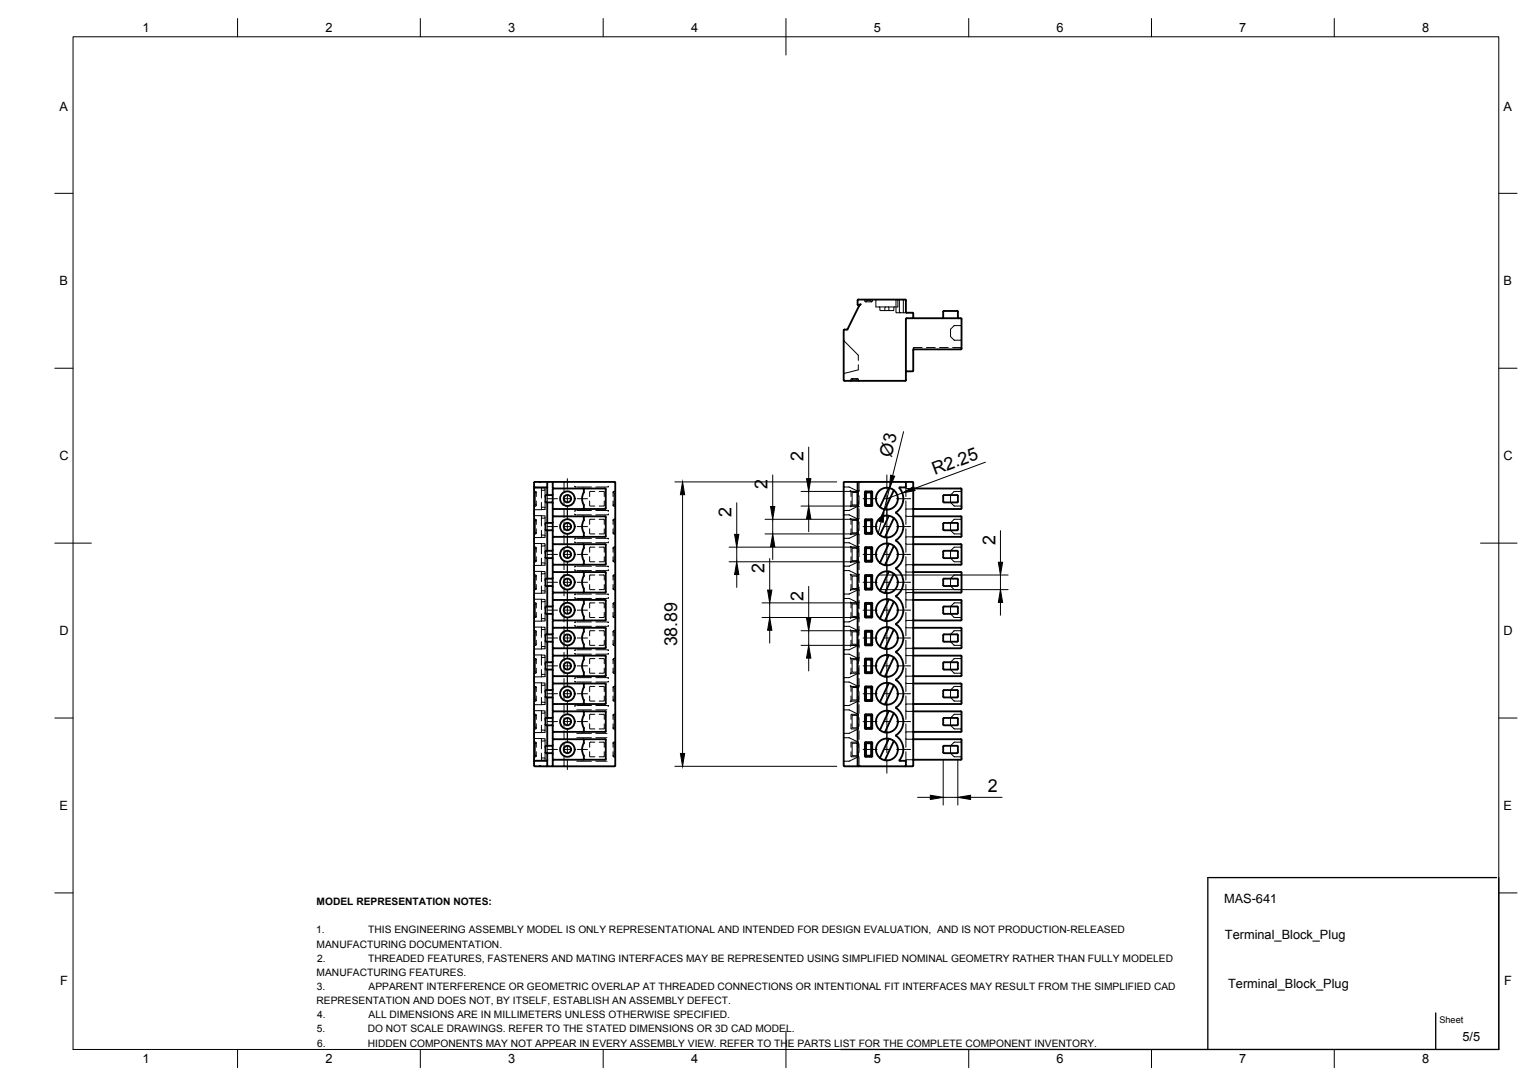
ISO-10303-21;
HEADER;
FILE_DESCRIPTION((''),'2;1');
FILE_NAME('Terminal_Block_Plug.step','2026-10-09T09:55:32-07:00',(''),(''),'','','');
FILE_SCHEMA (('AUTOMOTIVE_DESIGN { 1 0 10303 214 3 1 1 }'));
ENDSEC;
DATA;
#10=MECHANICAL_DESIGN_GEOMETRIC_PRESENTATION_REPRESENTATION('',(#83011,#83012,#83013,#83014,#83015,#83016,#83017,#83018,#83019,#83020,#83021,#83022,#83023,#83024,#83025,#83026,#83027,#83028,#83029,#83030,#83031,#83032,#83033,#83034,#83035,#83036,#83037,#83038,#83039,#83040,#83041,#83042,#83043,#83044,#83045,#83046,#83047,#83048,#83049,#83050,#83051,#83052,#83053,#83054,#83055,#83056,#83057,#83058,#83059,#83060,#83061,#83062,#83063,#83064,#83065,#83066,#83067,#83068,#83069,#83070,#83071,#83072,#83073,#83074,#83075,#83076,#83077,#83078,#83079,#83080,#83081,#83082,#83083,#83084,#83085,#83086,#83087,#83088,#83089,#83090,#83091,#83092,#83093,#83094,#83095,#83096,#83097,#83098,#83099,#83100,#83101,#83102,#83103,#83104,#83105,#83106,#83107,#83108,#83109,#83110,#83111,#83112,#83113,#83114,#83115,#83116,#83117,#83118,#83119,#83120,#83121,#83122,#83123,#83124,#83125,#83126,#83127,#83128,#83129,#83130,#83131,#83132,#83133,#83134,#83135,#83136,#83137,#83138,#83139,#83140,#83141,#83142,#83143,#83144,#83145,#83146,#83147,#83148,#83149,#83150,#83151,#83152,#83153,#83154,#83155,#83156,#83157,#83158,#83159,#83160,#83161,#83162,#83163,#83164,#83165,#83166,#83167,#83168,#83169,#83170,#83171,#83172,#83173,#83174,#83175,#83176,#83177,#83178,#83179,#83180,#83181,#83182,#83183,#83184,#83185,#83186,#83187,#83188,#83189,#83190,#83191,#83192,#83193,#83194,#83195,#83196,#83197,#83198,#83199,#83200,#83201,#83202,#83203,#83204,#83205,#83206,#83207,#83208,#83209,#83210,#83211,#83212,#83213,#83214,#83215,#83216,#83217,#83218,#83219,#83220,#83221,#83222,#83223,#83224,#83225,#83226,#83227,#83228,#83229,#83230,#83231,#83232,#83233,#83234,#83235,#83236,#83237,#83238,#83239,#83240,#83241,#83242,#83243,#83244,#83245,#83246,#83247,#83248,#83249,#83250,#83251,#83252,#83253,#83254,#83255,#83256,#83257,#83258,#83259,#83260,#83261,#83262,#83263,#83264,#83265,#83266,#83267,#83268,#83269,#83270,#83271,#83272,#83273,#83274,#83275,#83276,#83277,#83278,#83279,#83280,#83281,#83282,#83283,#83284,#83285,#83286,#83287,#83288,#83289,#83290,#83291,#83292,#83293,#83294,#83295,#83296,#83297,#83298,#83299,#83300,#83301,#83302,#83303,#83304,#83305,#83306,#83307,#83308,#83309,#83310,#83311,#83312,#83313,#83314,#83315,#83316,#83317,#83318,#83319,#83320,#83321,#83322,#83323,#83324,#83325,#83326,#83327,#83328,#83329,#83330,#83331,#83332,#83333,#83334,#83335,#83336,#83337,#83338,#83339,#83340,#83341,#83342,#83343,#83344,#83345,#83346,#83347,#83348,#83349,#83350,#83351,#83352,#83353,#83354,#83355,#83356,#83357,#83358,#83359,#83360,#83361,#83362,#83363,#83364,#83365,#83366,#83367,#83368,#83369,#83370,#83371,#83372,#83373,#83374,#83375,#83376,#83377,#83378,#83379,#83380,#83381,#83382,#83383,#83384,#83385,#83386,#83387,#83388,#83389,#83390,#83391,#83392,#83393,#83394,#83395,#83396,#83397,#83398,#83399,#83400,#83401,#83402,#83403,#83404,#83405,#83406,#83407,#83408,#83409,#83410,#83411,#83412,#83413,#83414,#83415,#83416,#83417,#83418,#83419,#83420,#83421,#83422,#83423,#83424,#83425,#83426,#83427,#83428,#83429,#83430,#83431,#83432,#83433,#83434,#83435,#83436,#83437,#83438,#83439,#83440,#83441,#83442,#83443,#83444,#83445,#83446,#83447,#83448,#83449,#83450,#83451,#83452,#83453,#83454,#83455,#83456,#83457,#83458,#83459,#83460,#83461,#83462,#83463,#83464,#83465,#83466,#83467,#83468,#83469,#83470,#83471,#83472,#83473,#83474,#83475,#83476,#83477,#83478,#83479,#83480,#83481,#83482,#83483,#83484,#83485,#83486,#83487,#83488,#83489,#83490,#83491,#83492,#83493,#83494,#83495,#83496,#83497,#83498,#83499,#83500,#83501,#83502,#83503,#83504,#83505,#83506,#83507,#83508,#83509,#83510,#83511,#83512,#83513,#83514,#83515,#83516,#83517,#83518,#83519,#83520,#83521,#83522,#83523,#83524,#83525,#83526,#83527,#83528,#83529,#83530,#83531,#83532,#83533,#83534,#83535,#83536,#83537,#83538,#83539,#83540,#83541,#83542,#83543,#83544,#83545,#83546,#83547,#83548,#83549,#83550,#83551,#83552,#83553,#83554,#83555,#83556,#83557,#83558,#83559,#83560,#83561,#83562,#83563,#83564,#83565,#83566,#83567,#83568,#83569,#83570,#83571,#83572,#83573,#83574,#83575,#83576,#83577,#83578,#83579,#83580,#83581,#83582,#83583,#83584,#83585,#83586,#83587,#83588,#83589,#83590,#83591,#83592,#83593,#83594,#83595,#83596,#83597,#83598,#83599,#83600,#83601,#83602,#83603,#83604,#83605,#83606,#83607,#83608,#83609,#83610,#83611,#83612,#83613,#83614,#83615,#83616,#83617,#83618,#83619,#83620,#83621,#83622,#83623,#83624,#83625,#83626,#83627,#83628,#83629,#83630,#83631,#83632,#83633,#83634,#83635,#83636,#83637,#83638,#83639,#83640,#83641,#83642,#83643,#83644,#83645,#83646,#83647,#83648,#83649,#83650,#83651,#83652,#83653,#83654,#83655,#83656,#83657,#83658,#83659,#83660,#83661,#83662,#83663,#83664,#83665,#83666,#83667,#83668,#83669,#83670,#83671,#83672,#83673,#83674,#83675,#83676,#83677,#83678,#83679,#83680,#83681,#83682,#83683,#83684,#83685,#83686,#83687,#83688,#83689,#83690,#83691,#83692,#83693,#83694,#83695,#83696,#83697,#83698,#83699,#83700,#83701,#83702,#83703,#83704,#83705,#83706,#83707,#83708,#83709,#83710,#83711,#83712,#83713,#83714,#83715,#83716,#83717,#83718,#83719,#83720,#83721,#83722,#83723,#83724,#83725,#83726,#83727,#83728,#83729,#83730,#83731,#83732,#83733,#83734,#83735,#83736,#83737,#83738,#83739,#83740,#83741,#83742,#83743,#83744,#83745,#83746,#83747,#83748,#83749,#83750,#83751,#83752,#83753,#83754,#83755,#83756,#83757,#83758,#83759,#83760,#83761,#83762,#83763,#83764,#83765,#83766,#83767,#83768,#83769,#83770,#83771,#83772,#83773,#83774,#83775,#83776,#83777,#83778,#83779,#83780,#83781,#83782,#83783,#83784,#83785,#83786,#83787,#83788,#83789,#83790,#83791,#83792,#83793,#83794,#83795,#83796,#83797,#83798,#83799,#83800,#83801,#83802,#83803,#83804,#83805,#83806,#83807,#83808,#83809,#83810,#83811,#83812,#83813,#83814,#83815,#83816,#83817,#83818,#83819,#83820,#83821,#83822,#83823,#83824,#83825,#83826,#83827,#83828,#83829,#83830,#83831,#83832,#83833,#83834,#83835,#83836,#83837,#83838,#83839,#83840,#83841,#83842,#83843,#83844,#83845,#83846,#83847,#83848,#83849,#83850,#83851,#83852,#83853,#83854,#83855,#83856,#83857,#83858,#83859,#83860,#83861,#83862,#83863,#83864,#83865,#83866,#83867,#83868,#83869,#83870,#83871,#83872,#83873,#83874,#83875,#83876,#83877,#83878,#83879,#83880,#83881,#83882,#83883,#83884,#83885,#83886,#83887,#83888,#83889,#83890,#83891,#83892,#83893,#83894,#83895,#83896,#83897,#83898,#83899,#83900,#83901,#83902,#83903,#83904,#83905,#83906,#83907,#83908,#83909,#83910,#83911,#83912,#83913,#83914,#83915,#83916,#83917,#83918,#83919,#83920,#83921,#83922,#83923,#83924,#83925,#83926,#83927,#83928,#83929,#83930,#83931,#83932,#83933,#83934,#83935,#83936,#83937,#83938,#83939,#83940,#83941,#83942,#83943,#83944,#83945,#83946,#83947,#83948,#83949,#83950,#83951,#83952,#83953,#83954,#83955,#83956,#83957,#83958,#83959,#83960,#83961,#83962,#83963,#83964,#83965,#83966,#83967,#83968,#83969,#83970,#83971,#83972,#83973,#83974,#83975,#83976,#83977,#83978,#83979,#83980,#83981,#83982,#83983,#83984,#83985,#83986,#83987,#83988,#83989,#83990,#83991,#83992,#83993,#83994,#83995,#83996,#83997,#83998,#83999,#84000,#84001,#84002,#84003,#84004,#84005,#84006,#84007,#84008,#84009,#84010,#84011,#84012,#84013,#84014,#84015,#84016,#84017,#84018,#84019,#84020,#84021,#84022,#84023,#84024,#84025,#84026,#84027,#84028,#84029,#84030,#84031,#84032,#84033,#84034,#84035,#84036,#84037,#84038,#84039,#84040,#84041,#84042,#84043,#84044,#84045,#84046,#84047,#84048,#84049,#84050,#84051,#84052,#84053,#84054,#84055,#84056,#84057,#84058,#84059,#84060,#84061,#84062,#84063,#84064,#84065,#84066,#84067,#84068,#84069,#84070,#84071,#84072,#84073,#84074,#84075,#84076,#84077,#84078,#84079,#84080,#84081,#84082,#84083,#84084,#84085,#84086,#84087,#84088,#84089,#84090,#84091,#84092,#84093,#84094,#84095,#84096,#84097,#84098,#84099,#84100,#84101,#84102,#84103,#84104,#84105,#84106,#84107,#84108,#84109,#84110,#84111,#84112,#84113,#84114,#84115,#84116,#84117,#84118,#84119,#84120,#84121,#84122,#84123,#84124,#84125,#84126,#84127,#84128,#84129,#84130,#84131,#84132,#84133,#84134,#84135,#84136,#84137,#84138,#84139,#84140,#84141,#84142,#84143,#84144,#84145,#84146,#84147,#84148,#84149,#84150,#84151,#84152,#84153,#84154,#84155,#84156,#84157,#84158,#84159,#84160,#84161,#84162,#84163,#84164,#84165,#84166,#84167,#84168,#84169,#84170,#84171,#84172,#84173,#84174,#84175,#84176,#84177,#84178,#84179,#84180,#84181,#84182,#84183,#84184,#84185,#84186,#84187,#84188,#84189,#84190,#84191,#84192,#84193,#84194,#84195,#84196,#84197,#84198,#84199,#84200,#84201,#84202,#84203,#84204,#84205,#84206,#84207,#84208,#84209,#84210,#84211,#84212,#84213,#84214,#84215,#84216,#84217,#84218,#84219,#84220,#84221,#84222,#84223,#84224,#84225,#84226,#84227,#84228,#84229,#84230,#84231,#84232,#84233,#84234,#84235,#84236,#84237,#84238,#84239,#84240,#84241,#84242,#84243,#84244,#84245,#84246,#84247,#84248,#84249,#84250,#84251,#84252,#84253,#84254,#84255,#84256,#84257,#84258,#84259,#84260,#84261,#84262,#84263,#84264,#84265,#84266,#84267,#84268,#84269,#84270,#84271,#84272,#84273,#84274,#84275,#84276,#84277,#84278,#84279,#84280,#84281,#84282,#84283,#84284,#84285,#84286,#84287,#84288,#84289,#84290,#84291,#84292,#84293,#84294,#84295,#84296,#84297,#84298,#84299,#84300,#84301,#84302,#84303,#84304,#84305,#84306,#84307,#84308,#84309,#84310,#84311,#84312,#84313,#84314,#84315,#84316,#84317,#84318,#84319,#84320,#84321,#84322,#84323,#84324,#84325,#84326,#84327,#84328,#84329,#84330,#84331,#84332,#84333,#84334,#84335,#84336,#84337,#84338,#84339,#84340,#84341,#84342,#84343,#84344,#84345,#84346,#84347,#84348,#84349,#84350,#84351,#84352,#84353,#84354,#84355,#84356,#84357,#84358,#84359,#84360,#84361,#84362,#84363,#84364,#84365,#84366,#84367,#84368,#84369,#84370,#84371,#84372,#84373,#84374,#84375,#84376,#84377,#84378,#84379,#84380,#84381,#84382,#84383,#84384,#84385,#84386,#84387,#84388,#84389,#84390,#84391,#84392,#84393,#84394,#84395,#84396,#84397,#84398,#84399,#84400,#84401,#84402,#84403,#84404,#84405,#84406,#84407,#84408,#84409,#84410,#84411,#84412,#84413,#84414,#84415,#84416,#84417,#84418,#84419,#84420,#84421,#84422,#84423,#84424,#84425,#84426,#84427,#84428,#84429,#84430,#84431,#84432,#84433,#84434,#84435,#84436,#84437,#84438,#84439,#84440,#84441,#84442,#84443,#84444,#84445,#84446,#84447,#84448,#84449,#84450,#84451,#84452,#84453,#84454,#84455,#84456,#84457,#84458,#84459,#84460,#84461,#84462,#84463,#84464,#84465,#84466,#84467,#84468,#84469,#84470,#84471,#84472,#84473,#84474,#84475,#84476,#84477,#84478,#84479,#84480,#84481,#84482,#84483,#84484,#84485,#84486,#84487,#84488,#84489,#84490,#84491,#84492,#84493,#84494,#84495,#84496,#84497,#84498,#84499,#84500,#84501,#84502,#84503,#84504,#84505,#84506,#84507,#84508,#84509,#84510,#84511,#84512,#84513,#84514,#84515,#84516,#84517,#84518,#84519,#84520,#84521,#84522,#84523,#84524,#84525,#84526,#84527,#84528,#84529,#84530,#84531,#84532,#84533,#84534,#84535,#84536,#84537,#84538,#84539,#84540,#84541,#84542,#84543,#84544,#84545,#84546,#84547,#84548,#84549,#84550,#84551,#84552,#84553,#84554,#84555,#84556,#84557,#84558,#84559,#84560,#84561,#84562,#84563,#84564,#84565,#84566,#84567,#84568,#84569,#84570,#84571,#84572,#84573,#84574,#84575,#84576,#84577,#84578,#84579,#84580,#84581,#84582,#84583,#84584,#84585,#84586,#84587,#84588,#84589,#84590,#84591,#84592,#84593,#84594,#84595,#84596,#84597,#84598,#84599,#84600,#84601,#84602,#84603,#84604,#84605,#84606,#84607,#84608,#84609,#84610,#84611,#84612,#84613,#84614,#84615,#84616,#84617,#84618,#84619,#84620,#84621,#84622,#84623,#84624,#84625,#84626,#84627,#84628,#84629,#84630,#84631,#84632,#84633,#84634,#84635,#84636,#84637,#84638,#84639,#84640,#84641,#84642,#84643,#84644,#84645,#84646,#84647,#84648,#84649,#84650,#84651,#84652,#84653,#84654,#84655,#84656,#84657,#84658,#84659,#84660,#84661,#84662,#84663,#84664,#84665,#84666,#84667,#84668,#84669,#84670,#84671,#84672,#84673,#84674,#84675,#84676,#84677,#84678,#84679,#84680,#84681,#84682,#84683,#84684,#84685,#84686,#84687,#84688,#84689,#84690,#84691,#84692,#84693,#84694,#84695,#84696,#84697,#84698,#84699,#84700,#84701,#84702,#84703,#84704,#84705,#84706,#84707,#84708,#84709,#84710,#84711,#84712,#84713,#84714,#84715,#84716,#84717,#84718,#84719,#84720,#84721,#84722,#84723,#84724,#84725,#84726,#84727,#84728,#84729,#84730,#84731,#84732,#84733,#84734,#84735,#84736,#84737,#84738,#84739,#84740,#84741,#84742,#84743,#84744,#84745,#84746,#84747,#84748,#84749,#84750,#84751,#84752,#84753,#84754,#84755,#84756,#84757,#84758,#84759,#84760,#84761,#84762,#84763,#84764,#84765,#84766,#84767,#84768,#84769,#84770,#84771,#84772,#84773,#84774,#84775,#84776,#84777,#84778,#84779,#84780,#84781,#84782,#84783,#84784,#84785,#84786,#84787,#84788,#84789,#84790,#84791,#84792,#84793,#84794,#84795,#84796,#84797,#84798,#84799,#84800,#84801,#84802,#84803,#84804,#84805,#84806,#84807,#84808,#84809,#84810,#84811,#84812,#84813,#84814,#84815,#84816,#84817,#84818,#84819,#84820,#84821,#84822,#84823,#84824,#84825,#84826,#84827,#84828,#84829,#84830,#84831,#84832,#84833,#84834,#84835,#84836,#84837,#84838,#84839,#84840,#84841,#84842,#84843,#84844,#84845,#84846,#84847,#84848,#84849,#84850,#84851,#84852,#84853,#84854,#84855,#84856,#84857,#84858,#84859,#84860,#84861,#84862,#84863,#84864,#84865,#84866,#84867,#84868,#84869,#84870,#84871,#84872,#84873,#84874,#84875,#84876,#84877,#84878,#84879,#84880,#84881,#84882,#84883,#84884,#84885,#84886,#84887,#84888,#84889,#84890,#84891,#84892,#84893,#84894,#84895,#84896,#84897,#84898,#84899,#84900,#84901,#84902,#84903,#84904,#84905,#84906,#84907,#84908,#84909,#84910,#84911,#84912,#84913,#84914,#84915,#84916,#84917,#84918,#84919,#84920,#84921,#84922,#84923,#84924,#84925,#84926,#84927,#84928,#84929,#84930,#84931,#84932,#84933,#84934,#84935,#84936,#84937,#84938,#84939,#84940,#84941,#84942,#84943,#84944,#84945,#84946,#84947,#84948,#84949,#84950,#84951,#84952,#84953,#84954,#84955,#84956,#84957,#84958,#84959,#84960,#84961,#84962,#84963,#84964,#84965,#84966,#84967,#84968,#84969,#84970,#84971,#84972,#84973,#84974,#84975,#84976,#84977,#84978,#84979,#84980,#84981,#84982,#84983,#84984,#84985,#84986,#84987,#84988,#84989,#84990,#84991,#84992,#84993,#84994,#84995,#84996,#84997,#84998,#84999,#85000,#85001,#85002,#85003,#85004,#85005,#85006,#85007,#85008,#85009,#85010,#85011,#85012,#85013,#85014,#85015,#85016,#85017,#85018,#85019,#85020,#85021,#85022,#85023,#85024,#85025,#85026,#85027,#85028,#85029,#85030,#85031,#85032,#85033,#85034,#85035,#85036,#85037,#85038,#85039,#85040,#85041,#85042,#85043,#85044,#85045,#85046,#85047,#85048,#85049,#85050,#85051,#85052,#85053,#85054,#85055,#85056,#85057,#85058,#85059,#85060,#85061,#85062,#85063,#85064,#85065,#85066,#85067,#85068,#85069,#85070,#85071,#85072,#85073,#85074,#85075,#85076,#85077,#85078,#85079,#85080,#85081,#85082,#85083,#85084,#85085,#85086,#85087,#85088,#85089,#85090,#85091,#85092,#85093,#85094,#85095,#85096,#85097,#85098,#85099,#85100,#85101,#85102,#85103,#85104,#85105,#85106,#85107,#85108,#85109,#85110,#85111,#85112,#85113,#85114,#85115,#85116,#85117,#85118,#85119,#85120,#85121,#85122,#85123,#85124,#85125,#85126,#85127,#85128,#85129,#85130,#85131,#85132,#85133,#85134,#85135,#85136,#85137,#85138,#85139,#85140,#85141,#85142,#85143,#85144,#85145,#85146,#85147,#85148,#85149,#85150,#85151,#85152,#85153,#85154,#85155,#85156,#85157,#85158,#85159,#85160,#85161,#85162,#85163,#85164,#85165,#85166,#85167,#85168,#85169,#85170,#85171,#85172,#85173,#85174,#85175,#85176,#85177,#85178,#85179,#85180,#85181,#85182,#85183,#85184,#85185,#85186,#85187,#85188,#85189,#85190,#85191,#85192,#85193,#85194,#85195,#85196,#85197,#85198,#85199,#85200,#85201,#85202,#85203,#85204,#85205,#85206,#85207,#85208,#85209,#85210,#85211,#85212,#85213,#85214,#85215,#85216,#85217,#85218,#85219,#85220,#85221,#85222,#85223,#85224,#85225,#85226,#85227,#85228,#85229,#85230,#85231,#85232,#85233,#85234,#85235,#85236,#85237,#85238,#85239,#85240,#85241,#85242,#85243,#85244,#85245,#85246,#85247,#85248,#85249,#85250,#85251,#85252,#85253,#85254,#85255,#85256,#85257,#85258,#85259,#85260,#85261,#85262,#85263,#85264,#85265,#85266,#85267,#85268,#85269,#85270,#85271,#85272,#85273,#85274,#85275,#85276,#85277,#85278,#85279,#85280,#85281,#85282,#85283,#85284,#85285,#85286,#85287,#85288,#85289,#85290,#85291,#85292,#85293,#85294,#85295,#85296,#85297,#85298,#85299,#85300,#85301,#85302,#85303,#85304,#85305,#85306,#85307,#85308,#85309,#85310,#85311,#85312,#85313,#85314,#85315,#85316,#85317,#85318,#85319,#85320,#85321,#85322,#85323,#85324,#85325,#85326,#85327,#85328,#85329,#85330,#85331,#85332,#85333,#85334,#85335,#85336,#85337,#85338,#85339,#85340,#85341,#85342,#85343,#85344,#85345,#85346,#85347,#85348,#85349,#85350,#85351,#85352,#85353,#85354,#85355,#85356,#85357,#85358,#85359,#85360,#85361,#85362,#85363,#85364,#85365,#85366),#170127);
#25=SHAPE_REPRESENTATION_RELATIONSHIP('SRR','None',#170146,#28) ;
#28=ADVANCED_BREP_SHAPE_REPRESENTATION('',(#33),#170126) ;
#33=MANIFOLD_SOLID_BREP('Body1',#91087) ;
#128=(
BOUNDED_SURFACE()
B_SPLINE_SURFACE(3,2,((#157489,#157490,#157491),(#157492,#157493,#157494),
(#157495,#157496,#157497),(#157498,#157499,#157500),(#157501,#157502,#157503),
(#157504,#157505,#157506)),.UNSPECIFIED.,.F.,.F.,.F.)
B_SPLINE_SURFACE_WITH_KNOTS((4,2,4),(3,3),(0.,0.785398163397448,1.5707963267949),
(0.,1.),.UNSPECIFIED.)
GEOMETRIC_REPRESENTATION_ITEM()
RATIONAL_B_SPLINE_SURFACE(((1.,0.923879532511288,1.),(1.,0.924029717224457,
1.),(1.,0.903812846803813,1.),(1.,0.828237960765067,1.),(1.,0.772793297349054,
1.),(1.,0.707106781186551,1.)))
REPRESENTATION_ITEM('')
SURFACE()
) ;
#129=(
BOUNDED_SURFACE()
B_SPLINE_SURFACE(3,2,((#157529,#157530,#157531),(#157532,#157533,#157534),
(#157535,#157536,#157537),(#157538,#157539,#157540),(#157541,#157542,#157543),
(#157544,#157545,#157546)),.UNSPECIFIED.,.F.,.F.,.F.)
B_SPLINE_SURFACE_WITH_KNOTS((4,2,4),(3,3),(1.5707963267949,2.35619449019234,
3.14159265358979),(0.,1.),.UNSPECIFIED.)
GEOMETRIC_REPRESENTATION_ITEM()
RATIONAL_B_SPLINE_SURFACE(((1.,0.707106781186551,1.),(1.,0.772793297349013,
1.),(1.,0.828237960765125,1.),(1.,0.903812846803755,1.),(1.,0.924029717224501,
1.),(1.,0.923879532511288,1.)))
REPRESENTATION_ITEM('')
SURFACE()
) ;
#130=(
BOUNDED_SURFACE()
B_SPLINE_SURFACE(3,2,((#157548,#157549,#157550),(#157551,#157552,#157553),
(#157554,#157555,#157556),(#157557,#157558,#157559),(#157560,#157561,#157562),
(#157563,#157564,#157565)),.UNSPECIFIED.,.F.,.F.,.F.)
B_SPLINE_SURFACE_WITH_KNOTS((4,2,4),(3,3),(4.71185725581867,5.49778714378214,
6.2837170317456),(0.,1.00053172456602),.UNSPECIFIED.)
GEOMETRIC_REPRESENTATION_ITEM()
RATIONAL_B_SPLINE_SURFACE(((1.,0.70690521752879,1.00031169139202),(1.,0.729483947708843,
1.00028768006101),(1.,0.750534083362416,1.00026529431252),(1.,0.779901566764209,
1.00023406348779),(1.,0.788212408697306,1.00022522533015),(1.,0.788092590029068,
1.00022535275121)))
REPRESENTATION_ITEM('')
SURFACE()
) ;
#131=(
BOUNDED_SURFACE()
B_SPLINE_SURFACE(3,2,((#157577,#157578,#157579),(#157580,#157581,#157582),
(#157583,#157584,#157585),(#157586,#157587,#157588),(#157589,#157590,#157591),
(#157592,#157593,#157594)),.UNSPECIFIED.,.F.,.F.,.F.)
B_SPLINE_SURFACE_WITH_KNOTS((4,2,4),(3,3),(3.14106092902388,3.92699081698724,
4.71292070495061),(0.,1.00053172456592),.UNSPECIFIED.)
GEOMETRIC_REPRESENTATION_ITEM()
RATIONAL_B_SPLINE_SURFACE(((1.,0.788092590029089,1.00022535275116),(1.,
0.788212408697304,1.0002252253301),(1.,0.77990156676426,1.00023406348774),
(1.,0.750534083362408,1.00026529431247),(1.,0.729483947708901,1.00028768006096),
(1.,0.706905217528829,1.00031169139196)))
REPRESENTATION_ITEM('')
SURFACE()
) ;
#132=(
BOUNDED_SURFACE()
B_SPLINE_SURFACE(3,2,((#157852,#157853,#157854),(#157855,#157856,#157857),
(#157858,#157859,#157860),(#157861,#157862,#157863),(#157864,#157865,#157866),
(#157867,#157868,#157869),(#157870,#157871,#157872),(#157873,#157874,#157875),
(#157876,#157877,#157878),(#157879,#157880,#157881)),.UNSPECIFIED.,.F.,
 .F.,.F.)
B_SPLINE_SURFACE_WITH_KNOTS((4,2,2,2,4),(3,3),(-3.3881317890172E-21,5.50005871024832E-5,
0.000110001174204966,0.000165001761307449,0.000220002348409933),(-9.32574651155486E-5,
1.),.UNSPECIFIED.)
GEOMETRIC_REPRESENTATION_ITEM()
RATIONAL_B_SPLINE_SURFACE(((1.00005463405283,0.707079466707411,1.),(1.00005694771662,
0.694674755787634,1.),(1.00005645688428,0.697306353922579,1.),(1.00005591567353,
0.70020805593976,1.),(1.0000556235962,0.701774028840071,1.),(1.00005562454822,
0.701768924610627,1.),(1.00005591789343,0.700196153956614,1.),(1.00005645795057,
0.697300636998118,1.),(1.00005694973354,0.694663942070733,1.),(1.00005463405283,
0.707079466707407,1.)))
REPRESENTATION_ITEM('')
SURFACE()
) ;
#133=(
BOUNDED_SURFACE()
B_SPLINE_SURFACE(3,2,((#157886,#157887,#157888),(#157889,#157890,#157891),
(#157892,#157893,#157894),(#157895,#157896,#157897),(#157898,#157899,#157900),
(#157901,#157902,#157903),(#157904,#157905,#157906),(#157907,#157908,#157909),
(#157910,#157911,#157912),(#157913,#157914,#157915)),.UNSPECIFIED.,.F.,
 .F.,.F.)
B_SPLINE_SURFACE_WITH_KNOTS((4,2,2,2,4),(3,3),(-1.89735380184963E-19,5.50005871024829E-5,
0.000110001174204966,0.000165001761307449,0.000220002348409932),(0.,1.00009325746512),
 .UNSPECIFIED.)
GEOMETRIC_REPRESENTATION_ITEM()
RATIONAL_B_SPLINE_SURFACE(((1.,0.707079466707407,1.00005463405283),(1.,
0.69467475578763,1.00005694771662),(1.,0.697306353922582,1.00005645688428),
(1.,0.700208055939751,1.00005591567353),(1.,0.701774028840056,1.0000556235962),
(1.,0.701768924610644,1.00005562454822),(1.,0.700196153956613,1.00005591789343),
(1.,0.697300636998124,1.00005645795057),(1.,0.694663942070735,1.00005694973354),
(1.,0.70707946670741,1.00005463405283)))
REPRESENTATION_ITEM('')
SURFACE()
) ;
#134=(
BOUNDED_SURFACE()
B_SPLINE_SURFACE(3,2,((#163040,#163041,#163042),(#163043,#163044,#163045),
(#163046,#163047,#163048),(#163049,#163050,#163051),(#163052,#163053,#163054),
(#163055,#163056,#163057)),.UNSPECIFIED.,.F.,.F.,.F.)
B_SPLINE_SURFACE_WITH_KNOTS((4,2,4),(3,3),(0.,0.785398163397448,1.5707963267949),
(0.,1.),.UNSPECIFIED.)
GEOMETRIC_REPRESENTATION_ITEM()
RATIONAL_B_SPLINE_SURFACE(((1.,0.923879532511288,1.),(1.,0.924029717224521,
1.),(1.,0.903812846803727,1.),(1.,0.828237960765152,1.),(1.,0.772793297348994,
1.),(1.,0.707106781186548,1.)))
REPRESENTATION_ITEM('')
SURFACE()
) ;
#135=(
BOUNDED_SURFACE()
B_SPLINE_SURFACE(3,2,((#163080,#163081,#163082),(#163083,#163084,#163085),
(#163086,#163087,#163088),(#163089,#163090,#163091),(#163092,#163093,#163094),
(#163095,#163096,#163097)),.UNSPECIFIED.,.F.,.F.,.F.)
B_SPLINE_SURFACE_WITH_KNOTS((4,2,4),(3,3),(1.5707963267949,2.35619449019234,
3.14159265358979),(0.,1.),.UNSPECIFIED.)
GEOMETRIC_REPRESENTATION_ITEM()
RATIONAL_B_SPLINE_SURFACE(((1.,0.707106781186551,1.),(1.,0.772793297348998,
1.),(1.,0.828237960765139,1.),(1.,0.90381284680374,1.),(1.,0.924029717224511,
1.),(1.,0.923879532511288,1.)))
REPRESENTATION_ITEM('')
SURFACE()
) ;
#136=(
BOUNDED_SURFACE()
B_SPLINE_SURFACE(3,2,((#163099,#163100,#163101),(#163102,#163103,#163104),
(#163105,#163106,#163107),(#163108,#163109,#163110),(#163111,#163112,#163113),
(#163114,#163115,#163116)),.UNSPECIFIED.,.F.,.F.,.F.)
B_SPLINE_SURFACE_WITH_KNOTS((4,2,4),(3,3),(4.71185725581866,5.49778714378214,
6.28371703174562),(0.,1.00053172456603),.UNSPECIFIED.)
GEOMETRIC_REPRESENTATION_ITEM()
RATIONAL_B_SPLINE_SURFACE(((1.,0.706905217528784,1.00031169139203),(1.,
0.729483947708883,1.00028768006102),(1.,0.750534083362363,1.00026529431253),
(1.,0.779901566764257,1.00023406348779),(1.,0.788212408697267,1.00022522533015),
(1.,0.788092590029066,1.00022535275121)))
REPRESENTATION_ITEM('')
SURFACE()
) ;
#137=(
BOUNDED_SURFACE()
B_SPLINE_SURFACE(3,2,((#163128,#163129,#163130),(#163131,#163132,#163133),
(#163134,#163135,#163136),(#163137,#163138,#163139),(#163140,#163141,#163142),
(#163143,#163144,#163145)),.UNSPECIFIED.,.F.,.F.,.F.)
B_SPLINE_SURFACE_WITH_KNOTS((4,2,4),(3,3),(3.14106092902389,3.92699081698724,
4.71292070495059),(0.,1.0005317245659),.UNSPECIFIED.)
GEOMETRIC_REPRESENTATION_ITEM()
RATIONAL_B_SPLINE_SURFACE(((1.,0.788092590029092,1.00022535275116),(1.,
0.788212408697299,1.0002252253301),(1.,0.779901566764274,1.00023406348774),
(1.,0.7505340833624,1.00026529431246),(1.,0.729483947708915,1.00028768006095),
(1.,0.706905217528834,1.00031169139195)))
REPRESENTATION_ITEM('')
SURFACE()
) ;
#138=(
BOUNDED_SURFACE()
B_SPLINE_SURFACE(3,2,((#163546,#163547,#163548),(#163549,#163550,#163551),
(#163552,#163553,#163554),(#163555,#163556,#163557),(#163558,#163559,#163560),
(#163561,#163562,#163563),(#163564,#163565,#163566),(#163567,#163568,#163569)),
 .UNSPECIFIED.,.F.,.F.,.F.)
B_SPLINE_SURFACE_WITH_KNOTS((4,2,2,4),(3,3),(1.5707963267949,2.35619449019234,
2.74889357189107,3.14159265358979),(0.,1.),.UNSPECIFIED.)
GEOMETRIC_REPRESENTATION_ITEM()
RATIONAL_B_SPLINE_SURFACE(((1.,1.,1.),(1.,1.00267605951749,1.),(1.,0.941599607549753,
1.),(1.,0.828238301901781,1.),(1.,0.787677905717216,1.),(1.,0.726552333979994,
1.),(1.,0.706675310150435,1.),(1.,0.707106781186544,1.)))
REPRESENTATION_ITEM('')
SURFACE()
) ;
#139=(
BOUNDED_SURFACE()
B_SPLINE_SURFACE(3,2,((#163573,#163574,#163575),(#163576,#163577,#163578),
(#163579,#163580,#163581),(#163582,#163583,#163584),(#163585,#163586,#163587),
(#163588,#163589,#163590),(#163591,#163592,#163593),(#163594,#163595,#163596)),
 .UNSPECIFIED.,.F.,.F.,.F.)
B_SPLINE_SURFACE_WITH_KNOTS((4,2,2,4),(3,3),(4.71238898038469,5.49778714378214,
5.89048622548086,6.28318530717959),(0.,1.),.UNSPECIFIED.)
GEOMETRIC_REPRESENTATION_ITEM()
RATIONAL_B_SPLINE_SURFACE(((1.,1.,1.),(1.,1.00267605951751,1.),(1.,0.941599607549725,
1.),(1.,0.828238301901795,1.),(1.,0.787677905717217,1.),(1.,0.726552333979995,
1.),(1.,0.706675310150434,1.),(1.,0.707106781186544,1.)))
REPRESENTATION_ITEM('')
SURFACE()
) ;
#140=(
BOUNDED_SURFACE()
B_SPLINE_SURFACE(3,2,((#163601,#163602,#163603),(#163604,#163605,#163606),
(#163607,#163608,#163609),(#163610,#163611,#163612),(#163613,#163614,#163615),
(#163616,#163617,#163618),(#163619,#163620,#163621),(#163622,#163623,#163624)),
 .UNSPECIFIED.,.F.,.F.,.F.)
B_SPLINE_SURFACE_WITH_KNOTS((4,2,2,4),(3,3),(1.5707963267949,2.35619449019234,
2.74889357189107,3.14159265358979),(0.,1.),.UNSPECIFIED.)
GEOMETRIC_REPRESENTATION_ITEM()
RATIONAL_B_SPLINE_SURFACE(((1.,1.,1.),(1.,1.00267605951744,1.),(1.,0.941599607549824,
1.),(1.,0.828238301901746,1.),(1.,0.787677905717207,1.),(1.,0.726552333980003,
1.),(1.,0.706675310150422,1.),(1.,0.707106781186548,1.)))
REPRESENTATION_ITEM('')
SURFACE()
) ;
#141=(
BOUNDED_SURFACE()
B_SPLINE_SURFACE(3,2,((#163646,#163647,#163648),(#163649,#163650,#163651),
(#163652,#163653,#163654),(#163655,#163656,#163657),(#163658,#163659,#163660),
(#163661,#163662,#163663),(#163664,#163665,#163666),(#163667,#163668,#163669)),
 .UNSPECIFIED.,.F.,.F.,.F.)
B_SPLINE_SURFACE_WITH_KNOTS((4,2,2,4),(3,3),(4.71238898038469,5.49778714378214,
5.89048622548086,6.28318530717959),(0.,1.),.UNSPECIFIED.)
GEOMETRIC_REPRESENTATION_ITEM()
RATIONAL_B_SPLINE_SURFACE(((1.,1.,1.),(1.,1.00267605951747,1.),(1.,0.941599607549785,
1.),(1.,0.828238301901765,1.),(1.,0.787677905717207,1.),(1.,0.726552333980003,
1.),(1.,0.706675310150422,1.),(1.,0.707106781186548,1.)))
REPRESENTATION_ITEM('')
SURFACE()
) ;
#142=(
BOUNDED_SURFACE()
B_SPLINE_SURFACE(3,2,((#163670,#163671,#163672),(#163673,#163674,#163675),
(#163676,#163677,#163678),(#163679,#163680,#163681),(#163682,#163683,#163684),
(#163685,#163686,#163687),(#163688,#163689,#163690),(#163691,#163692,#163693)),
 .UNSPECIFIED.,.F.,.F.,.F.)
B_SPLINE_SURFACE_WITH_KNOTS((4,2,2,4),(3,3),(3.38657131671666,3.71802573263366,
4.04948014855067,4.71238898038469),(-0.000420825309489484,1.00042070189283),
 .UNSPECIFIED.)
GEOMETRIC_REPRESENTATION_ITEM()
RATIONAL_B_SPLINE_SURFACE(((1.00022935632051,0.727377552434629,1.00022928902823),
(1.00021435583198,0.74520775606903,1.00021429294078),(1.00019031910525,
0.773778807684193,1.00019026326634),(1.00013753195033,0.836523812238417,
1.00013749159897),(1.00010896375305,0.870481157936262,1.0001089317835),
(1.00003378452308,0.959842312830291,1.00003377461082),(0.999998875499962,
1.00133662744396,0.999998875829887),(1.,1.,1.)))
REPRESENTATION_ITEM('')
SURFACE()
) ;
#143=(
BOUNDED_SURFACE()
B_SPLINE_SURFACE(3,2,((#163695,#163696,#163697),(#163698,#163699,#163700),
(#163701,#163702,#163703),(#163704,#163705,#163706)),.UNSPECIFIED.,.F.,
 .F.,.F.)
B_SPLINE_SURFACE_WITH_KNOTS((4,4),(3,3),(1.32581766366803,1.5707963267949),
(0.,1.),.UNSPECIFIED.)
GEOMETRIC_REPRESENTATION_ITEM()
RATIONAL_B_SPLINE_SURFACE(((1.,0.727606875108995,1.),(1.,0.721005575721677,
1.),(1.,0.714109499479742,1.),(1.,0.707106781186548,1.)))
REPRESENTATION_ITEM('')
SURFACE()
) ;
#144=(
BOUNDED_SURFACE()
B_SPLINE_SURFACE(3,2,((#163722,#163723,#163724),(#163725,#163726,#163727),
(#163728,#163729,#163730),(#163731,#163732,#163733)),.UNSPECIFIED.,.F.,
 .F.,.F.)
B_SPLINE_SURFACE_WITH_KNOTS((4,4),(3,3),(3.92699081698724,4.71238898038469),
(0.,1.),.UNSPECIFIED.)
GEOMETRIC_REPRESENTATION_ITEM()
RATIONAL_B_SPLINE_SURFACE(((1.,0.866025403784441,1.),(1.,0.82836361504933,
1.),(1.,0.772698924407957,1.),(1.,0.707106781186548,1.)))
REPRESENTATION_ITEM('')
SURFACE()
) ;
#145=(
BOUNDED_SURFACE()
B_SPLINE_SURFACE(3,2,((#163735,#163736,#163737),(#163738,#163739,#163740),
(#163741,#163742,#163743),(#163744,#163745,#163746)),.UNSPECIFIED.,.F.,
 .F.,.F.)
B_SPLINE_SURFACE_WITH_KNOTS((4,4),(3,3),(1.5707963267949,2.35619449019234),
(0.,1.),.UNSPECIFIED.)
GEOMETRIC_REPRESENTATION_ITEM()
RATIONAL_B_SPLINE_SURFACE(((1.,1.,1.),(1.,1.00150544078213,1.),(1.,0.943158245625731,
1.),(1.,0.866025403784441,1.)))
REPRESENTATION_ITEM('')
SURFACE()
) ;
#146=(
BOUNDED_SURFACE()
B_SPLINE_SURFACE(3,2,((#163747,#163748,#163749),(#163750,#163751,#163752),
(#163753,#163754,#163755),(#163756,#163757,#163758)),.UNSPECIFIED.,.F.,
 .F.,.F.)
B_SPLINE_SURFACE_WITH_KNOTS((4,4),(3,3),(7.06858347057708,7.85398163397448),
(0.,1.),.UNSPECIFIED.)
GEOMETRIC_REPRESENTATION_ITEM()
RATIONAL_B_SPLINE_SURFACE(((1.,0.866025403784455,1.),(1.,0.943158245625741,
1.),(1.,1.00150544078213,1.),(1.,1.,1.)))
REPRESENTATION_ITEM('')
SURFACE()
) ;
#147=(
BOUNDED_SURFACE()
B_SPLINE_SURFACE(3,2,((#163760,#163761,#163762),(#163763,#163764,#163765),
(#163766,#163767,#163768),(#163769,#163770,#163771)),.UNSPECIFIED.,.F.,
 .F.,.F.)
B_SPLINE_SURFACE_WITH_KNOTS((4,4),(3,3),(1.5707963267949,2.35619449019239),
(0.,1.),.UNSPECIFIED.)
GEOMETRIC_REPRESENTATION_ITEM()
RATIONAL_B_SPLINE_SURFACE(((1.,0.707106781186545,1.),(1.,0.77269892440796,
1.),(1.,0.82836361504934,1.),(1.,0.866025403784447,1.)))
REPRESENTATION_ITEM('')
SURFACE()
) ;
#148=(
BOUNDED_SURFACE()
B_SPLINE_SURFACE(3,2,((#163787,#163788,#163789),(#163790,#163791,#163792),
(#163793,#163794,#163795),(#163796,#163797,#163798)),.UNSPECIFIED.,.F.,
 .F.,.F.)
B_SPLINE_SURFACE_WITH_KNOTS((4,4),(3,3),(4.71238898038469,4.95736764351155),
(0.,1.),.UNSPECIFIED.)
GEOMETRIC_REPRESENTATION_ITEM()
RATIONAL_B_SPLINE_SURFACE(((1.,0.707106781186548,1.),(1.,0.714109499479746,
1.),(1.,0.721005575721676,1.),(1.,0.727606875108995,1.)))
REPRESENTATION_ITEM('')
SURFACE()
) ;
#149=(
BOUNDED_SURFACE()
B_SPLINE_SURFACE(3,2,((#163800,#163801,#163802),(#163803,#163804,#163805),
(#163806,#163807,#163808),(#163809,#163810,#163811),(#163812,#163813,#163814),
(#163815,#163816,#163817),(#163818,#163819,#163820),(#163821,#163822,#163823)),
 .UNSPECIFIED.,.F.,.F.,.F.)
B_SPLINE_SURFACE_WITH_KNOTS((4,2,2,4),(3,3),(3.38657131671666,3.71802573263366,
4.04948014855067,4.71238898038469),(-0.000420825307952133,1.00042070189548),
 .UNSPECIFIED.)
GEOMETRIC_REPRESENTATION_ITEM()
RATIONAL_B_SPLINE_SURFACE(((1.00022935631968,0.727377552434324,1.00022928902968),
(1.0002143558312,0.745207756068745,1.00021429294214),(1.00019031910455,
0.77377880768394,1.00019026326754),(1.00013753194982,0.836523812238234,
1.00013749159984),(1.00010896375265,0.87048115793612,1.00010893178419),
(1.00003378452295,0.959842312830239,1.00003377461103),(0.999998875499966,
1.00133662744397,0.99999887582988),(1.,1.,1.)))
REPRESENTATION_ITEM('')
SURFACE()
) ;
#150=(
BOUNDED_SURFACE()
B_SPLINE_SURFACE(3,2,((#164038,#164039,#164040),(#164041,#164042,#164043),
(#164044,#164045,#164046),(#164047,#164048,#164049),(#164050,#164051,#164052),
(#164053,#164054,#164055),(#164056,#164057,#164058),(#164059,#164060,#164061)),
 .UNSPECIFIED.,.F.,.F.,.F.)
B_SPLINE_SURFACE_WITH_KNOTS((4,2,2,4),(3,3),(1.5707963267949,2.35619449019234,
2.74889357189107,3.14159265358979),(0.,1.),.UNSPECIFIED.)
GEOMETRIC_REPRESENTATION_ITEM()
RATIONAL_B_SPLINE_SURFACE(((1.,1.,1.),(1.,1.00267605951747,1.),(1.,0.941599607549782,
1.),(1.,0.828238301901767,1.),(1.,0.787677905717159,1.),(1.,0.726552333980051,
1.),(1.,0.706675310150383,1.),(1.,0.707106781186548,1.)))
REPRESENTATION_ITEM('')
SURFACE()
) ;
#151=(
BOUNDED_SURFACE()
B_SPLINE_SURFACE(3,2,((#164065,#164066,#164067),(#164068,#164069,#164070),
(#164071,#164072,#164073),(#164074,#164075,#164076),(#164077,#164078,#164079),
(#164080,#164081,#164082),(#164083,#164084,#164085),(#164086,#164087,#164088)),
 .UNSPECIFIED.,.F.,.F.,.F.)
B_SPLINE_SURFACE_WITH_KNOTS((4,2,2,4),(3,3),(4.71238898038469,5.49778714378214,
5.89048622548086,6.28318530717959),(0.,1.),.UNSPECIFIED.)
GEOMETRIC_REPRESENTATION_ITEM()
RATIONAL_B_SPLINE_SURFACE(((1.,1.,1.),(1.,1.00267605951742,1.),(1.,0.941599607549842,
1.),(1.,0.828238301901737,1.),(1.,0.787677905717144,1.),(1.,0.726552333980065,
1.),(1.,0.706675310150372,1.),(1.,0.707106781186548,1.)))
REPRESENTATION_ITEM('')
SURFACE()
) ;
#152=(
BOUNDED_SURFACE()
B_SPLINE_SURFACE(3,2,((#164093,#164094,#164095),(#164096,#164097,#164098),
(#164099,#164100,#164101),(#164102,#164103,#164104),(#164105,#164106,#164107),
(#164108,#164109,#164110),(#164111,#164112,#164113),(#164114,#164115,#164116)),
 .UNSPECIFIED.,.F.,.F.,.F.)
B_SPLINE_SURFACE_WITH_KNOTS((4,2,2,4),(3,3),(1.5707963267949,2.35619449019234,
2.74889357189107,3.14159265358979),(0.,1.),.UNSPECIFIED.)
GEOMETRIC_REPRESENTATION_ITEM()
RATIONAL_B_SPLINE_SURFACE(((1.,1.,1.),(1.,1.0026760595174,1.),(1.,0.941599607549881,
1.),(1.,0.828238301901717,1.),(1.,0.787677905717207,1.),(1.,0.726552333980003,
1.),(1.,0.706675310150419,1.),(1.,0.707106781186548,1.)))
REPRESENTATION_ITEM('')
SURFACE()
) ;
#153=(
BOUNDED_SURFACE()
B_SPLINE_SURFACE(3,2,((#164138,#164139,#164140),(#164141,#164142,#164143),
(#164144,#164145,#164146),(#164147,#164148,#164149),(#164150,#164151,#164152),
(#164153,#164154,#164155),(#164156,#164157,#164158),(#164159,#164160,#164161)),
 .UNSPECIFIED.,.F.,.F.,.F.)
B_SPLINE_SURFACE_WITH_KNOTS((4,2,2,4),(3,3),(4.71238898038469,5.49778714378214,
5.89048622548086,6.28318530717959),(0.,1.),.UNSPECIFIED.)
GEOMETRIC_REPRESENTATION_ITEM()
RATIONAL_B_SPLINE_SURFACE(((1.,1.,1.),(1.,1.00267605951742,1.),(1.,0.941599607549842,
1.),(1.,0.828238301901737,1.),(1.,0.787677905717207,1.),(1.,0.726552333980003,
1.),(1.,0.706675310150423,1.),(1.,0.707106781186548,1.)))
REPRESENTATION_ITEM('')
SURFACE()
) ;
#154=(
BOUNDED_SURFACE()
B_SPLINE_SURFACE(3,2,((#164162,#164163,#164164),(#164165,#164166,#164167),
(#164168,#164169,#164170),(#164171,#164172,#164173),(#164174,#164175,#164176),
(#164177,#164178,#164179),(#164180,#164181,#164182),(#164183,#164184,#164185)),
 .UNSPECIFIED.,.F.,.F.,.F.)
B_SPLINE_SURFACE_WITH_KNOTS((4,2,2,4),(3,3),(3.38657131671666,3.71802573263366,
4.04948014855067,4.71238898038469),(-0.000420825308263448,1.00042070189224),
 .UNSPECIFIED.)
GEOMETRIC_REPRESENTATION_ITEM()
RATIONAL_B_SPLINE_SURFACE(((1.00022935631984,0.727377552435123,1.00022928902791),
(1.00021435583136,0.745207756069495,1.00021429294048),(1.0001903191047,
0.773778807684603,1.00019026326607),(1.00013753194992,0.836523812238713,
1.00013749159878),(1.00010896375274,0.8704811579365,1.00010893178334),(1.00003378452297,
0.959842312830357,1.00003377461078),(0.999998875499966,1.00133662744397,
0.999998875829888),(1.,1.,1.)))
REPRESENTATION_ITEM('')
SURFACE()
) ;
#155=(
BOUNDED_SURFACE()
B_SPLINE_SURFACE(3,2,((#164187,#164188,#164189),(#164190,#164191,#164192),
(#164193,#164194,#164195),(#164196,#164197,#164198)),.UNSPECIFIED.,.F.,
 .F.,.F.)
B_SPLINE_SURFACE_WITH_KNOTS((4,4),(3,3),(1.32581766366803,1.5707963267949),
(0.,1.),.UNSPECIFIED.)
GEOMETRIC_REPRESENTATION_ITEM()
RATIONAL_B_SPLINE_SURFACE(((1.,0.727606875108995,1.),(1.,0.721005575721675,
1.),(1.,0.71410949947975,1.),(1.,0.707106781186548,1.)))
REPRESENTATION_ITEM('')
SURFACE()
) ;
#156=(
BOUNDED_SURFACE()
B_SPLINE_SURFACE(3,2,((#164214,#164215,#164216),(#164217,#164218,#164219),
(#164220,#164221,#164222),(#164223,#164224,#164225)),.UNSPECIFIED.,.F.,
 .F.,.F.)
B_SPLINE_SURFACE_WITH_KNOTS((4,4),(3,3),(3.92699081698723,4.71238898038469),
(0.,1.),.UNSPECIFIED.)
GEOMETRIC_REPRESENTATION_ITEM()
RATIONAL_B_SPLINE_SURFACE(((1.,0.866025403784441,1.),(1.,0.828363615049339,
1.),(1.,0.772698924407948,1.),(1.,0.707106781186548,1.)))
REPRESENTATION_ITEM('')
SURFACE()
) ;
#157=(
BOUNDED_SURFACE()
B_SPLINE_SURFACE(3,2,((#164227,#164228,#164229),(#164230,#164231,#164232),
(#164233,#164234,#164235),(#164236,#164237,#164238)),.UNSPECIFIED.,.F.,
 .F.,.F.)
B_SPLINE_SURFACE_WITH_KNOTS((4,4),(3,3),(1.5707963267949,2.35619449019234),
(0.,1.),.UNSPECIFIED.)
GEOMETRIC_REPRESENTATION_ITEM()
RATIONAL_B_SPLINE_SURFACE(((1.,1.,1.),(1.,1.00150544078213,1.),(1.,0.943158245625731,
1.),(1.,0.866025403784441,1.)))
REPRESENTATION_ITEM('')
SURFACE()
) ;
#158=(
BOUNDED_SURFACE()
B_SPLINE_SURFACE(3,2,((#164239,#164240,#164241),(#164242,#164243,#164244),
(#164245,#164246,#164247),(#164248,#164249,#164250)),.UNSPECIFIED.,.F.,
 .F.,.F.)
B_SPLINE_SURFACE_WITH_KNOTS((4,4),(3,3),(7.06858347057708,7.85398163397448),
(0.,1.),.UNSPECIFIED.)
GEOMETRIC_REPRESENTATION_ITEM()
RATIONAL_B_SPLINE_SURFACE(((1.,0.866025403784455,1.),(1.,0.943158245625741,
1.),(1.,1.00150544078213,1.),(1.,1.,1.)))
REPRESENTATION_ITEM('')
SURFACE()
) ;
#159=(
BOUNDED_SURFACE()
B_SPLINE_SURFACE(3,2,((#164252,#164253,#164254),(#164255,#164256,#164257),
(#164258,#164259,#164260),(#164261,#164262,#164263)),.UNSPECIFIED.,.F.,
 .F.,.F.)
B_SPLINE_SURFACE_WITH_KNOTS((4,4),(3,3),(1.5707963267949,2.35619449019239),
(0.,1.),.UNSPECIFIED.)
GEOMETRIC_REPRESENTATION_ITEM()
RATIONAL_B_SPLINE_SURFACE(((1.,0.707106781186545,1.),(1.,0.772698924407959,
1.),(1.,0.828363615049342,1.),(1.,0.866025403784447,1.)))
REPRESENTATION_ITEM('')
SURFACE()
) ;
#160=(
BOUNDED_SURFACE()
B_SPLINE_SURFACE(3,2,((#164279,#164280,#164281),(#164282,#164283,#164284),
(#164285,#164286,#164287),(#164288,#164289,#164290)),.UNSPECIFIED.,.F.,
 .F.,.F.)
B_SPLINE_SURFACE_WITH_KNOTS((4,4),(3,3),(4.71238898038469,4.95736764351155),
(0.,1.),.UNSPECIFIED.)
GEOMETRIC_REPRESENTATION_ITEM()
RATIONAL_B_SPLINE_SURFACE(((1.,0.707106781186548,1.),(1.,0.714109499479743,
1.),(1.,0.721005575721684,1.),(1.,0.727606875108989,1.)))
REPRESENTATION_ITEM('')
SURFACE()
) ;
#161=(
BOUNDED_SURFACE()
B_SPLINE_SURFACE(3,2,((#164292,#164293,#164294),(#164295,#164296,#164297),
(#164298,#164299,#164300),(#164301,#164302,#164303),(#164304,#164305,#164306),
(#164307,#164308,#164309),(#164310,#164311,#164312),(#164313,#164314,#164315)),
 .UNSPECIFIED.,.F.,.F.,.F.)
B_SPLINE_SURFACE_WITH_KNOTS((4,2,2,4),(3,3),(3.38657131671666,3.71802573263366,
4.04948014855067,4.71238898038469),(-0.000420825308919027,1.00042070189557),
 .UNSPECIFIED.)
GEOMETRIC_REPRESENTATION_ITEM()
RATIONAL_B_SPLINE_SURFACE(((1.00022935632021,0.727377552434032,1.00022928902973),
(1.00021435583169,0.745207756068483,1.00021429294218),(1.00019031910499,
0.773778807683706,1.00019026326758),(1.00013753195014,0.836523812238065,
1.00013749159987),(1.0001089637529,0.870481157935983,1.0001089317842),(1.00003378452302,
0.959842312830197,1.00003377461104),(0.999998875499964,1.00133662744398,
0.999998875829879),(1.,1.,1.)))
REPRESENTATION_ITEM('')
SURFACE()
) ;
#162=(
BOUNDED_SURFACE()
B_SPLINE_SURFACE(3,2,((#164530,#164531,#164532),(#164533,#164534,#164535),
(#164536,#164537,#164538),(#164539,#164540,#164541),(#164542,#164543,#164544),
(#164545,#164546,#164547),(#164548,#164549,#164550),(#164551,#164552,#164553)),
 .UNSPECIFIED.,.F.,.F.,.F.)
B_SPLINE_SURFACE_WITH_KNOTS((4,2,2,4),(3,3),(1.5707963267949,2.35619449019234,
2.74889357189107,3.14159265358979),(0.,1.),.UNSPECIFIED.)
GEOMETRIC_REPRESENTATION_ITEM()
RATIONAL_B_SPLINE_SURFACE(((1.,1.,1.),(1.,1.00267605951747,1.),(1.,0.941599607549782,
1.),(1.,0.828238301901767,1.),(1.,0.787677905717283,1.),(1.,0.726552333979927,
1.),(1.,0.706675310150483,1.),(1.,0.707106781186548,1.)))
REPRESENTATION_ITEM('')
SURFACE()
) ;
#163=(
BOUNDED_SURFACE()
B_SPLINE_SURFACE(3,2,((#164557,#164558,#164559),(#164560,#164561,#164562),
(#164563,#164564,#164565),(#164566,#164567,#164568),(#164569,#164570,#164571),
(#164572,#164573,#164574),(#164575,#164576,#164577),(#164578,#164579,#164580)),
 .UNSPECIFIED.,.F.,.F.,.F.)
B_SPLINE_SURFACE_WITH_KNOTS((4,2,2,4),(3,3),(4.71238898038469,5.49778714378214,
5.89048622548086,6.28318530717959),(0.,1.),.UNSPECIFIED.)
GEOMETRIC_REPRESENTATION_ITEM()
RATIONAL_B_SPLINE_SURFACE(((1.,1.,1.),(1.,1.00267605951751,1.),(1.,0.941599607549728,
1.),(1.,0.828238301901794,1.),(1.,0.787677905717269,1.),(1.,0.726552333979941,
1.),(1.,0.706675310150473,1.),(1.,0.707106781186548,1.)))
REPRESENTATION_ITEM('')
SURFACE()
) ;
#164=(
BOUNDED_SURFACE()
B_SPLINE_SURFACE(3,2,((#164585,#164586,#164587),(#164588,#164589,#164590),
(#164591,#164592,#164593),(#164594,#164595,#164596),(#164597,#164598,#164599),
(#164600,#164601,#164602),(#164603,#164604,#164605),(#164606,#164607,#164608)),
 .UNSPECIFIED.,.F.,.F.,.F.)
B_SPLINE_SURFACE_WITH_KNOTS((4,2,2,4),(3,3),(1.5707963267949,2.35619449019234,
2.74889357189107,3.14159265358979),(0.,1.),.UNSPECIFIED.)
GEOMETRIC_REPRESENTATION_ITEM()
RATIONAL_B_SPLINE_SURFACE(((1.,1.,1.),(1.,1.00267605951739,1.),(1.,0.941599607549883,
1.),(1.,0.828238301901719,1.),(1.,0.787677905717209,1.),(1.,0.726552333979999,
1.),(1.,0.706675310150425,1.),(1.,0.707106781186548,1.)))
REPRESENTATION_ITEM('')
SURFACE()
) ;
#165=(
BOUNDED_SURFACE()
B_SPLINE_SURFACE(3,2,((#164630,#164631,#164632),(#164633,#164634,#164635),
(#164636,#164637,#164638),(#164639,#164640,#164641),(#164642,#164643,#164644),
(#164645,#164646,#164647),(#164648,#164649,#164650),(#164651,#164652,#164653)),
 .UNSPECIFIED.,.F.,.F.,.F.)
B_SPLINE_SURFACE_WITH_KNOTS((4,2,2,4),(3,3),(4.71238898038469,5.49778714378214,
5.89048622548086,6.28318530717959),(0.,1.),.UNSPECIFIED.)
GEOMETRIC_REPRESENTATION_ITEM()
RATIONAL_B_SPLINE_SURFACE(((1.,1.,1.),(1.,1.00267605951742,1.),(1.,0.941599607549841,
1.),(1.,0.82823830190174,1.),(1.,0.787677905717209,1.),(1.,0.726552333979999,
1.),(1.,0.706675310150426,1.),(1.,0.707106781186548,1.)))
REPRESENTATION_ITEM('')
SURFACE()
) ;
#166=(
BOUNDED_SURFACE()
B_SPLINE_SURFACE(3,2,((#164654,#164655,#164656),(#164657,#164658,#164659),
(#164660,#164661,#164662),(#164663,#164664,#164665),(#164666,#164667,#164668),
(#164669,#164670,#164671),(#164672,#164673,#164674),(#164675,#164676,#164677)),
 .UNSPECIFIED.,.F.,.F.,.F.)
B_SPLINE_SURFACE_WITH_KNOTS((4,2,2,4),(3,3),(3.38657131671666,3.71802573263366,
4.04948014855067,4.71238898038469),(-0.000420825307961358,1.00042070189188),
 .UNSPECIFIED.)
GEOMETRIC_REPRESENTATION_ITEM()
RATIONAL_B_SPLINE_SURFACE(((1.00022935631968,0.727377552435299,1.00022928902772),
(1.00021435583119,0.74520775606967,1.0002142929403),(1.00019031910456,0.773778807684758,
1.00019026326591),(1.00013753194983,0.836523812238825,1.00013749159866),
(1.00010896375265,0.870481157936586,1.00010893178325),(1.00003378452295,
0.959842312830383,1.00003377461075),(0.999998875499967,1.00133662744397,
0.999998875829889),(1.,1.,1.)))
REPRESENTATION_ITEM('')
SURFACE()
) ;
#167=(
BOUNDED_SURFACE()
B_SPLINE_SURFACE(3,2,((#164679,#164680,#164681),(#164682,#164683,#164684),
(#164685,#164686,#164687),(#164688,#164689,#164690)),.UNSPECIFIED.,.F.,
 .F.,.F.)
B_SPLINE_SURFACE_WITH_KNOTS((4,4),(3,3),(1.32581766366803,1.5707963267949),
(0.,1.),.UNSPECIFIED.)
GEOMETRIC_REPRESENTATION_ITEM()
RATIONAL_B_SPLINE_SURFACE(((1.,0.727606875108989,1.),(1.,0.721005575721685,
1.),(1.,0.714109499479745,1.),(1.,0.707106781186548,1.)))
REPRESENTATION_ITEM('')
SURFACE()
) ;
#168=(
BOUNDED_SURFACE()
B_SPLINE_SURFACE(3,2,((#164706,#164707,#164708),(#164709,#164710,#164711),
(#164712,#164713,#164714),(#164715,#164716,#164717)),.UNSPECIFIED.,.F.,
 .F.,.F.)
B_SPLINE_SURFACE_WITH_KNOTS((4,4),(3,3),(3.92699081698723,4.71238898038469),
(0.,1.),.UNSPECIFIED.)
GEOMETRIC_REPRESENTATION_ITEM()
RATIONAL_B_SPLINE_SURFACE(((1.,0.866025403784441,1.),(1.,0.828363615049344,
1.),(1.,0.772698924407949,1.),(1.,0.707106781186548,1.)))
REPRESENTATION_ITEM('')
SURFACE()
) ;
#169=(
BOUNDED_SURFACE()
B_SPLINE_SURFACE(3,2,((#164719,#164720,#164721),(#164722,#164723,#164724),
(#164725,#164726,#164727),(#164728,#164729,#164730)),.UNSPECIFIED.,.F.,
 .F.,.F.)
B_SPLINE_SURFACE_WITH_KNOTS((4,4),(3,3),(1.5707963267949,2.35619449019234),
(0.,1.),.UNSPECIFIED.)
GEOMETRIC_REPRESENTATION_ITEM()
RATIONAL_B_SPLINE_SURFACE(((1.,1.,1.),(1.,1.00150544078213,1.),(1.,0.943158245625731,
1.),(1.,0.866025403784441,1.)))
REPRESENTATION_ITEM('')
SURFACE()
) ;
#170=(
BOUNDED_SURFACE()
B_SPLINE_SURFACE(3,2,((#164731,#164732,#164733),(#164734,#164735,#164736),
(#164737,#164738,#164739),(#164740,#164741,#164742)),.UNSPECIFIED.,.F.,
 .F.,.F.)
B_SPLINE_SURFACE_WITH_KNOTS((4,4),(3,3),(7.06858347057709,7.85398163397448),
(0.,1.),.UNSPECIFIED.)
GEOMETRIC_REPRESENTATION_ITEM()
RATIONAL_B_SPLINE_SURFACE(((1.,0.866025403784455,1.),(1.,0.943158245625743,
1.),(1.,1.00150544078213,1.),(1.,1.,1.)))
REPRESENTATION_ITEM('')
SURFACE()
) ;
#171=(
BOUNDED_SURFACE()
B_SPLINE_SURFACE(3,2,((#164744,#164745,#164746),(#164747,#164748,#164749),
(#164750,#164751,#164752),(#164753,#164754,#164755)),.UNSPECIFIED.,.F.,
 .F.,.F.)
B_SPLINE_SURFACE_WITH_KNOTS((4,4),(3,3),(1.5707963267949,2.35619449019239),
(0.,1.),.UNSPECIFIED.)
GEOMETRIC_REPRESENTATION_ITEM()
RATIONAL_B_SPLINE_SURFACE(((1.,0.707106781186545,1.),(1.,0.772698924407961,
1.),(1.,0.828363615049341,1.),(1.,0.866025403784449,1.)))
REPRESENTATION_ITEM('')
SURFACE()
) ;
#172=(
BOUNDED_SURFACE()
B_SPLINE_SURFACE(3,2,((#164771,#164772,#164773),(#164774,#164775,#164776),
(#164777,#164778,#164779),(#164780,#164781,#164782)),.UNSPECIFIED.,.F.,
 .F.,.F.)
B_SPLINE_SURFACE_WITH_KNOTS((4,4),(3,3),(4.71238898038469,4.95736764351155),
(0.,1.),.UNSPECIFIED.)
GEOMETRIC_REPRESENTATION_ITEM()
RATIONAL_B_SPLINE_SURFACE(((1.,0.707106781186548,1.),(1.,0.714109499479746,
1.),(1.,0.721005575721676,1.),(1.,0.727606875108995,1.)))
REPRESENTATION_ITEM('')
SURFACE()
) ;
#173=(
BOUNDED_SURFACE()
B_SPLINE_SURFACE(3,2,((#164784,#164785,#164786),(#164787,#164788,#164789),
(#164790,#164791,#164792),(#164793,#164794,#164795),(#164796,#164797,#164798),
(#164799,#164800,#164801),(#164802,#164803,#164804),(#164805,#164806,#164807)),
 .UNSPECIFIED.,.F.,.F.,.F.)
B_SPLINE_SURFACE_WITH_KNOTS((4,2,2,4),(3,3),(3.38657131671666,3.71802573263366,
4.04948014855067,4.71238898038469),(-0.00042082530997056,1.00042070189335),
 .UNSPECIFIED.)
GEOMETRIC_REPRESENTATION_ITEM()
RATIONAL_B_SPLINE_SURFACE(((1.00022935632077,0.727377552434356,1.00022928902852),
(1.00021435583222,0.745207756068763,1.00021429294105),(1.00019031910547,
0.773778807683983,1.00019026326658),(1.00013753195048,0.836523812238235,
1.00013749159914),(1.00010896375318,0.870481157936081,1.00010893178364),
(1.00003378452311,0.95984231283035,1.00003377461086),(0.999998875499962,
1.00133662744389,0.999998875829885),(1.,1.,1.)))
REPRESENTATION_ITEM('')
SURFACE()
) ;
#174=(
BOUNDED_SURFACE()
B_SPLINE_SURFACE(3,2,((#165022,#165023,#165024),(#165025,#165026,#165027),
(#165028,#165029,#165030),(#165031,#165032,#165033),(#165034,#165035,#165036),
(#165037,#165038,#165039),(#165040,#165041,#165042),(#165043,#165044,#165045)),
 .UNSPECIFIED.,.F.,.F.,.F.)
B_SPLINE_SURFACE_WITH_KNOTS((4,2,2,4),(3,3),(1.5707963267949,2.35619449019234,
2.74889357189107,3.14159265358979),(0.,1.),.UNSPECIFIED.)
GEOMETRIC_REPRESENTATION_ITEM()
RATIONAL_B_SPLINE_SURFACE(((1.,1.,1.),(1.,1.00267605951743,1.),(1.,0.941599607549841,
1.),(1.,0.82823830190174,1.),(1.,0.787677905717223,1.),(1.,0.726552333979985,
1.),(1.,0.706675310150436,1.),(1.,0.707106781186548,1.)))
REPRESENTATION_ITEM('')
SURFACE()
) ;
#175=(
BOUNDED_SURFACE()
B_SPLINE_SURFACE(3,2,((#165049,#165050,#165051),(#165052,#165053,#165054),
(#165055,#165056,#165057),(#165058,#165059,#165060),(#165061,#165062,#165063),
(#165064,#165065,#165066),(#165067,#165068,#165069),(#165070,#165071,#165072)),
 .UNSPECIFIED.,.F.,.F.,.F.)
B_SPLINE_SURFACE_WITH_KNOTS((4,2,2,4),(3,3),(4.71238898038469,5.49778714378214,
5.89048622548086,6.28318530717959),(0.,1.),.UNSPECIFIED.)
GEOMETRIC_REPRESENTATION_ITEM()
RATIONAL_B_SPLINE_SURFACE(((1.,1.,1.),(1.,1.00267605951742,1.),(1.,0.941599607549841,
1.),(1.,0.82823830190174,1.),(1.,0.787677905717209,1.),(1.,0.726552333979999,
1.),(1.,0.706675310150426,1.),(1.,0.707106781186548,1.)))
REPRESENTATION_ITEM('')
SURFACE()
) ;
#176=(
BOUNDED_SURFACE()
B_SPLINE_SURFACE(3,2,((#165077,#165078,#165079),(#165080,#165081,#165082),
(#165083,#165084,#165085),(#165086,#165087,#165088),(#165089,#165090,#165091),
(#165092,#165093,#165094),(#165095,#165096,#165097),(#165098,#165099,#165100)),
 .UNSPECIFIED.,.F.,.F.,.F.)
B_SPLINE_SURFACE_WITH_KNOTS((4,2,2,4),(3,3),(1.5707963267949,2.35619449019234,
2.74889357189107,3.14159265358979),(0.,1.),.UNSPECIFIED.)
GEOMETRIC_REPRESENTATION_ITEM()
RATIONAL_B_SPLINE_SURFACE(((1.,1.,1.),(1.,1.00267605951739,1.),(1.,0.941599607549883,
1.),(1.,0.828238301901719,1.),(1.,0.787677905717209,1.),(1.,0.726552333979999,
1.),(1.,0.706675310150425,1.),(1.,0.707106781186548,1.)))
REPRESENTATION_ITEM('')
SURFACE()
) ;
#177=(
BOUNDED_SURFACE()
B_SPLINE_SURFACE(3,2,((#165122,#165123,#165124),(#165125,#165126,#165127),
(#165128,#165129,#165130),(#165131,#165132,#165133),(#165134,#165135,#165136),
(#165137,#165138,#165139),(#165140,#165141,#165142),(#165143,#165144,#165145)),
 .UNSPECIFIED.,.F.,.F.,.F.)
B_SPLINE_SURFACE_WITH_KNOTS((4,2,2,4),(3,3),(4.71238898038469,5.49778714378214,
5.89048622548086,6.28318530717959),(0.,1.),.UNSPECIFIED.)
GEOMETRIC_REPRESENTATION_ITEM()
RATIONAL_B_SPLINE_SURFACE(((1.,1.,1.),(1.,1.00267605951742,1.),(1.,0.941599607549841,
1.),(1.,0.82823830190174,1.),(1.,0.787677905717209,1.),(1.,0.726552333979999,
1.),(1.,0.706675310150426,1.),(1.,0.707106781186548,1.)))
REPRESENTATION_ITEM('')
SURFACE()
) ;
#178=(
BOUNDED_SURFACE()
B_SPLINE_SURFACE(3,2,((#165146,#165147,#165148),(#165149,#165150,#165151),
(#165152,#165153,#165154),(#165155,#165156,#165157),(#165158,#165159,#165160),
(#165161,#165162,#165163),(#165164,#165165,#165166),(#165167,#165168,#165169)),
 .UNSPECIFIED.,.F.,.F.,.F.)
B_SPLINE_SURFACE_WITH_KNOTS((4,2,2,4),(3,3),(3.38657131671666,3.71802573263366,
4.04948014855067,4.71238898038469),(-0.000420825307131761,1.00042070189354),
 .UNSPECIFIED.)
GEOMETRIC_REPRESENTATION_ITEM()
RATIONAL_B_SPLINE_SURFACE(((1.00022935631923,0.727377552435078,1.00022928902862),
(1.00021435583078,0.745207756069438,1.00021429294114),(1.00019031910419,
0.773778807684582,1.00019026326667),(1.00013753194956,0.836523812238669,
1.0001374915992),(1.00010896375244,0.870481157936476,1.00010893178368),
(1.00003378452288,0.959842312830354,1.00003377461088),(0.999998875499969,
1.00133662744396,0.999998875829884),(1.,1.,1.)))
REPRESENTATION_ITEM('')
SURFACE()
) ;
#179=(
BOUNDED_SURFACE()
B_SPLINE_SURFACE(3,2,((#165171,#165172,#165173),(#165174,#165175,#165176),
(#165177,#165178,#165179),(#165180,#165181,#165182)),.UNSPECIFIED.,.F.,
 .F.,.F.)
B_SPLINE_SURFACE_WITH_KNOTS((4,4),(3,3),(1.32581766366803,1.5707963267949),
(0.,1.),.UNSPECIFIED.)
GEOMETRIC_REPRESENTATION_ITEM()
RATIONAL_B_SPLINE_SURFACE(((1.,0.727606875108995,1.),(1.,0.721005575721675,
1.),(1.,0.71410949947975,1.),(1.,0.707106781186548,1.)))
REPRESENTATION_ITEM('')
SURFACE()
) ;
#180=(
BOUNDED_SURFACE()
B_SPLINE_SURFACE(3,2,((#165198,#165199,#165200),(#165201,#165202,#165203),
(#165204,#165205,#165206),(#165207,#165208,#165209)),.UNSPECIFIED.,.F.,
 .F.,.F.)
B_SPLINE_SURFACE_WITH_KNOTS((4,4),(3,3),(3.92699081698722,4.71238898038469),
(0.,1.),.UNSPECIFIED.)
GEOMETRIC_REPRESENTATION_ITEM()
RATIONAL_B_SPLINE_SURFACE(((1.,0.866025403784442,1.),(1.,0.828363615049333,
1.),(1.,0.772698924407957,1.),(1.,0.707106781186545,1.)))
REPRESENTATION_ITEM('')
SURFACE()
) ;
#181=(
BOUNDED_SURFACE()
B_SPLINE_SURFACE(3,2,((#165211,#165212,#165213),(#165214,#165215,#165216),
(#165217,#165218,#165219),(#165220,#165221,#165222)),.UNSPECIFIED.,.F.,
 .F.,.F.)
B_SPLINE_SURFACE_WITH_KNOTS((4,4),(3,3),(1.5707963267949,2.35619449019234),
(0.,1.),.UNSPECIFIED.)
GEOMETRIC_REPRESENTATION_ITEM()
RATIONAL_B_SPLINE_SURFACE(((1.,1.,1.),(1.,1.00150544078214,1.),(1.,0.943158245625729,
1.),(1.,0.866025403784442,1.)))
REPRESENTATION_ITEM('')
SURFACE()
) ;
#182=(
BOUNDED_SURFACE()
B_SPLINE_SURFACE(3,2,((#165223,#165224,#165225),(#165226,#165227,#165228),
(#165229,#165230,#165231),(#165232,#165233,#165234)),.UNSPECIFIED.,.F.,
 .F.,.F.)
B_SPLINE_SURFACE_WITH_KNOTS((4,4),(3,3),(7.06858347057709,7.85398163397448),
(0.,1.),.UNSPECIFIED.)
GEOMETRIC_REPRESENTATION_ITEM()
RATIONAL_B_SPLINE_SURFACE(((1.,0.866025403784455,1.),(1.,0.943158245625743,
1.),(1.,1.00150544078213,1.),(1.,1.,1.)))
REPRESENTATION_ITEM('')
SURFACE()
) ;
#183=(
BOUNDED_SURFACE()
B_SPLINE_SURFACE(3,2,((#165236,#165237,#165238),(#165239,#165240,#165241),
(#165242,#165243,#165244),(#165245,#165246,#165247)),.UNSPECIFIED.,.F.,
 .F.,.F.)
B_SPLINE_SURFACE_WITH_KNOTS((4,4),(3,3),(1.5707963267949,2.35619449019239),
(0.,1.),.UNSPECIFIED.)
GEOMETRIC_REPRESENTATION_ITEM()
RATIONAL_B_SPLINE_SURFACE(((1.,0.707106781186545,1.),(1.,0.772698924407961,
1.),(1.,0.828363615049341,1.),(1.,0.866025403784449,1.)))
REPRESENTATION_ITEM('')
SURFACE()
) ;
#184=(
BOUNDED_SURFACE()
B_SPLINE_SURFACE(3,2,((#165263,#165264,#165265),(#165266,#165267,#165268),
(#165269,#165270,#165271),(#165272,#165273,#165274)),.UNSPECIFIED.,.F.,
 .F.,.F.)
B_SPLINE_SURFACE_WITH_KNOTS((4,4),(3,3),(4.71238898038469,4.95736764351155),
(0.,1.),.UNSPECIFIED.)
GEOMETRIC_REPRESENTATION_ITEM()
RATIONAL_B_SPLINE_SURFACE(((1.,0.707106781186548,1.),(1.,0.714109499479746,
1.),(1.,0.721005575721676,1.),(1.,0.727606875108995,1.)))
REPRESENTATION_ITEM('')
SURFACE()
) ;
#185=(
BOUNDED_SURFACE()
B_SPLINE_SURFACE(3,2,((#165276,#165277,#165278),(#165279,#165280,#165281),
(#165282,#165283,#165284),(#165285,#165286,#165287),(#165288,#165289,#165290),
(#165291,#165292,#165293),(#165294,#165295,#165296),(#165297,#165298,#165299)),
 .UNSPECIFIED.,.F.,.F.,.F.)
B_SPLINE_SURFACE_WITH_KNOTS((4,2,2,4),(3,3),(3.38657131671666,3.71802573263366,
4.04948014855067,4.71238898038469),(-0.000420825309824966,1.00042070189421),
 .UNSPECIFIED.)
GEOMETRIC_REPRESENTATION_ITEM()
RATIONAL_B_SPLINE_SURFACE(((1.0002293563207,0.72737755243416,1.00022928902899),
(1.00021435583215,0.74520775606858,1.00021429294149),(1.0001903191054,0.77377880768382,
1.00019026326696),(1.00013753195043,0.836523812238119,1.00013749159943),
(1.00010896375314,0.870481157935989,1.00010893178386),(1.0000337845231,
0.959842312830321,1.00003377461093),(0.999998875499962,1.0013366274439,
0.999998875829883),(1.,1.,1.)))
REPRESENTATION_ITEM('')
SURFACE()
) ;
#186=(
BOUNDED_SURFACE()
B_SPLINE_SURFACE(3,2,((#165514,#165515,#165516),(#165517,#165518,#165519),
(#165520,#165521,#165522),(#165523,#165524,#165525),(#165526,#165527,#165528),
(#165529,#165530,#165531),(#165532,#165533,#165534),(#165535,#165536,#165537)),
 .UNSPECIFIED.,.F.,.F.,.F.)
B_SPLINE_SURFACE_WITH_KNOTS((4,2,2,4),(3,3),(1.5707963267949,2.35619449019234,
2.74889357189107,3.14159265358979),(0.,1.),.UNSPECIFIED.)
GEOMETRIC_REPRESENTATION_ITEM()
RATIONAL_B_SPLINE_SURFACE(((1.,1.,1.),(1.,1.00267605951751,1.),(1.,0.94159960754973,
1.),(1.,0.828238301901795,1.),(1.,0.787677905717223,1.),(1.,0.726552333979985,
1.),(1.,0.706675310150446,1.),(1.,0.707106781186535,1.)))
REPRESENTATION_ITEM('')
SURFACE()
) ;
#187=(
BOUNDED_SURFACE()
B_SPLINE_SURFACE(3,2,((#165541,#165542,#165543),(#165544,#165545,#165546),
(#165547,#165548,#165549),(#165550,#165551,#165552),(#165553,#165554,#165555),
(#165556,#165557,#165558),(#165559,#165560,#165561),(#165562,#165563,#165564)),
 .UNSPECIFIED.,.F.,.F.,.F.)
B_SPLINE_SURFACE_WITH_KNOTS((4,2,2,4),(3,3),(4.71238898038469,5.49778714378214,
5.89048622548086,6.28318530717959),(0.,1.),.UNSPECIFIED.)
GEOMETRIC_REPRESENTATION_ITEM()
RATIONAL_B_SPLINE_SURFACE(((1.,1.,1.),(1.,1.00267605951751,1.),(1.,0.94159960754973,
1.),(1.,0.828238301901796,1.),(1.,0.787677905717209,1.),(1.,0.726552333979999,
1.),(1.,0.706675310150435,1.),(1.,0.707106781186535,1.)))
REPRESENTATION_ITEM('')
SURFACE()
) ;
#188=(
BOUNDED_SURFACE()
B_SPLINE_SURFACE(3,2,((#165569,#165570,#165571),(#165572,#165573,#165574),
(#165575,#165576,#165577),(#165578,#165579,#165580),(#165581,#165582,#165583),
(#165584,#165585,#165586),(#165587,#165588,#165589),(#165590,#165591,#165592)),
 .UNSPECIFIED.,.F.,.F.,.F.)
B_SPLINE_SURFACE_WITH_KNOTS((4,2,2,4),(3,3),(1.5707963267949,2.35619449019234,
2.74889357189107,3.14159265358979),(0.,1.),.UNSPECIFIED.)
GEOMETRIC_REPRESENTATION_ITEM()
RATIONAL_B_SPLINE_SURFACE(((1.,1.,1.),(1.,1.00267605951731,1.),(1.,0.941599607549997,
1.),(1.,0.828238301901662,1.),(1.,0.787677905717218,1.),(1.,0.726552333980008,
1.),(1.,0.706675310150421,1.),(1.,0.707106781186548,1.)))
REPRESENTATION_ITEM('')
SURFACE()
) ;
#189=(
BOUNDED_SURFACE()
B_SPLINE_SURFACE(3,2,((#165614,#165615,#165616),(#165617,#165618,#165619),
(#165620,#165621,#165622),(#165623,#165624,#165625),(#165626,#165627,#165628),
(#165629,#165630,#165631),(#165632,#165633,#165634),(#165635,#165636,#165637)),
 .UNSPECIFIED.,.F.,.F.,.F.)
B_SPLINE_SURFACE_WITH_KNOTS((4,2,2,4),(3,3),(4.71238898038469,5.49778714378214,
5.89048622548086,6.28318530717959),(0.,1.),.UNSPECIFIED.)
GEOMETRIC_REPRESENTATION_ITEM()
RATIONAL_B_SPLINE_SURFACE(((1.,1.,1.),(1.,1.00267605951734,1.),(1.,0.941599607549954,
1.),(1.,0.828238301901683,1.),(1.,0.787677905717218,1.),(1.,0.726552333980008,
1.),(1.,0.706675310150422,1.),(1.,0.707106781186548,1.)))
REPRESENTATION_ITEM('')
SURFACE()
) ;
#190=(
BOUNDED_SURFACE()
B_SPLINE_SURFACE(3,2,((#165638,#165639,#165640),(#165641,#165642,#165643),
(#165644,#165645,#165646),(#165647,#165648,#165649),(#165650,#165651,#165652),
(#165653,#165654,#165655),(#165656,#165657,#165658),(#165659,#165660,#165661)),
 .UNSPECIFIED.,.F.,.F.,.F.)
B_SPLINE_SURFACE_WITH_KNOTS((4,2,2,4),(3,3),(3.38657131671666,3.71802573263366,
4.04948014855067,4.71238898038469),(-0.000420825307381943,1.00042070189293),
 .UNSPECIFIED.)
GEOMETRIC_REPRESENTATION_ITEM()
RATIONAL_B_SPLINE_SURFACE(((1.00022935631936,0.727377552435165,1.00022928902829),
(1.00021435583091,0.745207756069537,1.00021429294084),(1.0001903191043,
0.773778807684663,1.00019026326638),(1.00013753194964,0.836523812238728,
1.000137491599),(1.00010896375251,0.870481157936522,1.00010893178353),(1.0000337845229,
0.959842312830368,1.00003377461083),(0.999998875499968,1.00133662744396,
0.999998875829886),(1.,1.,1.)))
REPRESENTATION_ITEM('')
SURFACE()
) ;
#191=(
BOUNDED_SURFACE()
B_SPLINE_SURFACE(3,2,((#165663,#165664,#165665),(#165666,#165667,#165668),
(#165669,#165670,#165671),(#165672,#165673,#165674)),.UNSPECIFIED.,.F.,
 .F.,.F.)
B_SPLINE_SURFACE_WITH_KNOTS((4,4),(3,3),(1.32581766366803,1.5707963267949),
(0.,1.),.UNSPECIFIED.)
GEOMETRIC_REPRESENTATION_ITEM()
RATIONAL_B_SPLINE_SURFACE(((1.,0.727606875108984,1.),(1.,0.7210055757217,
1.),(1.,0.714109499479712,1.),(1.,0.70710678118656,1.)))
REPRESENTATION_ITEM('')
SURFACE()
) ;
#192=(
BOUNDED_SURFACE()
B_SPLINE_SURFACE(3,2,((#165690,#165691,#165692),(#165693,#165694,#165695),
(#165696,#165697,#165698),(#165699,#165700,#165701)),.UNSPECIFIED.,.F.,
 .F.,.F.)
B_SPLINE_SURFACE_WITH_KNOTS((4,4),(3,3),(3.92699081698722,4.71238898038469),
(0.,1.),.UNSPECIFIED.)
GEOMETRIC_REPRESENTATION_ITEM()
RATIONAL_B_SPLINE_SURFACE(((1.,0.866025403784442,1.),(1.,0.82836361504934,
1.),(1.,0.772698924407942,1.),(1.,0.707106781186558,1.)))
REPRESENTATION_ITEM('')
SURFACE()
) ;
#193=(
BOUNDED_SURFACE()
B_SPLINE_SURFACE(3,2,((#165703,#165704,#165705),(#165706,#165707,#165708),
(#165709,#165710,#165711),(#165712,#165713,#165714)),.UNSPECIFIED.,.F.,
 .F.,.F.)
B_SPLINE_SURFACE_WITH_KNOTS((4,4),(3,3),(1.5707963267949,2.35619449019234),
(0.,1.),.UNSPECIFIED.)
GEOMETRIC_REPRESENTATION_ITEM()
RATIONAL_B_SPLINE_SURFACE(((1.,1.,1.),(1.,1.00150544078214,1.),(1.,0.943158245625727,
1.),(1.,0.866025403784442,1.)))
REPRESENTATION_ITEM('')
SURFACE()
) ;
#194=(
BOUNDED_SURFACE()
B_SPLINE_SURFACE(3,2,((#165715,#165716,#165717),(#165718,#165719,#165720),
(#165721,#165722,#165723),(#165724,#165725,#165726)),.UNSPECIFIED.,.F.,
 .F.,.F.)
B_SPLINE_SURFACE_WITH_KNOTS((4,4),(3,3),(7.06858347057709,7.85398163397448),
(0.,1.),.UNSPECIFIED.)
GEOMETRIC_REPRESENTATION_ITEM()
RATIONAL_B_SPLINE_SURFACE(((1.,0.866025403784455,1.),(1.,0.943158245625744,
1.),(1.,1.00150544078213,1.),(1.,1.,1.)))
REPRESENTATION_ITEM('')
SURFACE()
) ;
#195=(
BOUNDED_SURFACE()
B_SPLINE_SURFACE(3,2,((#165728,#165729,#165730),(#165731,#165732,#165733),
(#165734,#165735,#165736),(#165737,#165738,#165739)),.UNSPECIFIED.,.F.,
 .F.,.F.)
B_SPLINE_SURFACE_WITH_KNOTS((4,4),(3,3),(1.5707963267949,2.35619449019239),
(0.,1.),.UNSPECIFIED.)
GEOMETRIC_REPRESENTATION_ITEM()
RATIONAL_B_SPLINE_SURFACE(((1.,0.707106781186533,1.),(1.,0.772698924407975,
1.),(1.,0.828363615049334,1.),(1.,0.866025403784449,1.)))
REPRESENTATION_ITEM('')
SURFACE()
) ;
#196=(
BOUNDED_SURFACE()
B_SPLINE_SURFACE(3,2,((#165755,#165756,#165757),(#165758,#165759,#165760),
(#165761,#165762,#165763),(#165764,#165765,#165766)),.UNSPECIFIED.,.F.,
 .F.,.F.)
B_SPLINE_SURFACE_WITH_KNOTS((4,4),(3,3),(4.71238898038469,4.95736764351155),
(0.,1.),.UNSPECIFIED.)
GEOMETRIC_REPRESENTATION_ITEM()
RATIONAL_B_SPLINE_SURFACE(((1.,0.707106781186535,1.),(1.,0.714109499479782,
1.),(1.,0.721005575721652,1.),(1.,0.727606875109006,1.)))
REPRESENTATION_ITEM('')
SURFACE()
) ;
#197=(
BOUNDED_SURFACE()
B_SPLINE_SURFACE(3,2,((#165768,#165769,#165770),(#165771,#165772,#165773),
(#165774,#165775,#165776),(#165777,#165778,#165779),(#165780,#165781,#165782),
(#165783,#165784,#165785),(#165786,#165787,#165788),(#165789,#165790,#165791)),
 .UNSPECIFIED.,.F.,.F.,.F.)
B_SPLINE_SURFACE_WITH_KNOTS((4,2,2,4),(3,3),(3.38657131671666,3.71802573263366,
4.04948014855067,4.71238898038469),(-0.00042082530954674,1.00042070189244),
 .UNSPECIFIED.)
GEOMETRIC_REPRESENTATION_ITEM()
RATIONAL_B_SPLINE_SURFACE(((1.00022935632055,0.727377552434729,1.00022928902802),
(1.000214355832,0.745207756069095,1.00021429294059),(1.00019031910528,0.773778807684285,
1.00019026326617),(1.00013753195035,0.836523812238453,1.00013749159884),
(1.00010896375307,0.870481157936255,1.0001089317834),(1.00003378452308,
0.959842312830403,1.00003377461079),(0.999998875499963,1.00133662744389,
0.999998875829888),(1.,1.,1.)))
REPRESENTATION_ITEM('')
SURFACE()
) ;
#198=(
BOUNDED_SURFACE()
B_SPLINE_SURFACE(3,2,((#166006,#166007,#166008),(#166009,#166010,#166011),
(#166012,#166013,#166014),(#166015,#166016,#166017),(#166018,#166019,#166020),
(#166021,#166022,#166023),(#166024,#166025,#166026),(#166027,#166028,#166029)),
 .UNSPECIFIED.,.F.,.F.,.F.)
B_SPLINE_SURFACE_WITH_KNOTS((4,2,2,4),(3,3),(1.5707963267949,2.35619449019234,
2.74889357189107,3.14159265358979),(0.,1.),.UNSPECIFIED.)
GEOMETRIC_REPRESENTATION_ITEM()
RATIONAL_B_SPLINE_SURFACE(((1.,1.,1.),(1.,1.00267605951743,1.),(1.,0.941599607549841,
1.),(1.,0.82823830190174,1.),(1.,0.787677905717349,1.),(1.,0.726552333979859,
1.),(1.,0.706675310150533,1.),(1.,0.707106781186548,1.)))
REPRESENTATION_ITEM('')
SURFACE()
) ;
#199=(
BOUNDED_SURFACE()
B_SPLINE_SURFACE(3,2,((#166033,#166034,#166035),(#166036,#166037,#166038),
(#166039,#166040,#166041),(#166042,#166043,#166044),(#166045,#166046,#166047),
(#166048,#166049,#166050),(#166051,#166052,#166053),(#166054,#166055,#166056)),
 .UNSPECIFIED.,.F.,.F.,.F.)
B_SPLINE_SURFACE_WITH_KNOTS((4,2,2,4),(3,3),(4.71238898038469,5.49778714378214,
5.89048622548086,6.28318530717959),(0.,1.),.UNSPECIFIED.)
GEOMETRIC_REPRESENTATION_ITEM()
RATIONAL_B_SPLINE_SURFACE(((1.,1.,1.),(1.,1.00267605951742,1.),(1.,0.941599607549841,
1.),(1.,0.82823830190174,1.),(1.,0.787677905717335,1.),(1.,0.726552333979873,
1.),(1.,0.706675310150523,1.),(1.,0.707106781186548,1.)))
REPRESENTATION_ITEM('')
SURFACE()
) ;
#200=(
BOUNDED_SURFACE()
B_SPLINE_SURFACE(3,2,((#166061,#166062,#166063),(#166064,#166065,#166066),
(#166067,#166068,#166069),(#166070,#166071,#166072),(#166073,#166074,#166075),
(#166076,#166077,#166078),(#166079,#166080,#166081),(#166082,#166083,#166084)),
 .UNSPECIFIED.,.F.,.F.,.F.)
B_SPLINE_SURFACE_WITH_KNOTS((4,2,2,4),(3,3),(1.5707963267949,2.35619449019234,
2.74889357189107,3.14159265358979),(0.,1.),.UNSPECIFIED.)
GEOMETRIC_REPRESENTATION_ITEM()
RATIONAL_B_SPLINE_SURFACE(((1.,1.,1.),(1.,1.00267605951739,1.),(1.,0.941599607549887,
1.),(1.,0.828238301901723,1.),(1.,0.787677905717337,1.),(1.,0.726552333979871,
1.),(1.,0.706675310150514,1.),(1.,0.707106781186548,1.)))
REPRESENTATION_ITEM('')
SURFACE()
) ;
#201=(
BOUNDED_SURFACE()
B_SPLINE_SURFACE(3,2,((#166106,#166107,#166108),(#166109,#166110,#166111),
(#166112,#166113,#166114),(#166115,#166116,#166117),(#166118,#166119,#166120),
(#166121,#166122,#166123),(#166124,#166125,#166126),(#166127,#166128,#166129)),
 .UNSPECIFIED.,.F.,.F.,.F.)
B_SPLINE_SURFACE_WITH_KNOTS((4,2,2,4),(3,3),(4.71238898038469,5.49778714378214,
5.89048622548086,6.28318530717959),(0.,1.),.UNSPECIFIED.)
GEOMETRIC_REPRESENTATION_ITEM()
RATIONAL_B_SPLINE_SURFACE(((1.,1.,1.),(1.,1.00267605951742,1.),(1.,0.941599607549844,
1.),(1.,0.828238301901744,1.),(1.,0.787677905717337,1.),(1.,0.726552333979871,
1.),(1.,0.706675310150515,1.),(1.,0.707106781186548,1.)))
REPRESENTATION_ITEM('')
SURFACE()
) ;
#202=(
BOUNDED_SURFACE()
B_SPLINE_SURFACE(3,2,((#166130,#166131,#166132),(#166133,#166134,#166135),
(#166136,#166137,#166138),(#166139,#166140,#166141),(#166142,#166143,#166144),
(#166145,#166146,#166147),(#166148,#166149,#166150),(#166151,#166152,#166153)),
 .UNSPECIFIED.,.F.,.F.,.F.)
B_SPLINE_SURFACE_WITH_KNOTS((4,2,2,4),(3,3),(3.38657131671666,3.71802573263366,
4.04948014855067,4.71238898038469),(-0.000420825307658434,1.00042070189319),
 .UNSPECIFIED.)
GEOMETRIC_REPRESENTATION_ITEM()
RATIONAL_B_SPLINE_SURFACE(((1.00022935631952,0.727377552435029,1.00022928902843),
(1.00021435583105,0.745207756069326,1.00021429294096),(1.00019031910442,
0.773778807684626,1.00019026326651),(1.00013753194973,0.836523812238567,
1.00013749159909),(1.00010896375258,0.870481157936425,1.00010893178359),
(1.00003378452293,0.959842312830407,1.00003377461085),(0.999998875499967,
1.00133662744392,0.999998875829886),(1.,1.,1.)))
REPRESENTATION_ITEM('')
SURFACE()
) ;
#203=(
BOUNDED_SURFACE()
B_SPLINE_SURFACE(3,2,((#166155,#166156,#166157),(#166158,#166159,#166160),
(#166161,#166162,#166163),(#166164,#166165,#166166)),.UNSPECIFIED.,.F.,
 .F.,.F.)
B_SPLINE_SURFACE_WITH_KNOTS((4,4),(3,3),(1.32581766366803,1.5707963267949),
(0.,1.),.UNSPECIFIED.)
GEOMETRIC_REPRESENTATION_ITEM()
RATIONAL_B_SPLINE_SURFACE(((1.,0.727606875108995,1.),(1.,0.72100557572167,
1.),(1.,0.714109499479753,1.),(1.,0.707106781186548,1.)))
REPRESENTATION_ITEM('')
SURFACE()
) ;
#204=(
BOUNDED_SURFACE()
B_SPLINE_SURFACE(3,2,((#166182,#166183,#166184),(#166185,#166186,#166187),
(#166188,#166189,#166190),(#166191,#166192,#166193)),.UNSPECIFIED.,.F.,
 .F.,.F.)
B_SPLINE_SURFACE_WITH_KNOTS((4,4),(3,3),(3.92699081698722,4.71238898038469),
(0.,1.),.UNSPECIFIED.)
GEOMETRIC_REPRESENTATION_ITEM()
RATIONAL_B_SPLINE_SURFACE(((1.,0.866025403784439,1.),(1.,0.828363615049346,
1.),(1.,0.772698924407957,1.),(1.,0.707106781186545,1.)))
REPRESENTATION_ITEM('')
SURFACE()
) ;
#205=(
BOUNDED_SURFACE()
B_SPLINE_SURFACE(3,2,((#166195,#166196,#166197),(#166198,#166199,#166200),
(#166201,#166202,#166203),(#166204,#166205,#166206)),.UNSPECIFIED.,.F.,
 .F.,.F.)
B_SPLINE_SURFACE_WITH_KNOTS((4,4),(3,3),(1.5707963267949,2.35619449019234),
(0.,1.),.UNSPECIFIED.)
GEOMETRIC_REPRESENTATION_ITEM()
RATIONAL_B_SPLINE_SURFACE(((1.,1.,1.),(1.,1.00150544078214,1.),(1.,0.943158245625728,
1.),(1.,0.866025403784442,1.)))
REPRESENTATION_ITEM('')
SURFACE()
) ;
#206=(
BOUNDED_SURFACE()
B_SPLINE_SURFACE(3,2,((#166207,#166208,#166209),(#166210,#166211,#166212),
(#166213,#166214,#166215),(#166216,#166217,#166218)),.UNSPECIFIED.,.F.,
 .F.,.F.)
B_SPLINE_SURFACE_WITH_KNOTS((4,4),(3,3),(7.06858347057709,7.85398163397448),
(0.,1.),.UNSPECIFIED.)
GEOMETRIC_REPRESENTATION_ITEM()
RATIONAL_B_SPLINE_SURFACE(((1.,0.866025403784455,1.),(1.,0.943158245625744,
1.),(1.,1.00150544078213,1.),(1.,1.,1.)))
REPRESENTATION_ITEM('')
SURFACE()
) ;
#207=(
BOUNDED_SURFACE()
B_SPLINE_SURFACE(3,2,((#166220,#166221,#166222),(#166223,#166224,#166225),
(#166226,#166227,#166228),(#166229,#166230,#166231)),.UNSPECIFIED.,.F.,
 .F.,.F.)
B_SPLINE_SURFACE_WITH_KNOTS((4,4),(3,3),(1.5707963267949,2.35619449019239),
(0.,1.),.UNSPECIFIED.)
GEOMETRIC_REPRESENTATION_ITEM()
RATIONAL_B_SPLINE_SURFACE(((1.,0.707106781186545,1.),(1.,0.772698924407971,
1.),(1.,0.828363615049334,1.),(1.,0.866025403784449,1.)))
REPRESENTATION_ITEM('')
SURFACE()
) ;
#208=(
BOUNDED_SURFACE()
B_SPLINE_SURFACE(3,2,((#166247,#166248,#166249),(#166250,#166251,#166252),
(#166253,#166254,#166255),(#166256,#166257,#166258)),.UNSPECIFIED.,.F.,
 .F.,.F.)
B_SPLINE_SURFACE_WITH_KNOTS((4,4),(3,3),(4.71238898038469,4.95736764351155),
(0.,1.),.UNSPECIFIED.)
GEOMETRIC_REPRESENTATION_ITEM()
RATIONAL_B_SPLINE_SURFACE(((1.,0.707106781186548,1.),(1.,0.714109499479749,
1.),(1.,0.721005575721671,1.),(1.,0.727606875108995,1.)))
REPRESENTATION_ITEM('')
SURFACE()
) ;
#209=(
BOUNDED_SURFACE()
B_SPLINE_SURFACE(3,2,((#166260,#166261,#166262),(#166263,#166264,#166265),
(#166266,#166267,#166268),(#166269,#166270,#166271),(#166272,#166273,#166274),
(#166275,#166276,#166277),(#166278,#166279,#166280),(#166281,#166282,#166283)),
 .UNSPECIFIED.,.F.,.F.,.F.)
B_SPLINE_SURFACE_WITH_KNOTS((4,2,2,4),(3,3),(3.38657131671666,3.71802573263366,
4.04948014855067,4.71238898038469),(-0.00042082530851535,1.00042070189436),
 .UNSPECIFIED.)
GEOMETRIC_REPRESENTATION_ITEM()
RATIONAL_B_SPLINE_SURFACE(((1.00022935631998,0.727377552434477,1.00022928902906),
(1.00021435583148,0.745207756068811,1.00021429294157),(1.00019031910481,
0.773778807684169,1.00019026326703),(1.00013753195001,0.836523812238236,
1.00013749159947),(1.0001089637528,0.870481157936111,1.0001089317839),(1.00003378452299,
0.95984231283043,1.00003377461095),(0.999998875499966,1.00133662744384,
0.999998875829883),(1.,1.,1.)))
REPRESENTATION_ITEM('')
SURFACE()
) ;
#210=(
BOUNDED_SURFACE()
B_SPLINE_SURFACE(3,2,((#166498,#166499,#166500),(#166501,#166502,#166503),
(#166504,#166505,#166506),(#166507,#166508,#166509),(#166510,#166511,#166512),
(#166513,#166514,#166515),(#166516,#166517,#166518),(#166519,#166520,#166521)),
 .UNSPECIFIED.,.F.,.F.,.F.)
B_SPLINE_SURFACE_WITH_KNOTS((4,2,2,4),(3,3),(1.5707963267949,2.35619449019234,
2.74889357189107,3.14159265358979),(0.,1.),.UNSPECIFIED.)
GEOMETRIC_REPRESENTATION_ITEM()
RATIONAL_B_SPLINE_SURFACE(((1.,1.,1.),(1.,1.00267605951734,1.),(1.,0.941599607549954,
1.),(1.,0.828238301901683,1.),(1.,0.787677905717223,1.),(1.,0.726552333979985,
1.),(1.,0.706675310150426,1.),(1.,0.70710678118656,1.)))
REPRESENTATION_ITEM('')
SURFACE()
) ;
#211=(
BOUNDED_SURFACE()
B_SPLINE_SURFACE(3,2,((#166525,#166526,#166527),(#166528,#166529,#166530),
(#166531,#166532,#166533),(#166534,#166535,#166536),(#166537,#166538,#166539),
(#166540,#166541,#166542),(#166543,#166544,#166545),(#166546,#166547,#166548)),
 .UNSPECIFIED.,.F.,.F.,.F.)
B_SPLINE_SURFACE_WITH_KNOTS((4,2,2,4),(3,3),(4.71238898038469,5.49778714378214,
5.89048622548086,6.28318530717959),(0.,1.),.UNSPECIFIED.)
GEOMETRIC_REPRESENTATION_ITEM()
RATIONAL_B_SPLINE_SURFACE(((1.,1.,1.),(1.,1.00267605951734,1.),(1.,0.941599607549954,
1.),(1.,0.828238301901683,1.),(1.,0.787677905717209,1.),(1.,0.726552333979999,
1.),(1.,0.706675310150416,1.),(1.,0.70710678118656,1.)))
REPRESENTATION_ITEM('')
SURFACE()
) ;
#212=(
BOUNDED_SURFACE()
B_SPLINE_SURFACE(3,2,((#166553,#166554,#166555),(#166556,#166557,#166558),
(#166559,#166560,#166561),(#166562,#166563,#166564),(#166565,#166566,#166567),
(#166568,#166569,#166570),(#166571,#166572,#166573),(#166574,#166575,#166576)),
 .UNSPECIFIED.,.F.,.F.,.F.)
B_SPLINE_SURFACE_WITH_KNOTS((4,2,2,4),(3,3),(1.5707963267949,2.35619449019234,
2.74889357189107,3.14159265358979),(0.,1.),.UNSPECIFIED.)
GEOMETRIC_REPRESENTATION_ITEM()
RATIONAL_B_SPLINE_SURFACE(((1.,1.,1.),(1.,1.00267605951746,1.),(1.,0.941599607549799,
1.),(1.,0.828238301901763,1.),(1.,0.787677905717196,1.),(1.,0.72655233398001,
1.),(1.,0.706675310150416,1.),(1.,0.707106781186548,1.)))
REPRESENTATION_ITEM('')
SURFACE()
) ;
#213=(
BOUNDED_SURFACE()
B_SPLINE_SURFACE(3,2,((#166598,#166599,#166600),(#166601,#166602,#166603),
(#166604,#166605,#166606),(#166607,#166608,#166609),(#166610,#166611,#166612),
(#166613,#166614,#166615),(#166616,#166617,#166618),(#166619,#166620,#166621)),
 .UNSPECIFIED.,.F.,.F.,.F.)
B_SPLINE_SURFACE_WITH_KNOTS((4,2,2,4),(3,3),(4.71238898038469,5.49778714378214,
5.89048622548086,6.28318530717959),(0.,1.),.UNSPECIFIED.)
GEOMETRIC_REPRESENTATION_ITEM()
RATIONAL_B_SPLINE_SURFACE(((1.,1.,1.),(1.,1.00267605951749,1.),(1.,0.941599607549756,
1.),(1.,0.828238301901784,1.),(1.,0.787677905717196,1.),(1.,0.72655233398001,
1.),(1.,0.706675310150417,1.),(1.,0.707106781186548,1.)))
REPRESENTATION_ITEM('')
SURFACE()
) ;
#214=(
BOUNDED_SURFACE()
B_SPLINE_SURFACE(3,2,((#166622,#166623,#166624),(#166625,#166626,#166627),
(#166628,#166629,#166630),(#166631,#166632,#166633),(#166634,#166635,#166636),
(#166637,#166638,#166639),(#166640,#166641,#166642),(#166643,#166644,#166645)),
 .UNSPECIFIED.,.F.,.F.,.F.)
B_SPLINE_SURFACE_WITH_KNOTS((4,2,2,4),(3,3),(3.38657131671666,3.71802573263366,
4.04948014855067,4.71238898038469),(-0.000420825308972864,1.00042070189455),
 .UNSPECIFIED.)
GEOMETRIC_REPRESENTATION_ITEM()
RATIONAL_B_SPLINE_SURFACE(((1.00022935632023,0.727377552434312,1.00022928902917),
(1.00021435583172,0.745207756068707,1.00021429294166),(1.00019031910501,
0.773778807683938,1.00019026326711),(1.00013753195016,0.836523812238204,
1.00013749159953),(1.00010896375292,0.870481157936108,1.00010893178394),
(1.00003378452303,0.959842312830239,1.00003377461096),(0.999998875499964,
1.00133662744397,0.999998875829882),(1.,1.,1.)))
REPRESENTATION_ITEM('')
SURFACE()
) ;
#215=(
BOUNDED_SURFACE()
B_SPLINE_SURFACE(3,2,((#166647,#166648,#166649),(#166650,#166651,#166652),
(#166653,#166654,#166655),(#166656,#166657,#166658)),.UNSPECIFIED.,.F.,
 .F.,.F.)
B_SPLINE_SURFACE_WITH_KNOTS((4,4),(3,3),(1.32581766366803,1.5707963267949),
(0.,1.),.UNSPECIFIED.)
GEOMETRIC_REPRESENTATION_ITEM()
RATIONAL_B_SPLINE_SURFACE(((1.,0.727606875109006,1.),(1.,0.72100557572165,
1.),(1.,0.714109499479786,1.),(1.,0.707106781186535,1.)))
REPRESENTATION_ITEM('')
SURFACE()
) ;
#216=(
BOUNDED_SURFACE()
B_SPLINE_SURFACE(3,2,((#166674,#166675,#166676),(#166677,#166678,#166679),
(#166680,#166681,#166682),(#166683,#166684,#166685)),.UNSPECIFIED.,.F.,
 .F.,.F.)
B_SPLINE_SURFACE_WITH_KNOTS((4,4),(3,3),(3.92699081698722,4.71238898038469),
(0.,1.),.UNSPECIFIED.)
GEOMETRIC_REPRESENTATION_ITEM()
RATIONAL_B_SPLINE_SURFACE(((1.,0.866025403784442,1.),(1.,0.828363615049326,
1.),(1.,0.772698924407971,1.),(1.,0.707106781186533,1.)))
REPRESENTATION_ITEM('')
SURFACE()
) ;
#217=(
BOUNDED_SURFACE()
B_SPLINE_SURFACE(3,2,((#166687,#166688,#166689),(#166690,#166691,#166692),
(#166693,#166694,#166695),(#166696,#166697,#166698)),.UNSPECIFIED.,.F.,
 .F.,.F.)
B_SPLINE_SURFACE_WITH_KNOTS((4,4),(3,3),(1.5707963267949,2.35619449019234),
(0.,1.),.UNSPECIFIED.)
GEOMETRIC_REPRESENTATION_ITEM()
RATIONAL_B_SPLINE_SURFACE(((1.,1.,1.),(1.,1.00150544078214,1.),(1.,0.943158245625729,
1.),(1.,0.866025403784442,1.)))
REPRESENTATION_ITEM('')
SURFACE()
) ;
#218=(
BOUNDED_SURFACE()
B_SPLINE_SURFACE(3,2,((#166699,#166700,#166701),(#166702,#166703,#166704),
(#166705,#166706,#166707),(#166708,#166709,#166710)),.UNSPECIFIED.,.F.,
 .F.,.F.)
B_SPLINE_SURFACE_WITH_KNOTS((4,4),(3,3),(7.06858347057706,7.85398163397448),
(0.,1.),.UNSPECIFIED.)
GEOMETRIC_REPRESENTATION_ITEM()
RATIONAL_B_SPLINE_SURFACE(((1.,0.866025403784446,1.),(1.,0.943158245625744,
1.),(1.,1.00150544078213,1.),(1.,1.,1.)))
REPRESENTATION_ITEM('')
SURFACE()
) ;
#219=(
BOUNDED_SURFACE()
B_SPLINE_SURFACE(3,2,((#166712,#166713,#166714),(#166715,#166716,#166717),
(#166718,#166719,#166720),(#166721,#166722,#166723)),.UNSPECIFIED.,.F.,
 .F.,.F.)
B_SPLINE_SURFACE_WITH_KNOTS((4,4),(3,3),(1.5707963267949,2.35619449019237),
(0.,1.),.UNSPECIFIED.)
GEOMETRIC_REPRESENTATION_ITEM()
RATIONAL_B_SPLINE_SURFACE(((1.,0.707106781186545,1.),(1.,0.772698924407959,
1.),(1.,0.828363615049336,1.),(1.,0.86602540378444,1.)))
REPRESENTATION_ITEM('')
SURFACE()
) ;
#220=(
BOUNDED_SURFACE()
B_SPLINE_SURFACE(3,2,((#166739,#166740,#166741),(#166742,#166743,#166744),
(#166745,#166746,#166747),(#166748,#166749,#166750)),.UNSPECIFIED.,.F.,
 .F.,.F.)
B_SPLINE_SURFACE_WITH_KNOTS((4,4),(3,3),(4.71238898038469,4.95736764351155),
(0.,1.),.UNSPECIFIED.)
GEOMETRIC_REPRESENTATION_ITEM()
RATIONAL_B_SPLINE_SURFACE(((1.,0.707106781186548,1.),(1.,0.714109499479746,
1.),(1.,0.721005575721677,1.),(1.,0.727606875108994,1.)))
REPRESENTATION_ITEM('')
SURFACE()
) ;
#221=(
BOUNDED_SURFACE()
B_SPLINE_SURFACE(3,2,((#166752,#166753,#166754),(#166755,#166756,#166757),
(#166758,#166759,#166760),(#166761,#166762,#166763),(#166764,#166765,#166766),
(#166767,#166768,#166769),(#166770,#166771,#166772),(#166773,#166774,#166775)),
 .UNSPECIFIED.,.F.,.F.,.F.)
B_SPLINE_SURFACE_WITH_KNOTS((4,2,2,4),(3,3),(3.38657131671663,3.71802573263365,
4.04948014855066,4.71238898038469),(-0.000420825310317862,1.0004207018963),
 .UNSPECIFIED.)
GEOMETRIC_REPRESENTATION_ITEM()
RATIONAL_B_SPLINE_SURFACE(((1.00022935632096,0.72737755243345,1.00022928903013),
(1.0002143558324,0.745207756067913,1.00021429294255),(1.00019031910563,
0.773778807683235,1.00019026326791),(1.0001375319506,0.83652381223769,1.00013749160011),
(1.00010896375327,0.870481157935671,1.0001089317844),(1.00003378452314,
0.959842312830171,1.0000337746111),(0.99999887549996,1.00133662744394,0.999998875829878),
(1.,1.,1.)))
REPRESENTATION_ITEM('')
SURFACE()
) ;
#222=(
BOUNDED_SURFACE()
B_SPLINE_SURFACE(3,2,((#166990,#166991,#166992),(#166993,#166994,#166995),
(#166996,#166997,#166998),(#166999,#167000,#167001),(#167002,#167003,#167004),
(#167005,#167006,#167007),(#167008,#167009,#167010),(#167011,#167012,#167013)),
 .UNSPECIFIED.,.F.,.F.,.F.)
B_SPLINE_SURFACE_WITH_KNOTS((4,2,2,4),(3,3),(1.5707963267949,2.35619449019234,
2.74889357189107,3.14159265358979),(0.,1.),.UNSPECIFIED.)
GEOMETRIC_REPRESENTATION_ITEM()
RATIONAL_B_SPLINE_SURFACE(((1.,1.,1.),(1.,1.00267605951749,1.),(1.,0.94159960754976,
1.),(1.,0.828238301901782,1.),(1.,0.787677905717208,1.),(1.,0.726552333979998,
1.),(1.,0.706675310150427,1.),(1.,0.707106781186548,1.)))
REPRESENTATION_ITEM('')
SURFACE()
) ;
#223=(
BOUNDED_SURFACE()
B_SPLINE_SURFACE(3,2,((#167017,#167018,#167019),(#167020,#167021,#167022),
(#167023,#167024,#167025),(#167026,#167027,#167028),(#167029,#167030,#167031),
(#167032,#167033,#167034),(#167035,#167036,#167037),(#167038,#167039,#167040)),
 .UNSPECIFIED.,.F.,.F.,.F.)
B_SPLINE_SURFACE_WITH_KNOTS((4,2,2,4),(3,3),(4.71238898038469,5.49778714378214,
5.89048622548086,6.28318530717959),(0.,1.),.UNSPECIFIED.)
GEOMETRIC_REPRESENTATION_ITEM()
RATIONAL_B_SPLINE_SURFACE(((1.,1.,1.),(1.,1.00267605951749,1.),(1.,0.941599607549756,
1.),(1.,0.828238301901784,1.),(1.,0.787677905717196,1.),(1.,0.72655233398001,
1.),(1.,0.706675310150417,1.),(1.,0.707106781186548,1.)))
REPRESENTATION_ITEM('')
SURFACE()
) ;
#224=(
BOUNDED_SURFACE()
B_SPLINE_SURFACE(3,2,((#167045,#167046,#167047),(#167048,#167049,#167050),
(#167051,#167052,#167053),(#167054,#167055,#167056),(#167057,#167058,#167059),
(#167060,#167061,#167062),(#167063,#167064,#167065),(#167066,#167067,#167068)),
 .UNSPECIFIED.,.F.,.F.,.F.)
B_SPLINE_SURFACE_WITH_KNOTS((4,2,2,4),(3,3),(1.5707963267949,2.35619449019234,
2.74889357189107,3.14159265358979),(0.,1.),.UNSPECIFIED.)
GEOMETRIC_REPRESENTATION_ITEM()
RATIONAL_B_SPLINE_SURFACE(((1.,1.,1.),(1.,1.00267605951746,1.),(1.,0.941599607549799,
1.),(1.,0.828238301901763,1.),(1.,0.787677905717196,1.),(1.,0.72655233398001,
1.),(1.,0.706675310150416,1.),(1.,0.707106781186548,1.)))
REPRESENTATION_ITEM('')
SURFACE()
) ;
#225=(
BOUNDED_SURFACE()
B_SPLINE_SURFACE(3,2,((#167090,#167091,#167092),(#167093,#167094,#167095),
(#167096,#167097,#167098),(#167099,#167100,#167101),(#167102,#167103,#167104),
(#167105,#167106,#167107),(#167108,#167109,#167110),(#167111,#167112,#167113)),
 .UNSPECIFIED.,.F.,.F.,.F.)
B_SPLINE_SURFACE_WITH_KNOTS((4,2,2,4),(3,3),(4.71238898038469,5.49778714378214,
5.89048622548086,6.28318530717959),(0.,1.),.UNSPECIFIED.)
GEOMETRIC_REPRESENTATION_ITEM()
RATIONAL_B_SPLINE_SURFACE(((1.,1.,1.),(1.,1.00267605951749,1.),(1.,0.941599607549756,
1.),(1.,0.828238301901784,1.),(1.,0.787677905717196,1.),(1.,0.72655233398001,
1.),(1.,0.706675310150417,1.),(1.,0.707106781186548,1.)))
REPRESENTATION_ITEM('')
SURFACE()
) ;
#226=(
BOUNDED_SURFACE()
B_SPLINE_SURFACE(3,2,((#167114,#167115,#167116),(#167117,#167118,#167119),
(#167120,#167121,#167122),(#167123,#167124,#167125),(#167126,#167127,#167128),
(#167129,#167130,#167131),(#167132,#167133,#167134),(#167135,#167136,#167137)),
 .UNSPECIFIED.,.F.,.F.,.F.)
B_SPLINE_SURFACE_WITH_KNOTS((4,2,2,4),(3,3),(3.38657131671664,3.71802573263365,
4.04948014855067,4.71238898038469),(-0.000420825293764194,1.00042070189636),
 .UNSPECIFIED.)
GEOMETRIC_REPRESENTATION_ITEM()
RATIONAL_B_SPLINE_SURFACE(((1.00022935631194,0.727377552437947,1.00022928903016),
(1.00021435582396,0.745207756072161,1.00021429294259),(1.00019031909813,
0.773778807686912,1.00019026326795),(1.00013753194518,0.836523812240446,
1.00013749160012),(1.00010896374898,0.870481157937832,1.00010893178441),
(1.00003378452181,0.959842312830787,1.0000337746111),(0.999998875500004,
1.00133662744395,0.999998875829878),(1.,1.,1.)))
REPRESENTATION_ITEM('')
SURFACE()
) ;
#227=(
BOUNDED_SURFACE()
B_SPLINE_SURFACE(3,2,((#167139,#167140,#167141),(#167142,#167143,#167144),
(#167145,#167146,#167147),(#167148,#167149,#167150)),.UNSPECIFIED.,.F.,
 .F.,.F.)
B_SPLINE_SURFACE_WITH_KNOTS((4,4),(3,3),(1.32581766366803,1.5707963267949),
(0.,1.),.UNSPECIFIED.)
GEOMETRIC_REPRESENTATION_ITEM()
RATIONAL_B_SPLINE_SURFACE(((1.,0.727606875108994,1.),(1.,0.721005575721676,
1.),(1.,0.714109499479749,1.),(1.,0.707106781186548,1.)))
REPRESENTATION_ITEM('')
SURFACE()
) ;
#228=(
BOUNDED_SURFACE()
B_SPLINE_SURFACE(3,2,((#167166,#167167,#167168),(#167169,#167170,#167171),
(#167172,#167173,#167174),(#167175,#167176,#167177)),.UNSPECIFIED.,.F.,
 .F.,.F.)
B_SPLINE_SURFACE_WITH_KNOTS((4,4),(3,3),(3.92699081698722,4.71238898038469),
(0.,1.),.UNSPECIFIED.)
GEOMETRIC_REPRESENTATION_ITEM()
RATIONAL_B_SPLINE_SURFACE(((1.,0.866025403784442,1.),(1.,0.828363615049332,
1.),(1.,0.772698924407958,1.),(1.,0.707106781186545,1.)))
REPRESENTATION_ITEM('')
SURFACE()
) ;
#229=(
BOUNDED_SURFACE()
B_SPLINE_SURFACE(3,2,((#167179,#167180,#167181),(#167182,#167183,#167184),
(#167185,#167186,#167187),(#167188,#167189,#167190)),.UNSPECIFIED.,.F.,
 .F.,.F.)
B_SPLINE_SURFACE_WITH_KNOTS((4,4),(3,3),(1.5707963267949,2.35619449019233),
(0.,1.),.UNSPECIFIED.)
GEOMETRIC_REPRESENTATION_ITEM()
RATIONAL_B_SPLINE_SURFACE(((1.,1.,1.),(1.,1.00150544078213,1.),(1.,0.943158245625741,
1.),(1.,0.866025403784444,1.)))
REPRESENTATION_ITEM('')
SURFACE()
) ;
#230=(
BOUNDED_SURFACE()
B_SPLINE_SURFACE(3,2,((#167191,#167192,#167193),(#167194,#167195,#167196),
(#167197,#167198,#167199),(#167200,#167201,#167202)),.UNSPECIFIED.,.F.,
 .F.,.F.)
B_SPLINE_SURFACE_WITH_KNOTS((4,4),(3,3),(7.06858347057706,7.85398163397448),
(0.,1.),.UNSPECIFIED.)
GEOMETRIC_REPRESENTATION_ITEM()
RATIONAL_B_SPLINE_SURFACE(((1.,0.866025403784446,1.),(1.,0.943158245625744,
1.),(1.,1.00150544078213,1.),(1.,1.,1.)))
REPRESENTATION_ITEM('')
SURFACE()
) ;
#231=(
BOUNDED_SURFACE()
B_SPLINE_SURFACE(3,2,((#167204,#167205,#167206),(#167207,#167208,#167209),
(#167210,#167211,#167212),(#167213,#167214,#167215)),.UNSPECIFIED.,.F.,
 .F.,.F.)
B_SPLINE_SURFACE_WITH_KNOTS((4,4),(3,3),(1.5707963267949,2.35619449019237),
(0.,1.),.UNSPECIFIED.)
GEOMETRIC_REPRESENTATION_ITEM()
RATIONAL_B_SPLINE_SURFACE(((1.,0.707106781186545,1.),(1.,0.772698924407959,
1.),(1.,0.828363615049336,1.),(1.,0.86602540378444,1.)))
REPRESENTATION_ITEM('')
SURFACE()
) ;
#232=(
BOUNDED_SURFACE()
B_SPLINE_SURFACE(3,2,((#167231,#167232,#167233),(#167234,#167235,#167236),
(#167237,#167238,#167239),(#167240,#167241,#167242)),.UNSPECIFIED.,.F.,
 .F.,.F.)
B_SPLINE_SURFACE_WITH_KNOTS((4,4),(3,3),(4.71238898038469,4.95736764351155),
(0.,1.),.UNSPECIFIED.)
GEOMETRIC_REPRESENTATION_ITEM()
RATIONAL_B_SPLINE_SURFACE(((1.,0.707106781186548,1.),(1.,0.714109499479746,
1.),(1.,0.721005575721677,1.),(1.,0.727606875108994,1.)))
REPRESENTATION_ITEM('')
SURFACE()
) ;
#233=(
BOUNDED_SURFACE()
B_SPLINE_SURFACE(3,2,((#167244,#167245,#167246),(#167247,#167248,#167249),
(#167250,#167251,#167252),(#167253,#167254,#167255),(#167256,#167257,#167258),
(#167259,#167260,#167261),(#167262,#167263,#167264),(#167265,#167266,#167267)),
 .UNSPECIFIED.,.F.,.F.,.F.)
B_SPLINE_SURFACE_WITH_KNOTS((4,2,2,4),(3,3),(3.38657131671663,3.71802573263365,
4.04948014855066,4.71238898038469),(-0.00042082531042703,1.00042070189448),
 .UNSPECIFIED.)
GEOMETRIC_REPRESENTATION_ITEM()
RATIONAL_B_SPLINE_SURFACE(((1.00022935632103,0.727377552433915,1.00022928902914),
(1.00021435583246,0.745207756068348,1.00021429294162),(1.00019031910567,
0.773778807683621,1.00019026326709),(1.00013753195063,0.836523812237968,
1.00013749159951),(1.00010896375329,0.870481157935892,1.00010893178393),
(1.00003378452315,0.959842312830238,1.00003377461096),(0.99999887549996,
1.00133662744394,0.999998875829883),(1.,1.,1.)))
REPRESENTATION_ITEM('')
SURFACE()
) ;
#234=(
BOUNDED_SURFACE()
B_SPLINE_SURFACE(3,2,((#168899,#168900,#168901),(#168902,#168903,#168904),
(#168905,#168906,#168907),(#168908,#168909,#168910),(#168911,#168912,#168913),
(#168914,#168915,#168916),(#168917,#168918,#168919),(#168920,#168921,#168922),
(#168923,#168924,#168925),(#168926,#168927,#168928)),.UNSPECIFIED.,.F.,
 .F.,.F.)
B_SPLINE_SURFACE_WITH_KNOTS((4,2,2,2,4),(3,3),(-3.3881317890172E-21,5.50005871024831E-5,
0.000110001174204966,0.000165001761307449,0.000220002348409932),(-9.32574651119021E-5,
1.),.UNSPECIFIED.)
GEOMETRIC_REPRESENTATION_ITEM()
RATIONAL_B_SPLINE_SURFACE(((1.00005463405283,0.707079466707422,1.),(1.00005694771662,
0.694674755787659,1.),(1.00005645688428,0.697306353922547,1.),(1.00005591567353,
0.700208055939803,1.),(1.0000556235962,0.701774028840045,1.),(1.00005562454822,
0.70176892461066,1.),(1.00005591789343,0.70019615395662,1.),(1.00005645795057,
0.697300636998116,1.),(1.00005694973354,0.694663942070735,1.),(1.00005463405283,
0.707079466707408,1.)))
REPRESENTATION_ITEM('')
SURFACE()
) ;
#235=(
BOUNDED_SURFACE()
B_SPLINE_SURFACE(3,2,((#168933,#168934,#168935),(#168936,#168937,#168938),
(#168939,#168940,#168941),(#168942,#168943,#168944),(#168945,#168946,#168947),
(#168948,#168949,#168950),(#168951,#168952,#168953),(#168954,#168955,#168956),
(#168957,#168958,#168959),(#168960,#168961,#168962)),.UNSPECIFIED.,.F.,
 .F.,.F.)
B_SPLINE_SURFACE_WITH_KNOTS((4,2,2,2,4),(3,3),(-3.3881317890172E-21,5.50005871024829E-5,
0.000110001174204966,0.000165001761307449,0.000220002348409932),(0.,1.00009325746509),
 .UNSPECIFIED.)
GEOMETRIC_REPRESENTATION_ITEM()
RATIONAL_B_SPLINE_SURFACE(((1.,0.707079466707414,1.00005463405282),(1.,
0.694674755787651,1.00005694771661),(1.,0.697306353922573,1.00005645688426),
(1.,0.700208055939776,1.00005591567352),(1.,0.701774028840086,1.00005562359619),
(1.,0.701768924610626,1.0000556245482),(1.,0.700196153956618,1.00005591789341),
(1.,0.697300636998131,1.00005645795056),(1.,0.694663942070735,1.00005694973353),
(1.,0.707079466707415,1.00005463405282)))
REPRESENTATION_ITEM('')
SURFACE()
) ;
#236=(
BOUNDED_SURFACE()
B_SPLINE_SURFACE(3,2,((#168967,#168968,#168969),(#168970,#168971,#168972),
(#168973,#168974,#168975),(#168976,#168977,#168978),(#168979,#168980,#168981),
(#168982,#168983,#168984),(#168985,#168986,#168987),(#168988,#168989,#168990),
(#168991,#168992,#168993),(#168994,#168995,#168996)),.UNSPECIFIED.,.F.,
 .F.,.F.)
B_SPLINE_SURFACE_WITH_KNOTS((4,2,2,2,4),(3,3),(0.,5.5000587102484E-5,0.000110001174204968,
0.000165001761307452,0.000220002348409936),(-9.32574651108896E-5,1.),
 .UNSPECIFIED.)
GEOMETRIC_REPRESENTATION_ITEM()
RATIONAL_B_SPLINE_SURFACE(((1.00005463405283,0.707079466707377,1.),(1.00005694771662,
0.694674755787608,1.),(1.00005645688428,0.697306353922581,1.),(1.00005591567353,
0.700208055939738,1.),(1.0000556235962,0.7017740288401,1.),(1.00005562454822,
0.701768924610595,1.),(1.00005591789342,0.700196153956602,1.),(1.00005645795057,
0.697300636998131,1.),(1.00005694973354,0.694663942070724,1.),(1.00005463405283,
0.70707946670741,1.)))
REPRESENTATION_ITEM('')
SURFACE()
) ;
#237=(
BOUNDED_SURFACE()
B_SPLINE_SURFACE(3,2,((#169001,#169002,#169003),(#169004,#169005,#169006),
(#169007,#169008,#169009),(#169010,#169011,#169012),(#169013,#169014,#169015),
(#169016,#169017,#169018),(#169019,#169020,#169021),(#169022,#169023,#169024),
(#169025,#169026,#169027),(#169028,#169029,#169030)),.UNSPECIFIED.,.F.,
 .F.,.F.)
B_SPLINE_SURFACE_WITH_KNOTS((4,2,2,2,4),(3,3),(0.,5.5000587102483E-5,0.000110001174204966,
0.000165001761307449,0.000220002348409932),(0.,1.00009325746509),
 .UNSPECIFIED.)
GEOMETRIC_REPRESENTATION_ITEM()
RATIONAL_B_SPLINE_SURFACE(((1.,0.707079466707415,1.00005463405282),(1.,
0.694674755787641,1.00005694771661),(1.,0.697306353922585,1.00005645688426),
(1.,0.700208055939766,1.00005591567351),(1.,0.701774028840102,1.00005562359619),
(1.,0.701768924610621,1.0000556245482),(1.,0.700196153956564,1.00005591789341),
(1.,0.697300636998199,1.00005645795056),(1.,0.694663942070693,1.00005694973353),
(1.,0.707079466707429,1.00005463405282)))
REPRESENTATION_ITEM('')
SURFACE()
) ;
#238=(
BOUNDED_SURFACE()
B_SPLINE_SURFACE(3,2,((#169035,#169036,#169037),(#169038,#169039,#169040),
(#169041,#169042,#169043),(#169044,#169045,#169046),(#169047,#169048,#169049),
(#169050,#169051,#169052),(#169053,#169054,#169055),(#169056,#169057,#169058),
(#169059,#169060,#169061),(#169062,#169063,#169064)),.UNSPECIFIED.,.F.,
 .F.,.F.)
B_SPLINE_SURFACE_WITH_KNOTS((4,2,2,2,4),(3,3),(6.7762635780344E-21,5.50005871024835E-5,
0.000110001174204967,0.00016500176130745,0.000220002348409934),(-9.32574651090946E-5,
1.),.UNSPECIFIED.)
GEOMETRIC_REPRESENTATION_ITEM()
RATIONAL_B_SPLINE_SURFACE(((1.00005463405283,0.707079466707396,1.),(1.00005694771662,
0.694674755787625,1.),(1.00005645688428,0.697306353922589,1.),(1.00005591567353,
0.700208055939743,1.),(1.0000556235962,0.701774028840088,1.),(1.00005562454822,
0.701768924610605,1.),(1.00005591789342,0.700196153956601,1.),(1.00005645795057,
0.697300636998125,1.),(1.00005694973354,0.694663942070733,1.),(1.00005463405283,
0.707079466707409,1.)))
REPRESENTATION_ITEM('')
SURFACE()
) ;
#239=(
BOUNDED_SURFACE()
B_SPLINE_SURFACE(3,2,((#169069,#169070,#169071),(#169072,#169073,#169074),
(#169075,#169076,#169077),(#169078,#169079,#169080),(#169081,#169082,#169083),
(#169084,#169085,#169086),(#169087,#169088,#169089),(#169090,#169091,#169092),
(#169093,#169094,#169095),(#169096,#169097,#169098)),.UNSPECIFIED.,.F.,
 .F.,.F.)
B_SPLINE_SURFACE_WITH_KNOTS((4,2,2,2,4),(3,3),(3.3881317890172E-21,5.50005871024834E-5,
0.000110001174204967,0.00016500176130745,0.000220002348409934),(0.,1.00009325746519),
 .UNSPECIFIED.)
GEOMETRIC_REPRESENTATION_ITEM()
RATIONAL_B_SPLINE_SURFACE(((1.,0.707079466707384,1.00005463405288),(1.,
0.694674755787592,1.00005694771667),(1.,0.697306353922578,1.00005645688433),
(1.,0.700208055939709,1.00005591567358),(1.,0.701774028840076,1.00005562359625),
(1.,0.701768924610577,1.00005562454827),(1.,0.700196153956582,1.00005591789348),
(1.,0.697300636998093,1.00005645795062),(1.,0.694663942070696,1.00005694973359),
(1.,0.70707946670737,1.00005463405288)))
REPRESENTATION_ITEM('')
SURFACE()
) ;
#240=(
BOUNDED_SURFACE()
B_SPLINE_SURFACE(3,2,((#169103,#169104,#169105),(#169106,#169107,#169108),
(#169109,#169110,#169111),(#169112,#169113,#169114),(#169115,#169116,#169117),
(#169118,#169119,#169120),(#169121,#169122,#169123),(#169124,#169125,#169126),
(#169127,#169128,#169129),(#169130,#169131,#169132)),.UNSPECIFIED.,.F.,
 .F.,.F.)
B_SPLINE_SURFACE_WITH_KNOTS((4,2,2,2,4),(3,3),(-3.3881317890172E-21,5.50005871024834E-5,
0.000110001174204967,0.00016500176130745,0.000220002348409933),(-9.32574651049742E-5,
1.),.UNSPECIFIED.)
GEOMETRIC_REPRESENTATION_ITEM()
RATIONAL_B_SPLINE_SURFACE(((1.00005463405282,0.707079466707415,1.),(1.00005694771662,
0.694674755787666,1.),(1.00005645688427,0.697306353922507,1.),(1.00005591567352,
0.700208055939813,1.),(1.0000556235962,0.701774028840077,1.),(1.00005562454821,
0.701768924610621,1.),(1.00005591789342,0.700196153956683,1.),(1.00005645795056,
0.697300636998053,1.),(1.00005694973354,0.694663942070781,1.),(1.00005463405282,
0.707079466707411,1.)))
REPRESENTATION_ITEM('')
SURFACE()
) ;
#241=(
BOUNDED_SURFACE()
B_SPLINE_SURFACE(3,2,((#169137,#169138,#169139),(#169140,#169141,#169142),
(#169143,#169144,#169145),(#169146,#169147,#169148),(#169149,#169150,#169151),
(#169152,#169153,#169154),(#169155,#169156,#169157),(#169158,#169159,#169160),
(#169161,#169162,#169163),(#169164,#169165,#169166)),.UNSPECIFIED.,.F.,
 .F.,.F.)
B_SPLINE_SURFACE_WITH_KNOTS((4,2,2,2,4),(3,3),(3.3881317890172E-21,5.50005871024834E-5,
0.000110001174204967,0.00016500176130745,0.000220002348409934),(0.,1.00009325746519),
 .UNSPECIFIED.)
GEOMETRIC_REPRESENTATION_ITEM()
RATIONAL_B_SPLINE_SURFACE(((1.,0.707079466707385,1.00005463405287),(1.,
0.694674755787593,1.00005694771667),(1.,0.69730635392258,1.00005645688432),
(1.,0.70020805593971,1.00005591567357),(1.,0.701774028840128,1.00005562359625),
(1.,0.701768924610516,1.00005562454826),(1.,0.700196153956523,1.00005591789347),
(1.,0.697300636998155,1.00005645795062),(1.,0.694663942070652,1.00005694973359),
(1.,0.707079466707371,1.00005463405287)))
REPRESENTATION_ITEM('')
SURFACE()
) ;
#242=(
BOUNDED_SURFACE()
B_SPLINE_SURFACE(3,2,((#169171,#169172,#169173),(#169174,#169175,#169176),
(#169177,#169178,#169179),(#169180,#169181,#169182),(#169183,#169184,#169185),
(#169186,#169187,#169188),(#169189,#169190,#169191),(#169192,#169193,#169194),
(#169195,#169196,#169197),(#169198,#169199,#169200)),.UNSPECIFIED.,.F.,
 .F.,.F.)
B_SPLINE_SURFACE_WITH_KNOTS((4,2,2,2,4),(3,3),(-3.3881317890172E-21,5.50005871024834E-5,
0.000110001174204967,0.00016500176130745,0.000220002348409933),(-9.3257465103702E-5,
1.),.UNSPECIFIED.)
GEOMETRIC_REPRESENTATION_ITEM()
RATIONAL_B_SPLINE_SURFACE(((1.00005463405282,0.707079466707416,1.),(1.00005694771662,
0.694674755787666,1.),(1.00005645688427,0.697306353922507,1.),(1.00005591567352,
0.700208055939814,1.),(1.0000556235962,0.701774028840078,1.),(1.00005562454821,
0.701768924610622,1.),(1.00005591789342,0.700196153956684,1.),(1.00005645795056,
0.697300636998054,1.),(1.00005694973353,0.694663942070781,1.),(1.00005463405282,
0.707079466707412,1.)))
REPRESENTATION_ITEM('')
SURFACE()
) ;
#243=(
BOUNDED_SURFACE()
B_SPLINE_SURFACE(3,2,((#169205,#169206,#169207),(#169208,#169209,#169210),
(#169211,#169212,#169213),(#169214,#169215,#169216),(#169217,#169218,#169219),
(#169220,#169221,#169222),(#169223,#169224,#169225),(#169226,#169227,#169228),
(#169229,#169230,#169231),(#169232,#169233,#169234)),.UNSPECIFIED.,.F.,
 .F.,.F.)
B_SPLINE_SURFACE_WITH_KNOTS((4,2,2,2,4),(3,3),(3.3881317890172E-21,5.50005871024832E-5,
0.000110001174204966,0.00016500176130745,0.000220002348409933),(0.,1.00009325746505),
 .UNSPECIFIED.)
GEOMETRIC_REPRESENTATION_ITEM()
RATIONAL_B_SPLINE_SURFACE(((1.,0.707079466707425,1.00005463405279),(1.,
0.694674755787719,1.00005694771658),(1.,0.697306353922511,1.00005645688424),
(1.,0.700208055939858,1.00005591567349),(1.,0.701774028840035,1.00005562359617),
(1.,0.701768924610702,1.00005562454818),(1.,0.700196153956624,1.00005591789339),
(1.,0.697300636998136,1.00005645795053),(1.,0.694663942070728,1.0000569497335),
(1.,0.707079466707431,1.00005463405279)))
REPRESENTATION_ITEM('')
SURFACE()
) ;
#244=(
BOUNDED_SURFACE()
B_SPLINE_SURFACE(3,2,((#169239,#169240,#169241),(#169242,#169243,#169244),
(#169245,#169246,#169247),(#169248,#169249,#169250),(#169251,#169252,#169253),
(#169254,#169255,#169256),(#169257,#169258,#169259),(#169260,#169261,#169262),
(#169263,#169264,#169265),(#169266,#169267,#169268)),.UNSPECIFIED.,.F.,
 .F.,.F.)
B_SPLINE_SURFACE_WITH_KNOTS((4,2,2,2,4),(3,3),(-3.3881317890172E-21,5.50005871024834E-5,
0.000110001174204967,0.00016500176130745,0.000220002348409933),(-9.32574651063451E-5,
1.),.UNSPECIFIED.)
GEOMETRIC_REPRESENTATION_ITEM()
RATIONAL_B_SPLINE_SURFACE(((1.00005463405282,0.707079466707415,1.),(1.00005694771662,
0.694674755787663,1.),(1.00005645688427,0.697306353922506,1.),(1.00005591567352,
0.700208055939813,1.),(1.0000556235962,0.701774028840077,1.),(1.00005562454821,
0.701768924610621,1.),(1.00005591789342,0.700196153956578,1.),(1.00005645795057,
0.697300636998158,1.),(1.00005694973354,0.6946639420707,1.),(1.00005463405282,
0.707079466707411,1.)))
REPRESENTATION_ITEM('')
SURFACE()
) ;
#245=(
BOUNDED_SURFACE()
B_SPLINE_SURFACE(3,2,((#169273,#169274,#169275),(#169276,#169277,#169278),
(#169279,#169280,#169281),(#169282,#169283,#169284),(#169285,#169286,#169287),
(#169288,#169289,#169290),(#169291,#169292,#169293),(#169294,#169295,#169296),
(#169297,#169298,#169299),(#169300,#169301,#169302)),.UNSPECIFIED.,.F.,
 .F.,.F.)
B_SPLINE_SURFACE_WITH_KNOTS((4,2,2,2,4),(3,3),(3.3881317890172E-21,5.50005871024832E-5,
0.000110001174204966,0.00016500176130745,0.000220002348409933),(0.,1.00009325746505),
 .UNSPECIFIED.)
GEOMETRIC_REPRESENTATION_ITEM()
RATIONAL_B_SPLINE_SURFACE(((1.,0.707079466707427,1.00005463405279),(1.,
0.694674755787585,1.00005694771658),(1.,0.6973063539227,1.00005645688424),
(1.,0.700208055939672,1.00005591567349),(1.,0.70177402884015,1.00005562359616),
(1.,0.701768924610591,1.00005562454818),(1.,0.700196153956506,1.00005591789339),
(1.,0.697300636998258,1.00005645795053),(1.,0.694663942070653,1.0000569497335),
(1.,0.707079466707433,1.00005463405279)))
REPRESENTATION_ITEM('')
SURFACE()
) ;
#246=(
BOUNDED_SURFACE()
B_SPLINE_SURFACE(3,2,((#169307,#169308,#169309),(#169310,#169311,#169312),
(#169313,#169314,#169315),(#169316,#169317,#169318),(#169319,#169320,#169321),
(#169322,#169323,#169324),(#169325,#169326,#169327),(#169328,#169329,#169330),
(#169331,#169332,#169333),(#169334,#169335,#169336)),.UNSPECIFIED.,.F.,
 .F.,.F.)
B_SPLINE_SURFACE_WITH_KNOTS((4,2,2,2,4),(3,3),(-3.3881317890172E-21,5.50005871024834E-5,
0.000110001174204967,0.00016500176130745,0.000220002348409933),(-9.32574651063668E-5,
1.),.UNSPECIFIED.)
GEOMETRIC_REPRESENTATION_ITEM()
RATIONAL_B_SPLINE_SURFACE(((1.00005463405283,0.707079466707403,1.),(1.00005694771662,
0.694674755787773,1.),(1.00005645688427,0.697306353922386,1.),(1.00005591567352,
0.700208055939933,1.),(1.0000556235962,0.701774028840204,1.),(1.00005562454821,
0.701768924610519,1.),(1.00005591789342,0.700196153956681,1.),(1.00005645795057,
0.697300636998076,1.),(1.00005694973354,0.694663942070754,1.),(1.00005463405283,
0.707079466707411,1.)))
REPRESENTATION_ITEM('')
SURFACE()
) ;
#247=(
BOUNDED_SURFACE()
B_SPLINE_SURFACE(3,2,((#169341,#169342,#169343),(#169344,#169345,#169346),
(#169347,#169348,#169349),(#169350,#169351,#169352),(#169353,#169354,#169355),
(#169356,#169357,#169358),(#169359,#169360,#169361),(#169362,#169363,#169364),
(#169365,#169366,#169367),(#169368,#169369,#169370)),.UNSPECIFIED.,.F.,
 .F.,.F.)
B_SPLINE_SURFACE_WITH_KNOTS((4,2,2,2,4),(3,3),(3.3881317890172E-21,5.50005871024832E-5,
0.000110001174204966,0.00016500176130745,0.000220002348409933),(0.,1.00009325746505),
 .UNSPECIFIED.)
GEOMETRIC_REPRESENTATION_ITEM()
RATIONAL_B_SPLINE_SURFACE(((1.,0.707079466707425,1.00005463405279),(1.,
0.694674755787727,1.00005694771658),(1.,0.69730635392251,1.00005645688424),
(1.,0.700208055939857,1.00005591567349),(1.,0.701774028839934,1.00005562359617),
(1.,0.701768924610827,1.00005562454818),(1.,0.700196153956623,1.00005591789339),
(1.,0.697300636998135,1.00005645795053),(1.,0.694663942070729,1.0000569497335),
(1.,0.707079466707418,1.00005463405279)))
REPRESENTATION_ITEM('')
SURFACE()
) ;
#248=(
BOUNDED_SURFACE()
B_SPLINE_SURFACE(3,2,((#169375,#169376,#169377),(#169378,#169379,#169380),
(#169381,#169382,#169383),(#169384,#169385,#169386),(#169387,#169388,#169389),
(#169390,#169391,#169392),(#169393,#169394,#169395),(#169396,#169397,#169398),
(#169399,#169400,#169401),(#169402,#169403,#169404)),.UNSPECIFIED.,.F.,
 .F.,.F.)
B_SPLINE_SURFACE_WITH_KNOTS((4,2,2,2,4),(3,3),(-3.3881317890172E-21,5.50005871024821E-5,
0.000110001174204964,0.000165001761307446,0.000220002348409928),(-9.325746516207E-5,
1.),.UNSPECIFIED.)
GEOMETRIC_REPRESENTATION_ITEM()
RATIONAL_B_SPLINE_SURFACE(((1.00005463405286,0.707079466707472,1.),(1.00005694771665,
0.6946747557876,1.),(1.00005645688431,0.697306353922669,1.),(1.00005591567356,
0.700208055939717,1.),(1.00005562359623,0.701774028840023,1.),(1.00005562454825,
0.701768924610666,1.),(1.00005591789346,0.700196153956725,1.),(1.0000564579506,
0.697300636997996,1.),(1.00005694973357,0.694663942070795,1.),(1.00005463405286,
0.707079466707395,1.)))
REPRESENTATION_ITEM('')
SURFACE()
) ;
#249=(
BOUNDED_SURFACE()
B_SPLINE_SURFACE(3,2,((#169409,#169410,#169411),(#169412,#169413,#169414),
(#169415,#169416,#169417),(#169418,#169419,#169420),(#169421,#169422,#169423),
(#169424,#169425,#169426),(#169427,#169428,#169429),(#169430,#169431,#169432),
(#169433,#169434,#169435),(#169436,#169437,#169438)),.UNSPECIFIED.,.F.,
 .F.,.F.)
B_SPLINE_SURFACE_WITH_KNOTS((4,2,2,2,4),(3,3),(3.3881317890172E-21,5.50005871024832E-5,
0.000110001174204966,0.00016500176130745,0.000220002348409933),(0.,1.00009325746505),
 .UNSPECIFIED.)
GEOMETRIC_REPRESENTATION_ITEM()
RATIONAL_B_SPLINE_SURFACE(((1.,0.707079466707427,1.00005463405279),(1.,
0.694674755787857,1.00005694771658),(1.,0.697306353922324,1.00005645688424),
(1.,0.700208055940047,1.00005591567349),(1.,0.701774028839924,1.00005562359616),
(1.,0.701768924610816,1.00005562454818),(1.,0.700196153956747,1.00005591789339),
(1.,0.697300636998016,1.00005645795053),(1.,0.694663942070808,1.0000569497335),
(1.,0.707079466707432,1.00005463405279)))
REPRESENTATION_ITEM('')
SURFACE()
) ;
#250=(
BOUNDED_SURFACE()
B_SPLINE_SURFACE(3,2,((#169443,#169444,#169445),(#169446,#169447,#169448),
(#169449,#169450,#169451),(#169452,#169453,#169454),(#169455,#169456,#169457),
(#169458,#169459,#169460),(#169461,#169462,#169463),(#169464,#169465,#169466),
(#169467,#169468,#169469),(#169470,#169471,#169472)),.UNSPECIFIED.,.F.,
 .F.,.F.)
B_SPLINE_SURFACE_WITH_KNOTS((4,2,2,2,4),(3,3),(-3.3881317890172E-21,5.50005871024821E-5,
0.000110001174204964,0.000165001761307446,0.000220002348409928),(-9.32574651622988E-5,
1.),.UNSPECIFIED.)
GEOMETRIC_REPRESENTATION_ITEM()
RATIONAL_B_SPLINE_SURFACE(((1.00005463405286,0.707079466707472,1.),(1.00005694771665,
0.6946747557876,1.),(1.00005645688431,0.697306353922669,1.),(1.00005591567356,
0.700208055939717,1.),(1.00005562359623,0.701774028840023,1.),(1.00005562454825,
0.701768924610666,1.),(1.00005591789346,0.700196153956725,1.),(1.0000564579506,
0.697300636997996,1.),(1.00005694973357,0.694663942070795,1.),(1.00005463405286,
0.707079466707394,1.)))
REPRESENTATION_ITEM('')
SURFACE()
) ;
#251=(
BOUNDED_SURFACE()
B_SPLINE_SURFACE(3,2,((#169477,#169478,#169479),(#169480,#169481,#169482),
(#169483,#169484,#169485),(#169486,#169487,#169488),(#169489,#169490,#169491),
(#169492,#169493,#169494),(#169495,#169496,#169497),(#169498,#169499,#169500),
(#169501,#169502,#169503),(#169504,#169505,#169506)),.UNSPECIFIED.,.F.,
 .F.,.F.)
B_SPLINE_SURFACE_WITH_KNOTS((4,2,2,2,4),(3,3),(0.,5.50005871024826E-5,0.000110001174204965,
0.000165001761307448,0.00022000234840993),(0.,1.00009325746516),
 .UNSPECIFIED.)
GEOMETRIC_REPRESENTATION_ITEM()
RATIONAL_B_SPLINE_SURFACE(((1.,0.707079466707393,1.00005463405286),(1.,
0.6946747557876,1.00005694771665),(1.,0.697306353922587,1.00005645688431),
(1.,0.700208055939715,1.00005591567356),(1.,0.701774028840065,1.00005562359623),
(1.,0.701768924610603,1.00005562454825),(1.,0.700196153956427,1.00005591789346),
(1.,0.697300636998359,1.0000564579506),(1.,0.694663942070582,1.00005694973357),
(1.,0.707079466707472,1.00005463405286)))
REPRESENTATION_ITEM('')
SURFACE()
) ;
#252=(
BOUNDED_SURFACE()
B_SPLINE_SURFACE(3,2,((#169610,#169611,#169612),(#169613,#169614,#169615),
(#169616,#169617,#169618),(#169619,#169620,#169621),(#169622,#169623,#169624),
(#169625,#169626,#169627),(#169628,#169629,#169630),(#169631,#169632,#169633),
(#169634,#169635,#169636),(#169637,#169638,#169639)),.UNSPECIFIED.,.F.,
 .F.,.F.)
B_SPLINE_SURFACE_WITH_KNOTS((4,2,2,2,4),(3,3),(-8.470329472543E-22,1.20923255006762E-5,
2.41846510013524E-5,4.83693020027048E-5,9.67386040054096E-5),(-0.000804444758851847,
1.00077659724948),.UNSPECIFIED.)
GEOMETRIC_REPRESENTATION_ITEM()
RATIONAL_B_SPLINE_SURFACE(((1.00092876437359,0.422280884438106,1.00089658833676),
(1.00092908313811,0.422082603407448,1.00089689605803),(1.00086201767711,
0.46379931855613,1.00083215400736),(1.00071445154572,0.555589849432173,
1.00068970014494),(1.00063665558035,0.603981258051229,1.00061459933661),
(1.00042751802664,0.734071048305621,1.00041270712717),(1.00031984666358,
0.801045844505129,1.00030876592199),(1.0000701654339,0.956355009333009,
1.00006773462836),(1.00000277537655,0.998273633088197,1.00000267922663),
(1.,1.,1.)))
REPRESENTATION_ITEM('')
SURFACE()
) ;
#253=(
BOUNDED_SURFACE()
B_SPLINE_SURFACE(3,2,((#169641,#169642,#169643),(#169644,#169645,#169646),
(#169647,#169648,#169649),(#169650,#169651,#169652),(#169653,#169654,#169655),
(#169656,#169657,#169658),(#169659,#169660,#169661),(#169662,#169663,#169664),
(#169665,#169666,#169667),(#169668,#169669,#169670)),.UNSPECIFIED.,.F.,
 .F.,.F.)
B_SPLINE_SURFACE_WITH_KNOTS((4,2,2,2,4),(3,3),(0.,9.64580201362678E-6,1.92916040272536E-5,
3.85832080545071E-5,7.71664161090142E-5),(-0.000370411631943625,1.00037041163331),
 .UNSPECIFIED.)
GEOMETRIC_REPRESENTATION_ITEM()
RATIONAL_B_SPLINE_SURFACE(((1.00032019601253,0.567623377417556,1.00032019601371),
(1.00032045653552,0.567271580252903,1.0003204565367),(1.00030818786187,
0.583838581291787,1.00030818786301),(1.00027173235979,0.63306626136058,
1.0002717323608),(1.00024819709674,0.664847099196012,1.00024819709766),
(1.00017892209811,0.758392579986913,1.00017892209877),(1.000134718753,0.818082558353675,
1.0001347187535),(1.00003314780627,0.955238866321452,1.00003314780639),
(0.999999834267815,1.00022379642419,0.999999834267814),(1.,1.,1.)))
REPRESENTATION_ITEM('')
SURFACE()
) ;
#254=(
BOUNDED_SURFACE()
B_SPLINE_SURFACE(3,2,((#169672,#169673,#169674),(#169675,#169676,#169677),
(#169678,#169679,#169680),(#169681,#169682,#169683),(#169684,#169685,#169686),
(#169687,#169688,#169689),(#169690,#169691,#169692),(#169693,#169694,#169695),
(#169696,#169697,#169698),(#169699,#169700,#169701)),.UNSPECIFIED.,.F.,
 .F.,.F.)
B_SPLINE_SURFACE_WITH_KNOTS((4,2,2,2,4),(3,3),(0.,9.64580201362836E-6,1.92916040272567E-5,
3.85832080545134E-5,7.71664161090269E-5),(-0.000370411633304617,1.00037041163335),
 .UNSPECIFIED.)
GEOMETRIC_REPRESENTATION_ITEM()
RATIONAL_B_SPLINE_SURFACE(((1.0003201960137,0.56762337741697,1.00032019601374),
(1.00032045653669,0.567271580252287,1.00032045653673),(1.00030818786301,
0.583838581291198,1.00030818786303),(1.00027173236079,0.633066261360079,
1.00027173236081),(1.00024819709765,0.664847099195498,1.00024819709767),
(1.00017892209876,0.758392579986697,1.00017892209878),(1.0001347187535,
0.818082558353415,1.00013471875351),(1.00003314780639,0.955238866321388,
1.00003314780639),(0.999999834267815,1.0002237964242,0.999999834267813),
(1.,1.,1.)))
REPRESENTATION_ITEM('')
SURFACE()
) ;
#255=(
BOUNDED_SURFACE()
B_SPLINE_SURFACE(3,2,((#169703,#169704,#169705),(#169706,#169707,#169708),
(#169709,#169710,#169711),(#169712,#169713,#169714),(#169715,#169716,#169717),
(#169718,#169719,#169720),(#169721,#169722,#169723),(#169724,#169725,#169726),
(#169727,#169728,#169729),(#169730,#169731,#169732)),.UNSPECIFIED.,.F.,
 .F.,.F.)
B_SPLINE_SURFACE_WITH_KNOTS((4,2,2,2,4),(3,3),(0.,9.64580201362833E-6,1.92916040272567E-5,
3.85832080545133E-5,7.71664161090267E-5),(-0.000370411633799105,1.00037041163132),
 .UNSPECIFIED.)
GEOMETRIC_REPRESENTATION_ITEM()
RATIONAL_B_SPLINE_SURFACE(((1.00032019601413,0.567623377417628,1.00032019601199),
(1.00032045653712,0.567271580252937,1.00032045653497),(1.00030818786341,
0.583838581291844,1.00030818786135),(1.00027173236115,0.63306626136063,
1.00027173235934),(1.00024819709798,0.66484709919601,1.00024819709632),
(1.000178922099,0.758392579987061,1.0001789220978),(1.00013471875369,0.818082558353688,
1.00013471875278),(1.00003314780643,0.955238866321459,1.00003314780621),
(0.999999834267814,1.00022379642419,0.999999834267815),(1.,1.,1.)))
REPRESENTATION_ITEM('')
SURFACE()
) ;
#256=(
BOUNDED_SURFACE()
B_SPLINE_SURFACE(3,2,((#169734,#169735,#169736),(#169737,#169738,#169739),
(#169740,#169741,#169742),(#169743,#169744,#169745),(#169746,#169747,#169748),
(#169749,#169750,#169751),(#169752,#169753,#169754),(#169755,#169756,#169757),
(#169758,#169759,#169760),(#169761,#169762,#169763)),.UNSPECIFIED.,.F.,
 .F.,.F.)
B_SPLINE_SURFACE_WITH_KNOTS((4,2,2,2,4),(3,3),(-4.25210539521659E-19,9.64580201362817E-6,
1.92916040272568E-5,3.8583208054514E-5,7.71664161090284E-5),(-0.00037041163343029,
1.00037041163324),.UNSPECIFIED.)
GEOMETRIC_REPRESENTATION_ITEM()
RATIONAL_B_SPLINE_SURFACE(((1.00032019601381,0.567623377416959,1.00032019601364),
(1.0003204565368,0.56727158025228,1.00032045653663),(1.00030818786311,0.583838581291188,
1.00030818786295),(1.00027173236089,0.633066261360063,1.00027173236074),
(1.00024819709774,0.664847099195502,1.00024819709761),(1.00017892209882,
0.758392579986709,1.00017892209873),(1.00013471875355,0.818082558353424,
1.00013471875348),(1.0000331478064,0.955238866321397,1.00003314780639),
(0.999999834267814,1.00022379642418,0.999999834267814),(1.,1.,1.)))
REPRESENTATION_ITEM('')
SURFACE()
) ;
#257=(
BOUNDED_SURFACE()
B_SPLINE_SURFACE(3,2,((#169765,#169766,#169767),(#169768,#169769,#169770),
(#169771,#169772,#169773),(#169774,#169775,#169776),(#169777,#169778,#169779),
(#169780,#169781,#169782),(#169783,#169784,#169785),(#169786,#169787,#169788),
(#169789,#169790,#169791),(#169792,#169793,#169794)),.UNSPECIFIED.,.F.,
 .F.,.F.)
B_SPLINE_SURFACE_WITH_KNOTS((4,2,2,2,4),(3,3),(-4.25210539521659E-19,9.64580201362817E-6,
1.92916040272568E-5,3.8583208054514E-5,7.71664161090284E-5),(-0.000370411633405951,
1.00037041163366),.UNSPECIFIED.)
GEOMETRIC_REPRESENTATION_ITEM()
RATIONAL_B_SPLINE_SURFACE(((1.00032019601379,0.567623377416788,1.00032019601401),
(1.00032045653678,0.567271580252109,1.00032045653699),(1.00030818786309,
0.583838581291024,1.0003081878633),(1.00027173236087,0.633066261359918,
1.00027173236105),(1.00024819709772,0.66484709919537,1.00024819709789),
(1.00017892209881,0.758392579986613,1.00017892209894),(1.00013471875354,
0.818082558353352,1.00013471875363),(1.0000331478064,0.955238866321379,
1.00003314780643),(0.999999834267814,1.00022379642418,0.999999834267814),
(1.,1.,1.)))
REPRESENTATION_ITEM('')
SURFACE()
) ;
#258=(
BOUNDED_SURFACE()
B_SPLINE_SURFACE(3,2,((#169796,#169797,#169798),(#169799,#169800,#169801),
(#169802,#169803,#169804),(#169805,#169806,#169807),(#169808,#169809,#169810),
(#169811,#169812,#169813),(#169814,#169815,#169816),(#169817,#169818,#169819),
(#169820,#169821,#169822),(#169823,#169824,#169825)),.UNSPECIFIED.,.F.,
 .F.,.F.)
B_SPLINE_SURFACE_WITH_KNOTS((4,2,2,2,4),(3,3),(-8.92772726406033E-19,9.64580201362776E-6,
1.92916040272564E-5,3.85832080545137E-5,7.71664161090283E-5),(-0.000370411626210755,
1.00037041164027),.UNSPECIFIED.)
GEOMETRIC_REPRESENTATION_ITEM()
RATIONAL_B_SPLINE_SURFACE(((1.00032019600757,0.567623377417044,1.00032019601972),
(1.00032045653055,0.567271580252367,1.00032045654271),(1.0003081878571,
0.583838581291261,1.0003081878688),(1.00027173235558,0.633066261360144,
1.0002717323659),(1.0002481970929,0.664847099195559,1.00024819710231),(1.00017892209533,
0.758392579986733,1.00017892210213),(1.00013471875092,0.818082558353452,
1.00013471875604),(1.00003314780575,0.955238866321398,1.00003314780701),
(0.999999834267817,1.00022379642419,0.99999983426781),(1.,1.,1.)))
REPRESENTATION_ITEM('')
SURFACE()
) ;
#259=(
BOUNDED_SURFACE()
B_SPLINE_SURFACE(3,2,((#169827,#169828,#169829),(#169830,#169831,#169832),
(#169833,#169834,#169835),(#169836,#169837,#169838),(#169839,#169840,#169841),
(#169842,#169843,#169844),(#169845,#169846,#169847),(#169848,#169849,#169850),
(#169851,#169852,#169853),(#169854,#169855,#169856)),.UNSPECIFIED.,.F.,
 .F.,.F.)
B_SPLINE_SURFACE_WITH_KNOTS((4,2,2,2,4),(3,3),(0.,9.64580201362838E-6,1.92916040272568E-5,
3.85832080545135E-5,7.71664161090271E-5),(-0.000370411640884523,1.00037041162619),
 .UNSPECIFIED.)
GEOMETRIC_REPRESENTATION_ITEM()
RATIONAL_B_SPLINE_SURFACE(((1.00032019602025,0.567623377416787,1.00032019600755),
(1.00032045654325,0.567271580252103,1.00032045653053),(1.00030818786931,
0.58383858129102,1.00030818785708),(1.00027173236636,0.633066261359912,
1.00027173235557),(1.00024819710274,0.66484709919538,1.00024819709289),
(1.00017892210243,0.758392579986544,1.00017892209533),(1.00013471875626,
0.81808255835334,1.00013471875092),(1.00003314780707,0.955238866321376,
1.00003314780575),(0.99999983426781,1.00022379642419,0.999999834267817),
(1.,1.,1.)))
REPRESENTATION_ITEM('')
SURFACE()
) ;
#260=(
BOUNDED_SURFACE()
B_SPLINE_SURFACE(3,2,((#169858,#169859,#169860),(#169861,#169862,#169863),
(#169864,#169865,#169866),(#169867,#169868,#169869),(#169870,#169871,#169872),
(#169873,#169874,#169875),(#169876,#169877,#169878),(#169879,#169880,#169881),
(#169882,#169883,#169884),(#169885,#169886,#169887)),.UNSPECIFIED.,.F.,
 .F.,.F.)
B_SPLINE_SURFACE_WITH_KNOTS((4,2,2,2,4),(3,3),(0.,9.64580201362832E-6,1.92916040272566E-5,
3.85832080545133E-5,7.71664161090265E-5),(-0.000370411633605454,1.00037041163324),
 .UNSPECIFIED.)
GEOMETRIC_REPRESENTATION_ITEM()
RATIONAL_B_SPLINE_SURFACE(((1.00032019601396,0.567623377416892,1.00032019601364),
(1.00032045653695,0.567271580252197,1.00032045653663),(1.00030818786325,
0.583838581291129,1.00030818786294),(1.00027173236101,0.633066261360012,
1.00027173236073),(1.00024819709786,0.664847099195459,1.00024819709761),
(1.00017892209891,0.758392579986615,1.00017892209872),(1.00013471875361,
0.8180825583534,1.00013471875347),(1.00003314780642,0.955238866321366,1.00003314780638),
(0.999999834267813,1.0002237964242,0.999999834267813),(1.,1.,1.)))
REPRESENTATION_ITEM('')
SURFACE()
) ;
#261=(
BOUNDED_SURFACE()
B_SPLINE_SURFACE(3,2,((#169893,#169894,#169895),(#169896,#169897,#169898),
(#169899,#169900,#169901),(#169902,#169903,#169904),(#169905,#169906,#169907),
(#169908,#169909,#169910),(#169911,#169912,#169913),(#169914,#169915,#169916),
(#169917,#169918,#169919),(#169920,#169921,#169922)),.UNSPECIFIED.,.F.,
 .F.,.F.)
B_SPLINE_SURFACE_WITH_KNOTS((4,2,2,2,4),(3,3),(0.,9.6458020136283E-6,1.92916040272566E-5,
3.85832080545132E-5,7.71664161090264E-5),(-0.000370411633385564,1.00037041163303),
 .UNSPECIFIED.)
GEOMETRIC_REPRESENTATION_ITEM()
RATIONAL_B_SPLINE_SURFACE(((1.00032019601377,0.567623377417072,1.00032019601346),
(1.00032045653676,0.567271580252374,1.00032045653645),(1.00030818786307,
0.58383858129131,1.00030818786277),(1.00027173236085,0.633066261360156,
1.00027173236059),(1.00024819709771,0.664847099195593,1.00024819709747),
(1.0001789220988,0.758392579986717,1.00017892209863),(1.00013471875353,
0.81808255835345,1.0001347187534),(1.0000331478064,0.955238866321428,1.00003314780636),
(0.999999834267813,1.00022379642417,0.999999834267814),(1.,1.,1.)))
REPRESENTATION_ITEM('')
SURFACE()
) ;
#262=(
BOUNDED_SURFACE()
B_SPLINE_SURFACE(3,2,((#169928,#169929,#169930),(#169931,#169932,#169933),
(#169934,#169935,#169936),(#169937,#169938,#169939),(#169940,#169941,#169942),
(#169943,#169944,#169945),(#169946,#169947,#169948),(#169949,#169950,#169951),
(#169952,#169953,#169954),(#169955,#169956,#169957)),.UNSPECIFIED.,.F.,
 .F.,.F.)
B_SPLINE_SURFACE_WITH_KNOTS((4,2,2,2,4),(3,3),(-4.26904605416167E-19,1.20923255006779E-5,
2.41846510013563E-5,4.8369302002713E-5,9.67386040054264E-5),(-0.000768510511548604,
1.00084741984056),.UNSPECIFIED.)
GEOMETRIC_REPRESENTATION_ITEM()
RATIONAL_B_SPLINE_SURFACE(((1.00088724495747,0.422260730021251,1.00097842287518),
(1.00088754947197,0.422062442073261,1.00097875868317),(1.00082348210054,
0.463780612559125,1.00090810741463),(1.00068251275493,0.555574345656711,
1.00075265132409),(1.00060819457483,0.603967442467466,1.00067069582031),
(1.00040840629136,0.734061771058594,1.0004503762512),(1.00030554826122,
0.801038903753378,1.00033694799359),(1.00006702876336,0.95635348672563,
1.00007391698856),(1.00000265130631,0.9982735728619,1.00000292376837),(1.,
1.,1.)))
REPRESENTATION_ITEM('')
SURFACE()
) ;
#263=(
BOUNDED_SURFACE()
B_SPLINE_SURFACE(3,2,((#170041,#170042,#170043),(#170044,#170045,#170046),
(#170047,#170048,#170049),(#170050,#170051,#170052),(#170053,#170054,#170055),
(#170056,#170057,#170058),(#170059,#170060,#170061),(#170062,#170063,#170064)),
 .UNSPECIFIED.,.F.,.F.,.F.)
B_SPLINE_SURFACE_WITH_KNOTS((4,2,2,4),(3,3),(3.40064005737571,3.72857728812795,
4.0565145188802,4.71238898038469),(0.,1.00035627873587),.UNSPECIFIED.)
GEOMETRIC_REPRESENTATION_ITEM()
RATIONAL_B_SPLINE_SURFACE(((1.,0.571144599242878,1.00030558412011),(1.,
0.605472570854249,1.00028112346745),(1.,0.655758245054346,1.00024529203457),
(1.,0.758559230914953,1.000172040424),(1.,0.810907017329345,1.00013473961766),
(1.,0.944519775683756,1.00003953284837),(1.,1.00147328708535,0.999998950198279),
(1.,1.,1.)))
REPRESENTATION_ITEM('')
SURFACE()
) ;
#264=(
BOUNDED_SURFACE()
B_SPLINE_SURFACE(3,2,((#170066,#170067,#170068),(#170069,#170070,#170071),
(#170072,#170073,#170074),(#170075,#170076,#170077)),.UNSPECIFIED.,.F.,
 .F.,.F.)
B_SPLINE_SURFACE_WITH_KNOTS((4,4),(3,3),(0.000567067675011747,0.00061979582196747),
(0.,1.),.UNSPECIFIED.)
GEOMETRIC_REPRESENTATION_ITEM()
RATIONAL_B_SPLINE_SURFACE(((1.,0.571297336894462,1.),(1.,0.558391514685631,
1.),(1.,0.550506809043631,1.),(1.,0.550571663591217,1.)))
REPRESENTATION_ITEM('')
SURFACE()
) ;
#265=(
BOUNDED_SURFACE()
B_SPLINE_SURFACE(3,2,((#170078,#170079,#170080),(#170081,#170082,#170083),
(#170084,#170085,#170086),(#170087,#170088,#170089),(#170090,#170091,#170092),
(#170093,#170094,#170095),(#170096,#170097,#170098),(#170099,#170100,#170101)),
 .UNSPECIFIED.,.F.,.F.,.F.)
B_SPLINE_SURFACE_WITH_KNOTS((4,2,2,4),(3,3),(6.54223271101527,6.87016994175507,
7.19810717249488,7.85398163397448),(-0.000356360340643563,1.00035627873694),
 .UNSPECIFIED.)
GEOMETRIC_REPRESENTATION_ITEM()
RATIONAL_B_SPLINE_SURFACE(((1.00030565413832,0.570991717771645,1.00030558412101),
(1.00028118788101,0.605331926871258,1.00028112346828),(1.00024534823811,
0.655635527273589,1.0002452920353),(1.00017207984346,0.758473160372548,
1.0001720404245),(1.00013477049042,0.810839608102769,1.00013473961805),
(1.00003954190649,0.944499997695579,1.00003953284848),(0.999998949957739,
1.00147381229284,0.999998950198277),(1.,1.,1.)))
REPRESENTATION_ITEM('')
SURFACE()
) ;
#266=(
BOUNDED_SURFACE()
B_SPLINE_SURFACE(3,2,((#170103,#170104,#170105),(#170106,#170107,#170108),
(#170109,#170110,#170111),(#170112,#170113,#170114)),.UNSPECIFIED.,.F.,
 .F.,.F.)
B_SPLINE_SURFACE_WITH_KNOTS((4,4),(3,3),(0.000567067675015788,0.000619795821981054),
(0.,1.00004537587559),.UNSPECIFIED.)
GEOMETRIC_REPRESENTATION_ITEM()
RATIONAL_B_SPLINE_SURFACE(((1.,0.571277884142694,1.00003890728278),(1.,
0.558371476316907,1.0000400785619),(1.,0.55048641289642,1.00004079414521),
(1.,0.550551270386939,1.00004078825928)))
REPRESENTATION_ITEM('')
SURFACE()
) ;
#367=ELLIPSE('',#98719,0.113705760628021,0.0999999999999901) ;
#368=ELLIPSE('',#98720,0.149345237620599,0.0999999999999305) ;
#369=ELLIPSE('',#98721,0.149345237620645,0.0999999999999468) ;
#370=ELLIPSE('',#98722,0.113705760627924,0.0999999999999499) ;
#371=ELLIPSE('',#98829,0.37480415029708,0.108393547954855) ;
#372=ELLIPSE('',#98830,0.293533022904216,0.0776808743108713) ;
#373=ELLIPSE('',#98841,0.0594417542785182,0.0546700434940687) ;
#374=ELLIPSE('',#98843,0.335126724531724,0.0994337530748851) ;
#375=ELLIPSE('',#98844,0.35994804660384,0.105243435885102) ;
#376=ELLIPSE('',#98845,0.108850968875591,0.0580464239932984) ;
#377=ELLIPSE('',#98864,0.0629103936951647,0.0573206382682852) ;
#378=ELLIPSE('',#98870,0.335126724504839,0.0994337530612308) ;
#379=ELLIPSE('',#98871,0.359948046537181,0.105243435873707) ;
#380=ELLIPSE('',#98875,0.0702807513773626,0.0453069706635111) ;
#381=ELLIPSE('',#98876,0.359930277252907,0.105237474483862) ;
#382=ELLIPSE('',#98877,0.335173749742838,0.0994597385892411) ;
#383=ELLIPSE('',#99074,0.111803398874898,0.0999999999999263) ;
#384=ELLIPSE('',#99089,0.111803398874933,0.0999999999999485) ;
#385=ELLIPSE('',#99211,0.113705760627989,0.0999999999999707) ;
#386=ELLIPSE('',#99212,0.149345237619608,0.0999999999995642) ;
#387=ELLIPSE('',#99213,0.149345237620654,0.0999999999999208) ;
#388=ELLIPSE('',#99214,0.113705760628105,0.100000000000041) ;
#389=ELLIPSE('',#99220,0.113705760628277,0.100000000000111) ;
#390=ELLIPSE('',#99221,0.149345237618997,0.0999999999993761) ;
#391=ELLIPSE('',#99222,0.149345237620065,0.0999999999997663) ;
#392=ELLIPSE('',#99223,0.113705760628311,0.100000000000123) ;
#393=ELLIPSE('',#99229,0.113705760628234,0.100000000000072) ;
#394=ELLIPSE('',#99230,0.149345237619401,0.0999999999995206) ;
#395=ELLIPSE('',#99231,0.149345237620857,0.100000000000031) ;
#396=ELLIPSE('',#99232,0.113705760627957,0.0999999999999554) ;
#397=ELLIPSE('',#99238,0.113705760628047,0.100000000000004) ;
#398=ELLIPSE('',#99239,0.149345237619215,0.0999999999994726) ;
#399=ELLIPSE('',#99240,0.14934523762126,0.10000000000015) ;
#400=ELLIPSE('',#99241,0.113705760628205,0.100000000000077) ;
#401=ELLIPSE('',#99247,0.113705760628038,0.0999999999999974) ;
#402=ELLIPSE('',#99248,0.149345237619726,0.0999999999996396) ;
#403=ELLIPSE('',#99249,0.149345237619801,0.0999999999996606) ;
#404=ELLIPSE('',#99250,0.11370576062794,0.0999999999999675) ;
#405=ELLIPSE('',#99256,0.113705760628114,0.100000000000042) ;
#406=ELLIPSE('',#99257,0.149345237621322,0.100000000000178) ;
#407=ELLIPSE('',#99258,0.14934523761991,0.0999999999997026) ;
#408=ELLIPSE('',#99259,0.113705760627855,0.0999999999999047) ;
#409=ELLIPSE('',#99265,0.113705760627948,0.099999999999958) ;
#410=ELLIPSE('',#99266,0.149345237620904,0.100000000000041) ;
#411=ELLIPSE('',#99267,0.149345237620801,0.100000000000004) ;
#412=ELLIPSE('',#99268,0.113705760627834,0.0999999999999106) ;
#413=ELLIPSE('',#99274,0.113705760628053,0.100000000000007) ;
#414=ELLIPSE('',#99275,0.149345237620591,0.0999999999999292) ;
#415=ELLIPSE('',#99276,0.149345237621263,0.100000000000161) ;
#416=ELLIPSE('',#99277,0.113705760627995,0.0999999999999786) ;
#417=ELLIPSE('',#99283,0.113705760627941,0.0999999999999602) ;
#418=ELLIPSE('',#99284,0.149345237620714,0.0999999999999713) ;
#419=ELLIPSE('',#99285,0.149345237620732,0.0999999999999782) ;
#420=ELLIPSE('',#99286,0.113705760627987,0.0999999999999783) ;
#421=ELLIPSE('',#99291,0.180453309435584,0.153056323384521) ;
#422=ELLIPSE('',#99292,0.180453309425237,0.153056323367989) ;
#423=ELLIPSE('',#99294,0.18045330947415,0.153056323451711) ;
#424=ELLIPSE('',#99295,0.180453309589905,0.153056323648943) ;
#425=ELLIPSE('',#99297,0.180453309654479,0.153056323758989) ;
#426=ELLIPSE('',#99298,0.180453309391707,0.15305632331313) ;
#427=ELLIPSE('',#99300,0.180453309365101,0.153056323267468) ;
#428=ELLIPSE('',#99301,0.180453309556384,0.153056323594097) ;
#429=ELLIPSE('',#99303,0.180453309198145,0.153056322983094) ;
#430=ELLIPSE('',#99304,0.180453309480796,0.153056323464846) ;
#431=ELLIPSE('',#99306,0.180453309173328,0.153056322941511) ;
#432=ELLIPSE('',#99307,0.180453309202449,0.153056322990444) ;
#433=ELLIPSE('',#99309,0.180453309242158,0.153056323057428) ;
#434=ELLIPSE('',#99310,0.180453309451238,0.153056323414422) ;
#435=ELLIPSE('',#99312,0.180453309481229,0.153056323465124) ;
#436=ELLIPSE('',#99313,0.180453309451544,0.153056323414031) ;
#437=ELLIPSE('',#99316,0.25539026404391,0.166311404124396) ;
#438=ELLIPSE('',#99317,0.255390264039982,0.166311404121025) ;
#439=ELLIPSE('',#99319,0.255390264047263,0.166311404128388) ;
#440=ELLIPSE('',#99320,0.255390264044952,0.166311404125431) ;
#441=ELLIPSE('',#99322,0.255390264049319,0.166311404131415) ;
#442=ELLIPSE('',#99323,0.255390264043609,0.166311404123759) ;
#443=ELLIPSE('',#99325,0.255390264047487,0.166311404129269) ;
#444=ELLIPSE('',#99326,0.255390264041227,0.166311404120253) ;
#445=ELLIPSE('',#99328,0.255390264048306,0.166311404130063) ;
#446=ELLIPSE('',#99329,0.255390264042795,0.166311404122152) ;
#447=ELLIPSE('',#99331,0.255390264044007,0.166311404124825) ;
#448=ELLIPSE('',#99332,0.255390264041525,0.166311404120579) ;
#449=ELLIPSE('',#99334,0.255390264028709,0.166311404112411) ;
#450=ELLIPSE('',#99335,0.255390264039117,0.166311404117828) ;
#451=ELLIPSE('',#99337,0.255390264033842,0.166311404118425) ;
#452=ELLIPSE('',#99338,0.255390264029649,0.166311404113467) ;
#453=ELLIPSE('',#100045,0.239471272541672,0.104190452490447) ;
#454=ELLIPSE('',#100046,0.239594752726074,0.104223676986789) ;
#455=ELLIPSE('',#100048,0.239594752697272,0.104223676980424) ;
#456=ELLIPSE('',#100049,0.239471272492843,0.104190452477864) ;
#457=ELLIPSE('',#100051,0.239594752684102,0.1042236769773) ;
#458=ELLIPSE('',#100052,0.239471272466969,0.10419045247166) ;
#459=ELLIPSE('',#100054,0.239594752734068,0.104223676990242) ;
#460=ELLIPSE('',#100055,0.239471272561877,0.104190452494461) ;
#461=ELLIPSE('',#100057,0.239471272527132,0.104190452486722) ;
#462=ELLIPSE('',#100058,0.239594752734183,0.104223676988681) ;
#463=ELLIPSE('',#100060,0.23959475268759,0.104223676978089) ;
#464=ELLIPSE('',#100061,0.239471272489249,0.104190452477087) ;
#465=ELLIPSE('',#100063,0.2395947526905,0.104223676978911) ;
#466=ELLIPSE('',#100064,0.239471272497335,0.104190452479123) ;
#467=ELLIPSE('',#100066,0.239594752708729,0.104223676983616) ;
#468=ELLIPSE('',#100067,0.239471272526268,0.104190452487083) ;
#469=ELLIPSE('',#100069,0.239471272514144,0.104190452483521) ;
#470=ELLIPSE('',#100070,0.239594752716605,0.104223676986095) ;
#471=ELLIPSE('',#100072,0.239594752699331,0.104223676981028) ;
#472=ELLIPSE('',#100073,0.239471272496544,0.10419045247883) ;
#473=ELLIPSE('',#100075,0.239594752723358,0.10422367698701) ;
#474=ELLIPSE('',#100076,0.239471272495837,0.104190452478645) ;
#475=ELLIPSE('',#100078,0.239594752698616,0.104223676981038) ;
#476=ELLIPSE('',#100079,0.239471272522506,0.104190452485985) ;
#477=ELLIPSE('',#100081,0.239471272517247,0.104190452484287) ;
#478=ELLIPSE('',#100082,0.239594752720674,0.104223676987029) ;
#479=ELLIPSE('',#100084,0.239594752709324,0.104223676983649) ;
#480=ELLIPSE('',#100085,0.239471272554278,0.104190452493733) ;
#481=ELLIPSE('',#100087,0.239594752719202,0.104223676985857) ;
#482=ELLIPSE('',#100088,0.239471272507799,0.104190452481569) ;
#483=ELLIPSE('',#100090,0.239594752706474,0.104223676983052) ;
#484=ELLIPSE('',#100091,0.239471272527043,0.104190452487123) ;
#485=ELLIPSE('',#100093,0.239471272527633,0.104190452486785) ;
#486=ELLIPSE('',#100094,0.239594752719546,0.104223676986731) ;
#487=ELLIPSE('',#100096,0.239594752703205,0.10422367698204) ;
#488=ELLIPSE('',#100097,0.239471272482974,0.10419045247551) ;
#489=ELLIPSE('',#100099,0.23959475271894,0.104223676985872) ;
#490=ELLIPSE('',#100100,0.239471272513673,0.104190452482924) ;
#491=ELLIPSE('',#100102,0.239594752701382,0.104223676981721) ;
#492=ELLIPSE('',#100103,0.239471272535599,0.104190452489416) ;
#493=ELLIPSE('',#100105,0.239471272525269,0.104190452486334) ;
#494=ELLIPSE('',#100106,0.239594752716578,0.104223676986044) ;
#495=ELLIPSE('',#100108,0.23959475276603,0.104223676998289) ;
#496=ELLIPSE('',#100109,0.239471272489896,0.104190452477545) ;
#497=ELLIPSE('',#100111,0.239594752717894,0.104223676985692) ;
#498=ELLIPSE('',#100112,0.239471272524125,0.10419045248605) ;
#499=ELLIPSE('',#100114,0.239594752691381,0.104223676979494) ;
#500=ELLIPSE('',#100115,0.239471272558152,0.10419045249462) ;
#501=ELLIPSE('',#100117,0.239471272517302,0.104190452484572) ;
#502=ELLIPSE('',#100118,0.239594752726099,0.104223676988114) ;
#503=ELLIPSE('',#100120,0.239594752760816,0.104223676997006) ;
#504=ELLIPSE('',#100121,0.239471272488601,0.104190452477342) ;
#505=ELLIPSE('',#100123,0.239594752734497,0.104223676990487) ;
#506=ELLIPSE('',#100124,0.239471272528897,0.104190452487192) ;
#507=ELLIPSE('',#100126,0.239594752719834,0.104223676986734) ;
#508=ELLIPSE('',#100127,0.239471272551583,0.104190452493005) ;
#509=ELLIPSE('',#100129,0.239471272526413,0.1041904524868) ;
#510=ELLIPSE('',#100130,0.239594752719693,0.104223676986493) ;
#511=ELLIPSE('',#100132,0.23959475272552,0.104223676988002) ;
#512=ELLIPSE('',#100133,0.23947127255968,0.104190452495628) ;
#513=ELLIPSE('',#100135,0.239594752745901,0.104223676993333) ;
#514=ELLIPSE('',#100136,0.239471272534012,0.104190452488509) ;
#515=ELLIPSE('',#100138,0.239594752723728,0.104223676987511) ;
#516=ELLIPSE('',#100139,0.239471272544375,0.10419045249119) ;
#517=ELLIPSE('',#100231,0.111803398874902,0.0999999999999214) ;
#518=ELLIPSE('',#100246,0.111803398875015,0.100000000000024) ;
#519=ELLIPSE('',#100249,0.19738899237826,0.0801201351308594) ;
#520=ELLIPSE('',#100250,0.197388988783904,0.0801201312644544) ;
#521=ELLIPSE('',#100251,0.111803398883664,0.100000000015977) ;
#522=ELLIPSE('',#100252,0.236436524449966,0.104276779744234) ;
#523=ELLIPSE('',#100253,0.222726289984573,0.0995178910570516) ;
#524=ELLIPSE('',#100255,0.222704123466412,0.099498796196121) ;
#525=ELLIPSE('',#100256,0.236408404049101,0.104269413800199) ;
#526=ELLIPSE('',#100257,0.236436524432732,0.104276779737213) ;
#527=ELLIPSE('',#100258,0.222726289984934,0.0995178910577687) ;
#528=ELLIPSE('',#100260,0.197388992378616,0.0801201351309043) ;
#529=ELLIPSE('',#100261,0.197388992379545,0.080120135131515) ;
#530=ELLIPSE('',#100263,0.222704123474636,0.0994987962024968) ;
#531=ELLIPSE('',#100264,0.236408404032557,0.104269413795424) ;
#532=ELLIPSE('',#100265,0.111803398978043,0.100000000180811) ;
#533=ELLIPSE('',#100266,0.197388988784215,0.080120131264687) ;
#534=ELLIPSE('',#100267,0.197388992379424,0.0801201351317529) ;
#535=ELLIPSE('',#100269,0.197388992379045,0.0801201351315553) ;
#536=ELLIPSE('',#100270,0.197388988782772,0.0801201312636463) ;
#537=ELLIPSE('',#100271,0.111803398854216,0.0999999999644239) ;
#538=ELLIPSE('',#100272,0.236436524483533,0.104276779754402) ;
#539=ELLIPSE('',#100273,0.222726289977912,0.0995178910519717) ;
#540=ELLIPSE('',#100275,0.2227041234645,0.0994987961949076) ;
#541=ELLIPSE('',#100276,0.236408403975384,0.104269413775528) ;
#542=ELLIPSE('',#100277,0.236436524415503,0.104276779732904) ;
#543=ELLIPSE('',#100278,0.222726289980937,0.0995178910544354) ;
#544=ELLIPSE('',#100280,0.197388992380326,0.0801201351322599) ;
#545=ELLIPSE('',#100281,0.197388992379516,0.0801201351314597) ;
#546=ELLIPSE('',#100283,0.222704123471206,0.0994987961995229) ;
#547=ELLIPSE('',#100284,0.236408404041556,0.104269413798962) ;
#548=ELLIPSE('',#100285,0.1118033989916,0.100000000205665) ;
#549=ELLIPSE('',#100286,0.197388988782326,0.0801201312633943) ;
#550=ELLIPSE('',#100287,0.197388992380803,0.0801201351327621) ;
#551=ELLIPSE('',#100289,0.197388992379311,0.0801201351317526) ;
#552=ELLIPSE('',#100290,0.197388988782863,0.0801201312636897) ;
#553=ELLIPSE('',#100291,0.111803398885653,0.100000000017746) ;
#554=ELLIPSE('',#100292,0.236436524510541,0.104276779762262) ;
#555=ELLIPSE('',#100293,0.222726289989238,0.0995178910616732) ;
#556=ELLIPSE('',#100295,0.222704123468478,0.099498796197896) ;
#557=ELLIPSE('',#100296,0.236408403942723,0.10426941376595) ;
#558=ELLIPSE('',#100297,0.236436524607894,0.10427677979644) ;
#559=ELLIPSE('',#100298,0.222726289996681,0.0995178910669966) ;
#560=ELLIPSE('',#100300,0.197388992379108,0.0801201351314067) ;
#561=ELLIPSE('',#100301,0.197388992378061,0.0801201351307853) ;
#562=ELLIPSE('',#100303,0.222704123464741,0.0994987961955434) ;
#563=ELLIPSE('',#100304,0.236408404096636,0.104269413815376) ;
#564=ELLIPSE('',#100305,0.111803399145635,0.100000000475424) ;
#565=ELLIPSE('',#100306,0.197388988779542,0.0801201312609667) ;
#566=ELLIPSE('',#100307,0.197388992378485,0.0801201351306929) ;
#567=ELLIPSE('',#100309,0.197388992378957,0.0801201351310294) ;
#568=ELLIPSE('',#100310,0.19738898878374,0.0801201312642938) ;
#569=ELLIPSE('',#100311,0.111803399036703,0.100000000285152) ;
#570=ELLIPSE('',#100312,0.236436524495273,0.104276779757397) ;
#571=ELLIPSE('',#100313,0.222726289990922,0.099517891062712) ;
#572=ELLIPSE('',#100315,0.222704123464531,0.0994987961947874) ;
#573=ELLIPSE('',#100316,0.236408404057535,0.10426941380379) ;
#574=ELLIPSE('',#100317,0.236436524486579,0.104276779756148) ;
#575=ELLIPSE('',#100318,0.222726289984491,0.0995178910572093) ;
#576=ELLIPSE('',#100320,0.197388992378839,0.0801201351314571) ;
#577=ELLIPSE('',#100321,0.197388992377843,0.0801201351307153) ;
#578=ELLIPSE('',#100323,0.222704123467226,0.0994987961965839) ;
#579=ELLIPSE('',#100324,0.236408404080475,0.104269413810236) ;
#580=ELLIPSE('',#100325,0.111803399487092,0.100000001075964) ;
#581=ELLIPSE('',#100326,0.197388988782072,0.080120131262859) ;
#582=ELLIPSE('',#100327,0.197388992379507,0.0801201351315046) ;
#583=ELLIPSE('',#100329,0.19738899237792,0.0801201351302709) ;
#584=ELLIPSE('',#100330,0.197388988782827,0.0801201312637812) ;
#585=ELLIPSE('',#100331,0.111803399293401,0.100000000733944) ;
#586=ELLIPSE('',#100332,0.236436524534394,0.104276779769979) ;
#587=ELLIPSE('',#100333,0.22272629000147,0.0995178910705121) ;
#588=ELLIPSE('',#100335,0.222704123464496,0.0994987961947227) ;
#589=ELLIPSE('',#100336,0.236408403913088,0.104269413756808) ;
#590=ELLIPSE('',#100337,0.236436524427347,0.104276779737167) ;
#591=ELLIPSE('',#100338,0.222726289994107,0.0995178910649231) ;
#592=ELLIPSE('',#100340,0.197388992379256,0.0801201351317907) ;
#593=ELLIPSE('',#100341,0.19738899237989,0.0801201351321866) ;
#594=ELLIPSE('',#100343,0.222704123455483,0.0994987961875182) ;
#595=ELLIPSE('',#100344,0.236408404037391,0.104269413796386) ;
#596=ELLIPSE('',#100345,0.111803399309713,0.100000000765477) ;
#597=ELLIPSE('',#100346,0.197388988785316,0.0801201312652288) ;
#598=ELLIPSE('',#100347,0.197388992379548,0.0801201351314808) ;
#599=ELLIPSE('',#100349,0.19738899237924,0.0801201351312266) ;
#600=ELLIPSE('',#100350,0.197388988776506,0.0801201312591199) ;
#601=ELLIPSE('',#100351,0.111803398888132,0.100000000025592) ;
#602=ELLIPSE('',#100352,0.236436524490662,0.104276779756003) ;
#603=ELLIPSE('',#100353,0.222726290011381,0.0995178910787348) ;
#604=ELLIPSE('',#100355,0.222704123464471,0.0994987961944618) ;
#605=ELLIPSE('',#100356,0.236408403978192,0.104269413778509) ;
#606=ELLIPSE('',#100357,0.236436524480116,0.104276779754641) ;
#607=ELLIPSE('',#100358,0.222726289983351,0.0995178910561129) ;
#608=ELLIPSE('',#100360,0.197388992377652,0.080120135130641) ;
#609=ELLIPSE('',#100361,0.197388992377957,0.0801201351307889) ;
#610=ELLIPSE('',#100363,0.222704123465533,0.0994987961961162) ;
#611=ELLIPSE('',#100364,0.236408404086778,0.104269413812232) ;
#612=ELLIPSE('',#100365,0.111803400137024,0.100000002213876) ;
#613=ELLIPSE('',#100366,0.1973889887795,0.0801201312608118) ;
#614=ELLIPSE('',#100367,0.197388992378253,0.0801201351305352) ;
#615=ELLIPSE('',#100369,0.197388992377339,0.080120135129837) ;
#616=ELLIPSE('',#100370,0.197388988783307,0.0801201312640243) ;
#617=ELLIPSE('',#100371,0.11180339860087,0.0999999995158049) ;
#618=ELLIPSE('',#100372,0.236436524487559,0.104276779755015) ;
#619=ELLIPSE('',#100373,0.222726290004162,0.0995178910729244) ;
#620=ELLIPSE('',#100375,0.222704123462615,0.0994987961928787) ;
#621=ELLIPSE('',#100376,0.236408404066321,0.104269413806983) ;
#622=ELLIPSE('',#100377,0.236436524282318,0.104276779688654) ;
#623=ELLIPSE('',#100378,0.222726289995458,0.0995178910658395) ;
#624=ELLIPSE('',#100380,0.197388992379746,0.0801201351321519) ;
#625=ELLIPSE('',#100381,0.197388992378042,0.0801201351301879) ;
#626=ELLIPSE('',#100383,0.222704123484497,0.099498796209647) ;
#627=ELLIPSE('',#100384,0.236408404052811,0.104269413801709) ;
#628=ELLIPSE('',#100385,0.111803399379941,0.100000000890385) ;
#629=ELLIPSE('',#100386,0.197388988782014,0.0801201312627937) ;
#630=ELLIPSE('',#100387,0.197388992380941,0.0801201351337526) ;
#631=ELLIPSE('',#100389,0.19738899238036,0.0801201351332252) ;
#632=ELLIPSE('',#100390,0.197388988775444,0.0801201312580623) ;
#633=ELLIPSE('',#100391,0.111803398688121,0.0999999996752641) ;
#634=ELLIPSE('',#100392,0.236436524475147,0.104276779747239) ;
#635=ELLIPSE('',#100393,0.222726289922601,0.0995178910101093) ;
#636=ELLIPSE('',#100395,0.222704123486384,0.0994987962122068) ;
#637=ELLIPSE('',#100396,0.236408404061106,0.104269413803139) ;
#638=ELLIPSE('',#100397,0.236436524346302,0.104276779709588) ;
#639=ELLIPSE('',#100398,0.22272628996843,0.0995178910441956) ;
#640=ELLIPSE('',#100400,0.197388992380072,0.0801201351314788) ;
#641=ELLIPSE('',#100401,0.197388992377762,0.0801201351300403) ;
#642=ELLIPSE('',#100403,0.22270412347746,0.0994987962033312) ;
#643=ELLIPSE('',#100404,0.236408404072224,0.104269413808533) ;
#644=ELLIPSE('',#100405,0.11180339854823,0.0999999994295695) ;
#645=ELLIPSE('',#100406,0.197388988782537,0.0801201312629481) ;
#646=ELLIPSE('',#100407,0.197388992380398,0.0801201351334049) ;
#714=FACE_BOUND('',#26275,.T.) ;
#715=FACE_BOUND('',#26276,.T.) ;
#716=FACE_BOUND('',#26277,.T.) ;
#717=FACE_BOUND('',#26278,.T.) ;
#718=FACE_BOUND('',#26279,.T.) ;
#719=FACE_BOUND('',#26280,.T.) ;
#720=FACE_BOUND('',#26281,.T.) ;
#721=FACE_BOUND('',#26282,.T.) ;
#722=FACE_BOUND('',#26283,.T.) ;
#723=FACE_BOUND('',#26284,.T.) ;
#724=FACE_BOUND('',#26285,.T.) ;
#725=FACE_BOUND('',#26286,.T.) ;
#726=FACE_BOUND('',#26287,.T.) ;
#727=FACE_BOUND('',#26288,.T.) ;
#728=FACE_BOUND('',#26289,.T.) ;
#729=FACE_BOUND('',#26290,.T.) ;
#730=FACE_BOUND('',#26291,.T.) ;
#731=FACE_BOUND('',#26292,.T.) ;
#732=FACE_BOUND('',#26293,.T.) ;
#733=FACE_BOUND('',#26294,.T.) ;
#734=FACE_BOUND('',#26296,.T.) ;
#735=FACE_BOUND('',#26298,.T.) ;
#736=FACE_BOUND('',#26300,.T.) ;
#737=FACE_BOUND('',#26302,.T.) ;
#738=FACE_BOUND('',#26304,.T.) ;
#739=FACE_BOUND('',#26306,.T.) ;
#740=FACE_BOUND('',#26308,.T.) ;
#741=FACE_BOUND('',#26310,.T.) ;
#742=FACE_BOUND('',#26312,.T.) ;
#743=FACE_BOUND('',#26337,.T.) ;
#744=FACE_BOUND('',#26338,.T.) ;
#745=FACE_BOUND('',#26339,.T.) ;
#746=FACE_BOUND('',#26340,.T.) ;
#747=FACE_BOUND('',#26341,.T.) ;
#748=FACE_BOUND('',#26342,.T.) ;
#749=FACE_BOUND('',#26343,.T.) ;
#750=FACE_BOUND('',#26344,.T.) ;
#751=FACE_BOUND('',#26345,.T.) ;
#752=FACE_BOUND('',#26346,.T.) ;
#753=FACE_BOUND('',#26348,.T.) ;
#754=FACE_BOUND('',#26356,.T.) ;
#755=FACE_BOUND('',#26357,.T.) ;
#756=FACE_BOUND('',#26358,.T.) ;
#757=FACE_BOUND('',#26359,.T.) ;
#758=FACE_BOUND('',#26360,.T.) ;
#759=FACE_BOUND('',#26361,.T.) ;
#760=FACE_BOUND('',#26362,.T.) ;
#761=FACE_BOUND('',#26363,.T.) ;
#762=FACE_BOUND('',#26364,.T.) ;
#763=FACE_BOUND('',#26365,.T.) ;
#764=FACE_BOUND('',#26380,.T.) ;
#765=FACE_BOUND('',#26396,.T.) ;
#766=FACE_BOUND('',#26403,.T.) ;
#767=FACE_BOUND('',#26715,.T.) ;
#768=FACE_BOUND('',#26721,.T.) ;
#769=FACE_BOUND('',#26727,.T.) ;
#770=FACE_BOUND('',#26733,.T.) ;
#771=FACE_BOUND('',#26739,.T.) ;
#772=FACE_BOUND('',#26745,.T.) ;
#773=FACE_BOUND('',#26751,.T.) ;
#774=FACE_BOUND('',#26757,.T.) ;
#775=FACE_BOUND('',#26763,.T.) ;
#776=FACE_BOUND('',#26817,.T.) ;
#777=FACE_BOUND('',#26822,.T.) ;
#778=FACE_BOUND('',#26827,.T.) ;
#779=FACE_BOUND('',#26832,.T.) ;
#780=FACE_BOUND('',#26837,.T.) ;
#781=FACE_BOUND('',#26842,.T.) ;
#782=FACE_BOUND('',#26847,.T.) ;
#783=FACE_BOUND('',#26852,.T.) ;
#784=FACE_BOUND('',#26857,.T.) ;
#785=FACE_BOUND('',#26904,.T.) ;
#786=FACE_BOUND('',#26910,.T.) ;
#787=FACE_BOUND('',#26916,.T.) ;
#788=FACE_BOUND('',#26922,.T.) ;
#789=FACE_BOUND('',#26928,.T.) ;
#790=FACE_BOUND('',#26934,.T.) ;
#791=FACE_BOUND('',#26940,.T.) ;
#792=FACE_BOUND('',#26946,.T.) ;
#793=FACE_BOUND('',#26952,.T.) ;
#1513=PLANE('',#98472) ;
#1514=PLANE('',#98523) ;
#1515=PLANE('',#98528) ;
#1516=PLANE('',#98533) ;
#1517=PLANE('',#98538) ;
#1518=PLANE('',#98543) ;
#1519=PLANE('',#98548) ;
#1520=PLANE('',#98553) ;
#1521=PLANE('',#98558) ;
#1522=PLANE('',#98563) ;
#1523=PLANE('',#98568) ;
#1524=PLANE('',#98569) ;
#1525=PLANE('',#98570) ;
#1526=PLANE('',#98571) ;
#1527=PLANE('',#98572) ;
#1528=PLANE('',#98573) ;
#1529=PLANE('',#98574) ;
#1530=PLANE('',#98575) ;
#1531=PLANE('',#98576) ;
#1532=PLANE('',#98577) ;
#1533=PLANE('',#98618) ;
#1534=PLANE('',#98622) ;
#1535=PLANE('',#98626) ;
#1536=PLANE('',#98630) ;
#1537=PLANE('',#98634) ;
#1538=PLANE('',#98638) ;
#1539=PLANE('',#98642) ;
#1540=PLANE('',#98646) ;
#1541=PLANE('',#98650) ;
#1542=PLANE('',#98654) ;
#1543=PLANE('',#98655) ;
#1544=PLANE('',#98684) ;
#1545=PLANE('',#98685) ;
#1546=PLANE('',#98690) ;
#1547=PLANE('',#98691) ;
#1548=PLANE('',#98692) ;
#1549=PLANE('',#98696) ;
#1550=PLANE('',#98697) ;
#1551=PLANE('',#98698) ;
#1552=PLANE('',#98699) ;
#1553=PLANE('',#98708) ;
#1554=PLANE('',#98712) ;
#1555=PLANE('',#98716) ;
#1556=PLANE('',#98717) ;
#1557=PLANE('',#98718) ;
#1558=PLANE('',#98723) ;
#1559=PLANE('',#98724) ;
#1560=PLANE('',#98725) ;
#1561=PLANE('',#98726) ;
#1562=PLANE('',#98727) ;
#1563=PLANE('',#98728) ;
#1564=PLANE('',#98729) ;
#1565=PLANE('',#98730) ;
#1566=PLANE('',#98731) ;
#1567=PLANE('',#98736) ;
#1568=PLANE('',#98737) ;
#1569=PLANE('',#98738) ;
#1570=PLANE('',#98739) ;
#1571=PLANE('',#98740) ;
#1572=PLANE('',#98741) ;
#1573=PLANE('',#98744) ;
#1574=PLANE('',#98745) ;
#1575=PLANE('',#98749) ;
#1576=PLANE('',#98750) ;
#1577=PLANE('',#98754) ;
#1578=PLANE('',#98755) ;
#1579=PLANE('',#98756) ;
#1580=PLANE('',#98760) ;
#1581=PLANE('',#98762) ;
#1582=PLANE('',#98763) ;
#1583=PLANE('',#98764) ;
#1584=PLANE('',#98765) ;
#1585=PLANE('',#98766) ;
#1586=PLANE('',#98767) ;
#1587=PLANE('',#98772) ;
#1588=PLANE('',#98773) ;
#1589=PLANE('',#98774) ;
#1590=PLANE('',#98775) ;
#1591=PLANE('',#98776) ;
#1592=PLANE('',#98777) ;
#1593=PLANE('',#98778) ;
#1594=PLANE('',#98779) ;
#1595=PLANE('',#98780) ;
#1596=PLANE('',#98785) ;
#1597=PLANE('',#98786) ;
#1598=PLANE('',#98794) ;
#1599=PLANE('',#98798) ;
#1600=PLANE('',#98802) ;
#1601=PLANE('',#98806) ;
#1602=PLANE('',#98807) ;
#1603=PLANE('',#99208) ;
#1604=PLANE('',#99209) ;
#1605=PLANE('',#99210) ;
#1606=PLANE('',#99215) ;
#1607=PLANE('',#99216) ;
#1608=PLANE('',#99217) ;
#1609=PLANE('',#99218) ;
#1610=PLANE('',#99219) ;
#1611=PLANE('',#99224) ;
#1612=PLANE('',#99225) ;
#1613=PLANE('',#99226) ;
#1614=PLANE('',#99227) ;
#1615=PLANE('',#99228) ;
#1616=PLANE('',#99233) ;
#1617=PLANE('',#99234) ;
#1618=PLANE('',#99235) ;
#1619=PLANE('',#99236) ;
#1620=PLANE('',#99237) ;
#1621=PLANE('',#99242) ;
#1622=PLANE('',#99243) ;
#1623=PLANE('',#99244) ;
#1624=PLANE('',#99245) ;
#1625=PLANE('',#99246) ;
#1626=PLANE('',#99251) ;
#1627=PLANE('',#99252) ;
#1628=PLANE('',#99253) ;
#1629=PLANE('',#99254) ;
#1630=PLANE('',#99255) ;
#1631=PLANE('',#99260) ;
#1632=PLANE('',#99261) ;
#1633=PLANE('',#99262) ;
#1634=PLANE('',#99263) ;
#1635=PLANE('',#99264) ;
#1636=PLANE('',#99269) ;
#1637=PLANE('',#99270) ;
#1638=PLANE('',#99271) ;
#1639=PLANE('',#99272) ;
#1640=PLANE('',#99273) ;
#1641=PLANE('',#99278) ;
#1642=PLANE('',#99279) ;
#1643=PLANE('',#99280) ;
#1644=PLANE('',#99281) ;
#1645=PLANE('',#99282) ;
#1646=PLANE('',#99287) ;
#1647=PLANE('',#99288) ;
#1648=PLANE('',#99289) ;
#1649=PLANE('',#99290) ;
#1650=PLANE('',#99293) ;
#1651=PLANE('',#99296) ;
#1652=PLANE('',#99299) ;
#1653=PLANE('',#99302) ;
#1654=PLANE('',#99305) ;
#1655=PLANE('',#99308) ;
#1656=PLANE('',#99311) ;
#1657=PLANE('',#99314) ;
#1658=PLANE('',#99315) ;
#1659=PLANE('',#99318) ;
#1660=PLANE('',#99321) ;
#1661=PLANE('',#99324) ;
#1662=PLANE('',#99327) ;
#1663=PLANE('',#99330) ;
#1664=PLANE('',#99333) ;
#1665=PLANE('',#99336) ;
#1666=PLANE('',#99339) ;
#1667=PLANE('',#99340) ;
#1668=PLANE('',#99341) ;
#1669=PLANE('',#99342) ;
#1670=PLANE('',#99343) ;
#1671=PLANE('',#99344) ;
#1672=PLANE('',#99345) ;
#1673=PLANE('',#99346) ;
#1674=PLANE('',#99347) ;
#1675=PLANE('',#99348) ;
#1676=PLANE('',#99349) ;
#1677=PLANE('',#99350) ;
#1678=PLANE('',#99351) ;
#1679=PLANE('',#99352) ;
#1680=PLANE('',#99353) ;
#1681=PLANE('',#99354) ;
#1682=PLANE('',#99355) ;
#1683=PLANE('',#99356) ;
#1684=PLANE('',#99357) ;
#1685=PLANE('',#99358) ;
#1686=PLANE('',#99359) ;
#1687=PLANE('',#99360) ;
#1688=PLANE('',#99361) ;
#1689=PLANE('',#99362) ;
#1690=PLANE('',#99363) ;
#1691=PLANE('',#99364) ;
#1692=PLANE('',#99365) ;
#1693=PLANE('',#99366) ;
#1694=PLANE('',#99367) ;
#1695=PLANE('',#99368) ;
#1696=PLANE('',#99369) ;
#1697=PLANE('',#99370) ;
#1698=PLANE('',#99371) ;
#1699=PLANE('',#99372) ;
#1700=PLANE('',#99373) ;
#1701=PLANE('',#99374) ;
#1702=PLANE('',#99375) ;
#1703=PLANE('',#99380) ;
#1704=PLANE('',#99381) ;
#1705=PLANE('',#99382) ;
#1706=PLANE('',#99383) ;
#1707=PLANE('',#99384) ;
#1708=PLANE('',#99389) ;
#1709=PLANE('',#99390) ;
#1710=PLANE('',#99391) ;
#1711=PLANE('',#99392) ;
#1712=PLANE('',#99393) ;
#1713=PLANE('',#99398) ;
#1714=PLANE('',#99399) ;
#1715=PLANE('',#99400) ;
#1716=PLANE('',#99401) ;
#1717=PLANE('',#99402) ;
#1718=PLANE('',#99407) ;
#1719=PLANE('',#99408) ;
#1720=PLANE('',#99409) ;
#1721=PLANE('',#99410) ;
#1722=PLANE('',#99411) ;
#1723=PLANE('',#99416) ;
#1724=PLANE('',#99417) ;
#1725=PLANE('',#99418) ;
#1726=PLANE('',#99419) ;
#1727=PLANE('',#99420) ;
#1728=PLANE('',#99425) ;
#1729=PLANE('',#99426) ;
#1730=PLANE('',#99427) ;
#1731=PLANE('',#99428) ;
#1732=PLANE('',#99429) ;
#1733=PLANE('',#99434) ;
#1734=PLANE('',#99435) ;
#1735=PLANE('',#99436) ;
#1736=PLANE('',#99437) ;
#1737=PLANE('',#99438) ;
#1738=PLANE('',#99443) ;
#1739=PLANE('',#99444) ;
#1740=PLANE('',#99445) ;
#1741=PLANE('',#99446) ;
#1742=PLANE('',#99447) ;
#1743=PLANE('',#99452) ;
#1744=PLANE('',#99453) ;
#1745=PLANE('',#99454) ;
#1746=PLANE('',#99455) ;
#1747=PLANE('',#99456) ;
#1748=PLANE('',#99457) ;
#1749=PLANE('',#99458) ;
#1750=PLANE('',#99459) ;
#1751=PLANE('',#99460) ;
#1752=PLANE('',#99461) ;
#1753=PLANE('',#99462) ;
#1754=PLANE('',#99463) ;
#1755=PLANE('',#99464) ;
#1756=PLANE('',#99465) ;
#1757=PLANE('',#99469) ;
#1758=PLANE('',#99470) ;
#1759=PLANE('',#99474) ;
#1760=PLANE('',#99475) ;
#1761=PLANE('',#99479) ;
#1762=PLANE('',#99480) ;
#1763=PLANE('',#99484) ;
#1764=PLANE('',#99485) ;
#1765=PLANE('',#99489) ;
#1766=PLANE('',#99490) ;
#1767=PLANE('',#99494) ;
#1768=PLANE('',#99495) ;
#1769=PLANE('',#99499) ;
#1770=PLANE('',#99500) ;
#1771=PLANE('',#99504) ;
#1772=PLANE('',#99505) ;
#1773=PLANE('',#99509) ;
#1774=PLANE('',#99510) ;
#1775=PLANE('',#99514) ;
#1776=PLANE('',#99515) ;
#1777=PLANE('',#99519) ;
#1778=PLANE('',#99520) ;
#1779=PLANE('',#99524) ;
#1780=PLANE('',#99525) ;
#1781=PLANE('',#99529) ;
#1782=PLANE('',#99530) ;
#1783=PLANE('',#99534) ;
#1784=PLANE('',#99535) ;
#1785=PLANE('',#99539) ;
#1786=PLANE('',#99540) ;
#1787=PLANE('',#99544) ;
#1788=PLANE('',#99545) ;
#1789=PLANE('',#99549) ;
#1790=PLANE('',#99550) ;
#1791=PLANE('',#99554) ;
#1792=PLANE('',#99555) ;
#1793=PLANE('',#99556) ;
#1794=PLANE('',#99560) ;
#1795=PLANE('',#99562) ;
#1796=PLANE('',#99563) ;
#1797=PLANE('',#99567) ;
#1798=PLANE('',#99569) ;
#1799=PLANE('',#99570) ;
#1800=PLANE('',#99574) ;
#1801=PLANE('',#99576) ;
#1802=PLANE('',#99577) ;
#1803=PLANE('',#99581) ;
#1804=PLANE('',#99583) ;
#1805=PLANE('',#99584) ;
#1806=PLANE('',#99588) ;
#1807=PLANE('',#99590) ;
#1808=PLANE('',#99591) ;
#1809=PLANE('',#99595) ;
#1810=PLANE('',#99597) ;
#1811=PLANE('',#99598) ;
#1812=PLANE('',#99602) ;
#1813=PLANE('',#99604) ;
#1814=PLANE('',#99605) ;
#1815=PLANE('',#99609) ;
#1816=PLANE('',#99611) ;
#1817=PLANE('',#99612) ;
#1818=PLANE('',#99616) ;
#1819=PLANE('',#99618) ;
#1820=PLANE('',#99619) ;
#1821=PLANE('',#99620) ;
#1822=PLANE('',#99621) ;
#1823=PLANE('',#99622) ;
#1824=PLANE('',#99623) ;
#1825=PLANE('',#99624) ;
#1826=PLANE('',#99625) ;
#1827=PLANE('',#99626) ;
#1828=PLANE('',#99627) ;
#1829=PLANE('',#99628) ;
#1830=PLANE('',#99629) ;
#1831=PLANE('',#99630) ;
#1832=PLANE('',#99631) ;
#1833=PLANE('',#99632) ;
#1834=PLANE('',#99633) ;
#1835=PLANE('',#99634) ;
#1836=PLANE('',#99635) ;
#1837=PLANE('',#99636) ;
#1838=PLANE('',#99637) ;
#1839=PLANE('',#99638) ;
#1840=PLANE('',#99639) ;
#1841=PLANE('',#99640) ;
#1842=PLANE('',#99641) ;
#1843=PLANE('',#99642) ;
#1844=PLANE('',#99643) ;
#1845=PLANE('',#99644) ;
#1846=PLANE('',#99645) ;
#1847=PLANE('',#99646) ;
#1848=PLANE('',#99647) ;
#1849=PLANE('',#99648) ;
#1850=PLANE('',#99649) ;
#1851=PLANE('',#99650) ;
#1852=PLANE('',#99651) ;
#1853=PLANE('',#99652) ;
#1854=PLANE('',#99653) ;
#1855=PLANE('',#99654) ;
#1856=PLANE('',#99655) ;
#1857=PLANE('',#99656) ;
#1858=PLANE('',#99657) ;
#1859=PLANE('',#99658) ;
#1860=PLANE('',#99659) ;
#1861=PLANE('',#99660) ;
#1862=PLANE('',#99661) ;
#1863=PLANE('',#99662) ;
#1864=PLANE('',#99663) ;
#1865=PLANE('',#99668) ;
#1866=PLANE('',#99669) ;
#1867=PLANE('',#99670) ;
#1868=PLANE('',#99671) ;
#1869=PLANE('',#99672) ;
#1870=PLANE('',#99677) ;
#1871=PLANE('',#99678) ;
#1872=PLANE('',#99679) ;
#1873=PLANE('',#99680) ;
#1874=PLANE('',#99681) ;
#1875=PLANE('',#99686) ;
#1876=PLANE('',#99687) ;
#1877=PLANE('',#99688) ;
#1878=PLANE('',#99689) ;
#1879=PLANE('',#99690) ;
#1880=PLANE('',#99695) ;
#1881=PLANE('',#99696) ;
#1882=PLANE('',#99697) ;
#1883=PLANE('',#99698) ;
#1884=PLANE('',#99699) ;
#1885=PLANE('',#99704) ;
#1886=PLANE('',#99705) ;
#1887=PLANE('',#99706) ;
#1888=PLANE('',#99707) ;
#1889=PLANE('',#99708) ;
#1890=PLANE('',#99713) ;
#1891=PLANE('',#99714) ;
#1892=PLANE('',#99715) ;
#1893=PLANE('',#99716) ;
#1894=PLANE('',#99717) ;
#1895=PLANE('',#99722) ;
#1896=PLANE('',#99723) ;
#1897=PLANE('',#99724) ;
#1898=PLANE('',#99725) ;
#1899=PLANE('',#99726) ;
#1900=PLANE('',#99731) ;
#1901=PLANE('',#99732) ;
#1902=PLANE('',#99733) ;
#1903=PLANE('',#99734) ;
#1904=PLANE('',#99735) ;
#1905=PLANE('',#99740) ;
#1906=PLANE('',#99741) ;
#1907=PLANE('',#99742) ;
#1908=PLANE('',#99743) ;
#1909=PLANE('',#99744) ;
#1910=PLANE('',#99745) ;
#1911=PLANE('',#99746) ;
#1912=PLANE('',#99747) ;
#1913=PLANE('',#99748) ;
#1914=PLANE('',#99749) ;
#1915=PLANE('',#99750) ;
#1916=PLANE('',#99751) ;
#1917=PLANE('',#99752) ;
#1918=PLANE('',#99753) ;
#1919=PLANE('',#99754) ;
#1920=PLANE('',#99755) ;
#1921=PLANE('',#99756) ;
#1922=PLANE('',#99757) ;
#1923=PLANE('',#99758) ;
#1924=PLANE('',#99759) ;
#1925=PLANE('',#99760) ;
#1926=PLANE('',#99761) ;
#1927=PLANE('',#99762) ;
#1928=PLANE('',#99763) ;
#1929=PLANE('',#99764) ;
#1930=PLANE('',#99765) ;
#1931=PLANE('',#99766) ;
#1932=PLANE('',#99767) ;
#1933=PLANE('',#99768) ;
#1934=PLANE('',#99769) ;
#1935=PLANE('',#99770) ;
#1936=PLANE('',#99771) ;
#1937=PLANE('',#99772) ;
#1938=PLANE('',#99773) ;
#1939=PLANE('',#99774) ;
#1940=PLANE('',#99775) ;
#1941=PLANE('',#99776) ;
#1942=PLANE('',#99777) ;
#1943=PLANE('',#99778) ;
#1944=PLANE('',#99779) ;
#1945=PLANE('',#99780) ;
#1946=PLANE('',#99781) ;
#1947=PLANE('',#99782) ;
#1948=PLANE('',#99783) ;
#1949=PLANE('',#99784) ;
#1950=PLANE('',#99785) ;
#1951=PLANE('',#99786) ;
#1952=PLANE('',#99787) ;
#1953=PLANE('',#99788) ;
#1954=PLANE('',#99792) ;
#1955=PLANE('',#99796) ;
#1956=PLANE('',#99800) ;
#1957=PLANE('',#99804) ;
#1958=PLANE('',#99805) ;
#1959=PLANE('',#99809) ;
#1960=PLANE('',#99813) ;
#1961=PLANE('',#99817) ;
#1962=PLANE('',#99821) ;
#1963=PLANE('',#99822) ;
#1964=PLANE('',#99826) ;
#1965=PLANE('',#99830) ;
#1966=PLANE('',#99834) ;
#1967=PLANE('',#99838) ;
#1968=PLANE('',#99839) ;
#1969=PLANE('',#99843) ;
#1970=PLANE('',#99847) ;
#1971=PLANE('',#99851) ;
#1972=PLANE('',#99855) ;
#1973=PLANE('',#99856) ;
#1974=PLANE('',#99860) ;
#1975=PLANE('',#99864) ;
#1976=PLANE('',#99868) ;
#1977=PLANE('',#99872) ;
#1978=PLANE('',#99873) ;
#1979=PLANE('',#99877) ;
#1980=PLANE('',#99881) ;
#1981=PLANE('',#99885) ;
#1982=PLANE('',#99889) ;
#1983=PLANE('',#99890) ;
#1984=PLANE('',#99894) ;
#1985=PLANE('',#99898) ;
#1986=PLANE('',#99902) ;
#1987=PLANE('',#99906) ;
#1988=PLANE('',#99907) ;
#1989=PLANE('',#99911) ;
#1990=PLANE('',#99915) ;
#1991=PLANE('',#99919) ;
#1992=PLANE('',#99923) ;
#1993=PLANE('',#99924) ;
#1994=PLANE('',#99928) ;
#1995=PLANE('',#99932) ;
#1996=PLANE('',#99936) ;
#1997=PLANE('',#99940) ;
#1998=PLANE('',#99941) ;
#2197=B_SPLINE_CURVE_WITH_KNOTS('',3,(#152042,#152043,#152044,#152045,#152046,
#152047,#152048,#152049,#152050,#152051,#152052,#152053,#152054,#152055,
#152056,#152057,#152058,#152059,#152060,#152061,#152062,#152063,#152064,
#152065,#152066,#152067,#152068,#152069,#152070,#152071,#152072,#152073,
#152074,#152075,#152076,#152077,#152078,#152079,#152080,#152081,#152082,
#152083,#152084,#152085,#152086,#152087,#152088,#152089,#152090,#152091,
#152092,#152093,#152094,#152095,#152096,#152097,#152098,#152099,#152100,
#152101,#152102,#152103,#152104,#152105,#152106,#152107,#152108,#152109,
#152110,#152111,#152112,#152113,#152114,#152115,#152116,#152117,#152118,
#152119,#152120),.UNSPECIFIED.,.F.,.F.,(4,2,2,2,2,2,2,2,2,1,2,2,2,2,2,2,
2,2,1,2,2,2,2,2,2,2,2,2,2,1,2,2,2,2,2,2,2,2,2,2,4),(-2.04439259789017E-6,
0.,1.16813469870535E-6,2.3362693974107E-6,4.67253879482139E-6,9.34507758964279E-6,
1.56893443514872E-5,2.5897054707271E-5,3.53798289796446E-5,3.67345110185551E-5,
3.74570081059741E-5,3.91084300200745E-5,4.3512221791009E-5,4.45654530819768E-5,
6.26353541277857E-5,6.56193588433549E-5,7.12078702674521E-5,7.16407948146347E-5,
7.25009999533889E-5,7.34840915405366E-5,7.61056691062638E-5,8.65919793691728E-5,
8.89786567925481E-5,9.40446697643188E-5,9.57333407549091E-5,9.79849020756961E-5,
0.000106991147358844,0.000113571562047159,0.000119834164740902,0.000121170237394284,
0.000122506310047666,0.00012517845535443,0.000130522745967958,0.000132049686143252,
0.000136121526610702,0.000138121518246153,0.000141418986123913,0.000147599170335016,
0.000149659231738717,0.000157899477353521,0.000165007876130274),
 .UNSPECIFIED.) ;
#2198=B_SPLINE_CURVE_WITH_KNOTS('',3,(#152123,#152124,#152125,#152126,#152127,
#152128,#152129,#152130,#152131,#152132,#152133,#152134,#152135,#152136,
#152137,#152138,#152139,#152140,#152141,#152142,#152143,#152144,#152145,
#152146,#152147,#152148,#152149,#152150,#152151,#152152,#152153,#152154,
#152155,#152156,#152157,#152158,#152159,#152160,#152161,#152162,#152163,
#152164,#152165,#152166,#152167,#152168,#152169,#152170,#152171,#152172),
 .UNSPECIFIED.,.F.,.F.,(4,2,2,2,2,2,2,2,2,2,2,2,2,2,2,2,2,2,2,2,2,2,2,2,
4),(-2.08053324537705E-6,4.2351647362715E-22,1.73126834661496E-6,3.96468142042611E-6,
7.52178969731147E-6,1.32303807352218E-5,2.25750184175543E-5,3.87948997653528E-5,
5.72367363101908E-5,6.41156850334219E-5,7.29633420205792E-5,7.57300836966956E-5,
9.46996266571652E-5,9.75514675378546E-5,0.000111620796538317,0.000116439892133749,
0.000117409636556728,0.000134179897042086,0.000142027094744281,0.000142768074549618,
0.000154973322944091,0.000157365523939564,0.000159579629273015,0.000173553148900826,
0.000174961243144783),.UNSPECIFIED.) ;
#2199=B_SPLINE_CURVE_WITH_KNOTS('',3,(#152186,#152187,#152188,#152189,#152190,
#152191,#152192,#152193,#152194,#152195,#152196,#152197,#152198,#152199,
#152200,#152201,#152202,#152203,#152204,#152205,#152206,#152207,#152208,
#152209,#152210,#152211,#152212,#152213,#152214,#152215,#152216,#152217,
#152218,#152219,#152220,#152221,#152222,#152223,#152224,#152225,#152226,
#152227,#152228,#152229,#152230,#152231,#152232,#152233,#152234,#152235,
#152236,#152237,#152238,#152239,#152240,#152241,#152242,#152243,#152244,
#152245,#152246,#152247,#152248,#152249,#152250,#152251,#152252,#152253,
#152254,#152255,#152256,#152257,#152258,#152259,#152260,#152261,#152262,
#152263,#152264),.UNSPECIFIED.,.F.,.F.,(4,2,2,2,2,2,2,2,2,1,2,2,2,2,2,2,
2,2,1,2,2,2,2,2,2,2,2,2,2,1,2,2,2,2,2,2,2,2,2,2,4),(-2.0443925978901E-6,
-4.2351647362715E-22,1.16813469870574E-6,2.33626939741147E-6,4.67253879482294E-6,
9.34507758964589E-6,1.56893443514892E-5,2.5897054707273E-5,3.53798289796464E-5,
3.67345110185569E-5,3.74570081059758E-5,3.91084300200762E-5,4.35122217910106E-5,
4.45654530819776E-5,6.26353541267333E-5,6.56193588433769E-5,7.12078702674526E-5,
7.16407948146629E-5,7.2500999953418E-5,7.34840915405668E-5,7.61056691062967E-5,
8.65919793692166E-5,8.89786567925514E-5,9.40446697643274E-5,9.57333407549194E-5,
9.79849020757087E-5,0.000106991147358866,0.000113571562047158,0.000119834164740905,
0.000121170237394289,0.000122506310047672,0.000125178455354439,0.000130522745967973,
0.000132049686143269,0.000136121526610723,0.000138121518246146,0.000141418986123914,
0.000147599170335021,0.000149659231738723,0.000157899477353533,0.000165007876130275),
 .UNSPECIFIED.) ;
#2200=B_SPLINE_CURVE_WITH_KNOTS('',3,(#152267,#152268,#152269,#152270,#152271,
#152272,#152273,#152274,#152275,#152276,#152277,#152278,#152279,#152280,
#152281,#152282,#152283,#152284,#152285,#152286,#152287,#152288,#152289,
#152290,#152291,#152292,#152293,#152294,#152295,#152296,#152297,#152298,
#152299,#152300,#152301,#152302,#152303,#152304,#152305,#152306,#152307,
#152308,#152309,#152310,#152311,#152312,#152313,#152314,#152315,#152316,
#152317,#152318,#152319,#152320,#152321,#152322,#152323,#152324,#152325,
#152326,#152327,#152328,#152329,#152330,#152331,#152332,#152333,#152334,
#152335,#152336,#152337,#152338,#152339,#152340,#152341,#152342,#152343,
#152344,#152345,#152346,#152347),.UNSPECIFIED.,.F.,.F.,(4,2,2,2,2,2,2,2,
2,2,1,2,2,2,2,2,2,2,2,1,2,2,2,2,2,2,2,2,2,2,1,2,2,2,2,2,2,2,2,2,2,4),(-2.04439259788975E-6,
-1.02219629894488E-6,0.,1.16813469870559E-6,2.33626939741118E-6,4.67253879482236E-6,
9.34507758964471E-6,1.56893443514874E-5,2.58970547072708E-5,3.53798289796441E-5,
3.67345110185546E-5,3.74570081059735E-5,3.91084300200739E-5,4.35122217910083E-5,
4.45654530819754E-5,6.26353541276203E-5,6.56193588433579E-5,7.12078702674436E-5,
7.1640794814638E-5,7.25009999533923E-5,7.348409154054E-5,7.61056691062674E-5,
8.65919793691769E-5,8.89786567925471E-5,9.40446697643204E-5,9.57333407549114E-5,
9.79849020756996E-5,0.000106991147358852,0.000113571562047158,0.000119834164740902,
0.000121170237394284,0.000122506310047666,0.00012517845535443,0.000130522745967958,
0.000132049686143252,0.000136121526610702,0.000138121518246153,0.000141418986123913,
0.000147599170335002,0.000149659231738699,0.000157899477353485,0.000165007876130273),
 .UNSPECIFIED.) ;
#2201=B_SPLINE_CURVE_WITH_KNOTS('',3,(#152361,#152362,#152363,#152364,#152365,
#152366,#152367,#152368,#152369,#152370,#152371,#152372,#152373,#152374,
#152375,#152376,#152377,#152378,#152379,#152380,#152381,#152382,#152383,
#152384,#152385,#152386,#152387,#152388,#152389,#152390,#152391,#152392,
#152393,#152394,#152395,#152396,#152397,#152398,#152399,#152400,#152401,
#152402,#152403,#152404,#152405,#152406,#152407,#152408,#152409,#152410,
#152411,#152412,#152413,#152414,#152415,#152416,#152417,#152418,#152419,
#152420,#152421,#152422,#152423,#152424,#152425,#152426,#152427,#152428,
#152429,#152430,#152431,#152432,#152433,#152434,#152435,#152436,#152437,
#152438,#152439,#152440,#152441,#152442),.UNSPECIFIED.,.F.,.F.,(4,2,1,2,
2,2,2,2,2,2,2,1,2,2,2,2,2,2,2,2,1,2,2,2,2,2,2,2,2,2,2,1,2,2,2,2,2,2,2,2,
2,2,4),(-2.04439246668907E-6,-1.98050532921559E-6,-1.02219629894998E-6,
0.,1.16813469870384E-6,2.33626939740767E-6,4.67253879481535E-6,9.34507758963069E-6,
1.56893443514762E-5,2.58970547072613E-5,3.53798289796358E-5,3.67345110185464E-5,
3.74570081059654E-5,3.9108430020066E-5,4.35122217910009E-5,4.45654530819649E-5,
6.26353541268739E-5,6.56193588433615E-5,7.12078702674378E-5,7.16407948146413E-5,
7.25009999533956E-5,7.34840915405433E-5,7.61056691062706E-5,8.65919793691797E-5,
8.89786567925395E-5,9.40446697643135E-5,9.57333407549048E-5,9.79849020756933E-5,
0.000106991147358847,0.000113571562047149,0.000119834164740893,0.000121170237394276,
0.00012250631004766,0.000125178455354427,0.000130522745967961,0.000132049686143256,
0.000136121526610711,0.00013812151824614,0.000141418986123901,0.000147599170334991,
0.000149659231738688,0.000157899477353475,0.000165007876130261),
 .UNSPECIFIED.) ;
#2202=B_SPLINE_CURVE_WITH_KNOTS('',3,(#152445,#152446,#152447,#152448,#152449,
#152450,#152451,#152452,#152453,#152454,#152455,#152456,#152457,#152458,
#152459,#152460,#152461,#152462,#152463,#152464,#152465,#152466,#152467,
#152468,#152469,#152470,#152471,#152472,#152473,#152474,#152475,#152476,
#152477,#152478,#152479,#152480,#152481,#152482,#152483,#152484,#152485,
#152486,#152487,#152488,#152489,#152490,#152491,#152492,#152493,#152494,
#152495,#152496,#152497,#152498,#152499,#152500,#152501,#152502,#152503,
#152504,#152505,#152506,#152507,#152508,#152509,#152510,#152511,#152512,
#152513,#152514,#152515,#152516,#152517,#152518,#152519,#152520,#152521,
#152522,#152523),.UNSPECIFIED.,.F.,.F.,(4,2,2,2,2,2,2,2,2,1,2,2,2,2,2,2,
2,2,1,2,2,2,2,2,2,2,2,2,2,1,2,2,2,2,2,2,2,2,2,2,4),(-2.04439259788986E-6,
0.,1.16813469870571E-6,2.33626939741142E-6,4.67253879482284E-6,9.34507758964569E-6,
1.56893443514882E-5,2.58970547072723E-5,3.53798289796464E-5,3.6734511018557E-5,
3.7457008105976E-5,3.91084300200765E-5,4.35122217910112E-5,4.45654530819765E-5,
6.26353541265572E-5,6.56193588433932E-5,7.12078702674494E-5,7.16407948146812E-5,
7.25009999534366E-5,7.34840915405856E-5,7.61056691063164E-5,8.65919793692397E-5,
8.89786567925485E-5,9.40446697643211E-5,9.57333407549119E-5,9.79849020756997E-5,
0.000106991147358851,0.000113571562047157,0.000119834164740902,0.000121170237394286,
0.000122506310047671,0.000125178455354439,0.000130522745967977,0.000132049686143273,
0.00013612152661073,0.00013812151824615,0.000141418986123912,0.000147599170335004,
0.000149659231738701,0.000157899477353491,0.000165007876130273),
 .UNSPECIFIED.) ;
#2203=B_SPLINE_CURVE_WITH_KNOTS('',3,(#152537,#152538,#152539,#152540,#152541,
#152542,#152543,#152544,#152545,#152546,#152547,#152548,#152549,#152550,
#152551,#152552,#152553,#152554,#152555,#152556,#152557,#152558,#152559,
#152560,#152561,#152562,#152563,#152564,#152565,#152566,#152567,#152568,
#152569,#152570,#152571,#152572,#152573,#152574,#152575,#152576,#152577,
#152578,#152579,#152580,#152581,#152582,#152583,#152584,#152585,#152586,
#152587,#152588,#152589,#152590,#152591,#152592,#152593,#152594,#152595,
#152596,#152597,#152598,#152599,#152600,#152601,#152602,#152603,#152604,
#152605,#152606,#152607,#152608,#152609,#152610,#152611,#152612,#152613,
#152614,#152615,#152616),.UNSPECIFIED.,.F.,.F.,(4,1,2,2,2,2,2,2,2,2,1,2,
2,2,2,2,2,2,2,1,2,2,2,2,2,2,2,2,2,2,1,2,2,2,2,2,2,2,2,2,2,4),(-2.04439259788173E-6,
-1.02219629894086E-6,0.,1.16813469870681E-6,2.33626939741361E-6,4.67253879482722E-6,
9.34507758965445E-6,1.56893443514986E-5,2.58970547072802E-5,3.53798289796539E-5,
3.67345110185645E-5,3.74570081059834E-5,3.91084300200839E-5,4.35122217910184E-5,
4.45654530819858E-5,6.26353541299918E-5,6.56193588433716E-5,7.1207870267458E-5,
7.16407948146529E-5,7.25009999534074E-5,7.34840915405553E-5,7.61056691062832E-5,
8.65919793691949E-5,8.89786567925583E-5,9.40446697643248E-5,9.57333407549136E-5,
9.79849020756987E-5,0.000106991147358839,0.000113571562047167,0.000119834164740911,
0.000121170237394293,0.000122506310047674,0.000125178455354437,0.000130522745967964,
0.000132049686143257,0.000136121526610706,0.000138121518246156,0.00014141898612392,
0.000147599170335024,0.000149659231738725,0.00015789947735353,0.000165007876130282),
 .UNSPECIFIED.) ;
#2204=B_SPLINE_CURVE_WITH_KNOTS('',3,(#152619,#152620,#152621,#152622,#152623,
#152624,#152625,#152626,#152627,#152628,#152629,#152630,#152631,#152632,
#152633,#152634,#152635,#152636,#152637,#152638,#152639,#152640,#152641,
#152642,#152643,#152644,#152645,#152646,#152647,#152648,#152649,#152650,
#152651,#152652,#152653,#152654,#152655,#152656,#152657,#152658,#152659,
#152660,#152661,#152662,#152663,#152664,#152665,#152666,#152667,#152668,
#152669,#152670,#152671,#152672,#152673,#152674,#152675,#152676,#152677,
#152678,#152679,#152680,#152681,#152682,#152683,#152684,#152685,#152686,
#152687,#152688,#152689,#152690,#152691,#152692,#152693,#152694,#152695,
#152696,#152697,#152698,#152699),.UNSPECIFIED.,.F.,.F.,(4,2,2,2,2,2,2,2,
2,2,1,2,2,2,2,2,2,2,2,1,2,2,2,2,2,2,2,2,2,2,1,2,2,2,2,2,2,2,2,2,2,4),(-2.0443925978812E-6,
-1.0221962989406E-6,4.2351647362715E-22,1.1681346987067E-6,2.33626939741339E-6,
4.67253879482678E-6,9.34507758965356E-6,1.56893443514987E-5,2.58970547072825E-5,
3.53798289796548E-5,3.67345110185651E-5,3.7457008105984E-5,3.91084300200842E-5,
4.35122217910181E-5,4.45654530819845E-5,6.2635354127915E-5,6.56193588433688E-5,
7.12078702674513E-5,7.16407948146474E-5,7.25009999534015E-5,7.3484091540549E-5,
7.61056691062757E-5,8.65919793691826E-5,8.89786567925572E-5,9.40446697643321E-5,
9.57333407549237E-5,9.79849020757126E-5,0.000106991147358868,0.000113571562047162,
0.000119834164740911,0.000121170237394293,0.000122506310047674,0.000125178455354437,
0.000130522745967964,0.000132049686143257,0.000136121526610706,0.000138121518246158,
0.000141418986123922,0.00014759917033502,0.00014965923173872,0.000157899477353517,
0.000165007876130284),.UNSPECIFIED.) ;
#2205=B_SPLINE_CURVE_WITH_KNOTS('',3,(#152713,#152714,#152715,#152716,#152717,
#152718,#152719,#152720,#152721,#152722,#152723,#152724,#152725,#152726,
#152727,#152728,#152729,#152730,#152731,#152732,#152733,#152734,#152735,
#152736,#152737,#152738,#152739,#152740,#152741,#152742,#152743,#152744,
#152745,#152746,#152747,#152748,#152749,#152750,#152751,#152752,#152753,
#152754,#152755,#152756,#152757,#152758,#152759,#152760,#152761,#152762,
#152763,#152764,#152765,#152766,#152767,#152768,#152769,#152770,#152771,
#152772,#152773,#152774,#152775,#152776,#152777,#152778,#152779,#152780,
#152781,#152782,#152783,#152784,#152785,#152786,#152787,#152788,#152789,
#152790,#152791),.UNSPECIFIED.,.F.,.F.,(4,2,2,2,2,2,2,2,2,1,2,2,2,2,2,2,
2,2,1,2,2,2,2,2,2,2,2,2,2,1,2,2,2,2,2,2,2,2,2,2,4),(-2.04439259789012E-6,
-4.2351647362715E-22,1.16813469870576E-6,2.33626939741152E-6,4.67253879482304E-6,
9.34507758964607E-6,1.56893443514891E-5,2.5897054707274E-5,3.53798289796481E-5,
3.67345110185587E-5,3.74570081059777E-5,3.91084300200782E-5,4.35122217910129E-5,
4.45654530819766E-5,6.26353541292069E-5,6.56193588434199E-5,7.12078702674474E-5,
7.16407948147103E-5,7.25009999534661E-5,7.34840915406156E-5,7.61056691063475E-5,
8.6591979369275E-5,8.89786567925508E-5,9.40446697643281E-5,9.57333407549205E-5,
9.79849020757104E-5,0.00010699114735887,0.000113571562047157,0.000119834164740904,
0.00012117023739429,0.000122506310047677,0.00012517845535445,0.000130522745967996,
0.000132049686143294,0.000136121526610758,0.000138121518246149,0.000141418986123913,
0.000147599170334991,0.000149659231738683,0.000157899477353454,0.000165007876130274),
 .UNSPECIFIED.) ;
#2206=B_SPLINE_CURVE_WITH_KNOTS('',3,(#152794,#152795,#152796,#152797,#152798,
#152799,#152800,#152801,#152802,#152803,#152804,#152805,#152806,#152807,
#152808,#152809,#152810,#152811,#152812,#152813,#152814,#152815,#152816,
#152817,#152818,#152819,#152820,#152821,#152822,#152823,#152824,#152825,
#152826,#152827,#152828,#152829,#152830,#152831,#152832,#152833,#152834,
#152835,#152836,#152837,#152838,#152839,#152840,#152841,#152842,#152843,
#152844,#152845,#152846,#152847,#152848,#152849,#152850,#152851,#152852,
#152853,#152854,#152855,#152856,#152857,#152858,#152859,#152860,#152861,
#152862,#152863,#152864,#152865,#152866,#152867,#152868,#152869,#152870,
#152871,#152872,#152873,#152874),.UNSPECIFIED.,.F.,.F.,(4,2,2,2,2,2,2,2,
2,2,1,2,2,2,2,2,2,2,2,1,2,2,2,2,2,2,2,2,2,2,1,2,2,2,2,2,2,2,2,2,2,4),(-2.04439259790034E-6,
-1.02219629895017E-6,0.,1.16813469870406E-6,2.33626939740812E-6,4.67253879481623E-6,
9.34507758963246E-6,1.56893443514797E-5,2.58970547072656E-5,3.53798289796408E-5,
3.67345110185516E-5,3.74570081059706E-5,3.91084300200713E-5,4.35122217910066E-5,
4.45654530819667E-5,6.26353541284101E-5,6.5619358843395E-5,7.12078702674452E-5,
7.1640794814688E-5,7.25009999534442E-5,7.34840915405941E-5,7.61056691063271E-5,
8.65919793692592E-5,8.89786567925412E-5,9.40446697643201E-5,9.5733340754913E-5,
9.79849020757036E-5,0.000106991147358866,0.000113571562047154,0.000119834164740894,
0.000121170237394276,0.000122506310047659,0.000125178455354423,0.000130522745967953,
0.000132049686143247,0.000136121526610698,0.000138121518246142,0.000141418986123903,
0.000147599170334999,0.000149659231738698,0.000157899477353493,0.000165007876130263),
 .UNSPECIFIED.) ;
#2207=B_SPLINE_CURVE_WITH_KNOTS('',3,(#152888,#152889,#152890,#152891,#152892,
#152893,#152894,#152895,#152896,#152897,#152898,#152899,#152900,#152901,
#152902,#152903,#152904,#152905,#152906,#152907,#152908,#152909,#152910,
#152911,#152912,#152913,#152914,#152915,#152916,#152917,#152918,#152919,
#152920,#152921,#152922,#152923,#152924,#152925,#152926,#152927,#152928,
#152929,#152930,#152931,#152932,#152933,#152934,#152935,#152936,#152937,
#152938,#152939,#152940,#152941,#152942,#152943,#152944,#152945,#152946,
#152947,#152948,#152949,#152950,#152951,#152952,#152953,#152954,#152955,
#152956,#152957,#152958,#152959,#152960,#152961,#152962,#152963,#152964,
#152965,#152966),.UNSPECIFIED.,.F.,.F.,(4,2,2,2,2,2,2,2,2,1,2,2,2,2,2,2,
2,2,1,2,2,2,2,2,2,2,2,2,2,1,2,2,2,2,2,2,2,2,2,2,4),(-2.04439259789012E-6,
-4.2351647362715E-22,1.16813469870576E-6,2.33626939741152E-6,4.67253879482304E-6,
9.34507758964607E-6,1.56893443514891E-5,2.5897054707274E-5,3.53798289796481E-5,
3.67345110185587E-5,3.74570081059777E-5,3.91084300200782E-5,4.35122217910129E-5,
4.45654530819766E-5,6.26353541312969E-5,6.56193588434229E-5,7.12078702674478E-5,
7.16407948147216E-5,7.25009999534786E-5,7.34840915406294E-5,7.61056691063649E-5,
8.65919793693069E-5,8.89786567925508E-5,9.4044669764314E-5,9.57333407549018E-5,
9.79849020756854E-5,0.00010699114735882,0.00011357156204716,0.000119834164740904,
0.000121170237394285,0.000122506310047666,0.000125178455354429,0.000130522745967953,
0.000132049686143246,0.000136121526610693,0.000138121518246146,0.000141418986123913,
0.00014759917033499,0.000149659231738683,0.000157899477353452,0.000165007876130274),
 .UNSPECIFIED.) ;
#2208=B_SPLINE_CURVE_WITH_KNOTS('',3,(#152969,#152970,#152971,#152972,#152973,
#152974,#152975,#152976,#152977,#152978,#152979,#152980,#152981,#152982,
#152983,#152984,#152985,#152986,#152987,#152988,#152989,#152990,#152991,
#152992,#152993,#152994,#152995,#152996,#152997,#152998,#152999,#153000,
#153001,#153002,#153003,#153004,#153005,#153006,#153007,#153008,#153009,
#153010,#153011,#153012,#153013,#153014,#153015,#153016,#153017,#153018,
#153019,#153020,#153021,#153022,#153023,#153024,#153025,#153026,#153027,
#153028,#153029,#153030,#153031,#153032,#153033,#153034,#153035,#153036,
#153037,#153038,#153039,#153040,#153041,#153042,#153043,#153044,#153045,
#153046,#153047,#153048,#153049),.UNSPECIFIED.,.F.,.F.,(4,2,2,2,2,2,2,2,
2,2,1,2,2,2,2,2,2,2,2,1,2,2,2,2,2,2,2,2,2,2,1,2,2,2,2,2,2,2,2,2,2,4),(-2.04439259789012E-6,
-1.02219629894506E-6,-4.2351647362715E-22,1.16813469870576E-6,2.33626939741152E-6,
4.67253879482304E-6,9.34507758964607E-6,1.56893443514891E-5,2.5897054707274E-5,
3.53798289796481E-5,3.67345110185587E-5,3.74570081059777E-5,3.91084300200782E-5,
4.35122217910129E-5,4.45654530819766E-5,6.26353541222793E-5,6.56193588434281E-5,
7.12078702674497E-5,7.16407948147244E-5,7.2500999953481E-5,7.34840915406315E-5,
7.61056691063659E-5,8.65919793693037E-5,8.89786567925508E-5,9.40446697643295E-5,
9.57333407549224E-5,9.79849020757129E-5,0.000106991147358875,0.000113571562047159,
0.000119834164740904,0.000121170237394286,0.000122506310047668,0.000125178455354432,
0.00013052274596796,0.000132049686143254,0.000136121526610704,0.000138121518246146,
0.000141418986123913,0.000147599170335,0.000149659231738696,0.000157899477353478,
0.000165007876130274),.UNSPECIFIED.) ;
#2209=B_SPLINE_CURVE_WITH_KNOTS('',3,(#153063,#153064,#153065,#153066,#153067,
#153068,#153069,#153070,#153071,#153072,#153073,#153074,#153075,#153076,
#153077,#153078,#153079,#153080,#153081,#153082,#153083,#153084,#153085,
#153086,#153087,#153088,#153089,#153090,#153091,#153092,#153093,#153094,
#153095,#153096,#153097,#153098,#153099,#153100,#153101,#153102,#153103,
#153104,#153105,#153106,#153107,#153108,#153109,#153110,#153111,#153112,
#153113,#153114,#153115,#153116,#153117,#153118,#153119,#153120,#153121,
#153122,#153123,#153124,#153125,#153126,#153127,#153128,#153129,#153130,
#153131,#153132,#153133,#153134,#153135,#153136,#153137,#153138,#153139,
#153140,#153141),.UNSPECIFIED.,.F.,.F.,(4,2,2,2,2,2,2,2,2,1,2,2,2,2,2,2,
2,2,1,2,2,2,2,2,2,2,2,2,2,1,2,2,2,2,2,2,2,2,2,2,4),(-2.04439259789117E-6,
4.2351647362715E-22,1.16813469870585E-6,2.3362693974117E-6,4.67253879482341E-6,
9.34507758964682E-6,1.56893443514892E-5,2.58970547072705E-5,3.53798289796436E-5,
3.67345110185541E-5,3.7457008105973E-5,3.91084300200733E-5,4.35122217910076E-5,
4.45654530819785E-5,6.26353541292637E-5,6.56193588433652E-5,7.12078702674523E-5,
7.16407948146479E-5,7.25009999534026E-5,7.34840915405508E-5,7.61056691062794E-5,
8.65919793691936E-5,8.89786567925488E-5,9.40446697643019E-5,9.57333407548862E-5,
9.79849020756654E-5,0.000106991147358782,0.000113571562047156,0.000119834164740906,
0.000121170237394291,0.000122506310047676,0.000125178455354446,0.000130522745967985,
0.000132049686143282,0.000136121526610741,0.000138121518246147,0.000141418986123914,
0.000147599170334984,0.000149659231738674,0.000157899477353434,0.000165007876130277),
 .UNSPECIFIED.) ;
#2210=B_SPLINE_CURVE_WITH_KNOTS('',3,(#153144,#153145,#153146,#153147,#153148,
#153149,#153150,#153151,#153152,#153153,#153154,#153155,#153156,#153157,
#153158,#153159,#153160,#153161,#153162,#153163,#153164,#153165,#153166,
#153167,#153168,#153169,#153170,#153171,#153172,#153173,#153174,#153175,
#153176,#153177,#153178,#153179,#153180,#153181,#153182,#153183,#153184,
#153185,#153186,#153187,#153188,#153189,#153190,#153191,#153192,#153193,
#153194,#153195,#153196,#153197,#153198,#153199,#153200,#153201,#153202,
#153203,#153204,#153205,#153206,#153207,#153208,#153209,#153210,#153211,
#153212,#153213,#153214,#153215,#153216,#153217,#153218,#153219,#153220,
#153221,#153222,#153223,#153224),.UNSPECIFIED.,.F.,.F.,(4,2,2,2,2,2,2,2,
2,2,1,2,2,2,2,2,2,2,2,1,2,2,2,2,2,2,2,2,2,2,1,2,2,2,2,2,2,2,2,2,2,4),(-2.04439259789012E-6,
-1.02219629894506E-6,-4.2351647362715E-22,1.16813469870576E-6,2.33626939741152E-6,
4.67253879482304E-6,9.34507758964607E-6,1.56893443514891E-5,2.5897054707274E-5,
3.53798289796481E-5,3.67345110185587E-5,3.74570081059777E-5,3.91084300200782E-5,
4.35122217910129E-5,4.45654530819766E-5,6.26353541228085E-5,6.56193588434328E-5,
7.12078702674523E-5,7.16407948147346E-5,7.2500999953492E-5,7.34840915406433E-5,
7.61056691063801E-5,8.65919793693274E-5,8.89786567925508E-5,9.40446697643413E-5,
9.57333407549381E-5,9.79849020757339E-5,0.000106991147358917,0.000113571562047154,
0.000119834164740904,0.000121170237394293,0.000122506310047682,0.000125178455354461,
0.000130522745968017,0.000132049686143319,0.000136121526610791,0.000138121518246147,
0.000141418986123913,0.000147599170334984,0.000149659231738674,0.000157899477353436,
0.000165007876130274),.UNSPECIFIED.) ;
#2211=B_SPLINE_CURVE_WITH_KNOTS('',3,(#153238,#153239,#153240,#153241,#153242,
#153243,#153244,#153245,#153246,#153247,#153248,#153249,#153250,#153251,
#153252,#153253,#153254,#153255,#153256,#153257,#153258,#153259,#153260,
#153261,#153262,#153263,#153264,#153265,#153266,#153267,#153268,#153269,
#153270,#153271,#153272,#153273,#153274,#153275,#153276,#153277,#153278,
#153279,#153280,#153281,#153282,#153283,#153284,#153285,#153286,#153287,
#153288,#153289,#153290,#153291,#153292,#153293,#153294,#153295,#153296,
#153297,#153298,#153299,#153300,#153301,#153302,#153303,#153304,#153305,
#153306,#153307,#153308,#153309,#153310,#153311,#153312,#153313,#153314,
#153315,#153316,#153317,#153318),.UNSPECIFIED.,.F.,.F.,(4,2,2,2,2,2,2,2,
2,2,1,2,2,2,2,2,2,2,2,1,2,2,2,2,2,2,2,2,2,2,1,2,2,2,2,2,2,2,2,2,2,4),(-2.04439259788935E-6,
-1.02219629894467E-6,0.,1.16813469870576E-6,2.33626939741152E-6,4.67253879482303E-6,
9.34507758964606E-6,1.56893443514906E-5,2.5897054707276E-5,3.53798289796491E-5,
3.67345110185596E-5,3.74570081059785E-5,3.91084300200788E-5,4.35122217910131E-5,
4.45654530819802E-5,6.26353541287885E-5,6.56193588433466E-5,7.12078702674531E-5,
7.16407948146223E-5,7.25009999533759E-5,7.3484091540523E-5,7.61056691062484E-5,
8.65919793691503E-5,8.89786567925503E-5,9.40446697643058E-5,9.57333407548909E-5,
9.79849020756711E-5,0.000106991147358792,0.000113571562047162,0.000119834164740905,
0.000121170237394295,0.000122506310047685,0.000125178455354465,0.000130522745968025,
0.000132049686143328,0.000136121526610802,0.000138121518246146,0.000141418986123915,
0.000147599170335001,0.000149659231738696,0.000157899477353478,0.000165007876130276),
 .UNSPECIFIED.) ;
#2212=B_SPLINE_CURVE_WITH_KNOTS('',3,(#153321,#153322,#153323,#153324,#153325,
#153326,#153327,#153328,#153329,#153330,#153331,#153332,#153333,#153334,
#153335,#153336,#153337,#153338,#153339,#153340,#153341,#153342,#153343,
#153344,#153345,#153346,#153347,#153348,#153349,#153350,#153351,#153352,
#153353,#153354,#153355,#153356,#153357,#153358,#153359,#153360,#153361,
#153362,#153363,#153364,#153365,#153366,#153367,#153368,#153369,#153370,
#153371,#153372,#153373,#153374,#153375,#153376,#153377,#153378,#153379,
#153380,#153381,#153382,#153383,#153384,#153385,#153386,#153387,#153388,
#153389,#153390,#153391,#153392,#153393,#153394,#153395,#153396,#153397,
#153398,#153399,#153400),.UNSPECIFIED.,.F.,.F.,(4,1,2,2,2,2,2,2,2,2,1,2,
2,2,2,2,2,2,2,1,2,2,2,2,2,2,2,2,2,2,1,2,2,2,2,2,2,2,2,2,2,4),(-2.04439259788868E-6,
-1.02219629894434E-6,0.,1.16813469870521E-6,2.33626939741041E-6,4.67253879482083E-6,
9.34507758964166E-6,1.56893443514874E-5,2.58970547072727E-5,3.53798289796463E-5,
3.67345110185568E-5,3.74570081059758E-5,3.91084300200762E-5,4.35122217910107E-5,
4.45654530819764E-5,6.26353541299785E-5,6.56193588432828E-5,7.1207870267458E-5,
7.16407948145442E-5,7.25009999532958E-5,7.34840915404405E-5,7.61056691061598E-5,
8.65919793690367E-5,8.89786567925501E-5,9.40446697643433E-5,9.57333407549411E-5,
9.7984902075738E-5,0.000106991147358926,0.000113571562047156,0.0001198341647409,
0.000121170237394275,0.00012250631004765,0.000125178455354399,0.000130522745967899,
0.000132049686143184,0.000136121526610612,0.000138121518246142,0.000141418986123913,
0.000147599170335002,0.000149659231738699,0.000157899477353484,0.000165007876130273),
 .UNSPECIFIED.) ;
#2213=B_SPLINE_CURVE_WITH_KNOTS('',3,(#153414,#153415,#153416,#153417,#153418,
#153419,#153420,#153421,#153422,#153423,#153424,#153425,#153426,#153427,
#153428,#153429,#153430,#153431,#153432,#153433,#153434,#153435,#153436,
#153437,#153438,#153439,#153440,#153441,#153442,#153443,#153444,#153445,
#153446,#153447,#153448,#153449,#153450,#153451,#153452,#153453,#153454,
#153455,#153456,#153457,#153458,#153459,#153460,#153461,#153462,#153463,
#153464,#153465,#153466,#153467,#153468,#153469,#153470,#153471,#153472,
#153473,#153474,#153475,#153476,#153477,#153478,#153479,#153480,#153481,
#153482,#153483,#153484,#153485,#153486,#153487,#153488,#153489,#153490,
#153491,#153492,#153493),.UNSPECIFIED.,.F.,.F.,(4,1,2,2,2,2,2,2,2,2,1,2,
2,2,2,2,2,2,2,1,2,2,2,2,2,2,2,2,2,2,1,2,2,2,2,2,2,2,2,2,2,4),(-2.04439259788983E-6,
-1.02219629894492E-6,0.,1.16813469870562E-6,2.33626939741123E-6,4.67253879482247E-6,
9.34507758964493E-6,1.56893443514854E-5,2.58970547072686E-5,3.537982897964E-5,
3.67345110185502E-5,3.7457008105969E-5,3.9108430020069E-5,4.35122217910025E-5,
4.45654530819757E-5,6.26353541202787E-5,6.56193588433876E-5,7.12078702674454E-5,
7.16407948146769E-5,7.25009999534325E-5,7.34840915405817E-5,7.61056691063131E-5,
8.65919793692386E-5,8.89786567925425E-5,9.40446697643215E-5,9.57333407549146E-5,
9.79849020757052E-5,0.000106991147358868,0.000113571562047158,0.000119834164740895,
0.000121170237394282,0.000122506310047669,0.000125178455354443,0.000130522745967992,
0.000132049686143291,0.000136121526610757,0.000138121518246138,0.000141418986123904,
0.000147599170334986,0.000149659231738681,0.000157899477353457,0.000165007876130264),
 .UNSPECIFIED.) ;
#2214=B_SPLINE_CURVE_WITH_KNOTS('',3,(#153496,#153497,#153498,#153499,#153500,
#153501,#153502,#153503,#153504,#153505,#153506,#153507,#153508,#153509,
#153510,#153511,#153512,#153513,#153514,#153515,#153516,#153517,#153518,
#153519,#153520,#153521,#153522,#153523,#153524,#153525,#153526,#153527,
#153528,#153529,#153530,#153531,#153532,#153533,#153534,#153535,#153536,
#153537,#153538,#153539,#153540,#153541,#153542,#153543,#153544,#153545,
#153546,#153547,#153548,#153549,#153550,#153551,#153552,#153553,#153554,
#153555,#153556,#153557,#153558,#153559,#153560,#153561,#153562,#153563,
#153564,#153565,#153566,#153567,#153568,#153569,#153570,#153571,#153572,
#153573,#153574),.UNSPECIFIED.,.F.,.F.,(4,2,2,2,2,2,2,2,2,1,2,2,2,2,2,2,
2,2,1,2,2,2,2,2,2,2,2,2,2,1,2,2,2,2,2,2,2,2,2,2,4),(-2.04439259789041E-6,
0.,1.16813469870559E-6,2.33626939741119E-6,4.67253879482237E-6,9.34507758964474E-6,
1.56893443514909E-5,2.5897054707274E-5,3.53798289796484E-5,3.6734511018559E-5,
3.74570081059781E-5,3.91084300200786E-5,4.35122217910135E-5,4.4565453081976E-5,
6.26353541290543E-5,6.56193588433348E-5,7.12078702674495E-5,7.16407948146086E-5,
7.2500999953362E-5,7.34840915405088E-5,7.61056691062334E-5,8.6591979369132E-5,
8.89786567925493E-5,9.4044669764311E-5,9.57333407548982E-5,9.79849020756812E-5,
0.000106991147358813,0.00011357156204716,0.000119834164740903,0.000121170237394283,
0.000122506310047663,0.000125178455354423,0.000130522745967942,0.000132049686143234,
0.000136121526610677,0.000138121518246148,0.000141418986123912,0.000147599170335,
0.000149659231738696,0.000157899477353481,0.000165007876130272),
 .UNSPECIFIED.) ;
#2215=B_SPLINE_CURVE_WITH_KNOTS('',3,(#153588,#153589,#153590,#153591,#153592,
#153593,#153594,#153595,#153596,#153597,#153598,#153599,#153600,#153601,
#153602,#153603,#153604,#153605,#153606,#153607,#153608,#153609,#153610,
#153611,#153612,#153613,#153614,#153615,#153616,#153617,#153618,#153619,
#153620,#153621,#153622,#153623,#153624,#153625,#153626,#153627,#153628,
#153629,#153630,#153631,#153632,#153633,#153634,#153635,#153636,#153637),
 .UNSPECIFIED.,.F.,.F.,(4,2,2,2,2,2,2,2,2,2,2,2,2,2,2,2,2,2,2,2,2,2,2,2,
4),(-2.0805332453777E-6,-4.2351647362715E-22,1.73126834661512E-6,3.9646814204225E-6,
7.52178969731448E-6,1.32303807352205E-5,2.25750184175528E-5,3.87948997653525E-5,
5.72571304993316E-5,6.41156850332471E-5,7.29633420187519E-5,7.57300836966873E-5,
9.46996265562493E-5,9.75514675378132E-5,0.000111620796538463,0.000116439892133737,
0.00011740963655672,0.000134179897041995,0.000142027094744273,0.000142768074549612,
0.000154973322948364,0.000157365523939684,0.000159579629273007,0.000173553148905421,
0.000174961243144775),.UNSPECIFIED.) ;
#2216=B_SPLINE_CURVE_WITH_KNOTS('',3,(#153640,#153641,#153642,#153643,#153644,
#153645,#153646,#153647,#153648,#153649,#153650,#153651,#153652,#153653,
#153654,#153655,#153656,#153657,#153658,#153659,#153660,#153661,#153662,
#153663,#153664,#153665,#153666,#153667,#153668,#153669,#153670,#153671,
#153672,#153673,#153674,#153675,#153676,#153677,#153678,#153679,#153680,
#153681,#153682,#153683,#153684,#153685,#153686,#153687,#153688,#153689,
#153690,#153691,#153692,#153693,#153694,#153695,#153696,#153697,#153698,
#153699,#153700,#153701,#153702,#153703,#153704,#153705,#153706,#153707,
#153708,#153709,#153710,#153711,#153712,#153713,#153714,#153715,#153716,
#153717,#153718),.UNSPECIFIED.,.F.,.F.,(4,2,2,2,2,2,2,2,2,1,2,2,2,2,2,2,
2,2,1,2,2,2,2,2,2,2,2,2,2,1,2,2,2,2,2,2,2,2,2,2,4),(-2.04439259789194E-6,
0.,1.16813469870674E-6,2.33626939741348E-6,4.67253879482696E-6,9.34507758965391E-6,
1.5689344351494E-5,2.58970547072731E-5,3.5379828979644E-5,3.67345110185541E-5,
3.74570081059728E-5,3.91084300200728E-5,4.3512221791006E-5,4.45654530819813E-5,
6.26353541219344E-5,6.56193588435038E-5,7.12078702674442E-5,7.16407948148223E-5,
7.25009999535821E-5,7.34840915407362E-5,7.61056691064803E-5,8.65919793694568E-5,
8.8978656792545E-5,9.4044669764307E-5,9.57333407548944E-5,9.79849020756775E-5,
0.00010699114735881,0.000113571562047152,0.000119834164740901,0.000121170237394268,
0.000122506310047635,0.000125178455354369,0.000130522745967838,0.000132049686143115,
0.000136121526610519,0.000138121518246145,0.000141418986123913,0.000147599170334989,
0.000149659231738682,0.00015789947735345,0.000165007876130276),
 .UNSPECIFIED.) ;
#2217=B_SPLINE_CURVE_WITH_KNOTS('',3,(#153914,#153915,#153916,#153917,#153918,
#153919,#153920,#153921,#153922,#153923),.UNSPECIFIED.,.F.,.F.,(4,2,2,2,
4),(0.015568479421891,0.0195166960586068,0.0234649126953226,0.0272193439053862,
0.0309737751154498),.UNSPECIFIED.) ;
#2218=B_SPLINE_CURVE_WITH_KNOTS('',3,(#153927,#153928,#153929,#153930,#153931,
#153932,#153933,#153934,#153935,#153936),.UNSPECIFIED.,.F.,.F.,(4,2,2,2,
4),(-0.0304066187772768,-0.0266397364244227,-0.0228728540715686,-0.0190171760180443,
-0.0151614979645201),.UNSPECIFIED.) ;
#2219=B_SPLINE_CURVE_WITH_KNOTS('',3,(#153940,#153941,#153942,#153943,#153944,
#153945,#153946,#153947,#153948,#153949),.UNSPECIFIED.,.F.,.F.,(4,2,2,2,
4),(-0.045651798047763,-0.0418195667444863,-0.0379873354412096,-0.0341969771092432,
-0.0304066187772768),.UNSPECIFIED.) ;
#2220=B_SPLINE_CURVE_WITH_KNOTS('',3,(#153953,#153954,#153955,#153956,#153957,
#153958,#153959,#153960,#153961,#153962,#153963,#153964,#153965,#153966,
#153967,#153968,#153969,#153970,#153971,#153972,#153973,#153974,#153975,
#153976,#153977,#153978,#153979,#153980,#153981,#153982,#153983),
 .UNSPECIFIED.,.F.,.F.,(4,3,3,3,3,3,3,3,3,3,4),(0.,1.7421454496146E-5,3.27267941377286E-5,
5.03532648038955E-5,6.54304063451112E-5,8.35242149508461E-5,9.84987277349577E-5,
0.000117634019508126,0.000132578862231984,0.000151533502617316,0.000159722162354116),
 .UNSPECIFIED.) ;
#2221=B_SPLINE_CURVE_WITH_KNOTS('',3,(#153987,#153988,#153989,#153990,#153991,
#153992,#153993,#153994,#153995,#153996),.UNSPECIFIED.,.F.,.F.,(4,2,2,2,
4),(0.015568479421891,0.0195166960586069,0.0234649126953227,0.0272193439053863,
0.0309737751154499),.UNSPECIFIED.) ;
#2222=B_SPLINE_CURVE_WITH_KNOTS('',3,(#154000,#154001,#154002,#154003,#154004,
#154005,#154006,#154007,#154008,#154009),.UNSPECIFIED.,.F.,.F.,(4,2,2,2,
4),(-0.0304066810505573,-0.0266163227185909,-0.0228259643866245,-0.0189937330833478,
-0.0151615017800711),.UNSPECIFIED.) ;
#2223=B_SPLINE_CURVE_WITH_KNOTS('',3,(#154013,#154014,#154015,#154016,#154017,
#154018,#154019,#154020,#154021,#154022),.UNSPECIFIED.,.F.,.F.,(4,2,2,2,
4),(-0.045651801863314,-0.0417961238097898,-0.0379404457562656,-0.0341735634034114,
-0.0304066810505573),.UNSPECIFIED.) ;
#2224=B_SPLINE_CURVE_WITH_KNOTS('',3,(#154026,#154027,#154028,#154029,#154030,
#154031,#154032,#154033,#154034,#154035,#154036,#154037,#154038,#154039,
#154040,#154041,#154042,#154043,#154044,#154045,#154046,#154047,#154048,
#154049,#154050,#154051,#154052,#154053,#154054,#154055,#154056),
 .UNSPECIFIED.,.F.,.F.,(4,3,3,3,3,3,3,3,3,3,4),(0.,1.74214544961505E-5,
3.27267941377285E-5,5.03532648039079E-5,6.54304063451121E-5,8.35242149508558E-5,
9.84987277349571E-5,0.000117634019508131,0.000132578862231983,0.0001515335026173,
0.000159722162354115),.UNSPECIFIED.) ;
#2225=B_SPLINE_CURVE_WITH_KNOTS('',3,(#154064,#154065,#154066,#154067,#154068,
#154069,#154070,#154071,#154072,#154073),.UNSPECIFIED.,.F.,.F.,(4,2,2,2,
4),(0.0155684794218909,0.0195166960586067,0.0234649126953226,0.0272193439053862,
0.0309737751154498),.UNSPECIFIED.) ;
#2226=B_SPLINE_CURVE_WITH_KNOTS('',3,(#154077,#154078,#154079,#154080,#154081,
#154082,#154083,#154084,#154085,#154086),.UNSPECIFIED.,.F.,.F.,(4,2,2,2,
4),(-0.0304066187772767,-0.0266397364244226,-0.0228728540715685,-0.0190171760180443,
-0.0151614979645201),.UNSPECIFIED.) ;
#2227=B_SPLINE_CURVE_WITH_KNOTS('',3,(#154090,#154091,#154092,#154093,#154094,
#154095,#154096,#154097,#154098,#154099),.UNSPECIFIED.,.F.,.F.,(4,2,2,2,
4),(-0.0456517980477629,-0.0418195667444862,-0.0379873354412095,-0.0341969771092431,
-0.0304066187772767),.UNSPECIFIED.) ;
#2228=B_SPLINE_CURVE_WITH_KNOTS('',3,(#154103,#154104,#154105,#154106,#154107,
#154108,#154109,#154110,#154111,#154112,#154113,#154114,#154115,#154116,
#154117,#154118,#154119,#154120,#154121,#154122,#154123,#154124,#154125,
#154126,#154127,#154128,#154129,#154130,#154131,#154132,#154133),
 .UNSPECIFIED.,.F.,.F.,(4,3,3,3,3,3,3,3,3,3,4),(0.,1.74214544961512E-5,
3.27267941377284E-5,5.0353264803915E-5,6.54304063451114E-5,8.35242149508516E-5,
9.84987277349568E-5,0.000117634019508137,0.000132578862231983,0.0001515335026173,
0.000159722162354115),.UNSPECIFIED.) ;
#2229=B_SPLINE_CURVE_WITH_KNOTS('',3,(#154137,#154138,#154139,#154140,#154141,
#154142,#154143,#154144,#154145,#154146),.UNSPECIFIED.,.F.,.F.,(4,2,2,2,
4),(0.0155684794218909,0.0195166960586068,0.0234649126953226,0.0272193439053862,
0.0309737751154498),.UNSPECIFIED.) ;
#2230=B_SPLINE_CURVE_WITH_KNOTS('',3,(#154150,#154151,#154152,#154153,#154154,
#154155,#154156,#154157,#154158,#154159),.UNSPECIFIED.,.F.,.F.,(4,2,2,2,
4),(-0.0304066810505572,-0.0266163227185908,-0.0228259643866244,-0.0189937330833477,
-0.015161501780071),.UNSPECIFIED.) ;
#2231=B_SPLINE_CURVE_WITH_KNOTS('',3,(#154163,#154164,#154165,#154166,#154167,
#154168,#154169,#154170,#154171,#154172),.UNSPECIFIED.,.F.,.F.,(4,2,2,2,
4),(-0.0456518018633139,-0.0417961238097897,-0.0379404457562655,-0.0341735634034114,
-0.0304066810505572),.UNSPECIFIED.) ;
#2232=B_SPLINE_CURVE_WITH_KNOTS('',3,(#154176,#154177,#154178,#154179,#154180,
#154181,#154182,#154183,#154184,#154185,#154186,#154187,#154188,#154189,
#154190,#154191,#154192,#154193,#154194,#154195,#154196,#154197,#154198,
#154199,#154200,#154201,#154202,#154203,#154204,#154205,#154206),
 .UNSPECIFIED.,.F.,.F.,(4,3,3,3,3,3,3,3,3,3,4),(0.,1.74214544961498E-5,
3.27267941377288E-5,5.03532648039088E-5,6.54304063451117E-5,8.35242149508504E-5,
9.84987277349565E-5,0.000117634019508152,0.000132578862231984,0.000151533502617308,
0.000159722162354116),.UNSPECIFIED.) ;
#2233=B_SPLINE_CURVE_WITH_KNOTS('',3,(#154214,#154215,#154216,#154217,#154218,
#154219,#154220,#154221,#154222,#154223),.UNSPECIFIED.,.F.,.F.,(4,2,2,2,
4),(0.015568479421891,0.0195166960586068,0.0234649126953226,0.0272193439053862,
0.0309737751154498),.UNSPECIFIED.) ;
#2234=B_SPLINE_CURVE_WITH_KNOTS('',3,(#154227,#154228,#154229,#154230,#154231,
#154232,#154233,#154234,#154235,#154236),.UNSPECIFIED.,.F.,.F.,(4,2,2,2,
4),(-0.0304066187772769,-0.0266397364244227,-0.0228728540715686,-0.0190171760180443,
-0.0151614979645201),.UNSPECIFIED.) ;
#2235=B_SPLINE_CURVE_WITH_KNOTS('',3,(#154240,#154241,#154242,#154243,#154244,
#154245,#154246,#154247,#154248,#154249),.UNSPECIFIED.,.F.,.F.,(4,2,2,2,
4),(-0.0456517980477632,-0.0418195667444864,-0.0379873354412097,-0.0341969771092433,
-0.0304066187772769),.UNSPECIFIED.) ;
#2236=B_SPLINE_CURVE_WITH_KNOTS('',3,(#154253,#154254,#154255,#154256,#154257,
#154258,#154259,#154260,#154261,#154262,#154263,#154264,#154265,#154266,
#154267,#154268,#154269,#154270,#154271,#154272,#154273,#154274,#154275,
#154276,#154277,#154278,#154279,#154280,#154281,#154282,#154283),
 .UNSPECIFIED.,.F.,.F.,(4,3,3,3,3,3,3,3,3,3,4),(0.,1.74214544961577E-5,
3.27267941377284E-5,5.0353264803909E-5,6.54304063451126E-5,8.35242149508578E-5,
9.84987277349568E-5,0.000117634019508136,0.000132578862231983,0.000151533502617318,
0.000159722162354101),.UNSPECIFIED.) ;
#2237=B_SPLINE_CURVE_WITH_KNOTS('',3,(#154287,#154288,#154289,#154290,#154291,
#154292,#154293,#154294,#154295,#154296),.UNSPECIFIED.,.F.,.F.,(4,2,2,2,
4),(0.015568479421891,0.0195166960586068,0.0234649126953226,0.0272193439053862,
0.0309737751154499),.UNSPECIFIED.) ;
#2238=B_SPLINE_CURVE_WITH_KNOTS('',3,(#154300,#154301,#154302,#154303,#154304,
#154305,#154306,#154307,#154308,#154309),.UNSPECIFIED.,.F.,.F.,(4,2,2,2,
4),(-0.0304066810505573,-0.0266163227185909,-0.0228259643866245,-0.0189937330833478,
-0.0151615017800711),.UNSPECIFIED.) ;
#2239=B_SPLINE_CURVE_WITH_KNOTS('',3,(#154313,#154314,#154315,#154316,#154317,
#154318,#154319,#154320,#154321,#154322),.UNSPECIFIED.,.F.,.F.,(4,2,2,2,
4),(-0.045651801863314,-0.0417961238097898,-0.0379404457562655,-0.0341735634034114,
-0.0304066810505573),.UNSPECIFIED.) ;
#2240=B_SPLINE_CURVE_WITH_KNOTS('',3,(#154326,#154327,#154328,#154329,#154330,
#154331,#154332,#154333,#154334,#154335,#154336,#154337,#154338,#154339,
#154340,#154341,#154342,#154343,#154344,#154345,#154346,#154347,#154348,
#154349,#154350,#154351,#154352,#154353,#154354,#154355,#154356),
 .UNSPECIFIED.,.F.,.F.,(4,3,3,3,3,3,3,3,3,3,4),(0.,1.74214544961458E-5,
3.27267941377285E-5,5.03532648039101E-5,6.54304063451128E-5,8.35242149508591E-5,
9.84987277349573E-5,0.000117634019508134,0.000132578862231983,0.000151533502617299,
0.000159722162354101),.UNSPECIFIED.) ;
#2241=B_SPLINE_CURVE_WITH_KNOTS('',3,(#154364,#154365,#154366,#154367,#154368,
#154369,#154370,#154371,#154372,#154373),.UNSPECIFIED.,.F.,.F.,(4,2,2,2,
4),(0.015568479421891,0.0195166960586068,0.0234649126953226,0.0272193439053863,
0.0309737751154499),.UNSPECIFIED.) ;
#2242=B_SPLINE_CURVE_WITH_KNOTS('',3,(#154377,#154378,#154379,#154380,#154381,
#154382,#154383,#154384,#154385,#154386),.UNSPECIFIED.,.F.,.F.,(4,2,2,2,
4),(-0.0304066187772769,-0.0266397364244227,-0.0228728540715686,-0.0190171760180443,
-0.0151614979645201),.UNSPECIFIED.) ;
#2243=B_SPLINE_CURVE_WITH_KNOTS('',3,(#154390,#154391,#154392,#154393,#154394,
#154395,#154396,#154397,#154398,#154399),.UNSPECIFIED.,.F.,.F.,(4,2,2,2,
4),(-0.0456517980477631,-0.0418195667444864,-0.0379873354412096,-0.0341969771092433,
-0.0304066187772769),.UNSPECIFIED.) ;
#2244=B_SPLINE_CURVE_WITH_KNOTS('',3,(#154403,#154404,#154405,#154406,#154407,
#154408,#154409,#154410,#154411,#154412,#154413,#154414,#154415,#154416,
#154417,#154418,#154419,#154420,#154421,#154422,#154423,#154424,#154425,
#154426,#154427,#154428,#154429,#154430,#154431,#154432,#154433),
 .UNSPECIFIED.,.F.,.F.,(4,3,3,3,3,3,3,3,3,3,4),(0.,1.74214544961475E-5,
3.27267941377288E-5,5.03532648039243E-5,6.54304063451135E-5,8.35242149508581E-5,
9.84987277349581E-5,0.000117634019508135,0.000132578862231985,0.000151533502617287,
0.000159722162354101),.UNSPECIFIED.) ;
#2245=B_SPLINE_CURVE_WITH_KNOTS('',3,(#154437,#154438,#154439,#154440,#154441,
#154442,#154443,#154444,#154445,#154446),.UNSPECIFIED.,.F.,.F.,(4,2,2,2,
4),(0.015568479421891,0.0195166960586068,0.0234649126953226,0.0272193439053862,
0.0309737751154498),.UNSPECIFIED.) ;
#2246=B_SPLINE_CURVE_WITH_KNOTS('',3,(#154450,#154451,#154452,#154453,#154454,
#154455,#154456,#154457,#154458,#154459),.UNSPECIFIED.,.F.,.F.,(4,2,2,2,
4),(-0.0304066810505574,-0.026616322718591,-0.0228259643866246,-0.0189937330833478,
-0.0151615017800711),.UNSPECIFIED.) ;
#2247=B_SPLINE_CURVE_WITH_KNOTS('',3,(#154463,#154464,#154465,#154466,#154467,
#154468,#154469,#154470,#154471,#154472),.UNSPECIFIED.,.F.,.F.,(4,2,2,2,
4),(-0.0456518018633141,-0.0417961238097898,-0.0379404457562656,-0.0341735634034115,
-0.0304066810505573),.UNSPECIFIED.) ;
#2248=B_SPLINE_CURVE_WITH_KNOTS('',3,(#154476,#154477,#154478,#154479,#154480,
#154481,#154482,#154483,#154484,#154485,#154486,#154487,#154488,#154489,
#154490,#154491,#154492,#154493,#154494,#154495,#154496,#154497,#154498,
#154499,#154500,#154501,#154502,#154503,#154504,#154505,#154506),
 .UNSPECIFIED.,.F.,.F.,(4,3,3,3,3,3,3,3,3,3,4),(0.,1.74214544961482E-5,
3.27267941377286E-5,5.03532648038853E-5,6.54304063451119E-5,8.3524214950871E-5,
9.84987277349562E-5,0.000117634019508187,0.000132578862231985,0.000151533502617321,
0.000159722162354102),.UNSPECIFIED.) ;
#2249=B_SPLINE_CURVE_WITH_KNOTS('',3,(#154514,#154515,#154516,#154517,#154518,
#154519,#154520,#154521,#154522,#154523),.UNSPECIFIED.,.F.,.F.,(4,2,2,2,
4),(0.0155684794218922,0.0195166960586076,0.023464912695323,0.0272193439053864,
0.0309737751154497),.UNSPECIFIED.) ;
#2250=B_SPLINE_CURVE_WITH_KNOTS('',3,(#154527,#154528,#154529,#154530,#154531,
#154532,#154533,#154534,#154535,#154536),.UNSPECIFIED.,.F.,.F.,(4,2,2,2,
4),(-0.0304066187772768,-0.0266397364244227,-0.0228728540715685,-0.0190171760180443,
-0.0151614979645201),.UNSPECIFIED.) ;
#2251=B_SPLINE_CURVE_WITH_KNOTS('',3,(#154540,#154541,#154542,#154543,#154544,
#154545,#154546,#154547,#154548,#154549),.UNSPECIFIED.,.F.,.F.,(4,2,2,2,
4),(-0.0456517980477629,-0.0418195667444862,-0.0379873354412095,-0.0341969771092431,
-0.0304066187772767),.UNSPECIFIED.) ;
#2252=B_SPLINE_CURVE_WITH_KNOTS('',3,(#154553,#154554,#154555,#154556,#154557,
#154558,#154559,#154560,#154561,#154562,#154563,#154564,#154565,#154566,
#154567,#154568,#154569,#154570,#154571,#154572,#154573,#154574,#154575,
#154576,#154577,#154578,#154579,#154580,#154581,#154582,#154583),
 .UNSPECIFIED.,.F.,.F.,(4,3,3,3,3,3,3,3,3,3,4),(0.,1.74214544961346E-5,
3.27267941377278E-5,5.03532648038744E-5,6.54304063451099E-5,8.35242149508715E-5,
9.84987277349543E-5,0.000117634019508116,0.000132578862231983,0.000151533502617351,
0.000159722162354115),.UNSPECIFIED.) ;
#2253=B_SPLINE_CURVE_WITH_KNOTS('',3,(#154587,#154588,#154589,#154590,#154591,
#154592,#154593,#154594,#154595,#154596),.UNSPECIFIED.,.F.,.F.,(4,2,2,2,
4),(0.0155684794218919,0.0195166960586074,0.0234649126953229,0.0272193439053863,
0.0309737751154497),.UNSPECIFIED.) ;
#2254=B_SPLINE_CURVE_WITH_KNOTS('',3,(#154600,#154601,#154602,#154603,#154604,
#154605,#154606,#154607,#154608,#154609),.UNSPECIFIED.,.F.,.F.,(4,2,2,2,
4),(-0.0304066810505573,-0.0266163227185909,-0.0228259643866245,-0.0189937330833478,
-0.0151615017800711),.UNSPECIFIED.) ;
#2255=B_SPLINE_CURVE_WITH_KNOTS('',3,(#154613,#154614,#154615,#154616,#154617,
#154618,#154619,#154620,#154621,#154622),.UNSPECIFIED.,.F.,.F.,(4,2,2,2,
4),(-0.0456518018633141,-0.0417961238097899,-0.0379404457562657,-0.0341735634034116,
-0.0304066810505575),.UNSPECIFIED.) ;
#2256=B_SPLINE_CURVE_WITH_KNOTS('',3,(#154626,#154627,#154628,#154629,#154630,
#154631,#154632,#154633,#154634,#154635,#154636,#154637,#154638,#154639,
#154640,#154641,#154642,#154643,#154644,#154645,#154646,#154647,#154648,
#154649,#154650,#154651,#154652,#154653,#154654,#154655,#154656),
 .UNSPECIFIED.,.F.,.F.,(4,3,3,3,3,3,3,3,3,3,4),(0.,1.74214544961505E-5,
3.27267941377287E-5,5.03532648039035E-5,6.54304063451121E-5,8.35242149508726E-5,
9.84987277349566E-5,0.000117634019508169,0.000132578862231986,0.000151533502617341,
0.000159722162354098),.UNSPECIFIED.) ;
#2257=B_SPLINE_CURVE_WITH_KNOTS('',3,(#154664,#154665,#154666,#154667,#154668,
#154669,#154670,#154671,#154672,#154673),.UNSPECIFIED.,.F.,.F.,(4,2,2,2,
4),(0.0155684794218919,0.0195166960586075,0.023464912695323,0.0272193439053864,
0.0309737751154497),.UNSPECIFIED.) ;
#2258=B_SPLINE_CURVE_WITH_KNOTS('',3,(#154677,#154678,#154679,#154680,#154681,
#154682,#154683,#154684,#154685,#154686),.UNSPECIFIED.,.F.,.F.,(4,2,2,2,
4),(-0.0304066187772767,-0.0266397364244226,-0.0228728540715685,-0.0190171760180443,
-0.0151614979645201),.UNSPECIFIED.) ;
#2259=B_SPLINE_CURVE_WITH_KNOTS('',3,(#154690,#154691,#154692,#154693,#154694,
#154695,#154696,#154697,#154698,#154699),.UNSPECIFIED.,.F.,.F.,(4,2,2,2,
4),(-0.0456517980477628,-0.0418195667444863,-0.0379873354412098,-0.0341969771092433,
-0.0304066187772768),.UNSPECIFIED.) ;
#2260=B_SPLINE_CURVE_WITH_KNOTS('',3,(#154703,#154704,#154705,#154706,#154707,
#154708,#154709,#154710,#154711,#154712,#154713,#154714,#154715,#154716,
#154717,#154718,#154719,#154720,#154721,#154722,#154723,#154724,#154725,
#154726,#154727,#154728,#154729,#154730,#154731,#154732,#154733),
 .UNSPECIFIED.,.F.,.F.,(4,3,3,3,3,3,3,3,3,3,4),(0.,1.74214544961313E-5,
3.27267941377278E-5,5.03532648038729E-5,6.54304063451099E-5,8.35242149508288E-5,
9.84987277349543E-5,0.000117634019508168,0.000132578862231983,0.000151533502617396,
0.000159722162354101),.UNSPECIFIED.) ;
#2261=B_SPLINE_CURVE_WITH_KNOTS('',3,(#154737,#154738,#154739,#154740,#154741,
#154742,#154743,#154744,#154745,#154746),.UNSPECIFIED.,.F.,.F.,(4,2,2,2,
4),(0.0155684794218909,0.0195166960586067,0.0234649126953226,0.0272193439053862,
0.0309737751154498),.UNSPECIFIED.) ;
#2262=B_SPLINE_CURVE_WITH_KNOTS('',3,(#154750,#154751,#154752,#154753,#154754,
#154755,#154756,#154757,#154758,#154759),.UNSPECIFIED.,.F.,.F.,(4,2,2,2,
4),(-0.0304066810505572,-0.0266163227185908,-0.0228259643866244,-0.0189937330833477,
-0.0151615017800711),.UNSPECIFIED.) ;
#2263=B_SPLINE_CURVE_WITH_KNOTS('',3,(#154763,#154764,#154765,#154766,#154767,
#154768,#154769,#154770,#154771,#154772),.UNSPECIFIED.,.F.,.F.,(4,2,2,2,
4),(-0.0456518018633141,-0.0417961238097899,-0.0379404457562657,-0.0341735634034116,
-0.0304066810505575),.UNSPECIFIED.) ;
#2264=B_SPLINE_CURVE_WITH_KNOTS('',3,(#154776,#154777,#154778,#154779,#154780,
#154781,#154782,#154783,#154784,#154785,#154786,#154787,#154788,#154789,
#154790,#154791,#154792,#154793,#154794,#154795,#154796,#154797,#154798,
#154799,#154800,#154801,#154802,#154803,#154804,#154805,#154806),
 .UNSPECIFIED.,.F.,.F.,(4,3,3,3,3,3,3,3,3,3,4),(0.,1.74214544961324E-5,
3.27267941377287E-5,5.03532648039218E-5,6.54304063451121E-5,8.35242149508849E-5,
9.84987277349566E-5,0.000117634019508209,0.000132578862231986,0.000151533502617305,
0.000159722162354113),.UNSPECIFIED.) ;
#2265=B_SPLINE_CURVE_WITH_KNOTS('',3,(#154814,#154815,#154816,#154817,#154818,
#154819,#154820,#154821,#154822,#154823),.UNSPECIFIED.,.F.,.F.,(4,2,2,2,
4),(0.0155684794218922,0.0195166960586077,0.0234649126953232,0.0272193439053865,
0.0309737751154498),.UNSPECIFIED.) ;
#2266=B_SPLINE_CURVE_WITH_KNOTS('',3,(#154827,#154828,#154829,#154830,#154831,
#154832,#154833,#154834,#154835,#154836),.UNSPECIFIED.,.F.,.F.,(4,2,2,2,
4),(-0.0304066187772767,-0.0266397364244226,-0.0228728540715685,-0.0190171760180443,
-0.0151614979645201),.UNSPECIFIED.) ;
#2267=B_SPLINE_CURVE_WITH_KNOTS('',3,(#154840,#154841,#154842,#154843,#154844,
#154845,#154846,#154847,#154848,#154849),.UNSPECIFIED.,.F.,.F.,(4,2,2,2,
4),(-0.0456517980477626,-0.0418195667444861,-0.0379873354412096,-0.0341969771092432,
-0.0304066187772767),.UNSPECIFIED.) ;
#2268=B_SPLINE_CURVE_WITH_KNOTS('',3,(#154853,#154854,#154855,#154856,#154857,
#154858,#154859,#154860,#154861,#154862,#154863,#154864,#154865,#154866,
#154867,#154868,#154869,#154870,#154871,#154872,#154873,#154874,#154875,
#154876,#154877,#154878,#154879,#154880,#154881,#154882,#154883),
 .UNSPECIFIED.,.F.,.F.,(4,3,3,3,3,3,3,3,3,3,4),(0.,1.74214544961345E-5,
3.27267941377278E-5,5.03532648038844E-5,6.54304063451099E-5,8.3524214950855E-5,
9.84987277349543E-5,0.000117634019508163,0.000132578862231983,0.00015153350261733,
0.000159722162354115),.UNSPECIFIED.) ;
#2269=B_SPLINE_CURVE_WITH_KNOTS('',3,(#154887,#154888,#154889,#154890,#154891,
#154892,#154893,#154894,#154895,#154896),.UNSPECIFIED.,.F.,.F.,(4,2,2,2,
4),(0.0155684794218909,0.0195166960586067,0.0234649126953226,0.0272193439053862,
0.0309737751154498),.UNSPECIFIED.) ;
#2270=B_SPLINE_CURVE_WITH_KNOTS('',3,(#154900,#154901,#154902,#154903,#154904,
#154905,#154906,#154907,#154908,#154909),.UNSPECIFIED.,.F.,.F.,(4,2,2,2,
4),(-0.0304066810505572,-0.0266163227185908,-0.0228259643866244,-0.0189937330833477,
-0.0151615017800711),.UNSPECIFIED.) ;
#2271=B_SPLINE_CURVE_WITH_KNOTS('',3,(#154913,#154914,#154915,#154916,#154917,
#154918,#154919,#154920,#154921,#154922),.UNSPECIFIED.,.F.,.F.,(4,2,2,2,
4),(-0.0456518018633141,-0.0417961238097899,-0.0379404457562657,-0.0341735634034116,
-0.0304066810505575),.UNSPECIFIED.) ;
#2272=B_SPLINE_CURVE_WITH_KNOTS('',3,(#154926,#154927,#154928,#154929,#154930,
#154931,#154932,#154933,#154934,#154935,#154936,#154937,#154938,#154939,
#154940,#154941,#154942,#154943,#154944,#154945,#154946,#154947,#154948,
#154949,#154950,#154951,#154952,#154953,#154954,#154955,#154956),
 .UNSPECIFIED.,.F.,.F.,(4,3,3,3,3,3,3,3,3,3,4),(0.,1.74214544961354E-5,
3.27267941377287E-5,5.03532648039094E-5,6.54304063451121E-5,8.35242149508793E-5,
9.84987277349566E-5,0.000117634019508197,0.000132578862231986,0.000151533502617206,
0.000159722162354098),.UNSPECIFIED.) ;
#2273=B_SPLINE_CURVE_WITH_KNOTS('',3,(#154964,#154965,#154966,#154967,#154968,
#154969,#154970,#154971,#154972,#154973),.UNSPECIFIED.,.F.,.F.,(4,2,2,2,
4),(0.0155684794218921,0.0195166960586076,0.0234649126953232,0.0272193439053865,
0.0309737751154498),.UNSPECIFIED.) ;
#2274=B_SPLINE_CURVE_WITH_KNOTS('',3,(#154977,#154978,#154979,#154980,#154981,
#154982,#154983,#154984,#154985,#154986),.UNSPECIFIED.,.F.,.F.,(4,2,2,2,
4),(-0.0304066187772767,-0.0266397364244226,-0.0228728540715685,-0.0190171760180442,
-0.01516149796452),.UNSPECIFIED.) ;
#2275=B_SPLINE_CURVE_WITH_KNOTS('',3,(#154990,#154991,#154992,#154993,#154994,
#154995,#154996,#154997,#154998,#154999),.UNSPECIFIED.,.F.,.F.,(4,2,2,2,
4),(-0.0456517980477622,-0.0418195667444857,-0.0379873354412092,-0.0341969771092428,
-0.0304066187772765),.UNSPECIFIED.) ;
#2276=B_SPLINE_CURVE_WITH_KNOTS('',3,(#155003,#155004,#155005,#155006,#155007,
#155008,#155009,#155010,#155011,#155012,#155013,#155014,#155015,#155016,
#155017,#155018,#155019,#155020,#155021,#155022,#155023,#155024,#155025,
#155026,#155027,#155028,#155029,#155030,#155031,#155032,#155033),
 .UNSPECIFIED.,.F.,.F.,(4,3,3,3,3,3,3,3,3,3,4),(0.,1.74214544961244E-5,
3.27267941377278E-5,5.03532648038767E-5,6.54304063451099E-5,8.3524214950855E-5,
9.84987277349543E-5,0.000117634019508207,0.000132578862231983,0.000151533502617196,
0.000159722162354101),.UNSPECIFIED.) ;
#2277=B_SPLINE_CURVE_WITH_KNOTS('',3,(#155037,#155038,#155039,#155040,#155041,
#155042,#155043,#155044,#155045,#155046),.UNSPECIFIED.,.F.,.F.,(4,2,2,2,
4),(0.015568479421892,0.0195166960586076,0.0234649126953231,0.0272193439053864,
0.0309737751154497),.UNSPECIFIED.) ;
#2278=B_SPLINE_CURVE_WITH_KNOTS('',3,(#155050,#155051,#155052,#155053,#155054,
#155055,#155056,#155057,#155058,#155059),.UNSPECIFIED.,.F.,.F.,(4,2,2,2,
4),(-0.0304066810505572,-0.0266163227185908,-0.0228259643866244,-0.0189937330833477,
-0.0151615017800711),.UNSPECIFIED.) ;
#2279=B_SPLINE_CURVE_WITH_KNOTS('',3,(#155063,#155064,#155065,#155066,#155067,
#155068,#155069,#155070,#155071,#155072),.UNSPECIFIED.,.F.,.F.,(4,2,2,2,
4),(-0.0456518018633141,-0.0417961238097899,-0.0379404457562657,-0.0341735634034116,
-0.0304066810505575),.UNSPECIFIED.) ;
#2280=B_SPLINE_CURVE_WITH_KNOTS('',3,(#155076,#155077,#155078,#155079,#155080,
#155081,#155082,#155083,#155084,#155085,#155086,#155087,#155088,#155089,
#155090,#155091,#155092,#155093,#155094,#155095,#155096,#155097,#155098,
#155099,#155100,#155101,#155102,#155103,#155104,#155105,#155106),
 .UNSPECIFIED.,.F.,.F.,(4,3,3,3,3,3,3,3,3,3,4),(0.,1.74214544961202E-5,
3.27267941377275E-5,5.03532648039345E-5,6.54304063451101E-5,8.35242149508574E-5,
9.84987277349543E-5,0.000117634019508031,0.000132578862231981,0.000151533502617366,
0.000159722162354098),.UNSPECIFIED.) ;
#2281=B_SPLINE_CURVE_WITH_KNOTS('',3,(#155114,#155115,#155116,#155117,#155118,
#155119,#155120,#155121,#155122,#155123),.UNSPECIFIED.,.F.,.F.,(4,2,2,2,
4),(0.0155684794218921,0.0195166960586076,0.0234649126953232,0.0272193439053865,
0.0309737751154498),.UNSPECIFIED.) ;
#2282=B_SPLINE_CURVE_WITH_KNOTS('',3,(#155127,#155128,#155129,#155130,#155131,
#155132,#155133,#155134,#155135,#155136),.UNSPECIFIED.,.F.,.F.,(4,2,2,2,
4),(-0.0304066187772767,-0.0266397364244226,-0.0228728540715685,-0.0190171760180442,
-0.01516149796452),.UNSPECIFIED.) ;
#2283=B_SPLINE_CURVE_WITH_KNOTS('',3,(#155140,#155141,#155142,#155143,#155144,
#155145,#155146,#155147,#155148,#155149),.UNSPECIFIED.,.F.,.F.,(4,2,2,2,
4),(-0.0456517980477626,-0.041819566744486,-0.0379873354412094,-0.034196977109243,
-0.0304066187772766),.UNSPECIFIED.) ;
#2284=B_SPLINE_CURVE_WITH_KNOTS('',3,(#155153,#155154,#155155,#155156,#155157,
#155158,#155159,#155160,#155161,#155162,#155163,#155164,#155165,#155166,
#155167,#155168,#155169,#155170,#155171,#155172,#155173,#155174,#155175,
#155176,#155177,#155178,#155179,#155180,#155181,#155182,#155183),
 .UNSPECIFIED.,.F.,.F.,(4,3,3,3,3,3,3,3,3,3,4),(0.,1.74214544961506E-5,
3.27267941377281E-5,5.03532648039511E-5,6.54304063451099E-5,8.35242149508654E-5,
9.84987277349558E-5,0.000117634019508106,0.000132578862231983,0.000151533502617118,
0.000159722162354107),.UNSPECIFIED.) ;
#2285=B_SPLINE_CURVE_WITH_KNOTS('',3,(#155187,#155188,#155189,#155190,#155191,
#155192,#155193,#155194,#155195,#155196),.UNSPECIFIED.,.F.,.F.,(4,2,2,2,
4),(0.0155684794218909,0.0195166960586068,0.0234649126953227,0.0272193439053862,
0.0309737751154498),.UNSPECIFIED.) ;
#2286=B_SPLINE_CURVE_WITH_KNOTS('',3,(#155200,#155201,#155202,#155203,#155204,
#155205,#155206,#155207,#155208,#155209),.UNSPECIFIED.,.F.,.F.,(4,2,2,2,
4),(-0.0304066810505572,-0.0266163227185907,-0.0228259643866243,-0.0189937330833476,
-0.0151615017800709),.UNSPECIFIED.) ;
#2287=B_SPLINE_CURVE_WITH_KNOTS('',3,(#155213,#155214,#155215,#155216,#155217,
#155218,#155219,#155220,#155221,#155222),.UNSPECIFIED.,.F.,.F.,(4,2,2,2,
4),(-0.0456518018633141,-0.0417961238097899,-0.0379404457562657,-0.0341735634034116,
-0.0304066810505575),.UNSPECIFIED.) ;
#2288=B_SPLINE_CURVE_WITH_KNOTS('',3,(#155226,#155227,#155228,#155229,#155230,
#155231,#155232,#155233,#155234,#155235,#155236,#155237,#155238,#155239,
#155240,#155241,#155242,#155243,#155244,#155245,#155246,#155247,#155248,
#155249,#155250,#155251,#155252,#155253,#155254,#155255,#155256),
 .UNSPECIFIED.,.F.,.F.,(4,3,3,3,3,3,3,3,3,3,4),(0.,1.74214544961235E-5,
3.27267941377286E-5,5.03532648039153E-5,6.54304063451125E-5,8.35242149508653E-5,
9.84987277349577E-5,0.000117634019508158,0.000132578862231986,0.000151533502617377,
0.000159722162354107),.UNSPECIFIED.) ;
#2289=B_SPLINE_CURVE_WITH_KNOTS('',3,(#155354,#155355,#155356,#155357,#155358,
#155359,#155360,#155361,#155362,#155363),.UNSPECIFIED.,.F.,.F.,(4,2,2,2,
4),(0.015568479421891,0.0195166960586068,0.0234649126953226,0.0272193439053862,
0.0309737751154498),.UNSPECIFIED.) ;
#2290=B_SPLINE_CURVE_WITH_KNOTS('',3,(#155367,#155368,#155369,#155370,#155371,
#155372,#155373,#155374,#155375,#155376),.UNSPECIFIED.,.F.,.F.,(4,2,2,2,
4),(-0.0304066187772769,-0.0266397364244227,-0.0228728540715685,-0.0190171760180443,
-0.0151614979645201),.UNSPECIFIED.) ;
#2291=B_SPLINE_CURVE_WITH_KNOTS('',3,(#155380,#155381,#155382,#155383,#155384,
#155385,#155386,#155387,#155388,#155389),.UNSPECIFIED.,.F.,.F.,(4,2,2,2,
4),(-0.0456517980477631,-0.0418195667444864,-0.0379873354412096,-0.0341969771092432,
-0.0304066187772769),.UNSPECIFIED.) ;
#2292=B_SPLINE_CURVE_WITH_KNOTS('',3,(#155393,#155394,#155395,#155396,#155397,
#155398,#155399,#155400,#155401,#155402,#155403,#155404,#155405,#155406,
#155407,#155408,#155409,#155410,#155411,#155412,#155413,#155414,#155415,
#155416,#155417,#155418,#155419,#155420,#155421,#155422,#155423),
 .UNSPECIFIED.,.F.,.F.,(4,3,3,3,3,3,3,3,3,3,4),(0.,1.74214544961506E-5,
3.27267941377286E-5,5.03532648039032E-5,6.54304063451112E-5,8.35242149508585E-5,
9.8498727734957E-5,0.000117634019508128,0.000132578862231984,0.000151533502617294,
0.000159722162354116),.UNSPECIFIED.) ;
#2293=B_SPLINE_CURVE_WITH_KNOTS('',3,(#155427,#155428,#155429,#155430,#155431,
#155432,#155433,#155434,#155435,#155436),.UNSPECIFIED.,.F.,.F.,(4,2,2,2,
4),(0.015568479421891,0.0195166960586068,0.0234649126953226,0.0272193439053862,
0.0309737751154498),.UNSPECIFIED.) ;
#2294=B_SPLINE_CURVE_WITH_KNOTS('',3,(#155440,#155441,#155442,#155443,#155444,
#155445,#155446,#155447,#155448,#155449),.UNSPECIFIED.,.F.,.F.,(4,2,2,2,
4),(-0.0304066810505573,-0.0266163227185909,-0.0228259643866245,-0.0189937330833478,
-0.0151615017800711),.UNSPECIFIED.) ;
#2295=B_SPLINE_CURVE_WITH_KNOTS('',3,(#155453,#155454,#155455,#155456,#155457,
#155458,#155459,#155460,#155461,#155462),.UNSPECIFIED.,.F.,.F.,(4,2,2,2,
4),(-0.045651801863314,-0.0417961238097898,-0.0379404457562656,-0.0341735634034115,
-0.0304066810505573),.UNSPECIFIED.) ;
#2296=B_SPLINE_CURVE_WITH_KNOTS('',3,(#155466,#155467,#155468,#155469,#155470,
#155471,#155472,#155473,#155474,#155475,#155476,#155477,#155478,#155479,
#155480,#155481,#155482,#155483,#155484,#155485,#155486,#155487,#155488,
#155489,#155490,#155491,#155492,#155493,#155494,#155495,#155496),
 .UNSPECIFIED.,.F.,.F.,(4,3,3,3,3,3,3,3,3,3,4),(0.,1.74214544961524E-5,
3.27267941377286E-5,5.03532648039125E-5,6.54304063451117E-5,8.35242149508611E-5,
9.84987277349575E-5,0.000117634019508132,0.000132578862231984,0.000151533502617307,
0.000159722162354116),.UNSPECIFIED.) ;
#2297=B_SPLINE_CURVE_WITH_KNOTS('',3,(#156379,#156380,#156381,#156382,#156383,
#156384),.UNSPECIFIED.,.F.,.F.,(4,2,4),(3.14159265358979,3.92699081698724,
4.71238898038469),.UNSPECIFIED.) ;
#2298=B_SPLINE_CURVE_WITH_KNOTS('',3,(#156388,#156389,#156390,#156391,#156392,
#156393),.UNSPECIFIED.,.F.,.F.,(4,2,4),(4.71238898038469,5.49778714378214,
6.28318530717959),.UNSPECIFIED.) ;
#2299=B_SPLINE_CURVE_WITH_KNOTS('',3,(#156397,#156398,#156399,#156400,#156401,
#156402),.UNSPECIFIED.,.F.,.F.,(4,2,4),(0.,0.785398163397448,1.5707963267949),
 .UNSPECIFIED.) ;
#2300=B_SPLINE_CURVE_WITH_KNOTS('',3,(#156406,#156407,#156408,#156409,#156410,
#156411),.UNSPECIFIED.,.F.,.F.,(4,2,4),(1.5707963267949,2.35619449019234,
3.14159265358979),.UNSPECIFIED.) ;
#2301=B_SPLINE_CURVE_WITH_KNOTS('',3,(#156479,#156480,#156481,#156482,#156483,
#156484),.UNSPECIFIED.,.F.,.F.,(4,2,4),(3.14159265358979,3.92699081698724,
4.71238898038469),.UNSPECIFIED.) ;
#2302=B_SPLINE_CURVE_WITH_KNOTS('',3,(#156488,#156489,#156490,#156491,#156492,
#156493),.UNSPECIFIED.,.F.,.F.,(4,2,4),(4.71238898038469,5.49778714378214,
6.28318530717959),.UNSPECIFIED.) ;
#2303=B_SPLINE_CURVE_WITH_KNOTS('',3,(#156497,#156498,#156499,#156500,#156501,
#156502),.UNSPECIFIED.,.F.,.F.,(4,2,4),(0.,0.785398163397448,1.5707963267949),
 .UNSPECIFIED.) ;
#2304=B_SPLINE_CURVE_WITH_KNOTS('',3,(#156506,#156507,#156508,#156509,#156510,
#156511),.UNSPECIFIED.,.F.,.F.,(4,2,4),(1.5707963267949,2.35619449019234,
3.14159265358979),.UNSPECIFIED.) ;
#2305=B_SPLINE_CURVE_WITH_KNOTS('',3,(#157479,#157480,#157481,#157482,#157483,
#157484),.UNSPECIFIED.,.F.,.F.,(4,2,4),(4.71238898038469,5.49778714378214,
6.28318530717959),.UNSPECIFIED.) ;
#2306=B_SPLINE_CURVE_WITH_KNOTS('',3,(#157514,#157515,#157516,#157517,#157518,
#157519),.UNSPECIFIED.,.F.,.F.,(4,2,4),(3.14159265358979,3.92699081698724,
4.71238898038469),.UNSPECIFIED.) ;
#2307=B_SPLINE_CURVE_WITH_KNOTS('',3,(#157689,#157690,#157691,#157692,#157693,
#157694,#157695,#157696,#157697,#157698,#157699,#157700,#157701,#157702,
#157703,#157704,#157705,#157706,#157707,#157708,#157709,#157710,#157711,
#157712,#157713,#157714,#157715,#157716,#157717,#157718,#157719,#157720,
#157721,#157722),.UNSPECIFIED.,.F.,.F.,(4,2,2,2,2,2,2,2,2,2,2,2,2,2,2,2,
4),(0.,8.71783727051651E-6,1.76441105356865E-5,3.58270994901032E-5,4.83658434534696E-5,
6.68919645678521E-5,7.05613987999434E-5,8.27232142756399E-5,9.8736263280299E-5,
0.000104111574538336,0.000114567411933631,0.000115616565506963,0.000123791392829713,
0.00012426720927833,0.000126967031952651,0.00013254691974501,0.000134871234237328),
 .UNSPECIFIED.) ;
#2308=B_SPLINE_CURVE_WITH_KNOTS('',3,(#157729,#157730,#157731,#157732,#157733,
#157734,#157735,#157736,#157737,#157738,#157739,#157740,#157741,#157742,
#157743,#157744,#157745,#157746,#157747,#157748,#157749,#157750,#157751,
#157752,#157753,#157754),.UNSPECIFIED.,.F.,.F.,(4,2,2,2,2,2,2,2,2,2,2,2,
4),(0.,5.70004774914365E-6,8.25511347640861E-6,9.93040049428829E-6,2.64556965229606E-5,
3.0587336112473E-5,4.24593515817714E-5,6.43784914888441E-5,7.66562101644909E-5,
9.74321373320278E-5,9.92796257088233E-5,0.000111632960404945,0.000135309975333051),
 .UNSPECIFIED.) ;
#2309=B_SPLINE_CURVE_WITH_KNOTS('',3,(#157757,#157758,#157759,#157760,#157761,
#157762,#157763,#157764,#157765,#157766,#157767,#157768,#157769,#157770,
#157771,#157772,#157773,#157774,#157775,#157776,#157777,#157778,#157779,
#157780,#157781,#157782,#157783,#157784,#157785,#157786,#157787,#157788,
#157789,#157790,#157791,#157792,#157793,#157794,#157795,#157796,#157797,
#157798,#157799,#157800,#157801,#157802,#157803,#157804,#157805,#157806,
#157807,#157808,#157809,#157810,#157811),.UNSPECIFIED.,.F.,.F.,(4,3,3,3,
3,3,3,3,3,3,3,3,3,3,3,3,3,3,4),(0.,1.96170179200463E-5,2.35258500143173E-5,
3.58003153605657E-5,5.29187212185648E-5,5.64435994881288E-5,5.82792926524093E-5,
7.046492538053E-5,8.72923312905478E-5,9.05038369578109E-5,9.22578228185112E-5,
0.000103663146463144,0.000113866005521512,0.000117768598772948,0.000124579094175181,
0.000129312863866852,0.000130178750830806,0.000132692979584748,0.000134419842078312),
 .UNSPECIFIED.) ;
#2310=B_SPLINE_CURVE_WITH_KNOTS('',3,(#157820,#157821,#157822,#157823,#157824,
#157825,#157826,#157827,#157828,#157829,#157830,#157831,#157832,#157833,
#157834,#157835,#157836,#157837,#157838,#157839,#157840,#157841,#157842,
#157843,#157844,#157845),.UNSPECIFIED.,.F.,.F.,(4,2,2,2,2,2,2,2,2,2,2,2,
4),(2.16840434497101E-19,5.55321021973507E-6,8.2551134764302E-6,1.91711188535186E-5,
3.04852632940551E-5,5.08165579103458E-5,5.19149958125389E-5,6.39742577536716E-5,
8.61162395509796E-5,9.85980048375157E-5,0.000117622240611177,0.000125683481931498,
0.000134262298488522),.UNSPECIFIED.) ;
#2311=B_SPLINE_CURVE_WITH_KNOTS('',3,(#161903,#161904,#161905,#161906,#161907,
#161908,#161909,#161910,#161911,#161912,#161913,#161914,#161915,#161916),
 .UNSPECIFIED.,.F.,.F.,(4,2,2,2,2,2,4),(0.784956998631289,0.966941694311738,
1.14311721215536,1.16348181627601,1.34745079132926,1.51752882030803,1.5707963267949),
 .UNSPECIFIED.) ;
#2312=B_SPLINE_CURVE_WITH_KNOTS('',3,(#161918,#161919,#161920,#161921,#161922,
#161923,#161924,#161925,#161926,#161927,#161928,#161929,#161930,#161931),
 .UNSPECIFIED.,.F.,.F.,(4,2,2,2,2,2,4),(1.5707963267949,1.74016540886056,
1.92604436639238,2.10178657601615,2.12292067848492,2.30714825223632,2.35663565495862),
 .UNSPECIFIED.) ;
#2313=B_SPLINE_CURVE_WITH_KNOTS('',3,(#161935,#161936,#161937,#161938,#161939,
#161940,#161941,#161942,#161943,#161944,#161945,#161946,#161947,#161948),
 .UNSPECIFIED.,.F.,.F.,(4,2,2,2,2,2,4),(1.5707963267949,1.74016540886327,
1.92604436640156,2.10178657606191,2.12292067849459,2.30714825224118,2.35663565495873),
 .UNSPECIFIED.) ;
#2314=B_SPLINE_CURVE_WITH_KNOTS('',3,(#161952,#161953,#161954,#161955,#161956,
#161957,#161958,#161959,#161960,#161961,#161962,#161963,#161964,#161965),
 .UNSPECIFIED.,.F.,.F.,(4,2,2,2,2,2,4),(3.92654965222093,4.10853434790149,
4.28470986572121,4.30507446986523,4.48904344491852,4.65912147389766,4.71238898038469),
 .UNSPECIFIED.) ;
#2315=B_SPLINE_CURVE_WITH_KNOTS('',3,(#161968,#161969,#161970,#161971,#161972,
#161973,#161974,#161975,#161976,#161977,#161978,#161979,#161980,#161981),
 .UNSPECIFIED.,.F.,.F.,(4,2,2,2,2,2,4),(4.71238898038469,4.88175806245295,
5.06763701999115,5.24337922965399,5.26451333208407,5.44874090583052,5.49822830854846),
 .UNSPECIFIED.) ;
#2316=B_SPLINE_CURVE_WITH_KNOTS('',3,(#161985,#161986,#161987,#161988,#161989,
#161990,#161991,#161992,#161993,#161994,#161995,#161996,#161997,#161998),
 .UNSPECIFIED.,.F.,.F.,(4,2,2,2,2,2,4),(0.784956998631145,0.96694169431173,
1.14311721212928,1.16348181627549,1.34745079132874,1.51752882030789,1.5707963267949),
 .UNSPECIFIED.) ;
#2317=B_SPLINE_CURVE_WITH_KNOTS('',3,(#162001,#162002,#162003,#162004,#162005,
#162006,#162007,#162008,#162009,#162010,#162011,#162012,#162013,#162014),
 .UNSPECIFIED.,.F.,.F.,(4,2,2,2,2,2,4),(4.71238898038469,4.88175806245252,
5.06763701999072,5.24337922963828,5.26451333208419,5.44874090583056,5.49822830854825),
 .UNSPECIFIED.) ;
#2318=B_SPLINE_CURVE_WITH_KNOTS('',3,(#162018,#162019,#162020,#162021,#162022,
#162023,#162024,#162025,#162026,#162027,#162028,#162029,#162030,#162031),
 .UNSPECIFIED.,.F.,.F.,(4,2,2,2,2,2,4),(3.92654965222105,4.1085343479052,
4.28470986576985,4.30507446986799,4.48904344491476,4.65912147389089,4.71238898038469),
 .UNSPECIFIED.) ;
#2319=B_SPLINE_CURVE_WITH_KNOTS('',3,(#162035,#162036,#162037,#162038,#162039,
#162040,#162041,#162042,#162043,#162044,#162045,#162046,#162047,#162048),
 .UNSPECIFIED.,.F.,.F.,(4,2,2,2,2,2,4),(0.784956998631336,0.966941694311724,
1.14311721213576,1.16348181627607,1.34745079132915,1.51752882030789,1.5707963267949),
 .UNSPECIFIED.) ;
#2320=B_SPLINE_CURVE_WITH_KNOTS('',3,(#162050,#162051,#162052,#162053,#162054,
#162055,#162056,#162057,#162058,#162059,#162060,#162061,#162062,#162063),
 .UNSPECIFIED.,.F.,.F.,(4,2,2,2,2,2,4),(1.5707963267949,1.74016540886059,
1.92604436639241,2.10178657602066,2.122920678485,2.30714825223642,2.35663565495861),
 .UNSPECIFIED.) ;
#2321=B_SPLINE_CURVE_WITH_KNOTS('',3,(#162067,#162068,#162069,#162070,#162071,
#162072,#162073,#162074,#162075,#162076,#162077,#162078,#162079,#162080),
 .UNSPECIFIED.,.F.,.F.,(4,2,2,2,2,2,4),(1.5707963267949,1.74016540886221,
1.92604436639984,2.10178657605964,2.12292067849308,2.30714825223984,2.3566356549586),
 .UNSPECIFIED.) ;
#2322=B_SPLINE_CURVE_WITH_KNOTS('',3,(#162084,#162085,#162086,#162087,#162088,
#162089,#162090,#162091,#162092,#162093,#162094,#162095,#162096,#162097),
 .UNSPECIFIED.,.F.,.F.,(4,2,2,2,2,2,4),(3.92654965222098,4.10853434790153,
4.28470986572269,4.30507446986533,4.48904344491862,4.6591214738977,4.71238898038469),
 .UNSPECIFIED.) ;
#2323=B_SPLINE_CURVE_WITH_KNOTS('',3,(#162100,#162101,#162102,#162103,#162104,
#162105,#162106,#162107,#162108,#162109,#162110,#162111,#162112,#162113),
 .UNSPECIFIED.,.F.,.F.,(4,2,2,2,2,2,4),(4.71238898038469,4.88175806245294,
5.06763701999115,5.24337922965432,5.26451333208408,5.44874090583055,5.49822830854844),
 .UNSPECIFIED.) ;
#2324=B_SPLINE_CURVE_WITH_KNOTS('',3,(#162117,#162118,#162119,#162120,#162121,
#162122,#162123,#162124,#162125,#162126,#162127,#162128,#162129,#162130),
 .UNSPECIFIED.,.F.,.F.,(4,2,2,2,2,2,4),(0.784956998631396,0.96694169431207,
1.14311721213661,1.16348181627586,1.34745079132829,1.51752882030632,1.5707963267949),
 .UNSPECIFIED.) ;
#2325=B_SPLINE_CURVE_WITH_KNOTS('',3,(#162133,#162134,#162135,#162136,#162137,
#162138,#162139,#162140,#162141,#162142,#162143,#162144,#162145,#162146),
 .UNSPECIFIED.,.F.,.F.,(4,2,2,2,2,2,4),(4.71238898038469,4.88175806245104,
5.06763701998726,5.243379229698,5.26451333208011,5.44874090582758,5.49822830854818),
 .UNSPECIFIED.) ;
#2326=B_SPLINE_CURVE_WITH_KNOTS('',3,(#162150,#162151,#162152,#162153,#162154,
#162155,#162156,#162157,#162158,#162159,#162160,#162161,#162162,#162163),
 .UNSPECIFIED.,.F.,.F.,(4,2,2,2,2,2,4),(3.92654965222123,4.1085343479017,
4.28470986568251,4.30507446986548,4.48904344491786,4.65912147389568,4.71238898038469),
 .UNSPECIFIED.) ;
#2327=B_SPLINE_CURVE_WITH_KNOTS('',3,(#162167,#162168,#162169,#162170,#162171,
#162172,#162173,#162174,#162175,#162176,#162177,#162178,#162179,#162180),
 .UNSPECIFIED.,.F.,.F.,(4,2,2,2,2,2,4),(0.784956998631411,0.966941694312594,
1.14311721209517,1.16348181627623,1.3474507913276,1.51752882030504,1.5707963267949),
 .UNSPECIFIED.) ;
#2328=B_SPLINE_CURVE_WITH_KNOTS('',3,(#162182,#162183,#162184,#162185,#162186,
#162187,#162188,#162189,#162190,#162191,#162192,#162193,#162194,#162195),
 .UNSPECIFIED.,.F.,.F.,(4,2,2,2,2,2,4),(1.5707963267949,1.74016540886207,
1.92604436639947,2.10178657612721,2.12292067849245,2.30714825223912,2.35663565495845),
 .UNSPECIFIED.) ;
#2329=B_SPLINE_CURVE_WITH_KNOTS('',3,(#162199,#162200,#162201,#162202,#162203,
#162204,#162205,#162206,#162207,#162208,#162209,#162210,#162211,#162212),
 .UNSPECIFIED.,.F.,.F.,(4,2,2,2,2,2,4),(1.5707963267949,1.74016540886209,
1.92604436639968,2.10178657607307,2.12292067849299,2.30714825223981,2.35663565495851),
 .UNSPECIFIED.) ;
#2330=B_SPLINE_CURVE_WITH_KNOTS('',3,(#162216,#162217,#162218,#162219,#162220,
#162221,#162222,#162223,#162224,#162225,#162226,#162227,#162228,#162229),
 .UNSPECIFIED.,.F.,.F.,(4,2,2,2,2,2,4),(3.92654965222121,4.10853434790169,
4.28470986572592,4.30507446986558,4.48904344491809,4.65912147389607,4.71238898038469),
 .UNSPECIFIED.) ;
#2331=B_SPLINE_CURVE_WITH_KNOTS('',3,(#162232,#162233,#162234,#162235,#162236,
#162237,#162238,#162239,#162240,#162241,#162242,#162243,#162244,#162245),
 .UNSPECIFIED.,.F.,.F.,(4,2,2,2,2,2,4),(4.71238898038469,4.88175806245171,
5.06763701998878,5.24337922965182,5.26451333208185,5.44874090582863,5.49822830854819),
 .UNSPECIFIED.) ;
#2332=B_SPLINE_CURVE_WITH_KNOTS('',3,(#162249,#162250,#162251,#162252,#162253,
#162254,#162255,#162256,#162257,#162258,#162259,#162260,#162261,#162262),
 .UNSPECIFIED.,.F.,.F.,(4,2,2,2,2,2,4),(0.784956998631413,0.966941694312171,
1.14311721212413,1.163481816276,1.34745079132843,1.51752882030641,1.5707963267949),
 .UNSPECIFIED.) ;
#2333=B_SPLINE_CURVE_WITH_KNOTS('',3,(#162265,#162266,#162267,#162268,#162269,
#162270,#162271,#162272,#162273,#162274,#162275,#162276,#162277,#162278),
 .UNSPECIFIED.,.F.,.F.,(4,2,2,2,2,2,4),(4.71238898038469,4.88175806245124,
5.06763701998751,5.24337922969634,5.2645133320804,5.44874090582779,5.49822830854818),
 .UNSPECIFIED.) ;
#2334=B_SPLINE_CURVE_WITH_KNOTS('',3,(#162282,#162283,#162284,#162285,#162286,
#162287,#162288,#162289,#162290,#162291,#162292,#162293,#162294,#162295),
 .UNSPECIFIED.,.F.,.F.,(4,2,2,2,2,2,4),(3.92654965222121,4.10853434790165,
4.28470986568095,4.30507446986543,4.48904344491779,4.65912147389564,4.71238898038469),
 .UNSPECIFIED.) ;
#2335=B_SPLINE_CURVE_WITH_KNOTS('',3,(#162299,#162300,#162301,#162302,#162303,
#162304,#162305,#162306,#162307,#162308,#162309,#162310,#162311,#162312),
 .UNSPECIFIED.,.F.,.F.,(4,2,2,2,2,2,4),(0.784956998631375,0.966941694312727,
1.14311721209632,1.16348181627625,1.34745079132752,1.51752882030494,1.5707963267949),
 .UNSPECIFIED.) ;
#2336=B_SPLINE_CURVE_WITH_KNOTS('',3,(#162314,#162315,#162316,#162317,#162318,
#162319,#162320,#162321,#162322,#162323,#162324,#162325,#162326,#162327),
 .UNSPECIFIED.,.F.,.F.,(4,2,2,2,2,2,4),(1.5707963267949,1.74016540886203,
1.9260443663994,2.10178657612866,2.1229206784924,2.30714825223906,2.35663565495846),
 .UNSPECIFIED.) ;
#2337=B_SPLINE_CURVE_WITH_KNOTS('',3,(#162331,#162332,#162333,#162334,#162335,
#162336,#162337,#162338,#162339,#162340,#162341,#162342,#162343,#162344),
 .UNSPECIFIED.,.F.,.F.,(4,2,2,2,2,2,4),(1.5707963267949,1.74016540886207,
1.92604436639964,2.10178657606564,2.122920678493,2.30714825223986,2.35663565495852),
 .UNSPECIFIED.) ;
#2338=B_SPLINE_CURVE_WITH_KNOTS('',3,(#162348,#162349,#162350,#162351,#162352,
#162353,#162354,#162355,#162356,#162357,#162358,#162359,#162360,#162361),
 .UNSPECIFIED.,.F.,.F.,(4,2,2,2,2,2,4),(3.92654965222121,4.10853434790162,
4.28470986571305,4.30507446986553,4.48904344491808,4.65912147389608,4.71238898038469),
 .UNSPECIFIED.) ;
#2339=B_SPLINE_CURVE_WITH_KNOTS('',3,(#162364,#162365,#162366,#162367,#162368,
#162369,#162370,#162371,#162372,#162373,#162374,#162375,#162376,#162377),
 .UNSPECIFIED.,.F.,.F.,(4,2,2,2,2,2,4),(4.71238898038469,4.88175806245168,
5.06763701998876,5.24337922964848,5.26451333208179,5.44874090582859,5.49822830854817),
 .UNSPECIFIED.) ;
#2340=B_SPLINE_CURVE_WITH_KNOTS('',3,(#162381,#162382,#162383,#162384,#162385,
#162386,#162387,#162388,#162389,#162390,#162391,#162392,#162393,#162394),
 .UNSPECIFIED.,.F.,.F.,(4,2,2,2,2,2,4),(0.784956998631362,0.966941694311931,
1.14311721213235,1.16348181627574,1.34745079132811,1.51752882030616,1.5707963267949),
 .UNSPECIFIED.) ;
#2341=B_SPLINE_CURVE_WITH_KNOTS('',3,(#162397,#162398,#162399,#162400,#162401,
#162402,#162403,#162404,#162405,#162406,#162407,#162408,#162409,#162410),
 .UNSPECIFIED.,.F.,.F.,(4,2,2,2,2,2,4),(4.71238898038469,4.88175806245117,
5.06763701998738,5.24337922970193,5.26451333208026,5.44874090582769,5.49822830854819),
 .UNSPECIFIED.) ;
#2342=B_SPLINE_CURVE_WITH_KNOTS('',3,(#162414,#162415,#162416,#162417,#162418,
#162419,#162420,#162421,#162422,#162423,#162424,#162425,#162426,#162427),
 .UNSPECIFIED.,.F.,.F.,(4,2,2,2,2,2,4),(3.92654965222123,4.1085343479017,
4.28470986570811,4.30507446986548,4.48904344491786,4.65912147389568,4.71238898038469),
 .UNSPECIFIED.) ;
#2343=B_SPLINE_CURVE_WITH_KNOTS('',3,(#162431,#162432,#162433,#162434,#162435,
#162436,#162437,#162438,#162439,#162440,#162441,#162442,#162443,#162444),
 .UNSPECIFIED.,.F.,.F.,(4,2,2,2,2,2,4),(0.784956998631398,0.966941694312289,
1.14311721210181,1.16348181627595,1.34745079132735,1.51752882030477,1.5707963267949),
 .UNSPECIFIED.) ;
#2344=B_SPLINE_CURVE_WITH_KNOTS('',3,(#162446,#162447,#162448,#162449,#162450,
#162451,#162452,#162453,#162454,#162455,#162456,#162457,#162458,#162459),
 .UNSPECIFIED.,.F.,.F.,(4,2,2,2,2,2,4),(1.5707963267949,1.74016540886207,
1.92604436639947,2.10178657613724,2.12292067849245,2.3071482522391,2.35663565495846),
 .UNSPECIFIED.) ;
#2345=B_SPLINE_CURVE_WITH_KNOTS('',3,(#162463,#162464,#162465,#162466,#162467,
#162468,#162469,#162470,#162471,#162472,#162473,#162474,#162475,#162476),
 .UNSPECIFIED.,.F.,.F.,(4,2,2,2,2,2,4),(1.5707963267949,1.74016540886204,
1.9260443663996,2.10178657605896,2.12292067849293,2.30714825223977,2.35663565495851),
 .UNSPECIFIED.) ;
#2346=B_SPLINE_CURVE_WITH_KNOTS('',3,(#162480,#162481,#162482,#162483,#162484,
#162485,#162486,#162487,#162488,#162489,#162490,#162491,#162492,#162493),
 .UNSPECIFIED.,.F.,.F.,(4,2,2,2,2,2,4),(3.92654965222119,4.10853434790172,
4.28470986572196,4.3050744698657,4.48904344491821,4.6591214738962,4.71238898038469),
 .UNSPECIFIED.) ;
#2347=B_SPLINE_CURVE_WITH_KNOTS('',3,(#162496,#162497,#162498,#162499,#162500,
#162501,#162502,#162503,#162504,#162505,#162506,#162507,#162508,#162509),
 .UNSPECIFIED.,.F.,.F.,(4,2,2,2,2,2,4),(4.71238898038469,4.88175806245162,
5.06763701998873,5.2433792296528,5.26451333208183,5.44874090582879,5.49822830854821),
 .UNSPECIFIED.) ;
#2348=B_SPLINE_CURVE_WITH_KNOTS('',3,(#162513,#162514,#162515,#162516,#162517,
#162518,#162519,#162520,#162521,#162522,#162523,#162524,#162525,#162526),
 .UNSPECIFIED.,.F.,.F.,(4,2,2,2,2,2,4),(0.784956998631419,0.966941694312359,
1.14311721212337,1.16348181627619,1.34745079132836,1.51752882030628,1.5707963267949),
 .UNSPECIFIED.) ;
#2349=B_SPLINE_CURVE_WITH_KNOTS('',3,(#162529,#162530,#162531,#162532,#162533,
#162534,#162535,#162536,#162537,#162538,#162539,#162540,#162541,#162542),
 .UNSPECIFIED.,.F.,.F.,(4,2,2,2,2,2,4),(4.71238898038469,4.88175806245117,
5.06763701998736,5.24337922970041,5.26451333208017,5.44874090582767,5.49822830854818),
 .UNSPECIFIED.) ;
#2350=B_SPLINE_CURVE_WITH_KNOTS('',3,(#162546,#162547,#162548,#162549,#162550,
#162551,#162552,#162553,#162554,#162555,#162556,#162557,#162558,#162559),
 .UNSPECIFIED.,.F.,.F.,(4,2,2,2,2,2,4),(3.92654965222123,4.10853434790176,
4.28470986571068,4.30507446986555,4.48904344491787,4.65912147389569,4.71238898038469),
 .UNSPECIFIED.) ;
#2351=B_SPLINE_CURVE_WITH_KNOTS('',3,(#162563,#162564,#162565,#162566,#162567,
#162568,#162569,#162570,#162571,#162572,#162573,#162574,#162575,#162576),
 .UNSPECIFIED.,.F.,.F.,(4,2,2,2,2,2,4),(0.784956998631419,0.966941694312394,
1.14311721209636,1.16348181627596,1.34745079132737,1.51752882030475,1.5707963267949),
 .UNSPECIFIED.) ;
#2352=B_SPLINE_CURVE_WITH_KNOTS('',3,(#162578,#162579,#162580,#162581,#162582,
#162583,#162584,#162585,#162586,#162587,#162588,#162589,#162590,#162591),
 .UNSPECIFIED.,.F.,.F.,(4,2,2,2,2,2,4),(1.5707963267949,1.74016540886206,
1.92604436639944,2.1017865761314,2.1229206784924,2.30714825223909,2.35663565495846),
 .UNSPECIFIED.) ;
#2353=B_SPLINE_CURVE_WITH_KNOTS('',3,(#162595,#162596,#162597,#162598,#162599,
#162600,#162601,#162602,#162603,#162604,#162605,#162606,#162607,#162608),
 .UNSPECIFIED.,.F.,.F.,(4,2,2,2,2,2,4),(1.5707963267949,1.74016540886189,
1.92604436639889,2.10178657606285,2.12292067849207,2.30714825223932,2.35663565495855),
 .UNSPECIFIED.) ;
#2354=B_SPLINE_CURVE_WITH_KNOTS('',3,(#162612,#162613,#162614,#162615,#162616,
#162617,#162618,#162619,#162620,#162621,#162622,#162623,#162624,#162625),
 .UNSPECIFIED.,.F.,.F.,(4,2,2,2,2,2,4),(3.92654965222116,4.10853434790171,
4.28470986572152,4.30507446986565,4.48904344491819,4.65912147389622,4.71238898038469),
 .UNSPECIFIED.) ;
#2355=B_SPLINE_CURVE_WITH_KNOTS('',3,(#162628,#162629,#162630,#162631,#162632,
#162633,#162634,#162635,#162636,#162637,#162638,#162639,#162640,#162641),
 .UNSPECIFIED.,.F.,.F.,(4,2,2,2,2,2,4),(4.71238898038469,4.88175806245176,
5.06763701998884,5.24337922965909,5.26451333208186,5.44874090582875,5.49822830854823),
 .UNSPECIFIED.) ;
#2356=B_SPLINE_CURVE_WITH_KNOTS('',3,(#162645,#162646,#162647,#162648,#162649,
#162650,#162651,#162652,#162653,#162654,#162655,#162656,#162657,#162658),
 .UNSPECIFIED.,.F.,.F.,(4,2,2,2,2,2,4),(0.784956998631252,0.966941694313067,
1.14311721213665,1.16348181627663,1.34745079132838,1.51752882030642,1.5707963267949),
 .UNSPECIFIED.) ;
#2357=B_SPLINE_CURVE_WITH_KNOTS('',3,(#162661,#162662,#162663,#162664,#162665,
#162666,#162667,#162668,#162669,#162670,#162671,#162672,#162673,#162674),
 .UNSPECIFIED.,.F.,.F.,(4,2,2,2,2,2,4),(4.71238898038469,4.88175806245219,
5.06763701999001,5.24337922963567,5.26451333208336,5.44874090582993,5.4982283085483),
 .UNSPECIFIED.) ;
#2358=B_SPLINE_CURVE_WITH_KNOTS('',3,(#162678,#162679,#162680,#162681,#162682,
#162683,#162684,#162685,#162686,#162687,#162688,#162689,#162690,#162691),
 .UNSPECIFIED.,.F.,.F.,(4,2,2,2,2,2,4),(3.92654965222115,4.10853434790203,
4.28470986568823,4.3050744698658,4.48904344491754,4.65912147389529,4.71238898038469),
 .UNSPECIFIED.) ;
#2359=B_SPLINE_CURVE_WITH_KNOTS('',3,(#162695,#162696,#162697,#162698,#162699,
#162700,#162701,#162702,#162703,#162704,#162705,#162706,#162707,#162708),
 .UNSPECIFIED.,.F.,.F.,(4,2,2,2,2,2,4),(0.784956998631286,0.966941694311768,
1.14311721213309,1.16348181627596,1.34745079132886,1.5175288203073,1.5707963267949),
 .UNSPECIFIED.) ;
#2360=B_SPLINE_CURVE_WITH_KNOTS('',3,(#162710,#162711,#162712,#162713,#162714,
#162715,#162716,#162717,#162718,#162719,#162720,#162721,#162722,#162723),
 .UNSPECIFIED.,.F.,.F.,(4,2,2,2,2,2,4),(1.5707963267949,1.74016540886205,
1.926044366399,2.10178657613527,2.12292067849206,2.30714825223934,2.35663565495854),
 .UNSPECIFIED.) ;
#2361=B_SPLINE_CURVE_WITH_KNOTS('',3,(#162727,#162728,#162729,#162730,#162731,
#162732,#162733,#162734,#162735,#162736,#162737,#162738,#162739,#162740),
 .UNSPECIFIED.,.F.,.F.,(4,2,2,2,2,2,4),(1.5707963267949,1.74016540886187,
1.9260443663989,2.10178657606494,2.1229206784921,2.30714825223936,2.35663565495855),
 .UNSPECIFIED.) ;
#2362=B_SPLINE_CURVE_WITH_KNOTS('',3,(#162744,#162745,#162746,#162747,#162748,
#162749,#162750,#162751,#162752,#162753,#162754,#162755,#162756,#162757),
 .UNSPECIFIED.,.F.,.F.,(4,2,2,2,2,2,4),(3.92654965222115,4.10853434790176,
4.28470986571692,4.3050744698657,4.48904344491822,4.65912147389629,4.71238898038469),
 .UNSPECIFIED.) ;
#2363=B_SPLINE_CURVE_WITH_KNOTS('',3,(#162760,#162761,#162762,#162763,#162764,
#162765,#162766,#162767,#162768,#162769,#162770,#162771,#162772,#162773),
 .UNSPECIFIED.,.F.,.F.,(4,2,2,2,2,2,4),(4.71238898038469,4.88175806245178,
5.06763701998822,5.24337922965634,5.26451333208117,5.44874090582883,5.4982283085483),
 .UNSPECIFIED.) ;
#2364=B_SPLINE_CURVE_WITH_KNOTS('',3,(#162777,#162778,#162779,#162780,#162781,
#162782,#162783,#162784,#162785,#162786,#162787,#162788,#162789,#162790),
 .UNSPECIFIED.,.F.,.F.,(4,2,2,2,2,2,4),(0.784956998631253,0.966941694312816,
1.1431172121299,1.16348181627639,1.34745079132795,1.51752882030599,1.5707963267949),
 .UNSPECIFIED.) ;
#2365=B_SPLINE_CURVE_WITH_KNOTS('',3,(#162793,#162794,#162795,#162796,#162797,
#162798,#162799,#162800,#162801,#162802,#162803,#162804,#162805,#162806),
 .UNSPECIFIED.,.F.,.F.,(4,2,2,2,2,2,4),(4.71238898038469,4.88175806245208,
5.06763701998989,5.24337922963223,5.26451333208325,5.4487409058299,5.49822830854831),
 .UNSPECIFIED.) ;
#2366=B_SPLINE_CURVE_WITH_KNOTS('',3,(#162810,#162811,#162812,#162813,#162814,
#162815,#162816,#162817,#162818,#162819,#162820,#162821,#162822,#162823),
 .UNSPECIFIED.,.F.,.F.,(4,2,2,2,2,2,4),(3.92654965222114,4.10853434790186,
4.2847098656881,4.30507446986561,4.48904344491734,4.65912147389511,4.71238898038469),
 .UNSPECIFIED.) ;
#2367=B_SPLINE_CURVE_WITH_KNOTS('',3,(#162827,#162828,#162829,#162830,#162831,
#162832,#162833,#162834,#162835,#162836,#162837,#162838,#162839,#162840),
 .UNSPECIFIED.,.F.,.F.,(4,2,2,2,2,2,4),(0.784956998631275,0.966941694311846,
1.14311721212765,1.16348181627603,1.34745079132913,1.51752882030757,1.5707963267949),
 .UNSPECIFIED.) ;
#2368=B_SPLINE_CURVE_WITH_KNOTS('',3,(#162842,#162843,#162844,#162845,#162846,
#162847,#162848,#162849,#162850,#162851,#162852,#162853,#162854,#162855),
 .UNSPECIFIED.,.F.,.F.,(4,2,2,2,2,2,4),(1.5707963267949,1.74016540886206,
1.92604436639903,2.10178657606026,2.12292067849211,2.30714825223937,2.35663565495855),
 .UNSPECIFIED.) ;
#2369=B_SPLINE_CURVE_WITH_KNOTS('',3,(#162859,#162860,#162861,#162862,#162863,
#162864,#162865,#162866,#162867,#162868,#162869,#162870,#162871,#162872),
 .UNSPECIFIED.,.F.,.F.,(4,2,2,2,2,2,4),(1.5707963267949,1.74016540886233,
1.92604436640004,2.10178657606526,2.12292067849322,2.30714825223986,2.35663565495855),
 .UNSPECIFIED.) ;
#2370=B_SPLINE_CURVE_WITH_KNOTS('',3,(#162876,#162877,#162878,#162879,#162880,
#162881,#162882,#162883,#162884,#162885,#162886,#162887,#162888,#162889),
 .UNSPECIFIED.,.F.,.F.,(4,2,2,2,2,2,4),(3.92654965222116,4.10853434790169,
4.28470986572823,4.30507446986562,4.48904344491821,4.65912147389623,4.71238898038469),
 .UNSPECIFIED.) ;
#2371=B_SPLINE_CURVE_WITH_KNOTS('',3,(#162892,#162893,#162894,#162895,#162896,
#162897,#162898,#162899,#162900,#162901,#162902,#162903,#162904,#162905),
 .UNSPECIFIED.,.F.,.F.,(4,2,2,2,2,2,4),(4.71238898038469,4.88175806245184,
5.06763701998833,5.24337922965272,5.26451333208122,5.44874090582878,5.49822830854832),
 .UNSPECIFIED.) ;
#2372=B_SPLINE_CURVE_WITH_KNOTS('',3,(#162909,#162910,#162911,#162912,#162913,
#162914,#162915,#162916,#162917,#162918,#162919,#162920,#162921,#162922),
 .UNSPECIFIED.,.F.,.F.,(4,2,2,2,2,2,4),(0.784956998631356,0.966941694311965,
1.14311721213089,1.16348181627574,1.34745079132755,1.51752882030535,1.5707963267949),
 .UNSPECIFIED.) ;
#2373=B_SPLINE_CURVE_WITH_KNOTS('',3,(#162925,#162926,#162927,#162928,#162929,
#162930,#162931,#162932,#162933,#162934,#162935,#162936,#162937,#162938),
 .UNSPECIFIED.,.F.,.F.,(4,2,2,2,2,2,4),(4.71238898038469,4.88175806245187,
5.06763701998943,5.24337922964722,5.26451333208265,5.44874090582937,5.49822830854828),
 .UNSPECIFIED.) ;
#2374=B_SPLINE_CURVE_WITH_KNOTS('',3,(#162942,#162943,#162944,#162945,#162946,
#162947,#162948,#162949,#162950,#162951,#162952,#162953,#162954,#162955),
 .UNSPECIFIED.,.F.,.F.,(4,2,2,2,2,2,4),(3.92654965222114,4.10853434790249,
4.28470986571866,4.30507446986622,4.48904344491771,4.65912147389542,4.71238898038469),
 .UNSPECIFIED.) ;
#2375=B_SPLINE_CURVE_WITH_KNOTS('',3,(#163030,#163031,#163032,#163033,#163034,
#163035),.UNSPECIFIED.,.F.,.F.,(4,2,4),(4.71238898038469,5.49778714378214,
6.28318530717959),.UNSPECIFIED.) ;
#2376=B_SPLINE_CURVE_WITH_KNOTS('',3,(#163065,#163066,#163067,#163068,#163069,
#163070),.UNSPECIFIED.,.F.,.F.,(4,2,4),(3.14159265358979,3.92699081698724,
4.71238898038469),.UNSPECIFIED.) ;
#2377=B_SPLINE_CURVE_WITH_KNOTS('',3,(#167426,#167427,#167428,#167429,#167430,
#167431,#167432,#167433,#167434,#167435,#167436,#167437,#167438,#167439,
#167440,#167441,#167442,#167443,#167444,#167445,#167446,#167447,#167448,
#167449,#167450,#167451),.UNSPECIFIED.,.F.,.F.,(4,2,2,2,2,2,2,2,2,2,2,2,
4),(6.1331736667335E-19,5.70004774914534E-6,8.25511347640713E-6,9.93040049428836E-6,
2.64556965228396E-5,3.0587336112471E-5,4.24593515817707E-5,6.43784914888407E-5,
7.6656210164489E-5,9.74321373319979E-5,9.92796257088188E-5,0.000111632960404942,
0.000135309975333047),.UNSPECIFIED.) ;
#2378=B_SPLINE_CURVE_WITH_KNOTS('',3,(#167458,#167459,#167460,#167461,#167462,
#167463,#167464,#167465,#167466,#167467,#167468,#167469,#167470,#167471,
#167472,#167473,#167474,#167475,#167476,#167477,#167478,#167479,#167480,
#167481,#167482,#167483,#167484,#167485,#167486,#167487,#167488,#167489,
#167490,#167491),.UNSPECIFIED.,.F.,.F.,(4,2,2,2,2,2,2,2,2,2,2,2,2,2,2,2,
4),(0.,8.71783727051893E-6,1.76441105360345E-5,3.58270994901034E-5,4.83658434534685E-5,
6.68919645679043E-5,7.05613987999435E-5,8.27232142756391E-5,9.87362632805838E-5,
0.000104111574538336,0.000114567411933464,0.000115616565506961,0.000123791392829615,
0.000124267209278334,0.000126967031952647,0.000132546919744955,0.000134871234237328),
 .UNSPECIFIED.) ;
#2379=B_SPLINE_CURVE_WITH_KNOTS('',3,(#167493,#167494,#167495,#167496,#167497,
#167498,#167499,#167500,#167501,#167502,#167503,#167504,#167505,#167506,
#167507,#167508,#167509,#167510,#167511,#167512,#167513,#167514,#167515,
#167516,#167517,#167518),.UNSPECIFIED.,.F.,.F.,(4,2,2,2,2,2,2,2,2,2,2,2,
4),(4.33680868994202E-19,5.700047749144E-6,8.25511347640865E-6,9.93040049428814E-6,
2.64556965230734E-5,3.05873361124735E-5,4.24593515817708E-5,6.43784914888414E-5,
7.66562101644896E-5,9.74321373319674E-5,9.92796257088195E-5,0.000111632960404942,
0.000135309975333047),.UNSPECIFIED.) ;
#2380=B_SPLINE_CURVE_WITH_KNOTS('',3,(#167522,#167523,#167524,#167525,#167526,
#167527,#167528,#167529,#167530,#167531,#167532,#167533,#167534,#167535,
#167536,#167537,#167538,#167539,#167540,#167541,#167542,#167543,#167544,
#167545,#167546,#167547),.UNSPECIFIED.,.F.,.F.,(4,2,2,2,2,2,2,2,2,2,2,2,
4),(9.69739903612216E-19,5.70004774917064E-6,8.25511347641042E-6,9.93040049429001E-6,
2.64556965230525E-5,3.05873361124729E-5,4.24593515817735E-5,6.43784914888468E-5,
7.6656210164492E-5,9.74321373319885E-5,9.92796257088266E-5,0.000111632960404945,
0.000135309975333051),.UNSPECIFIED.) ;
#2381=B_SPLINE_CURVE_WITH_KNOTS('',3,(#167554,#167555,#167556,#167557,#167558,
#167559,#167560,#167561,#167562,#167563,#167564,#167565,#167566,#167567,
#167568,#167569,#167570,#167571,#167572,#167573,#167574,#167575,#167576,
#167577,#167578,#167579,#167580,#167581,#167582,#167583,#167584,#167585,
#167586,#167587),.UNSPECIFIED.,.F.,.F.,(4,2,2,2,2,2,2,2,2,2,2,2,2,2,2,2,
4),(0.,8.71783727085515E-6,1.7644110536621E-5,3.58270994901043E-5,4.83658434534726E-5,
6.68919645677967E-5,7.05613987999456E-5,8.27232142756448E-5,9.87362632804046E-5,
0.000104111574538337,0.00011456741193359,0.000115616565506969,0.000123791392829788,
0.000124267209278257,0.00012696703195266,0.000132546919745185,0.000134871234237334),
 .UNSPECIFIED.) ;
#2382=B_SPLINE_CURVE_WITH_KNOTS('',3,(#167591,#167592,#167593,#167594,#167595,
#167596,#167597,#167598,#167599,#167600,#167601,#167602,#167603,#167604,
#167605,#167606,#167607,#167608,#167609,#167610,#167611,#167612,#167613,
#167614,#167615,#167616),.UNSPECIFIED.,.F.,.F.,(4,2,2,2,2,2,2,2,2,2,2,2,
4),(9.69739903612216E-19,5.70004774915885E-6,8.25511347641042E-6,9.93040049429001E-6,
2.64556965230698E-5,3.05873361124735E-5,4.24593515817735E-5,6.43784914888452E-5,
7.6656210164492E-5,9.74321373321103E-5,9.92796257088256E-5,0.000111632960404945,
0.000135309975333051),.UNSPECIFIED.) ;
#2383=B_SPLINE_CURVE_WITH_KNOTS('',3,(#167623,#167624,#167625,#167626,#167627,
#167628,#167629,#167630,#167631,#167632,#167633,#167634,#167635,#167636,
#167637,#167638,#167639,#167640,#167641,#167642,#167643,#167644,#167645,
#167646,#167647,#167648,#167649,#167650,#167651,#167652,#167653,#167654,
#167655,#167656),.UNSPECIFIED.,.F.,.F.,(4,2,2,2,2,2,2,2,2,2,2,2,2,2,2,2,
4),(0.,8.717837270643E-6,1.76441105351036E-5,3.58270994901016E-5,4.83658434534694E-5,
6.68919645660009E-5,7.05613987999433E-5,8.27232142756404E-5,9.8736263280134E-5,
0.000104111574538333,0.000114567411932816,0.000115616565506965,0.000123791392829682,
0.000124267209278245,0.000126967031952653,0.000132546919745188,0.00013487123423733),
 .UNSPECIFIED.) ;
#2384=B_SPLINE_CURVE_WITH_KNOTS('',3,(#167660,#167661,#167662,#167663,#167664,
#167665,#167666,#167667,#167668,#167669,#167670,#167671,#167672,#167673,
#167674,#167675,#167676,#167677,#167678,#167679,#167680,#167681,#167682,
#167683,#167684,#167685),.UNSPECIFIED.,.F.,.F.,(4,2,2,2,2,2,2,2,2,2,2,2,
4),(0.,5.70004774913574E-6,8.2551134764029E-6,9.93040049428637E-6,2.64556965229031E-5,
3.05873361124737E-5,4.24593515817696E-5,6.43784914888402E-5,7.66562101644865E-5,
9.74321373305911E-5,9.92796257088035E-5,0.000111632960404936,0.00013530997533304),
 .UNSPECIFIED.) ;
#2385=B_SPLINE_CURVE_WITH_KNOTS('',3,(#167692,#167693,#167694,#167695,#167696,
#167697,#167698,#167699,#167700,#167701,#167702,#167703,#167704,#167705,
#167706,#167707,#167708,#167709,#167710,#167711,#167712,#167713,#167714,
#167715,#167716,#167717,#167718,#167719,#167720,#167721,#167722,#167723,
#167724,#167725),.UNSPECIFIED.,.F.,.F.,(4,2,2,2,2,2,2,2,2,2,2,2,2,2,2,2,
4),(0.,1.27221745291788E-5,3.17734837391886E-5,3.5827099490101E-5,4.83658434534691E-5,
6.6891964566145E-5,7.0561398799944E-5,8.272321427564E-5,9.87362632794886E-5,
0.00010411157453835,0.000114567411933352,0.000115616565506964,0.000123791392830442,
0.00012426720927844,0.000126967031952657,0.000132546919744853,0.000134871234237328),
 .UNSPECIFIED.) ;
#2386=B_SPLINE_CURVE_WITH_KNOTS('',3,(#167729,#167730,#167731,#167732,#167733,
#167734,#167735,#167736,#167737,#167738,#167739,#167740,#167741,#167742,
#167743,#167744,#167745,#167746,#167747,#167748,#167749,#167750,#167751,
#167752,#167753,#167754),.UNSPECIFIED.,.F.,.F.,(4,2,2,2,2,2,2,2,2,2,2,2,
4),(0.,5.70004774912575E-6,8.2551134764029E-6,9.93040049428637E-6,2.64556965228879E-5,
3.05873361124728E-5,4.24593515817696E-5,6.43784914888337E-5,7.66562101644865E-5,
9.74321373308457E-5,9.92796257088009E-5,0.000111632960404936,0.00013530997533304),
 .UNSPECIFIED.) ;
#2387=B_SPLINE_CURVE_WITH_KNOTS('',3,(#167761,#167762,#167763,#167764,#167765,
#167766,#167767,#167768,#167769,#167770,#167771,#167772,#167773,#167774,
#167775,#167776,#167777,#167778,#167779,#167780,#167781,#167782,#167783,
#167784,#167785,#167786,#167787,#167788,#167789,#167790,#167791,#167792,
#167793,#167794),.UNSPECIFIED.,.F.,.F.,(4,2,2,2,2,2,2,2,2,2,2,2,2,2,2,2,
4),(0.,8.71783727022481E-6,1.7644110536595E-5,3.58270994901018E-5,4.83658434534691E-5,
6.68919645661972E-5,7.05613987999443E-5,8.272321427564E-5,9.87362632793253E-5,
0.00010411157453835,0.000114567411933539,0.000115616565506964,0.000123791392830457,
0.000124267209278436,0.000126967031952657,0.000132546919744863,0.000134871234237328),
 .UNSPECIFIED.) ;
#2388=B_SPLINE_CURVE_WITH_KNOTS('',3,(#167798,#167799,#167800,#167801,#167802,
#167803,#167804,#167805,#167806,#167807,#167808,#167809,#167810,#167811,
#167812,#167813,#167814,#167815,#167816,#167817,#167818,#167819,#167820,
#167821,#167822,#167823),.UNSPECIFIED.,.F.,.F.,(4,2,2,2,2,2,2,2,2,2,2,2,
4),(0.,5.70004774913546E-6,8.2551134764029E-6,9.93040049428637E-6,2.64556965229398E-5,
3.05873361124753E-5,4.24593515817696E-5,6.43784914888368E-5,7.66562101644865E-5,
9.74321373310438E-5,9.92796257088069E-5,0.000111632960404936,0.00013530997533304),
 .UNSPECIFIED.) ;
#2389=B_SPLINE_CURVE_WITH_KNOTS('',3,(#167830,#167831,#167832,#167833,#167834,
#167835,#167836,#167837,#167838,#167839,#167840,#167841,#167842,#167843,
#167844,#167845,#167846,#167847,#167848,#167849,#167850,#167851,#167852,
#167853,#167854,#167855,#167856,#167857,#167858,#167859,#167860,#167861,
#167862,#167863),.UNSPECIFIED.,.F.,.F.,(4,2,2,2,2,2,2,2,2,2,2,2,2,2,2,2,
4),(0.,8.7178372714199E-6,1.76441105365042E-5,3.58270994900995E-5,4.83658434534691E-5,
6.68919645658283E-5,7.0561398799945E-5,8.272321427564E-5,9.87362632792552E-5,
0.000104111574538349,0.000114567411933256,0.000115616565506964,0.000123791392830476,
0.000124267209278436,0.000126967031952657,0.000132546919744827,0.000134871234237328),
 .UNSPECIFIED.) ;
#2390=B_SPLINE_CURVE_WITH_KNOTS('',3,(#167867,#167868,#167869,#167870,#167871,
#167872,#167873,#167874,#167875,#167876,#167877,#167878,#167879,#167880,
#167881,#167882,#167883,#167884,#167885,#167886,#167887,#167888,#167889,
#167890,#167891,#167892),.UNSPECIFIED.,.F.,.F.,(4,2,2,2,2,2,2,2,2,2,2,2,
4),(0.,5.7000477491356E-6,8.2551134764029E-6,9.93040049428637E-6,2.64556965228419E-5,
3.05873361124732E-5,4.24593515817696E-5,6.43784914888367E-5,7.66562101644865E-5,
9.74321373305317E-5,9.92796257088022E-5,0.000111632960404936,0.00013530997533304),
 .UNSPECIFIED.) ;
#2391=B_SPLINE_CURVE_WITH_KNOTS('',3,(#167899,#167900,#167901,#167902,#167903,
#167904,#167905,#167906,#167907,#167908,#167909,#167910,#167911,#167912,
#167913,#167914,#167915,#167916,#167917,#167918,#167919,#167920,#167921,
#167922,#167923,#167924,#167925,#167926,#167927,#167928,#167929,#167930,
#167931,#167932),.UNSPECIFIED.,.F.,.F.,(4,2,2,2,2,2,2,2,2,2,2,2,2,2,2,2,
4),(0.,1.27221745291788E-5,3.17734837391183E-5,3.58270994901062E-5,4.83658434534691E-5,
6.68919645661017E-5,7.05613987999452E-5,8.272321427564E-5,9.87362632793197E-5,
0.000104111574538349,0.00011456741193351,0.000115616565506964,0.000123791392830282,
0.000124267209278427,0.000126967031952657,0.000132546919744846,0.000134871234237328),
 .UNSPECIFIED.) ;
#2392=B_SPLINE_CURVE_WITH_KNOTS('',3,(#167936,#167937,#167938,#167939,#167940,
#167941,#167942,#167943,#167944,#167945,#167946,#167947,#167948,#167949,
#167950,#167951,#167952,#167953,#167954,#167955,#167956,#167957,#167958,
#167959,#167960,#167961),.UNSPECIFIED.,.F.,.F.,(4,2,2,2,2,2,2,2,2,2,2,2,
4),(5.65450672847475E-18,5.70004774919696E-6,8.25511347639078E-6,9.93040049428371E-6,
2.64556965223417E-5,3.05873361124641E-5,4.24593515817652E-5,6.43784914888292E-5,
7.66562101644793E-5,9.74321373329595E-5,9.92796257088198E-5,0.000111632960404932,
0.000135309975333043),.UNSPECIFIED.) ;
#2393=B_SPLINE_CURVE_WITH_KNOTS('',3,(#167968,#167969,#167970,#167971,#167972,
#167973,#167974,#167975,#167976,#167977,#167978,#167979,#167980,#167981,
#167982,#167983,#167984,#167985,#167986,#167987,#167988,#167989,#167990,
#167991,#167992,#167993,#167994,#167995,#167996,#167997,#167998,#167999,
#168000,#168001),.UNSPECIFIED.,.F.,.F.,(4,2,2,2,2,2,2,2,2,2,2,2,2,2,2,2,
4),(0.,1.27221745291825E-5,3.17734837389246E-5,3.58270994900963E-5,4.8365843453465E-5,
6.68919645660607E-5,7.05613987999433E-5,8.27232142756395E-5,9.87362632792754E-5,
0.000104111574538343,0.000114567411932696,0.000115616565506954,0.000123791392829404,
0.000124267209278547,0.000126967031952634,0.000132546919744699,0.000134871234237319),
 .UNSPECIFIED.) ;
#2394=B_SPLINE_CURVE_WITH_KNOTS('',3,(#168008,#168009,#168010,#168011,#168012,
#168013,#168014,#168015,#168016,#168017,#168018,#168019,#168020,#168021,
#168022,#168023,#168024,#168025,#168026,#168027,#168028,#168029,#168030,
#168031,#168032,#168033,#168034,#168035,#168036,#168037,#168038,#168039,
#168040,#168041),.UNSPECIFIED.,.F.,.F.,(4,2,2,2,2,2,2,2,2,2,2,2,2,2,2,2,
4),(0.,1.27221745291825E-5,3.17734837389621E-5,3.58270994901002E-5,4.8365843453465E-5,
6.68919645658703E-5,7.05613987999433E-5,8.27232142756395E-5,9.87362632795784E-5,
0.000104111574538341,0.000114567411933155,0.000115616565506954,0.000123791392830688,
0.00012426720927855,0.000126967031952634,0.000132546919744675,0.000134871234237319),
 .UNSPECIFIED.) ;
#2395=B_SPLINE_CURVE_WITH_KNOTS('',3,(#168044,#168045,#168046,#168047,#168048,
#168049,#168050,#168051,#168052,#168053,#168054,#168055,#168056,#168057,
#168058,#168059,#168060,#168061,#168062,#168063,#168064,#168065,#168066,
#168067,#168068,#168069,#168070,#168071,#168072,#168073,#168074,#168075,
#168076,#168077,#168078,#168079,#168080,#168081,#168082,#168083,#168084,
#168085,#168086,#168087,#168088,#168089,#168090,#168091,#168092,#168093,
#168094,#168095,#168096,#168097,#168098),.UNSPECIFIED.,.F.,.F.,(4,3,3,3,
3,3,3,3,3,3,3,3,3,3,3,3,3,3,4),(0.,1.96170179200497E-5,2.35258500143173E-5,
3.58003153605656E-5,5.29187212186161E-5,5.64435994880342E-5,5.827929265241E-5,
7.04649253805291E-5,8.72923312913114E-5,9.05038369578067E-5,9.22578228185119E-5,
0.000103663146463146,0.00011386600552152,0.000117768598772948,0.000124579094175181,
0.000129312863866763,0.000130178750830829,0.000132692979584749,0.000134419842078313),
 .UNSPECIFIED.) ;
#2396=B_SPLINE_CURVE_WITH_KNOTS('',3,(#168107,#168108,#168109,#168110,#168111,
#168112,#168113,#168114,#168115,#168116,#168117,#168118,#168119,#168120,
#168121,#168122,#168123,#168124,#168125,#168126,#168127,#168128,#168129,
#168130,#168131,#168132),.UNSPECIFIED.,.F.,.F.,(4,2,2,2,2,2,2,2,2,2,2,2,
4),(0.,5.55321021973765E-6,8.25511347643081E-6,1.91711188535185E-5,3.04852632940538E-5,
5.08165579102967E-5,5.19149958125378E-5,6.39742577536705E-5,8.61162395509785E-5,
9.85980048375137E-5,0.000117622240611127,0.000125683481931241,0.00013426229848852),
 .UNSPECIFIED.) ;
#2397=B_SPLINE_CURVE_WITH_KNOTS('',3,(#168139,#168140,#168141,#168142,#168143,
#168144,#168145,#168146,#168147,#168148,#168149,#168150,#168151,#168152,
#168153,#168154,#168155,#168156,#168157,#168158,#168159,#168160,#168161,
#168162,#168163,#168164,#168165,#168166,#168167,#168168,#168169,#168170,
#168171,#168172,#168173,#168174,#168175,#168176,#168177,#168178,#168179,
#168180,#168181,#168182,#168183,#168184,#168185,#168186,#168187,#168188,
#168189,#168190,#168191,#168192,#168193),.UNSPECIFIED.,.F.,.F.,(4,3,3,3,
3,3,3,3,3,3,3,3,3,3,3,3,3,3,4),(0.,1.96170179200542E-5,2.35258500143173E-5,
3.58003153605654E-5,5.29187212186038E-5,5.64435994880909E-5,5.8279292652409E-5,
7.04649253805292E-5,8.72923312915481E-5,9.05038369577458E-5,9.22578228185104E-5,
0.000103663146463144,0.000113866005521528,0.000117768598772953,0.00012457909417518,
0.000129312863866768,0.00013017875083082,0.000132692979584748,0.000134419842078312),
 .UNSPECIFIED.) ;
#2398=B_SPLINE_CURVE_WITH_KNOTS('',3,(#168202,#168203,#168204,#168205,#168206,
#168207,#168208,#168209,#168210,#168211,#168212,#168213,#168214,#168215,
#168216,#168217,#168218,#168219,#168220,#168221,#168222,#168223,#168224,
#168225,#168226,#168227),.UNSPECIFIED.,.F.,.F.,(4,2,2,2,2,2,2,2,2,2,2,2,
4),(0.,5.55321021971803E-6,8.2551134764307E-6,1.91711188535182E-5,3.04852632940564E-5,
5.08165579104009E-5,5.1914995812538E-5,6.39742577536707E-5,8.61162395509773E-5,
9.85980048375135E-5,0.000117622240611135,0.000125683481931497,0.00013426229848852),
 .UNSPECIFIED.) ;
#2399=B_SPLINE_CURVE_WITH_KNOTS('',3,(#168234,#168235,#168236,#168237,#168238,
#168239,#168240,#168241,#168242,#168243,#168244,#168245,#168246,#168247,
#168248,#168249,#168250,#168251,#168252,#168253,#168254,#168255,#168256,
#168257,#168258,#168259,#168260,#168261,#168262,#168263,#168264,#168265,
#168266,#168267,#168268,#168269,#168270,#168271,#168272,#168273,#168274,
#168275,#168276,#168277,#168278,#168279,#168280,#168281,#168282,#168283,
#168284,#168285,#168286,#168287,#168288),.UNSPECIFIED.,.F.,.F.,(4,3,3,3,
3,3,3,3,3,3,3,3,3,3,3,3,3,3,4),(0.,1.96170179192311E-5,2.35258500143173E-5,
3.58003153605661E-5,5.29187212162782E-5,5.6443599488185E-5,5.82792926524099E-5,
7.046492538053E-5,8.72923312900606E-5,9.05038369578505E-5,9.22578228185119E-5,
0.000103663146463143,0.000113866005521194,0.000117768598772959,0.000124579094175181,
0.000129312863866605,0.000130178750830851,0.000132692979584745,0.000134419842078313),
 .UNSPECIFIED.) ;
#2400=B_SPLINE_CURVE_WITH_KNOTS('',3,(#168297,#168298,#168299,#168300,#168301,
#168302,#168303,#168304,#168305,#168306,#168307,#168308,#168309,#168310,
#168311,#168312,#168313,#168314,#168315,#168316,#168317,#168318,#168319,
#168320,#168321,#168322),.UNSPECIFIED.,.F.,.F.,(4,2,2,2,2,2,2,2,2,2,2,2,
4),(0.,5.55321021971055E-6,8.25511347643257E-6,1.91711188535176E-5,3.04852632940549E-5,
5.08165579107018E-5,5.19149958125369E-5,6.39742577536715E-5,8.61162395509772E-5,
9.85980048375149E-5,0.000117622240611143,0.00012568348193157,0.00013426229848852),
 .UNSPECIFIED.) ;
#2401=B_SPLINE_CURVE_WITH_KNOTS('',3,(#168329,#168330,#168331,#168332,#168333,
#168334,#168335,#168336,#168337,#168338,#168339,#168340,#168341,#168342,
#168343,#168344,#168345,#168346,#168347,#168348,#168349,#168350,#168351,
#168352,#168353,#168354,#168355,#168356,#168357,#168358,#168359,#168360,
#168361,#168362,#168363,#168364,#168365,#168366,#168367,#168368,#168369,
#168370,#168371,#168372,#168373,#168374,#168375,#168376,#168377,#168378,
#168379,#168380,#168381,#168382,#168383),.UNSPECIFIED.,.F.,.F.,(4,3,3,3,
3,3,3,3,3,3,3,3,3,3,3,3,3,3,4),(0.,1.96170179203663E-5,2.35258500143174E-5,
3.58003153605658E-5,5.2918721219628E-5,5.64435994880167E-5,5.82792926524091E-5,
7.04649253805322E-5,8.72923312915083E-5,9.05038369581538E-5,9.2257822818511E-5,
0.000103663146463142,0.00011386600552163,0.000117768598772992,0.000124579094175182,
0.000129312863867062,0.0001301787508309,0.000132692979584746,0.000134419842078314),
 .UNSPECIFIED.) ;
#2402=B_SPLINE_CURVE_WITH_KNOTS('',3,(#168392,#168393,#168394,#168395,#168396,
#168397,#168398,#168399,#168400,#168401,#168402,#168403,#168404,#168405,
#168406,#168407,#168408,#168409,#168410,#168411,#168412,#168413,#168414,
#168415,#168416,#168417),.UNSPECIFIED.,.F.,.F.,(4,2,2,2,2,2,2,2,2,2,2,2,
4),(0.,5.55321021972969E-6,8.25511347643257E-6,1.91711188535176E-5,3.04852632940556E-5,
5.08165579107454E-5,5.19149958125369E-5,6.39742577536697E-5,8.61162395509772E-5,
9.85980048375132E-5,0.000117622240611155,0.00012568348193195,0.00013426229848852),
 .UNSPECIFIED.) ;
#2403=B_SPLINE_CURVE_WITH_KNOTS('',3,(#168424,#168425,#168426,#168427,#168428,
#168429,#168430,#168431,#168432,#168433,#168434,#168435,#168436,#168437,
#168438,#168439,#168440,#168441,#168442,#168443,#168444,#168445,#168446,
#168447,#168448,#168449,#168450,#168451,#168452,#168453,#168454,#168455,
#168456,#168457,#168458,#168459,#168460,#168461,#168462,#168463,#168464,
#168465,#168466,#168467,#168468,#168469,#168470,#168471,#168472,#168473,
#168474,#168475,#168476,#168477,#168478),.UNSPECIFIED.,.F.,.F.,(4,3,3,3,
3,3,3,3,3,3,3,3,3,3,3,3,3,3,4),(0.,1.96170179208962E-5,2.35258500143174E-5,
3.58003153605662E-5,5.29187212198585E-5,5.64435994880185E-5,5.82792926524091E-5,
7.04649253805333E-5,8.72923312910633E-5,9.05038369581232E-5,9.2257822818511E-5,
0.000103663146463146,0.000113866005521589,0.000117768598772995,0.000124579094175182,
0.000129312863867127,0.000130178750830904,0.000132692979584746,0.000134419842078314),
 .UNSPECIFIED.) ;
#2404=B_SPLINE_CURVE_WITH_KNOTS('',3,(#168487,#168488,#168489,#168490,#168491,
#168492,#168493,#168494,#168495,#168496,#168497,#168498,#168499,#168500,
#168501,#168502,#168503,#168504,#168505,#168506,#168507,#168508,#168509,
#168510,#168511,#168512),.UNSPECIFIED.,.F.,.F.,(4,2,2,2,2,2,2,2,2,2,2,2,
4),(0.,5.55321021973998E-6,8.25511347643153E-6,1.91711188535163E-5,3.0485263294052E-5,
5.0816557910318E-5,5.19149958125372E-5,6.39742577536688E-5,8.61162395509784E-5,
9.85980048375113E-5,0.000117622240611307,0.000125683481932561,0.000134262298488521),
 .UNSPECIFIED.) ;
#2405=B_SPLINE_CURVE_WITH_KNOTS('',3,(#168519,#168520,#168521,#168522,#168523,
#168524,#168525,#168526,#168527,#168528,#168529,#168530,#168531,#168532,
#168533,#168534,#168535,#168536,#168537,#168538,#168539,#168540,#168541,
#168542,#168543,#168544,#168545,#168546,#168547,#168548,#168549,#168550,
#168551,#168552,#168553,#168554,#168555,#168556,#168557,#168558,#168559,
#168560,#168561,#168562,#168563,#168564,#168565,#168566,#168567,#168568,
#168569,#168570,#168571,#168572,#168573),.UNSPECIFIED.,.F.,.F.,(4,3,3,3,
3,3,3,3,3,3,3,3,3,3,3,3,3,3,4),(0.,1.96170179192042E-5,2.35258500143174E-5,
3.58003153605655E-5,5.2918721218618E-5,5.64435994880514E-5,5.82792926524091E-5,
7.04649253805306E-5,8.72923312917556E-5,9.05038369587251E-5,9.2257822818511E-5,
0.000103663146463134,0.000113866005521224,0.000117768598772955,0.000124579094175182,
0.0001293128638668,0.000130178750830747,0.000132692979584746,0.000134419842078314),
 .UNSPECIFIED.) ;
#2406=B_SPLINE_CURVE_WITH_KNOTS('',3,(#168582,#168583,#168584,#168585,#168586,
#168587,#168588,#168589,#168590,#168591,#168592,#168593,#168594,#168595,
#168596,#168597,#168598,#168599,#168600,#168601,#168602,#168603,#168604,
#168605,#168606,#168607),.UNSPECIFIED.,.F.,.F.,(4,2,2,2,2,2,2,2,2,2,2,2,
4),(0.,5.55321021976979E-6,8.25511347643153E-6,1.91711188535163E-5,3.0485263294054E-5,
5.08165579104287E-5,5.19149958125372E-5,6.39742577536726E-5,8.61162395509784E-5,
9.85980048375128E-5,0.000117622240611284,0.000125683481932007,0.000134262298488521),
 .UNSPECIFIED.) ;
#2407=B_SPLINE_CURVE_WITH_KNOTS('',3,(#168614,#168615,#168616,#168617,#168618,
#168619,#168620,#168621,#168622,#168623,#168624,#168625,#168626,#168627,
#168628,#168629,#168630,#168631,#168632,#168633,#168634,#168635,#168636,
#168637,#168638,#168639,#168640,#168641,#168642,#168643,#168644,#168645,
#168646,#168647,#168648,#168649,#168650,#168651,#168652,#168653,#168654,
#168655,#168656,#168657,#168658,#168659,#168660,#168661,#168662,#168663,
#168664,#168665,#168666,#168667,#168668),.UNSPECIFIED.,.F.,.F.,(4,3,3,3,
3,3,3,3,3,3,3,3,3,3,3,3,3,3,4),(0.,1.96170179208898E-5,2.35258500143174E-5,
3.58003153605655E-5,5.29187212199216E-5,5.64435994880236E-5,5.82792926524091E-5,
7.04649253805303E-5,8.7292331290714E-5,9.05038369585905E-5,9.2257822818511E-5,
0.000103663146463137,0.00011386600552116,0.000117768598772957,0.000124579094175182,
0.000129312863866651,0.000130178750830784,0.000132692979584746,0.000134419842078314),
 .UNSPECIFIED.) ;
#2408=B_SPLINE_CURVE_WITH_KNOTS('',3,(#168677,#168678,#168679,#168680,#168681,
#168682,#168683,#168684,#168685,#168686,#168687,#168688,#168689,#168690,
#168691,#168692,#168693,#168694,#168695,#168696,#168697,#168698,#168699,
#168700,#168701,#168702),.UNSPECIFIED.,.F.,.F.,(4,2,2,2,2,2,2,2,2,2,2,2,
4),(0.,5.55321021976964E-6,8.25511347643153E-6,1.91711188535163E-5,3.04852632940513E-5,
5.08165579102757E-5,5.19149958125372E-5,6.39742577536695E-5,8.61162395509784E-5,
9.85980048375118E-5,0.000117622240611266,0.000125683481932165,0.000134262298488521),
 .UNSPECIFIED.) ;
#2409=B_SPLINE_CURVE_WITH_KNOTS('',3,(#168709,#168710,#168711,#168712,#168713,
#168714,#168715,#168716,#168717,#168718,#168719,#168720,#168721,#168722,
#168723,#168724,#168725,#168726,#168727,#168728,#168729,#168730,#168731,
#168732,#168733,#168734,#168735,#168736,#168737,#168738,#168739,#168740,
#168741,#168742,#168743,#168744,#168745,#168746,#168747,#168748,#168749,
#168750,#168751,#168752,#168753,#168754,#168755,#168756,#168757,#168758,
#168759,#168760,#168761,#168762,#168763),.UNSPECIFIED.,.F.,.F.,(4,3,3,3,
3,3,3,3,3,3,3,3,3,3,3,3,3,3,4),(0.,1.96170179198987E-5,2.35258500143176E-5,
3.58003153605645E-5,5.29187212179511E-5,5.64435994874837E-5,5.82792926524096E-5,
7.04649253805232E-5,8.72923312922054E-5,9.05038369575662E-5,9.22578228185116E-5,
0.000103663146463143,0.000113866005521635,0.000117768598772949,0.000124579094175177,
0.000129312863866761,0.000130178750830864,0.000132692979584753,0.000134419842078312),
 .UNSPECIFIED.) ;
#2410=B_SPLINE_CURVE_WITH_KNOTS('',3,(#168772,#168773,#168774,#168775,#168776,
#168777,#168778,#168779,#168780,#168781,#168782,#168783,#168784,#168785,
#168786,#168787,#168788,#168789,#168790,#168791,#168792,#168793,#168794,
#168795,#168796,#168797),.UNSPECIFIED.,.F.,.F.,(4,2,2,2,2,2,2,2,2,2,2,2,
4),(0.,5.55321021972859E-6,8.25511347643153E-6,1.91711188535163E-5,3.0485263294052E-5,
5.08165579103031E-5,5.19149958125372E-5,6.39742577536713E-5,8.61162395509784E-5,
9.85980048375125E-5,0.000117622240611228,0.000125683481931749,0.000134262298488521),
 .UNSPECIFIED.) ;
#2411=B_SPLINE_CURVE_WITH_KNOTS('',3,(#168804,#168805,#168806,#168807,#168808,
#168809,#168810,#168811,#168812,#168813,#168814,#168815,#168816,#168817,
#168818,#168819,#168820,#168821,#168822,#168823,#168824,#168825,#168826,
#168827,#168828,#168829,#168830,#168831,#168832,#168833,#168834,#168835,
#168836,#168837,#168838,#168839,#168840,#168841,#168842,#168843,#168844,
#168845,#168846,#168847,#168848,#168849,#168850,#168851,#168852,#168853,
#168854,#168855,#168856,#168857,#168858),.UNSPECIFIED.,.F.,.F.,(4,3,3,3,
3,3,3,3,3,3,3,3,3,3,3,3,3,3,4),(0.,1.96170179200225E-5,2.35258500143176E-5,
3.58003153605643E-5,5.29187212193709E-5,5.64435994873347E-5,5.82792926524096E-5,
7.04649253805203E-5,8.72923312916406E-5,9.05038369574672E-5,9.22578228185116E-5,
0.000103663146463146,0.000113866005521278,0.000117768598772934,0.000124579094175177,
0.00012931286386678,0.00013017875083066,0.000132692979584753,0.000134419842078312),
 .UNSPECIFIED.) ;
#2412=B_SPLINE_CURVE_WITH_KNOTS('',3,(#168867,#168868,#168869,#168870,#168871,
#168872,#168873,#168874,#168875,#168876,#168877,#168878,#168879,#168880,
#168881,#168882,#168883,#168884,#168885,#168886,#168887,#168888,#168889,
#168890,#168891,#168892),.UNSPECIFIED.,.F.,.F.,(4,2,2,2,2,2,2,2,2,2,2,2,
4),(0.,5.55321021961745E-6,8.25511347643483E-6,1.91711188535197E-5,3.04852632940677E-5,
5.08165579107201E-5,5.19149958125403E-5,6.39742577536799E-5,8.61162395509805E-5,
9.85980048375172E-5,0.000117622240610844,0.000125683481932884,0.000134262298488518),
 .UNSPECIFIED.) ;
#2413=B_SPLINE_CURVE_WITH_KNOTS('',3,(#169558,#169559,#169560,#169561,#169562,
#169563,#169564,#169565,#169566,#169567,#169568,#169569,#169570,#169571,
#169572,#169573,#169574,#169575,#169576,#169577,#169578,#169579,#169580,
#169581,#169582,#169583,#169584,#169585,#169586,#169587,#169588,#169589,
#169590,#169591,#169592,#169593,#169594,#169595,#169596,#169597,#169598,
#169599,#169600,#169601,#169602,#169603,#169604,#169605,#169606,#169607),
 .UNSPECIFIED.,.F.,.F.,(4,2,2,2,2,2,2,2,2,2,2,2,2,2,2,2,2,2,2,2,2,2,2,2,
4),(-2.08039868634433E-6,0.,1.80285080514979E-6,4.0751335740202E-6,7.68982405736938E-6,
1.34802948057236E-5,2.29326054193163E-5,3.92630132602966E-5,5.80367880477344E-5,
6.50818237188975E-5,7.31401178077086E-5,7.59246603911382E-5,9.50727127604295E-5,
9.80359284023885E-5,0.000112225222383658,0.000116796661227539,0.000117770724301747,
0.000134602167593749,0.000142446541904567,0.000143188584796264,0.000155450849073387,
0.000157760323312202,0.000160014008022128,0.000173898693194695,0.000175397121695959),
 .UNSPECIFIED.) ;
#2414=B_SPLINE_CURVE_WITH_KNOTS('',3,(#169958,#169959,#169960,#169961,#169962,
#169963,#169964,#169965,#169966,#169967,#169968,#169969,#169970,#169971,
#169972,#169973,#169974,#169975,#169976,#169977,#169978,#169979,#169980,
#169981,#169982,#169983,#169984,#169985,#169986,#169987,#169988,#169989,
#169990,#169991,#169992,#169993,#169994,#169995,#169996,#169997,#169998,
#169999,#170000,#170001,#170002,#170003,#170004,#170005,#170006,#170007),
 .UNSPECIFIED.,.F.,.F.,(4,2,2,2,2,2,2,2,2,2,2,2,2,2,2,2,2,2,2,2,2,2,2,2,
4),(-2.08039868634673E-6,0.,1.80285080513718E-6,4.07513357401502E-6,7.68982405736462E-6,
1.34802948057175E-5,2.29326054193016E-5,3.92630132602916E-5,5.80367882596256E-5,
6.50818237191735E-5,7.31401178093195E-5,7.59246603911372E-5,9.50727128359684E-5,
9.80359284024087E-5,0.000112225222382539,0.000116796661227535,0.00011777072430175,
0.000134602167593809,0.000142446541904572,0.000143188584796265,0.000155450849073815,
0.000157760323312273,0.000160014008022131,0.000173898693194877,0.000175397121695963),
 .UNSPECIFIED.) ;
#2420=CONICAL_SURFACE('',#98416,1.,0.78539816339745) ;
#2421=CONICAL_SURFACE('',#98418,1.,0.78539816339745) ;
#2422=CONICAL_SURFACE('',#98420,1.,0.78539816339745) ;
#2423=CONICAL_SURFACE('',#98422,1.,0.78539816339745) ;
#2424=CONICAL_SURFACE('',#98424,1.,0.78539816339745) ;
#2425=CONICAL_SURFACE('',#98426,1.,0.78539816339745) ;
#2426=CONICAL_SURFACE('',#98428,1.,0.78539816339745) ;
#2427=CONICAL_SURFACE('',#98430,0.999999999999999,0.78539816339745) ;
#2428=CONICAL_SURFACE('',#98432,1.,0.78539816339745) ;
#2429=CONICAL_SURFACE('',#98469,1.,0.78539816339745) ;
#5767=LINE('',#152015,#11321) ;
#5768=LINE('',#152018,#11322) ;
#5769=LINE('',#153721,#11323) ;
#5770=LINE('',#153722,#11324) ;
#5771=LINE('',#153725,#11325) ;
#5772=LINE('',#153726,#11326) ;
#5773=LINE('',#153729,#11327) ;
#5774=LINE('',#153730,#11328) ;
#5775=LINE('',#153733,#11329) ;
#5776=LINE('',#153734,#11330) ;
#5777=LINE('',#153737,#11331) ;
#5778=LINE('',#153738,#11332) ;
#5779=LINE('',#153741,#11333) ;
#5780=LINE('',#153742,#11334) ;
#5781=LINE('',#153745,#11335) ;
#5782=LINE('',#153746,#11336) ;
#5783=LINE('',#153925,#11337) ;
#5784=LINE('',#153951,#11338) ;
#5785=LINE('',#153998,#11339) ;
#5786=LINE('',#154024,#11340) ;
#5787=LINE('',#154058,#11341) ;
#5788=LINE('',#154075,#11342) ;
#5789=LINE('',#154101,#11343) ;
#5790=LINE('',#154148,#11344) ;
#5791=LINE('',#154174,#11345) ;
#5792=LINE('',#154208,#11346) ;
#5793=LINE('',#154225,#11347) ;
#5794=LINE('',#154251,#11348) ;
#5795=LINE('',#154298,#11349) ;
#5796=LINE('',#154324,#11350) ;
#5797=LINE('',#154358,#11351) ;
#5798=LINE('',#154375,#11352) ;
#5799=LINE('',#154401,#11353) ;
#5800=LINE('',#154448,#11354) ;
#5801=LINE('',#154474,#11355) ;
#5802=LINE('',#154508,#11356) ;
#5803=LINE('',#154525,#11357) ;
#5804=LINE('',#154551,#11358) ;
#5805=LINE('',#154598,#11359) ;
#5806=LINE('',#154624,#11360) ;
#5807=LINE('',#154658,#11361) ;
#5808=LINE('',#154675,#11362) ;
#5809=LINE('',#154701,#11363) ;
#5810=LINE('',#154748,#11364) ;
#5811=LINE('',#154774,#11365) ;
#5812=LINE('',#154808,#11366) ;
#5813=LINE('',#154825,#11367) ;
#5814=LINE('',#154851,#11368) ;
#5815=LINE('',#154898,#11369) ;
#5816=LINE('',#154924,#11370) ;
#5817=LINE('',#154958,#11371) ;
#5818=LINE('',#154975,#11372) ;
#5819=LINE('',#155001,#11373) ;
#5820=LINE('',#155048,#11374) ;
#5821=LINE('',#155074,#11375) ;
#5822=LINE('',#155108,#11376) ;
#5823=LINE('',#155125,#11377) ;
#5824=LINE('',#155151,#11378) ;
#5825=LINE('',#155198,#11379) ;
#5826=LINE('',#155224,#11380) ;
#5827=LINE('',#155258,#11381) ;
#5828=LINE('',#155262,#11382) ;
#5829=LINE('',#155266,#11383) ;
#5830=LINE('',#155270,#11384) ;
#5831=LINE('',#155274,#11385) ;
#5832=LINE('',#155278,#11386) ;
#5833=LINE('',#155282,#11387) ;
#5834=LINE('',#155286,#11388) ;
#5835=LINE('',#155290,#11389) ;
#5836=LINE('',#155294,#11390) ;
#5837=LINE('',#155296,#11391) ;
#5838=LINE('',#155298,#11392) ;
#5839=LINE('',#155300,#11393) ;
#5840=LINE('',#155302,#11394) ;
#5841=LINE('',#155304,#11395) ;
#5842=LINE('',#155306,#11396) ;
#5843=LINE('',#155308,#11397) ;
#5844=LINE('',#155310,#11398) ;
#5845=LINE('',#155312,#11399) ;
#5846=LINE('',#155333,#11400) ;
#5847=LINE('',#155334,#11401) ;
#5848=LINE('',#155338,#11402) ;
#5849=LINE('',#155339,#11403) ;
#5850=LINE('',#155343,#11404) ;
#5851=LINE('',#155344,#11405) ;
#5852=LINE('',#155347,#11406) ;
#5853=LINE('',#155348,#11407) ;
#5854=LINE('',#155365,#11408) ;
#5855=LINE('',#155391,#11409) ;
#5856=LINE('',#155438,#11410) ;
#5857=LINE('',#155464,#11411) ;
#5858=LINE('',#155498,#11412) ;
#5859=LINE('',#155502,#11413) ;
#5860=LINE('',#155504,#11414) ;
#5861=LINE('',#155508,#11415) ;
#5862=LINE('',#155510,#11416) ;
#5863=LINE('',#155512,#11417) ;
#5864=LINE('',#155513,#11418) ;
#5865=LINE('',#155525,#11419) ;
#5866=LINE('',#155527,#11420) ;
#5867=LINE('',#155528,#11421) ;
#5868=LINE('',#155533,#11422) ;
#5869=LINE('',#155537,#11423) ;
#5870=LINE('',#155541,#11424) ;
#5871=LINE('',#155544,#11425) ;
#5872=LINE('',#155549,#11426) ;
#5873=LINE('',#155553,#11427) ;
#5874=LINE('',#155557,#11428) ;
#5875=LINE('',#155560,#11429) ;
#5876=LINE('',#155565,#11430) ;
#5877=LINE('',#155569,#11431) ;
#5878=LINE('',#155573,#11432) ;
#5879=LINE('',#155576,#11433) ;
#5880=LINE('',#155581,#11434) ;
#5881=LINE('',#155585,#11435) ;
#5882=LINE('',#155589,#11436) ;
#5883=LINE('',#155592,#11437) ;
#5884=LINE('',#155597,#11438) ;
#5885=LINE('',#155601,#11439) ;
#5886=LINE('',#155605,#11440) ;
#5887=LINE('',#155608,#11441) ;
#5888=LINE('',#155613,#11442) ;
#5889=LINE('',#155617,#11443) ;
#5890=LINE('',#155621,#11444) ;
#5891=LINE('',#155624,#11445) ;
#5892=LINE('',#155629,#11446) ;
#5893=LINE('',#155633,#11447) ;
#5894=LINE('',#155637,#11448) ;
#5895=LINE('',#155640,#11449) ;
#5896=LINE('',#155645,#11450) ;
#5897=LINE('',#155649,#11451) ;
#5898=LINE('',#155653,#11452) ;
#5899=LINE('',#155656,#11453) ;
#5900=LINE('',#155661,#11454) ;
#5901=LINE('',#155665,#11455) ;
#5902=LINE('',#155669,#11456) ;
#5903=LINE('',#155672,#11457) ;
#5904=LINE('',#155677,#11458) ;
#5905=LINE('',#155681,#11459) ;
#5906=LINE('',#155685,#11460) ;
#5907=LINE('',#155688,#11461) ;
#5908=LINE('',#155692,#11462) ;
#5909=LINE('',#155694,#11463) ;
#5910=LINE('',#155696,#11464) ;
#5911=LINE('',#155697,#11465) ;
#5912=LINE('',#155700,#11466) ;
#5913=LINE('',#155704,#11467) ;
#5914=LINE('',#155708,#11468) ;
#5915=LINE('',#155712,#11469) ;
#5916=LINE('',#155717,#11470) ;
#5917=LINE('',#155719,#11471) ;
#5918=LINE('',#155721,#11472) ;
#5919=LINE('',#155722,#11473) ;
#5920=LINE('',#155725,#11474) ;
#5921=LINE('',#155729,#11475) ;
#5922=LINE('',#155733,#11476) ;
#5923=LINE('',#155737,#11477) ;
#5924=LINE('',#155742,#11478) ;
#5925=LINE('',#155744,#11479) ;
#5926=LINE('',#155746,#11480) ;
#5927=LINE('',#155747,#11481) ;
#5928=LINE('',#155750,#11482) ;
#5929=LINE('',#155754,#11483) ;
#5930=LINE('',#155758,#11484) ;
#5931=LINE('',#155762,#11485) ;
#5932=LINE('',#155767,#11486) ;
#5933=LINE('',#155769,#11487) ;
#5934=LINE('',#155771,#11488) ;
#5935=LINE('',#155772,#11489) ;
#5936=LINE('',#155775,#11490) ;
#5937=LINE('',#155779,#11491) ;
#5938=LINE('',#155783,#11492) ;
#5939=LINE('',#155787,#11493) ;
#5940=LINE('',#155792,#11494) ;
#5941=LINE('',#155794,#11495) ;
#5942=LINE('',#155796,#11496) ;
#5943=LINE('',#155797,#11497) ;
#5944=LINE('',#155800,#11498) ;
#5945=LINE('',#155804,#11499) ;
#5946=LINE('',#155808,#11500) ;
#5947=LINE('',#155812,#11501) ;
#5948=LINE('',#155817,#11502) ;
#5949=LINE('',#155819,#11503) ;
#5950=LINE('',#155821,#11504) ;
#5951=LINE('',#155822,#11505) ;
#5952=LINE('',#155825,#11506) ;
#5953=LINE('',#155829,#11507) ;
#5954=LINE('',#155833,#11508) ;
#5955=LINE('',#155837,#11509) ;
#5956=LINE('',#155842,#11510) ;
#5957=LINE('',#155844,#11511) ;
#5958=LINE('',#155846,#11512) ;
#5959=LINE('',#155847,#11513) ;
#5960=LINE('',#155850,#11514) ;
#5961=LINE('',#155854,#11515) ;
#5962=LINE('',#155858,#11516) ;
#5963=LINE('',#155862,#11517) ;
#5964=LINE('',#155867,#11518) ;
#5965=LINE('',#155869,#11519) ;
#5966=LINE('',#155871,#11520) ;
#5967=LINE('',#155872,#11521) ;
#5968=LINE('',#155875,#11522) ;
#5969=LINE('',#155879,#11523) ;
#5970=LINE('',#155883,#11524) ;
#5971=LINE('',#155887,#11525) ;
#5972=LINE('',#155892,#11526) ;
#5973=LINE('',#155894,#11527) ;
#5974=LINE('',#155896,#11528) ;
#5975=LINE('',#155897,#11529) ;
#5976=LINE('',#155900,#11530) ;
#5977=LINE('',#155904,#11531) ;
#5978=LINE('',#155908,#11532) ;
#5979=LINE('',#155912,#11533) ;
#5980=LINE('',#155915,#11534) ;
#5981=LINE('',#155917,#11535) ;
#5982=LINE('',#155919,#11536) ;
#5983=LINE('',#155921,#11537) ;
#5984=LINE('',#155923,#11538) ;
#5985=LINE('',#155925,#11539) ;
#5986=LINE('',#155927,#11540) ;
#5987=LINE('',#155929,#11541) ;
#5988=LINE('',#155931,#11542) ;
#5989=LINE('',#155935,#11543) ;
#5990=LINE('',#155937,#11544) ;
#5991=LINE('',#155939,#11545) ;
#5992=LINE('',#155941,#11546) ;
#5993=LINE('',#155943,#11547) ;
#5994=LINE('',#155949,#11548) ;
#5995=LINE('',#155955,#11549) ;
#5996=LINE('',#155961,#11550) ;
#5997=LINE('',#155967,#11551) ;
#5998=LINE('',#155973,#11552) ;
#5999=LINE('',#155979,#11553) ;
#6000=LINE('',#155985,#11554) ;
#6001=LINE('',#155991,#11555) ;
#6002=LINE('',#155997,#11556) ;
#6003=LINE('',#156003,#11557) ;
#6004=LINE('',#156009,#11558) ;
#6005=LINE('',#156015,#11559) ;
#6006=LINE('',#156021,#11560) ;
#6007=LINE('',#156027,#11561) ;
#6008=LINE('',#156033,#11562) ;
#6009=LINE('',#156039,#11563) ;
#6010=LINE('',#156045,#11564) ;
#6011=LINE('',#156051,#11565) ;
#6012=LINE('',#156057,#11566) ;
#6013=LINE('',#156066,#11567) ;
#6014=LINE('',#156068,#11568) ;
#6015=LINE('',#156070,#11569) ;
#6016=LINE('',#156072,#11570) ;
#6017=LINE('',#156074,#11571) ;
#6018=LINE('',#156083,#11572) ;
#6019=LINE('',#156085,#11573) ;
#6020=LINE('',#156087,#11574) ;
#6021=LINE('',#156089,#11575) ;
#6022=LINE('',#156091,#11576) ;
#6023=LINE('',#156100,#11577) ;
#6024=LINE('',#156102,#11578) ;
#6025=LINE('',#156104,#11579) ;
#6026=LINE('',#156106,#11580) ;
#6027=LINE('',#156108,#11581) ;
#6028=LINE('',#156117,#11582) ;
#6029=LINE('',#156119,#11583) ;
#6030=LINE('',#156121,#11584) ;
#6031=LINE('',#156123,#11585) ;
#6032=LINE('',#156125,#11586) ;
#6033=LINE('',#156134,#11587) ;
#6034=LINE('',#156136,#11588) ;
#6035=LINE('',#156138,#11589) ;
#6036=LINE('',#156140,#11590) ;
#6037=LINE('',#156142,#11591) ;
#6038=LINE('',#156151,#11592) ;
#6039=LINE('',#156153,#11593) ;
#6040=LINE('',#156155,#11594) ;
#6041=LINE('',#156157,#11595) ;
#6042=LINE('',#156159,#11596) ;
#6043=LINE('',#156168,#11597) ;
#6044=LINE('',#156170,#11598) ;
#6045=LINE('',#156172,#11599) ;
#6046=LINE('',#156174,#11600) ;
#6047=LINE('',#156176,#11601) ;
#6048=LINE('',#156185,#11602) ;
#6049=LINE('',#156187,#11603) ;
#6050=LINE('',#156189,#11604) ;
#6051=LINE('',#156191,#11605) ;
#6052=LINE('',#156193,#11606) ;
#6053=LINE('',#156202,#11607) ;
#6054=LINE('',#156204,#11608) ;
#6055=LINE('',#156206,#11609) ;
#6056=LINE('',#156208,#11610) ;
#6057=LINE('',#156210,#11611) ;
#6058=LINE('',#156217,#11612) ;
#6059=LINE('',#156219,#11613) ;
#6060=LINE('',#156221,#11614) ;
#6061=LINE('',#156222,#11615) ;
#6062=LINE('',#156226,#11616) ;
#6063=LINE('',#156228,#11617) ;
#6064=LINE('',#156230,#11618) ;
#6065=LINE('',#156232,#11619) ;
#6066=LINE('',#156236,#11620) ;
#6067=LINE('',#156240,#11621) ;
#6068=LINE('',#156242,#11622) ;
#6069=LINE('',#156244,#11623) ;
#6070=LINE('',#156248,#11624) ;
#6071=LINE('',#156252,#11625) ;
#6072=LINE('',#156254,#11626) ;
#6073=LINE('',#156256,#11627) ;
#6074=LINE('',#156260,#11628) ;
#6075=LINE('',#156264,#11629) ;
#6076=LINE('',#156266,#11630) ;
#6077=LINE('',#156268,#11631) ;
#6078=LINE('',#156272,#11632) ;
#6079=LINE('',#156276,#11633) ;
#6080=LINE('',#156278,#11634) ;
#6081=LINE('',#156280,#11635) ;
#6082=LINE('',#156284,#11636) ;
#6083=LINE('',#156288,#11637) ;
#6084=LINE('',#156290,#11638) ;
#6085=LINE('',#156292,#11639) ;
#6086=LINE('',#156296,#11640) ;
#6087=LINE('',#156300,#11641) ;
#6088=LINE('',#156302,#11642) ;
#6089=LINE('',#156304,#11643) ;
#6090=LINE('',#156308,#11644) ;
#6091=LINE('',#156312,#11645) ;
#6092=LINE('',#156314,#11646) ;
#6093=LINE('',#156316,#11647) ;
#6094=LINE('',#156320,#11648) ;
#6095=LINE('',#156324,#11649) ;
#6096=LINE('',#156326,#11650) ;
#6097=LINE('',#156328,#11651) ;
#6098=LINE('',#156332,#11652) ;
#6099=LINE('',#156336,#11653) ;
#6100=LINE('',#156338,#11654) ;
#6101=LINE('',#156340,#11655) ;
#6102=LINE('',#156344,#11656) ;
#6103=LINE('',#156348,#11657) ;
#6104=LINE('',#156350,#11658) ;
#6105=LINE('',#156351,#11659) ;
#6106=LINE('',#156355,#11660) ;
#6107=LINE('',#156361,#11661) ;
#6108=LINE('',#156371,#11662) ;
#6109=LINE('',#156373,#11663) ;
#6110=LINE('',#156375,#11664) ;
#6111=LINE('',#156376,#11665) ;
#6112=LINE('',#156386,#11666) ;
#6113=LINE('',#156395,#11667) ;
#6114=LINE('',#156404,#11668) ;
#6115=LINE('',#156412,#11669) ;
#6116=LINE('',#156415,#11670) ;
#6117=LINE('',#156417,#11671) ;
#6118=LINE('',#156419,#11672) ;
#6119=LINE('',#156420,#11673) ;
#6120=LINE('',#156423,#11674) ;
#6121=LINE('',#156425,#11675) ;
#6122=LINE('',#156427,#11676) ;
#6123=LINE('',#156428,#11677) ;
#6124=LINE('',#156431,#11678) ;
#6125=LINE('',#156433,#11679) ;
#6126=LINE('',#156435,#11680) ;
#6127=LINE('',#156436,#11681) ;
#6128=LINE('',#156439,#11682) ;
#6129=LINE('',#156441,#11683) ;
#6130=LINE('',#156443,#11684) ;
#6131=LINE('',#156444,#11685) ;
#6132=LINE('',#156447,#11686) ;
#6133=LINE('',#156449,#11687) ;
#6134=LINE('',#156451,#11688) ;
#6135=LINE('',#156452,#11689) ;
#6136=LINE('',#156455,#11690) ;
#6137=LINE('',#156457,#11691) ;
#6138=LINE('',#156459,#11692) ;
#6139=LINE('',#156460,#11693) ;
#6140=LINE('',#156463,#11694) ;
#6141=LINE('',#156465,#11695) ;
#6142=LINE('',#156467,#11696) ;
#6143=LINE('',#156468,#11697) ;
#6144=LINE('',#156471,#11698) ;
#6145=LINE('',#156473,#11699) ;
#6146=LINE('',#156475,#11700) ;
#6147=LINE('',#156476,#11701) ;
#6148=LINE('',#156486,#11702) ;
#6149=LINE('',#156495,#11703) ;
#6150=LINE('',#156504,#11704) ;
#6151=LINE('',#156512,#11705) ;
#6152=LINE('',#156516,#11706) ;
#6153=LINE('',#156518,#11707) ;
#6154=LINE('',#156520,#11708) ;
#6155=LINE('',#156521,#11709) ;
#6156=LINE('',#156524,#11710) ;
#6157=LINE('',#156528,#11711) ;
#6158=LINE('',#156532,#11712) ;
#6159=LINE('',#156536,#11713) ;
#6160=LINE('',#156541,#11714) ;
#6161=LINE('',#156543,#11715) ;
#6162=LINE('',#156545,#11716) ;
#6163=LINE('',#156546,#11717) ;
#6164=LINE('',#156548,#11718) ;
#6165=LINE('',#156552,#11719) ;
#6166=LINE('',#156554,#11720) ;
#6167=LINE('',#156556,#11721) ;
#6168=LINE('',#156558,#11722) ;
#6169=LINE('',#156565,#11723) ;
#6170=LINE('',#156569,#11724) ;
#6171=LINE('',#156571,#11725) ;
#6172=LINE('',#156573,#11726) ;
#6173=LINE('',#156574,#11727) ;
#6174=LINE('',#156577,#11728) ;
#6175=LINE('',#156579,#11729) ;
#6176=LINE('',#156580,#11730) ;
#6177=LINE('',#156584,#11731) ;
#6178=LINE('',#156586,#11732) ;
#6179=LINE('',#156588,#11733) ;
#6180=LINE('',#156589,#11734) ;
#6181=LINE('',#156593,#11735) ;
#6182=LINE('',#156595,#11736) ;
#6183=LINE('',#156597,#11737) ;
#6184=LINE('',#156598,#11738) ;
#6185=LINE('',#156601,#11739) ;
#6186=LINE('',#156603,#11740) ;
#6187=LINE('',#156605,#11741) ;
#6188=LINE('',#156606,#11742) ;
#6189=LINE('',#156609,#11743) ;
#6190=LINE('',#156611,#11744) ;
#6191=LINE('',#156613,#11745) ;
#6192=LINE('',#156614,#11746) ;
#6193=LINE('',#156617,#11747) ;
#6194=LINE('',#156619,#11748) ;
#6195=LINE('',#156621,#11749) ;
#6196=LINE('',#156622,#11750) ;
#6197=LINE('',#156625,#11751) ;
#6198=LINE('',#156627,#11752) ;
#6199=LINE('',#156629,#11753) ;
#6200=LINE('',#156630,#11754) ;
#6201=LINE('',#156633,#11755) ;
#6202=LINE('',#156635,#11756) ;
#6203=LINE('',#156637,#11757) ;
#6204=LINE('',#156638,#11758) ;
#6205=LINE('',#156641,#11759) ;
#6206=LINE('',#156643,#11760) ;
#6207=LINE('',#156645,#11761) ;
#6208=LINE('',#156646,#11762) ;
#6209=LINE('',#156649,#11763) ;
#6210=LINE('',#156651,#11764) ;
#6211=LINE('',#156653,#11765) ;
#6212=LINE('',#156654,#11766) ;
#6213=LINE('',#156657,#11767) ;
#6214=LINE('',#156659,#11768) ;
#6215=LINE('',#156661,#11769) ;
#6216=LINE('',#156662,#11770) ;
#6217=LINE('',#156667,#11771) ;
#6218=LINE('',#156671,#11772) ;
#6219=LINE('',#156675,#11773) ;
#6220=LINE('',#156678,#11774) ;
#6221=LINE('',#156683,#11775) ;
#6222=LINE('',#156687,#11776) ;
#6223=LINE('',#156691,#11777) ;
#6224=LINE('',#156694,#11778) ;
#6225=LINE('',#156698,#11779) ;
#6226=LINE('',#156700,#11780) ;
#6227=LINE('',#156702,#11781) ;
#6228=LINE('',#156706,#11782) ;
#6229=LINE('',#156708,#11783) ;
#6230=LINE('',#156710,#11784) ;
#6231=LINE('',#156714,#11785) ;
#6232=LINE('',#156716,#11786) ;
#6233=LINE('',#156718,#11787) ;
#6234=LINE('',#156720,#11788) ;
#6235=LINE('',#156724,#11789) ;
#6236=LINE('',#156725,#11790) ;
#6237=LINE('',#156729,#11791) ;
#6238=LINE('',#156731,#11792) ;
#6239=LINE('',#156733,#11793) ;
#6240=LINE('',#156735,#11794) ;
#6241=LINE('',#156737,#11795) ;
#6242=LINE('',#156741,#11796) ;
#6243=LINE('',#156743,#11797) ;
#6244=LINE('',#156745,#11798) ;
#6245=LINE('',#156747,#11799) ;
#6246=LINE('',#156751,#11800) ;
#6247=LINE('',#156753,#11801) ;
#6248=LINE('',#156755,#11802) ;
#6249=LINE('',#156760,#11803) ;
#6250=LINE('',#156762,#11804) ;
#6251=LINE('',#156764,#11805) ;
#6252=LINE('',#156765,#11806) ;
#6253=LINE('',#156769,#11807) ;
#6254=LINE('',#156771,#11808) ;
#6255=LINE('',#156773,#11809) ;
#6256=LINE('',#156774,#11810) ;
#6257=LINE('',#156778,#11811) ;
#6258=LINE('',#156782,#11812) ;
#6259=LINE('',#156786,#11813) ;
#6260=LINE('',#156791,#11814) ;
#6261=LINE('',#156793,#11815) ;
#6262=LINE('',#156794,#11816) ;
#6263=LINE('',#156798,#11817) ;
#6264=LINE('',#156800,#11818) ;
#6265=LINE('',#156802,#11819) ;
#6266=LINE('',#156803,#11820) ;
#6267=LINE('',#156807,#11821) ;
#6268=LINE('',#156808,#11822) ;
#6269=LINE('',#156810,#11823) ;
#6270=LINE('',#156812,#11824) ;
#6271=LINE('',#156813,#11825) ;
#6272=LINE('',#156817,#11826) ;
#6273=LINE('',#156818,#11827) ;
#6274=LINE('',#156820,#11828) ;
#6275=LINE('',#156822,#11829) ;
#6276=LINE('',#156823,#11830) ;
#6277=LINE('',#156827,#11831) ;
#6278=LINE('',#156829,#11832) ;
#6279=LINE('',#156831,#11833) ;
#6280=LINE('',#156832,#11834) ;
#6281=LINE('',#156836,#11835) ;
#6282=LINE('',#156838,#11836) ;
#6283=LINE('',#156840,#11837) ;
#6284=LINE('',#156841,#11838) ;
#6285=LINE('',#156845,#11839) ;
#6286=LINE('',#156847,#11840) ;
#6287=LINE('',#156849,#11841) ;
#6288=LINE('',#156850,#11842) ;
#6289=LINE('',#156854,#11843) ;
#6290=LINE('',#156856,#11844) ;
#6291=LINE('',#156858,#11845) ;
#6292=LINE('',#156859,#11846) ;
#6293=LINE('',#156863,#11847) ;
#6294=LINE('',#156865,#11848) ;
#6295=LINE('',#156867,#11849) ;
#6296=LINE('',#156868,#11850) ;
#6297=LINE('',#156871,#11851) ;
#6298=LINE('',#156875,#11852) ;
#6299=LINE('',#156879,#11853) ;
#6300=LINE('',#156883,#11854) ;
#6301=LINE('',#156887,#11855) ;
#6302=LINE('',#156889,#11856) ;
#6303=LINE('',#156890,#11857) ;
#6304=LINE('',#156893,#11858) ;
#6305=LINE('',#156895,#11859) ;
#6306=LINE('',#156896,#11860) ;
#6307=LINE('',#156900,#11861) ;
#6308=LINE('',#156901,#11862) ;
#6309=LINE('',#156902,#11863) ;
#6310=LINE('',#156905,#11864) ;
#6311=LINE('',#156907,#11865) ;
#6312=LINE('',#156908,#11866) ;
#6313=LINE('',#156912,#11867) ;
#6314=LINE('',#156914,#11868) ;
#6315=LINE('',#156916,#11869) ;
#6316=LINE('',#156917,#11870) ;
#6317=LINE('',#156920,#11871) ;
#6318=LINE('',#156922,#11872) ;
#6319=LINE('',#156925,#11873) ;
#6320=LINE('',#156927,#11874) ;
#6321=LINE('',#156931,#11875) ;
#6322=LINE('',#156932,#11876) ;
#6323=LINE('',#156936,#11877) ;
#6324=LINE('',#156938,#11878) ;
#6325=LINE('',#156940,#11879) ;
#6326=LINE('',#156941,#11880) ;
#6327=LINE('',#156949,#11881) ;
#6328=LINE('',#156951,#11882) ;
#6329=LINE('',#156953,#11883) ;
#6330=LINE('',#156955,#11884) ;
#6331=LINE('',#156959,#11885) ;
#6332=LINE('',#156961,#11886) ;
#6333=LINE('',#156962,#11887) ;
#6334=LINE('',#156966,#11888) ;
#6335=LINE('',#156968,#11889) ;
#6336=LINE('',#156970,#11890) ;
#6337=LINE('',#156971,#11891) ;
#6338=LINE('',#156975,#11892) ;
#6339=LINE('',#156981,#11893) ;
#6340=LINE('',#156983,#11894) ;
#6341=LINE('',#156985,#11895) ;
#6342=LINE('',#156989,#11896) ;
#6343=LINE('',#156991,#11897) ;
#6344=LINE('',#156992,#11898) ;
#6345=LINE('',#156995,#11899) ;
#6346=LINE('',#156997,#11900) ;
#6347=LINE('',#156998,#11901) ;
#6348=LINE('',#157002,#11902) ;
#6349=LINE('',#157004,#11903) ;
#6350=LINE('',#157006,#11904) ;
#6351=LINE('',#157007,#11905) ;
#6352=LINE('',#157011,#11906) ;
#6353=LINE('',#157013,#11907) ;
#6354=LINE('',#157015,#11908) ;
#6355=LINE('',#157016,#11909) ;
#6356=LINE('',#157020,#11910) ;
#6357=LINE('',#157024,#11911) ;
#6358=LINE('',#157029,#11912) ;
#6359=LINE('',#157033,#11913) ;
#6360=LINE('',#157035,#11914) ;
#6361=LINE('',#157037,#11915) ;
#6362=LINE('',#157038,#11916) ;
#6363=LINE('',#157043,#11917) ;
#6364=LINE('',#157045,#11918) ;
#6365=LINE('',#157047,#11919) ;
#6366=LINE('',#157048,#11920) ;
#6367=LINE('',#157052,#11921) ;
#6368=LINE('',#157054,#11922) ;
#6369=LINE('',#157056,#11923) ;
#6370=LINE('',#157057,#11924) ;
#6371=LINE('',#157061,#11925) ;
#6372=LINE('',#157063,#11926) ;
#6373=LINE('',#157065,#11927) ;
#6374=LINE('',#157066,#11928) ;
#6375=LINE('',#157070,#11929) ;
#6376=LINE('',#157072,#11930) ;
#6377=LINE('',#157074,#11931) ;
#6378=LINE('',#157075,#11932) ;
#6379=LINE('',#157079,#11933) ;
#6380=LINE('',#157081,#11934) ;
#6381=LINE('',#157083,#11935) ;
#6382=LINE('',#157084,#11936) ;
#6383=LINE('',#157087,#11937) ;
#6384=LINE('',#157091,#11938) ;
#6385=LINE('',#157095,#11939) ;
#6386=LINE('',#157099,#11940) ;
#6387=LINE('',#157104,#11941) ;
#6388=LINE('',#157105,#11942) ;
#6389=LINE('',#157106,#11943) ;
#6390=LINE('',#157110,#11944) ;
#6391=LINE('',#157111,#11945) ;
#6392=LINE('',#157112,#11946) ;
#6393=LINE('',#157115,#11947) ;
#6394=LINE('',#157117,#11948) ;
#6395=LINE('',#157118,#11949) ;
#6396=LINE('',#157122,#11950) ;
#6397=LINE('',#157123,#11951) ;
#6398=LINE('',#157124,#11952) ;
#6399=LINE('',#157128,#11953) ;
#6400=LINE('',#157130,#11954) ;
#6401=LINE('',#157132,#11955) ;
#6402=LINE('',#157133,#11956) ;
#6403=LINE('',#157135,#11957) ;
#6404=LINE('',#157137,#11958) ;
#6405=LINE('',#157138,#11959) ;
#6406=LINE('',#157140,#11960) ;
#6407=LINE('',#157141,#11961) ;
#6408=LINE('',#157143,#11962) ;
#6409=LINE('',#157144,#11963) ;
#6410=LINE('',#157151,#11964) ;
#6411=LINE('',#157153,#11965) ;
#6412=LINE('',#157154,#11966) ;
#6413=LINE('',#157158,#11967) ;
#6414=LINE('',#157159,#11968) ;
#6415=LINE('',#157160,#11969) ;
#6416=LINE('',#157168,#11970) ;
#6417=LINE('',#157172,#11971) ;
#6418=LINE('',#157176,#11972) ;
#6419=LINE('',#157178,#11973) ;
#6420=LINE('',#157179,#11974) ;
#6421=LINE('',#157184,#11975) ;
#6422=LINE('',#157188,#11976) ;
#6423=LINE('',#157190,#11977) ;
#6424=LINE('',#157191,#11978) ;
#6425=LINE('',#157196,#11979) ;
#6426=LINE('',#157200,#11980) ;
#6427=LINE('',#157202,#11981) ;
#6428=LINE('',#157203,#11982) ;
#6429=LINE('',#157208,#11983) ;
#6430=LINE('',#157211,#11984) ;
#6431=LINE('',#157212,#11985) ;
#6432=LINE('',#157216,#11986) ;
#6433=LINE('',#157218,#11987) ;
#6434=LINE('',#157220,#11988) ;
#6435=LINE('',#157221,#11989) ;
#6436=LINE('',#157921,#11990) ;
#6437=LINE('',#157923,#11991) ;
#6438=LINE('',#157925,#11992) ;
#6439=LINE('',#157926,#11993) ;
#6440=LINE('',#157930,#11994) ;
#6441=LINE('',#157932,#11995) ;
#6442=LINE('',#157934,#11996) ;
#6443=LINE('',#157935,#11997) ;
#6444=LINE('',#157939,#11998) ;
#6445=LINE('',#157943,#11999) ;
#6446=LINE('',#157947,#12000) ;
#6447=LINE('',#157952,#12001) ;
#6448=LINE('',#157954,#12002) ;
#6449=LINE('',#157955,#12003) ;
#6450=LINE('',#157959,#12004) ;
#6451=LINE('',#157961,#12005) ;
#6452=LINE('',#157963,#12006) ;
#6453=LINE('',#157964,#12007) ;
#6454=LINE('',#157968,#12008) ;
#6455=LINE('',#157970,#12009) ;
#6456=LINE('',#157972,#12010) ;
#6457=LINE('',#157973,#12011) ;
#6458=LINE('',#157977,#12012) ;
#6459=LINE('',#157979,#12013) ;
#6460=LINE('',#157981,#12014) ;
#6461=LINE('',#157982,#12015) ;
#6462=LINE('',#157986,#12016) ;
#6463=LINE('',#157990,#12017) ;
#6464=LINE('',#157994,#12018) ;
#6465=LINE('',#157999,#12019) ;
#6466=LINE('',#158001,#12020) ;
#6467=LINE('',#158002,#12021) ;
#6468=LINE('',#158006,#12022) ;
#6469=LINE('',#158008,#12023) ;
#6470=LINE('',#158010,#12024) ;
#6471=LINE('',#158011,#12025) ;
#6472=LINE('',#158015,#12026) ;
#6473=LINE('',#158017,#12027) ;
#6474=LINE('',#158019,#12028) ;
#6475=LINE('',#158020,#12029) ;
#6476=LINE('',#158024,#12030) ;
#6477=LINE('',#158026,#12031) ;
#6478=LINE('',#158028,#12032) ;
#6479=LINE('',#158029,#12033) ;
#6480=LINE('',#158033,#12034) ;
#6481=LINE('',#158037,#12035) ;
#6482=LINE('',#158041,#12036) ;
#6483=LINE('',#158046,#12037) ;
#6484=LINE('',#158048,#12038) ;
#6485=LINE('',#158049,#12039) ;
#6486=LINE('',#158053,#12040) ;
#6487=LINE('',#158055,#12041) ;
#6488=LINE('',#158057,#12042) ;
#6489=LINE('',#158058,#12043) ;
#6490=LINE('',#158062,#12044) ;
#6491=LINE('',#158064,#12045) ;
#6492=LINE('',#158066,#12046) ;
#6493=LINE('',#158067,#12047) ;
#6494=LINE('',#158071,#12048) ;
#6495=LINE('',#158073,#12049) ;
#6496=LINE('',#158075,#12050) ;
#6497=LINE('',#158076,#12051) ;
#6498=LINE('',#158080,#12052) ;
#6499=LINE('',#158084,#12053) ;
#6500=LINE('',#158088,#12054) ;
#6501=LINE('',#158093,#12055) ;
#6502=LINE('',#158095,#12056) ;
#6503=LINE('',#158096,#12057) ;
#6504=LINE('',#158100,#12058) ;
#6505=LINE('',#158102,#12059) ;
#6506=LINE('',#158104,#12060) ;
#6507=LINE('',#158105,#12061) ;
#6508=LINE('',#158109,#12062) ;
#6509=LINE('',#158111,#12063) ;
#6510=LINE('',#158113,#12064) ;
#6511=LINE('',#158114,#12065) ;
#6512=LINE('',#158118,#12066) ;
#6513=LINE('',#158120,#12067) ;
#6514=LINE('',#158122,#12068) ;
#6515=LINE('',#158123,#12069) ;
#6516=LINE('',#158127,#12070) ;
#6517=LINE('',#158131,#12071) ;
#6518=LINE('',#158135,#12072) ;
#6519=LINE('',#158140,#12073) ;
#6520=LINE('',#158142,#12074) ;
#6521=LINE('',#158143,#12075) ;
#6522=LINE('',#158147,#12076) ;
#6523=LINE('',#158149,#12077) ;
#6524=LINE('',#158151,#12078) ;
#6525=LINE('',#158152,#12079) ;
#6526=LINE('',#158156,#12080) ;
#6527=LINE('',#158158,#12081) ;
#6528=LINE('',#158160,#12082) ;
#6529=LINE('',#158161,#12083) ;
#6530=LINE('',#158165,#12084) ;
#6531=LINE('',#158167,#12085) ;
#6532=LINE('',#158169,#12086) ;
#6533=LINE('',#158170,#12087) ;
#6534=LINE('',#158174,#12088) ;
#6535=LINE('',#158178,#12089) ;
#6536=LINE('',#158182,#12090) ;
#6537=LINE('',#158187,#12091) ;
#6538=LINE('',#158189,#12092) ;
#6539=LINE('',#158190,#12093) ;
#6540=LINE('',#158194,#12094) ;
#6541=LINE('',#158196,#12095) ;
#6542=LINE('',#158198,#12096) ;
#6543=LINE('',#158199,#12097) ;
#6544=LINE('',#158203,#12098) ;
#6545=LINE('',#158205,#12099) ;
#6546=LINE('',#158207,#12100) ;
#6547=LINE('',#158208,#12101) ;
#6548=LINE('',#158212,#12102) ;
#6549=LINE('',#158214,#12103) ;
#6550=LINE('',#158216,#12104) ;
#6551=LINE('',#158217,#12105) ;
#6552=LINE('',#158221,#12106) ;
#6553=LINE('',#158225,#12107) ;
#6554=LINE('',#158229,#12108) ;
#6555=LINE('',#158234,#12109) ;
#6556=LINE('',#158236,#12110) ;
#6557=LINE('',#158237,#12111) ;
#6558=LINE('',#158241,#12112) ;
#6559=LINE('',#158243,#12113) ;
#6560=LINE('',#158245,#12114) ;
#6561=LINE('',#158246,#12115) ;
#6562=LINE('',#158250,#12116) ;
#6563=LINE('',#158252,#12117) ;
#6564=LINE('',#158254,#12118) ;
#6565=LINE('',#158255,#12119) ;
#6566=LINE('',#158259,#12120) ;
#6567=LINE('',#158261,#12121) ;
#6568=LINE('',#158263,#12122) ;
#6569=LINE('',#158264,#12123) ;
#6570=LINE('',#158268,#12124) ;
#6571=LINE('',#158272,#12125) ;
#6572=LINE('',#158276,#12126) ;
#6573=LINE('',#158281,#12127) ;
#6574=LINE('',#158283,#12128) ;
#6575=LINE('',#158284,#12129) ;
#6576=LINE('',#158288,#12130) ;
#6577=LINE('',#158290,#12131) ;
#6578=LINE('',#158292,#12132) ;
#6579=LINE('',#158293,#12133) ;
#6580=LINE('',#158297,#12134) ;
#6581=LINE('',#158299,#12135) ;
#6582=LINE('',#158301,#12136) ;
#6583=LINE('',#158302,#12137) ;
#6584=LINE('',#158306,#12138) ;
#6585=LINE('',#158308,#12139) ;
#6586=LINE('',#158310,#12140) ;
#6587=LINE('',#158311,#12141) ;
#6588=LINE('',#158315,#12142) ;
#6589=LINE('',#158319,#12143) ;
#6590=LINE('',#158323,#12144) ;
#6591=LINE('',#158328,#12145) ;
#6592=LINE('',#158330,#12146) ;
#6593=LINE('',#158331,#12147) ;
#6594=LINE('',#158335,#12148) ;
#6595=LINE('',#158337,#12149) ;
#6596=LINE('',#158339,#12150) ;
#6597=LINE('',#158340,#12151) ;
#6598=LINE('',#158344,#12152) ;
#6599=LINE('',#158345,#12153) ;
#6600=LINE('',#158347,#12154) ;
#6601=LINE('',#158349,#12155) ;
#6602=LINE('',#158350,#12156) ;
#6603=LINE('',#158354,#12157) ;
#6604=LINE('',#158358,#12158) ;
#6605=LINE('',#158359,#12159) ;
#6606=LINE('',#158361,#12160) ;
#6607=LINE('',#158363,#12161) ;
#6608=LINE('',#158368,#12162) ;
#6609=LINE('',#158372,#12163) ;
#6610=LINE('',#158373,#12164) ;
#6611=LINE('',#158375,#12165) ;
#6612=LINE('',#158377,#12166) ;
#6613=LINE('',#158382,#12167) ;
#6614=LINE('',#158386,#12168) ;
#6615=LINE('',#158387,#12169) ;
#6616=LINE('',#158389,#12170) ;
#6617=LINE('',#158391,#12171) ;
#6618=LINE('',#158396,#12172) ;
#6619=LINE('',#158400,#12173) ;
#6620=LINE('',#158401,#12174) ;
#6621=LINE('',#158403,#12175) ;
#6622=LINE('',#158405,#12176) ;
#6623=LINE('',#158410,#12177) ;
#6624=LINE('',#158414,#12178) ;
#6625=LINE('',#158415,#12179) ;
#6626=LINE('',#158417,#12180) ;
#6627=LINE('',#158419,#12181) ;
#6628=LINE('',#158424,#12182) ;
#6629=LINE('',#158428,#12183) ;
#6630=LINE('',#158429,#12184) ;
#6631=LINE('',#158431,#12185) ;
#6632=LINE('',#158433,#12186) ;
#6633=LINE('',#158438,#12187) ;
#6634=LINE('',#158442,#12188) ;
#6635=LINE('',#158443,#12189) ;
#6636=LINE('',#158445,#12190) ;
#6637=LINE('',#158447,#12191) ;
#6638=LINE('',#158452,#12192) ;
#6639=LINE('',#158456,#12193) ;
#6640=LINE('',#158457,#12194) ;
#6641=LINE('',#158459,#12195) ;
#6642=LINE('',#158461,#12196) ;
#6643=LINE('',#158466,#12197) ;
#6644=LINE('',#158467,#12198) ;
#6645=LINE('',#158469,#12199) ;
#6646=LINE('',#158471,#12200) ;
#6647=LINE('',#158472,#12201) ;
#6648=LINE('',#158476,#12202) ;
#6649=LINE('',#158480,#12203) ;
#6650=LINE('',#158481,#12204) ;
#6651=LINE('',#158483,#12205) ;
#6652=LINE('',#158485,#12206) ;
#6653=LINE('',#158490,#12207) ;
#6654=LINE('',#158494,#12208) ;
#6655=LINE('',#158495,#12209) ;
#6656=LINE('',#158497,#12210) ;
#6657=LINE('',#158499,#12211) ;
#6658=LINE('',#158504,#12212) ;
#6659=LINE('',#158508,#12213) ;
#6660=LINE('',#158509,#12214) ;
#6661=LINE('',#158511,#12215) ;
#6662=LINE('',#158513,#12216) ;
#6663=LINE('',#158518,#12217) ;
#6664=LINE('',#158522,#12218) ;
#6665=LINE('',#158523,#12219) ;
#6666=LINE('',#158525,#12220) ;
#6667=LINE('',#158527,#12221) ;
#6668=LINE('',#158532,#12222) ;
#6669=LINE('',#158536,#12223) ;
#6670=LINE('',#158537,#12224) ;
#6671=LINE('',#158539,#12225) ;
#6672=LINE('',#158541,#12226) ;
#6673=LINE('',#158546,#12227) ;
#6674=LINE('',#158550,#12228) ;
#6675=LINE('',#158551,#12229) ;
#6676=LINE('',#158553,#12230) ;
#6677=LINE('',#158555,#12231) ;
#6678=LINE('',#158560,#12232) ;
#6679=LINE('',#158564,#12233) ;
#6680=LINE('',#158565,#12234) ;
#6681=LINE('',#158567,#12235) ;
#6682=LINE('',#158569,#12236) ;
#6683=LINE('',#158574,#12237) ;
#6684=LINE('',#158578,#12238) ;
#6685=LINE('',#158579,#12239) ;
#6686=LINE('',#158581,#12240) ;
#6687=LINE('',#158583,#12241) ;
#6688=LINE('',#158588,#12242) ;
#6689=LINE('',#158590,#12243) ;
#6690=LINE('',#158592,#12244) ;
#6691=LINE('',#158593,#12245) ;
#6692=LINE('',#158597,#12246) ;
#6693=LINE('',#158599,#12247) ;
#6694=LINE('',#158601,#12248) ;
#6695=LINE('',#158602,#12249) ;
#6696=LINE('',#158606,#12250) ;
#6697=LINE('',#158608,#12251) ;
#6698=LINE('',#158610,#12252) ;
#6699=LINE('',#158611,#12253) ;
#6700=LINE('',#158615,#12254) ;
#6701=LINE('',#158617,#12255) ;
#6702=LINE('',#158619,#12256) ;
#6703=LINE('',#158620,#12257) ;
#6704=LINE('',#158624,#12258) ;
#6705=LINE('',#158626,#12259) ;
#6706=LINE('',#158628,#12260) ;
#6707=LINE('',#158629,#12261) ;
#6708=LINE('',#158633,#12262) ;
#6709=LINE('',#158635,#12263) ;
#6710=LINE('',#158637,#12264) ;
#6711=LINE('',#158638,#12265) ;
#6712=LINE('',#158642,#12266) ;
#6713=LINE('',#158644,#12267) ;
#6714=LINE('',#158646,#12268) ;
#6715=LINE('',#158647,#12269) ;
#6716=LINE('',#158651,#12270) ;
#6717=LINE('',#158653,#12271) ;
#6718=LINE('',#158655,#12272) ;
#6719=LINE('',#158656,#12273) ;
#6720=LINE('',#158660,#12274) ;
#6721=LINE('',#158662,#12275) ;
#6722=LINE('',#158664,#12276) ;
#6723=LINE('',#158665,#12277) ;
#6724=LINE('',#158669,#12278) ;
#6725=LINE('',#158671,#12279) ;
#6726=LINE('',#158673,#12280) ;
#6727=LINE('',#158674,#12281) ;
#6728=LINE('',#158678,#12282) ;
#6729=LINE('',#158680,#12283) ;
#6730=LINE('',#158682,#12284) ;
#6731=LINE('',#158683,#12285) ;
#6732=LINE('',#158687,#12286) ;
#6733=LINE('',#158689,#12287) ;
#6734=LINE('',#158691,#12288) ;
#6735=LINE('',#158692,#12289) ;
#6736=LINE('',#158696,#12290) ;
#6737=LINE('',#158698,#12291) ;
#6738=LINE('',#158700,#12292) ;
#6739=LINE('',#158701,#12293) ;
#6740=LINE('',#158705,#12294) ;
#6741=LINE('',#158707,#12295) ;
#6742=LINE('',#158709,#12296) ;
#6743=LINE('',#158710,#12297) ;
#6744=LINE('',#158714,#12298) ;
#6745=LINE('',#158716,#12299) ;
#6746=LINE('',#158718,#12300) ;
#6747=LINE('',#158719,#12301) ;
#6748=LINE('',#158723,#12302) ;
#6749=LINE('',#158725,#12303) ;
#6750=LINE('',#158727,#12304) ;
#6751=LINE('',#158728,#12305) ;
#6752=LINE('',#158732,#12306) ;
#6753=LINE('',#158734,#12307) ;
#6754=LINE('',#158736,#12308) ;
#6755=LINE('',#158737,#12309) ;
#6756=LINE('',#158741,#12310) ;
#6757=LINE('',#158743,#12311) ;
#6758=LINE('',#158745,#12312) ;
#6759=LINE('',#158746,#12313) ;
#6760=LINE('',#158750,#12314) ;
#6761=LINE('',#158752,#12315) ;
#6762=LINE('',#158754,#12316) ;
#6763=LINE('',#158755,#12317) ;
#6764=LINE('',#158759,#12318) ;
#6765=LINE('',#158761,#12319) ;
#6766=LINE('',#158763,#12320) ;
#6767=LINE('',#158764,#12321) ;
#6768=LINE('',#158768,#12322) ;
#6769=LINE('',#158770,#12323) ;
#6770=LINE('',#158772,#12324) ;
#6771=LINE('',#158773,#12325) ;
#6772=LINE('',#158777,#12326) ;
#6773=LINE('',#158779,#12327) ;
#6774=LINE('',#158781,#12328) ;
#6775=LINE('',#158782,#12329) ;
#6776=LINE('',#158786,#12330) ;
#6777=LINE('',#158788,#12331) ;
#6778=LINE('',#158790,#12332) ;
#6779=LINE('',#158791,#12333) ;
#6780=LINE('',#158795,#12334) ;
#6781=LINE('',#158797,#12335) ;
#6782=LINE('',#158799,#12336) ;
#6783=LINE('',#158800,#12337) ;
#6784=LINE('',#158804,#12338) ;
#6785=LINE('',#158806,#12339) ;
#6786=LINE('',#158808,#12340) ;
#6787=LINE('',#158809,#12341) ;
#6788=LINE('',#158813,#12342) ;
#6789=LINE('',#158815,#12343) ;
#6790=LINE('',#158817,#12344) ;
#6791=LINE('',#158818,#12345) ;
#6792=LINE('',#158822,#12346) ;
#6793=LINE('',#158824,#12347) ;
#6794=LINE('',#158826,#12348) ;
#6795=LINE('',#158827,#12349) ;
#6796=LINE('',#158831,#12350) ;
#6797=LINE('',#158833,#12351) ;
#6798=LINE('',#158835,#12352) ;
#6799=LINE('',#158836,#12353) ;
#6800=LINE('',#158840,#12354) ;
#6801=LINE('',#158842,#12355) ;
#6802=LINE('',#158844,#12356) ;
#6803=LINE('',#158845,#12357) ;
#6804=LINE('',#158849,#12358) ;
#6805=LINE('',#158851,#12359) ;
#6806=LINE('',#158853,#12360) ;
#6807=LINE('',#158854,#12361) ;
#6808=LINE('',#158858,#12362) ;
#6809=LINE('',#158860,#12363) ;
#6810=LINE('',#158862,#12364) ;
#6811=LINE('',#158863,#12365) ;
#6812=LINE('',#158867,#12366) ;
#6813=LINE('',#158869,#12367) ;
#6814=LINE('',#158871,#12368) ;
#6815=LINE('',#158872,#12369) ;
#6816=LINE('',#158876,#12370) ;
#6817=LINE('',#158878,#12371) ;
#6818=LINE('',#158880,#12372) ;
#6819=LINE('',#158881,#12373) ;
#6820=LINE('',#158885,#12374) ;
#6821=LINE('',#158887,#12375) ;
#6822=LINE('',#158889,#12376) ;
#6823=LINE('',#158890,#12377) ;
#6824=LINE('',#158894,#12378) ;
#6825=LINE('',#158896,#12379) ;
#6826=LINE('',#158898,#12380) ;
#6827=LINE('',#158899,#12381) ;
#6828=LINE('',#158903,#12382) ;
#6829=LINE('',#158905,#12383) ;
#6830=LINE('',#158907,#12384) ;
#6831=LINE('',#158908,#12385) ;
#6832=LINE('',#158912,#12386) ;
#6833=LINE('',#158914,#12387) ;
#6834=LINE('',#158916,#12388) ;
#6835=LINE('',#158917,#12389) ;
#6836=LINE('',#158920,#12390) ;
#6837=LINE('',#158924,#12391) ;
#6838=LINE('',#158928,#12392) ;
#6839=LINE('',#158932,#12393) ;
#6840=LINE('',#158936,#12394) ;
#6841=LINE('',#158938,#12395) ;
#6842=LINE('',#158939,#12396) ;
#6843=LINE('',#158942,#12397) ;
#6844=LINE('',#158944,#12398) ;
#6845=LINE('',#158945,#12399) ;
#6846=LINE('',#158949,#12400) ;
#6847=LINE('',#158950,#12401) ;
#6848=LINE('',#158951,#12402) ;
#6849=LINE('',#158954,#12403) ;
#6850=LINE('',#158956,#12404) ;
#6851=LINE('',#158957,#12405) ;
#6852=LINE('',#158961,#12406) ;
#6853=LINE('',#158963,#12407) ;
#6854=LINE('',#158965,#12408) ;
#6855=LINE('',#158966,#12409) ;
#6856=LINE('',#158969,#12410) ;
#6857=LINE('',#158973,#12411) ;
#6858=LINE('',#158977,#12412) ;
#6859=LINE('',#158981,#12413) ;
#6860=LINE('',#158985,#12414) ;
#6861=LINE('',#158987,#12415) ;
#6862=LINE('',#158988,#12416) ;
#6863=LINE('',#158991,#12417) ;
#6864=LINE('',#158993,#12418) ;
#6865=LINE('',#158994,#12419) ;
#6866=LINE('',#158998,#12420) ;
#6867=LINE('',#158999,#12421) ;
#6868=LINE('',#159000,#12422) ;
#6869=LINE('',#159003,#12423) ;
#6870=LINE('',#159005,#12424) ;
#6871=LINE('',#159006,#12425) ;
#6872=LINE('',#159010,#12426) ;
#6873=LINE('',#159012,#12427) ;
#6874=LINE('',#159014,#12428) ;
#6875=LINE('',#159015,#12429) ;
#6876=LINE('',#159018,#12430) ;
#6877=LINE('',#159022,#12431) ;
#6878=LINE('',#159026,#12432) ;
#6879=LINE('',#159030,#12433) ;
#6880=LINE('',#159034,#12434) ;
#6881=LINE('',#159036,#12435) ;
#6882=LINE('',#159037,#12436) ;
#6883=LINE('',#159040,#12437) ;
#6884=LINE('',#159042,#12438) ;
#6885=LINE('',#159043,#12439) ;
#6886=LINE('',#159047,#12440) ;
#6887=LINE('',#159048,#12441) ;
#6888=LINE('',#159049,#12442) ;
#6889=LINE('',#159052,#12443) ;
#6890=LINE('',#159054,#12444) ;
#6891=LINE('',#159055,#12445) ;
#6892=LINE('',#159059,#12446) ;
#6893=LINE('',#159061,#12447) ;
#6894=LINE('',#159063,#12448) ;
#6895=LINE('',#159064,#12449) ;
#6896=LINE('',#159067,#12450) ;
#6897=LINE('',#159071,#12451) ;
#6898=LINE('',#159075,#12452) ;
#6899=LINE('',#159079,#12453) ;
#6900=LINE('',#159083,#12454) ;
#6901=LINE('',#159085,#12455) ;
#6902=LINE('',#159086,#12456) ;
#6903=LINE('',#159089,#12457) ;
#6904=LINE('',#159091,#12458) ;
#6905=LINE('',#159092,#12459) ;
#6906=LINE('',#159096,#12460) ;
#6907=LINE('',#159097,#12461) ;
#6908=LINE('',#159098,#12462) ;
#6909=LINE('',#159101,#12463) ;
#6910=LINE('',#159103,#12464) ;
#6911=LINE('',#159104,#12465) ;
#6912=LINE('',#159108,#12466) ;
#6913=LINE('',#159110,#12467) ;
#6914=LINE('',#159112,#12468) ;
#6915=LINE('',#159113,#12469) ;
#6916=LINE('',#159116,#12470) ;
#6917=LINE('',#159120,#12471) ;
#6918=LINE('',#159124,#12472) ;
#6919=LINE('',#159128,#12473) ;
#6920=LINE('',#159132,#12474) ;
#6921=LINE('',#159134,#12475) ;
#6922=LINE('',#159135,#12476) ;
#6923=LINE('',#159138,#12477) ;
#6924=LINE('',#159140,#12478) ;
#6925=LINE('',#159141,#12479) ;
#6926=LINE('',#159145,#12480) ;
#6927=LINE('',#159146,#12481) ;
#6928=LINE('',#159147,#12482) ;
#6929=LINE('',#159150,#12483) ;
#6930=LINE('',#159152,#12484) ;
#6931=LINE('',#159153,#12485) ;
#6932=LINE('',#159157,#12486) ;
#6933=LINE('',#159159,#12487) ;
#6934=LINE('',#159161,#12488) ;
#6935=LINE('',#159162,#12489) ;
#6936=LINE('',#159165,#12490) ;
#6937=LINE('',#159169,#12491) ;
#6938=LINE('',#159173,#12492) ;
#6939=LINE('',#159177,#12493) ;
#6940=LINE('',#159181,#12494) ;
#6941=LINE('',#159183,#12495) ;
#6942=LINE('',#159184,#12496) ;
#6943=LINE('',#159187,#12497) ;
#6944=LINE('',#159189,#12498) ;
#6945=LINE('',#159190,#12499) ;
#6946=LINE('',#159194,#12500) ;
#6947=LINE('',#159195,#12501) ;
#6948=LINE('',#159196,#12502) ;
#6949=LINE('',#159199,#12503) ;
#6950=LINE('',#159201,#12504) ;
#6951=LINE('',#159202,#12505) ;
#6952=LINE('',#159206,#12506) ;
#6953=LINE('',#159208,#12507) ;
#6954=LINE('',#159210,#12508) ;
#6955=LINE('',#159211,#12509) ;
#6956=LINE('',#159214,#12510) ;
#6957=LINE('',#159218,#12511) ;
#6958=LINE('',#159222,#12512) ;
#6959=LINE('',#159226,#12513) ;
#6960=LINE('',#159230,#12514) ;
#6961=LINE('',#159232,#12515) ;
#6962=LINE('',#159233,#12516) ;
#6963=LINE('',#159236,#12517) ;
#6964=LINE('',#159238,#12518) ;
#6965=LINE('',#159239,#12519) ;
#6966=LINE('',#159243,#12520) ;
#6967=LINE('',#159244,#12521) ;
#6968=LINE('',#159245,#12522) ;
#6969=LINE('',#159248,#12523) ;
#6970=LINE('',#159250,#12524) ;
#6971=LINE('',#159251,#12525) ;
#6972=LINE('',#159255,#12526) ;
#6973=LINE('',#159257,#12527) ;
#6974=LINE('',#159259,#12528) ;
#6975=LINE('',#159260,#12529) ;
#6976=LINE('',#159263,#12530) ;
#6977=LINE('',#159267,#12531) ;
#6978=LINE('',#159271,#12532) ;
#6979=LINE('',#159275,#12533) ;
#6980=LINE('',#159279,#12534) ;
#6981=LINE('',#159281,#12535) ;
#6982=LINE('',#159282,#12536) ;
#6983=LINE('',#159285,#12537) ;
#6984=LINE('',#159287,#12538) ;
#6985=LINE('',#159288,#12539) ;
#6986=LINE('',#159292,#12540) ;
#6987=LINE('',#159293,#12541) ;
#6988=LINE('',#159294,#12542) ;
#6989=LINE('',#159297,#12543) ;
#6990=LINE('',#159299,#12544) ;
#6991=LINE('',#159300,#12545) ;
#6992=LINE('',#159304,#12546) ;
#6993=LINE('',#159306,#12547) ;
#6994=LINE('',#159308,#12548) ;
#6995=LINE('',#159309,#12549) ;
#6996=LINE('',#159312,#12550) ;
#6997=LINE('',#159316,#12551) ;
#6998=LINE('',#159320,#12552) ;
#6999=LINE('',#159324,#12553) ;
#7000=LINE('',#159328,#12554) ;
#7001=LINE('',#159330,#12555) ;
#7002=LINE('',#159331,#12556) ;
#7003=LINE('',#159334,#12557) ;
#7004=LINE('',#159336,#12558) ;
#7005=LINE('',#159337,#12559) ;
#7006=LINE('',#159341,#12560) ;
#7007=LINE('',#159342,#12561) ;
#7008=LINE('',#159343,#12562) ;
#7009=LINE('',#159346,#12563) ;
#7010=LINE('',#159348,#12564) ;
#7011=LINE('',#159349,#12565) ;
#7012=LINE('',#159353,#12566) ;
#7013=LINE('',#159355,#12567) ;
#7014=LINE('',#159357,#12568) ;
#7015=LINE('',#159358,#12569) ;
#7016=LINE('',#159362,#12570) ;
#7017=LINE('',#159364,#12571) ;
#7018=LINE('',#159366,#12572) ;
#7019=LINE('',#159367,#12573) ;
#7020=LINE('',#159371,#12574) ;
#7021=LINE('',#159373,#12575) ;
#7022=LINE('',#159375,#12576) ;
#7023=LINE('',#159376,#12577) ;
#7024=LINE('',#159380,#12578) ;
#7025=LINE('',#159382,#12579) ;
#7026=LINE('',#159384,#12580) ;
#7027=LINE('',#159385,#12581) ;
#7028=LINE('',#159389,#12582) ;
#7029=LINE('',#159391,#12583) ;
#7030=LINE('',#159393,#12584) ;
#7031=LINE('',#159394,#12585) ;
#7032=LINE('',#159398,#12586) ;
#7033=LINE('',#159400,#12587) ;
#7034=LINE('',#159402,#12588) ;
#7035=LINE('',#159403,#12589) ;
#7036=LINE('',#159407,#12590) ;
#7037=LINE('',#159409,#12591) ;
#7038=LINE('',#159411,#12592) ;
#7039=LINE('',#159412,#12593) ;
#7040=LINE('',#159416,#12594) ;
#7041=LINE('',#159418,#12595) ;
#7042=LINE('',#159420,#12596) ;
#7043=LINE('',#159421,#12597) ;
#7044=LINE('',#159425,#12598) ;
#7045=LINE('',#159427,#12599) ;
#7046=LINE('',#159429,#12600) ;
#7047=LINE('',#159430,#12601) ;
#7048=LINE('',#159438,#12602) ;
#7049=LINE('',#159440,#12603) ;
#7050=LINE('',#159442,#12604) ;
#7051=LINE('',#159444,#12605) ;
#7052=LINE('',#159448,#12606) ;
#7053=LINE('',#159450,#12607) ;
#7054=LINE('',#159451,#12608) ;
#7055=LINE('',#159455,#12609) ;
#7056=LINE('',#159457,#12610) ;
#7057=LINE('',#159459,#12611) ;
#7058=LINE('',#159460,#12612) ;
#7059=LINE('',#159464,#12613) ;
#7060=LINE('',#159470,#12614) ;
#7061=LINE('',#159472,#12615) ;
#7062=LINE('',#159474,#12616) ;
#7063=LINE('',#159478,#12617) ;
#7064=LINE('',#159480,#12618) ;
#7065=LINE('',#159481,#12619) ;
#7066=LINE('',#159485,#12620) ;
#7067=LINE('',#159487,#12621) ;
#7068=LINE('',#159489,#12622) ;
#7069=LINE('',#159490,#12623) ;
#7070=LINE('',#159498,#12624) ;
#7071=LINE('',#159500,#12625) ;
#7072=LINE('',#159502,#12626) ;
#7073=LINE('',#159504,#12627) ;
#7074=LINE('',#159508,#12628) ;
#7075=LINE('',#159510,#12629) ;
#7076=LINE('',#159511,#12630) ;
#7077=LINE('',#159515,#12631) ;
#7078=LINE('',#159517,#12632) ;
#7079=LINE('',#159519,#12633) ;
#7080=LINE('',#159520,#12634) ;
#7081=LINE('',#159524,#12635) ;
#7082=LINE('',#159530,#12636) ;
#7083=LINE('',#159532,#12637) ;
#7084=LINE('',#159534,#12638) ;
#7085=LINE('',#159538,#12639) ;
#7086=LINE('',#159540,#12640) ;
#7087=LINE('',#159541,#12641) ;
#7088=LINE('',#159545,#12642) ;
#7089=LINE('',#159547,#12643) ;
#7090=LINE('',#159549,#12644) ;
#7091=LINE('',#159550,#12645) ;
#7092=LINE('',#159558,#12646) ;
#7093=LINE('',#159560,#12647) ;
#7094=LINE('',#159562,#12648) ;
#7095=LINE('',#159564,#12649) ;
#7096=LINE('',#159568,#12650) ;
#7097=LINE('',#159570,#12651) ;
#7098=LINE('',#159571,#12652) ;
#7099=LINE('',#159575,#12653) ;
#7100=LINE('',#159577,#12654) ;
#7101=LINE('',#159579,#12655) ;
#7102=LINE('',#159580,#12656) ;
#7103=LINE('',#159584,#12657) ;
#7104=LINE('',#159590,#12658) ;
#7105=LINE('',#159592,#12659) ;
#7106=LINE('',#159594,#12660) ;
#7107=LINE('',#159598,#12661) ;
#7108=LINE('',#159600,#12662) ;
#7109=LINE('',#159601,#12663) ;
#7110=LINE('',#159605,#12664) ;
#7111=LINE('',#159607,#12665) ;
#7112=LINE('',#159609,#12666) ;
#7113=LINE('',#159610,#12667) ;
#7114=LINE('',#159618,#12668) ;
#7115=LINE('',#159620,#12669) ;
#7116=LINE('',#159622,#12670) ;
#7117=LINE('',#159624,#12671) ;
#7118=LINE('',#159628,#12672) ;
#7119=LINE('',#159630,#12673) ;
#7120=LINE('',#159631,#12674) ;
#7121=LINE('',#159635,#12675) ;
#7122=LINE('',#159637,#12676) ;
#7123=LINE('',#159639,#12677) ;
#7124=LINE('',#159640,#12678) ;
#7125=LINE('',#159644,#12679) ;
#7126=LINE('',#159650,#12680) ;
#7127=LINE('',#159652,#12681) ;
#7128=LINE('',#159654,#12682) ;
#7129=LINE('',#159658,#12683) ;
#7130=LINE('',#159660,#12684) ;
#7131=LINE('',#159661,#12685) ;
#7132=LINE('',#159665,#12686) ;
#7133=LINE('',#159667,#12687) ;
#7134=LINE('',#159669,#12688) ;
#7135=LINE('',#159670,#12689) ;
#7136=LINE('',#159678,#12690) ;
#7137=LINE('',#159680,#12691) ;
#7138=LINE('',#159682,#12692) ;
#7139=LINE('',#159684,#12693) ;
#7140=LINE('',#159688,#12694) ;
#7141=LINE('',#159690,#12695) ;
#7142=LINE('',#159691,#12696) ;
#7143=LINE('',#159695,#12697) ;
#7144=LINE('',#159697,#12698) ;
#7145=LINE('',#159699,#12699) ;
#7146=LINE('',#159700,#12700) ;
#7147=LINE('',#159704,#12701) ;
#7148=LINE('',#159710,#12702) ;
#7149=LINE('',#159712,#12703) ;
#7150=LINE('',#159714,#12704) ;
#7151=LINE('',#159718,#12705) ;
#7152=LINE('',#159720,#12706) ;
#7153=LINE('',#159721,#12707) ;
#7154=LINE('',#159725,#12708) ;
#7155=LINE('',#159727,#12709) ;
#7156=LINE('',#159729,#12710) ;
#7157=LINE('',#159730,#12711) ;
#7158=LINE('',#159738,#12712) ;
#7159=LINE('',#159740,#12713) ;
#7160=LINE('',#159742,#12714) ;
#7161=LINE('',#159744,#12715) ;
#7162=LINE('',#159748,#12716) ;
#7163=LINE('',#159750,#12717) ;
#7164=LINE('',#159751,#12718) ;
#7165=LINE('',#159755,#12719) ;
#7166=LINE('',#159757,#12720) ;
#7167=LINE('',#159759,#12721) ;
#7168=LINE('',#159760,#12722) ;
#7169=LINE('',#159764,#12723) ;
#7170=LINE('',#159770,#12724) ;
#7171=LINE('',#159772,#12725) ;
#7172=LINE('',#159774,#12726) ;
#7173=LINE('',#159778,#12727) ;
#7174=LINE('',#159780,#12728) ;
#7175=LINE('',#159781,#12729) ;
#7176=LINE('',#159785,#12730) ;
#7177=LINE('',#159787,#12731) ;
#7178=LINE('',#159789,#12732) ;
#7179=LINE('',#159790,#12733) ;
#7180=LINE('',#159798,#12734) ;
#7181=LINE('',#159800,#12735) ;
#7182=LINE('',#159802,#12736) ;
#7183=LINE('',#159804,#12737) ;
#7184=LINE('',#159808,#12738) ;
#7185=LINE('',#159810,#12739) ;
#7186=LINE('',#159811,#12740) ;
#7187=LINE('',#159815,#12741) ;
#7188=LINE('',#159817,#12742) ;
#7189=LINE('',#159819,#12743) ;
#7190=LINE('',#159820,#12744) ;
#7191=LINE('',#159824,#12745) ;
#7192=LINE('',#159830,#12746) ;
#7193=LINE('',#159832,#12747) ;
#7194=LINE('',#159834,#12748) ;
#7195=LINE('',#159838,#12749) ;
#7196=LINE('',#159840,#12750) ;
#7197=LINE('',#159841,#12751) ;
#7198=LINE('',#159845,#12752) ;
#7199=LINE('',#159847,#12753) ;
#7200=LINE('',#159849,#12754) ;
#7201=LINE('',#159850,#12755) ;
#7202=LINE('',#159858,#12756) ;
#7203=LINE('',#159860,#12757) ;
#7204=LINE('',#159862,#12758) ;
#7205=LINE('',#159864,#12759) ;
#7206=LINE('',#159868,#12760) ;
#7207=LINE('',#159870,#12761) ;
#7208=LINE('',#159871,#12762) ;
#7209=LINE('',#159875,#12763) ;
#7210=LINE('',#159877,#12764) ;
#7211=LINE('',#159879,#12765) ;
#7212=LINE('',#159880,#12766) ;
#7213=LINE('',#159884,#12767) ;
#7214=LINE('',#159890,#12768) ;
#7215=LINE('',#159892,#12769) ;
#7216=LINE('',#159894,#12770) ;
#7217=LINE('',#159898,#12771) ;
#7218=LINE('',#159900,#12772) ;
#7219=LINE('',#159901,#12773) ;
#7220=LINE('',#159905,#12774) ;
#7221=LINE('',#159907,#12775) ;
#7222=LINE('',#159909,#12776) ;
#7223=LINE('',#159910,#12777) ;
#7224=LINE('',#159918,#12778) ;
#7225=LINE('',#159920,#12779) ;
#7226=LINE('',#159922,#12780) ;
#7227=LINE('',#159924,#12781) ;
#7228=LINE('',#159928,#12782) ;
#7229=LINE('',#159930,#12783) ;
#7230=LINE('',#159931,#12784) ;
#7231=LINE('',#159935,#12785) ;
#7232=LINE('',#159937,#12786) ;
#7233=LINE('',#159939,#12787) ;
#7234=LINE('',#159940,#12788) ;
#7235=LINE('',#159944,#12789) ;
#7236=LINE('',#159950,#12790) ;
#7237=LINE('',#159952,#12791) ;
#7238=LINE('',#159954,#12792) ;
#7239=LINE('',#159958,#12793) ;
#7240=LINE('',#159960,#12794) ;
#7241=LINE('',#159961,#12795) ;
#7242=LINE('',#159965,#12796) ;
#7243=LINE('',#159967,#12797) ;
#7244=LINE('',#159969,#12798) ;
#7245=LINE('',#159970,#12799) ;
#7246=LINE('',#159974,#12800) ;
#7247=LINE('',#159976,#12801) ;
#7248=LINE('',#159978,#12802) ;
#7249=LINE('',#159979,#12803) ;
#7250=LINE('',#159983,#12804) ;
#7251=LINE('',#159985,#12805) ;
#7252=LINE('',#159987,#12806) ;
#7253=LINE('',#159988,#12807) ;
#7254=LINE('',#159992,#12808) ;
#7255=LINE('',#159996,#12809) ;
#7256=LINE('',#160001,#12810) ;
#7257=LINE('',#160005,#12811) ;
#7258=LINE('',#160007,#12812) ;
#7259=LINE('',#160009,#12813) ;
#7260=LINE('',#160010,#12814) ;
#7261=LINE('',#160014,#12815) ;
#7262=LINE('',#160016,#12816) ;
#7263=LINE('',#160018,#12817) ;
#7264=LINE('',#160019,#12818) ;
#7265=LINE('',#160023,#12819) ;
#7266=LINE('',#160025,#12820) ;
#7267=LINE('',#160027,#12821) ;
#7268=LINE('',#160028,#12822) ;
#7269=LINE('',#160032,#12823) ;
#7270=LINE('',#160036,#12824) ;
#7271=LINE('',#160041,#12825) ;
#7272=LINE('',#160045,#12826) ;
#7273=LINE('',#160047,#12827) ;
#7274=LINE('',#160049,#12828) ;
#7275=LINE('',#160050,#12829) ;
#7276=LINE('',#160054,#12830) ;
#7277=LINE('',#160056,#12831) ;
#7278=LINE('',#160058,#12832) ;
#7279=LINE('',#160059,#12833) ;
#7280=LINE('',#160063,#12834) ;
#7281=LINE('',#160065,#12835) ;
#7282=LINE('',#160067,#12836) ;
#7283=LINE('',#160068,#12837) ;
#7284=LINE('',#160072,#12838) ;
#7285=LINE('',#160076,#12839) ;
#7286=LINE('',#160081,#12840) ;
#7287=LINE('',#160085,#12841) ;
#7288=LINE('',#160087,#12842) ;
#7289=LINE('',#160089,#12843) ;
#7290=LINE('',#160090,#12844) ;
#7291=LINE('',#160094,#12845) ;
#7292=LINE('',#160096,#12846) ;
#7293=LINE('',#160098,#12847) ;
#7294=LINE('',#160099,#12848) ;
#7295=LINE('',#160103,#12849) ;
#7296=LINE('',#160105,#12850) ;
#7297=LINE('',#160107,#12851) ;
#7298=LINE('',#160108,#12852) ;
#7299=LINE('',#160112,#12853) ;
#7300=LINE('',#160116,#12854) ;
#7301=LINE('',#160121,#12855) ;
#7302=LINE('',#160125,#12856) ;
#7303=LINE('',#160127,#12857) ;
#7304=LINE('',#160129,#12858) ;
#7305=LINE('',#160130,#12859) ;
#7306=LINE('',#160134,#12860) ;
#7307=LINE('',#160136,#12861) ;
#7308=LINE('',#160138,#12862) ;
#7309=LINE('',#160139,#12863) ;
#7310=LINE('',#160143,#12864) ;
#7311=LINE('',#160145,#12865) ;
#7312=LINE('',#160147,#12866) ;
#7313=LINE('',#160148,#12867) ;
#7314=LINE('',#160152,#12868) ;
#7315=LINE('',#160156,#12869) ;
#7316=LINE('',#160161,#12870) ;
#7317=LINE('',#160165,#12871) ;
#7318=LINE('',#160167,#12872) ;
#7319=LINE('',#160169,#12873) ;
#7320=LINE('',#160170,#12874) ;
#7321=LINE('',#160174,#12875) ;
#7322=LINE('',#160176,#12876) ;
#7323=LINE('',#160178,#12877) ;
#7324=LINE('',#160179,#12878) ;
#7325=LINE('',#160183,#12879) ;
#7326=LINE('',#160185,#12880) ;
#7327=LINE('',#160187,#12881) ;
#7328=LINE('',#160188,#12882) ;
#7329=LINE('',#160192,#12883) ;
#7330=LINE('',#160196,#12884) ;
#7331=LINE('',#160201,#12885) ;
#7332=LINE('',#160205,#12886) ;
#7333=LINE('',#160207,#12887) ;
#7334=LINE('',#160209,#12888) ;
#7335=LINE('',#160210,#12889) ;
#7336=LINE('',#160214,#12890) ;
#7337=LINE('',#160216,#12891) ;
#7338=LINE('',#160218,#12892) ;
#7339=LINE('',#160219,#12893) ;
#7340=LINE('',#160223,#12894) ;
#7341=LINE('',#160225,#12895) ;
#7342=LINE('',#160227,#12896) ;
#7343=LINE('',#160228,#12897) ;
#7344=LINE('',#160232,#12898) ;
#7345=LINE('',#160236,#12899) ;
#7346=LINE('',#160241,#12900) ;
#7347=LINE('',#160245,#12901) ;
#7348=LINE('',#160247,#12902) ;
#7349=LINE('',#160249,#12903) ;
#7350=LINE('',#160250,#12904) ;
#7351=LINE('',#160254,#12905) ;
#7352=LINE('',#160256,#12906) ;
#7353=LINE('',#160258,#12907) ;
#7354=LINE('',#160259,#12908) ;
#7355=LINE('',#160263,#12909) ;
#7356=LINE('',#160265,#12910) ;
#7357=LINE('',#160267,#12911) ;
#7358=LINE('',#160268,#12912) ;
#7359=LINE('',#160272,#12913) ;
#7360=LINE('',#160276,#12914) ;
#7361=LINE('',#160281,#12915) ;
#7362=LINE('',#160285,#12916) ;
#7363=LINE('',#160287,#12917) ;
#7364=LINE('',#160289,#12918) ;
#7365=LINE('',#160290,#12919) ;
#7366=LINE('',#160294,#12920) ;
#7367=LINE('',#160296,#12921) ;
#7368=LINE('',#160298,#12922) ;
#7369=LINE('',#160299,#12923) ;
#7370=LINE('',#160303,#12924) ;
#7371=LINE('',#160305,#12925) ;
#7372=LINE('',#160307,#12926) ;
#7373=LINE('',#160308,#12927) ;
#7374=LINE('',#160312,#12928) ;
#7375=LINE('',#160316,#12929) ;
#7376=LINE('',#160321,#12930) ;
#7377=LINE('',#160325,#12931) ;
#7378=LINE('',#160327,#12932) ;
#7379=LINE('',#160329,#12933) ;
#7380=LINE('',#160330,#12934) ;
#7381=LINE('',#160343,#12935) ;
#7382=LINE('',#160345,#12936) ;
#7383=LINE('',#160347,#12937) ;
#7384=LINE('',#160348,#12938) ;
#7385=LINE('',#160352,#12939) ;
#7386=LINE('',#160354,#12940) ;
#7387=LINE('',#160356,#12941) ;
#7388=LINE('',#160357,#12942) ;
#7389=LINE('',#160361,#12943) ;
#7390=LINE('',#160363,#12944) ;
#7391=LINE('',#160365,#12945) ;
#7392=LINE('',#160366,#12946) ;
#7393=LINE('',#160370,#12947) ;
#7394=LINE('',#160372,#12948) ;
#7395=LINE('',#160374,#12949) ;
#7396=LINE('',#160375,#12950) ;
#7397=LINE('',#160379,#12951) ;
#7398=LINE('',#160381,#12952) ;
#7399=LINE('',#160383,#12953) ;
#7400=LINE('',#160384,#12954) ;
#7401=LINE('',#160388,#12955) ;
#7402=LINE('',#160390,#12956) ;
#7403=LINE('',#160392,#12957) ;
#7404=LINE('',#160393,#12958) ;
#7405=LINE('',#160397,#12959) ;
#7406=LINE('',#160399,#12960) ;
#7407=LINE('',#160401,#12961) ;
#7408=LINE('',#160402,#12962) ;
#7409=LINE('',#160406,#12963) ;
#7410=LINE('',#160408,#12964) ;
#7411=LINE('',#160410,#12965) ;
#7412=LINE('',#160411,#12966) ;
#7413=LINE('',#160415,#12967) ;
#7414=LINE('',#160417,#12968) ;
#7415=LINE('',#160419,#12969) ;
#7416=LINE('',#160420,#12970) ;
#7417=LINE('',#160424,#12971) ;
#7418=LINE('',#160426,#12972) ;
#7419=LINE('',#160428,#12973) ;
#7420=LINE('',#160429,#12974) ;
#7421=LINE('',#160433,#12975) ;
#7422=LINE('',#160435,#12976) ;
#7423=LINE('',#160437,#12977) ;
#7424=LINE('',#160438,#12978) ;
#7425=LINE('',#160442,#12979) ;
#7426=LINE('',#160444,#12980) ;
#7427=LINE('',#160446,#12981) ;
#7428=LINE('',#160447,#12982) ;
#7429=LINE('',#160451,#12983) ;
#7430=LINE('',#160453,#12984) ;
#7431=LINE('',#160455,#12985) ;
#7432=LINE('',#160456,#12986) ;
#7433=LINE('',#160460,#12987) ;
#7434=LINE('',#160462,#12988) ;
#7435=LINE('',#160464,#12989) ;
#7436=LINE('',#160465,#12990) ;
#7437=LINE('',#160469,#12991) ;
#7438=LINE('',#160471,#12992) ;
#7439=LINE('',#160473,#12993) ;
#7440=LINE('',#160474,#12994) ;
#7441=LINE('',#160478,#12995) ;
#7442=LINE('',#160480,#12996) ;
#7443=LINE('',#160482,#12997) ;
#7444=LINE('',#160483,#12998) ;
#7445=LINE('',#160487,#12999) ;
#7446=LINE('',#160489,#13000) ;
#7447=LINE('',#160491,#13001) ;
#7448=LINE('',#160492,#13002) ;
#7449=LINE('',#160496,#13003) ;
#7450=LINE('',#160498,#13004) ;
#7451=LINE('',#160500,#13005) ;
#7452=LINE('',#160501,#13006) ;
#7453=LINE('',#160505,#13007) ;
#7454=LINE('',#160507,#13008) ;
#7455=LINE('',#160509,#13009) ;
#7456=LINE('',#160510,#13010) ;
#7457=LINE('',#160514,#13011) ;
#7458=LINE('',#160516,#13012) ;
#7459=LINE('',#160518,#13013) ;
#7460=LINE('',#160519,#13014) ;
#7461=LINE('',#160523,#13015) ;
#7462=LINE('',#160525,#13016) ;
#7463=LINE('',#160527,#13017) ;
#7464=LINE('',#160528,#13018) ;
#7465=LINE('',#160532,#13019) ;
#7466=LINE('',#160534,#13020) ;
#7467=LINE('',#160536,#13021) ;
#7468=LINE('',#160537,#13022) ;
#7469=LINE('',#160541,#13023) ;
#7470=LINE('',#160543,#13024) ;
#7471=LINE('',#160545,#13025) ;
#7472=LINE('',#160546,#13026) ;
#7473=LINE('',#160550,#13027) ;
#7474=LINE('',#160552,#13028) ;
#7475=LINE('',#160554,#13029) ;
#7476=LINE('',#160555,#13030) ;
#7477=LINE('',#160559,#13031) ;
#7478=LINE('',#160561,#13032) ;
#7479=LINE('',#160563,#13033) ;
#7480=LINE('',#160564,#13034) ;
#7481=LINE('',#160568,#13035) ;
#7482=LINE('',#160570,#13036) ;
#7483=LINE('',#160572,#13037) ;
#7484=LINE('',#160573,#13038) ;
#7485=LINE('',#160577,#13039) ;
#7486=LINE('',#160579,#13040) ;
#7487=LINE('',#160581,#13041) ;
#7488=LINE('',#160582,#13042) ;
#7489=LINE('',#160586,#13043) ;
#7490=LINE('',#160588,#13044) ;
#7491=LINE('',#160590,#13045) ;
#7492=LINE('',#160591,#13046) ;
#7493=LINE('',#160595,#13047) ;
#7494=LINE('',#160597,#13048) ;
#7495=LINE('',#160599,#13049) ;
#7496=LINE('',#160600,#13050) ;
#7497=LINE('',#160604,#13051) ;
#7498=LINE('',#160606,#13052) ;
#7499=LINE('',#160608,#13053) ;
#7500=LINE('',#160609,#13054) ;
#7501=LINE('',#160613,#13055) ;
#7502=LINE('',#160615,#13056) ;
#7503=LINE('',#160617,#13057) ;
#7504=LINE('',#160618,#13058) ;
#7505=LINE('',#160622,#13059) ;
#7506=LINE('',#160624,#13060) ;
#7507=LINE('',#160626,#13061) ;
#7508=LINE('',#160627,#13062) ;
#7509=LINE('',#160631,#13063) ;
#7510=LINE('',#160633,#13064) ;
#7511=LINE('',#160635,#13065) ;
#7512=LINE('',#160636,#13066) ;
#7513=LINE('',#160640,#13067) ;
#7514=LINE('',#160642,#13068) ;
#7515=LINE('',#160644,#13069) ;
#7516=LINE('',#160645,#13070) ;
#7517=LINE('',#160649,#13071) ;
#7518=LINE('',#160651,#13072) ;
#7519=LINE('',#160653,#13073) ;
#7520=LINE('',#160654,#13074) ;
#7521=LINE('',#160658,#13075) ;
#7522=LINE('',#160660,#13076) ;
#7523=LINE('',#160662,#13077) ;
#7524=LINE('',#160663,#13078) ;
#7525=LINE('',#160667,#13079) ;
#7526=LINE('',#160669,#13080) ;
#7527=LINE('',#160671,#13081) ;
#7528=LINE('',#160672,#13082) ;
#7529=LINE('',#160675,#13083) ;
#7530=LINE('',#160679,#13084) ;
#7531=LINE('',#160683,#13085) ;
#7532=LINE('',#160687,#13086) ;
#7533=LINE('',#160692,#13087) ;
#7534=LINE('',#160693,#13088) ;
#7535=LINE('',#160694,#13089) ;
#7536=LINE('',#160698,#13090) ;
#7537=LINE('',#160699,#13091) ;
#7538=LINE('',#160700,#13092) ;
#7539=LINE('',#160703,#13093) ;
#7540=LINE('',#160705,#13094) ;
#7541=LINE('',#160706,#13095) ;
#7542=LINE('',#160710,#13096) ;
#7543=LINE('',#160711,#13097) ;
#7544=LINE('',#160712,#13098) ;
#7545=LINE('',#160716,#13099) ;
#7546=LINE('',#160718,#13100) ;
#7547=LINE('',#160720,#13101) ;
#7548=LINE('',#160721,#13102) ;
#7549=LINE('',#160724,#13103) ;
#7550=LINE('',#160728,#13104) ;
#7551=LINE('',#160732,#13105) ;
#7552=LINE('',#160736,#13106) ;
#7553=LINE('',#160741,#13107) ;
#7554=LINE('',#160742,#13108) ;
#7555=LINE('',#160743,#13109) ;
#7556=LINE('',#160747,#13110) ;
#7557=LINE('',#160748,#13111) ;
#7558=LINE('',#160749,#13112) ;
#7559=LINE('',#160752,#13113) ;
#7560=LINE('',#160754,#13114) ;
#7561=LINE('',#160755,#13115) ;
#7562=LINE('',#160759,#13116) ;
#7563=LINE('',#160760,#13117) ;
#7564=LINE('',#160761,#13118) ;
#7565=LINE('',#160765,#13119) ;
#7566=LINE('',#160767,#13120) ;
#7567=LINE('',#160769,#13121) ;
#7568=LINE('',#160770,#13122) ;
#7569=LINE('',#160773,#13123) ;
#7570=LINE('',#160777,#13124) ;
#7571=LINE('',#160781,#13125) ;
#7572=LINE('',#160785,#13126) ;
#7573=LINE('',#160790,#13127) ;
#7574=LINE('',#160791,#13128) ;
#7575=LINE('',#160792,#13129) ;
#7576=LINE('',#160796,#13130) ;
#7577=LINE('',#160797,#13131) ;
#7578=LINE('',#160798,#13132) ;
#7579=LINE('',#160801,#13133) ;
#7580=LINE('',#160803,#13134) ;
#7581=LINE('',#160804,#13135) ;
#7582=LINE('',#160808,#13136) ;
#7583=LINE('',#160809,#13137) ;
#7584=LINE('',#160810,#13138) ;
#7585=LINE('',#160814,#13139) ;
#7586=LINE('',#160816,#13140) ;
#7587=LINE('',#160818,#13141) ;
#7588=LINE('',#160819,#13142) ;
#7589=LINE('',#160822,#13143) ;
#7590=LINE('',#160826,#13144) ;
#7591=LINE('',#160830,#13145) ;
#7592=LINE('',#160834,#13146) ;
#7593=LINE('',#160839,#13147) ;
#7594=LINE('',#160840,#13148) ;
#7595=LINE('',#160841,#13149) ;
#7596=LINE('',#160845,#13150) ;
#7597=LINE('',#160846,#13151) ;
#7598=LINE('',#160847,#13152) ;
#7599=LINE('',#160850,#13153) ;
#7600=LINE('',#160852,#13154) ;
#7601=LINE('',#160853,#13155) ;
#7602=LINE('',#160857,#13156) ;
#7603=LINE('',#160858,#13157) ;
#7604=LINE('',#160859,#13158) ;
#7605=LINE('',#160863,#13159) ;
#7606=LINE('',#160865,#13160) ;
#7607=LINE('',#160867,#13161) ;
#7608=LINE('',#160868,#13162) ;
#7609=LINE('',#160871,#13163) ;
#7610=LINE('',#160875,#13164) ;
#7611=LINE('',#160879,#13165) ;
#7612=LINE('',#160883,#13166) ;
#7613=LINE('',#160888,#13167) ;
#7614=LINE('',#160889,#13168) ;
#7615=LINE('',#160890,#13169) ;
#7616=LINE('',#160894,#13170) ;
#7617=LINE('',#160895,#13171) ;
#7618=LINE('',#160896,#13172) ;
#7619=LINE('',#160899,#13173) ;
#7620=LINE('',#160901,#13174) ;
#7621=LINE('',#160902,#13175) ;
#7622=LINE('',#160906,#13176) ;
#7623=LINE('',#160907,#13177) ;
#7624=LINE('',#160908,#13178) ;
#7625=LINE('',#160912,#13179) ;
#7626=LINE('',#160914,#13180) ;
#7627=LINE('',#160916,#13181) ;
#7628=LINE('',#160917,#13182) ;
#7629=LINE('',#160920,#13183) ;
#7630=LINE('',#160924,#13184) ;
#7631=LINE('',#160928,#13185) ;
#7632=LINE('',#160932,#13186) ;
#7633=LINE('',#160937,#13187) ;
#7634=LINE('',#160938,#13188) ;
#7635=LINE('',#160939,#13189) ;
#7636=LINE('',#160943,#13190) ;
#7637=LINE('',#160944,#13191) ;
#7638=LINE('',#160945,#13192) ;
#7639=LINE('',#160948,#13193) ;
#7640=LINE('',#160950,#13194) ;
#7641=LINE('',#160951,#13195) ;
#7642=LINE('',#160955,#13196) ;
#7643=LINE('',#160956,#13197) ;
#7644=LINE('',#160957,#13198) ;
#7645=LINE('',#160961,#13199) ;
#7646=LINE('',#160963,#13200) ;
#7647=LINE('',#160965,#13201) ;
#7648=LINE('',#160966,#13202) ;
#7649=LINE('',#160969,#13203) ;
#7650=LINE('',#160973,#13204) ;
#7651=LINE('',#160977,#13205) ;
#7652=LINE('',#160981,#13206) ;
#7653=LINE('',#160986,#13207) ;
#7654=LINE('',#160987,#13208) ;
#7655=LINE('',#160988,#13209) ;
#7656=LINE('',#160992,#13210) ;
#7657=LINE('',#160993,#13211) ;
#7658=LINE('',#160994,#13212) ;
#7659=LINE('',#160997,#13213) ;
#7660=LINE('',#160999,#13214) ;
#7661=LINE('',#161000,#13215) ;
#7662=LINE('',#161004,#13216) ;
#7663=LINE('',#161005,#13217) ;
#7664=LINE('',#161006,#13218) ;
#7665=LINE('',#161010,#13219) ;
#7666=LINE('',#161012,#13220) ;
#7667=LINE('',#161014,#13221) ;
#7668=LINE('',#161015,#13222) ;
#7669=LINE('',#161018,#13223) ;
#7670=LINE('',#161022,#13224) ;
#7671=LINE('',#161026,#13225) ;
#7672=LINE('',#161030,#13226) ;
#7673=LINE('',#161035,#13227) ;
#7674=LINE('',#161036,#13228) ;
#7675=LINE('',#161037,#13229) ;
#7676=LINE('',#161041,#13230) ;
#7677=LINE('',#161042,#13231) ;
#7678=LINE('',#161043,#13232) ;
#7679=LINE('',#161046,#13233) ;
#7680=LINE('',#161048,#13234) ;
#7681=LINE('',#161049,#13235) ;
#7682=LINE('',#161053,#13236) ;
#7683=LINE('',#161054,#13237) ;
#7684=LINE('',#161055,#13238) ;
#7685=LINE('',#161059,#13239) ;
#7686=LINE('',#161061,#13240) ;
#7687=LINE('',#161063,#13241) ;
#7688=LINE('',#161064,#13242) ;
#7689=LINE('',#161067,#13243) ;
#7690=LINE('',#161071,#13244) ;
#7691=LINE('',#161075,#13245) ;
#7692=LINE('',#161079,#13246) ;
#7693=LINE('',#161084,#13247) ;
#7694=LINE('',#161085,#13248) ;
#7695=LINE('',#161086,#13249) ;
#7696=LINE('',#161090,#13250) ;
#7697=LINE('',#161091,#13251) ;
#7698=LINE('',#161092,#13252) ;
#7699=LINE('',#161095,#13253) ;
#7700=LINE('',#161097,#13254) ;
#7701=LINE('',#161098,#13255) ;
#7702=LINE('',#161102,#13256) ;
#7703=LINE('',#161103,#13257) ;
#7704=LINE('',#161104,#13258) ;
#7705=LINE('',#161108,#13259) ;
#7706=LINE('',#161110,#13260) ;
#7707=LINE('',#161112,#13261) ;
#7708=LINE('',#161113,#13262) ;
#7709=LINE('',#161117,#13263) ;
#7710=LINE('',#161119,#13264) ;
#7711=LINE('',#161121,#13265) ;
#7712=LINE('',#161122,#13266) ;
#7713=LINE('',#161126,#13267) ;
#7714=LINE('',#161128,#13268) ;
#7715=LINE('',#161130,#13269) ;
#7716=LINE('',#161131,#13270) ;
#7717=LINE('',#161135,#13271) ;
#7718=LINE('',#161137,#13272) ;
#7719=LINE('',#161139,#13273) ;
#7720=LINE('',#161140,#13274) ;
#7721=LINE('',#161144,#13275) ;
#7722=LINE('',#161146,#13276) ;
#7723=LINE('',#161148,#13277) ;
#7724=LINE('',#161149,#13278) ;
#7725=LINE('',#161153,#13279) ;
#7726=LINE('',#161155,#13280) ;
#7727=LINE('',#161157,#13281) ;
#7728=LINE('',#161158,#13282) ;
#7729=LINE('',#161162,#13283) ;
#7730=LINE('',#161164,#13284) ;
#7731=LINE('',#161166,#13285) ;
#7732=LINE('',#161167,#13286) ;
#7733=LINE('',#161171,#13287) ;
#7734=LINE('',#161173,#13288) ;
#7735=LINE('',#161175,#13289) ;
#7736=LINE('',#161176,#13290) ;
#7737=LINE('',#161180,#13291) ;
#7738=LINE('',#161182,#13292) ;
#7739=LINE('',#161184,#13293) ;
#7740=LINE('',#161185,#13294) ;
#7741=LINE('',#161187,#13295) ;
#7742=LINE('',#161189,#13296) ;
#7743=LINE('',#161191,#13297) ;
#7744=LINE('',#161193,#13298) ;
#7745=LINE('',#161195,#13299) ;
#7746=LINE('',#161197,#13300) ;
#7747=LINE('',#161199,#13301) ;
#7748=LINE('',#161201,#13302) ;
#7749=LINE('',#161203,#13303) ;
#7750=LINE('',#161205,#13304) ;
#7751=LINE('',#161206,#13305) ;
#7752=LINE('',#161208,#13306) ;
#7753=LINE('',#161209,#13307) ;
#7754=LINE('',#161211,#13308) ;
#7755=LINE('',#161212,#13309) ;
#7756=LINE('',#161214,#13310) ;
#7757=LINE('',#161215,#13311) ;
#7758=LINE('',#161217,#13312) ;
#7759=LINE('',#161218,#13313) ;
#7760=LINE('',#161220,#13314) ;
#7761=LINE('',#161221,#13315) ;
#7762=LINE('',#161223,#13316) ;
#7763=LINE('',#161224,#13317) ;
#7764=LINE('',#161226,#13318) ;
#7765=LINE('',#161227,#13319) ;
#7766=LINE('',#161229,#13320) ;
#7767=LINE('',#161230,#13321) ;
#7768=LINE('',#161232,#13322) ;
#7769=LINE('',#161233,#13323) ;
#7770=LINE('',#161235,#13324) ;
#7771=LINE('',#161236,#13325) ;
#7772=LINE('',#161238,#13326) ;
#7773=LINE('',#161239,#13327) ;
#7774=LINE('',#161241,#13328) ;
#7775=LINE('',#161242,#13329) ;
#7776=LINE('',#161244,#13330) ;
#7777=LINE('',#161245,#13331) ;
#7778=LINE('',#161247,#13332) ;
#7779=LINE('',#161248,#13333) ;
#7780=LINE('',#161250,#13334) ;
#7781=LINE('',#161251,#13335) ;
#7782=LINE('',#161253,#13336) ;
#7783=LINE('',#161254,#13337) ;
#7784=LINE('',#161256,#13338) ;
#7785=LINE('',#161257,#13339) ;
#7786=LINE('',#161259,#13340) ;
#7787=LINE('',#161260,#13341) ;
#7788=LINE('',#161262,#13342) ;
#7789=LINE('',#161263,#13343) ;
#7790=LINE('',#161265,#13344) ;
#7791=LINE('',#161266,#13345) ;
#7792=LINE('',#161268,#13346) ;
#7793=LINE('',#161269,#13347) ;
#7794=LINE('',#161271,#13348) ;
#7795=LINE('',#161272,#13349) ;
#7796=LINE('',#161274,#13350) ;
#7797=LINE('',#161275,#13351) ;
#7798=LINE('',#161277,#13352) ;
#7799=LINE('',#161278,#13353) ;
#7800=LINE('',#161280,#13354) ;
#7801=LINE('',#161281,#13355) ;
#7802=LINE('',#161283,#13356) ;
#7803=LINE('',#161284,#13357) ;
#7804=LINE('',#161288,#13358) ;
#7805=LINE('',#161292,#13359) ;
#7806=LINE('',#161296,#13360) ;
#7807=LINE('',#161298,#13361) ;
#7808=LINE('',#161299,#13362) ;
#7809=LINE('',#161304,#13363) ;
#7810=LINE('',#161308,#13364) ;
#7811=LINE('',#161310,#13365) ;
#7812=LINE('',#161311,#13366) ;
#7813=LINE('',#161316,#13367) ;
#7814=LINE('',#161320,#13368) ;
#7815=LINE('',#161322,#13369) ;
#7816=LINE('',#161323,#13370) ;
#7817=LINE('',#161328,#13371) ;
#7818=LINE('',#161331,#13372) ;
#7819=LINE('',#161332,#13373) ;
#7820=LINE('',#161336,#13374) ;
#7821=LINE('',#161338,#13375) ;
#7822=LINE('',#161340,#13376) ;
#7823=LINE('',#161341,#13377) ;
#7824=LINE('',#161345,#13378) ;
#7825=LINE('',#161349,#13379) ;
#7826=LINE('',#161353,#13380) ;
#7827=LINE('',#161355,#13381) ;
#7828=LINE('',#161356,#13382) ;
#7829=LINE('',#161361,#13383) ;
#7830=LINE('',#161365,#13384) ;
#7831=LINE('',#161367,#13385) ;
#7832=LINE('',#161368,#13386) ;
#7833=LINE('',#161373,#13387) ;
#7834=LINE('',#161377,#13388) ;
#7835=LINE('',#161379,#13389) ;
#7836=LINE('',#161380,#13390) ;
#7837=LINE('',#161385,#13391) ;
#7838=LINE('',#161388,#13392) ;
#7839=LINE('',#161389,#13393) ;
#7840=LINE('',#161393,#13394) ;
#7841=LINE('',#161395,#13395) ;
#7842=LINE('',#161397,#13396) ;
#7843=LINE('',#161398,#13397) ;
#7844=LINE('',#161402,#13398) ;
#7845=LINE('',#161406,#13399) ;
#7846=LINE('',#161410,#13400) ;
#7847=LINE('',#161412,#13401) ;
#7848=LINE('',#161413,#13402) ;
#7849=LINE('',#161418,#13403) ;
#7850=LINE('',#161422,#13404) ;
#7851=LINE('',#161424,#13405) ;
#7852=LINE('',#161425,#13406) ;
#7853=LINE('',#161430,#13407) ;
#7854=LINE('',#161434,#13408) ;
#7855=LINE('',#161436,#13409) ;
#7856=LINE('',#161437,#13410) ;
#7857=LINE('',#161442,#13411) ;
#7858=LINE('',#161445,#13412) ;
#7859=LINE('',#161446,#13413) ;
#7860=LINE('',#161450,#13414) ;
#7861=LINE('',#161452,#13415) ;
#7862=LINE('',#161454,#13416) ;
#7863=LINE('',#161455,#13417) ;
#7864=LINE('',#161459,#13418) ;
#7865=LINE('',#161463,#13419) ;
#7866=LINE('',#161467,#13420) ;
#7867=LINE('',#161469,#13421) ;
#7868=LINE('',#161470,#13422) ;
#7869=LINE('',#161475,#13423) ;
#7870=LINE('',#161479,#13424) ;
#7871=LINE('',#161481,#13425) ;
#7872=LINE('',#161482,#13426) ;
#7873=LINE('',#161487,#13427) ;
#7874=LINE('',#161491,#13428) ;
#7875=LINE('',#161493,#13429) ;
#7876=LINE('',#161494,#13430) ;
#7877=LINE('',#161499,#13431) ;
#7878=LINE('',#161502,#13432) ;
#7879=LINE('',#161503,#13433) ;
#7880=LINE('',#161507,#13434) ;
#7881=LINE('',#161509,#13435) ;
#7882=LINE('',#161511,#13436) ;
#7883=LINE('',#161512,#13437) ;
#7884=LINE('',#161516,#13438) ;
#7885=LINE('',#161520,#13439) ;
#7886=LINE('',#161524,#13440) ;
#7887=LINE('',#161526,#13441) ;
#7888=LINE('',#161527,#13442) ;
#7889=LINE('',#161532,#13443) ;
#7890=LINE('',#161536,#13444) ;
#7891=LINE('',#161538,#13445) ;
#7892=LINE('',#161539,#13446) ;
#7893=LINE('',#161544,#13447) ;
#7894=LINE('',#161548,#13448) ;
#7895=LINE('',#161550,#13449) ;
#7896=LINE('',#161551,#13450) ;
#7897=LINE('',#161556,#13451) ;
#7898=LINE('',#161559,#13452) ;
#7899=LINE('',#161560,#13453) ;
#7900=LINE('',#161564,#13454) ;
#7901=LINE('',#161566,#13455) ;
#7902=LINE('',#161568,#13456) ;
#7903=LINE('',#161569,#13457) ;
#7904=LINE('',#161573,#13458) ;
#7905=LINE('',#161577,#13459) ;
#7906=LINE('',#161581,#13460) ;
#7907=LINE('',#161583,#13461) ;
#7908=LINE('',#161584,#13462) ;
#7909=LINE('',#161589,#13463) ;
#7910=LINE('',#161593,#13464) ;
#7911=LINE('',#161595,#13465) ;
#7912=LINE('',#161596,#13466) ;
#7913=LINE('',#161601,#13467) ;
#7914=LINE('',#161605,#13468) ;
#7915=LINE('',#161607,#13469) ;
#7916=LINE('',#161608,#13470) ;
#7917=LINE('',#161613,#13471) ;
#7918=LINE('',#161616,#13472) ;
#7919=LINE('',#161617,#13473) ;
#7920=LINE('',#161621,#13474) ;
#7921=LINE('',#161623,#13475) ;
#7922=LINE('',#161625,#13476) ;
#7923=LINE('',#161626,#13477) ;
#7924=LINE('',#161630,#13478) ;
#7925=LINE('',#161634,#13479) ;
#7926=LINE('',#161638,#13480) ;
#7927=LINE('',#161640,#13481) ;
#7928=LINE('',#161641,#13482) ;
#7929=LINE('',#161646,#13483) ;
#7930=LINE('',#161650,#13484) ;
#7931=LINE('',#161652,#13485) ;
#7932=LINE('',#161653,#13486) ;
#7933=LINE('',#161658,#13487) ;
#7934=LINE('',#161662,#13488) ;
#7935=LINE('',#161664,#13489) ;
#7936=LINE('',#161665,#13490) ;
#7937=LINE('',#161670,#13491) ;
#7938=LINE('',#161673,#13492) ;
#7939=LINE('',#161674,#13493) ;
#7940=LINE('',#161678,#13494) ;
#7941=LINE('',#161680,#13495) ;
#7942=LINE('',#161682,#13496) ;
#7943=LINE('',#161683,#13497) ;
#7944=LINE('',#161687,#13498) ;
#7945=LINE('',#161691,#13499) ;
#7946=LINE('',#161695,#13500) ;
#7947=LINE('',#161697,#13501) ;
#7948=LINE('',#161698,#13502) ;
#7949=LINE('',#161703,#13503) ;
#7950=LINE('',#161707,#13504) ;
#7951=LINE('',#161709,#13505) ;
#7952=LINE('',#161710,#13506) ;
#7953=LINE('',#161715,#13507) ;
#7954=LINE('',#161719,#13508) ;
#7955=LINE('',#161721,#13509) ;
#7956=LINE('',#161722,#13510) ;
#7957=LINE('',#161727,#13511) ;
#7958=LINE('',#161730,#13512) ;
#7959=LINE('',#161731,#13513) ;
#7960=LINE('',#161735,#13514) ;
#7961=LINE('',#161737,#13515) ;
#7962=LINE('',#161739,#13516) ;
#7963=LINE('',#161740,#13517) ;
#7964=LINE('',#161744,#13518) ;
#7965=LINE('',#161748,#13519) ;
#7966=LINE('',#161752,#13520) ;
#7967=LINE('',#161754,#13521) ;
#7968=LINE('',#161755,#13522) ;
#7969=LINE('',#161760,#13523) ;
#7970=LINE('',#161764,#13524) ;
#7971=LINE('',#161766,#13525) ;
#7972=LINE('',#161767,#13526) ;
#7973=LINE('',#161772,#13527) ;
#7974=LINE('',#161776,#13528) ;
#7975=LINE('',#161778,#13529) ;
#7976=LINE('',#161779,#13530) ;
#7977=LINE('',#161784,#13531) ;
#7978=LINE('',#161787,#13532) ;
#7979=LINE('',#161788,#13533) ;
#7980=LINE('',#161792,#13534) ;
#7981=LINE('',#161794,#13535) ;
#7982=LINE('',#161796,#13536) ;
#7983=LINE('',#161797,#13537) ;
#11321=VECTOR('',#120481,1000.) ;
#11322=VECTOR('',#120484,1000.) ;
#11323=VECTOR('',#120659,1000.) ;
#11324=VECTOR('',#120660,1000.) ;
#11325=VECTOR('',#120665,1000.) ;
#11326=VECTOR('',#120666,1000.) ;
#11327=VECTOR('',#120671,1000.) ;
#11328=VECTOR('',#120672,1000.) ;
#11329=VECTOR('',#120677,1000.) ;
#11330=VECTOR('',#120678,1000.) ;
#11331=VECTOR('',#120683,1000.) ;
#11332=VECTOR('',#120684,1000.) ;
#11333=VECTOR('',#120689,1000.) ;
#11334=VECTOR('',#120690,1000.) ;
#11335=VECTOR('',#120695,1000.) ;
#11336=VECTOR('',#120696,1000.) ;
#11337=VECTOR('',#120917,1000.) ;
#11338=VECTOR('',#120920,1000.) ;
#11339=VECTOR('',#120923,1000.) ;
#11340=VECTOR('',#120926,1000.) ;
#11341=VECTOR('',#120929,1.5) ;
#11342=VECTOR('',#120934,1000.) ;
#11343=VECTOR('',#120937,1000.) ;
#11344=VECTOR('',#120940,1000.) ;
#11345=VECTOR('',#120943,1000.) ;
#11346=VECTOR('',#120946,1.5) ;
#11347=VECTOR('',#120951,1000.) ;
#11348=VECTOR('',#120954,1000.) ;
#11349=VECTOR('',#120957,1000.) ;
#11350=VECTOR('',#120960,1000.) ;
#11351=VECTOR('',#120963,1.5) ;
#11352=VECTOR('',#120968,1000.) ;
#11353=VECTOR('',#120971,1000.) ;
#11354=VECTOR('',#120974,1000.) ;
#11355=VECTOR('',#120977,1000.) ;
#11356=VECTOR('',#120980,1.5) ;
#11357=VECTOR('',#120985,1000.) ;
#11358=VECTOR('',#120988,1000.) ;
#11359=VECTOR('',#120991,1000.) ;
#11360=VECTOR('',#120994,1000.) ;
#11361=VECTOR('',#120997,1.5) ;
#11362=VECTOR('',#121002,1000.) ;
#11363=VECTOR('',#121005,1000.) ;
#11364=VECTOR('',#121008,1000.) ;
#11365=VECTOR('',#121011,1000.) ;
#11366=VECTOR('',#121014,1.5) ;
#11367=VECTOR('',#121019,1000.) ;
#11368=VECTOR('',#121022,1000.) ;
#11369=VECTOR('',#121025,1000.) ;
#11370=VECTOR('',#121028,1000.) ;
#11371=VECTOR('',#121031,1.5) ;
#11372=VECTOR('',#121036,1000.) ;
#11373=VECTOR('',#121039,1000.) ;
#11374=VECTOR('',#121042,1000.) ;
#11375=VECTOR('',#121045,1000.) ;
#11376=VECTOR('',#121048,1.5) ;
#11377=VECTOR('',#121053,1000.) ;
#11378=VECTOR('',#121056,1000.) ;
#11379=VECTOR('',#121059,1000.) ;
#11380=VECTOR('',#121062,1000.) ;
#11381=VECTOR('',#121065,1.5) ;
#11382=VECTOR('',#121070,1.) ;
#11383=VECTOR('',#121075,1.) ;
#11384=VECTOR('',#121080,1.) ;
#11385=VECTOR('',#121085,1.) ;
#11386=VECTOR('',#121090,1.) ;
#11387=VECTOR('',#121095,1.) ;
#11388=VECTOR('',#121100,1.) ;
#11389=VECTOR('',#121105,0.999999999999999) ;
#11390=VECTOR('',#121110,1.) ;
#11391=VECTOR('',#121113,1.) ;
#11392=VECTOR('',#121116,0.999999999999999) ;
#11393=VECTOR('',#121119,1.) ;
#11394=VECTOR('',#121122,1.) ;
#11395=VECTOR('',#121125,1.) ;
#11396=VECTOR('',#121128,1.) ;
#11397=VECTOR('',#121131,1.) ;
#11398=VECTOR('',#121134,1.) ;
#11399=VECTOR('',#121137,1.) ;
#11400=VECTOR('',#121166,1000.) ;
#11401=VECTOR('',#121167,1000.) ;
#11402=VECTOR('',#121172,1000.) ;
#11403=VECTOR('',#121173,1000.) ;
#11404=VECTOR('',#121178,1000.) ;
#11405=VECTOR('',#121179,1000.) ;
#11406=VECTOR('',#121184,1000.) ;
#11407=VECTOR('',#121185,1000.) ;
#11408=VECTOR('',#121190,1000.) ;
#11409=VECTOR('',#121193,1000.) ;
#11410=VECTOR('',#121196,1000.) ;
#11411=VECTOR('',#121199,1000.) ;
#11412=VECTOR('',#121202,1.5) ;
#11413=VECTOR('',#121207,1.) ;
#11414=VECTOR('',#121210,1.) ;
#11415=VECTOR('',#121213,1000.) ;
#11416=VECTOR('',#121214,1000.) ;
#11417=VECTOR('',#121215,1000.) ;
#11418=VECTOR('',#121216,1000.) ;
#11419=VECTOR('',#121237,1000.) ;
#11420=VECTOR('',#121238,1000.) ;
#11421=VECTOR('',#121239,1000.) ;
#11422=VECTOR('',#121242,1000.) ;
#11423=VECTOR('',#121245,1000.) ;
#11424=VECTOR('',#121248,1000.) ;
#11425=VECTOR('',#121251,1000.) ;
#11426=VECTOR('',#121254,1000.) ;
#11427=VECTOR('',#121257,1000.) ;
#11428=VECTOR('',#121260,1000.) ;
#11429=VECTOR('',#121263,1000.) ;
#11430=VECTOR('',#121266,1000.) ;
#11431=VECTOR('',#121269,1000.) ;
#11432=VECTOR('',#121272,1000.) ;
#11433=VECTOR('',#121275,1000.) ;
#11434=VECTOR('',#121278,1000.) ;
#11435=VECTOR('',#121281,1000.) ;
#11436=VECTOR('',#121284,1000.) ;
#11437=VECTOR('',#121287,1000.) ;
#11438=VECTOR('',#121290,1000.) ;
#11439=VECTOR('',#121293,1000.) ;
#11440=VECTOR('',#121296,1000.) ;
#11441=VECTOR('',#121299,1000.) ;
#11442=VECTOR('',#121302,1000.) ;
#11443=VECTOR('',#121305,1000.) ;
#11444=VECTOR('',#121308,1000.) ;
#11445=VECTOR('',#121311,1000.) ;
#11446=VECTOR('',#121314,1000.) ;
#11447=VECTOR('',#121317,1000.) ;
#11448=VECTOR('',#121320,1000.) ;
#11449=VECTOR('',#121323,1000.) ;
#11450=VECTOR('',#121326,1000.) ;
#11451=VECTOR('',#121329,1000.) ;
#11452=VECTOR('',#121332,1000.) ;
#11453=VECTOR('',#121335,1000.) ;
#11454=VECTOR('',#121338,1000.) ;
#11455=VECTOR('',#121341,1000.) ;
#11456=VECTOR('',#121344,1000.) ;
#11457=VECTOR('',#121347,1000.) ;
#11458=VECTOR('',#121350,1000.) ;
#11459=VECTOR('',#121353,1000.) ;
#11460=VECTOR('',#121356,1000.) ;
#11461=VECTOR('',#121359,1000.) ;
#11462=VECTOR('',#121362,1000.) ;
#11463=VECTOR('',#121363,1000.) ;
#11464=VECTOR('',#121364,1000.) ;
#11465=VECTOR('',#121365,1000.) ;
#11466=VECTOR('',#121366,1000.) ;
#11467=VECTOR('',#121369,1000.) ;
#11468=VECTOR('',#121372,1000.) ;
#11469=VECTOR('',#121375,1000.) ;
#11470=VECTOR('',#121380,1000.) ;
#11471=VECTOR('',#121381,1000.) ;
#11472=VECTOR('',#121382,1000.) ;
#11473=VECTOR('',#121383,1000.) ;
#11474=VECTOR('',#121384,1000.) ;
#11475=VECTOR('',#121387,1000.) ;
#11476=VECTOR('',#121390,1000.) ;
#11477=VECTOR('',#121393,1000.) ;
#11478=VECTOR('',#121398,1000.) ;
#11479=VECTOR('',#121399,1000.) ;
#11480=VECTOR('',#121400,1000.) ;
#11481=VECTOR('',#121401,1000.) ;
#11482=VECTOR('',#121402,1000.) ;
#11483=VECTOR('',#121405,1000.) ;
#11484=VECTOR('',#121408,1000.) ;
#11485=VECTOR('',#121411,1000.) ;
#11486=VECTOR('',#121416,1000.) ;
#11487=VECTOR('',#121417,1000.) ;
#11488=VECTOR('',#121418,1000.) ;
#11489=VECTOR('',#121419,1000.) ;
#11490=VECTOR('',#121420,1000.) ;
#11491=VECTOR('',#121423,1000.) ;
#11492=VECTOR('',#121426,1000.) ;
#11493=VECTOR('',#121429,1000.) ;
#11494=VECTOR('',#121434,1000.) ;
#11495=VECTOR('',#121435,1000.) ;
#11496=VECTOR('',#121436,1000.) ;
#11497=VECTOR('',#121437,1000.) ;
#11498=VECTOR('',#121438,1000.) ;
#11499=VECTOR('',#121441,1000.) ;
#11500=VECTOR('',#121444,1000.) ;
#11501=VECTOR('',#121447,1000.) ;
#11502=VECTOR('',#121452,1000.) ;
#11503=VECTOR('',#121453,1000.) ;
#11504=VECTOR('',#121454,1000.) ;
#11505=VECTOR('',#121455,1000.) ;
#11506=VECTOR('',#121456,1000.) ;
#11507=VECTOR('',#121459,1000.) ;
#11508=VECTOR('',#121462,1000.) ;
#11509=VECTOR('',#121465,1000.) ;
#11510=VECTOR('',#121470,1000.) ;
#11511=VECTOR('',#121471,1000.) ;
#11512=VECTOR('',#121472,1000.) ;
#11513=VECTOR('',#121473,1000.) ;
#11514=VECTOR('',#121474,1000.) ;
#11515=VECTOR('',#121477,1000.) ;
#11516=VECTOR('',#121480,1000.) ;
#11517=VECTOR('',#121483,1000.) ;
#11518=VECTOR('',#121488,1000.) ;
#11519=VECTOR('',#121489,1000.) ;
#11520=VECTOR('',#121490,1000.) ;
#11521=VECTOR('',#121491,1000.) ;
#11522=VECTOR('',#121492,1000.) ;
#11523=VECTOR('',#121495,1000.) ;
#11524=VECTOR('',#121498,1000.) ;
#11525=VECTOR('',#121501,1000.) ;
#11526=VECTOR('',#121506,1000.) ;
#11527=VECTOR('',#121507,1000.) ;
#11528=VECTOR('',#121508,1000.) ;
#11529=VECTOR('',#121509,1000.) ;
#11530=VECTOR('',#121510,1000.) ;
#11531=VECTOR('',#121513,1000.) ;
#11532=VECTOR('',#121516,1000.) ;
#11533=VECTOR('',#121519,1000.) ;
#11534=VECTOR('',#121524,1000.) ;
#11535=VECTOR('',#121527,1000.) ;
#11536=VECTOR('',#121530,1000.) ;
#11537=VECTOR('',#121533,1000.) ;
#11538=VECTOR('',#121536,1000.) ;
#11539=VECTOR('',#121539,1000.) ;
#11540=VECTOR('',#121542,1000.) ;
#11541=VECTOR('',#121545,1000.) ;
#11542=VECTOR('',#121548,1000.) ;
#11543=VECTOR('',#121551,1000.) ;
#11544=VECTOR('',#121552,1000.) ;
#11545=VECTOR('',#121553,1000.) ;
#11546=VECTOR('',#121554,1000.) ;
#11547=VECTOR('',#121555,1000.) ;
#11548=VECTOR('',#121560,1000.) ;
#11549=VECTOR('',#121565,1000.) ;
#11550=VECTOR('',#121570,1000.) ;
#11551=VECTOR('',#121575,1000.) ;
#11552=VECTOR('',#121580,1000.) ;
#11553=VECTOR('',#121585,1000.) ;
#11554=VECTOR('',#121590,1000.) ;
#11555=VECTOR('',#121595,1000.) ;
#11556=VECTOR('',#121600,1000.) ;
#11557=VECTOR('',#121605,1000.) ;
#11558=VECTOR('',#121610,1000.) ;
#11559=VECTOR('',#121615,1000.) ;
#11560=VECTOR('',#121620,1000.) ;
#11561=VECTOR('',#121625,1000.) ;
#11562=VECTOR('',#121630,1000.) ;
#11563=VECTOR('',#121635,1000.) ;
#11564=VECTOR('',#121640,1000.) ;
#11565=VECTOR('',#121645,1000.) ;
#11566=VECTOR('',#121650,1000.) ;
#11567=VECTOR('',#121659,1000.) ;
#11568=VECTOR('',#121660,1000.) ;
#11569=VECTOR('',#121661,1000.) ;
#11570=VECTOR('',#121662,1000.) ;
#11571=VECTOR('',#121663,1000.) ;
#11572=VECTOR('',#121672,1000.) ;
#11573=VECTOR('',#121673,1000.) ;
#11574=VECTOR('',#121674,1000.) ;
#11575=VECTOR('',#121675,1000.) ;
#11576=VECTOR('',#121676,1000.) ;
#11577=VECTOR('',#121685,1000.) ;
#11578=VECTOR('',#121686,1000.) ;
#11579=VECTOR('',#121687,1000.) ;
#11580=VECTOR('',#121688,1000.) ;
#11581=VECTOR('',#121689,1000.) ;
#11582=VECTOR('',#121698,1000.) ;
#11583=VECTOR('',#121699,1000.) ;
#11584=VECTOR('',#121700,1000.) ;
#11585=VECTOR('',#121701,1000.) ;
#11586=VECTOR('',#121702,1000.) ;
#11587=VECTOR('',#121711,1000.) ;
#11588=VECTOR('',#121712,1000.) ;
#11589=VECTOR('',#121713,1000.) ;
#11590=VECTOR('',#121714,1000.) ;
#11591=VECTOR('',#121715,1000.) ;
#11592=VECTOR('',#121724,1000.) ;
#11593=VECTOR('',#121725,1000.) ;
#11594=VECTOR('',#121726,1000.) ;
#11595=VECTOR('',#121727,1000.) ;
#11596=VECTOR('',#121728,1000.) ;
#11597=VECTOR('',#121737,1000.) ;
#11598=VECTOR('',#121738,1000.) ;
#11599=VECTOR('',#121739,1000.) ;
#11600=VECTOR('',#121740,1000.) ;
#11601=VECTOR('',#121741,1000.) ;
#11602=VECTOR('',#121750,1000.) ;
#11603=VECTOR('',#121751,1000.) ;
#11604=VECTOR('',#121752,1000.) ;
#11605=VECTOR('',#121753,1000.) ;
#11606=VECTOR('',#121754,1000.) ;
#11607=VECTOR('',#121763,1000.) ;
#11608=VECTOR('',#121764,1000.) ;
#11609=VECTOR('',#121765,1000.) ;
#11610=VECTOR('',#121766,1000.) ;
#11611=VECTOR('',#121767,1000.) ;
#11612=VECTOR('',#121774,1000.) ;
#11613=VECTOR('',#121775,1000.) ;
#11614=VECTOR('',#121776,1000.) ;
#11615=VECTOR('',#121777,1000.) ;
#11616=VECTOR('',#121780,1000.) ;
#11617=VECTOR('',#121781,1000.) ;
#11618=VECTOR('',#121782,1000.) ;
#11619=VECTOR('',#121783,1000.) ;
#11620=VECTOR('',#121786,1000.) ;
#11621=VECTOR('',#121789,1000.) ;
#11622=VECTOR('',#121790,1000.) ;
#11623=VECTOR('',#121791,1000.) ;
#11624=VECTOR('',#121794,1000.) ;
#11625=VECTOR('',#121797,1000.) ;
#11626=VECTOR('',#121798,1000.) ;
#11627=VECTOR('',#121799,1000.) ;
#11628=VECTOR('',#121802,1000.) ;
#11629=VECTOR('',#121805,1000.) ;
#11630=VECTOR('',#121806,1000.) ;
#11631=VECTOR('',#121807,1000.) ;
#11632=VECTOR('',#121810,1000.) ;
#11633=VECTOR('',#121813,1000.) ;
#11634=VECTOR('',#121814,1000.) ;
#11635=VECTOR('',#121815,1000.) ;
#11636=VECTOR('',#121818,1000.) ;
#11637=VECTOR('',#121821,1000.) ;
#11638=VECTOR('',#121822,1000.) ;
#11639=VECTOR('',#121823,1000.) ;
#11640=VECTOR('',#121826,1000.) ;
#11641=VECTOR('',#121829,1000.) ;
#11642=VECTOR('',#121830,1000.) ;
#11643=VECTOR('',#121831,1000.) ;
#11644=VECTOR('',#121834,1000.) ;
#11645=VECTOR('',#121837,1000.) ;
#11646=VECTOR('',#121838,1000.) ;
#11647=VECTOR('',#121839,1000.) ;
#11648=VECTOR('',#121842,1000.) ;
#11649=VECTOR('',#121845,1000.) ;
#11650=VECTOR('',#121846,1000.) ;
#11651=VECTOR('',#121847,1000.) ;
#11652=VECTOR('',#121850,1000.) ;
#11653=VECTOR('',#121853,1000.) ;
#11654=VECTOR('',#121854,1000.) ;
#11655=VECTOR('',#121855,1000.) ;
#11656=VECTOR('',#121858,1000.) ;
#11657=VECTOR('',#121861,1000.) ;
#11658=VECTOR('',#121862,1000.) ;
#11659=VECTOR('',#121863,1000.) ;
#11660=VECTOR('',#121866,1000.) ;
#11661=VECTOR('',#121873,1000.) ;
#11662=VECTOR('',#121884,1000.) ;
#11663=VECTOR('',#121885,1000.) ;
#11664=VECTOR('',#121886,1000.) ;
#11665=VECTOR('',#121887,1000.) ;
#11666=VECTOR('',#121888,1000.) ;
#11667=VECTOR('',#121889,1000.) ;
#11668=VECTOR('',#121890,1000.) ;
#11669=VECTOR('',#121891,1000.) ;
#11670=VECTOR('',#121892,1000.) ;
#11671=VECTOR('',#121893,1000.) ;
#11672=VECTOR('',#121894,1000.) ;
#11673=VECTOR('',#121895,1000.) ;
#11674=VECTOR('',#121896,1000.) ;
#11675=VECTOR('',#121897,1000.) ;
#11676=VECTOR('',#121898,1000.) ;
#11677=VECTOR('',#121899,1000.) ;
#11678=VECTOR('',#121900,1000.) ;
#11679=VECTOR('',#121901,1000.) ;
#11680=VECTOR('',#121902,1000.) ;
#11681=VECTOR('',#121903,1000.) ;
#11682=VECTOR('',#121904,1000.) ;
#11683=VECTOR('',#121905,1000.) ;
#11684=VECTOR('',#121906,1000.) ;
#11685=VECTOR('',#121907,1000.) ;
#11686=VECTOR('',#121908,1000.) ;
#11687=VECTOR('',#121909,1000.) ;
#11688=VECTOR('',#121910,1000.) ;
#11689=VECTOR('',#121911,1000.) ;
#11690=VECTOR('',#121912,1000.) ;
#11691=VECTOR('',#121913,1000.) ;
#11692=VECTOR('',#121914,1000.) ;
#11693=VECTOR('',#121915,1000.) ;
#11694=VECTOR('',#121916,1000.) ;
#11695=VECTOR('',#121917,1000.) ;
#11696=VECTOR('',#121918,1000.) ;
#11697=VECTOR('',#121919,1000.) ;
#11698=VECTOR('',#121920,1000.) ;
#11699=VECTOR('',#121921,1000.) ;
#11700=VECTOR('',#121922,1000.) ;
#11701=VECTOR('',#121923,1000.) ;
#11702=VECTOR('',#121924,1000.) ;
#11703=VECTOR('',#121925,1000.) ;
#11704=VECTOR('',#121926,1000.) ;
#11705=VECTOR('',#121927,1000.) ;
#11706=VECTOR('',#121930,1000.) ;
#11707=VECTOR('',#121931,1000.) ;
#11708=VECTOR('',#121932,1000.) ;
#11709=VECTOR('',#121933,1000.) ;
#11710=VECTOR('',#121934,1000.) ;
#11711=VECTOR('',#121937,1000.) ;
#11712=VECTOR('',#121940,1000.) ;
#11713=VECTOR('',#121943,1000.) ;
#11714=VECTOR('',#121948,1000.) ;
#11715=VECTOR('',#121949,1000.) ;
#11716=VECTOR('',#121950,1000.) ;
#11717=VECTOR('',#121951,1000.) ;
#11718=VECTOR('',#121954,1000.) ;
#11719=VECTOR('',#121957,1000.) ;
#11720=VECTOR('',#121958,1000.) ;
#11721=VECTOR('',#121959,1000.) ;
#11722=VECTOR('',#121960,1000.) ;
#11723=VECTOR('',#121967,1000.) ;
#11724=VECTOR('',#121970,1000.) ;
#11725=VECTOR('',#121971,1000.) ;
#11726=VECTOR('',#121972,1000.) ;
#11727=VECTOR('',#121973,1000.) ;
#11728=VECTOR('',#121976,1000.) ;
#11729=VECTOR('',#121977,1000.) ;
#11730=VECTOR('',#121978,1000.) ;
#11731=VECTOR('',#121981,1000.) ;
#11732=VECTOR('',#121982,1000.) ;
#11733=VECTOR('',#121983,1000.) ;
#11734=VECTOR('',#121984,1000.) ;
#11735=VECTOR('',#121987,1000.) ;
#11736=VECTOR('',#121988,1000.) ;
#11737=VECTOR('',#121989,1000.) ;
#11738=VECTOR('',#121990,1000.) ;
#11739=VECTOR('',#121991,1000.) ;
#11740=VECTOR('',#121992,1000.) ;
#11741=VECTOR('',#121993,1000.) ;
#11742=VECTOR('',#121994,1000.) ;
#11743=VECTOR('',#121995,1000.) ;
#11744=VECTOR('',#121996,1000.) ;
#11745=VECTOR('',#121997,1000.) ;
#11746=VECTOR('',#121998,1000.) ;
#11747=VECTOR('',#121999,1000.) ;
#11748=VECTOR('',#122000,1000.) ;
#11749=VECTOR('',#122001,1000.) ;
#11750=VECTOR('',#122002,1000.) ;
#11751=VECTOR('',#122003,1000.) ;
#11752=VECTOR('',#122004,1000.) ;
#11753=VECTOR('',#122005,1000.) ;
#11754=VECTOR('',#122006,1000.) ;
#11755=VECTOR('',#122007,1000.) ;
#11756=VECTOR('',#122008,1000.) ;
#11757=VECTOR('',#122009,1000.) ;
#11758=VECTOR('',#122010,1000.) ;
#11759=VECTOR('',#122011,1000.) ;
#11760=VECTOR('',#122012,1000.) ;
#11761=VECTOR('',#122013,1000.) ;
#11762=VECTOR('',#122014,1000.) ;
#11763=VECTOR('',#122015,1000.) ;
#11764=VECTOR('',#122016,1000.) ;
#11765=VECTOR('',#122017,1000.) ;
#11766=VECTOR('',#122018,1000.) ;
#11767=VECTOR('',#122019,1000.) ;
#11768=VECTOR('',#122020,1000.) ;
#11769=VECTOR('',#122021,1000.) ;
#11770=VECTOR('',#122022,1000.) ;
#11771=VECTOR('',#122025,1000.) ;
#11772=VECTOR('',#122028,1000.) ;
#11773=VECTOR('',#122031,1000.) ;
#11774=VECTOR('',#122034,1000.) ;
#11775=VECTOR('',#122037,1000.) ;
#11776=VECTOR('',#122040,1000.) ;
#11777=VECTOR('',#122043,1000.) ;
#11778=VECTOR('',#122046,1000.) ;
#11779=VECTOR('',#122049,1000.) ;
#11780=VECTOR('',#122050,1000.) ;
#11781=VECTOR('',#122051,1000.) ;
#11782=VECTOR('',#122054,1000.) ;
#11783=VECTOR('',#122055,1000.) ;
#11784=VECTOR('',#122056,1000.) ;
#11785=VECTOR('',#122059,1000.) ;
#11786=VECTOR('',#122060,1000.) ;
#11787=VECTOR('',#122061,1000.) ;
#11788=VECTOR('',#122062,1000.) ;
#11789=VECTOR('',#122065,1000.) ;
#11790=VECTOR('',#122066,1000.) ;
#11791=VECTOR('',#122069,1000.) ;
#11792=VECTOR('',#122070,1000.) ;
#11793=VECTOR('',#122071,1000.) ;
#11794=VECTOR('',#122072,1000.) ;
#11795=VECTOR('',#122073,1000.) ;
#11796=VECTOR('',#122076,1000.) ;
#11797=VECTOR('',#122077,1000.) ;
#11798=VECTOR('',#122078,1000.) ;
#11799=VECTOR('',#122079,1000.) ;
#11800=VECTOR('',#122082,1000.) ;
#11801=VECTOR('',#122083,1000.) ;
#11802=VECTOR('',#122084,1000.) ;
#11803=VECTOR('',#122089,1000.) ;
#11804=VECTOR('',#122090,1000.) ;
#11805=VECTOR('',#122091,1000.) ;
#11806=VECTOR('',#122092,1000.) ;
#11807=VECTOR('',#122095,1000.) ;
#11808=VECTOR('',#122096,1000.) ;
#11809=VECTOR('',#122097,1000.) ;
#11810=VECTOR('',#122098,1000.) ;
#11811=VECTOR('',#122101,1000.) ;
#11812=VECTOR('',#122104,1000.) ;
#11813=VECTOR('',#122107,1000.) ;
#11814=VECTOR('',#122114,1000.) ;
#11815=VECTOR('',#122115,1000.) ;
#11816=VECTOR('',#122116,1000.) ;
#11817=VECTOR('',#122119,1000.) ;
#11818=VECTOR('',#122120,1000.) ;
#11819=VECTOR('',#122121,1000.) ;
#11820=VECTOR('',#122122,1000.) ;
#11821=VECTOR('',#122125,1000.) ;
#11822=VECTOR('',#122126,1000.) ;
#11823=VECTOR('',#122127,1000.) ;
#11824=VECTOR('',#122128,1000.) ;
#11825=VECTOR('',#122129,1000.) ;
#11826=VECTOR('',#122132,1000.) ;
#11827=VECTOR('',#122133,1000.) ;
#11828=VECTOR('',#122134,1000.) ;
#11829=VECTOR('',#122135,1000.) ;
#11830=VECTOR('',#122136,1000.) ;
#11831=VECTOR('',#122139,1000.) ;
#11832=VECTOR('',#122140,1000.) ;
#11833=VECTOR('',#122141,1000.) ;
#11834=VECTOR('',#122142,1000.) ;
#11835=VECTOR('',#122145,1000.) ;
#11836=VECTOR('',#122146,1000.) ;
#11837=VECTOR('',#122147,1000.) ;
#11838=VECTOR('',#122148,1000.) ;
#11839=VECTOR('',#122151,1000.) ;
#11840=VECTOR('',#122152,1000.) ;
#11841=VECTOR('',#122153,1000.) ;
#11842=VECTOR('',#122154,1000.) ;
#11843=VECTOR('',#122157,1000.) ;
#11844=VECTOR('',#122158,1000.) ;
#11845=VECTOR('',#122159,1000.) ;
#11846=VECTOR('',#122160,1000.) ;
#11847=VECTOR('',#122163,1000.) ;
#11848=VECTOR('',#122164,1000.) ;
#11849=VECTOR('',#122165,1000.) ;
#11850=VECTOR('',#122166,1000.) ;
#11851=VECTOR('',#122167,1000.) ;
#11852=VECTOR('',#122170,1000.) ;
#11853=VECTOR('',#122173,1000.) ;
#11854=VECTOR('',#122176,1000.) ;
#11855=VECTOR('',#122181,1000.) ;
#11856=VECTOR('',#122182,1000.) ;
#11857=VECTOR('',#122183,1000.) ;
#11858=VECTOR('',#122186,1000.) ;
#11859=VECTOR('',#122187,1000.) ;
#11860=VECTOR('',#122188,1000.) ;
#11861=VECTOR('',#122191,1000.) ;
#11862=VECTOR('',#122192,1000.) ;
#11863=VECTOR('',#122193,1000.) ;
#11864=VECTOR('',#122196,1000.) ;
#11865=VECTOR('',#122197,1000.) ;
#11866=VECTOR('',#122198,1000.) ;
#11867=VECTOR('',#122201,1000.) ;
#11868=VECTOR('',#122202,1000.) ;
#11869=VECTOR('',#122203,1000.) ;
#11870=VECTOR('',#122204,1000.) ;
#11871=VECTOR('',#122207,1000.) ;
#11872=VECTOR('',#122208,1000.) ;
#11873=VECTOR('',#122211,1000.) ;
#11874=VECTOR('',#122212,1000.) ;
#11875=VECTOR('',#122215,1000.) ;
#11876=VECTOR('',#122216,1000.) ;
#11877=VECTOR('',#122219,1000.) ;
#11878=VECTOR('',#122220,1000.) ;
#11879=VECTOR('',#122221,1000.) ;
#11880=VECTOR('',#122222,1000.) ;
#11881=VECTOR('',#122229,1000.) ;
#11882=VECTOR('',#122230,1000.) ;
#11883=VECTOR('',#122231,1000.) ;
#11884=VECTOR('',#122232,1000.) ;
#11885=VECTOR('',#122235,1000.) ;
#11886=VECTOR('',#122236,1000.) ;
#11887=VECTOR('',#122237,1000.) ;
#11888=VECTOR('',#122240,1000.) ;
#11889=VECTOR('',#122241,1000.) ;
#11890=VECTOR('',#122242,1000.) ;
#11891=VECTOR('',#122243,1000.) ;
#11892=VECTOR('',#122246,1000.) ;
#11893=VECTOR('',#122251,1000.) ;
#11894=VECTOR('',#122252,1000.) ;
#11895=VECTOR('',#122253,1000.) ;
#11896=VECTOR('',#122256,1000.) ;
#11897=VECTOR('',#122257,1000.) ;
#11898=VECTOR('',#122258,1000.) ;
#11899=VECTOR('',#122261,1000.) ;
#11900=VECTOR('',#122262,1000.) ;
#11901=VECTOR('',#122263,1000.) ;
#11902=VECTOR('',#122266,1000.) ;
#11903=VECTOR('',#122267,1000.) ;
#11904=VECTOR('',#122268,1000.) ;
#11905=VECTOR('',#122269,1000.) ;
#11906=VECTOR('',#122272,1000.) ;
#11907=VECTOR('',#122273,1000.) ;
#11908=VECTOR('',#122274,1000.) ;
#11909=VECTOR('',#122275,1000.) ;
#11910=VECTOR('',#122278,1000.) ;
#11911=VECTOR('',#122281,1000.) ;
#11912=VECTOR('',#122286,1000.) ;
#11913=VECTOR('',#122289,1000.) ;
#11914=VECTOR('',#122290,1000.) ;
#11915=VECTOR('',#122291,1000.) ;
#11916=VECTOR('',#122292,1000.) ;
#11917=VECTOR('',#122297,1000.) ;
#11918=VECTOR('',#122298,1000.) ;
#11919=VECTOR('',#122299,1000.) ;
#11920=VECTOR('',#122300,1000.) ;
#11921=VECTOR('',#122303,1000.) ;
#11922=VECTOR('',#122304,1000.) ;
#11923=VECTOR('',#122305,1000.) ;
#11924=VECTOR('',#122306,1000.) ;
#11925=VECTOR('',#122309,1000.) ;
#11926=VECTOR('',#122310,1000.) ;
#11927=VECTOR('',#122311,1000.) ;
#11928=VECTOR('',#122312,1000.) ;
#11929=VECTOR('',#122315,1000.) ;
#11930=VECTOR('',#122316,1000.) ;
#11931=VECTOR('',#122317,1000.) ;
#11932=VECTOR('',#122318,1000.) ;
#11933=VECTOR('',#122321,1000.) ;
#11934=VECTOR('',#122322,1000.) ;
#11935=VECTOR('',#122323,1000.) ;
#11936=VECTOR('',#122324,1000.) ;
#11937=VECTOR('',#122325,1000.) ;
#11938=VECTOR('',#122328,1000.) ;
#11939=VECTOR('',#122331,1000.) ;
#11940=VECTOR('',#122334,1000.) ;
#11941=VECTOR('',#122339,1000.) ;
#11942=VECTOR('',#122340,1000.) ;
#11943=VECTOR('',#122341,1000.) ;
#11944=VECTOR('',#122344,1000.) ;
#11945=VECTOR('',#122345,1000.) ;
#11946=VECTOR('',#122346,1000.) ;
#11947=VECTOR('',#122349,1000.) ;
#11948=VECTOR('',#122350,1000.) ;
#11949=VECTOR('',#122351,1000.) ;
#11950=VECTOR('',#122354,1000.) ;
#11951=VECTOR('',#122355,1000.) ;
#11952=VECTOR('',#122356,1000.) ;
#11953=VECTOR('',#122359,1000.) ;
#11954=VECTOR('',#122360,1000.) ;
#11955=VECTOR('',#122361,1000.) ;
#11956=VECTOR('',#122362,1000.) ;
#11957=VECTOR('',#122365,1000.) ;
#11958=VECTOR('',#122368,1000.) ;
#11959=VECTOR('',#122369,1000.) ;
#11960=VECTOR('',#122372,1000.) ;
#11961=VECTOR('',#122373,1000.) ;
#11962=VECTOR('',#122376,1000.) ;
#11963=VECTOR('',#122377,1000.) ;
#11964=VECTOR('',#122388,1000.) ;
#11965=VECTOR('',#122389,1000.) ;
#11966=VECTOR('',#122390,1000.) ;
#11967=VECTOR('',#122393,1000.) ;
#11968=VECTOR('',#122394,1000.) ;
#11969=VECTOR('',#122395,1000.) ;
#11970=VECTOR('',#122406,1000.) ;
#11971=VECTOR('',#122409,1000.) ;
#11972=VECTOR('',#122414,1000.) ;
#11973=VECTOR('',#122415,1000.) ;
#11974=VECTOR('',#122416,1000.) ;
#11975=VECTOR('',#122421,1000.) ;
#11976=VECTOR('',#122426,1000.) ;
#11977=VECTOR('',#122427,1000.) ;
#11978=VECTOR('',#122428,1000.) ;
#11979=VECTOR('',#122433,1000.) ;
#11980=VECTOR('',#122438,1000.) ;
#11981=VECTOR('',#122439,1000.) ;
#11982=VECTOR('',#122440,1000.) ;
#11983=VECTOR('',#122445,1000.) ;
#11984=VECTOR('',#122450,1000.) ;
#11985=VECTOR('',#122451,1000.) ;
#11986=VECTOR('',#122454,1000.) ;
#11987=VECTOR('',#122455,1000.) ;
#11988=VECTOR('',#122456,1000.) ;
#11989=VECTOR('',#122457,1000.) ;
#11990=VECTOR('',#123260,1000.) ;
#11991=VECTOR('',#123261,1000.) ;
#11992=VECTOR('',#123262,1000.) ;
#11993=VECTOR('',#123263,1000.) ;
#11994=VECTOR('',#123266,1000.) ;
#11995=VECTOR('',#123267,1000.) ;
#11996=VECTOR('',#123268,1000.) ;
#11997=VECTOR('',#123269,1000.) ;
#11998=VECTOR('',#123272,1000.) ;
#11999=VECTOR('',#123275,1000.) ;
#12000=VECTOR('',#123278,1000.) ;
#12001=VECTOR('',#123285,1000.) ;
#12002=VECTOR('',#123286,1000.) ;
#12003=VECTOR('',#123287,1000.) ;
#12004=VECTOR('',#123290,1000.) ;
#12005=VECTOR('',#123291,1000.) ;
#12006=VECTOR('',#123292,1000.) ;
#12007=VECTOR('',#123293,1000.) ;
#12008=VECTOR('',#123296,1000.) ;
#12009=VECTOR('',#123297,1000.) ;
#12010=VECTOR('',#123298,1000.) ;
#12011=VECTOR('',#123299,1000.) ;
#12012=VECTOR('',#123302,1000.) ;
#12013=VECTOR('',#123303,1000.) ;
#12014=VECTOR('',#123304,1000.) ;
#12015=VECTOR('',#123305,1000.) ;
#12016=VECTOR('',#123308,1000.) ;
#12017=VECTOR('',#123311,1000.) ;
#12018=VECTOR('',#123314,1000.) ;
#12019=VECTOR('',#123321,1000.) ;
#12020=VECTOR('',#123322,1000.) ;
#12021=VECTOR('',#123323,1000.) ;
#12022=VECTOR('',#123326,1000.) ;
#12023=VECTOR('',#123327,1000.) ;
#12024=VECTOR('',#123328,1000.) ;
#12025=VECTOR('',#123329,1000.) ;
#12026=VECTOR('',#123332,1000.) ;
#12027=VECTOR('',#123333,1000.) ;
#12028=VECTOR('',#123334,1000.) ;
#12029=VECTOR('',#123335,1000.) ;
#12030=VECTOR('',#123338,1000.) ;
#12031=VECTOR('',#123339,1000.) ;
#12032=VECTOR('',#123340,1000.) ;
#12033=VECTOR('',#123341,1000.) ;
#12034=VECTOR('',#123344,1000.) ;
#12035=VECTOR('',#123347,1000.) ;
#12036=VECTOR('',#123350,1000.) ;
#12037=VECTOR('',#123357,1000.) ;
#12038=VECTOR('',#123358,1000.) ;
#12039=VECTOR('',#123359,1000.) ;
#12040=VECTOR('',#123362,1000.) ;
#12041=VECTOR('',#123363,1000.) ;
#12042=VECTOR('',#123364,1000.) ;
#12043=VECTOR('',#123365,1000.) ;
#12044=VECTOR('',#123368,1000.) ;
#12045=VECTOR('',#123369,1000.) ;
#12046=VECTOR('',#123370,1000.) ;
#12047=VECTOR('',#123371,1000.) ;
#12048=VECTOR('',#123374,1000.) ;
#12049=VECTOR('',#123375,1000.) ;
#12050=VECTOR('',#123376,1000.) ;
#12051=VECTOR('',#123377,1000.) ;
#12052=VECTOR('',#123380,1000.) ;
#12053=VECTOR('',#123383,1000.) ;
#12054=VECTOR('',#123386,1000.) ;
#12055=VECTOR('',#123393,1000.) ;
#12056=VECTOR('',#123394,1000.) ;
#12057=VECTOR('',#123395,1000.) ;
#12058=VECTOR('',#123398,1000.) ;
#12059=VECTOR('',#123399,1000.) ;
#12060=VECTOR('',#123400,1000.) ;
#12061=VECTOR('',#123401,1000.) ;
#12062=VECTOR('',#123404,1000.) ;
#12063=VECTOR('',#123405,1000.) ;
#12064=VECTOR('',#123406,1000.) ;
#12065=VECTOR('',#123407,1000.) ;
#12066=VECTOR('',#123410,1000.) ;
#12067=VECTOR('',#123411,1000.) ;
#12068=VECTOR('',#123412,1000.) ;
#12069=VECTOR('',#123413,1000.) ;
#12070=VECTOR('',#123416,1000.) ;
#12071=VECTOR('',#123419,1000.) ;
#12072=VECTOR('',#123422,1000.) ;
#12073=VECTOR('',#123429,1000.) ;
#12074=VECTOR('',#123430,1000.) ;
#12075=VECTOR('',#123431,1000.) ;
#12076=VECTOR('',#123434,1000.) ;
#12077=VECTOR('',#123435,1000.) ;
#12078=VECTOR('',#123436,1000.) ;
#12079=VECTOR('',#123437,1000.) ;
#12080=VECTOR('',#123440,1000.) ;
#12081=VECTOR('',#123441,1000.) ;
#12082=VECTOR('',#123442,1000.) ;
#12083=VECTOR('',#123443,1000.) ;
#12084=VECTOR('',#123446,1000.) ;
#12085=VECTOR('',#123447,1000.) ;
#12086=VECTOR('',#123448,1000.) ;
#12087=VECTOR('',#123449,1000.) ;
#12088=VECTOR('',#123452,1000.) ;
#12089=VECTOR('',#123455,1000.) ;
#12090=VECTOR('',#123458,1000.) ;
#12091=VECTOR('',#123465,1000.) ;
#12092=VECTOR('',#123466,1000.) ;
#12093=VECTOR('',#123467,1000.) ;
#12094=VECTOR('',#123470,1000.) ;
#12095=VECTOR('',#123471,1000.) ;
#12096=VECTOR('',#123472,1000.) ;
#12097=VECTOR('',#123473,1000.) ;
#12098=VECTOR('',#123476,1000.) ;
#12099=VECTOR('',#123477,1000.) ;
#12100=VECTOR('',#123478,1000.) ;
#12101=VECTOR('',#123479,1000.) ;
#12102=VECTOR('',#123482,1000.) ;
#12103=VECTOR('',#123483,1000.) ;
#12104=VECTOR('',#123484,1000.) ;
#12105=VECTOR('',#123485,1000.) ;
#12106=VECTOR('',#123488,1000.) ;
#12107=VECTOR('',#123491,1000.) ;
#12108=VECTOR('',#123494,1000.) ;
#12109=VECTOR('',#123501,1000.) ;
#12110=VECTOR('',#123502,1000.) ;
#12111=VECTOR('',#123503,1000.) ;
#12112=VECTOR('',#123506,1000.) ;
#12113=VECTOR('',#123507,1000.) ;
#12114=VECTOR('',#123508,1000.) ;
#12115=VECTOR('',#123509,1000.) ;
#12116=VECTOR('',#123512,1000.) ;
#12117=VECTOR('',#123513,1000.) ;
#12118=VECTOR('',#123514,1000.) ;
#12119=VECTOR('',#123515,1000.) ;
#12120=VECTOR('',#123518,1000.) ;
#12121=VECTOR('',#123519,1000.) ;
#12122=VECTOR('',#123520,1000.) ;
#12123=VECTOR('',#123521,1000.) ;
#12124=VECTOR('',#123524,1000.) ;
#12125=VECTOR('',#123527,1000.) ;
#12126=VECTOR('',#123530,1000.) ;
#12127=VECTOR('',#123537,1000.) ;
#12128=VECTOR('',#123538,1000.) ;
#12129=VECTOR('',#123539,1000.) ;
#12130=VECTOR('',#123542,1000.) ;
#12131=VECTOR('',#123543,1000.) ;
#12132=VECTOR('',#123544,1000.) ;
#12133=VECTOR('',#123545,1000.) ;
#12134=VECTOR('',#123548,1000.) ;
#12135=VECTOR('',#123549,1000.) ;
#12136=VECTOR('',#123550,1000.) ;
#12137=VECTOR('',#123551,1000.) ;
#12138=VECTOR('',#123554,1000.) ;
#12139=VECTOR('',#123555,1000.) ;
#12140=VECTOR('',#123556,1000.) ;
#12141=VECTOR('',#123557,1000.) ;
#12142=VECTOR('',#123560,1000.) ;
#12143=VECTOR('',#123563,1000.) ;
#12144=VECTOR('',#123566,1000.) ;
#12145=VECTOR('',#123573,1000.) ;
#12146=VECTOR('',#123574,1000.) ;
#12147=VECTOR('',#123575,1000.) ;
#12148=VECTOR('',#123578,1000.) ;
#12149=VECTOR('',#123579,1000.) ;
#12150=VECTOR('',#123580,1000.) ;
#12151=VECTOR('',#123581,1000.) ;
#12152=VECTOR('',#123584,1000.) ;
#12153=VECTOR('',#123585,1000.) ;
#12154=VECTOR('',#123586,1000.) ;
#12155=VECTOR('',#123587,1000.) ;
#12156=VECTOR('',#123588,1000.) ;
#12157=VECTOR('',#123591,1000.) ;
#12158=VECTOR('',#123594,1000.) ;
#12159=VECTOR('',#123595,1000.) ;
#12160=VECTOR('',#123596,1000.) ;
#12161=VECTOR('',#123597,1000.) ;
#12162=VECTOR('',#123602,1000.) ;
#12163=VECTOR('',#123605,1000.) ;
#12164=VECTOR('',#123606,1000.) ;
#12165=VECTOR('',#123607,1000.) ;
#12166=VECTOR('',#123608,1000.) ;
#12167=VECTOR('',#123613,1000.) ;
#12168=VECTOR('',#123616,1000.) ;
#12169=VECTOR('',#123617,1000.) ;
#12170=VECTOR('',#123618,1000.) ;
#12171=VECTOR('',#123619,1000.) ;
#12172=VECTOR('',#123624,1000.) ;
#12173=VECTOR('',#123627,1000.) ;
#12174=VECTOR('',#123628,1000.) ;
#12175=VECTOR('',#123629,1000.) ;
#12176=VECTOR('',#123630,1000.) ;
#12177=VECTOR('',#123635,1000.) ;
#12178=VECTOR('',#123638,1000.) ;
#12179=VECTOR('',#123639,1000.) ;
#12180=VECTOR('',#123640,1000.) ;
#12181=VECTOR('',#123641,1000.) ;
#12182=VECTOR('',#123646,1000.) ;
#12183=VECTOR('',#123649,1000.) ;
#12184=VECTOR('',#123650,1000.) ;
#12185=VECTOR('',#123651,1000.) ;
#12186=VECTOR('',#123652,1000.) ;
#12187=VECTOR('',#123657,1000.) ;
#12188=VECTOR('',#123660,1000.) ;
#12189=VECTOR('',#123661,1000.) ;
#12190=VECTOR('',#123662,1000.) ;
#12191=VECTOR('',#123663,1000.) ;
#12192=VECTOR('',#123668,1000.) ;
#12193=VECTOR('',#123671,1000.) ;
#12194=VECTOR('',#123672,1000.) ;
#12195=VECTOR('',#123673,1000.) ;
#12196=VECTOR('',#123674,1000.) ;
#12197=VECTOR('',#123679,1000.) ;
#12198=VECTOR('',#123680,1000.) ;
#12199=VECTOR('',#123681,1000.) ;
#12200=VECTOR('',#123682,1000.) ;
#12201=VECTOR('',#123683,1000.) ;
#12202=VECTOR('',#123686,1000.) ;
#12203=VECTOR('',#123689,1000.) ;
#12204=VECTOR('',#123690,1000.) ;
#12205=VECTOR('',#123691,1000.) ;
#12206=VECTOR('',#123692,1000.) ;
#12207=VECTOR('',#123697,1000.) ;
#12208=VECTOR('',#123700,1000.) ;
#12209=VECTOR('',#123701,1000.) ;
#12210=VECTOR('',#123702,1000.) ;
#12211=VECTOR('',#123703,1000.) ;
#12212=VECTOR('',#123708,1000.) ;
#12213=VECTOR('',#123711,1000.) ;
#12214=VECTOR('',#123712,1000.) ;
#12215=VECTOR('',#123713,1000.) ;
#12216=VECTOR('',#123714,1000.) ;
#12217=VECTOR('',#123719,1000.) ;
#12218=VECTOR('',#123722,1000.) ;
#12219=VECTOR('',#123723,1000.) ;
#12220=VECTOR('',#123724,1000.) ;
#12221=VECTOR('',#123725,1000.) ;
#12222=VECTOR('',#123730,1000.) ;
#12223=VECTOR('',#123733,1000.) ;
#12224=VECTOR('',#123734,1000.) ;
#12225=VECTOR('',#123735,1000.) ;
#12226=VECTOR('',#123736,1000.) ;
#12227=VECTOR('',#123741,1000.) ;
#12228=VECTOR('',#123744,1000.) ;
#12229=VECTOR('',#123745,1000.) ;
#12230=VECTOR('',#123746,1000.) ;
#12231=VECTOR('',#123747,1000.) ;
#12232=VECTOR('',#123752,1000.) ;
#12233=VECTOR('',#123755,1000.) ;
#12234=VECTOR('',#123756,1000.) ;
#12235=VECTOR('',#123757,1000.) ;
#12236=VECTOR('',#123758,1000.) ;
#12237=VECTOR('',#123763,1000.) ;
#12238=VECTOR('',#123766,1000.) ;
#12239=VECTOR('',#123767,1000.) ;
#12240=VECTOR('',#123768,1000.) ;
#12241=VECTOR('',#123769,1000.) ;
#12242=VECTOR('',#123774,1000.) ;
#12243=VECTOR('',#123775,1000.) ;
#12244=VECTOR('',#123776,1000.) ;
#12245=VECTOR('',#123777,1000.) ;
#12246=VECTOR('',#123780,1000.) ;
#12247=VECTOR('',#123781,1000.) ;
#12248=VECTOR('',#123782,1000.) ;
#12249=VECTOR('',#123783,1000.) ;
#12250=VECTOR('',#123786,1000.) ;
#12251=VECTOR('',#123787,1000.) ;
#12252=VECTOR('',#123788,1000.) ;
#12253=VECTOR('',#123789,1000.) ;
#12254=VECTOR('',#123792,1000.) ;
#12255=VECTOR('',#123793,1000.) ;
#12256=VECTOR('',#123794,1000.) ;
#12257=VECTOR('',#123795,1000.) ;
#12258=VECTOR('',#123798,1000.) ;
#12259=VECTOR('',#123799,1000.) ;
#12260=VECTOR('',#123800,1000.) ;
#12261=VECTOR('',#123801,1000.) ;
#12262=VECTOR('',#123804,1000.) ;
#12263=VECTOR('',#123805,1000.) ;
#12264=VECTOR('',#123806,1000.) ;
#12265=VECTOR('',#123807,1000.) ;
#12266=VECTOR('',#123810,1000.) ;
#12267=VECTOR('',#123811,1000.) ;
#12268=VECTOR('',#123812,1000.) ;
#12269=VECTOR('',#123813,1000.) ;
#12270=VECTOR('',#123816,1000.) ;
#12271=VECTOR('',#123817,1000.) ;
#12272=VECTOR('',#123818,1000.) ;
#12273=VECTOR('',#123819,1000.) ;
#12274=VECTOR('',#123822,1000.) ;
#12275=VECTOR('',#123823,1000.) ;
#12276=VECTOR('',#123824,1000.) ;
#12277=VECTOR('',#123825,1000.) ;
#12278=VECTOR('',#123828,1000.) ;
#12279=VECTOR('',#123829,1000.) ;
#12280=VECTOR('',#123830,1000.) ;
#12281=VECTOR('',#123831,1000.) ;
#12282=VECTOR('',#123834,1000.) ;
#12283=VECTOR('',#123835,1000.) ;
#12284=VECTOR('',#123836,1000.) ;
#12285=VECTOR('',#123837,1000.) ;
#12286=VECTOR('',#123840,1000.) ;
#12287=VECTOR('',#123841,1000.) ;
#12288=VECTOR('',#123842,1000.) ;
#12289=VECTOR('',#123843,1000.) ;
#12290=VECTOR('',#123846,1000.) ;
#12291=VECTOR('',#123847,1000.) ;
#12292=VECTOR('',#123848,1000.) ;
#12293=VECTOR('',#123849,1000.) ;
#12294=VECTOR('',#123852,1000.) ;
#12295=VECTOR('',#123853,1000.) ;
#12296=VECTOR('',#123854,1000.) ;
#12297=VECTOR('',#123855,1000.) ;
#12298=VECTOR('',#123858,1000.) ;
#12299=VECTOR('',#123859,1000.) ;
#12300=VECTOR('',#123860,1000.) ;
#12301=VECTOR('',#123861,1000.) ;
#12302=VECTOR('',#123864,1000.) ;
#12303=VECTOR('',#123865,1000.) ;
#12304=VECTOR('',#123866,1000.) ;
#12305=VECTOR('',#123867,1000.) ;
#12306=VECTOR('',#123870,1000.) ;
#12307=VECTOR('',#123871,1000.) ;
#12308=VECTOR('',#123872,1000.) ;
#12309=VECTOR('',#123873,1000.) ;
#12310=VECTOR('',#123876,1000.) ;
#12311=VECTOR('',#123877,1000.) ;
#12312=VECTOR('',#123878,1000.) ;
#12313=VECTOR('',#123879,1000.) ;
#12314=VECTOR('',#123882,1000.) ;
#12315=VECTOR('',#123883,1000.) ;
#12316=VECTOR('',#123884,1000.) ;
#12317=VECTOR('',#123885,1000.) ;
#12318=VECTOR('',#123888,1000.) ;
#12319=VECTOR('',#123889,1000.) ;
#12320=VECTOR('',#123890,1000.) ;
#12321=VECTOR('',#123891,1000.) ;
#12322=VECTOR('',#123894,1000.) ;
#12323=VECTOR('',#123895,1000.) ;
#12324=VECTOR('',#123896,1000.) ;
#12325=VECTOR('',#123897,1000.) ;
#12326=VECTOR('',#123900,1000.) ;
#12327=VECTOR('',#123901,1000.) ;
#12328=VECTOR('',#123902,1000.) ;
#12329=VECTOR('',#123903,1000.) ;
#12330=VECTOR('',#123906,1000.) ;
#12331=VECTOR('',#123907,1000.) ;
#12332=VECTOR('',#123908,1000.) ;
#12333=VECTOR('',#123909,1000.) ;
#12334=VECTOR('',#123912,1000.) ;
#12335=VECTOR('',#123913,1000.) ;
#12336=VECTOR('',#123914,1000.) ;
#12337=VECTOR('',#123915,1000.) ;
#12338=VECTOR('',#123918,1000.) ;
#12339=VECTOR('',#123919,1000.) ;
#12340=VECTOR('',#123920,1000.) ;
#12341=VECTOR('',#123921,1000.) ;
#12342=VECTOR('',#123924,1000.) ;
#12343=VECTOR('',#123925,1000.) ;
#12344=VECTOR('',#123926,1000.) ;
#12345=VECTOR('',#123927,1000.) ;
#12346=VECTOR('',#123930,1000.) ;
#12347=VECTOR('',#123931,1000.) ;
#12348=VECTOR('',#123932,1000.) ;
#12349=VECTOR('',#123933,1000.) ;
#12350=VECTOR('',#123936,1000.) ;
#12351=VECTOR('',#123937,1000.) ;
#12352=VECTOR('',#123938,1000.) ;
#12353=VECTOR('',#123939,1000.) ;
#12354=VECTOR('',#123942,1000.) ;
#12355=VECTOR('',#123943,1000.) ;
#12356=VECTOR('',#123944,1000.) ;
#12357=VECTOR('',#123945,1000.) ;
#12358=VECTOR('',#123948,1000.) ;
#12359=VECTOR('',#123949,1000.) ;
#12360=VECTOR('',#123950,1000.) ;
#12361=VECTOR('',#123951,1000.) ;
#12362=VECTOR('',#123954,1000.) ;
#12363=VECTOR('',#123955,1000.) ;
#12364=VECTOR('',#123956,1000.) ;
#12365=VECTOR('',#123957,1000.) ;
#12366=VECTOR('',#123960,1000.) ;
#12367=VECTOR('',#123961,1000.) ;
#12368=VECTOR('',#123962,1000.) ;
#12369=VECTOR('',#123963,1000.) ;
#12370=VECTOR('',#123966,1000.) ;
#12371=VECTOR('',#123967,1000.) ;
#12372=VECTOR('',#123968,1000.) ;
#12373=VECTOR('',#123969,1000.) ;
#12374=VECTOR('',#123972,1000.) ;
#12375=VECTOR('',#123973,1000.) ;
#12376=VECTOR('',#123974,1000.) ;
#12377=VECTOR('',#123975,1000.) ;
#12378=VECTOR('',#123978,1000.) ;
#12379=VECTOR('',#123979,1000.) ;
#12380=VECTOR('',#123980,1000.) ;
#12381=VECTOR('',#123981,1000.) ;
#12382=VECTOR('',#123984,1000.) ;
#12383=VECTOR('',#123985,1000.) ;
#12384=VECTOR('',#123986,1000.) ;
#12385=VECTOR('',#123987,1000.) ;
#12386=VECTOR('',#123990,1000.) ;
#12387=VECTOR('',#123991,1000.) ;
#12388=VECTOR('',#123992,1000.) ;
#12389=VECTOR('',#123993,1000.) ;
#12390=VECTOR('',#123994,1000.) ;
#12391=VECTOR('',#123997,1000.) ;
#12392=VECTOR('',#124000,1000.) ;
#12393=VECTOR('',#124003,1000.) ;
#12394=VECTOR('',#124008,1000.) ;
#12395=VECTOR('',#124009,1000.) ;
#12396=VECTOR('',#124010,1000.) ;
#12397=VECTOR('',#124013,1000.) ;
#12398=VECTOR('',#124014,1000.) ;
#12399=VECTOR('',#124015,1000.) ;
#12400=VECTOR('',#124018,1000.) ;
#12401=VECTOR('',#124019,1000.) ;
#12402=VECTOR('',#124020,1000.) ;
#12403=VECTOR('',#124023,1000.) ;
#12404=VECTOR('',#124024,1000.) ;
#12405=VECTOR('',#124025,1000.) ;
#12406=VECTOR('',#124028,1000.) ;
#12407=VECTOR('',#124029,1000.) ;
#12408=VECTOR('',#124030,1000.) ;
#12409=VECTOR('',#124031,1000.) ;
#12410=VECTOR('',#124032,1000.) ;
#12411=VECTOR('',#124035,1000.) ;
#12412=VECTOR('',#124038,1000.) ;
#12413=VECTOR('',#124041,1000.) ;
#12414=VECTOR('',#124046,1000.) ;
#12415=VECTOR('',#124047,1000.) ;
#12416=VECTOR('',#124048,1000.) ;
#12417=VECTOR('',#124051,1000.) ;
#12418=VECTOR('',#124052,1000.) ;
#12419=VECTOR('',#124053,1000.) ;
#12420=VECTOR('',#124056,1000.) ;
#12421=VECTOR('',#124057,1000.) ;
#12422=VECTOR('',#124058,1000.) ;
#12423=VECTOR('',#124061,1000.) ;
#12424=VECTOR('',#124062,1000.) ;
#12425=VECTOR('',#124063,1000.) ;
#12426=VECTOR('',#124066,1000.) ;
#12427=VECTOR('',#124067,1000.) ;
#12428=VECTOR('',#124068,1000.) ;
#12429=VECTOR('',#124069,1000.) ;
#12430=VECTOR('',#124070,1000.) ;
#12431=VECTOR('',#124073,1000.) ;
#12432=VECTOR('',#124076,1000.) ;
#12433=VECTOR('',#124079,1000.) ;
#12434=VECTOR('',#124084,1000.) ;
#12435=VECTOR('',#124085,1000.) ;
#12436=VECTOR('',#124086,1000.) ;
#12437=VECTOR('',#124089,1000.) ;
#12438=VECTOR('',#124090,1000.) ;
#12439=VECTOR('',#124091,1000.) ;
#12440=VECTOR('',#124094,1000.) ;
#12441=VECTOR('',#124095,1000.) ;
#12442=VECTOR('',#124096,1000.) ;
#12443=VECTOR('',#124099,1000.) ;
#12444=VECTOR('',#124100,1000.) ;
#12445=VECTOR('',#124101,1000.) ;
#12446=VECTOR('',#124104,1000.) ;
#12447=VECTOR('',#124105,1000.) ;
#12448=VECTOR('',#124106,1000.) ;
#12449=VECTOR('',#124107,1000.) ;
#12450=VECTOR('',#124108,1000.) ;
#12451=VECTOR('',#124111,1000.) ;
#12452=VECTOR('',#124114,1000.) ;
#12453=VECTOR('',#124117,1000.) ;
#12454=VECTOR('',#124122,1000.) ;
#12455=VECTOR('',#124123,1000.) ;
#12456=VECTOR('',#124124,1000.) ;
#12457=VECTOR('',#124127,1000.) ;
#12458=VECTOR('',#124128,1000.) ;
#12459=VECTOR('',#124129,1000.) ;
#12460=VECTOR('',#124132,1000.) ;
#12461=VECTOR('',#124133,1000.) ;
#12462=VECTOR('',#124134,1000.) ;
#12463=VECTOR('',#124137,1000.) ;
#12464=VECTOR('',#124138,1000.) ;
#12465=VECTOR('',#124139,1000.) ;
#12466=VECTOR('',#124142,1000.) ;
#12467=VECTOR('',#124143,1000.) ;
#12468=VECTOR('',#124144,1000.) ;
#12469=VECTOR('',#124145,1000.) ;
#12470=VECTOR('',#124146,1000.) ;
#12471=VECTOR('',#124149,1000.) ;
#12472=VECTOR('',#124152,1000.) ;
#12473=VECTOR('',#124155,1000.) ;
#12474=VECTOR('',#124160,1000.) ;
#12475=VECTOR('',#124161,1000.) ;
#12476=VECTOR('',#124162,1000.) ;
#12477=VECTOR('',#124165,1000.) ;
#12478=VECTOR('',#124166,1000.) ;
#12479=VECTOR('',#124167,1000.) ;
#12480=VECTOR('',#124170,1000.) ;
#12481=VECTOR('',#124171,1000.) ;
#12482=VECTOR('',#124172,1000.) ;
#12483=VECTOR('',#124175,1000.) ;
#12484=VECTOR('',#124176,1000.) ;
#12485=VECTOR('',#124177,1000.) ;
#12486=VECTOR('',#124180,1000.) ;
#12487=VECTOR('',#124181,1000.) ;
#12488=VECTOR('',#124182,1000.) ;
#12489=VECTOR('',#124183,1000.) ;
#12490=VECTOR('',#124184,1000.) ;
#12491=VECTOR('',#124187,1000.) ;
#12492=VECTOR('',#124190,1000.) ;
#12493=VECTOR('',#124193,1000.) ;
#12494=VECTOR('',#124198,1000.) ;
#12495=VECTOR('',#124199,1000.) ;
#12496=VECTOR('',#124200,1000.) ;
#12497=VECTOR('',#124203,1000.) ;
#12498=VECTOR('',#124204,1000.) ;
#12499=VECTOR('',#124205,1000.) ;
#12500=VECTOR('',#124208,1000.) ;
#12501=VECTOR('',#124209,1000.) ;
#12502=VECTOR('',#124210,1000.) ;
#12503=VECTOR('',#124213,1000.) ;
#12504=VECTOR('',#124214,1000.) ;
#12505=VECTOR('',#124215,1000.) ;
#12506=VECTOR('',#124218,1000.) ;
#12507=VECTOR('',#124219,1000.) ;
#12508=VECTOR('',#124220,1000.) ;
#12509=VECTOR('',#124221,1000.) ;
#12510=VECTOR('',#124222,1000.) ;
#12511=VECTOR('',#124225,1000.) ;
#12512=VECTOR('',#124228,1000.) ;
#12513=VECTOR('',#124231,1000.) ;
#12514=VECTOR('',#124236,1000.) ;
#12515=VECTOR('',#124237,1000.) ;
#12516=VECTOR('',#124238,1000.) ;
#12517=VECTOR('',#124241,1000.) ;
#12518=VECTOR('',#124242,1000.) ;
#12519=VECTOR('',#124243,1000.) ;
#12520=VECTOR('',#124246,1000.) ;
#12521=VECTOR('',#124247,1000.) ;
#12522=VECTOR('',#124248,1000.) ;
#12523=VECTOR('',#124251,1000.) ;
#12524=VECTOR('',#124252,1000.) ;
#12525=VECTOR('',#124253,1000.) ;
#12526=VECTOR('',#124256,1000.) ;
#12527=VECTOR('',#124257,1000.) ;
#12528=VECTOR('',#124258,1000.) ;
#12529=VECTOR('',#124259,1000.) ;
#12530=VECTOR('',#124260,1000.) ;
#12531=VECTOR('',#124263,1000.) ;
#12532=VECTOR('',#124266,1000.) ;
#12533=VECTOR('',#124269,1000.) ;
#12534=VECTOR('',#124274,1000.) ;
#12535=VECTOR('',#124275,1000.) ;
#12536=VECTOR('',#124276,1000.) ;
#12537=VECTOR('',#124279,1000.) ;
#12538=VECTOR('',#124280,1000.) ;
#12539=VECTOR('',#124281,1000.) ;
#12540=VECTOR('',#124284,1000.) ;
#12541=VECTOR('',#124285,1000.) ;
#12542=VECTOR('',#124286,1000.) ;
#12543=VECTOR('',#124289,1000.) ;
#12544=VECTOR('',#124290,1000.) ;
#12545=VECTOR('',#124291,1000.) ;
#12546=VECTOR('',#124294,1000.) ;
#12547=VECTOR('',#124295,1000.) ;
#12548=VECTOR('',#124296,1000.) ;
#12549=VECTOR('',#124297,1000.) ;
#12550=VECTOR('',#124298,1000.) ;
#12551=VECTOR('',#124301,1000.) ;
#12552=VECTOR('',#124304,1000.) ;
#12553=VECTOR('',#124307,1000.) ;
#12554=VECTOR('',#124312,1000.) ;
#12555=VECTOR('',#124313,1000.) ;
#12556=VECTOR('',#124314,1000.) ;
#12557=VECTOR('',#124317,1000.) ;
#12558=VECTOR('',#124318,1000.) ;
#12559=VECTOR('',#124319,1000.) ;
#12560=VECTOR('',#124322,1000.) ;
#12561=VECTOR('',#124323,1000.) ;
#12562=VECTOR('',#124324,1000.) ;
#12563=VECTOR('',#124327,1000.) ;
#12564=VECTOR('',#124328,1000.) ;
#12565=VECTOR('',#124329,1000.) ;
#12566=VECTOR('',#124332,1000.) ;
#12567=VECTOR('',#124333,1000.) ;
#12568=VECTOR('',#124334,1000.) ;
#12569=VECTOR('',#124335,1000.) ;
#12570=VECTOR('',#124338,1000.) ;
#12571=VECTOR('',#124339,1000.) ;
#12572=VECTOR('',#124340,1000.) ;
#12573=VECTOR('',#124341,1000.) ;
#12574=VECTOR('',#124344,1000.) ;
#12575=VECTOR('',#124345,1000.) ;
#12576=VECTOR('',#124346,1000.) ;
#12577=VECTOR('',#124347,1000.) ;
#12578=VECTOR('',#124350,1000.) ;
#12579=VECTOR('',#124351,1000.) ;
#12580=VECTOR('',#124352,1000.) ;
#12581=VECTOR('',#124353,1000.) ;
#12582=VECTOR('',#124356,1000.) ;
#12583=VECTOR('',#124357,1000.) ;
#12584=VECTOR('',#124358,1000.) ;
#12585=VECTOR('',#124359,1000.) ;
#12586=VECTOR('',#124362,1000.) ;
#12587=VECTOR('',#124363,1000.) ;
#12588=VECTOR('',#124364,1000.) ;
#12589=VECTOR('',#124365,1000.) ;
#12590=VECTOR('',#124368,1000.) ;
#12591=VECTOR('',#124369,1000.) ;
#12592=VECTOR('',#124370,1000.) ;
#12593=VECTOR('',#124371,1000.) ;
#12594=VECTOR('',#124374,1000.) ;
#12595=VECTOR('',#124375,1000.) ;
#12596=VECTOR('',#124376,1000.) ;
#12597=VECTOR('',#124377,1000.) ;
#12598=VECTOR('',#124380,1000.) ;
#12599=VECTOR('',#124381,1000.) ;
#12600=VECTOR('',#124382,1000.) ;
#12601=VECTOR('',#124383,1000.) ;
#12602=VECTOR('',#124390,1000.) ;
#12603=VECTOR('',#124391,1000.) ;
#12604=VECTOR('',#124392,1000.) ;
#12605=VECTOR('',#124393,1000.) ;
#12606=VECTOR('',#124396,1000.) ;
#12607=VECTOR('',#124397,1000.) ;
#12608=VECTOR('',#124398,1000.) ;
#12609=VECTOR('',#124401,1000.) ;
#12610=VECTOR('',#124402,1000.) ;
#12611=VECTOR('',#124403,1000.) ;
#12612=VECTOR('',#124404,1000.) ;
#12613=VECTOR('',#124407,1000.) ;
#12614=VECTOR('',#124412,1000.) ;
#12615=VECTOR('',#124413,1000.) ;
#12616=VECTOR('',#124414,1000.) ;
#12617=VECTOR('',#124417,1000.) ;
#12618=VECTOR('',#124418,1000.) ;
#12619=VECTOR('',#124419,1000.) ;
#12620=VECTOR('',#124422,1000.) ;
#12621=VECTOR('',#124423,1000.) ;
#12622=VECTOR('',#124424,1000.) ;
#12623=VECTOR('',#124425,1000.) ;
#12624=VECTOR('',#124432,1000.) ;
#12625=VECTOR('',#124433,1000.) ;
#12626=VECTOR('',#124434,1000.) ;
#12627=VECTOR('',#124435,1000.) ;
#12628=VECTOR('',#124438,1000.) ;
#12629=VECTOR('',#124439,1000.) ;
#12630=VECTOR('',#124440,1000.) ;
#12631=VECTOR('',#124443,1000.) ;
#12632=VECTOR('',#124444,1000.) ;
#12633=VECTOR('',#124445,1000.) ;
#12634=VECTOR('',#124446,1000.) ;
#12635=VECTOR('',#124449,1000.) ;
#12636=VECTOR('',#124454,1000.) ;
#12637=VECTOR('',#124455,1000.) ;
#12638=VECTOR('',#124456,1000.) ;
#12639=VECTOR('',#124459,1000.) ;
#12640=VECTOR('',#124460,1000.) ;
#12641=VECTOR('',#124461,1000.) ;
#12642=VECTOR('',#124464,1000.) ;
#12643=VECTOR('',#124465,1000.) ;
#12644=VECTOR('',#124466,1000.) ;
#12645=VECTOR('',#124467,1000.) ;
#12646=VECTOR('',#124474,1000.) ;
#12647=VECTOR('',#124475,1000.) ;
#12648=VECTOR('',#124476,1000.) ;
#12649=VECTOR('',#124477,1000.) ;
#12650=VECTOR('',#124480,1000.) ;
#12651=VECTOR('',#124481,1000.) ;
#12652=VECTOR('',#124482,1000.) ;
#12653=VECTOR('',#124485,1000.) ;
#12654=VECTOR('',#124486,1000.) ;
#12655=VECTOR('',#124487,1000.) ;
#12656=VECTOR('',#124488,1000.) ;
#12657=VECTOR('',#124491,1000.) ;
#12658=VECTOR('',#124496,1000.) ;
#12659=VECTOR('',#124497,1000.) ;
#12660=VECTOR('',#124498,1000.) ;
#12661=VECTOR('',#124501,1000.) ;
#12662=VECTOR('',#124502,1000.) ;
#12663=VECTOR('',#124503,1000.) ;
#12664=VECTOR('',#124506,1000.) ;
#12665=VECTOR('',#124507,1000.) ;
#12666=VECTOR('',#124508,1000.) ;
#12667=VECTOR('',#124509,1000.) ;
#12668=VECTOR('',#124516,1000.) ;
#12669=VECTOR('',#124517,1000.) ;
#12670=VECTOR('',#124518,1000.) ;
#12671=VECTOR('',#124519,1000.) ;
#12672=VECTOR('',#124522,1000.) ;
#12673=VECTOR('',#124523,1000.) ;
#12674=VECTOR('',#124524,1000.) ;
#12675=VECTOR('',#124527,1000.) ;
#12676=VECTOR('',#124528,1000.) ;
#12677=VECTOR('',#124529,1000.) ;
#12678=VECTOR('',#124530,1000.) ;
#12679=VECTOR('',#124533,1000.) ;
#12680=VECTOR('',#124538,1000.) ;
#12681=VECTOR('',#124539,1000.) ;
#12682=VECTOR('',#124540,1000.) ;
#12683=VECTOR('',#124543,1000.) ;
#12684=VECTOR('',#124544,1000.) ;
#12685=VECTOR('',#124545,1000.) ;
#12686=VECTOR('',#124548,1000.) ;
#12687=VECTOR('',#124549,1000.) ;
#12688=VECTOR('',#124550,1000.) ;
#12689=VECTOR('',#124551,1000.) ;
#12690=VECTOR('',#124558,1000.) ;
#12691=VECTOR('',#124559,1000.) ;
#12692=VECTOR('',#124560,1000.) ;
#12693=VECTOR('',#124561,1000.) ;
#12694=VECTOR('',#124564,1000.) ;
#12695=VECTOR('',#124565,1000.) ;
#12696=VECTOR('',#124566,1000.) ;
#12697=VECTOR('',#124569,1000.) ;
#12698=VECTOR('',#124570,1000.) ;
#12699=VECTOR('',#124571,1000.) ;
#12700=VECTOR('',#124572,1000.) ;
#12701=VECTOR('',#124575,1000.) ;
#12702=VECTOR('',#124580,1000.) ;
#12703=VECTOR('',#124581,1000.) ;
#12704=VECTOR('',#124582,1000.) ;
#12705=VECTOR('',#124585,1000.) ;
#12706=VECTOR('',#124586,1000.) ;
#12707=VECTOR('',#124587,1000.) ;
#12708=VECTOR('',#124590,1000.) ;
#12709=VECTOR('',#124591,1000.) ;
#12710=VECTOR('',#124592,1000.) ;
#12711=VECTOR('',#124593,1000.) ;
#12712=VECTOR('',#124600,1000.) ;
#12713=VECTOR('',#124601,1000.) ;
#12714=VECTOR('',#124602,1000.) ;
#12715=VECTOR('',#124603,1000.) ;
#12716=VECTOR('',#124606,1000.) ;
#12717=VECTOR('',#124607,1000.) ;
#12718=VECTOR('',#124608,1000.) ;
#12719=VECTOR('',#124611,1000.) ;
#12720=VECTOR('',#124612,1000.) ;
#12721=VECTOR('',#124613,1000.) ;
#12722=VECTOR('',#124614,1000.) ;
#12723=VECTOR('',#124617,1000.) ;
#12724=VECTOR('',#124622,1000.) ;
#12725=VECTOR('',#124623,1000.) ;
#12726=VECTOR('',#124624,1000.) ;
#12727=VECTOR('',#124627,1000.) ;
#12728=VECTOR('',#124628,1000.) ;
#12729=VECTOR('',#124629,1000.) ;
#12730=VECTOR('',#124632,1000.) ;
#12731=VECTOR('',#124633,1000.) ;
#12732=VECTOR('',#124634,1000.) ;
#12733=VECTOR('',#124635,1000.) ;
#12734=VECTOR('',#124642,1000.) ;
#12735=VECTOR('',#124643,1000.) ;
#12736=VECTOR('',#124644,1000.) ;
#12737=VECTOR('',#124645,1000.) ;
#12738=VECTOR('',#124648,1000.) ;
#12739=VECTOR('',#124649,1000.) ;
#12740=VECTOR('',#124650,1000.) ;
#12741=VECTOR('',#124653,1000.) ;
#12742=VECTOR('',#124654,1000.) ;
#12743=VECTOR('',#124655,1000.) ;
#12744=VECTOR('',#124656,1000.) ;
#12745=VECTOR('',#124659,1000.) ;
#12746=VECTOR('',#124664,1000.) ;
#12747=VECTOR('',#124665,1000.) ;
#12748=VECTOR('',#124666,1000.) ;
#12749=VECTOR('',#124669,1000.) ;
#12750=VECTOR('',#124670,1000.) ;
#12751=VECTOR('',#124671,1000.) ;
#12752=VECTOR('',#124674,1000.) ;
#12753=VECTOR('',#124675,1000.) ;
#12754=VECTOR('',#124676,1000.) ;
#12755=VECTOR('',#124677,1000.) ;
#12756=VECTOR('',#124684,1000.) ;
#12757=VECTOR('',#124685,1000.) ;
#12758=VECTOR('',#124686,1000.) ;
#12759=VECTOR('',#124687,1000.) ;
#12760=VECTOR('',#124690,1000.) ;
#12761=VECTOR('',#124691,1000.) ;
#12762=VECTOR('',#124692,1000.) ;
#12763=VECTOR('',#124695,1000.) ;
#12764=VECTOR('',#124696,1000.) ;
#12765=VECTOR('',#124697,1000.) ;
#12766=VECTOR('',#124698,1000.) ;
#12767=VECTOR('',#124701,1000.) ;
#12768=VECTOR('',#124706,1000.) ;
#12769=VECTOR('',#124707,1000.) ;
#12770=VECTOR('',#124708,1000.) ;
#12771=VECTOR('',#124711,1000.) ;
#12772=VECTOR('',#124712,1000.) ;
#12773=VECTOR('',#124713,1000.) ;
#12774=VECTOR('',#124716,1000.) ;
#12775=VECTOR('',#124717,1000.) ;
#12776=VECTOR('',#124718,1000.) ;
#12777=VECTOR('',#124719,1000.) ;
#12778=VECTOR('',#124726,1000.) ;
#12779=VECTOR('',#124727,1000.) ;
#12780=VECTOR('',#124728,1000.) ;
#12781=VECTOR('',#124729,1000.) ;
#12782=VECTOR('',#124732,1000.) ;
#12783=VECTOR('',#124733,1000.) ;
#12784=VECTOR('',#124734,1000.) ;
#12785=VECTOR('',#124737,1000.) ;
#12786=VECTOR('',#124738,1000.) ;
#12787=VECTOR('',#124739,1000.) ;
#12788=VECTOR('',#124740,1000.) ;
#12789=VECTOR('',#124743,1000.) ;
#12790=VECTOR('',#124748,1000.) ;
#12791=VECTOR('',#124749,1000.) ;
#12792=VECTOR('',#124750,1000.) ;
#12793=VECTOR('',#124753,1000.) ;
#12794=VECTOR('',#124754,1000.) ;
#12795=VECTOR('',#124755,1000.) ;
#12796=VECTOR('',#124758,1000.) ;
#12797=VECTOR('',#124759,1000.) ;
#12798=VECTOR('',#124760,1000.) ;
#12799=VECTOR('',#124761,1000.) ;
#12800=VECTOR('',#124764,1000.) ;
#12801=VECTOR('',#124765,1000.) ;
#12802=VECTOR('',#124766,1000.) ;
#12803=VECTOR('',#124767,1000.) ;
#12804=VECTOR('',#124770,1000.) ;
#12805=VECTOR('',#124771,1000.) ;
#12806=VECTOR('',#124772,1000.) ;
#12807=VECTOR('',#124773,1000.) ;
#12808=VECTOR('',#124776,1000.) ;
#12809=VECTOR('',#124779,1000.) ;
#12810=VECTOR('',#124784,1000.) ;
#12811=VECTOR('',#124787,1000.) ;
#12812=VECTOR('',#124788,1000.) ;
#12813=VECTOR('',#124789,1000.) ;
#12814=VECTOR('',#124790,1000.) ;
#12815=VECTOR('',#124793,1000.) ;
#12816=VECTOR('',#124794,1000.) ;
#12817=VECTOR('',#124795,1000.) ;
#12818=VECTOR('',#124796,1000.) ;
#12819=VECTOR('',#124799,1000.) ;
#12820=VECTOR('',#124800,1000.) ;
#12821=VECTOR('',#124801,1000.) ;
#12822=VECTOR('',#124802,1000.) ;
#12823=VECTOR('',#124805,1000.) ;
#12824=VECTOR('',#124808,1000.) ;
#12825=VECTOR('',#124813,1000.) ;
#12826=VECTOR('',#124816,1000.) ;
#12827=VECTOR('',#124817,1000.) ;
#12828=VECTOR('',#124818,1000.) ;
#12829=VECTOR('',#124819,1000.) ;
#12830=VECTOR('',#124822,1000.) ;
#12831=VECTOR('',#124823,1000.) ;
#12832=VECTOR('',#124824,1000.) ;
#12833=VECTOR('',#124825,1000.) ;
#12834=VECTOR('',#124828,1000.) ;
#12835=VECTOR('',#124829,1000.) ;
#12836=VECTOR('',#124830,1000.) ;
#12837=VECTOR('',#124831,1000.) ;
#12838=VECTOR('',#124834,1000.) ;
#12839=VECTOR('',#124837,1000.) ;
#12840=VECTOR('',#124842,1000.) ;
#12841=VECTOR('',#124845,1000.) ;
#12842=VECTOR('',#124846,1000.) ;
#12843=VECTOR('',#124847,1000.) ;
#12844=VECTOR('',#124848,1000.) ;
#12845=VECTOR('',#124851,1000.) ;
#12846=VECTOR('',#124852,1000.) ;
#12847=VECTOR('',#124853,1000.) ;
#12848=VECTOR('',#124854,1000.) ;
#12849=VECTOR('',#124857,1000.) ;
#12850=VECTOR('',#124858,1000.) ;
#12851=VECTOR('',#124859,1000.) ;
#12852=VECTOR('',#124860,1000.) ;
#12853=VECTOR('',#124863,1000.) ;
#12854=VECTOR('',#124866,1000.) ;
#12855=VECTOR('',#124871,1000.) ;
#12856=VECTOR('',#124874,1000.) ;
#12857=VECTOR('',#124875,1000.) ;
#12858=VECTOR('',#124876,1000.) ;
#12859=VECTOR('',#124877,1000.) ;
#12860=VECTOR('',#124880,1000.) ;
#12861=VECTOR('',#124881,1000.) ;
#12862=VECTOR('',#124882,1000.) ;
#12863=VECTOR('',#124883,1000.) ;
#12864=VECTOR('',#124886,1000.) ;
#12865=VECTOR('',#124887,1000.) ;
#12866=VECTOR('',#124888,1000.) ;
#12867=VECTOR('',#124889,1000.) ;
#12868=VECTOR('',#124892,1000.) ;
#12869=VECTOR('',#124895,1000.) ;
#12870=VECTOR('',#124900,1000.) ;
#12871=VECTOR('',#124903,1000.) ;
#12872=VECTOR('',#124904,1000.) ;
#12873=VECTOR('',#124905,1000.) ;
#12874=VECTOR('',#124906,1000.) ;
#12875=VECTOR('',#124909,1000.) ;
#12876=VECTOR('',#124910,1000.) ;
#12877=VECTOR('',#124911,1000.) ;
#12878=VECTOR('',#124912,1000.) ;
#12879=VECTOR('',#124915,1000.) ;
#12880=VECTOR('',#124916,1000.) ;
#12881=VECTOR('',#124917,1000.) ;
#12882=VECTOR('',#124918,1000.) ;
#12883=VECTOR('',#124921,1000.) ;
#12884=VECTOR('',#124924,1000.) ;
#12885=VECTOR('',#124929,1000.) ;
#12886=VECTOR('',#124932,1000.) ;
#12887=VECTOR('',#124933,1000.) ;
#12888=VECTOR('',#124934,1000.) ;
#12889=VECTOR('',#124935,1000.) ;
#12890=VECTOR('',#124938,1000.) ;
#12891=VECTOR('',#124939,1000.) ;
#12892=VECTOR('',#124940,1000.) ;
#12893=VECTOR('',#124941,1000.) ;
#12894=VECTOR('',#124944,1000.) ;
#12895=VECTOR('',#124945,1000.) ;
#12896=VECTOR('',#124946,1000.) ;
#12897=VECTOR('',#124947,1000.) ;
#12898=VECTOR('',#124950,1000.) ;
#12899=VECTOR('',#124953,1000.) ;
#12900=VECTOR('',#124958,1000.) ;
#12901=VECTOR('',#124961,1000.) ;
#12902=VECTOR('',#124962,1000.) ;
#12903=VECTOR('',#124963,1000.) ;
#12904=VECTOR('',#124964,1000.) ;
#12905=VECTOR('',#124967,1000.) ;
#12906=VECTOR('',#124968,1000.) ;
#12907=VECTOR('',#124969,1000.) ;
#12908=VECTOR('',#124970,1000.) ;
#12909=VECTOR('',#124973,1000.) ;
#12910=VECTOR('',#124974,1000.) ;
#12911=VECTOR('',#124975,1000.) ;
#12912=VECTOR('',#124976,1000.) ;
#12913=VECTOR('',#124979,1000.) ;
#12914=VECTOR('',#124982,1000.) ;
#12915=VECTOR('',#124987,1000.) ;
#12916=VECTOR('',#124990,1000.) ;
#12917=VECTOR('',#124991,1000.) ;
#12918=VECTOR('',#124992,1000.) ;
#12919=VECTOR('',#124993,1000.) ;
#12920=VECTOR('',#124996,1000.) ;
#12921=VECTOR('',#124997,1000.) ;
#12922=VECTOR('',#124998,1000.) ;
#12923=VECTOR('',#124999,1000.) ;
#12924=VECTOR('',#125002,1000.) ;
#12925=VECTOR('',#125003,1000.) ;
#12926=VECTOR('',#125004,1000.) ;
#12927=VECTOR('',#125005,1000.) ;
#12928=VECTOR('',#125008,1000.) ;
#12929=VECTOR('',#125011,1000.) ;
#12930=VECTOR('',#125016,1000.) ;
#12931=VECTOR('',#125019,1000.) ;
#12932=VECTOR('',#125020,1000.) ;
#12933=VECTOR('',#125021,1000.) ;
#12934=VECTOR('',#125022,1000.) ;
#12935=VECTOR('',#125043,1000.) ;
#12936=VECTOR('',#125044,1000.) ;
#12937=VECTOR('',#125045,1000.) ;
#12938=VECTOR('',#125046,1000.) ;
#12939=VECTOR('',#125049,1000.) ;
#12940=VECTOR('',#125050,1000.) ;
#12941=VECTOR('',#125051,1000.) ;
#12942=VECTOR('',#125052,1000.) ;
#12943=VECTOR('',#125055,1000.) ;
#12944=VECTOR('',#125056,1000.) ;
#12945=VECTOR('',#125057,1000.) ;
#12946=VECTOR('',#125058,1000.) ;
#12947=VECTOR('',#125061,1000.) ;
#12948=VECTOR('',#125062,1000.) ;
#12949=VECTOR('',#125063,1000.) ;
#12950=VECTOR('',#125064,1000.) ;
#12951=VECTOR('',#125067,1000.) ;
#12952=VECTOR('',#125068,1000.) ;
#12953=VECTOR('',#125069,1000.) ;
#12954=VECTOR('',#125070,1000.) ;
#12955=VECTOR('',#125073,1000.) ;
#12956=VECTOR('',#125074,1000.) ;
#12957=VECTOR('',#125075,1000.) ;
#12958=VECTOR('',#125076,1000.) ;
#12959=VECTOR('',#125079,1000.) ;
#12960=VECTOR('',#125080,1000.) ;
#12961=VECTOR('',#125081,1000.) ;
#12962=VECTOR('',#125082,1000.) ;
#12963=VECTOR('',#125085,1000.) ;
#12964=VECTOR('',#125086,1000.) ;
#12965=VECTOR('',#125087,1000.) ;
#12966=VECTOR('',#125088,1000.) ;
#12967=VECTOR('',#125091,1000.) ;
#12968=VECTOR('',#125092,1000.) ;
#12969=VECTOR('',#125093,1000.) ;
#12970=VECTOR('',#125094,1000.) ;
#12971=VECTOR('',#125097,1000.) ;
#12972=VECTOR('',#125098,1000.) ;
#12973=VECTOR('',#125099,1000.) ;
#12974=VECTOR('',#125100,1000.) ;
#12975=VECTOR('',#125103,1000.) ;
#12976=VECTOR('',#125104,1000.) ;
#12977=VECTOR('',#125105,1000.) ;
#12978=VECTOR('',#125106,1000.) ;
#12979=VECTOR('',#125109,1000.) ;
#12980=VECTOR('',#125110,1000.) ;
#12981=VECTOR('',#125111,1000.) ;
#12982=VECTOR('',#125112,1000.) ;
#12983=VECTOR('',#125115,1000.) ;
#12984=VECTOR('',#125116,1000.) ;
#12985=VECTOR('',#125117,1000.) ;
#12986=VECTOR('',#125118,1000.) ;
#12987=VECTOR('',#125121,1000.) ;
#12988=VECTOR('',#125122,1000.) ;
#12989=VECTOR('',#125123,1000.) ;
#12990=VECTOR('',#125124,1000.) ;
#12991=VECTOR('',#125127,1000.) ;
#12992=VECTOR('',#125128,1000.) ;
#12993=VECTOR('',#125129,1000.) ;
#12994=VECTOR('',#125130,1000.) ;
#12995=VECTOR('',#125133,1000.) ;
#12996=VECTOR('',#125134,1000.) ;
#12997=VECTOR('',#125135,1000.) ;
#12998=VECTOR('',#125136,1000.) ;
#12999=VECTOR('',#125139,1000.) ;
#13000=VECTOR('',#125140,1000.) ;
#13001=VECTOR('',#125141,1000.) ;
#13002=VECTOR('',#125142,1000.) ;
#13003=VECTOR('',#125145,1000.) ;
#13004=VECTOR('',#125146,1000.) ;
#13005=VECTOR('',#125147,1000.) ;
#13006=VECTOR('',#125148,1000.) ;
#13007=VECTOR('',#125151,1000.) ;
#13008=VECTOR('',#125152,1000.) ;
#13009=VECTOR('',#125153,1000.) ;
#13010=VECTOR('',#125154,1000.) ;
#13011=VECTOR('',#125157,1000.) ;
#13012=VECTOR('',#125158,1000.) ;
#13013=VECTOR('',#125159,1000.) ;
#13014=VECTOR('',#125160,1000.) ;
#13015=VECTOR('',#125163,1000.) ;
#13016=VECTOR('',#125164,1000.) ;
#13017=VECTOR('',#125165,1000.) ;
#13018=VECTOR('',#125166,1000.) ;
#13019=VECTOR('',#125169,1000.) ;
#13020=VECTOR('',#125170,1000.) ;
#13021=VECTOR('',#125171,1000.) ;
#13022=VECTOR('',#125172,1000.) ;
#13023=VECTOR('',#125175,1000.) ;
#13024=VECTOR('',#125176,1000.) ;
#13025=VECTOR('',#125177,1000.) ;
#13026=VECTOR('',#125178,1000.) ;
#13027=VECTOR('',#125181,1000.) ;
#13028=VECTOR('',#125182,1000.) ;
#13029=VECTOR('',#125183,1000.) ;
#13030=VECTOR('',#125184,1000.) ;
#13031=VECTOR('',#125187,1000.) ;
#13032=VECTOR('',#125188,1000.) ;
#13033=VECTOR('',#125189,1000.) ;
#13034=VECTOR('',#125190,1000.) ;
#13035=VECTOR('',#125193,1000.) ;
#13036=VECTOR('',#125194,1000.) ;
#13037=VECTOR('',#125195,1000.) ;
#13038=VECTOR('',#125196,1000.) ;
#13039=VECTOR('',#125199,1000.) ;
#13040=VECTOR('',#125200,1000.) ;
#13041=VECTOR('',#125201,1000.) ;
#13042=VECTOR('',#125202,1000.) ;
#13043=VECTOR('',#125205,1000.) ;
#13044=VECTOR('',#125206,1000.) ;
#13045=VECTOR('',#125207,1000.) ;
#13046=VECTOR('',#125208,1000.) ;
#13047=VECTOR('',#125211,1000.) ;
#13048=VECTOR('',#125212,1000.) ;
#13049=VECTOR('',#125213,1000.) ;
#13050=VECTOR('',#125214,1000.) ;
#13051=VECTOR('',#125217,1000.) ;
#13052=VECTOR('',#125218,1000.) ;
#13053=VECTOR('',#125219,1000.) ;
#13054=VECTOR('',#125220,1000.) ;
#13055=VECTOR('',#125223,1000.) ;
#13056=VECTOR('',#125224,1000.) ;
#13057=VECTOR('',#125225,1000.) ;
#13058=VECTOR('',#125226,1000.) ;
#13059=VECTOR('',#125229,1000.) ;
#13060=VECTOR('',#125230,1000.) ;
#13061=VECTOR('',#125231,1000.) ;
#13062=VECTOR('',#125232,1000.) ;
#13063=VECTOR('',#125235,1000.) ;
#13064=VECTOR('',#125236,1000.) ;
#13065=VECTOR('',#125237,1000.) ;
#13066=VECTOR('',#125238,1000.) ;
#13067=VECTOR('',#125241,1000.) ;
#13068=VECTOR('',#125242,1000.) ;
#13069=VECTOR('',#125243,1000.) ;
#13070=VECTOR('',#125244,1000.) ;
#13071=VECTOR('',#125247,1000.) ;
#13072=VECTOR('',#125248,1000.) ;
#13073=VECTOR('',#125249,1000.) ;
#13074=VECTOR('',#125250,1000.) ;
#13075=VECTOR('',#125253,1000.) ;
#13076=VECTOR('',#125254,1000.) ;
#13077=VECTOR('',#125255,1000.) ;
#13078=VECTOR('',#125256,1000.) ;
#13079=VECTOR('',#125259,1000.) ;
#13080=VECTOR('',#125260,1000.) ;
#13081=VECTOR('',#125261,1000.) ;
#13082=VECTOR('',#125262,1000.) ;
#13083=VECTOR('',#125263,1000.) ;
#13084=VECTOR('',#125266,1000.) ;
#13085=VECTOR('',#125269,1000.) ;
#13086=VECTOR('',#125272,1000.) ;
#13087=VECTOR('',#125277,1000.) ;
#13088=VECTOR('',#125278,1000.) ;
#13089=VECTOR('',#125279,1000.) ;
#13090=VECTOR('',#125282,1000.) ;
#13091=VECTOR('',#125283,1000.) ;
#13092=VECTOR('',#125284,1000.) ;
#13093=VECTOR('',#125287,1000.) ;
#13094=VECTOR('',#125288,1000.) ;
#13095=VECTOR('',#125289,1000.) ;
#13096=VECTOR('',#125292,1000.) ;
#13097=VECTOR('',#125293,1000.) ;
#13098=VECTOR('',#125294,1000.) ;
#13099=VECTOR('',#125297,1000.) ;
#13100=VECTOR('',#125298,1000.) ;
#13101=VECTOR('',#125299,1000.) ;
#13102=VECTOR('',#125300,1000.) ;
#13103=VECTOR('',#125301,1000.) ;
#13104=VECTOR('',#125304,1000.) ;
#13105=VECTOR('',#125307,1000.) ;
#13106=VECTOR('',#125310,1000.) ;
#13107=VECTOR('',#125315,1000.) ;
#13108=VECTOR('',#125316,1000.) ;
#13109=VECTOR('',#125317,1000.) ;
#13110=VECTOR('',#125320,1000.) ;
#13111=VECTOR('',#125321,1000.) ;
#13112=VECTOR('',#125322,1000.) ;
#13113=VECTOR('',#125325,1000.) ;
#13114=VECTOR('',#125326,1000.) ;
#13115=VECTOR('',#125327,1000.) ;
#13116=VECTOR('',#125330,1000.) ;
#13117=VECTOR('',#125331,1000.) ;
#13118=VECTOR('',#125332,1000.) ;
#13119=VECTOR('',#125335,1000.) ;
#13120=VECTOR('',#125336,1000.) ;
#13121=VECTOR('',#125337,1000.) ;
#13122=VECTOR('',#125338,1000.) ;
#13123=VECTOR('',#125339,1000.) ;
#13124=VECTOR('',#125342,1000.) ;
#13125=VECTOR('',#125345,1000.) ;
#13126=VECTOR('',#125348,1000.) ;
#13127=VECTOR('',#125353,1000.) ;
#13128=VECTOR('',#125354,1000.) ;
#13129=VECTOR('',#125355,1000.) ;
#13130=VECTOR('',#125358,1000.) ;
#13131=VECTOR('',#125359,1000.) ;
#13132=VECTOR('',#125360,1000.) ;
#13133=VECTOR('',#125363,1000.) ;
#13134=VECTOR('',#125364,1000.) ;
#13135=VECTOR('',#125365,1000.) ;
#13136=VECTOR('',#125368,1000.) ;
#13137=VECTOR('',#125369,1000.) ;
#13138=VECTOR('',#125370,1000.) ;
#13139=VECTOR('',#125373,1000.) ;
#13140=VECTOR('',#125374,1000.) ;
#13141=VECTOR('',#125375,1000.) ;
#13142=VECTOR('',#125376,1000.) ;
#13143=VECTOR('',#125377,1000.) ;
#13144=VECTOR('',#125380,1000.) ;
#13145=VECTOR('',#125383,1000.) ;
#13146=VECTOR('',#125386,1000.) ;
#13147=VECTOR('',#125391,1000.) ;
#13148=VECTOR('',#125392,1000.) ;
#13149=VECTOR('',#125393,1000.) ;
#13150=VECTOR('',#125396,1000.) ;
#13151=VECTOR('',#125397,1000.) ;
#13152=VECTOR('',#125398,1000.) ;
#13153=VECTOR('',#125401,1000.) ;
#13154=VECTOR('',#125402,1000.) ;
#13155=VECTOR('',#125403,1000.) ;
#13156=VECTOR('',#125406,1000.) ;
#13157=VECTOR('',#125407,1000.) ;
#13158=VECTOR('',#125408,1000.) ;
#13159=VECTOR('',#125411,1000.) ;
#13160=VECTOR('',#125412,1000.) ;
#13161=VECTOR('',#125413,1000.) ;
#13162=VECTOR('',#125414,1000.) ;
#13163=VECTOR('',#125415,1000.) ;
#13164=VECTOR('',#125418,1000.) ;
#13165=VECTOR('',#125421,1000.) ;
#13166=VECTOR('',#125424,1000.) ;
#13167=VECTOR('',#125429,1000.) ;
#13168=VECTOR('',#125430,1000.) ;
#13169=VECTOR('',#125431,1000.) ;
#13170=VECTOR('',#125434,1000.) ;
#13171=VECTOR('',#125435,1000.) ;
#13172=VECTOR('',#125436,1000.) ;
#13173=VECTOR('',#125439,1000.) ;
#13174=VECTOR('',#125440,1000.) ;
#13175=VECTOR('',#125441,1000.) ;
#13176=VECTOR('',#125444,1000.) ;
#13177=VECTOR('',#125445,1000.) ;
#13178=VECTOR('',#125446,1000.) ;
#13179=VECTOR('',#125449,1000.) ;
#13180=VECTOR('',#125450,1000.) ;
#13181=VECTOR('',#125451,1000.) ;
#13182=VECTOR('',#125452,1000.) ;
#13183=VECTOR('',#125453,1000.) ;
#13184=VECTOR('',#125456,1000.) ;
#13185=VECTOR('',#125459,1000.) ;
#13186=VECTOR('',#125462,1000.) ;
#13187=VECTOR('',#125467,1000.) ;
#13188=VECTOR('',#125468,1000.) ;
#13189=VECTOR('',#125469,1000.) ;
#13190=VECTOR('',#125472,1000.) ;
#13191=VECTOR('',#125473,1000.) ;
#13192=VECTOR('',#125474,1000.) ;
#13193=VECTOR('',#125477,1000.) ;
#13194=VECTOR('',#125478,1000.) ;
#13195=VECTOR('',#125479,1000.) ;
#13196=VECTOR('',#125482,1000.) ;
#13197=VECTOR('',#125483,1000.) ;
#13198=VECTOR('',#125484,1000.) ;
#13199=VECTOR('',#125487,1000.) ;
#13200=VECTOR('',#125488,1000.) ;
#13201=VECTOR('',#125489,1000.) ;
#13202=VECTOR('',#125490,1000.) ;
#13203=VECTOR('',#125491,1000.) ;
#13204=VECTOR('',#125494,1000.) ;
#13205=VECTOR('',#125497,1000.) ;
#13206=VECTOR('',#125500,1000.) ;
#13207=VECTOR('',#125505,1000.) ;
#13208=VECTOR('',#125506,1000.) ;
#13209=VECTOR('',#125507,1000.) ;
#13210=VECTOR('',#125510,1000.) ;
#13211=VECTOR('',#125511,1000.) ;
#13212=VECTOR('',#125512,1000.) ;
#13213=VECTOR('',#125515,1000.) ;
#13214=VECTOR('',#125516,1000.) ;
#13215=VECTOR('',#125517,1000.) ;
#13216=VECTOR('',#125520,1000.) ;
#13217=VECTOR('',#125521,1000.) ;
#13218=VECTOR('',#125522,1000.) ;
#13219=VECTOR('',#125525,1000.) ;
#13220=VECTOR('',#125526,1000.) ;
#13221=VECTOR('',#125527,1000.) ;
#13222=VECTOR('',#125528,1000.) ;
#13223=VECTOR('',#125529,1000.) ;
#13224=VECTOR('',#125532,1000.) ;
#13225=VECTOR('',#125535,1000.) ;
#13226=VECTOR('',#125538,1000.) ;
#13227=VECTOR('',#125543,1000.) ;
#13228=VECTOR('',#125544,1000.) ;
#13229=VECTOR('',#125545,1000.) ;
#13230=VECTOR('',#125548,1000.) ;
#13231=VECTOR('',#125549,1000.) ;
#13232=VECTOR('',#125550,1000.) ;
#13233=VECTOR('',#125553,1000.) ;
#13234=VECTOR('',#125554,1000.) ;
#13235=VECTOR('',#125555,1000.) ;
#13236=VECTOR('',#125558,1000.) ;
#13237=VECTOR('',#125559,1000.) ;
#13238=VECTOR('',#125560,1000.) ;
#13239=VECTOR('',#125563,1000.) ;
#13240=VECTOR('',#125564,1000.) ;
#13241=VECTOR('',#125565,1000.) ;
#13242=VECTOR('',#125566,1000.) ;
#13243=VECTOR('',#125567,1000.) ;
#13244=VECTOR('',#125570,1000.) ;
#13245=VECTOR('',#125573,1000.) ;
#13246=VECTOR('',#125576,1000.) ;
#13247=VECTOR('',#125581,1000.) ;
#13248=VECTOR('',#125582,1000.) ;
#13249=VECTOR('',#125583,1000.) ;
#13250=VECTOR('',#125586,1000.) ;
#13251=VECTOR('',#125587,1000.) ;
#13252=VECTOR('',#125588,1000.) ;
#13253=VECTOR('',#125591,1000.) ;
#13254=VECTOR('',#125592,1000.) ;
#13255=VECTOR('',#125593,1000.) ;
#13256=VECTOR('',#125596,1000.) ;
#13257=VECTOR('',#125597,1000.) ;
#13258=VECTOR('',#125598,1000.) ;
#13259=VECTOR('',#125601,1000.) ;
#13260=VECTOR('',#125602,1000.) ;
#13261=VECTOR('',#125603,1000.) ;
#13262=VECTOR('',#125604,1000.) ;
#13263=VECTOR('',#125607,1000.) ;
#13264=VECTOR('',#125608,1000.) ;
#13265=VECTOR('',#125609,1000.) ;
#13266=VECTOR('',#125610,1000.) ;
#13267=VECTOR('',#125613,1000.) ;
#13268=VECTOR('',#125614,1000.) ;
#13269=VECTOR('',#125615,1000.) ;
#13270=VECTOR('',#125616,1000.) ;
#13271=VECTOR('',#125619,1000.) ;
#13272=VECTOR('',#125620,1000.) ;
#13273=VECTOR('',#125621,1000.) ;
#13274=VECTOR('',#125622,1000.) ;
#13275=VECTOR('',#125625,1000.) ;
#13276=VECTOR('',#125626,1000.) ;
#13277=VECTOR('',#125627,1000.) ;
#13278=VECTOR('',#125628,1000.) ;
#13279=VECTOR('',#125631,1000.) ;
#13280=VECTOR('',#125632,1000.) ;
#13281=VECTOR('',#125633,1000.) ;
#13282=VECTOR('',#125634,1000.) ;
#13283=VECTOR('',#125637,1000.) ;
#13284=VECTOR('',#125638,1000.) ;
#13285=VECTOR('',#125639,1000.) ;
#13286=VECTOR('',#125640,1000.) ;
#13287=VECTOR('',#125643,1000.) ;
#13288=VECTOR('',#125644,1000.) ;
#13289=VECTOR('',#125645,1000.) ;
#13290=VECTOR('',#125646,1000.) ;
#13291=VECTOR('',#125649,1000.) ;
#13292=VECTOR('',#125650,1000.) ;
#13293=VECTOR('',#125651,1000.) ;
#13294=VECTOR('',#125652,1000.) ;
#13295=VECTOR('',#125655,1000.) ;
#13296=VECTOR('',#125658,1000.) ;
#13297=VECTOR('',#125661,1000.) ;
#13298=VECTOR('',#125664,1000.) ;
#13299=VECTOR('',#125667,1000.) ;
#13300=VECTOR('',#125670,1000.) ;
#13301=VECTOR('',#125673,1000.) ;
#13302=VECTOR('',#125676,1000.) ;
#13303=VECTOR('',#125679,1000.) ;
#13304=VECTOR('',#125682,1000.) ;
#13305=VECTOR('',#125683,1000.) ;
#13306=VECTOR('',#125686,1000.) ;
#13307=VECTOR('',#125687,1000.) ;
#13308=VECTOR('',#125690,1000.) ;
#13309=VECTOR('',#125691,1000.) ;
#13310=VECTOR('',#125694,1000.) ;
#13311=VECTOR('',#125695,1000.) ;
#13312=VECTOR('',#125698,1000.) ;
#13313=VECTOR('',#125699,1000.) ;
#13314=VECTOR('',#125702,1000.) ;
#13315=VECTOR('',#125703,1000.) ;
#13316=VECTOR('',#125706,1000.) ;
#13317=VECTOR('',#125707,1000.) ;
#13318=VECTOR('',#125710,1000.) ;
#13319=VECTOR('',#125711,1000.) ;
#13320=VECTOR('',#125714,1000.) ;
#13321=VECTOR('',#125715,1000.) ;
#13322=VECTOR('',#125718,1000.) ;
#13323=VECTOR('',#125719,1000.) ;
#13324=VECTOR('',#125722,1000.) ;
#13325=VECTOR('',#125723,1000.) ;
#13326=VECTOR('',#125726,1000.) ;
#13327=VECTOR('',#125727,1000.) ;
#13328=VECTOR('',#125730,1000.) ;
#13329=VECTOR('',#125731,1000.) ;
#13330=VECTOR('',#125734,1000.) ;
#13331=VECTOR('',#125735,1000.) ;
#13332=VECTOR('',#125738,1000.) ;
#13333=VECTOR('',#125739,1000.) ;
#13334=VECTOR('',#125742,1000.) ;
#13335=VECTOR('',#125743,1000.) ;
#13336=VECTOR('',#125746,1000.) ;
#13337=VECTOR('',#125747,1000.) ;
#13338=VECTOR('',#125750,1000.) ;
#13339=VECTOR('',#125751,1000.) ;
#13340=VECTOR('',#125754,1000.) ;
#13341=VECTOR('',#125755,1000.) ;
#13342=VECTOR('',#125758,1000.) ;
#13343=VECTOR('',#125759,1000.) ;
#13344=VECTOR('',#125762,1000.) ;
#13345=VECTOR('',#125763,1000.) ;
#13346=VECTOR('',#125766,1000.) ;
#13347=VECTOR('',#125767,1000.) ;
#13348=VECTOR('',#125770,1000.) ;
#13349=VECTOR('',#125771,1000.) ;
#13350=VECTOR('',#125774,1000.) ;
#13351=VECTOR('',#125775,1000.) ;
#13352=VECTOR('',#125778,1000.) ;
#13353=VECTOR('',#125779,1000.) ;
#13354=VECTOR('',#125782,1000.) ;
#13355=VECTOR('',#125783,1000.) ;
#13356=VECTOR('',#125786,1000.) ;
#13357=VECTOR('',#125787,1000.) ;
#13358=VECTOR('',#125790,1000.) ;
#13359=VECTOR('',#125793,1000.) ;
#13360=VECTOR('',#125798,1000.) ;
#13361=VECTOR('',#125799,1000.) ;
#13362=VECTOR('',#125800,1000.) ;
#13363=VECTOR('',#125805,1000.) ;
#13364=VECTOR('',#125810,1000.) ;
#13365=VECTOR('',#125811,1000.) ;
#13366=VECTOR('',#125812,1000.) ;
#13367=VECTOR('',#125817,1000.) ;
#13368=VECTOR('',#125822,1000.) ;
#13369=VECTOR('',#125823,1000.) ;
#13370=VECTOR('',#125824,1000.) ;
#13371=VECTOR('',#125829,1000.) ;
#13372=VECTOR('',#125834,1000.) ;
#13373=VECTOR('',#125835,1000.) ;
#13374=VECTOR('',#125838,1000.) ;
#13375=VECTOR('',#125839,1000.) ;
#13376=VECTOR('',#125840,1000.) ;
#13377=VECTOR('',#125841,1000.) ;
#13378=VECTOR('',#125844,1000.) ;
#13379=VECTOR('',#125847,1000.) ;
#13380=VECTOR('',#125852,1000.) ;
#13381=VECTOR('',#125853,1000.) ;
#13382=VECTOR('',#125854,1000.) ;
#13383=VECTOR('',#125859,1000.) ;
#13384=VECTOR('',#125864,1000.) ;
#13385=VECTOR('',#125865,1000.) ;
#13386=VECTOR('',#125866,1000.) ;
#13387=VECTOR('',#125871,1000.) ;
#13388=VECTOR('',#125876,1000.) ;
#13389=VECTOR('',#125877,1000.) ;
#13390=VECTOR('',#125878,1000.) ;
#13391=VECTOR('',#125883,1000.) ;
#13392=VECTOR('',#125888,1000.) ;
#13393=VECTOR('',#125889,1000.) ;
#13394=VECTOR('',#125892,1000.) ;
#13395=VECTOR('',#125893,1000.) ;
#13396=VECTOR('',#125894,1000.) ;
#13397=VECTOR('',#125895,1000.) ;
#13398=VECTOR('',#125898,1000.) ;
#13399=VECTOR('',#125901,1000.) ;
#13400=VECTOR('',#125906,1000.) ;
#13401=VECTOR('',#125907,1000.) ;
#13402=VECTOR('',#125908,1000.) ;
#13403=VECTOR('',#125913,1000.) ;
#13404=VECTOR('',#125918,1000.) ;
#13405=VECTOR('',#125919,1000.) ;
#13406=VECTOR('',#125920,1000.) ;
#13407=VECTOR('',#125925,1000.) ;
#13408=VECTOR('',#125930,1000.) ;
#13409=VECTOR('',#125931,1000.) ;
#13410=VECTOR('',#125932,1000.) ;
#13411=VECTOR('',#125937,1000.) ;
#13412=VECTOR('',#125942,1000.) ;
#13413=VECTOR('',#125943,1000.) ;
#13414=VECTOR('',#125946,1000.) ;
#13415=VECTOR('',#125947,1000.) ;
#13416=VECTOR('',#125948,1000.) ;
#13417=VECTOR('',#125949,1000.) ;
#13418=VECTOR('',#125952,1000.) ;
#13419=VECTOR('',#125955,1000.) ;
#13420=VECTOR('',#125960,1000.) ;
#13421=VECTOR('',#125961,1000.) ;
#13422=VECTOR('',#125962,1000.) ;
#13423=VECTOR('',#125967,1000.) ;
#13424=VECTOR('',#125972,1000.) ;
#13425=VECTOR('',#125973,1000.) ;
#13426=VECTOR('',#125974,1000.) ;
#13427=VECTOR('',#125979,1000.) ;
#13428=VECTOR('',#125984,1000.) ;
#13429=VECTOR('',#125985,1000.) ;
#13430=VECTOR('',#125986,1000.) ;
#13431=VECTOR('',#125991,1000.) ;
#13432=VECTOR('',#125996,1000.) ;
#13433=VECTOR('',#125997,1000.) ;
#13434=VECTOR('',#126000,1000.) ;
#13435=VECTOR('',#126001,1000.) ;
#13436=VECTOR('',#126002,1000.) ;
#13437=VECTOR('',#126003,1000.) ;
#13438=VECTOR('',#126006,1000.) ;
#13439=VECTOR('',#126009,1000.) ;
#13440=VECTOR('',#126014,1000.) ;
#13441=VECTOR('',#126015,1000.) ;
#13442=VECTOR('',#126016,1000.) ;
#13443=VECTOR('',#126021,1000.) ;
#13444=VECTOR('',#126026,1000.) ;
#13445=VECTOR('',#126027,1000.) ;
#13446=VECTOR('',#126028,1000.) ;
#13447=VECTOR('',#126033,1000.) ;
#13448=VECTOR('',#126038,1000.) ;
#13449=VECTOR('',#126039,1000.) ;
#13450=VECTOR('',#126040,1000.) ;
#13451=VECTOR('',#126045,1000.) ;
#13452=VECTOR('',#126050,1000.) ;
#13453=VECTOR('',#126051,1000.) ;
#13454=VECTOR('',#126054,1000.) ;
#13455=VECTOR('',#126055,1000.) ;
#13456=VECTOR('',#126056,1000.) ;
#13457=VECTOR('',#126057,1000.) ;
#13458=VECTOR('',#126060,1000.) ;
#13459=VECTOR('',#126063,1000.) ;
#13460=VECTOR('',#126068,1000.) ;
#13461=VECTOR('',#126069,1000.) ;
#13462=VECTOR('',#126070,1000.) ;
#13463=VECTOR('',#126075,1000.) ;
#13464=VECTOR('',#126080,1000.) ;
#13465=VECTOR('',#126081,1000.) ;
#13466=VECTOR('',#126082,1000.) ;
#13467=VECTOR('',#126087,1000.) ;
#13468=VECTOR('',#126092,1000.) ;
#13469=VECTOR('',#126093,1000.) ;
#13470=VECTOR('',#126094,1000.) ;
#13471=VECTOR('',#126099,1000.) ;
#13472=VECTOR('',#126104,1000.) ;
#13473=VECTOR('',#126105,1000.) ;
#13474=VECTOR('',#126108,1000.) ;
#13475=VECTOR('',#126109,1000.) ;
#13476=VECTOR('',#126110,1000.) ;
#13477=VECTOR('',#126111,1000.) ;
#13478=VECTOR('',#126114,1000.) ;
#13479=VECTOR('',#126117,1000.) ;
#13480=VECTOR('',#126122,1000.) ;
#13481=VECTOR('',#126123,1000.) ;
#13482=VECTOR('',#126124,1000.) ;
#13483=VECTOR('',#126129,1000.) ;
#13484=VECTOR('',#126134,1000.) ;
#13485=VECTOR('',#126135,1000.) ;
#13486=VECTOR('',#126136,1000.) ;
#13487=VECTOR('',#126141,1000.) ;
#13488=VECTOR('',#126146,1000.) ;
#13489=VECTOR('',#126147,1000.) ;
#13490=VECTOR('',#126148,1000.) ;
#13491=VECTOR('',#126153,1000.) ;
#13492=VECTOR('',#126158,1000.) ;
#13493=VECTOR('',#126159,1000.) ;
#13494=VECTOR('',#126162,1000.) ;
#13495=VECTOR('',#126163,1000.) ;
#13496=VECTOR('',#126164,1000.) ;
#13497=VECTOR('',#126165,1000.) ;
#13498=VECTOR('',#126168,1000.) ;
#13499=VECTOR('',#126171,1000.) ;
#13500=VECTOR('',#126176,1000.) ;
#13501=VECTOR('',#126177,1000.) ;
#13502=VECTOR('',#126178,1000.) ;
#13503=VECTOR('',#126183,1000.) ;
#13504=VECTOR('',#126188,1000.) ;
#13505=VECTOR('',#126189,1000.) ;
#13506=VECTOR('',#126190,1000.) ;
#13507=VECTOR('',#126195,1000.) ;
#13508=VECTOR('',#126200,1000.) ;
#13509=VECTOR('',#126201,1000.) ;
#13510=VECTOR('',#126202,1000.) ;
#13511=VECTOR('',#126207,1000.) ;
#13512=VECTOR('',#126212,1000.) ;
#13513=VECTOR('',#126213,1000.) ;
#13514=VECTOR('',#126216,1000.) ;
#13515=VECTOR('',#126217,1000.) ;
#13516=VECTOR('',#126218,1000.) ;
#13517=VECTOR('',#126219,1000.) ;
#13518=VECTOR('',#126222,1000.) ;
#13519=VECTOR('',#126225,1000.) ;
#13520=VECTOR('',#126230,1000.) ;
#13521=VECTOR('',#126231,1000.) ;
#13522=VECTOR('',#126232,1000.) ;
#13523=VECTOR('',#126237,1000.) ;
#13524=VECTOR('',#126242,1000.) ;
#13525=VECTOR('',#126243,1000.) ;
#13526=VECTOR('',#126244,1000.) ;
#13527=VECTOR('',#126249,1000.) ;
#13528=VECTOR('',#126254,1000.) ;
#13529=VECTOR('',#126255,1000.) ;
#13530=VECTOR('',#126256,1000.) ;
#13531=VECTOR('',#126261,1000.) ;
#13532=VECTOR('',#126266,1000.) ;
#13533=VECTOR('',#126267,1000.) ;
#13534=VECTOR('',#126270,1000.) ;
#13535=VECTOR('',#126271,1000.) ;
#13536=VECTOR('',#126272,1000.) ;
#13537=VECTOR('',#126273,1000.) ;
#15100=CYLINDRICAL_SURFACE('',#98152,0.0999999999999998) ;
#15101=CYLINDRICAL_SURFACE('',#98240,0.0645125000000003) ;
#15102=CYLINDRICAL_SURFACE('',#98242,0.0645125000000003) ;
#15103=CYLINDRICAL_SURFACE('',#98244,0.0645125000000003) ;
#15104=CYLINDRICAL_SURFACE('',#98246,0.0645125000000003) ;
#15105=CYLINDRICAL_SURFACE('',#98248,0.0645125000000003) ;
#15106=CYLINDRICAL_SURFACE('',#98250,0.0645125000000003) ;
#15107=CYLINDRICAL_SURFACE('',#98252,0.0645125000000003) ;
#15108=CYLINDRICAL_SURFACE('',#98362,1.5) ;
#15109=CYLINDRICAL_SURFACE('',#98368,1.5) ;
#15110=CYLINDRICAL_SURFACE('',#98374,1.5) ;
#15111=CYLINDRICAL_SURFACE('',#98380,1.5) ;
#15112=CYLINDRICAL_SURFACE('',#98386,1.5) ;
#15113=CYLINDRICAL_SURFACE('',#98392,1.5) ;
#15114=CYLINDRICAL_SURFACE('',#98398,1.5) ;
#15115=CYLINDRICAL_SURFACE('',#98404,1.5) ;
#15116=CYLINDRICAL_SURFACE('',#98410,1.5) ;
#15117=CYLINDRICAL_SURFACE('',#98434,1.) ;
#15118=CYLINDRICAL_SURFACE('',#98435,0.999999999999999) ;
#15119=CYLINDRICAL_SURFACE('',#98436,1.) ;
#15120=CYLINDRICAL_SURFACE('',#98437,1.) ;
#15121=CYLINDRICAL_SURFACE('',#98438,1.) ;
#15122=CYLINDRICAL_SURFACE('',#98439,1.) ;
#15123=CYLINDRICAL_SURFACE('',#98440,1.) ;
#15124=CYLINDRICAL_SURFACE('',#98441,1.) ;
#15125=CYLINDRICAL_SURFACE('',#98442,1.) ;
#15126=CYLINDRICAL_SURFACE('',#98455,0.0645125000000055) ;
#15127=CYLINDRICAL_SURFACE('',#98457,0.0645125000000061) ;
#15128=CYLINDRICAL_SURFACE('',#98459,0.0645124999999998) ;
#15129=CYLINDRICAL_SURFACE('',#98461,0.0645125000000003) ;
#15130=CYLINDRICAL_SURFACE('',#98463,1.5) ;
#15131=CYLINDRICAL_SURFACE('',#98471,1.) ;
#15132=CYLINDRICAL_SURFACE('',#98676,0.0999999999999998) ;
#15133=CYLINDRICAL_SURFACE('',#98679,0.0999999999999998) ;
#15134=CYLINDRICAL_SURFACE('',#98757,1.65625) ;
#15135=CYLINDRICAL_SURFACE('',#98781,2.25) ;
#15136=CYLINDRICAL_SURFACE('',#98783,2.25) ;
#15137=CYLINDRICAL_SURFACE('',#98787,2.25) ;
#15138=CYLINDRICAL_SURFACE('',#98789,2.25) ;
#15139=CYLINDRICAL_SURFACE('',#98791,0.0999999999999997) ;
#15140=CYLINDRICAL_SURFACE('',#98795,0.1) ;
#15141=CYLINDRICAL_SURFACE('',#98799,0.1) ;
#15142=CYLINDRICAL_SURFACE('',#98803,0.0999999999999997) ;
#15143=CYLINDRICAL_SURFACE('',#98808,0.0999999999999998) ;
#15144=CYLINDRICAL_SURFACE('',#98814,0.0999999999999998) ;
#15145=CYLINDRICAL_SURFACE('',#98817,0.1) ;
#15146=CYLINDRICAL_SURFACE('',#98819,0.1) ;
#15147=CYLINDRICAL_SURFACE('',#98821,0.100000000000003) ;
#15148=CYLINDRICAL_SURFACE('',#98824,0.0999999999999998) ;
#15149=CYLINDRICAL_SURFACE('',#98827,0.0999999999999998) ;
#15150=CYLINDRICAL_SURFACE('',#98836,0.0999999999999998) ;
#15151=CYLINDRICAL_SURFACE('',#98842,0.1) ;
#15152=CYLINDRICAL_SURFACE('',#98847,0.0999999999999998) ;
#15153=CYLINDRICAL_SURFACE('',#98849,0.1) ;
#15154=CYLINDRICAL_SURFACE('',#98851,0.1) ;
#15155=CYLINDRICAL_SURFACE('',#98853,0.100000000000003) ;
#15156=CYLINDRICAL_SURFACE('',#98856,0.0999999999999998) ;
#15157=CYLINDRICAL_SURFACE('',#98865,0.1) ;
#15158=CYLINDRICAL_SURFACE('',#98867,0.100000000000003) ;
#15159=CYLINDRICAL_SURFACE('',#98869,0.100000000000003) ;
#15160=CYLINDRICAL_SURFACE('',#98874,0.1) ;
#15161=CYLINDRICAL_SURFACE('',#98884,0.1) ;
#15162=CYLINDRICAL_SURFACE('',#98886,0.0999999999999994) ;
#15163=CYLINDRICAL_SURFACE('',#98888,0.1) ;
#15164=CYLINDRICAL_SURFACE('',#98891,0.0999999999999994) ;
#15165=CYLINDRICAL_SURFACE('',#98902,0.1) ;
#15166=CYLINDRICAL_SURFACE('',#98905,0.0999999999999994) ;
#15167=CYLINDRICAL_SURFACE('',#98907,0.1) ;
#15168=CYLINDRICAL_SURFACE('',#98911,0.0999999999999998) ;
#15169=CYLINDRICAL_SURFACE('',#98913,0.1) ;
#15170=CYLINDRICAL_SURFACE('',#98921,0.1) ;
#15171=CYLINDRICAL_SURFACE('',#98923,0.0999999999999998) ;
#15172=CYLINDRICAL_SURFACE('',#98925,0.1) ;
#15173=CYLINDRICAL_SURFACE('',#98927,0.1) ;
#15174=CYLINDRICAL_SURFACE('',#98930,0.1) ;
#15175=CYLINDRICAL_SURFACE('',#98940,0.1) ;
#15176=CYLINDRICAL_SURFACE('',#98942,0.0999999999999998) ;
#15177=CYLINDRICAL_SURFACE('',#98944,0.1) ;
#15178=CYLINDRICAL_SURFACE('',#98946,0.1) ;
#15179=CYLINDRICAL_SURFACE('',#98952,0.1) ;
#15180=CYLINDRICAL_SURFACE('',#98955,0.1) ;
#15181=CYLINDRICAL_SURFACE('',#98958,0.1) ;
#15182=CYLINDRICAL_SURFACE('',#98960,0.0999999999999998) ;
#15183=CYLINDRICAL_SURFACE('',#98966,0.1) ;
#15184=CYLINDRICAL_SURFACE('',#98970,0.1) ;
#15185=CYLINDRICAL_SURFACE('',#98972,0.1) ;
#15186=CYLINDRICAL_SURFACE('',#98978,0.1) ;
#15187=CYLINDRICAL_SURFACE('',#98980,0.0999999999999994) ;
#15188=CYLINDRICAL_SURFACE('',#98983,0.1) ;
#15189=CYLINDRICAL_SURFACE('',#98992,0.1) ;
#15190=CYLINDRICAL_SURFACE('',#98994,0.1) ;
#15191=CYLINDRICAL_SURFACE('',#98996,0.1) ;
#15192=CYLINDRICAL_SURFACE('',#98999,0.1) ;
#15193=CYLINDRICAL_SURFACE('',#99001,0.0999999999999998) ;
#15194=CYLINDRICAL_SURFACE('',#99003,0.1) ;
#15195=CYLINDRICAL_SURFACE('',#99014,0.1) ;
#15196=CYLINDRICAL_SURFACE('',#99016,0.1) ;
#15197=CYLINDRICAL_SURFACE('',#99018,0.0999999999999998) ;
#15198=CYLINDRICAL_SURFACE('',#99020,0.1) ;
#15199=CYLINDRICAL_SURFACE('',#99026,0.1) ;
#15200=CYLINDRICAL_SURFACE('',#99027,0.1) ;
#15201=CYLINDRICAL_SURFACE('',#99029,0.1) ;
#15202=CYLINDRICAL_SURFACE('',#99032,0.1) ;
#15203=CYLINDRICAL_SURFACE('',#99038,0.1) ;
#15204=CYLINDRICAL_SURFACE('',#99040,0.1) ;
#15205=CYLINDRICAL_SURFACE('',#99042,0.1) ;
#15206=CYLINDRICAL_SURFACE('',#99044,0.1) ;
#15207=CYLINDRICAL_SURFACE('',#99050,0.1) ;
#15208=CYLINDRICAL_SURFACE('',#99051,0.1) ;
#15209=CYLINDRICAL_SURFACE('',#99056,0.1) ;
#15210=CYLINDRICAL_SURFACE('',#99057,0.1) ;
#15211=CYLINDRICAL_SURFACE('',#99059,0.1) ;
#15212=CYLINDRICAL_SURFACE('',#99065,0.1) ;
#15213=CYLINDRICAL_SURFACE('',#99067,0.1) ;
#15214=CYLINDRICAL_SURFACE('',#99069,0.1) ;
#15215=CYLINDRICAL_SURFACE('',#99071,0.1) ;
#15216=CYLINDRICAL_SURFACE('',#99073,0.1) ;
#15217=CYLINDRICAL_SURFACE('',#99079,0.1) ;
#15218=CYLINDRICAL_SURFACE('',#99081,0.1) ;
#15219=CYLINDRICAL_SURFACE('',#99083,0.1) ;
#15220=CYLINDRICAL_SURFACE('',#99085,0.1) ;
#15221=CYLINDRICAL_SURFACE('',#99090,0.1) ;
#15222=CYLINDRICAL_SURFACE('',#99091,0.1) ;
#15223=CYLINDRICAL_SURFACE('',#99100,0.0999999999999998) ;
#15224=CYLINDRICAL_SURFACE('',#99102,0.0999999999999998) ;
#15225=CYLINDRICAL_SURFACE('',#99104,0.1) ;
#15226=CYLINDRICAL_SURFACE('',#99107,0.0999999999999998) ;
#15227=CYLINDRICAL_SURFACE('',#99109,0.1) ;
#15228=CYLINDRICAL_SURFACE('',#99111,0.1) ;
#15229=CYLINDRICAL_SURFACE('',#99122,0.0999999999999998) ;
#15230=CYLINDRICAL_SURFACE('',#99124,0.0999999999999998) ;
#15231=CYLINDRICAL_SURFACE('',#99126,0.0999999999999998) ;
#15232=CYLINDRICAL_SURFACE('',#99128,0.0999999999999998) ;
#15233=CYLINDRICAL_SURFACE('',#99134,0.1) ;
#15234=CYLINDRICAL_SURFACE('',#99135,0.1) ;
#15235=CYLINDRICAL_SURFACE('',#99137,0.0999999999999998) ;
#15236=CYLINDRICAL_SURFACE('',#99140,0.1) ;
#15237=CYLINDRICAL_SURFACE('',#99146,0.1) ;
#15238=CYLINDRICAL_SURFACE('',#99148,0.1) ;
#15239=CYLINDRICAL_SURFACE('',#99150,0.1) ;
#15240=CYLINDRICAL_SURFACE('',#99152,0.1) ;
#15241=CYLINDRICAL_SURFACE('',#99158,0.0999999999999998) ;
#15242=CYLINDRICAL_SURFACE('',#99159,0.0999999999999994) ;
#15243=CYLINDRICAL_SURFACE('',#99166,0.1) ;
#15244=CYLINDRICAL_SURFACE('',#99168,0.1) ;
#15245=CYLINDRICAL_SURFACE('',#99174,0.0999999999999994) ;
#15246=CYLINDRICAL_SURFACE('',#99175,0.1) ;
#15247=CYLINDRICAL_SURFACE('',#99176,0.1) ;
#15248=CYLINDRICAL_SURFACE('',#99177,0.1) ;
#15249=CYLINDRICAL_SURFACE('',#99178,0.1) ;
#15250=CYLINDRICAL_SURFACE('',#99179,0.0999999999999998) ;
#15251=CYLINDRICAL_SURFACE('',#99183,0.0999999999999998) ;
#15252=CYLINDRICAL_SURFACE('',#99190,0.1) ;
#15253=CYLINDRICAL_SURFACE('',#99196,0.1) ;
#15254=CYLINDRICAL_SURFACE('',#99557,1.65625) ;
#15255=CYLINDRICAL_SURFACE('',#99564,1.65625) ;
#15256=CYLINDRICAL_SURFACE('',#99571,1.65625) ;
#15257=CYLINDRICAL_SURFACE('',#99578,1.65625) ;
#15258=CYLINDRICAL_SURFACE('',#99585,1.65625) ;
#15259=CYLINDRICAL_SURFACE('',#99592,1.65625) ;
#15260=CYLINDRICAL_SURFACE('',#99599,1.65625) ;
#15261=CYLINDRICAL_SURFACE('',#99606,1.65625) ;
#15262=CYLINDRICAL_SURFACE('',#99613,1.65625) ;
#15263=CYLINDRICAL_SURFACE('',#99789,0.0999999999999994) ;
#15264=CYLINDRICAL_SURFACE('',#99793,0.1) ;
#15265=CYLINDRICAL_SURFACE('',#99797,0.1) ;
#15266=CYLINDRICAL_SURFACE('',#99801,0.0999999999999998) ;
#15267=CYLINDRICAL_SURFACE('',#99806,0.0999999999999994) ;
#15268=CYLINDRICAL_SURFACE('',#99810,0.0999999999999994) ;
#15269=CYLINDRICAL_SURFACE('',#99814,0.1) ;
#15270=CYLINDRICAL_SURFACE('',#99818,0.0999999999999994) ;
#15271=CYLINDRICAL_SURFACE('',#99823,0.0999999999999994) ;
#15272=CYLINDRICAL_SURFACE('',#99827,0.0999999999999994) ;
#15273=CYLINDRICAL_SURFACE('',#99831,0.0999999999999994) ;
#15274=CYLINDRICAL_SURFACE('',#99835,0.0999999999999994) ;
#15275=CYLINDRICAL_SURFACE('',#99840,0.0999999999999994) ;
#15276=CYLINDRICAL_SURFACE('',#99844,0.0999999999999994) ;
#15277=CYLINDRICAL_SURFACE('',#99848,0.0999999999999994) ;
#15278=CYLINDRICAL_SURFACE('',#99852,0.0999999999999994) ;
#15279=CYLINDRICAL_SURFACE('',#99857,0.0999999999999994) ;
#15280=CYLINDRICAL_SURFACE('',#99861,0.0999999999999994) ;
#15281=CYLINDRICAL_SURFACE('',#99865,0.0999999999999994) ;
#15282=CYLINDRICAL_SURFACE('',#99869,0.0999999999999994) ;
#15283=CYLINDRICAL_SURFACE('',#99874,0.0999999999999994) ;
#15284=CYLINDRICAL_SURFACE('',#99878,0.0999999999999994) ;
#15285=CYLINDRICAL_SURFACE('',#99882,0.0999999999999994) ;
#15286=CYLINDRICAL_SURFACE('',#99886,0.0999999999999994) ;
#15287=CYLINDRICAL_SURFACE('',#99891,0.0999999999999994) ;
#15288=CYLINDRICAL_SURFACE('',#99895,0.0999999999999994) ;
#15289=CYLINDRICAL_SURFACE('',#99899,0.0999999999999994) ;
#15290=CYLINDRICAL_SURFACE('',#99903,0.0999999999999994) ;
#15291=CYLINDRICAL_SURFACE('',#99908,0.0999999999999994) ;
#15292=CYLINDRICAL_SURFACE('',#99912,0.0999999999999994) ;
#15293=CYLINDRICAL_SURFACE('',#99916,0.0999999999999994) ;
#15294=CYLINDRICAL_SURFACE('',#99920,0.0999999999999994) ;
#15295=CYLINDRICAL_SURFACE('',#99925,0.100000000000003) ;
#15296=CYLINDRICAL_SURFACE('',#99929,0.100000000000003) ;
#15297=CYLINDRICAL_SURFACE('',#99933,0.100000000000003) ;
#15298=CYLINDRICAL_SURFACE('',#99937,0.100000000000003) ;
#15299=CYLINDRICAL_SURFACE('',#99948,0.1) ;
#15300=CYLINDRICAL_SURFACE('',#99950,0.0999999999999994) ;
#15301=CYLINDRICAL_SURFACE('',#99952,0.1) ;
#15302=CYLINDRICAL_SURFACE('',#99955,0.0999999999999994) ;
#15303=CYLINDRICAL_SURFACE('',#99966,0.0999999999999998) ;
#15304=CYLINDRICAL_SURFACE('',#99969,0.0999999999999994) ;
#15305=CYLINDRICAL_SURFACE('',#99971,0.0999999999999998) ;
#15306=CYLINDRICAL_SURFACE('',#99975,0.0999999999999998) ;
#15307=CYLINDRICAL_SURFACE('',#99977,0.1) ;
#15308=CYLINDRICAL_SURFACE('',#99985,0.0999999999999998) ;
#15309=CYLINDRICAL_SURFACE('',#99987,0.0999999999999998) ;
#15310=CYLINDRICAL_SURFACE('',#99989,0.1) ;
#15311=CYLINDRICAL_SURFACE('',#99991,0.1) ;
#15312=CYLINDRICAL_SURFACE('',#99994,0.1) ;
#15313=CYLINDRICAL_SURFACE('',#100004,0.0999999999999998) ;
#15314=CYLINDRICAL_SURFACE('',#100006,0.0999999999999998) ;
#15315=CYLINDRICAL_SURFACE('',#100008,0.1) ;
#15316=CYLINDRICAL_SURFACE('',#100010,0.1) ;
#15317=CYLINDRICAL_SURFACE('',#100016,0.1) ;
#15318=CYLINDRICAL_SURFACE('',#100019,0.1) ;
#15319=CYLINDRICAL_SURFACE('',#100021,0.0999999999999998) ;
#15320=CYLINDRICAL_SURFACE('',#100027,0.0999999999999998) ;
#15321=CYLINDRICAL_SURFACE('',#100031,0.1) ;
#15322=CYLINDRICAL_SURFACE('',#100033,0.1) ;
#15323=CYLINDRICAL_SURFACE('',#100039,0.0999999999999998) ;
#15324=CYLINDRICAL_SURFACE('',#100041,0.0999999999999994) ;
#15325=CYLINDRICAL_SURFACE('',#100044,0.100000000000003) ;
#15326=CYLINDRICAL_SURFACE('',#100047,0.0999999999999998) ;
#15327=CYLINDRICAL_SURFACE('',#100050,0.1) ;
#15328=CYLINDRICAL_SURFACE('',#100053,0.100000000000003) ;
#15329=CYLINDRICAL_SURFACE('',#100056,0.100000000000003) ;
#15330=CYLINDRICAL_SURFACE('',#100059,0.0999999999999998) ;
#15331=CYLINDRICAL_SURFACE('',#100062,0.1) ;
#15332=CYLINDRICAL_SURFACE('',#100065,0.0999999999999994) ;
#15333=CYLINDRICAL_SURFACE('',#100068,0.0999999999999994) ;
#15334=CYLINDRICAL_SURFACE('',#100071,0.0999999999999998) ;
#15335=CYLINDRICAL_SURFACE('',#100074,0.1) ;
#15336=CYLINDRICAL_SURFACE('',#100077,0.0999999999999994) ;
#15337=CYLINDRICAL_SURFACE('',#100080,0.0999999999999994) ;
#15338=CYLINDRICAL_SURFACE('',#100083,0.0999999999999998) ;
#15339=CYLINDRICAL_SURFACE('',#100086,0.1) ;
#15340=CYLINDRICAL_SURFACE('',#100089,0.0999999999999994) ;
#15341=CYLINDRICAL_SURFACE('',#100092,0.0999999999999994) ;
#15342=CYLINDRICAL_SURFACE('',#100095,0.0999999999999998) ;
#15343=CYLINDRICAL_SURFACE('',#100098,0.1) ;
#15344=CYLINDRICAL_SURFACE('',#100101,0.0999999999999994) ;
#15345=CYLINDRICAL_SURFACE('',#100104,0.0999999999999994) ;
#15346=CYLINDRICAL_SURFACE('',#100107,0.0999999999999998) ;
#15347=CYLINDRICAL_SURFACE('',#100110,0.1) ;
#15348=CYLINDRICAL_SURFACE('',#100113,0.0999999999999994) ;
#15349=CYLINDRICAL_SURFACE('',#100116,0.0999999999999994) ;
#15350=CYLINDRICAL_SURFACE('',#100119,0.0999999999999998) ;
#15351=CYLINDRICAL_SURFACE('',#100122,0.1) ;
#15352=CYLINDRICAL_SURFACE('',#100125,0.0999999999999994) ;
#15353=CYLINDRICAL_SURFACE('',#100128,0.0999999999999994) ;
#15354=CYLINDRICAL_SURFACE('',#100131,0.0999999999999998) ;
#15355=CYLINDRICAL_SURFACE('',#100134,0.1) ;
#15356=CYLINDRICAL_SURFACE('',#100137,0.1) ;
#15357=CYLINDRICAL_SURFACE('',#100140,0.0999999999999998) ;
#15358=CYLINDRICAL_SURFACE('',#100149,0.1) ;
#15359=CYLINDRICAL_SURFACE('',#100151,0.0999999999999998) ;
#15360=CYLINDRICAL_SURFACE('',#100153,0.0999999999999998) ;
#15361=CYLINDRICAL_SURFACE('',#100156,0.0999999999999998) ;
#15362=CYLINDRICAL_SURFACE('',#100158,0.0999999999999998) ;
#15363=CYLINDRICAL_SURFACE('',#100160,0.1) ;
#15364=CYLINDRICAL_SURFACE('',#100171,0.1) ;
#15365=CYLINDRICAL_SURFACE('',#100173,0.1) ;
#15366=CYLINDRICAL_SURFACE('',#100175,0.0999999999999998) ;
#15367=CYLINDRICAL_SURFACE('',#100177,0.1) ;
#15368=CYLINDRICAL_SURFACE('',#100183,0.1) ;
#15369=CYLINDRICAL_SURFACE('',#100184,0.0999999999999998) ;
#15370=CYLINDRICAL_SURFACE('',#100186,0.1) ;
#15371=CYLINDRICAL_SURFACE('',#100189,0.1) ;
#15372=CYLINDRICAL_SURFACE('',#100195,0.0999999999999998) ;
#15373=CYLINDRICAL_SURFACE('',#100197,0.0999999999999998) ;
#15374=CYLINDRICAL_SURFACE('',#100199,0.1) ;
#15375=CYLINDRICAL_SURFACE('',#100201,0.1) ;
#15376=CYLINDRICAL_SURFACE('',#100207,0.1) ;
#15377=CYLINDRICAL_SURFACE('',#100208,0.1) ;
#15378=CYLINDRICAL_SURFACE('',#100213,0.0999999999999998) ;
#15379=CYLINDRICAL_SURFACE('',#100214,0.1) ;
#15380=CYLINDRICAL_SURFACE('',#100216,0.1) ;
#15381=CYLINDRICAL_SURFACE('',#100222,0.1) ;
#15382=CYLINDRICAL_SURFACE('',#100224,0.1) ;
#15383=CYLINDRICAL_SURFACE('',#100226,0.1) ;
#15384=CYLINDRICAL_SURFACE('',#100228,0.1) ;
#15385=CYLINDRICAL_SURFACE('',#100230,0.1) ;
#15386=CYLINDRICAL_SURFACE('',#100236,0.0999999999999998) ;
#15387=CYLINDRICAL_SURFACE('',#100238,0.0999999999999998) ;
#15388=CYLINDRICAL_SURFACE('',#100240,0.1) ;
#15389=CYLINDRICAL_SURFACE('',#100242,0.1) ;
#15390=CYLINDRICAL_SURFACE('',#100247,0.1) ;
#15391=CYLINDRICAL_SURFACE('',#100248,0.1) ;
#15392=CYLINDRICAL_SURFACE('',#100254,0.1) ;
#15393=CYLINDRICAL_SURFACE('',#100259,0.1) ;
#15394=CYLINDRICAL_SURFACE('',#100262,0.1) ;
#15395=CYLINDRICAL_SURFACE('',#100268,0.1) ;
#15396=CYLINDRICAL_SURFACE('',#100274,0.1) ;
#15397=CYLINDRICAL_SURFACE('',#100279,0.1) ;
#15398=CYLINDRICAL_SURFACE('',#100282,0.1) ;
#15399=CYLINDRICAL_SURFACE('',#100288,0.1) ;
#15400=CYLINDRICAL_SURFACE('',#100294,0.1) ;
#15401=CYLINDRICAL_SURFACE('',#100299,0.1) ;
#15402=CYLINDRICAL_SURFACE('',#100302,0.1) ;
#15403=CYLINDRICAL_SURFACE('',#100308,0.1) ;
#15404=CYLINDRICAL_SURFACE('',#100314,0.1) ;
#15405=CYLINDRICAL_SURFACE('',#100319,0.1) ;
#15406=CYLINDRICAL_SURFACE('',#100322,0.1) ;
#15407=CYLINDRICAL_SURFACE('',#100328,0.1) ;
#15408=CYLINDRICAL_SURFACE('',#100334,0.1) ;
#15409=CYLINDRICAL_SURFACE('',#100339,0.1) ;
#15410=CYLINDRICAL_SURFACE('',#100342,0.1) ;
#15411=CYLINDRICAL_SURFACE('',#100348,0.1) ;
#15412=CYLINDRICAL_SURFACE('',#100354,0.1) ;
#15413=CYLINDRICAL_SURFACE('',#100359,0.1) ;
#15414=CYLINDRICAL_SURFACE('',#100362,0.1) ;
#15415=CYLINDRICAL_SURFACE('',#100368,0.1) ;
#15416=CYLINDRICAL_SURFACE('',#100374,0.1) ;
#15417=CYLINDRICAL_SURFACE('',#100379,0.1) ;
#15418=CYLINDRICAL_SURFACE('',#100382,0.1) ;
#15419=CYLINDRICAL_SURFACE('',#100388,0.1) ;
#15420=CYLINDRICAL_SURFACE('',#100394,0.1) ;
#15421=CYLINDRICAL_SURFACE('',#100399,0.1) ;
#15422=CYLINDRICAL_SURFACE('',#100402,0.1) ;
#15423=CYLINDRICAL_SURFACE('',#100408,0.1) ;
#15424=CYLINDRICAL_SURFACE('',#100417,0.0999999999999998) ;
#15425=CYLINDRICAL_SURFACE('',#100419,0.0999999999999998) ;
#15426=CYLINDRICAL_SURFACE('',#100421,0.1) ;
#15427=CYLINDRICAL_SURFACE('',#100424,0.0999999999999998) ;
#15428=CYLINDRICAL_SURFACE('',#100426,0.1) ;
#15429=CYLINDRICAL_SURFACE('',#100428,0.0999999999999998) ;
#15430=CYLINDRICAL_SURFACE('',#100439,0.0999999999999998) ;
#15431=CYLINDRICAL_SURFACE('',#100441,0.0999999999999998) ;
#15432=CYLINDRICAL_SURFACE('',#100443,0.0999999999999998) ;
#15433=CYLINDRICAL_SURFACE('',#100445,0.0999999999999998) ;
#15434=CYLINDRICAL_SURFACE('',#100451,0.0999999999999998) ;
#15435=CYLINDRICAL_SURFACE('',#100452,0.1) ;
#15436=CYLINDRICAL_SURFACE('',#100454,0.0999999999999998) ;
#15437=CYLINDRICAL_SURFACE('',#100457,0.0999999999999998) ;
#15438=CYLINDRICAL_SURFACE('',#100463,0.1) ;
#15439=CYLINDRICAL_SURFACE('',#100465,0.1) ;
#15440=CYLINDRICAL_SURFACE('',#100467,0.0999999999999998) ;
#15441=CYLINDRICAL_SURFACE('',#100469,0.0999999999999998) ;
#15442=CYLINDRICAL_SURFACE('',#100475,0.0999999999999998) ;
#15443=CYLINDRICAL_SURFACE('',#100476,0.0999999999999994) ;
#15444=CYLINDRICAL_SURFACE('',#100483,0.0999999999999998) ;
#15445=CYLINDRICAL_SURFACE('',#100485,0.1) ;
#15446=CYLINDRICAL_SURFACE('',#100491,0.0999999999999994) ;
#15447=CYLINDRICAL_SURFACE('',#100492,0.1) ;
#15448=CYLINDRICAL_SURFACE('',#100493,0.1) ;
#15449=CYLINDRICAL_SURFACE('',#100494,0.1) ;
#15450=CYLINDRICAL_SURFACE('',#100495,0.1) ;
#15451=CYLINDRICAL_SURFACE('',#100500,0.0999999999999994) ;
#15452=CYLINDRICAL_SURFACE('',#100502,0.1) ;
#15453=CYLINDRICAL_SURFACE('',#100506,0.1) ;
#15454=CYLINDRICAL_SURFACE('',#100517,0.0999999999999994) ;
#15455=CYLINDRICAL_SURFACE('',#100520,0.1) ;
#15456=CYLINDRICAL_SURFACE('',#100522,0.0999999999999998) ;
#15457=CYLINDRICAL_SURFACE('',#100526,0.0999999999999994) ;
#15458=CYLINDRICAL_SURFACE('',#100528,0.0999999999999994) ;
#15459=CYLINDRICAL_SURFACE('',#100530,0.0999999999999994) ;
#15460=CYLINDRICAL_SURFACE('',#100539,0.1) ;
#15461=CYLINDRICAL_SURFACE('',#100542,0.1) ;
#15462=CYLINDRICAL_SURFACE('',#100544,0.0999999999999998) ;
#15463=CYLINDRICAL_SURFACE('',#100546,0.0999999999999994) ;
#15464=CYLINDRICAL_SURFACE('',#100555,0.1) ;
#15465=CYLINDRICAL_SURFACE('',#100557,0.1) ;
#15466=CYLINDRICAL_SURFACE('',#100559,0.0999999999999998) ;
#15467=CYLINDRICAL_SURFACE('',#100561,0.0999999999999994) ;
#15468=CYLINDRICAL_SURFACE('',#100567,0.0999999999999998) ;
#15469=CYLINDRICAL_SURFACE('',#100569,0.1) ;
#15470=CYLINDRICAL_SURFACE('',#100571,0.1) ;
#15471=CYLINDRICAL_SURFACE('',#100574,0.1) ;
#15472=CYLINDRICAL_SURFACE('',#100581,0.0999999999999994) ;
#15473=CYLINDRICAL_SURFACE('',#100583,0.1) ;
#15474=CYLINDRICAL_SURFACE('',#100590,0.1) ;
#15475=CYLINDRICAL_SURFACE('',#100592,0.1) ;
#15476=CYLINDRICAL_SURFACE('',#100594,0.0999999999999998) ;
#15477=CYLINDRICAL_SURFACE('',#100596,0.0999999999999994) ;
#15478=CYLINDRICAL_SURFACE('',#100602,0.1) ;
#15479=CYLINDRICAL_SURFACE('',#100604,0.0999999999999994) ;
#15480=CYLINDRICAL_SURFACE('',#100608,0.0999999999999994) ;
#15481=CYLINDRICAL_SURFACE('',#100612,0.1) ;
#15482=CYLINDRICAL_SURFACE('',#100614,0.1) ;
#15483=CYLINDRICAL_SURFACE('',#100618,0.1) ;
#15484=CYLINDRICAL_SURFACE('',#100620,0.1) ;
#15485=CYLINDRICAL_SURFACE('',#100624,0.1) ;
#15486=CYLINDRICAL_SURFACE('',#100629,0.0999999999999998) ;
#15487=CYLINDRICAL_SURFACE('',#100631,0.1) ;
#15488=CYLINDRICAL_SURFACE('',#100635,0.0999999999999994) ;
#15489=CYLINDRICAL_SURFACE('',#100637,0.0999999999999994) ;
#15490=CYLINDRICAL_SURFACE('',#100641,0.1) ;
#15491=CYLINDRICAL_SURFACE('',#100647,0.1) ;
#15492=CYLINDRICAL_SURFACE('',#100649,0.0999999999999994) ;
#15493=CYLINDRICAL_SURFACE('',#100655,0.1) ;
#15494=CYLINDRICAL_SURFACE('',#100657,0.0999999999999994) ;
#15495=CYLINDRICAL_SURFACE('',#100660,0.1) ;
#15496=CYLINDRICAL_SURFACE('',#100662,0.1) ;
#15497=CYLINDRICAL_SURFACE('',#100665,0.0999999999999994) ;
#15498=CYLINDRICAL_SURFACE('',#100671,0.1) ;
#15499=CYLINDRICAL_SURFACE('',#100673,0.1) ;
#15500=CYLINDRICAL_SURFACE('',#100675,0.0999999999999994) ;
#15501=CYLINDRICAL_SURFACE('',#100677,0.0999999999999994) ;
#15502=CYLINDRICAL_SURFACE('',#100683,0.1) ;
#15503=CYLINDRICAL_SURFACE('',#100684,0.0999999999999994) ;
#15504=CYLINDRICAL_SURFACE('',#100693,0.0999999999999998) ;
#15505=CYLINDRICAL_SURFACE('',#100695,0.0999999999999998) ;
#15506=CYLINDRICAL_SURFACE('',#100697,0.0999999999999994) ;
#15507=CYLINDRICAL_SURFACE('',#100700,0.0999999999999998) ;
#15508=CYLINDRICAL_SURFACE('',#100702,0.1) ;
#15509=CYLINDRICAL_SURFACE('',#100704,0.1) ;
#15510=CYLINDRICAL_SURFACE('',#100715,0.0999999999999998) ;
#15511=CYLINDRICAL_SURFACE('',#100717,0.0999999999999998) ;
#15512=CYLINDRICAL_SURFACE('',#100719,0.0999999999999998) ;
#15513=CYLINDRICAL_SURFACE('',#100721,0.0999999999999998) ;
#15514=CYLINDRICAL_SURFACE('',#100727,0.1) ;
#15515=CYLINDRICAL_SURFACE('',#100728,0.0999999999999994) ;
#15516=CYLINDRICAL_SURFACE('',#100730,0.0999999999999998) ;
#15517=CYLINDRICAL_SURFACE('',#100733,0.1) ;
#15518=CYLINDRICAL_SURFACE('',#100739,0.0999999999999994) ;
#15519=CYLINDRICAL_SURFACE('',#100741,0.0999999999999994) ;
#15520=CYLINDRICAL_SURFACE('',#100743,0.1) ;
#15521=CYLINDRICAL_SURFACE('',#100745,0.1) ;
#15522=CYLINDRICAL_SURFACE('',#100751,0.0999999999999998) ;
#15523=CYLINDRICAL_SURFACE('',#100752,0.0999999999999994) ;
#15524=CYLINDRICAL_SURFACE('',#100759,0.1) ;
#15525=CYLINDRICAL_SURFACE('',#100761,0.0999999999999994) ;
#15526=CYLINDRICAL_SURFACE('',#100767,0.0999999999999994) ;
#15527=CYLINDRICAL_SURFACE('',#100768,0.0999999999999998) ;
#15528=CYLINDRICAL_SURFACE('',#100769,0.0999999999999998) ;
#15529=CYLINDRICAL_SURFACE('',#100770,0.0999999999999998) ;
#15530=CYLINDRICAL_SURFACE('',#100771,0.0999999999999998) ;
#15531=CYLINDRICAL_SURFACE('',#100776,0.0999999999999994) ;
#15532=CYLINDRICAL_SURFACE('',#100778,0.0999999999999994) ;
#15533=CYLINDRICAL_SURFACE('',#100782,0.0999999999999994) ;
#15534=CYLINDRICAL_SURFACE('',#100793,0.0999999999999994) ;
#15535=CYLINDRICAL_SURFACE('',#100796,0.0999999999999994) ;
#15536=CYLINDRICAL_SURFACE('',#100798,0.0999999999999998) ;
#15537=CYLINDRICAL_SURFACE('',#100802,0.0999999999999994) ;
#15538=CYLINDRICAL_SURFACE('',#100804,0.0999999999999994) ;
#15539=CYLINDRICAL_SURFACE('',#100806,0.0999999999999994) ;
#15540=CYLINDRICAL_SURFACE('',#100815,0.1) ;
#15541=CYLINDRICAL_SURFACE('',#100818,0.0999999999999994) ;
#15542=CYLINDRICAL_SURFACE('',#100820,0.0999999999999998) ;
#15543=CYLINDRICAL_SURFACE('',#100822,0.0999999999999994) ;
#15544=CYLINDRICAL_SURFACE('',#100831,0.0999999999999994) ;
#15545=CYLINDRICAL_SURFACE('',#100833,0.1) ;
#15546=CYLINDRICAL_SURFACE('',#100835,0.0999999999999998) ;
#15547=CYLINDRICAL_SURFACE('',#100837,0.0999999999999994) ;
#15548=CYLINDRICAL_SURFACE('',#100843,0.0999999999999998) ;
#15549=CYLINDRICAL_SURFACE('',#100845,0.1) ;
#15550=CYLINDRICAL_SURFACE('',#100847,0.1) ;
#15551=CYLINDRICAL_SURFACE('',#100850,0.1) ;
#15552=CYLINDRICAL_SURFACE('',#100857,0.0999999999999994) ;
#15553=CYLINDRICAL_SURFACE('',#100859,0.0999999999999994) ;
#15554=CYLINDRICAL_SURFACE('',#100866,0.0999999999999994) ;
#15555=CYLINDRICAL_SURFACE('',#100868,0.0999999999999994) ;
#15556=CYLINDRICAL_SURFACE('',#100870,0.0999999999999998) ;
#15557=CYLINDRICAL_SURFACE('',#100872,0.0999999999999994) ;
#15558=CYLINDRICAL_SURFACE('',#100878,0.1) ;
#15559=CYLINDRICAL_SURFACE('',#100880,0.0999999999999994) ;
#15560=CYLINDRICAL_SURFACE('',#100884,0.0999999999999994) ;
#15561=CYLINDRICAL_SURFACE('',#100888,0.1) ;
#15562=CYLINDRICAL_SURFACE('',#100890,0.0999999999999994) ;
#15563=CYLINDRICAL_SURFACE('',#100894,0.0999999999999994) ;
#15564=CYLINDRICAL_SURFACE('',#100896,0.1) ;
#15565=CYLINDRICAL_SURFACE('',#100900,0.1) ;
#15566=CYLINDRICAL_SURFACE('',#100905,0.0999999999999998) ;
#15567=CYLINDRICAL_SURFACE('',#100907,0.1) ;
#15568=CYLINDRICAL_SURFACE('',#100911,0.0999999999999994) ;
#15569=CYLINDRICAL_SURFACE('',#100913,0.0999999999999994) ;
#15570=CYLINDRICAL_SURFACE('',#100917,0.1) ;
#15571=CYLINDRICAL_SURFACE('',#100923,0.1) ;
#15572=CYLINDRICAL_SURFACE('',#100925,0.0999999999999994) ;
#15573=CYLINDRICAL_SURFACE('',#100931,0.0999999999999994) ;
#15574=CYLINDRICAL_SURFACE('',#100933,0.0999999999999994) ;
#15575=CYLINDRICAL_SURFACE('',#100936,0.0999999999999994) ;
#15576=CYLINDRICAL_SURFACE('',#100938,0.1) ;
#15577=CYLINDRICAL_SURFACE('',#100941,0.0999999999999994) ;
#15578=CYLINDRICAL_SURFACE('',#100947,0.0999999999999994) ;
#15579=CYLINDRICAL_SURFACE('',#100949,0.0999999999999994) ;
#15580=CYLINDRICAL_SURFACE('',#100951,0.0999999999999994) ;
#15581=CYLINDRICAL_SURFACE('',#100953,0.0999999999999994) ;
#15582=CYLINDRICAL_SURFACE('',#100959,0.1) ;
#15583=CYLINDRICAL_SURFACE('',#100960,0.0999999999999994) ;
#15584=CYLINDRICAL_SURFACE('',#100969,0.0999999999999998) ;
#15585=CYLINDRICAL_SURFACE('',#100971,0.0999999999999998) ;
#15586=CYLINDRICAL_SURFACE('',#100973,0.0999999999999994) ;
#15587=CYLINDRICAL_SURFACE('',#100976,0.0999999999999998) ;
#15588=CYLINDRICAL_SURFACE('',#100978,0.1) ;
#15589=CYLINDRICAL_SURFACE('',#100980,0.0999999999999994) ;
#15590=CYLINDRICAL_SURFACE('',#100991,0.0999999999999998) ;
#15591=CYLINDRICAL_SURFACE('',#100993,0.0999999999999998) ;
#15592=CYLINDRICAL_SURFACE('',#100995,0.0999999999999998) ;
#15593=CYLINDRICAL_SURFACE('',#100997,0.0999999999999998) ;
#15594=CYLINDRICAL_SURFACE('',#101003,0.0999999999999994) ;
#15595=CYLINDRICAL_SURFACE('',#101004,0.0999999999999994) ;
#15596=CYLINDRICAL_SURFACE('',#101006,0.0999999999999998) ;
#15597=CYLINDRICAL_SURFACE('',#101009,0.0999999999999994) ;
#15598=CYLINDRICAL_SURFACE('',#101015,0.0999999999999994) ;
#15599=CYLINDRICAL_SURFACE('',#101017,0.0999999999999994) ;
#15600=CYLINDRICAL_SURFACE('',#101019,0.0999999999999994) ;
#15601=CYLINDRICAL_SURFACE('',#101021,0.0999999999999994) ;
#15602=CYLINDRICAL_SURFACE('',#101027,0.0999999999999998) ;
#15603=CYLINDRICAL_SURFACE('',#101028,0.0999999999999994) ;
#15604=CYLINDRICAL_SURFACE('',#101035,0.0999999999999994) ;
#15605=CYLINDRICAL_SURFACE('',#101037,0.0999999999999994) ;
#15606=CYLINDRICAL_SURFACE('',#101043,0.0999999999999994) ;
#15607=CYLINDRICAL_SURFACE('',#101044,0.1) ;
#15608=CYLINDRICAL_SURFACE('',#101045,0.1) ;
#15609=CYLINDRICAL_SURFACE('',#101046,0.1) ;
#15610=CYLINDRICAL_SURFACE('',#101047,0.1) ;
#15611=CYLINDRICAL_SURFACE('',#101052,0.0999999999999994) ;
#15612=CYLINDRICAL_SURFACE('',#101054,0.0999999999999994) ;
#15613=CYLINDRICAL_SURFACE('',#101058,0.0999999999999994) ;
#15614=CYLINDRICAL_SURFACE('',#101069,0.0999999999999994) ;
#15615=CYLINDRICAL_SURFACE('',#101072,0.0999999999999994) ;
#15616=CYLINDRICAL_SURFACE('',#101074,0.0999999999999998) ;
#15617=CYLINDRICAL_SURFACE('',#101078,0.0999999999999994) ;
#15618=CYLINDRICAL_SURFACE('',#101080,0.0999999999999994) ;
#15619=CYLINDRICAL_SURFACE('',#101082,0.0999999999999994) ;
#15620=CYLINDRICAL_SURFACE('',#101091,0.1) ;
#15621=CYLINDRICAL_SURFACE('',#101094,0.0999999999999994) ;
#15622=CYLINDRICAL_SURFACE('',#101096,0.0999999999999998) ;
#15623=CYLINDRICAL_SURFACE('',#101098,0.0999999999999994) ;
#15624=CYLINDRICAL_SURFACE('',#101107,0.0999999999999994) ;
#15625=CYLINDRICAL_SURFACE('',#101109,0.1) ;
#15626=CYLINDRICAL_SURFACE('',#101111,0.0999999999999998) ;
#15627=CYLINDRICAL_SURFACE('',#101113,0.0999999999999994) ;
#15628=CYLINDRICAL_SURFACE('',#101119,0.0999999999999998) ;
#15629=CYLINDRICAL_SURFACE('',#101121,0.1) ;
#15630=CYLINDRICAL_SURFACE('',#101123,0.1) ;
#15631=CYLINDRICAL_SURFACE('',#101126,0.1) ;
#15632=CYLINDRICAL_SURFACE('',#101133,0.0999999999999994) ;
#15633=CYLINDRICAL_SURFACE('',#101135,0.0999999999999994) ;
#15634=CYLINDRICAL_SURFACE('',#101142,0.0999999999999994) ;
#15635=CYLINDRICAL_SURFACE('',#101144,0.0999999999999994) ;
#15636=CYLINDRICAL_SURFACE('',#101146,0.0999999999999998) ;
#15637=CYLINDRICAL_SURFACE('',#101148,0.0999999999999994) ;
#15638=CYLINDRICAL_SURFACE('',#101154,0.1) ;
#15639=CYLINDRICAL_SURFACE('',#101156,0.0999999999999994) ;
#15640=CYLINDRICAL_SURFACE('',#101160,0.0999999999999994) ;
#15641=CYLINDRICAL_SURFACE('',#101164,0.1) ;
#15642=CYLINDRICAL_SURFACE('',#101166,0.0999999999999994) ;
#15643=CYLINDRICAL_SURFACE('',#101170,0.0999999999999994) ;
#15644=CYLINDRICAL_SURFACE('',#101172,0.1) ;
#15645=CYLINDRICAL_SURFACE('',#101176,0.1) ;
#15646=CYLINDRICAL_SURFACE('',#101181,0.0999999999999998) ;
#15647=CYLINDRICAL_SURFACE('',#101183,0.1) ;
#15648=CYLINDRICAL_SURFACE('',#101187,0.0999999999999994) ;
#15649=CYLINDRICAL_SURFACE('',#101189,0.0999999999999994) ;
#15650=CYLINDRICAL_SURFACE('',#101193,0.1) ;
#15651=CYLINDRICAL_SURFACE('',#101199,0.1) ;
#15652=CYLINDRICAL_SURFACE('',#101201,0.0999999999999994) ;
#15653=CYLINDRICAL_SURFACE('',#101207,0.0999999999999994) ;
#15654=CYLINDRICAL_SURFACE('',#101209,0.0999999999999994) ;
#15655=CYLINDRICAL_SURFACE('',#101212,0.0999999999999994) ;
#15656=CYLINDRICAL_SURFACE('',#101214,0.1) ;
#15657=CYLINDRICAL_SURFACE('',#101217,0.0999999999999994) ;
#15658=CYLINDRICAL_SURFACE('',#101223,0.0999999999999994) ;
#15659=CYLINDRICAL_SURFACE('',#101225,0.0999999999999994) ;
#15660=CYLINDRICAL_SURFACE('',#101227,0.0999999999999994) ;
#15661=CYLINDRICAL_SURFACE('',#101229,0.0999999999999994) ;
#15662=CYLINDRICAL_SURFACE('',#101235,0.1) ;
#15663=CYLINDRICAL_SURFACE('',#101236,0.0999999999999994) ;
#15664=CYLINDRICAL_SURFACE('',#101245,0.0999999999999998) ;
#15665=CYLINDRICAL_SURFACE('',#101247,0.0999999999999998) ;
#15666=CYLINDRICAL_SURFACE('',#101249,0.0999999999999994) ;
#15667=CYLINDRICAL_SURFACE('',#101252,0.0999999999999998) ;
#15668=CYLINDRICAL_SURFACE('',#101254,0.1) ;
#15669=CYLINDRICAL_SURFACE('',#101256,0.0999999999999994) ;
#15670=CYLINDRICAL_SURFACE('',#101267,0.0999999999999998) ;
#15671=CYLINDRICAL_SURFACE('',#101269,0.0999999999999998) ;
#15672=CYLINDRICAL_SURFACE('',#101271,0.0999999999999998) ;
#15673=CYLINDRICAL_SURFACE('',#101273,0.0999999999999998) ;
#15674=CYLINDRICAL_SURFACE('',#101279,0.0999999999999994) ;
#15675=CYLINDRICAL_SURFACE('',#101280,0.0999999999999994) ;
#15676=CYLINDRICAL_SURFACE('',#101282,0.0999999999999998) ;
#15677=CYLINDRICAL_SURFACE('',#101285,0.0999999999999994) ;
#15678=CYLINDRICAL_SURFACE('',#101291,0.0999999999999994) ;
#15679=CYLINDRICAL_SURFACE('',#101293,0.0999999999999994) ;
#15680=CYLINDRICAL_SURFACE('',#101295,0.0999999999999994) ;
#15681=CYLINDRICAL_SURFACE('',#101297,0.0999999999999994) ;
#15682=CYLINDRICAL_SURFACE('',#101303,0.0999999999999998) ;
#15683=CYLINDRICAL_SURFACE('',#101304,0.0999999999999994) ;
#15684=CYLINDRICAL_SURFACE('',#101311,0.0999999999999994) ;
#15685=CYLINDRICAL_SURFACE('',#101313,0.0999999999999994) ;
#15686=CYLINDRICAL_SURFACE('',#101319,0.0999999999999994) ;
#15687=CYLINDRICAL_SURFACE('',#101320,0.1) ;
#15688=CYLINDRICAL_SURFACE('',#101321,0.1) ;
#15689=CYLINDRICAL_SURFACE('',#101322,0.1) ;
#15690=CYLINDRICAL_SURFACE('',#101323,0.1) ;
#15691=CYLINDRICAL_SURFACE('',#101328,0.0999999999999994) ;
#15692=CYLINDRICAL_SURFACE('',#101330,0.0999999999999994) ;
#15693=CYLINDRICAL_SURFACE('',#101334,0.0999999999999994) ;
#15694=CYLINDRICAL_SURFACE('',#101345,0.0999999999999994) ;
#15695=CYLINDRICAL_SURFACE('',#101348,0.0999999999999994) ;
#15696=CYLINDRICAL_SURFACE('',#101350,0.0999999999999998) ;
#15697=CYLINDRICAL_SURFACE('',#101354,0.0999999999999994) ;
#15698=CYLINDRICAL_SURFACE('',#101356,0.0999999999999994) ;
#15699=CYLINDRICAL_SURFACE('',#101358,0.0999999999999994) ;
#15700=CYLINDRICAL_SURFACE('',#101367,0.1) ;
#15701=CYLINDRICAL_SURFACE('',#101370,0.0999999999999994) ;
#15702=CYLINDRICAL_SURFACE('',#101372,0.0999999999999998) ;
#15703=CYLINDRICAL_SURFACE('',#101374,0.0999999999999994) ;
#15704=CYLINDRICAL_SURFACE('',#101383,0.0999999999999994) ;
#15705=CYLINDRICAL_SURFACE('',#101385,0.1) ;
#15706=CYLINDRICAL_SURFACE('',#101387,0.0999999999999998) ;
#15707=CYLINDRICAL_SURFACE('',#101389,0.0999999999999994) ;
#15708=CYLINDRICAL_SURFACE('',#101395,0.0999999999999998) ;
#15709=CYLINDRICAL_SURFACE('',#101397,0.1) ;
#15710=CYLINDRICAL_SURFACE('',#101399,0.1) ;
#15711=CYLINDRICAL_SURFACE('',#101402,0.1) ;
#15712=CYLINDRICAL_SURFACE('',#101409,0.0999999999999994) ;
#15713=CYLINDRICAL_SURFACE('',#101411,0.0999999999999994) ;
#15714=CYLINDRICAL_SURFACE('',#101418,0.0999999999999994) ;
#15715=CYLINDRICAL_SURFACE('',#101420,0.0999999999999994) ;
#15716=CYLINDRICAL_SURFACE('',#101422,0.0999999999999998) ;
#15717=CYLINDRICAL_SURFACE('',#101424,0.0999999999999994) ;
#15718=CYLINDRICAL_SURFACE('',#101430,0.1) ;
#15719=CYLINDRICAL_SURFACE('',#101432,0.0999999999999994) ;
#15720=CYLINDRICAL_SURFACE('',#101436,0.0999999999999994) ;
#15721=CYLINDRICAL_SURFACE('',#101440,0.1) ;
#15722=CYLINDRICAL_SURFACE('',#101442,0.0999999999999994) ;
#15723=CYLINDRICAL_SURFACE('',#101446,0.0999999999999994) ;
#15724=CYLINDRICAL_SURFACE('',#101448,0.1) ;
#15725=CYLINDRICAL_SURFACE('',#101452,0.1) ;
#15726=CYLINDRICAL_SURFACE('',#101457,0.0999999999999998) ;
#15727=CYLINDRICAL_SURFACE('',#101459,0.1) ;
#15728=CYLINDRICAL_SURFACE('',#101463,0.0999999999999994) ;
#15729=CYLINDRICAL_SURFACE('',#101465,0.0999999999999994) ;
#15730=CYLINDRICAL_SURFACE('',#101469,0.1) ;
#15731=CYLINDRICAL_SURFACE('',#101475,0.1) ;
#15732=CYLINDRICAL_SURFACE('',#101477,0.0999999999999994) ;
#15733=CYLINDRICAL_SURFACE('',#101483,0.0999999999999994) ;
#15734=CYLINDRICAL_SURFACE('',#101485,0.0999999999999994) ;
#15735=CYLINDRICAL_SURFACE('',#101488,0.0999999999999994) ;
#15736=CYLINDRICAL_SURFACE('',#101490,0.1) ;
#15737=CYLINDRICAL_SURFACE('',#101493,0.0999999999999994) ;
#15738=CYLINDRICAL_SURFACE('',#101499,0.0999999999999994) ;
#15739=CYLINDRICAL_SURFACE('',#101501,0.0999999999999994) ;
#15740=CYLINDRICAL_SURFACE('',#101503,0.0999999999999994) ;
#15741=CYLINDRICAL_SURFACE('',#101505,0.0999999999999994) ;
#15742=CYLINDRICAL_SURFACE('',#101511,0.1) ;
#15743=CYLINDRICAL_SURFACE('',#101512,0.0999999999999994) ;
#15744=CYLINDRICAL_SURFACE('',#101521,0.0999999999999998) ;
#15745=CYLINDRICAL_SURFACE('',#101523,0.0999999999999998) ;
#15746=CYLINDRICAL_SURFACE('',#101525,0.0999999999999994) ;
#15747=CYLINDRICAL_SURFACE('',#101528,0.0999999999999998) ;
#15748=CYLINDRICAL_SURFACE('',#101530,0.1) ;
#15749=CYLINDRICAL_SURFACE('',#101532,0.0999999999999994) ;
#15750=CYLINDRICAL_SURFACE('',#101543,0.0999999999999998) ;
#15751=CYLINDRICAL_SURFACE('',#101545,0.0999999999999998) ;
#15752=CYLINDRICAL_SURFACE('',#101547,0.0999999999999998) ;
#15753=CYLINDRICAL_SURFACE('',#101549,0.0999999999999998) ;
#15754=CYLINDRICAL_SURFACE('',#101555,0.0999999999999994) ;
#15755=CYLINDRICAL_SURFACE('',#101556,0.0999999999999994) ;
#15756=CYLINDRICAL_SURFACE('',#101558,0.0999999999999998) ;
#15757=CYLINDRICAL_SURFACE('',#101561,0.0999999999999994) ;
#15758=CYLINDRICAL_SURFACE('',#101567,0.0999999999999994) ;
#15759=CYLINDRICAL_SURFACE('',#101569,0.0999999999999994) ;
#15760=CYLINDRICAL_SURFACE('',#101571,0.0999999999999994) ;
#15761=CYLINDRICAL_SURFACE('',#101573,0.0999999999999994) ;
#15762=CYLINDRICAL_SURFACE('',#101579,0.0999999999999998) ;
#15763=CYLINDRICAL_SURFACE('',#101580,0.0999999999999994) ;
#15764=CYLINDRICAL_SURFACE('',#101587,0.0999999999999994) ;
#15765=CYLINDRICAL_SURFACE('',#101589,0.0999999999999994) ;
#15766=CYLINDRICAL_SURFACE('',#101595,0.0999999999999994) ;
#15767=CYLINDRICAL_SURFACE('',#101596,0.0999999999999995) ;
#15768=CYLINDRICAL_SURFACE('',#101597,0.0999999999999995) ;
#15769=CYLINDRICAL_SURFACE('',#101598,0.0999999999999995) ;
#15770=CYLINDRICAL_SURFACE('',#101599,0.0999999999999995) ;
#15771=CYLINDRICAL_SURFACE('',#101604,0.0999999999999994) ;
#15772=CYLINDRICAL_SURFACE('',#101606,0.0999999999999994) ;
#15773=CYLINDRICAL_SURFACE('',#101610,0.0999999999999994) ;
#15774=CYLINDRICAL_SURFACE('',#101621,0.0999999999999994) ;
#15775=CYLINDRICAL_SURFACE('',#101624,0.0999999999999994) ;
#15776=CYLINDRICAL_SURFACE('',#101626,0.0999999999999998) ;
#15777=CYLINDRICAL_SURFACE('',#101630,0.0999999999999994) ;
#15778=CYLINDRICAL_SURFACE('',#101632,0.0999999999999994) ;
#15779=CYLINDRICAL_SURFACE('',#101634,0.0999999999999994) ;
#15780=CYLINDRICAL_SURFACE('',#101643,0.1) ;
#15781=CYLINDRICAL_SURFACE('',#101646,0.0999999999999994) ;
#15782=CYLINDRICAL_SURFACE('',#101648,0.0999999999999998) ;
#15783=CYLINDRICAL_SURFACE('',#101650,0.0999999999999994) ;
#15784=CYLINDRICAL_SURFACE('',#101659,0.0999999999999994) ;
#15785=CYLINDRICAL_SURFACE('',#101661,0.1) ;
#15786=CYLINDRICAL_SURFACE('',#101663,0.0999999999999998) ;
#15787=CYLINDRICAL_SURFACE('',#101665,0.0999999999999994) ;
#15788=CYLINDRICAL_SURFACE('',#101671,0.0999999999999998) ;
#15789=CYLINDRICAL_SURFACE('',#101673,0.1) ;
#15790=CYLINDRICAL_SURFACE('',#101675,0.1) ;
#15791=CYLINDRICAL_SURFACE('',#101678,0.1) ;
#15792=CYLINDRICAL_SURFACE('',#101685,0.0999999999999994) ;
#15793=CYLINDRICAL_SURFACE('',#101687,0.0999999999999994) ;
#15794=CYLINDRICAL_SURFACE('',#101694,0.0999999999999994) ;
#15795=CYLINDRICAL_SURFACE('',#101696,0.0999999999999994) ;
#15796=CYLINDRICAL_SURFACE('',#101698,0.0999999999999998) ;
#15797=CYLINDRICAL_SURFACE('',#101700,0.0999999999999994) ;
#15798=CYLINDRICAL_SURFACE('',#101706,0.1) ;
#15799=CYLINDRICAL_SURFACE('',#101708,0.0999999999999994) ;
#15800=CYLINDRICAL_SURFACE('',#101712,0.0999999999999994) ;
#15801=CYLINDRICAL_SURFACE('',#101716,0.1) ;
#15802=CYLINDRICAL_SURFACE('',#101718,0.0999999999999994) ;
#15803=CYLINDRICAL_SURFACE('',#101722,0.0999999999999994) ;
#15804=CYLINDRICAL_SURFACE('',#101724,0.1) ;
#15805=CYLINDRICAL_SURFACE('',#101728,0.1) ;
#15806=CYLINDRICAL_SURFACE('',#101733,0.0999999999999998) ;
#15807=CYLINDRICAL_SURFACE('',#101735,0.1) ;
#15808=CYLINDRICAL_SURFACE('',#101739,0.0999999999999994) ;
#15809=CYLINDRICAL_SURFACE('',#101741,0.0999999999999994) ;
#15810=CYLINDRICAL_SURFACE('',#101745,0.1) ;
#15811=CYLINDRICAL_SURFACE('',#101751,0.1) ;
#15812=CYLINDRICAL_SURFACE('',#101753,0.0999999999999994) ;
#15813=CYLINDRICAL_SURFACE('',#101759,0.0999999999999994) ;
#15814=CYLINDRICAL_SURFACE('',#101761,0.0999999999999994) ;
#15815=CYLINDRICAL_SURFACE('',#101764,0.0999999999999994) ;
#15816=CYLINDRICAL_SURFACE('',#101766,0.1) ;
#15817=CYLINDRICAL_SURFACE('',#101769,0.0999999999999994) ;
#15818=CYLINDRICAL_SURFACE('',#101775,0.0999999999999994) ;
#15819=CYLINDRICAL_SURFACE('',#101777,0.0999999999999994) ;
#15820=CYLINDRICAL_SURFACE('',#101779,0.0999999999999994) ;
#15821=CYLINDRICAL_SURFACE('',#101781,0.0999999999999994) ;
#15822=CYLINDRICAL_SURFACE('',#101787,0.1) ;
#15823=CYLINDRICAL_SURFACE('',#101788,0.0999999999999994) ;
#15824=CYLINDRICAL_SURFACE('',#101797,0.0999999999999998) ;
#15825=CYLINDRICAL_SURFACE('',#101799,0.0999999999999998) ;
#15826=CYLINDRICAL_SURFACE('',#101801,0.0999999999999994) ;
#15827=CYLINDRICAL_SURFACE('',#101804,0.0999999999999998) ;
#15828=CYLINDRICAL_SURFACE('',#101806,0.1) ;
#15829=CYLINDRICAL_SURFACE('',#101808,0.0999999999999994) ;
#15830=CYLINDRICAL_SURFACE('',#101819,0.0999999999999998) ;
#15831=CYLINDRICAL_SURFACE('',#101821,0.0999999999999998) ;
#15832=CYLINDRICAL_SURFACE('',#101823,0.0999999999999998) ;
#15833=CYLINDRICAL_SURFACE('',#101825,0.0999999999999998) ;
#15834=CYLINDRICAL_SURFACE('',#101831,0.0999999999999994) ;
#15835=CYLINDRICAL_SURFACE('',#101832,0.0999999999999994) ;
#15836=CYLINDRICAL_SURFACE('',#101834,0.0999999999999998) ;
#15837=CYLINDRICAL_SURFACE('',#101837,0.0999999999999994) ;
#15838=CYLINDRICAL_SURFACE('',#101843,0.0999999999999994) ;
#15839=CYLINDRICAL_SURFACE('',#101845,0.0999999999999994) ;
#15840=CYLINDRICAL_SURFACE('',#101847,0.0999999999999994) ;
#15841=CYLINDRICAL_SURFACE('',#101849,0.0999999999999994) ;
#15842=CYLINDRICAL_SURFACE('',#101855,0.0999999999999998) ;
#15843=CYLINDRICAL_SURFACE('',#101856,0.0999999999999994) ;
#15844=CYLINDRICAL_SURFACE('',#101863,0.0999999999999994) ;
#15845=CYLINDRICAL_SURFACE('',#101865,0.0999999999999994) ;
#15846=CYLINDRICAL_SURFACE('',#101871,0.0999999999999994) ;
#15847=CYLINDRICAL_SURFACE('',#101872,0.0999999999999995) ;
#15848=CYLINDRICAL_SURFACE('',#101873,0.0999999999999995) ;
#15849=CYLINDRICAL_SURFACE('',#101874,0.0999999999999995) ;
#15850=CYLINDRICAL_SURFACE('',#101875,0.0999999999999995) ;
#15851=CYLINDRICAL_SURFACE('',#101880,0.0999999999999994) ;
#15852=CYLINDRICAL_SURFACE('',#101882,0.0999999999999994) ;
#15853=CYLINDRICAL_SURFACE('',#101886,0.0999999999999994) ;
#15854=CYLINDRICAL_SURFACE('',#101897,0.0999999999999994) ;
#15855=CYLINDRICAL_SURFACE('',#101900,0.0999999999999994) ;
#15856=CYLINDRICAL_SURFACE('',#101902,0.0999999999999998) ;
#15857=CYLINDRICAL_SURFACE('',#101906,0.0999999999999994) ;
#15858=CYLINDRICAL_SURFACE('',#101908,0.0999999999999994) ;
#15859=CYLINDRICAL_SURFACE('',#101910,0.0999999999999994) ;
#15860=CYLINDRICAL_SURFACE('',#101919,0.1) ;
#15861=CYLINDRICAL_SURFACE('',#101922,0.0999999999999994) ;
#15862=CYLINDRICAL_SURFACE('',#101924,0.0999999999999998) ;
#15863=CYLINDRICAL_SURFACE('',#101926,0.0999999999999994) ;
#15864=CYLINDRICAL_SURFACE('',#101935,0.0999999999999994) ;
#15865=CYLINDRICAL_SURFACE('',#101937,0.1) ;
#15866=CYLINDRICAL_SURFACE('',#101939,0.0999999999999998) ;
#15867=CYLINDRICAL_SURFACE('',#101941,0.0999999999999994) ;
#15868=CYLINDRICAL_SURFACE('',#101947,0.0999999999999998) ;
#15869=CYLINDRICAL_SURFACE('',#101949,0.1) ;
#15870=CYLINDRICAL_SURFACE('',#101951,0.1) ;
#15871=CYLINDRICAL_SURFACE('',#101954,0.1) ;
#15872=CYLINDRICAL_SURFACE('',#101961,0.0999999999999994) ;
#15873=CYLINDRICAL_SURFACE('',#101963,0.0999999999999994) ;
#15874=CYLINDRICAL_SURFACE('',#101970,0.0999999999999994) ;
#15875=CYLINDRICAL_SURFACE('',#101972,0.0999999999999994) ;
#15876=CYLINDRICAL_SURFACE('',#101974,0.0999999999999998) ;
#15877=CYLINDRICAL_SURFACE('',#101976,0.0999999999999994) ;
#15878=CYLINDRICAL_SURFACE('',#101982,0.1) ;
#15879=CYLINDRICAL_SURFACE('',#101984,0.0999999999999994) ;
#15880=CYLINDRICAL_SURFACE('',#101988,0.0999999999999994) ;
#15881=CYLINDRICAL_SURFACE('',#101992,0.1) ;
#15882=CYLINDRICAL_SURFACE('',#101994,0.0999999999999994) ;
#15883=CYLINDRICAL_SURFACE('',#101998,0.0999999999999994) ;
#15884=CYLINDRICAL_SURFACE('',#102000,0.1) ;
#15885=CYLINDRICAL_SURFACE('',#102004,0.1) ;
#15886=CYLINDRICAL_SURFACE('',#102009,0.0999999999999998) ;
#15887=CYLINDRICAL_SURFACE('',#102011,0.1) ;
#15888=CYLINDRICAL_SURFACE('',#102015,0.0999999999999994) ;
#15889=CYLINDRICAL_SURFACE('',#102017,0.0999999999999994) ;
#15890=CYLINDRICAL_SURFACE('',#102021,0.1) ;
#15891=CYLINDRICAL_SURFACE('',#102027,0.1) ;
#15892=CYLINDRICAL_SURFACE('',#102029,0.0999999999999994) ;
#15893=CYLINDRICAL_SURFACE('',#102035,0.0999999999999994) ;
#15894=CYLINDRICAL_SURFACE('',#102037,0.0999999999999994) ;
#15895=CYLINDRICAL_SURFACE('',#102040,0.0999999999999994) ;
#15896=CYLINDRICAL_SURFACE('',#102042,0.1) ;
#15897=CYLINDRICAL_SURFACE('',#102045,0.0999999999999994) ;
#15898=CYLINDRICAL_SURFACE('',#102051,0.0999999999999994) ;
#15899=CYLINDRICAL_SURFACE('',#102053,0.0999999999999994) ;
#15900=CYLINDRICAL_SURFACE('',#102055,0.0999999999999994) ;
#15901=CYLINDRICAL_SURFACE('',#102057,0.0999999999999994) ;
#15902=CYLINDRICAL_SURFACE('',#102063,0.1) ;
#15903=CYLINDRICAL_SURFACE('',#102064,0.0999999999999994) ;
#15904=CYLINDRICAL_SURFACE('',#102073,0.0999999999999998) ;
#15905=CYLINDRICAL_SURFACE('',#102075,0.0999999999999998) ;
#15906=CYLINDRICAL_SURFACE('',#102077,0.0999999999999994) ;
#15907=CYLINDRICAL_SURFACE('',#102080,0.0999999999999998) ;
#15908=CYLINDRICAL_SURFACE('',#102082,0.1) ;
#15909=CYLINDRICAL_SURFACE('',#102084,0.0999999999999994) ;
#15910=CYLINDRICAL_SURFACE('',#102095,0.0999999999999998) ;
#15911=CYLINDRICAL_SURFACE('',#102097,0.0999999999999998) ;
#15912=CYLINDRICAL_SURFACE('',#102099,0.0999999999999998) ;
#15913=CYLINDRICAL_SURFACE('',#102101,0.0999999999999998) ;
#15914=CYLINDRICAL_SURFACE('',#102107,0.0999999999999994) ;
#15915=CYLINDRICAL_SURFACE('',#102108,0.0999999999999994) ;
#15916=CYLINDRICAL_SURFACE('',#102110,0.0999999999999998) ;
#15917=CYLINDRICAL_SURFACE('',#102113,0.0999999999999994) ;
#15918=CYLINDRICAL_SURFACE('',#102119,0.0999999999999994) ;
#15919=CYLINDRICAL_SURFACE('',#102121,0.0999999999999994) ;
#15920=CYLINDRICAL_SURFACE('',#102123,0.0999999999999994) ;
#15921=CYLINDRICAL_SURFACE('',#102125,0.0999999999999994) ;
#15922=CYLINDRICAL_SURFACE('',#102131,0.0999999999999998) ;
#15923=CYLINDRICAL_SURFACE('',#102132,0.0999999999999994) ;
#15924=CYLINDRICAL_SURFACE('',#102139,0.0999999999999994) ;
#15925=CYLINDRICAL_SURFACE('',#102141,0.0999999999999994) ;
#15926=CYLINDRICAL_SURFACE('',#102147,0.0999999999999994) ;
#15927=CYLINDRICAL_SURFACE('',#102148,0.0999999999999995) ;
#15928=CYLINDRICAL_SURFACE('',#102149,0.0999999999999995) ;
#15929=CYLINDRICAL_SURFACE('',#102150,0.0999999999999995) ;
#15930=CYLINDRICAL_SURFACE('',#102151,0.0999999999999995) ;
#15931=CYLINDRICAL_SURFACE('',#102156,0.0999999999999994) ;
#15932=CYLINDRICAL_SURFACE('',#102158,0.0999999999999994) ;
#15933=CYLINDRICAL_SURFACE('',#102162,0.0999999999999994) ;
#15934=CYLINDRICAL_SURFACE('',#102173,0.0999999999999994) ;
#15935=CYLINDRICAL_SURFACE('',#102176,0.0999999999999994) ;
#15936=CYLINDRICAL_SURFACE('',#102178,0.0999999999999998) ;
#15937=CYLINDRICAL_SURFACE('',#102182,0.100000000000003) ;
#15938=CYLINDRICAL_SURFACE('',#102184,0.0999999999999994) ;
#15939=CYLINDRICAL_SURFACE('',#102186,0.100000000000003) ;
#15940=CYLINDRICAL_SURFACE('',#102195,0.1) ;
#15941=CYLINDRICAL_SURFACE('',#102198,0.0999999999999994) ;
#15942=CYLINDRICAL_SURFACE('',#102200,0.0999999999999998) ;
#15943=CYLINDRICAL_SURFACE('',#102202,0.100000000000003) ;
#15944=CYLINDRICAL_SURFACE('',#102211,0.0999999999999994) ;
#15945=CYLINDRICAL_SURFACE('',#102213,0.1) ;
#15946=CYLINDRICAL_SURFACE('',#102215,0.0999999999999998) ;
#15947=CYLINDRICAL_SURFACE('',#102217,0.100000000000003) ;
#15948=CYLINDRICAL_SURFACE('',#102223,0.0999999999999998) ;
#15949=CYLINDRICAL_SURFACE('',#102225,0.1) ;
#15950=CYLINDRICAL_SURFACE('',#102227,0.1) ;
#15951=CYLINDRICAL_SURFACE('',#102230,0.1) ;
#15952=CYLINDRICAL_SURFACE('',#102237,0.100000000000003) ;
#15953=CYLINDRICAL_SURFACE('',#102239,0.0999999999999994) ;
#15954=CYLINDRICAL_SURFACE('',#102246,0.0999999999999994) ;
#15955=CYLINDRICAL_SURFACE('',#102248,0.0999999999999994) ;
#15956=CYLINDRICAL_SURFACE('',#102250,0.0999999999999998) ;
#15957=CYLINDRICAL_SURFACE('',#102252,0.100000000000003) ;
#15958=CYLINDRICAL_SURFACE('',#102258,0.1) ;
#15959=CYLINDRICAL_SURFACE('',#102260,0.100000000000003) ;
#15960=CYLINDRICAL_SURFACE('',#102264,0.100000000000003) ;
#15961=CYLINDRICAL_SURFACE('',#102268,0.1) ;
#15962=CYLINDRICAL_SURFACE('',#102270,0.0999999999999994) ;
#15963=CYLINDRICAL_SURFACE('',#102274,0.0999999999999994) ;
#15964=CYLINDRICAL_SURFACE('',#102276,0.1) ;
#15965=CYLINDRICAL_SURFACE('',#102280,0.1) ;
#15966=CYLINDRICAL_SURFACE('',#102285,0.0999999999999998) ;
#15967=CYLINDRICAL_SURFACE('',#102287,0.1) ;
#15968=CYLINDRICAL_SURFACE('',#102291,0.100000000000003) ;
#15969=CYLINDRICAL_SURFACE('',#102293,0.0999999999999994) ;
#15970=CYLINDRICAL_SURFACE('',#102297,0.1) ;
#15971=CYLINDRICAL_SURFACE('',#102303,0.1) ;
#15972=CYLINDRICAL_SURFACE('',#102305,0.0999999999999994) ;
#15973=CYLINDRICAL_SURFACE('',#102311,0.0999999999999994) ;
#15974=CYLINDRICAL_SURFACE('',#102313,0.0999999999999994) ;
#15975=CYLINDRICAL_SURFACE('',#102316,0.0999999999999994) ;
#15976=CYLINDRICAL_SURFACE('',#102318,0.1) ;
#15977=CYLINDRICAL_SURFACE('',#102321,0.0999999999999994) ;
#15978=CYLINDRICAL_SURFACE('',#102327,0.0999999999999994) ;
#15979=CYLINDRICAL_SURFACE('',#102329,0.0999999999999994) ;
#15980=CYLINDRICAL_SURFACE('',#102331,0.0999999999999994) ;
#15981=CYLINDRICAL_SURFACE('',#102333,0.0999999999999994) ;
#15982=CYLINDRICAL_SURFACE('',#102339,0.1) ;
#15983=CYLINDRICAL_SURFACE('',#102340,0.100000000000003) ;
#15984=CYLINDRICAL_SURFACE('',#102349,0.0999999999999998) ;
#15985=CYLINDRICAL_SURFACE('',#102351,0.0999999999999998) ;
#15986=CYLINDRICAL_SURFACE('',#102353,0.100000000000003) ;
#15987=CYLINDRICAL_SURFACE('',#102356,0.0999999999999998) ;
#15988=CYLINDRICAL_SURFACE('',#102358,0.1) ;
#15989=CYLINDRICAL_SURFACE('',#102360,0.0999999999999994) ;
#15990=CYLINDRICAL_SURFACE('',#102371,0.0999999999999998) ;
#15991=CYLINDRICAL_SURFACE('',#102373,0.0999999999999998) ;
#15992=CYLINDRICAL_SURFACE('',#102375,0.0999999999999998) ;
#15993=CYLINDRICAL_SURFACE('',#102377,0.0999999999999998) ;
#15994=CYLINDRICAL_SURFACE('',#102383,0.0999999999999994) ;
#15995=CYLINDRICAL_SURFACE('',#102384,0.0999999999999994) ;
#15996=CYLINDRICAL_SURFACE('',#102386,0.0999999999999998) ;
#15997=CYLINDRICAL_SURFACE('',#102389,0.0999999999999994) ;
#15998=CYLINDRICAL_SURFACE('',#102395,0.0999999999999994) ;
#15999=CYLINDRICAL_SURFACE('',#102397,0.0999999999999994) ;
#16000=CYLINDRICAL_SURFACE('',#102399,0.0999999999999994) ;
#16001=CYLINDRICAL_SURFACE('',#102401,0.0999999999999994) ;
#16002=CYLINDRICAL_SURFACE('',#102407,0.0999999999999998) ;
#16003=CYLINDRICAL_SURFACE('',#102408,0.0999999999999994) ;
#16004=CYLINDRICAL_SURFACE('',#102415,0.0999999999999994) ;
#16005=CYLINDRICAL_SURFACE('',#102417,0.0999999999999994) ;
#16006=CYLINDRICAL_SURFACE('',#102423,0.0999999999999994) ;
#16007=CYLINDRICAL_SURFACE('',#102424,0.0999999999999995) ;
#16008=CYLINDRICAL_SURFACE('',#102425,0.0999999999999995) ;
#16009=CYLINDRICAL_SURFACE('',#102426,0.0999999999999995) ;
#16010=CYLINDRICAL_SURFACE('',#102427,0.0999999999999995) ;
#16011=CYLINDRICAL_SURFACE('',#102432,0.0999999999999994) ;
#16012=CYLINDRICAL_SURFACE('',#102434,0.100000000000003) ;
#16013=CYLINDRICAL_SURFACE('',#102438,0.100000000000003) ;
#16014=CYLINDRICAL_SURFACE('',#102449,0.0999999999999994) ;
#16015=CYLINDRICAL_SURFACE('',#102452,0.100000000000003) ;
#16016=CYLINDRICAL_SURFACE('',#102454,0.0999999999999998) ;
#16017=CYLINDRICAL_SURFACE('',#102458,0.100000000000003) ;
#16018=CYLINDRICAL_SURFACE('',#102460,0.0999999999999994) ;
#16019=CYLINDRICAL_SURFACE('',#102462,0.100000000000003) ;
#16020=CYLINDRICAL_SURFACE('',#102471,0.1) ;
#16021=CYLINDRICAL_SURFACE('',#102474,0.100000000000003) ;
#16022=CYLINDRICAL_SURFACE('',#102476,0.0999999999999998) ;
#16023=CYLINDRICAL_SURFACE('',#102478,0.100000000000003) ;
#16024=CYLINDRICAL_SURFACE('',#102487,0.100000000000003) ;
#16025=CYLINDRICAL_SURFACE('',#102489,0.1) ;
#16026=CYLINDRICAL_SURFACE('',#102491,0.0999999999999998) ;
#16027=CYLINDRICAL_SURFACE('',#102493,0.100000000000003) ;
#16028=CYLINDRICAL_SURFACE('',#102499,0.0999999999999998) ;
#16029=CYLINDRICAL_SURFACE('',#102501,0.1) ;
#16030=CYLINDRICAL_SURFACE('',#102503,0.1) ;
#16031=CYLINDRICAL_SURFACE('',#102506,0.1) ;
#16032=CYLINDRICAL_SURFACE('',#102513,0.100000000000003) ;
#16033=CYLINDRICAL_SURFACE('',#102515,0.100000000000003) ;
#16034=CYLINDRICAL_SURFACE('',#102522,0.100000000000003) ;
#16035=CYLINDRICAL_SURFACE('',#102524,0.100000000000003) ;
#16036=CYLINDRICAL_SURFACE('',#102526,0.0999999999999998) ;
#16037=CYLINDRICAL_SURFACE('',#102528,0.100000000000003) ;
#16038=CYLINDRICAL_SURFACE('',#102534,0.1) ;
#16039=CYLINDRICAL_SURFACE('',#102536,0.100000000000003) ;
#16040=CYLINDRICAL_SURFACE('',#102540,0.100000000000003) ;
#16041=CYLINDRICAL_SURFACE('',#102544,0.1) ;
#16042=CYLINDRICAL_SURFACE('',#102546,0.0999999999999994) ;
#16043=CYLINDRICAL_SURFACE('',#102550,0.100000000000003) ;
#16044=CYLINDRICAL_SURFACE('',#102552,0.1) ;
#16045=CYLINDRICAL_SURFACE('',#102556,0.1) ;
#16046=CYLINDRICAL_SURFACE('',#102561,0.0999999999999998) ;
#16047=CYLINDRICAL_SURFACE('',#102563,0.1) ;
#16048=CYLINDRICAL_SURFACE('',#102567,0.100000000000003) ;
#16049=CYLINDRICAL_SURFACE('',#102569,0.0999999999999994) ;
#16050=CYLINDRICAL_SURFACE('',#102573,0.1) ;
#16051=CYLINDRICAL_SURFACE('',#102579,0.1) ;
#16052=CYLINDRICAL_SURFACE('',#102581,0.100000000000003) ;
#16053=CYLINDRICAL_SURFACE('',#102587,0.100000000000003) ;
#16054=CYLINDRICAL_SURFACE('',#102589,0.0999999999999994) ;
#16055=CYLINDRICAL_SURFACE('',#102592,0.100000000000003) ;
#16056=CYLINDRICAL_SURFACE('',#102594,0.1) ;
#16057=CYLINDRICAL_SURFACE('',#102597,0.100000000000003) ;
#16058=CYLINDRICAL_SURFACE('',#102603,0.100000000000003) ;
#16059=CYLINDRICAL_SURFACE('',#102605,0.100000000000003) ;
#16060=CYLINDRICAL_SURFACE('',#102607,0.100000000000003) ;
#16061=CYLINDRICAL_SURFACE('',#102609,0.100000000000003) ;
#16062=CYLINDRICAL_SURFACE('',#102615,0.1) ;
#16063=CYLINDRICAL_SURFACE('',#102616,0.100000000000003) ;
#16064=CYLINDRICAL_SURFACE('',#102625,0.0999999999999998) ;
#16065=CYLINDRICAL_SURFACE('',#102627,0.0999999999999998) ;
#16066=CYLINDRICAL_SURFACE('',#102629,0.100000000000003) ;
#16067=CYLINDRICAL_SURFACE('',#102632,0.0999999999999998) ;
#16068=CYLINDRICAL_SURFACE('',#102634,0.1) ;
#16069=CYLINDRICAL_SURFACE('',#102636,0.100000000000003) ;
#16070=CYLINDRICAL_SURFACE('',#102647,0.0999999999999998) ;
#16071=CYLINDRICAL_SURFACE('',#102649,0.0999999999999998) ;
#16072=CYLINDRICAL_SURFACE('',#102651,0.0999999999999998) ;
#16073=CYLINDRICAL_SURFACE('',#102653,0.0999999999999998) ;
#16074=CYLINDRICAL_SURFACE('',#102659,0.100000000000003) ;
#16075=CYLINDRICAL_SURFACE('',#102660,0.100000000000003) ;
#16076=CYLINDRICAL_SURFACE('',#102662,0.0999999999999998) ;
#16077=CYLINDRICAL_SURFACE('',#102665,0.100000000000003) ;
#16078=CYLINDRICAL_SURFACE('',#102671,0.100000000000003) ;
#16079=CYLINDRICAL_SURFACE('',#102673,0.100000000000003) ;
#16080=CYLINDRICAL_SURFACE('',#102675,0.100000000000003) ;
#16081=CYLINDRICAL_SURFACE('',#102677,0.100000000000003) ;
#16082=CYLINDRICAL_SURFACE('',#102683,0.0999999999999998) ;
#16083=CYLINDRICAL_SURFACE('',#102684,0.0999999999999994) ;
#16084=CYLINDRICAL_SURFACE('',#102691,0.100000000000003) ;
#16085=CYLINDRICAL_SURFACE('',#102693,0.100000000000003) ;
#16086=CYLINDRICAL_SURFACE('',#102699,0.0999999999999994) ;
#16087=CYLINDRICAL_SURFACE('',#102700,0.0999999999999995) ;
#16088=CYLINDRICAL_SURFACE('',#102701,0.0999999999999995) ;
#16089=CYLINDRICAL_SURFACE('',#102702,0.0999999999999995) ;
#16090=CYLINDRICAL_SURFACE('',#102703,0.0999999999999995) ;
#16091=CYLINDRICAL_SURFACE('',#102704,0.0999999999999998) ;
#16092=CYLINDRICAL_SURFACE('',#102707,0.0999999999999998) ;
#16093=CYLINDRICAL_SURFACE('',#102710,0.0999999999999998) ;
#16094=CYLINDRICAL_SURFACE('',#102713,0.0999999999999998) ;
#16095=CYLINDRICAL_SURFACE('',#102716,0.0999999999999998) ;
#16096=CYLINDRICAL_SURFACE('',#102719,0.0999999999999998) ;
#16097=CYLINDRICAL_SURFACE('',#102722,0.0999999999999998) ;
#16098=CYLINDRICAL_SURFACE('',#102725,0.0999999999999998) ;
#16099=CYLINDRICAL_SURFACE('',#102728,0.0999999999999998) ;
#16100=CYLINDRICAL_SURFACE('',#102733,0.0999999999999998) ;
#16101=CYLINDRICAL_SURFACE('',#102741,0.0999999999999998) ;
#16102=CYLINDRICAL_SURFACE('',#102748,0.0999999999999998) ;
#16103=CYLINDRICAL_SURFACE('',#102755,0.0999999999999998) ;
#16104=CYLINDRICAL_SURFACE('',#102762,0.0999999999999998) ;
#16105=CYLINDRICAL_SURFACE('',#102769,0.0999999999999998) ;
#16106=CYLINDRICAL_SURFACE('',#102776,0.0999999999999998) ;
#16107=CYLINDRICAL_SURFACE('',#102783,0.0999999999999998) ;
#16108=CYLINDRICAL_SURFACE('',#102788,0.0999999999999998) ;
#16109=CYLINDRICAL_SURFACE('',#102795,0.1) ;
#16110=CYLINDRICAL_SURFACE('',#102801,0.0999999999999998) ;
#16111=CYLINDRICAL_SURFACE('',#102807,0.0999999999999994) ;
#16112=CYLINDRICAL_SURFACE('',#102813,0.1) ;
#16113=CYLINDRICAL_SURFACE('',#102819,0.0999999999999994) ;
#16114=CYLINDRICAL_SURFACE('',#102825,0.0999999999999994) ;
#16115=CYLINDRICAL_SURFACE('',#102831,0.0999999999999994) ;
#16116=CYLINDRICAL_SURFACE('',#102837,0.0999999999999994) ;
#16117=CYLINDRICAL_SURFACE('',#102843,0.0999999999999994) ;
#16118=CYLINDRICAL_SURFACE('',#102849,0.0999999999999994) ;
#16119=CYLINDRICAL_SURFACE('',#102855,0.0999999999999994) ;
#16120=CYLINDRICAL_SURFACE('',#102861,0.0999999999999994) ;
#16121=CYLINDRICAL_SURFACE('',#102867,0.0999999999999994) ;
#16122=CYLINDRICAL_SURFACE('',#102873,0.0999999999999994) ;
#16123=CYLINDRICAL_SURFACE('',#102879,0.100000000000003) ;
#16124=CYLINDRICAL_SURFACE('',#102885,0.0999999999999994) ;
#16125=CYLINDRICAL_SURFACE('',#102891,0.100000000000003) ;
#16126=CYLINDRICAL_SURFACE('',#102897,0.100000000000003) ;
#16127=CYLINDRICAL_SURFACE('',#102973,2.25) ;
#16128=CYLINDRICAL_SURFACE('',#102975,2.25) ;
#16129=CYLINDRICAL_SURFACE('',#102977,2.25) ;
#16130=CYLINDRICAL_SURFACE('',#102979,2.25) ;
#16131=CYLINDRICAL_SURFACE('',#102981,2.25) ;
#16132=CYLINDRICAL_SURFACE('',#102983,2.25) ;
#16133=CYLINDRICAL_SURFACE('',#102987,0.0999999999999998) ;
#16134=CYLINDRICAL_SURFACE('',#102991,0.0999999999999998) ;
#16135=CYLINDRICAL_SURFACE('',#102995,0.100000000000003) ;
#16136=CYLINDRICAL_SURFACE('',#102999,0.0999999999999998) ;
#16137=CYLINDRICAL_SURFACE('',#103006,0.1) ;
#16138=CYLINDRICAL_SURFACE('',#103008,0.0999999999999998) ;
#16139=CYLINDRICAL_SURFACE('',#103010,0.0999999999999998) ;
#16140=CYLINDRICAL_SURFACE('',#103017,0.0999999999999998) ;
#16141=CYLINDRICAL_SURFACE('',#103019,0.0999999999999998) ;
#16142=CYLINDRICAL_SURFACE('',#103021,0.0999999999999998) ;
#16143=CYLINDRICAL_SURFACE('',#103024,0.1) ;
#16144=CYLINDRICAL_SURFACE('',#103035,0.0999999999999998) ;
#16145=CYLINDRICAL_SURFACE('',#103040,0.0999999999999998) ;
#16146=CYLINDRICAL_SURFACE('',#103045,0.1) ;
#16147=CYLINDRICAL_SURFACE('',#103047,0.0999999999999998) ;
#16148=CYLINDRICAL_SURFACE('',#103054,0.1) ;
#16149=CYLINDRICAL_SURFACE('',#103056,0.0999999999999998) ;
#16150=CYLINDRICAL_SURFACE('',#103058,0.0999999999999998) ;
#16151=CYLINDRICAL_SURFACE('',#103060,0.0999999999999998) ;
#16152=CYLINDRICAL_SURFACE('',#103066,0.0999999999999998) ;
#16153=CYLINDRICAL_SURFACE('',#103068,0.0999999999999998) ;
#16154=CYLINDRICAL_SURFACE('',#103072,0.1) ;
#16689=SPHERICAL_SURFACE('',#98811,0.1) ;
#16690=SPHERICAL_SURFACE('',#98831,0.1) ;
#16691=SPHERICAL_SURFACE('',#98834,0.1) ;
#16692=SPHERICAL_SURFACE('',#98839,0.1) ;
#16693=SPHERICAL_SURFACE('',#98860,0.1) ;
#16694=SPHERICAL_SURFACE('',#98862,0.1) ;
#16695=SPHERICAL_SURFACE('',#98878,0.1) ;
#16696=SPHERICAL_SURFACE('',#98894,0.1) ;
#16697=SPHERICAL_SURFACE('',#98900,0.1) ;
#16698=SPHERICAL_SURFACE('',#98915,0.1) ;
#16699=SPHERICAL_SURFACE('',#98935,0.1) ;
#16700=SPHERICAL_SURFACE('',#98938,0.1) ;
#16701=SPHERICAL_SURFACE('',#98948,0.1) ;
#16702=SPHERICAL_SURFACE('',#98962,0.1) ;
#16703=SPHERICAL_SURFACE('',#99008,0.1) ;
#16704=SPHERICAL_SURFACE('',#99010,0.1) ;
#16705=SPHERICAL_SURFACE('',#99022,0.1) ;
#16706=SPHERICAL_SURFACE('',#99024,0.1) ;
#16707=SPHERICAL_SURFACE('',#99034,0.1) ;
#16708=SPHERICAL_SURFACE('',#99036,0.1) ;
#16709=SPHERICAL_SURFACE('',#99046,0.1) ;
#16710=SPHERICAL_SURFACE('',#99048,0.1) ;
#16711=SPHERICAL_SURFACE('',#99053,0.1) ;
#16712=SPHERICAL_SURFACE('',#99063,0.1) ;
#16713=SPHERICAL_SURFACE('',#99075,0.1) ;
#16714=SPHERICAL_SURFACE('',#99087,0.1) ;
#16715=SPHERICAL_SURFACE('',#99116,0.1) ;
#16716=SPHERICAL_SURFACE('',#99118,0.1) ;
#16717=SPHERICAL_SURFACE('',#99130,0.1) ;
#16718=SPHERICAL_SURFACE('',#99132,0.1) ;
#16719=SPHERICAL_SURFACE('',#99142,0.1) ;
#16720=SPHERICAL_SURFACE('',#99144,0.1) ;
#16721=SPHERICAL_SURFACE('',#99154,0.1) ;
#16722=SPHERICAL_SURFACE('',#99156,0.1) ;
#16723=SPHERICAL_SURFACE('',#99162,0.1) ;
#16724=SPHERICAL_SURFACE('',#99164,0.1) ;
#16725=SPHERICAL_SURFACE('',#99170,0.1) ;
#16726=SPHERICAL_SURFACE('',#99172,0.1) ;
#16727=SPHERICAL_SURFACE('',#99193,0.1) ;
#16728=SPHERICAL_SURFACE('',#99199,0.1) ;
#16729=SPHERICAL_SURFACE('',#99942,0.1) ;
#16730=SPHERICAL_SURFACE('',#99958,0.1) ;
#16731=SPHERICAL_SURFACE('',#99964,0.1) ;
#16732=SPHERICAL_SURFACE('',#99979,0.1) ;
#16733=SPHERICAL_SURFACE('',#99999,0.1) ;
#16734=SPHERICAL_SURFACE('',#100002,0.1) ;
#16735=SPHERICAL_SURFACE('',#100012,0.1) ;
#16736=SPHERICAL_SURFACE('',#100023,0.1) ;
#16737=SPHERICAL_SURFACE('',#100165,0.1) ;
#16738=SPHERICAL_SURFACE('',#100167,0.1) ;
#16739=SPHERICAL_SURFACE('',#100179,0.1) ;
#16740=SPHERICAL_SURFACE('',#100181,0.1) ;
#16741=SPHERICAL_SURFACE('',#100191,0.1) ;
#16742=SPHERICAL_SURFACE('',#100193,0.1) ;
#16743=SPHERICAL_SURFACE('',#100203,0.1) ;
#16744=SPHERICAL_SURFACE('',#100205,0.1) ;
#16745=SPHERICAL_SURFACE('',#100210,0.1) ;
#16746=SPHERICAL_SURFACE('',#100220,0.1) ;
#16747=SPHERICAL_SURFACE('',#100232,0.1) ;
#16748=SPHERICAL_SURFACE('',#100244,0.1) ;
#16749=SPHERICAL_SURFACE('',#100433,0.1) ;
#16750=SPHERICAL_SURFACE('',#100435,0.1) ;
#16751=SPHERICAL_SURFACE('',#100447,0.1) ;
#16752=SPHERICAL_SURFACE('',#100449,0.1) ;
#16753=SPHERICAL_SURFACE('',#100459,0.1) ;
#16754=SPHERICAL_SURFACE('',#100461,0.1) ;
#16755=SPHERICAL_SURFACE('',#100471,0.1) ;
#16756=SPHERICAL_SURFACE('',#100473,0.1) ;
#16757=SPHERICAL_SURFACE('',#100479,0.1) ;
#16758=SPHERICAL_SURFACE('',#100481,0.1) ;
#16759=SPHERICAL_SURFACE('',#100487,0.1) ;
#16760=SPHERICAL_SURFACE('',#100489,0.1) ;
#16761=SPHERICAL_SURFACE('',#100496,0.1) ;
#16762=SPHERICAL_SURFACE('',#100509,0.1) ;
#16763=SPHERICAL_SURFACE('',#100514,0.1) ;
#16764=SPHERICAL_SURFACE('',#100537,0.1) ;
#16765=SPHERICAL_SURFACE('',#100548,0.1) ;
#16766=SPHERICAL_SURFACE('',#100550,0.1) ;
#16767=SPHERICAL_SURFACE('',#100565,0.1) ;
#16768=SPHERICAL_SURFACE('',#100579,0.1) ;
#16769=SPHERICAL_SURFACE('',#100586,0.1) ;
#16770=SPHERICAL_SURFACE('',#100598,0.1) ;
#16771=SPHERICAL_SURFACE('',#100600,0.1) ;
#16772=SPHERICAL_SURFACE('',#100606,0.1) ;
#16773=SPHERICAL_SURFACE('',#100616,0.1) ;
#16774=SPHERICAL_SURFACE('',#100622,0.1) ;
#16775=SPHERICAL_SURFACE('',#100633,0.1) ;
#16776=SPHERICAL_SURFACE('',#100639,0.1) ;
#16777=SPHERICAL_SURFACE('',#100667,0.1) ;
#16778=SPHERICAL_SURFACE('',#100669,0.1) ;
#16779=SPHERICAL_SURFACE('',#100679,0.1) ;
#16780=SPHERICAL_SURFACE('',#100681,0.1) ;
#16781=SPHERICAL_SURFACE('',#100709,0.1) ;
#16782=SPHERICAL_SURFACE('',#100711,0.1) ;
#16783=SPHERICAL_SURFACE('',#100723,0.1) ;
#16784=SPHERICAL_SURFACE('',#100725,0.1) ;
#16785=SPHERICAL_SURFACE('',#100735,0.1) ;
#16786=SPHERICAL_SURFACE('',#100737,0.1) ;
#16787=SPHERICAL_SURFACE('',#100747,0.1) ;
#16788=SPHERICAL_SURFACE('',#100749,0.1) ;
#16789=SPHERICAL_SURFACE('',#100755,0.1) ;
#16790=SPHERICAL_SURFACE('',#100757,0.1) ;
#16791=SPHERICAL_SURFACE('',#100763,0.1) ;
#16792=SPHERICAL_SURFACE('',#100765,0.1) ;
#16793=SPHERICAL_SURFACE('',#100772,0.1) ;
#16794=SPHERICAL_SURFACE('',#100785,0.1) ;
#16795=SPHERICAL_SURFACE('',#100790,0.1) ;
#16796=SPHERICAL_SURFACE('',#100813,0.1) ;
#16797=SPHERICAL_SURFACE('',#100824,0.1) ;
#16798=SPHERICAL_SURFACE('',#100826,0.1) ;
#16799=SPHERICAL_SURFACE('',#100841,0.1) ;
#16800=SPHERICAL_SURFACE('',#100855,0.1) ;
#16801=SPHERICAL_SURFACE('',#100862,0.1) ;
#16802=SPHERICAL_SURFACE('',#100874,0.1) ;
#16803=SPHERICAL_SURFACE('',#100876,0.1) ;
#16804=SPHERICAL_SURFACE('',#100882,0.1) ;
#16805=SPHERICAL_SURFACE('',#100892,0.1) ;
#16806=SPHERICAL_SURFACE('',#100898,0.1) ;
#16807=SPHERICAL_SURFACE('',#100909,0.1) ;
#16808=SPHERICAL_SURFACE('',#100915,0.1) ;
#16809=SPHERICAL_SURFACE('',#100943,0.1) ;
#16810=SPHERICAL_SURFACE('',#100945,0.1) ;
#16811=SPHERICAL_SURFACE('',#100955,0.1) ;
#16812=SPHERICAL_SURFACE('',#100957,0.1) ;
#16813=SPHERICAL_SURFACE('',#100985,0.1) ;
#16814=SPHERICAL_SURFACE('',#100987,0.1) ;
#16815=SPHERICAL_SURFACE('',#100999,0.1) ;
#16816=SPHERICAL_SURFACE('',#101001,0.1) ;
#16817=SPHERICAL_SURFACE('',#101011,0.1) ;
#16818=SPHERICAL_SURFACE('',#101013,0.1) ;
#16819=SPHERICAL_SURFACE('',#101023,0.1) ;
#16820=SPHERICAL_SURFACE('',#101025,0.1) ;
#16821=SPHERICAL_SURFACE('',#101031,0.1) ;
#16822=SPHERICAL_SURFACE('',#101033,0.1) ;
#16823=SPHERICAL_SURFACE('',#101039,0.1) ;
#16824=SPHERICAL_SURFACE('',#101041,0.1) ;
#16825=SPHERICAL_SURFACE('',#101048,0.1) ;
#16826=SPHERICAL_SURFACE('',#101061,0.1) ;
#16827=SPHERICAL_SURFACE('',#101066,0.1) ;
#16828=SPHERICAL_SURFACE('',#101089,0.1) ;
#16829=SPHERICAL_SURFACE('',#101100,0.1) ;
#16830=SPHERICAL_SURFACE('',#101102,0.1) ;
#16831=SPHERICAL_SURFACE('',#101117,0.1) ;
#16832=SPHERICAL_SURFACE('',#101131,0.1) ;
#16833=SPHERICAL_SURFACE('',#101138,0.1) ;
#16834=SPHERICAL_SURFACE('',#101150,0.1) ;
#16835=SPHERICAL_SURFACE('',#101152,0.1) ;
#16836=SPHERICAL_SURFACE('',#101158,0.1) ;
#16837=SPHERICAL_SURFACE('',#101168,0.1) ;
#16838=SPHERICAL_SURFACE('',#101174,0.1) ;
#16839=SPHERICAL_SURFACE('',#101185,0.1) ;
#16840=SPHERICAL_SURFACE('',#101191,0.1) ;
#16841=SPHERICAL_SURFACE('',#101219,0.1) ;
#16842=SPHERICAL_SURFACE('',#101221,0.1) ;
#16843=SPHERICAL_SURFACE('',#101231,0.1) ;
#16844=SPHERICAL_SURFACE('',#101233,0.1) ;
#16845=SPHERICAL_SURFACE('',#101261,0.1) ;
#16846=SPHERICAL_SURFACE('',#101263,0.1) ;
#16847=SPHERICAL_SURFACE('',#101275,0.1) ;
#16848=SPHERICAL_SURFACE('',#101277,0.1) ;
#16849=SPHERICAL_SURFACE('',#101287,0.1) ;
#16850=SPHERICAL_SURFACE('',#101289,0.1) ;
#16851=SPHERICAL_SURFACE('',#101299,0.1) ;
#16852=SPHERICAL_SURFACE('',#101301,0.1) ;
#16853=SPHERICAL_SURFACE('',#101307,0.1) ;
#16854=SPHERICAL_SURFACE('',#101309,0.1) ;
#16855=SPHERICAL_SURFACE('',#101315,0.1) ;
#16856=SPHERICAL_SURFACE('',#101317,0.1) ;
#16857=SPHERICAL_SURFACE('',#101324,0.1) ;
#16858=SPHERICAL_SURFACE('',#101337,0.1) ;
#16859=SPHERICAL_SURFACE('',#101342,0.1) ;
#16860=SPHERICAL_SURFACE('',#101365,0.1) ;
#16861=SPHERICAL_SURFACE('',#101376,0.1) ;
#16862=SPHERICAL_SURFACE('',#101378,0.1) ;
#16863=SPHERICAL_SURFACE('',#101393,0.1) ;
#16864=SPHERICAL_SURFACE('',#101407,0.1) ;
#16865=SPHERICAL_SURFACE('',#101414,0.1) ;
#16866=SPHERICAL_SURFACE('',#101426,0.1) ;
#16867=SPHERICAL_SURFACE('',#101428,0.1) ;
#16868=SPHERICAL_SURFACE('',#101434,0.1) ;
#16869=SPHERICAL_SURFACE('',#101444,0.1) ;
#16870=SPHERICAL_SURFACE('',#101450,0.1) ;
#16871=SPHERICAL_SURFACE('',#101461,0.1) ;
#16872=SPHERICAL_SURFACE('',#101467,0.1) ;
#16873=SPHERICAL_SURFACE('',#101495,0.1) ;
#16874=SPHERICAL_SURFACE('',#101497,0.1) ;
#16875=SPHERICAL_SURFACE('',#101507,0.1) ;
#16876=SPHERICAL_SURFACE('',#101509,0.1) ;
#16877=SPHERICAL_SURFACE('',#101537,0.1) ;
#16878=SPHERICAL_SURFACE('',#101539,0.1) ;
#16879=SPHERICAL_SURFACE('',#101551,0.1) ;
#16880=SPHERICAL_SURFACE('',#101553,0.1) ;
#16881=SPHERICAL_SURFACE('',#101563,0.1) ;
#16882=SPHERICAL_SURFACE('',#101565,0.1) ;
#16883=SPHERICAL_SURFACE('',#101575,0.1) ;
#16884=SPHERICAL_SURFACE('',#101577,0.1) ;
#16885=SPHERICAL_SURFACE('',#101583,0.1) ;
#16886=SPHERICAL_SURFACE('',#101585,0.1) ;
#16887=SPHERICAL_SURFACE('',#101591,0.1) ;
#16888=SPHERICAL_SURFACE('',#101593,0.1) ;
#16889=SPHERICAL_SURFACE('',#101600,0.1) ;
#16890=SPHERICAL_SURFACE('',#101613,0.1) ;
#16891=SPHERICAL_SURFACE('',#101618,0.1) ;
#16892=SPHERICAL_SURFACE('',#101641,0.1) ;
#16893=SPHERICAL_SURFACE('',#101652,0.1) ;
#16894=SPHERICAL_SURFACE('',#101654,0.1) ;
#16895=SPHERICAL_SURFACE('',#101669,0.1) ;
#16896=SPHERICAL_SURFACE('',#101683,0.1) ;
#16897=SPHERICAL_SURFACE('',#101690,0.1) ;
#16898=SPHERICAL_SURFACE('',#101702,0.1) ;
#16899=SPHERICAL_SURFACE('',#101704,0.1) ;
#16900=SPHERICAL_SURFACE('',#101710,0.1) ;
#16901=SPHERICAL_SURFACE('',#101720,0.1) ;
#16902=SPHERICAL_SURFACE('',#101726,0.1) ;
#16903=SPHERICAL_SURFACE('',#101737,0.1) ;
#16904=SPHERICAL_SURFACE('',#101743,0.1) ;
#16905=SPHERICAL_SURFACE('',#101771,0.1) ;
#16906=SPHERICAL_SURFACE('',#101773,0.1) ;
#16907=SPHERICAL_SURFACE('',#101783,0.1) ;
#16908=SPHERICAL_SURFACE('',#101785,0.1) ;
#16909=SPHERICAL_SURFACE('',#101813,0.1) ;
#16910=SPHERICAL_SURFACE('',#101815,0.1) ;
#16911=SPHERICAL_SURFACE('',#101827,0.1) ;
#16912=SPHERICAL_SURFACE('',#101829,0.1) ;
#16913=SPHERICAL_SURFACE('',#101839,0.1) ;
#16914=SPHERICAL_SURFACE('',#101841,0.1) ;
#16915=SPHERICAL_SURFACE('',#101851,0.1) ;
#16916=SPHERICAL_SURFACE('',#101853,0.1) ;
#16917=SPHERICAL_SURFACE('',#101859,0.1) ;
#16918=SPHERICAL_SURFACE('',#101861,0.1) ;
#16919=SPHERICAL_SURFACE('',#101867,0.1) ;
#16920=SPHERICAL_SURFACE('',#101869,0.1) ;
#16921=SPHERICAL_SURFACE('',#101876,0.1) ;
#16922=SPHERICAL_SURFACE('',#101889,0.1) ;
#16923=SPHERICAL_SURFACE('',#101894,0.1) ;
#16924=SPHERICAL_SURFACE('',#101917,0.1) ;
#16925=SPHERICAL_SURFACE('',#101928,0.1) ;
#16926=SPHERICAL_SURFACE('',#101930,0.1) ;
#16927=SPHERICAL_SURFACE('',#101945,0.1) ;
#16928=SPHERICAL_SURFACE('',#101959,0.1) ;
#16929=SPHERICAL_SURFACE('',#101966,0.1) ;
#16930=SPHERICAL_SURFACE('',#101978,0.1) ;
#16931=SPHERICAL_SURFACE('',#101980,0.1) ;
#16932=SPHERICAL_SURFACE('',#101986,0.1) ;
#16933=SPHERICAL_SURFACE('',#101996,0.1) ;
#16934=SPHERICAL_SURFACE('',#102002,0.1) ;
#16935=SPHERICAL_SURFACE('',#102013,0.1) ;
#16936=SPHERICAL_SURFACE('',#102019,0.1) ;
#16937=SPHERICAL_SURFACE('',#102047,0.1) ;
#16938=SPHERICAL_SURFACE('',#102049,0.1) ;
#16939=SPHERICAL_SURFACE('',#102059,0.1) ;
#16940=SPHERICAL_SURFACE('',#102061,0.1) ;
#16941=SPHERICAL_SURFACE('',#102089,0.1) ;
#16942=SPHERICAL_SURFACE('',#102091,0.1) ;
#16943=SPHERICAL_SURFACE('',#102103,0.1) ;
#16944=SPHERICAL_SURFACE('',#102105,0.1) ;
#16945=SPHERICAL_SURFACE('',#102115,0.1) ;
#16946=SPHERICAL_SURFACE('',#102117,0.1) ;
#16947=SPHERICAL_SURFACE('',#102127,0.1) ;
#16948=SPHERICAL_SURFACE('',#102129,0.1) ;
#16949=SPHERICAL_SURFACE('',#102135,0.1) ;
#16950=SPHERICAL_SURFACE('',#102137,0.1) ;
#16951=SPHERICAL_SURFACE('',#102143,0.1) ;
#16952=SPHERICAL_SURFACE('',#102145,0.1) ;
#16953=SPHERICAL_SURFACE('',#102152,0.1) ;
#16954=SPHERICAL_SURFACE('',#102165,0.1) ;
#16955=SPHERICAL_SURFACE('',#102170,0.1) ;
#16956=SPHERICAL_SURFACE('',#102193,0.1) ;
#16957=SPHERICAL_SURFACE('',#102204,0.1) ;
#16958=SPHERICAL_SURFACE('',#102206,0.1) ;
#16959=SPHERICAL_SURFACE('',#102221,0.1) ;
#16960=SPHERICAL_SURFACE('',#102235,0.1) ;
#16961=SPHERICAL_SURFACE('',#102242,0.1) ;
#16962=SPHERICAL_SURFACE('',#102254,0.1) ;
#16963=SPHERICAL_SURFACE('',#102256,0.1) ;
#16964=SPHERICAL_SURFACE('',#102262,0.1) ;
#16965=SPHERICAL_SURFACE('',#102272,0.1) ;
#16966=SPHERICAL_SURFACE('',#102278,0.1) ;
#16967=SPHERICAL_SURFACE('',#102289,0.1) ;
#16968=SPHERICAL_SURFACE('',#102295,0.1) ;
#16969=SPHERICAL_SURFACE('',#102323,0.1) ;
#16970=SPHERICAL_SURFACE('',#102325,0.1) ;
#16971=SPHERICAL_SURFACE('',#102335,0.1) ;
#16972=SPHERICAL_SURFACE('',#102337,0.1) ;
#16973=SPHERICAL_SURFACE('',#102365,0.1) ;
#16974=SPHERICAL_SURFACE('',#102367,0.1) ;
#16975=SPHERICAL_SURFACE('',#102379,0.1) ;
#16976=SPHERICAL_SURFACE('',#102381,0.1) ;
#16977=SPHERICAL_SURFACE('',#102391,0.1) ;
#16978=SPHERICAL_SURFACE('',#102393,0.1) ;
#16979=SPHERICAL_SURFACE('',#102403,0.1) ;
#16980=SPHERICAL_SURFACE('',#102405,0.1) ;
#16981=SPHERICAL_SURFACE('',#102411,0.1) ;
#16982=SPHERICAL_SURFACE('',#102413,0.1) ;
#16983=SPHERICAL_SURFACE('',#102419,0.1) ;
#16984=SPHERICAL_SURFACE('',#102421,0.1) ;
#16985=SPHERICAL_SURFACE('',#102428,0.1) ;
#16986=SPHERICAL_SURFACE('',#102441,0.1) ;
#16987=SPHERICAL_SURFACE('',#102446,0.1) ;
#16988=SPHERICAL_SURFACE('',#102469,0.1) ;
#16989=SPHERICAL_SURFACE('',#102480,0.1) ;
#16990=SPHERICAL_SURFACE('',#102482,0.1) ;
#16991=SPHERICAL_SURFACE('',#102497,0.1) ;
#16992=SPHERICAL_SURFACE('',#102511,0.1) ;
#16993=SPHERICAL_SURFACE('',#102518,0.1) ;
#16994=SPHERICAL_SURFACE('',#102530,0.1) ;
#16995=SPHERICAL_SURFACE('',#102532,0.1) ;
#16996=SPHERICAL_SURFACE('',#102538,0.1) ;
#16997=SPHERICAL_SURFACE('',#102548,0.1) ;
#16998=SPHERICAL_SURFACE('',#102554,0.1) ;
#16999=SPHERICAL_SURFACE('',#102565,0.1) ;
#17000=SPHERICAL_SURFACE('',#102571,0.1) ;
#17001=SPHERICAL_SURFACE('',#102599,0.1) ;
#17002=SPHERICAL_SURFACE('',#102601,0.1) ;
#17003=SPHERICAL_SURFACE('',#102611,0.1) ;
#17004=SPHERICAL_SURFACE('',#102613,0.1) ;
#17005=SPHERICAL_SURFACE('',#102641,0.1) ;
#17006=SPHERICAL_SURFACE('',#102643,0.1) ;
#17007=SPHERICAL_SURFACE('',#102655,0.1) ;
#17008=SPHERICAL_SURFACE('',#102657,0.1) ;
#17009=SPHERICAL_SURFACE('',#102667,0.1) ;
#17010=SPHERICAL_SURFACE('',#102669,0.1) ;
#17011=SPHERICAL_SURFACE('',#102679,0.1) ;
#17012=SPHERICAL_SURFACE('',#102681,0.1) ;
#17013=SPHERICAL_SURFACE('',#102687,0.1) ;
#17014=SPHERICAL_SURFACE('',#102689,0.1) ;
#17015=SPHERICAL_SURFACE('',#102695,0.1) ;
#17016=SPHERICAL_SURFACE('',#102697,0.1) ;
#17017=SPHERICAL_SURFACE('',#102798,0.1) ;
#17018=SPHERICAL_SURFACE('',#102804,0.1) ;
#17019=SPHERICAL_SURFACE('',#102810,0.1) ;
#17020=SPHERICAL_SURFACE('',#102816,0.1) ;
#17021=SPHERICAL_SURFACE('',#102822,0.1) ;
#17022=SPHERICAL_SURFACE('',#102828,0.1) ;
#17023=SPHERICAL_SURFACE('',#102834,0.1) ;
#17024=SPHERICAL_SURFACE('',#102840,0.1) ;
#17025=SPHERICAL_SURFACE('',#102846,0.1) ;
#17026=SPHERICAL_SURFACE('',#102852,0.1) ;
#17027=SPHERICAL_SURFACE('',#102858,0.1) ;
#17028=SPHERICAL_SURFACE('',#102864,0.1) ;
#17029=SPHERICAL_SURFACE('',#102870,0.1) ;
#17030=SPHERICAL_SURFACE('',#102876,0.1) ;
#17031=SPHERICAL_SURFACE('',#102882,0.1) ;
#17032=SPHERICAL_SURFACE('',#102888,0.1) ;
#17033=SPHERICAL_SURFACE('',#102894,0.1) ;
#17034=SPHERICAL_SURFACE('',#102900,0.1) ;
#17035=SPHERICAL_SURFACE('',#102985,0.1) ;
#17036=SPHERICAL_SURFACE('',#102993,0.1) ;
#17037=SPHERICAL_SURFACE('',#102997,0.1) ;
#17038=SPHERICAL_SURFACE('',#103001,0.1) ;
#17039=SPHERICAL_SURFACE('',#103012,0.1) ;
#17040=SPHERICAL_SURFACE('',#103022,0.1) ;
#17041=SPHERICAL_SURFACE('',#103032,0.1) ;
#17042=SPHERICAL_SURFACE('',#103042,0.1) ;
#17043=SPHERICAL_SURFACE('',#103052,0.1) ;
#17044=SPHERICAL_SURFACE('',#103062,0.1) ;
#17045=SPHERICAL_SURFACE('',#103070,0.1) ;
#17046=SPHERICAL_SURFACE('',#103074,0.1) ;
#20398=FACE_OUTER_BOUND('',#26181,.T.) ;
#20399=FACE_OUTER_BOUND('',#26182,.T.) ;
#20400=FACE_OUTER_BOUND('',#26183,.T.) ;
#20401=FACE_OUTER_BOUND('',#26184,.T.) ;
#20402=FACE_OUTER_BOUND('',#26185,.T.) ;
#20403=FACE_OUTER_BOUND('',#26186,.T.) ;
#20404=FACE_OUTER_BOUND('',#26187,.T.) ;
#20405=FACE_OUTER_BOUND('',#26188,.T.) ;
#20406=FACE_OUTER_BOUND('',#26189,.T.) ;
#20407=FACE_OUTER_BOUND('',#26190,.T.) ;
#20408=FACE_OUTER_BOUND('',#26191,.T.) ;
#20409=FACE_OUTER_BOUND('',#26192,.T.) ;
#20410=FACE_OUTER_BOUND('',#26193,.T.) ;
#20411=FACE_OUTER_BOUND('',#26194,.T.) ;
#20412=FACE_OUTER_BOUND('',#26195,.T.) ;
#20413=FACE_OUTER_BOUND('',#26196,.T.) ;
#20414=FACE_OUTER_BOUND('',#26197,.T.) ;
#20415=FACE_OUTER_BOUND('',#26198,.T.) ;
#20416=FACE_OUTER_BOUND('',#26199,.T.) ;
#20417=FACE_OUTER_BOUND('',#26200,.T.) ;
#20418=FACE_OUTER_BOUND('',#26201,.T.) ;
#20419=FACE_OUTER_BOUND('',#26202,.T.) ;
#20420=FACE_OUTER_BOUND('',#26203,.T.) ;
#20421=FACE_OUTER_BOUND('',#26204,.T.) ;
#20422=FACE_OUTER_BOUND('',#26205,.T.) ;
#20423=FACE_OUTER_BOUND('',#26206,.T.) ;
#20424=FACE_OUTER_BOUND('',#26207,.T.) ;
#20425=FACE_OUTER_BOUND('',#26208,.T.) ;
#20426=FACE_OUTER_BOUND('',#26209,.T.) ;
#20427=FACE_OUTER_BOUND('',#26210,.T.) ;
#20428=FACE_OUTER_BOUND('',#26211,.T.) ;
#20429=FACE_OUTER_BOUND('',#26212,.T.) ;
#20430=FACE_OUTER_BOUND('',#26213,.T.) ;
#20431=FACE_OUTER_BOUND('',#26214,.T.) ;
#20432=FACE_OUTER_BOUND('',#26215,.T.) ;
#20433=FACE_OUTER_BOUND('',#26216,.T.) ;
#20434=FACE_OUTER_BOUND('',#26217,.T.) ;
#20435=FACE_OUTER_BOUND('',#26218,.T.) ;
#20436=FACE_OUTER_BOUND('',#26219,.T.) ;
#20437=FACE_OUTER_BOUND('',#26220,.T.) ;
#20438=FACE_OUTER_BOUND('',#26221,.T.) ;
#20439=FACE_OUTER_BOUND('',#26222,.T.) ;
#20440=FACE_OUTER_BOUND('',#26223,.T.) ;
#20441=FACE_OUTER_BOUND('',#26224,.T.) ;
#20442=FACE_OUTER_BOUND('',#26225,.T.) ;
#20443=FACE_OUTER_BOUND('',#26226,.T.) ;
#20444=FACE_OUTER_BOUND('',#26227,.T.) ;
#20445=FACE_OUTER_BOUND('',#26228,.T.) ;
#20446=FACE_OUTER_BOUND('',#26229,.T.) ;
#20447=FACE_OUTER_BOUND('',#26230,.T.) ;
#20448=FACE_OUTER_BOUND('',#26231,.T.) ;
#20449=FACE_OUTER_BOUND('',#26232,.T.) ;
#20450=FACE_OUTER_BOUND('',#26233,.T.) ;
#20451=FACE_OUTER_BOUND('',#26234,.T.) ;
#20452=FACE_OUTER_BOUND('',#26235,.T.) ;
#20453=FACE_OUTER_BOUND('',#26236,.T.) ;
#20454=FACE_OUTER_BOUND('',#26237,.T.) ;
#20455=FACE_OUTER_BOUND('',#26238,.T.) ;
#20456=FACE_OUTER_BOUND('',#26239,.T.) ;
#20457=FACE_OUTER_BOUND('',#26240,.T.) ;
#20458=FACE_OUTER_BOUND('',#26241,.T.) ;
#20459=FACE_OUTER_BOUND('',#26242,.T.) ;
#20460=FACE_OUTER_BOUND('',#26243,.T.) ;
#20461=FACE_OUTER_BOUND('',#26244,.T.) ;
#20462=FACE_OUTER_BOUND('',#26245,.T.) ;
#20463=FACE_OUTER_BOUND('',#26246,.T.) ;
#20464=FACE_OUTER_BOUND('',#26247,.T.) ;
#20465=FACE_OUTER_BOUND('',#26248,.T.) ;
#20466=FACE_OUTER_BOUND('',#26249,.T.) ;
#20467=FACE_OUTER_BOUND('',#26250,.T.) ;
#20468=FACE_OUTER_BOUND('',#26251,.T.) ;
#20469=FACE_OUTER_BOUND('',#26252,.T.) ;
#20470=FACE_OUTER_BOUND('',#26253,.T.) ;
#20471=FACE_OUTER_BOUND('',#26254,.T.) ;
#20472=FACE_OUTER_BOUND('',#26255,.T.) ;
#20473=FACE_OUTER_BOUND('',#26256,.T.) ;
#20474=FACE_OUTER_BOUND('',#26257,.T.) ;
#20475=FACE_OUTER_BOUND('',#26258,.T.) ;
#20476=FACE_OUTER_BOUND('',#26259,.T.) ;
#20477=FACE_OUTER_BOUND('',#26260,.T.) ;
#20478=FACE_OUTER_BOUND('',#26261,.T.) ;
#20479=FACE_OUTER_BOUND('',#26262,.T.) ;
#20480=FACE_OUTER_BOUND('',#26263,.T.) ;
#20481=FACE_OUTER_BOUND('',#26264,.T.) ;
#20482=FACE_OUTER_BOUND('',#26265,.T.) ;
#20483=FACE_OUTER_BOUND('',#26266,.T.) ;
#20484=FACE_OUTER_BOUND('',#26267,.T.) ;
#20485=FACE_OUTER_BOUND('',#26268,.T.) ;
#20486=FACE_OUTER_BOUND('',#26269,.T.) ;
#20487=FACE_OUTER_BOUND('',#26270,.T.) ;
#20488=FACE_OUTER_BOUND('',#26271,.T.) ;
#20489=FACE_OUTER_BOUND('',#26272,.T.) ;
#20490=FACE_OUTER_BOUND('',#26273,.T.) ;
#20491=FACE_OUTER_BOUND('',#26274,.T.) ;
#20492=FACE_OUTER_BOUND('',#26295,.T.) ;
#20493=FACE_OUTER_BOUND('',#26297,.T.) ;
#20494=FACE_OUTER_BOUND('',#26299,.T.) ;
#20495=FACE_OUTER_BOUND('',#26301,.T.) ;
#20496=FACE_OUTER_BOUND('',#26303,.T.) ;
#20497=FACE_OUTER_BOUND('',#26305,.T.) ;
#20498=FACE_OUTER_BOUND('',#26307,.T.) ;
#20499=FACE_OUTER_BOUND('',#26309,.T.) ;
#20500=FACE_OUTER_BOUND('',#26311,.T.) ;
#20501=FACE_OUTER_BOUND('',#26313,.T.) ;
#20502=FACE_OUTER_BOUND('',#26314,.T.) ;
#20503=FACE_OUTER_BOUND('',#26315,.T.) ;
#20504=FACE_OUTER_BOUND('',#26316,.T.) ;
#20505=FACE_OUTER_BOUND('',#26317,.T.) ;
#20506=FACE_OUTER_BOUND('',#26318,.T.) ;
#20507=FACE_OUTER_BOUND('',#26319,.T.) ;
#20508=FACE_OUTER_BOUND('',#26320,.T.) ;
#20509=FACE_OUTER_BOUND('',#26321,.T.) ;
#20510=FACE_OUTER_BOUND('',#26322,.T.) ;
#20511=FACE_OUTER_BOUND('',#26323,.T.) ;
#20512=FACE_OUTER_BOUND('',#26324,.T.) ;
#20513=FACE_OUTER_BOUND('',#26325,.T.) ;
#20514=FACE_OUTER_BOUND('',#26326,.T.) ;
#20515=FACE_OUTER_BOUND('',#26327,.T.) ;
#20516=FACE_OUTER_BOUND('',#26328,.T.) ;
#20517=FACE_OUTER_BOUND('',#26329,.T.) ;
#20518=FACE_OUTER_BOUND('',#26330,.T.) ;
#20519=FACE_OUTER_BOUND('',#26331,.T.) ;
#20520=FACE_OUTER_BOUND('',#26332,.T.) ;
#20521=FACE_OUTER_BOUND('',#26333,.T.) ;
#20522=FACE_OUTER_BOUND('',#26334,.T.) ;
#20523=FACE_OUTER_BOUND('',#26335,.T.) ;
#20524=FACE_OUTER_BOUND('',#26336,.T.) ;
#20525=FACE_OUTER_BOUND('',#26347,.T.) ;
#20526=FACE_OUTER_BOUND('',#26349,.T.) ;
#20527=FACE_OUTER_BOUND('',#26350,.T.) ;
#20528=FACE_OUTER_BOUND('',#26351,.T.) ;
#20529=FACE_OUTER_BOUND('',#26352,.T.) ;
#20530=FACE_OUTER_BOUND('',#26353,.T.) ;
#20531=FACE_OUTER_BOUND('',#26354,.T.) ;
#20532=FACE_OUTER_BOUND('',#26355,.T.) ;
#20533=FACE_OUTER_BOUND('',#26366,.T.) ;
#20534=FACE_OUTER_BOUND('',#26367,.T.) ;
#20535=FACE_OUTER_BOUND('',#26368,.T.) ;
#20536=FACE_OUTER_BOUND('',#26369,.T.) ;
#20537=FACE_OUTER_BOUND('',#26370,.T.) ;
#20538=FACE_OUTER_BOUND('',#26371,.T.) ;
#20539=FACE_OUTER_BOUND('',#26372,.T.) ;
#20540=FACE_OUTER_BOUND('',#26373,.T.) ;
#20541=FACE_OUTER_BOUND('',#26374,.T.) ;
#20542=FACE_OUTER_BOUND('',#26375,.T.) ;
#20543=FACE_OUTER_BOUND('',#26376,.T.) ;
#20544=FACE_OUTER_BOUND('',#26377,.T.) ;
#20545=FACE_OUTER_BOUND('',#26378,.T.) ;
#20546=FACE_OUTER_BOUND('',#26379,.T.) ;
#20547=FACE_OUTER_BOUND('',#26381,.T.) ;
#20548=FACE_OUTER_BOUND('',#26382,.T.) ;
#20549=FACE_OUTER_BOUND('',#26383,.T.) ;
#20550=FACE_OUTER_BOUND('',#26384,.T.) ;
#20551=FACE_OUTER_BOUND('',#26385,.T.) ;
#20552=FACE_OUTER_BOUND('',#26386,.T.) ;
#20553=FACE_OUTER_BOUND('',#26387,.T.) ;
#20554=FACE_OUTER_BOUND('',#26388,.T.) ;
#20555=FACE_OUTER_BOUND('',#26389,.T.) ;
#20556=FACE_OUTER_BOUND('',#26390,.T.) ;
#20557=FACE_OUTER_BOUND('',#26391,.T.) ;
#20558=FACE_OUTER_BOUND('',#26392,.T.) ;
#20559=FACE_OUTER_BOUND('',#26393,.T.) ;
#20560=FACE_OUTER_BOUND('',#26394,.T.) ;
#20561=FACE_OUTER_BOUND('',#26395,.T.) ;
#20562=FACE_OUTER_BOUND('',#26397,.T.) ;
#20563=FACE_OUTER_BOUND('',#26398,.T.) ;
#20564=FACE_OUTER_BOUND('',#26399,.T.) ;
#20565=FACE_OUTER_BOUND('',#26400,.T.) ;
#20566=FACE_OUTER_BOUND('',#26401,.T.) ;
#20567=FACE_OUTER_BOUND('',#26402,.T.) ;
#20568=FACE_OUTER_BOUND('',#26404,.T.) ;
#20569=FACE_OUTER_BOUND('',#26405,.T.) ;
#20570=FACE_OUTER_BOUND('',#26406,.T.) ;
#20571=FACE_OUTER_BOUND('',#26407,.T.) ;
#20572=FACE_OUTER_BOUND('',#26408,.T.) ;
#20573=FACE_OUTER_BOUND('',#26409,.T.) ;
#20574=FACE_OUTER_BOUND('',#26410,.T.) ;
#20575=FACE_OUTER_BOUND('',#26411,.T.) ;
#20576=FACE_OUTER_BOUND('',#26412,.T.) ;
#20577=FACE_OUTER_BOUND('',#26413,.T.) ;
#20578=FACE_OUTER_BOUND('',#26414,.T.) ;
#20579=FACE_OUTER_BOUND('',#26415,.T.) ;
#20580=FACE_OUTER_BOUND('',#26416,.T.) ;
#20581=FACE_OUTER_BOUND('',#26417,.T.) ;
#20582=FACE_OUTER_BOUND('',#26418,.T.) ;
#20583=FACE_OUTER_BOUND('',#26419,.T.) ;
#20584=FACE_OUTER_BOUND('',#26420,.T.) ;
#20585=FACE_OUTER_BOUND('',#26421,.T.) ;
#20586=FACE_OUTER_BOUND('',#26422,.T.) ;
#20587=FACE_OUTER_BOUND('',#26423,.T.) ;
#20588=FACE_OUTER_BOUND('',#26424,.T.) ;
#20589=FACE_OUTER_BOUND('',#26425,.T.) ;
#20590=FACE_OUTER_BOUND('',#26426,.T.) ;
#20591=FACE_OUTER_BOUND('',#26427,.T.) ;
#20592=FACE_OUTER_BOUND('',#26428,.T.) ;
#20593=FACE_OUTER_BOUND('',#26429,.T.) ;
#20594=FACE_OUTER_BOUND('',#26430,.T.) ;
#20595=FACE_OUTER_BOUND('',#26431,.T.) ;
#20596=FACE_OUTER_BOUND('',#26432,.T.) ;
#20597=FACE_OUTER_BOUND('',#26433,.T.) ;
#20598=FACE_OUTER_BOUND('',#26434,.T.) ;
#20599=FACE_OUTER_BOUND('',#26435,.T.) ;
#20600=FACE_OUTER_BOUND('',#26436,.T.) ;
#20601=FACE_OUTER_BOUND('',#26437,.T.) ;
#20602=FACE_OUTER_BOUND('',#26438,.T.) ;
#20603=FACE_OUTER_BOUND('',#26439,.T.) ;
#20604=FACE_OUTER_BOUND('',#26440,.T.) ;
#20605=FACE_OUTER_BOUND('',#26441,.T.) ;
#20606=FACE_OUTER_BOUND('',#26442,.T.) ;
#20607=FACE_OUTER_BOUND('',#26443,.T.) ;
#20608=FACE_OUTER_BOUND('',#26444,.T.) ;
#20609=FACE_OUTER_BOUND('',#26445,.T.) ;
#20610=FACE_OUTER_BOUND('',#26446,.T.) ;
#20611=FACE_OUTER_BOUND('',#26447,.T.) ;
#20612=FACE_OUTER_BOUND('',#26448,.T.) ;
#20613=FACE_OUTER_BOUND('',#26449,.T.) ;
#20614=FACE_OUTER_BOUND('',#26450,.T.) ;
#20615=FACE_OUTER_BOUND('',#26451,.T.) ;
#20616=FACE_OUTER_BOUND('',#26452,.T.) ;
#20617=FACE_OUTER_BOUND('',#26453,.T.) ;
#20618=FACE_OUTER_BOUND('',#26454,.T.) ;
#20619=FACE_OUTER_BOUND('',#26455,.T.) ;
#20620=FACE_OUTER_BOUND('',#26456,.T.) ;
#20621=FACE_OUTER_BOUND('',#26457,.T.) ;
#20622=FACE_OUTER_BOUND('',#26458,.T.) ;
#20623=FACE_OUTER_BOUND('',#26459,.T.) ;
#20624=FACE_OUTER_BOUND('',#26460,.T.) ;
#20625=FACE_OUTER_BOUND('',#26461,.T.) ;
#20626=FACE_OUTER_BOUND('',#26462,.T.) ;
#20627=FACE_OUTER_BOUND('',#26463,.T.) ;
#20628=FACE_OUTER_BOUND('',#26464,.T.) ;
#20629=FACE_OUTER_BOUND('',#26465,.T.) ;
#20630=FACE_OUTER_BOUND('',#26466,.T.) ;
#20631=FACE_OUTER_BOUND('',#26467,.T.) ;
#20632=FACE_OUTER_BOUND('',#26468,.T.) ;
#20633=FACE_OUTER_BOUND('',#26469,.T.) ;
#20634=FACE_OUTER_BOUND('',#26470,.T.) ;
#20635=FACE_OUTER_BOUND('',#26471,.T.) ;
#20636=FACE_OUTER_BOUND('',#26472,.T.) ;
#20637=FACE_OUTER_BOUND('',#26473,.T.) ;
#20638=FACE_OUTER_BOUND('',#26474,.T.) ;
#20639=FACE_OUTER_BOUND('',#26475,.T.) ;
#20640=FACE_OUTER_BOUND('',#26476,.T.) ;
#20641=FACE_OUTER_BOUND('',#26477,.T.) ;
#20642=FACE_OUTER_BOUND('',#26478,.T.) ;
#20643=FACE_OUTER_BOUND('',#26479,.T.) ;
#20644=FACE_OUTER_BOUND('',#26480,.T.) ;
#20645=FACE_OUTER_BOUND('',#26481,.T.) ;
#20646=FACE_OUTER_BOUND('',#26482,.T.) ;
#20647=FACE_OUTER_BOUND('',#26483,.T.) ;
#20648=FACE_OUTER_BOUND('',#26484,.T.) ;
#20649=FACE_OUTER_BOUND('',#26485,.T.) ;
#20650=FACE_OUTER_BOUND('',#26486,.T.) ;
#20651=FACE_OUTER_BOUND('',#26487,.T.) ;
#20652=FACE_OUTER_BOUND('',#26488,.T.) ;
#20653=FACE_OUTER_BOUND('',#26489,.T.) ;
#20654=FACE_OUTER_BOUND('',#26490,.T.) ;
#20655=FACE_OUTER_BOUND('',#26491,.T.) ;
#20656=FACE_OUTER_BOUND('',#26492,.T.) ;
#20657=FACE_OUTER_BOUND('',#26493,.T.) ;
#20658=FACE_OUTER_BOUND('',#26494,.T.) ;
#20659=FACE_OUTER_BOUND('',#26495,.T.) ;
#20660=FACE_OUTER_BOUND('',#26496,.T.) ;
#20661=FACE_OUTER_BOUND('',#26497,.T.) ;
#20662=FACE_OUTER_BOUND('',#26498,.T.) ;
#20663=FACE_OUTER_BOUND('',#26499,.T.) ;
#20664=FACE_OUTER_BOUND('',#26500,.T.) ;
#20665=FACE_OUTER_BOUND('',#26501,.T.) ;
#20666=FACE_OUTER_BOUND('',#26502,.T.) ;
#20667=FACE_OUTER_BOUND('',#26503,.T.) ;
#20668=FACE_OUTER_BOUND('',#26504,.T.) ;
#20669=FACE_OUTER_BOUND('',#26505,.T.) ;
#20670=FACE_OUTER_BOUND('',#26506,.T.) ;
#20671=FACE_OUTER_BOUND('',#26507,.T.) ;
#20672=FACE_OUTER_BOUND('',#26508,.T.) ;
#20673=FACE_OUTER_BOUND('',#26509,.T.) ;
#20674=FACE_OUTER_BOUND('',#26510,.T.) ;
#20675=FACE_OUTER_BOUND('',#26511,.T.) ;
#20676=FACE_OUTER_BOUND('',#26512,.T.) ;
#20677=FACE_OUTER_BOUND('',#26513,.T.) ;
#20678=FACE_OUTER_BOUND('',#26514,.T.) ;
#20679=FACE_OUTER_BOUND('',#26515,.T.) ;
#20680=FACE_OUTER_BOUND('',#26516,.T.) ;
#20681=FACE_OUTER_BOUND('',#26517,.T.) ;
#20682=FACE_OUTER_BOUND('',#26518,.T.) ;
#20683=FACE_OUTER_BOUND('',#26519,.T.) ;
#20684=FACE_OUTER_BOUND('',#26520,.T.) ;
#20685=FACE_OUTER_BOUND('',#26521,.T.) ;
#20686=FACE_OUTER_BOUND('',#26522,.T.) ;
#20687=FACE_OUTER_BOUND('',#26523,.T.) ;
#20688=FACE_OUTER_BOUND('',#26524,.T.) ;
#20689=FACE_OUTER_BOUND('',#26525,.T.) ;
#20690=FACE_OUTER_BOUND('',#26526,.T.) ;
#20691=FACE_OUTER_BOUND('',#26527,.T.) ;
#20692=FACE_OUTER_BOUND('',#26528,.T.) ;
#20693=FACE_OUTER_BOUND('',#26529,.T.) ;
#20694=FACE_OUTER_BOUND('',#26530,.T.) ;
#20695=FACE_OUTER_BOUND('',#26531,.T.) ;
#20696=FACE_OUTER_BOUND('',#26532,.T.) ;
#20697=FACE_OUTER_BOUND('',#26533,.T.) ;
#20698=FACE_OUTER_BOUND('',#26534,.T.) ;
#20699=FACE_OUTER_BOUND('',#26535,.T.) ;
#20700=FACE_OUTER_BOUND('',#26536,.T.) ;
#20701=FACE_OUTER_BOUND('',#26537,.T.) ;
#20702=FACE_OUTER_BOUND('',#26538,.T.) ;
#20703=FACE_OUTER_BOUND('',#26539,.T.) ;
#20704=FACE_OUTER_BOUND('',#26540,.T.) ;
#20705=FACE_OUTER_BOUND('',#26541,.T.) ;
#20706=FACE_OUTER_BOUND('',#26542,.T.) ;
#20707=FACE_OUTER_BOUND('',#26543,.T.) ;
#20708=FACE_OUTER_BOUND('',#26544,.T.) ;
#20709=FACE_OUTER_BOUND('',#26545,.T.) ;
#20710=FACE_OUTER_BOUND('',#26546,.T.) ;
#20711=FACE_OUTER_BOUND('',#26547,.T.) ;
#20712=FACE_OUTER_BOUND('',#26548,.T.) ;
#20713=FACE_OUTER_BOUND('',#26549,.T.) ;
#20714=FACE_OUTER_BOUND('',#26550,.T.) ;
#20715=FACE_OUTER_BOUND('',#26551,.T.) ;
#20716=FACE_OUTER_BOUND('',#26552,.T.) ;
#20717=FACE_OUTER_BOUND('',#26553,.T.) ;
#20718=FACE_OUTER_BOUND('',#26554,.T.) ;
#20719=FACE_OUTER_BOUND('',#26555,.T.) ;
#20720=FACE_OUTER_BOUND('',#26556,.T.) ;
#20721=FACE_OUTER_BOUND('',#26557,.T.) ;
#20722=FACE_OUTER_BOUND('',#26558,.T.) ;
#20723=FACE_OUTER_BOUND('',#26559,.T.) ;
#20724=FACE_OUTER_BOUND('',#26560,.T.) ;
#20725=FACE_OUTER_BOUND('',#26561,.T.) ;
#20726=FACE_OUTER_BOUND('',#26562,.T.) ;
#20727=FACE_OUTER_BOUND('',#26563,.T.) ;
#20728=FACE_OUTER_BOUND('',#26564,.T.) ;
#20729=FACE_OUTER_BOUND('',#26565,.T.) ;
#20730=FACE_OUTER_BOUND('',#26566,.T.) ;
#20731=FACE_OUTER_BOUND('',#26567,.T.) ;
#20732=FACE_OUTER_BOUND('',#26568,.T.) ;
#20733=FACE_OUTER_BOUND('',#26569,.T.) ;
#20734=FACE_OUTER_BOUND('',#26570,.T.) ;
#20735=FACE_OUTER_BOUND('',#26571,.T.) ;
#20736=FACE_OUTER_BOUND('',#26572,.T.) ;
#20737=FACE_OUTER_BOUND('',#26573,.T.) ;
#20738=FACE_OUTER_BOUND('',#26574,.T.) ;
#20739=FACE_OUTER_BOUND('',#26575,.T.) ;
#20740=FACE_OUTER_BOUND('',#26576,.T.) ;
#20741=FACE_OUTER_BOUND('',#26577,.T.) ;
#20742=FACE_OUTER_BOUND('',#26578,.T.) ;
#20743=FACE_OUTER_BOUND('',#26579,.T.) ;
#20744=FACE_OUTER_BOUND('',#26580,.T.) ;
#20745=FACE_OUTER_BOUND('',#26581,.T.) ;
#20746=FACE_OUTER_BOUND('',#26582,.T.) ;
#20747=FACE_OUTER_BOUND('',#26583,.T.) ;
#20748=FACE_OUTER_BOUND('',#26584,.T.) ;
#20749=FACE_OUTER_BOUND('',#26585,.T.) ;
#20750=FACE_OUTER_BOUND('',#26586,.T.) ;
#20751=FACE_OUTER_BOUND('',#26587,.T.) ;
#20752=FACE_OUTER_BOUND('',#26588,.T.) ;
#20753=FACE_OUTER_BOUND('',#26589,.T.) ;
#20754=FACE_OUTER_BOUND('',#26590,.T.) ;
#20755=FACE_OUTER_BOUND('',#26591,.T.) ;
#20756=FACE_OUTER_BOUND('',#26592,.T.) ;
#20757=FACE_OUTER_BOUND('',#26593,.T.) ;
#20758=FACE_OUTER_BOUND('',#26594,.T.) ;
#20759=FACE_OUTER_BOUND('',#26595,.T.) ;
#20760=FACE_OUTER_BOUND('',#26596,.T.) ;
#20761=FACE_OUTER_BOUND('',#26597,.T.) ;
#20762=FACE_OUTER_BOUND('',#26598,.T.) ;
#20763=FACE_OUTER_BOUND('',#26599,.T.) ;
#20764=FACE_OUTER_BOUND('',#26600,.T.) ;
#20765=FACE_OUTER_BOUND('',#26601,.T.) ;
#20766=FACE_OUTER_BOUND('',#26602,.T.) ;
#20767=FACE_OUTER_BOUND('',#26603,.T.) ;
#20768=FACE_OUTER_BOUND('',#26604,.T.) ;
#20769=FACE_OUTER_BOUND('',#26605,.T.) ;
#20770=FACE_OUTER_BOUND('',#26606,.T.) ;
#20771=FACE_OUTER_BOUND('',#26607,.T.) ;
#20772=FACE_OUTER_BOUND('',#26608,.T.) ;
#20773=FACE_OUTER_BOUND('',#26609,.T.) ;
#20774=FACE_OUTER_BOUND('',#26610,.T.) ;
#20775=FACE_OUTER_BOUND('',#26611,.T.) ;
#20776=FACE_OUTER_BOUND('',#26612,.T.) ;
#20777=FACE_OUTER_BOUND('',#26613,.T.) ;
#20778=FACE_OUTER_BOUND('',#26614,.T.) ;
#20779=FACE_OUTER_BOUND('',#26615,.T.) ;
#20780=FACE_OUTER_BOUND('',#26616,.T.) ;
#20781=FACE_OUTER_BOUND('',#26617,.T.) ;
#20782=FACE_OUTER_BOUND('',#26618,.T.) ;
#20783=FACE_OUTER_BOUND('',#26619,.T.) ;
#20784=FACE_OUTER_BOUND('',#26620,.T.) ;
#20785=FACE_OUTER_BOUND('',#26621,.T.) ;
#20786=FACE_OUTER_BOUND('',#26622,.T.) ;
#20787=FACE_OUTER_BOUND('',#26623,.T.) ;
#20788=FACE_OUTER_BOUND('',#26624,.T.) ;
#20789=FACE_OUTER_BOUND('',#26625,.T.) ;
#20790=FACE_OUTER_BOUND('',#26626,.T.) ;
#20791=FACE_OUTER_BOUND('',#26627,.T.) ;
#20792=FACE_OUTER_BOUND('',#26628,.T.) ;
#20793=FACE_OUTER_BOUND('',#26629,.T.) ;
#20794=FACE_OUTER_BOUND('',#26630,.T.) ;
#20795=FACE_OUTER_BOUND('',#26631,.T.) ;
#20796=FACE_OUTER_BOUND('',#26632,.T.) ;
#20797=FACE_OUTER_BOUND('',#26633,.T.) ;
#20798=FACE_OUTER_BOUND('',#26634,.T.) ;
#20799=FACE_OUTER_BOUND('',#26635,.T.) ;
#20800=FACE_OUTER_BOUND('',#26636,.T.) ;
#20801=FACE_OUTER_BOUND('',#26637,.T.) ;
#20802=FACE_OUTER_BOUND('',#26638,.T.) ;
#20803=FACE_OUTER_BOUND('',#26639,.T.) ;
#20804=FACE_OUTER_BOUND('',#26640,.T.) ;
#20805=FACE_OUTER_BOUND('',#26641,.T.) ;
#20806=FACE_OUTER_BOUND('',#26642,.T.) ;
#20807=FACE_OUTER_BOUND('',#26643,.T.) ;
#20808=FACE_OUTER_BOUND('',#26644,.T.) ;
#20809=FACE_OUTER_BOUND('',#26645,.T.) ;
#20810=FACE_OUTER_BOUND('',#26646,.T.) ;
#20811=FACE_OUTER_BOUND('',#26647,.T.) ;
#20812=FACE_OUTER_BOUND('',#26648,.T.) ;
#20813=FACE_OUTER_BOUND('',#26649,.T.) ;
#20814=FACE_OUTER_BOUND('',#26650,.T.) ;
#20815=FACE_OUTER_BOUND('',#26651,.T.) ;
#20816=FACE_OUTER_BOUND('',#26652,.T.) ;
#20817=FACE_OUTER_BOUND('',#26653,.T.) ;
#20818=FACE_OUTER_BOUND('',#26654,.T.) ;
#20819=FACE_OUTER_BOUND('',#26655,.T.) ;
#20820=FACE_OUTER_BOUND('',#26656,.T.) ;
#20821=FACE_OUTER_BOUND('',#26657,.T.) ;
#20822=FACE_OUTER_BOUND('',#26658,.T.) ;
#20823=FACE_OUTER_BOUND('',#26659,.T.) ;
#20824=FACE_OUTER_BOUND('',#26660,.T.) ;
#20825=FACE_OUTER_BOUND('',#26661,.T.) ;
#20826=FACE_OUTER_BOUND('',#26662,.T.) ;
#20827=FACE_OUTER_BOUND('',#26663,.T.) ;
#20828=FACE_OUTER_BOUND('',#26664,.T.) ;
#20829=FACE_OUTER_BOUND('',#26665,.T.) ;
#20830=FACE_OUTER_BOUND('',#26666,.T.) ;
#20831=FACE_OUTER_BOUND('',#26667,.T.) ;
#20832=FACE_OUTER_BOUND('',#26668,.T.) ;
#20833=FACE_OUTER_BOUND('',#26669,.T.) ;
#20834=FACE_OUTER_BOUND('',#26670,.T.) ;
#20835=FACE_OUTER_BOUND('',#26671,.T.) ;
#20836=FACE_OUTER_BOUND('',#26672,.T.) ;
#20837=FACE_OUTER_BOUND('',#26673,.T.) ;
#20838=FACE_OUTER_BOUND('',#26674,.T.) ;
#20839=FACE_OUTER_BOUND('',#26675,.T.) ;
#20840=FACE_OUTER_BOUND('',#26676,.T.) ;
#20841=FACE_OUTER_BOUND('',#26677,.T.) ;
#20842=FACE_OUTER_BOUND('',#26678,.T.) ;
#20843=FACE_OUTER_BOUND('',#26679,.T.) ;
#20844=FACE_OUTER_BOUND('',#26680,.T.) ;
#20845=FACE_OUTER_BOUND('',#26681,.T.) ;
#20846=FACE_OUTER_BOUND('',#26682,.T.) ;
#20847=FACE_OUTER_BOUND('',#26683,.T.) ;
#20848=FACE_OUTER_BOUND('',#26684,.T.) ;
#20849=FACE_OUTER_BOUND('',#26685,.T.) ;
#20850=FACE_OUTER_BOUND('',#26686,.T.) ;
#20851=FACE_OUTER_BOUND('',#26687,.T.) ;
#20852=FACE_OUTER_BOUND('',#26688,.T.) ;
#20853=FACE_OUTER_BOUND('',#26689,.T.) ;
#20854=FACE_OUTER_BOUND('',#26690,.T.) ;
#20855=FACE_OUTER_BOUND('',#26691,.T.) ;
#20856=FACE_OUTER_BOUND('',#26692,.T.) ;
#20857=FACE_OUTER_BOUND('',#26693,.T.) ;
#20858=FACE_OUTER_BOUND('',#26694,.T.) ;
#20859=FACE_OUTER_BOUND('',#26695,.T.) ;
#20860=FACE_OUTER_BOUND('',#26696,.T.) ;
#20861=FACE_OUTER_BOUND('',#26697,.T.) ;
#20862=FACE_OUTER_BOUND('',#26698,.T.) ;
#20863=FACE_OUTER_BOUND('',#26699,.T.) ;
#20864=FACE_OUTER_BOUND('',#26700,.T.) ;
#20865=FACE_OUTER_BOUND('',#26701,.T.) ;
#20866=FACE_OUTER_BOUND('',#26702,.T.) ;
#20867=FACE_OUTER_BOUND('',#26703,.T.) ;
#20868=FACE_OUTER_BOUND('',#26704,.T.) ;
#20869=FACE_OUTER_BOUND('',#26705,.T.) ;
#20870=FACE_OUTER_BOUND('',#26706,.T.) ;
#20871=FACE_OUTER_BOUND('',#26707,.T.) ;
#20872=FACE_OUTER_BOUND('',#26708,.T.) ;
#20873=FACE_OUTER_BOUND('',#26709,.T.) ;
#20874=FACE_OUTER_BOUND('',#26710,.T.) ;
#20875=FACE_OUTER_BOUND('',#26711,.T.) ;
#20876=FACE_OUTER_BOUND('',#26712,.T.) ;
#20877=FACE_OUTER_BOUND('',#26713,.T.) ;
#20878=FACE_OUTER_BOUND('',#26714,.T.) ;
#20879=FACE_OUTER_BOUND('',#26716,.T.) ;
#20880=FACE_OUTER_BOUND('',#26717,.T.) ;
#20881=FACE_OUTER_BOUND('',#26718,.T.) ;
#20882=FACE_OUTER_BOUND('',#26719,.T.) ;
#20883=FACE_OUTER_BOUND('',#26720,.T.) ;
#20884=FACE_OUTER_BOUND('',#26722,.T.) ;
#20885=FACE_OUTER_BOUND('',#26723,.T.) ;
#20886=FACE_OUTER_BOUND('',#26724,.T.) ;
#20887=FACE_OUTER_BOUND('',#26725,.T.) ;
#20888=FACE_OUTER_BOUND('',#26726,.T.) ;
#20889=FACE_OUTER_BOUND('',#26728,.T.) ;
#20890=FACE_OUTER_BOUND('',#26729,.T.) ;
#20891=FACE_OUTER_BOUND('',#26730,.T.) ;
#20892=FACE_OUTER_BOUND('',#26731,.T.) ;
#20893=FACE_OUTER_BOUND('',#26732,.T.) ;
#20894=FACE_OUTER_BOUND('',#26734,.T.) ;
#20895=FACE_OUTER_BOUND('',#26735,.T.) ;
#20896=FACE_OUTER_BOUND('',#26736,.T.) ;
#20897=FACE_OUTER_BOUND('',#26737,.T.) ;
#20898=FACE_OUTER_BOUND('',#26738,.T.) ;
#20899=FACE_OUTER_BOUND('',#26740,.T.) ;
#20900=FACE_OUTER_BOUND('',#26741,.T.) ;
#20901=FACE_OUTER_BOUND('',#26742,.T.) ;
#20902=FACE_OUTER_BOUND('',#26743,.T.) ;
#20903=FACE_OUTER_BOUND('',#26744,.T.) ;
#20904=FACE_OUTER_BOUND('',#26746,.T.) ;
#20905=FACE_OUTER_BOUND('',#26747,.T.) ;
#20906=FACE_OUTER_BOUND('',#26748,.T.) ;
#20907=FACE_OUTER_BOUND('',#26749,.T.) ;
#20908=FACE_OUTER_BOUND('',#26750,.T.) ;
#20909=FACE_OUTER_BOUND('',#26752,.T.) ;
#20910=FACE_OUTER_BOUND('',#26753,.T.) ;
#20911=FACE_OUTER_BOUND('',#26754,.T.) ;
#20912=FACE_OUTER_BOUND('',#26755,.T.) ;
#20913=FACE_OUTER_BOUND('',#26756,.T.) ;
#20914=FACE_OUTER_BOUND('',#26758,.T.) ;
#20915=FACE_OUTER_BOUND('',#26759,.T.) ;
#20916=FACE_OUTER_BOUND('',#26760,.T.) ;
#20917=FACE_OUTER_BOUND('',#26761,.T.) ;
#20918=FACE_OUTER_BOUND('',#26762,.T.) ;
#20919=FACE_OUTER_BOUND('',#26764,.T.) ;
#20920=FACE_OUTER_BOUND('',#26765,.T.) ;
#20921=FACE_OUTER_BOUND('',#26766,.T.) ;
#20922=FACE_OUTER_BOUND('',#26767,.T.) ;
#20923=FACE_OUTER_BOUND('',#26768,.T.) ;
#20924=FACE_OUTER_BOUND('',#26769,.T.) ;
#20925=FACE_OUTER_BOUND('',#26770,.T.) ;
#20926=FACE_OUTER_BOUND('',#26771,.T.) ;
#20927=FACE_OUTER_BOUND('',#26772,.T.) ;
#20928=FACE_OUTER_BOUND('',#26773,.T.) ;
#20929=FACE_OUTER_BOUND('',#26774,.T.) ;
#20930=FACE_OUTER_BOUND('',#26775,.T.) ;
#20931=FACE_OUTER_BOUND('',#26776,.T.) ;
#20932=FACE_OUTER_BOUND('',#26777,.T.) ;
#20933=FACE_OUTER_BOUND('',#26778,.T.) ;
#20934=FACE_OUTER_BOUND('',#26779,.T.) ;
#20935=FACE_OUTER_BOUND('',#26780,.T.) ;
#20936=FACE_OUTER_BOUND('',#26781,.T.) ;
#20937=FACE_OUTER_BOUND('',#26782,.T.) ;
#20938=FACE_OUTER_BOUND('',#26783,.T.) ;
#20939=FACE_OUTER_BOUND('',#26784,.T.) ;
#20940=FACE_OUTER_BOUND('',#26785,.T.) ;
#20941=FACE_OUTER_BOUND('',#26786,.T.) ;
#20942=FACE_OUTER_BOUND('',#26787,.T.) ;
#20943=FACE_OUTER_BOUND('',#26788,.T.) ;
#20944=FACE_OUTER_BOUND('',#26789,.T.) ;
#20945=FACE_OUTER_BOUND('',#26790,.T.) ;
#20946=FACE_OUTER_BOUND('',#26791,.T.) ;
#20947=FACE_OUTER_BOUND('',#26792,.T.) ;
#20948=FACE_OUTER_BOUND('',#26793,.T.) ;
#20949=FACE_OUTER_BOUND('',#26794,.T.) ;
#20950=FACE_OUTER_BOUND('',#26795,.T.) ;
#20951=FACE_OUTER_BOUND('',#26796,.T.) ;
#20952=FACE_OUTER_BOUND('',#26797,.T.) ;
#20953=FACE_OUTER_BOUND('',#26798,.T.) ;
#20954=FACE_OUTER_BOUND('',#26799,.T.) ;
#20955=FACE_OUTER_BOUND('',#26800,.T.) ;
#20956=FACE_OUTER_BOUND('',#26801,.T.) ;
#20957=FACE_OUTER_BOUND('',#26802,.T.) ;
#20958=FACE_OUTER_BOUND('',#26803,.T.) ;
#20959=FACE_OUTER_BOUND('',#26804,.T.) ;
#20960=FACE_OUTER_BOUND('',#26805,.T.) ;
#20961=FACE_OUTER_BOUND('',#26806,.T.) ;
#20962=FACE_OUTER_BOUND('',#26807,.T.) ;
#20963=FACE_OUTER_BOUND('',#26808,.T.) ;
#20964=FACE_OUTER_BOUND('',#26809,.T.) ;
#20965=FACE_OUTER_BOUND('',#26810,.T.) ;
#20966=FACE_OUTER_BOUND('',#26811,.T.) ;
#20967=FACE_OUTER_BOUND('',#26812,.T.) ;
#20968=FACE_OUTER_BOUND('',#26813,.T.) ;
#20969=FACE_OUTER_BOUND('',#26814,.T.) ;
#20970=FACE_OUTER_BOUND('',#26815,.T.) ;
#20971=FACE_OUTER_BOUND('',#26816,.T.) ;
#20972=FACE_OUTER_BOUND('',#26818,.T.) ;
#20973=FACE_OUTER_BOUND('',#26819,.T.) ;
#20974=FACE_OUTER_BOUND('',#26820,.T.) ;
#20975=FACE_OUTER_BOUND('',#26821,.T.) ;
#20976=FACE_OUTER_BOUND('',#26823,.T.) ;
#20977=FACE_OUTER_BOUND('',#26824,.T.) ;
#20978=FACE_OUTER_BOUND('',#26825,.T.) ;
#20979=FACE_OUTER_BOUND('',#26826,.T.) ;
#20980=FACE_OUTER_BOUND('',#26828,.T.) ;
#20981=FACE_OUTER_BOUND('',#26829,.T.) ;
#20982=FACE_OUTER_BOUND('',#26830,.T.) ;
#20983=FACE_OUTER_BOUND('',#26831,.T.) ;
#20984=FACE_OUTER_BOUND('',#26833,.T.) ;
#20985=FACE_OUTER_BOUND('',#26834,.T.) ;
#20986=FACE_OUTER_BOUND('',#26835,.T.) ;
#20987=FACE_OUTER_BOUND('',#26836,.T.) ;
#20988=FACE_OUTER_BOUND('',#26838,.T.) ;
#20989=FACE_OUTER_BOUND('',#26839,.T.) ;
#20990=FACE_OUTER_BOUND('',#26840,.T.) ;
#20991=FACE_OUTER_BOUND('',#26841,.T.) ;
#20992=FACE_OUTER_BOUND('',#26843,.T.) ;
#20993=FACE_OUTER_BOUND('',#26844,.T.) ;
#20994=FACE_OUTER_BOUND('',#26845,.T.) ;
#20995=FACE_OUTER_BOUND('',#26846,.T.) ;
#20996=FACE_OUTER_BOUND('',#26848,.T.) ;
#20997=FACE_OUTER_BOUND('',#26849,.T.) ;
#20998=FACE_OUTER_BOUND('',#26850,.T.) ;
#20999=FACE_OUTER_BOUND('',#26851,.T.) ;
#21000=FACE_OUTER_BOUND('',#26853,.T.) ;
#21001=FACE_OUTER_BOUND('',#26854,.T.) ;
#21002=FACE_OUTER_BOUND('',#26855,.T.) ;
#21003=FACE_OUTER_BOUND('',#26856,.T.) ;
#21004=FACE_OUTER_BOUND('',#26858,.T.) ;
#21005=FACE_OUTER_BOUND('',#26859,.T.) ;
#21006=FACE_OUTER_BOUND('',#26860,.T.) ;
#21007=FACE_OUTER_BOUND('',#26861,.T.) ;
#21008=FACE_OUTER_BOUND('',#26862,.T.) ;
#21009=FACE_OUTER_BOUND('',#26863,.T.) ;
#21010=FACE_OUTER_BOUND('',#26864,.T.) ;
#21011=FACE_OUTER_BOUND('',#26865,.T.) ;
#21012=FACE_OUTER_BOUND('',#26866,.T.) ;
#21013=FACE_OUTER_BOUND('',#26867,.T.) ;
#21014=FACE_OUTER_BOUND('',#26868,.T.) ;
#21015=FACE_OUTER_BOUND('',#26869,.T.) ;
#21016=FACE_OUTER_BOUND('',#26870,.T.) ;
#21017=FACE_OUTER_BOUND('',#26871,.T.) ;
#21018=FACE_OUTER_BOUND('',#26872,.T.) ;
#21019=FACE_OUTER_BOUND('',#26873,.T.) ;
#21020=FACE_OUTER_BOUND('',#26874,.T.) ;
#21021=FACE_OUTER_BOUND('',#26875,.T.) ;
#21022=FACE_OUTER_BOUND('',#26876,.T.) ;
#21023=FACE_OUTER_BOUND('',#26877,.T.) ;
#21024=FACE_OUTER_BOUND('',#26878,.T.) ;
#21025=FACE_OUTER_BOUND('',#26879,.T.) ;
#21026=FACE_OUTER_BOUND('',#26880,.T.) ;
#21027=FACE_OUTER_BOUND('',#26881,.T.) ;
#21028=FACE_OUTER_BOUND('',#26882,.T.) ;
#21029=FACE_OUTER_BOUND('',#26883,.T.) ;
#21030=FACE_OUTER_BOUND('',#26884,.T.) ;
#21031=FACE_OUTER_BOUND('',#26885,.T.) ;
#21032=FACE_OUTER_BOUND('',#26886,.T.) ;
#21033=FACE_OUTER_BOUND('',#26887,.T.) ;
#21034=FACE_OUTER_BOUND('',#26888,.T.) ;
#21035=FACE_OUTER_BOUND('',#26889,.T.) ;
#21036=FACE_OUTER_BOUND('',#26890,.T.) ;
#21037=FACE_OUTER_BOUND('',#26891,.T.) ;
#21038=FACE_OUTER_BOUND('',#26892,.T.) ;
#21039=FACE_OUTER_BOUND('',#26893,.T.) ;
#21040=FACE_OUTER_BOUND('',#26894,.T.) ;
#21041=FACE_OUTER_BOUND('',#26895,.T.) ;
#21042=FACE_OUTER_BOUND('',#26896,.T.) ;
#21043=FACE_OUTER_BOUND('',#26897,.T.) ;
#21044=FACE_OUTER_BOUND('',#26898,.T.) ;
#21045=FACE_OUTER_BOUND('',#26899,.T.) ;
#21046=FACE_OUTER_BOUND('',#26900,.T.) ;
#21047=FACE_OUTER_BOUND('',#26901,.T.) ;
#21048=FACE_OUTER_BOUND('',#26902,.T.) ;
#21049=FACE_OUTER_BOUND('',#26903,.T.) ;
#21050=FACE_OUTER_BOUND('',#26905,.T.) ;
#21051=FACE_OUTER_BOUND('',#26906,.T.) ;
#21052=FACE_OUTER_BOUND('',#26907,.T.) ;
#21053=FACE_OUTER_BOUND('',#26908,.T.) ;
#21054=FACE_OUTER_BOUND('',#26909,.T.) ;
#21055=FACE_OUTER_BOUND('',#26911,.T.) ;
#21056=FACE_OUTER_BOUND('',#26912,.T.) ;
#21057=FACE_OUTER_BOUND('',#26913,.T.) ;
#21058=FACE_OUTER_BOUND('',#26914,.T.) ;
#21059=FACE_OUTER_BOUND('',#26915,.T.) ;
#21060=FACE_OUTER_BOUND('',#26917,.T.) ;
#21061=FACE_OUTER_BOUND('',#26918,.T.) ;
#21062=FACE_OUTER_BOUND('',#26919,.T.) ;
#21063=FACE_OUTER_BOUND('',#26920,.T.) ;
#21064=FACE_OUTER_BOUND('',#26921,.T.) ;
#21065=FACE_OUTER_BOUND('',#26923,.T.) ;
#21066=FACE_OUTER_BOUND('',#26924,.T.) ;
#21067=FACE_OUTER_BOUND('',#26925,.T.) ;
#21068=FACE_OUTER_BOUND('',#26926,.T.) ;
#21069=FACE_OUTER_BOUND('',#26927,.T.) ;
#21070=FACE_OUTER_BOUND('',#26929,.T.) ;
#21071=FACE_OUTER_BOUND('',#26930,.T.) ;
#21072=FACE_OUTER_BOUND('',#26931,.T.) ;
#21073=FACE_OUTER_BOUND('',#26932,.T.) ;
#21074=FACE_OUTER_BOUND('',#26933,.T.) ;
#21075=FACE_OUTER_BOUND('',#26935,.T.) ;
#21076=FACE_OUTER_BOUND('',#26936,.T.) ;
#21077=FACE_OUTER_BOUND('',#26937,.T.) ;
#21078=FACE_OUTER_BOUND('',#26938,.T.) ;
#21079=FACE_OUTER_BOUND('',#26939,.T.) ;
#21080=FACE_OUTER_BOUND('',#26941,.T.) ;
#21081=FACE_OUTER_BOUND('',#26942,.T.) ;
#21082=FACE_OUTER_BOUND('',#26943,.T.) ;
#21083=FACE_OUTER_BOUND('',#26944,.T.) ;
#21084=FACE_OUTER_BOUND('',#26945,.T.) ;
#21085=FACE_OUTER_BOUND('',#26947,.T.) ;
#21086=FACE_OUTER_BOUND('',#26948,.T.) ;
#21087=FACE_OUTER_BOUND('',#26949,.T.) ;
#21088=FACE_OUTER_BOUND('',#26950,.T.) ;
#21089=FACE_OUTER_BOUND('',#26951,.T.) ;
#21090=FACE_OUTER_BOUND('',#26953,.T.) ;
#21091=FACE_OUTER_BOUND('',#26954,.T.) ;
#21092=FACE_OUTER_BOUND('',#26955,.T.) ;
#21093=FACE_OUTER_BOUND('',#26956,.T.) ;
#21094=FACE_OUTER_BOUND('',#26957,.T.) ;
#21095=FACE_OUTER_BOUND('',#26958,.T.) ;
#21096=FACE_OUTER_BOUND('',#26959,.T.) ;
#21097=FACE_OUTER_BOUND('',#26960,.T.) ;
#21098=FACE_OUTER_BOUND('',#26961,.T.) ;
#21099=FACE_OUTER_BOUND('',#26962,.T.) ;
#21100=FACE_OUTER_BOUND('',#26963,.T.) ;
#21101=FACE_OUTER_BOUND('',#26964,.T.) ;
#21102=FACE_OUTER_BOUND('',#26965,.T.) ;
#21103=FACE_OUTER_BOUND('',#26966,.T.) ;
#21104=FACE_OUTER_BOUND('',#26967,.T.) ;
#21105=FACE_OUTER_BOUND('',#26968,.T.) ;
#21106=FACE_OUTER_BOUND('',#26969,.T.) ;
#21107=FACE_OUTER_BOUND('',#26970,.T.) ;
#21108=FACE_OUTER_BOUND('',#26971,.T.) ;
#21109=FACE_OUTER_BOUND('',#26972,.T.) ;
#21110=FACE_OUTER_BOUND('',#26973,.T.) ;
#21111=FACE_OUTER_BOUND('',#26974,.T.) ;
#21112=FACE_OUTER_BOUND('',#26975,.T.) ;
#21113=FACE_OUTER_BOUND('',#26976,.T.) ;
#21114=FACE_OUTER_BOUND('',#26977,.T.) ;
#21115=FACE_OUTER_BOUND('',#26978,.T.) ;
#21116=FACE_OUTER_BOUND('',#26979,.T.) ;
#21117=FACE_OUTER_BOUND('',#26980,.T.) ;
#21118=FACE_OUTER_BOUND('',#26981,.T.) ;
#21119=FACE_OUTER_BOUND('',#26982,.T.) ;
#21120=FACE_OUTER_BOUND('',#26983,.T.) ;
#21121=FACE_OUTER_BOUND('',#26984,.T.) ;
#21122=FACE_OUTER_BOUND('',#26985,.T.) ;
#21123=FACE_OUTER_BOUND('',#26986,.T.) ;
#21124=FACE_OUTER_BOUND('',#26987,.T.) ;
#21125=FACE_OUTER_BOUND('',#26988,.T.) ;
#21126=FACE_OUTER_BOUND('',#26989,.T.) ;
#21127=FACE_OUTER_BOUND('',#26990,.T.) ;
#21128=FACE_OUTER_BOUND('',#26991,.T.) ;
#21129=FACE_OUTER_BOUND('',#26992,.T.) ;
#21130=FACE_OUTER_BOUND('',#26993,.T.) ;
#21131=FACE_OUTER_BOUND('',#26994,.T.) ;
#21132=FACE_OUTER_BOUND('',#26995,.T.) ;
#21133=FACE_OUTER_BOUND('',#26996,.T.) ;
#21134=FACE_OUTER_BOUND('',#26997,.T.) ;
#21135=FACE_OUTER_BOUND('',#26998,.T.) ;
#21136=FACE_OUTER_BOUND('',#26999,.T.) ;
#21137=FACE_OUTER_BOUND('',#27000,.T.) ;
#21138=FACE_OUTER_BOUND('',#27001,.T.) ;
#21139=FACE_OUTER_BOUND('',#27002,.T.) ;
#21140=FACE_OUTER_BOUND('',#27003,.T.) ;
#21141=FACE_OUTER_BOUND('',#27004,.T.) ;
#21142=FACE_OUTER_BOUND('',#27005,.T.) ;
#21143=FACE_OUTER_BOUND('',#27006,.T.) ;
#21144=FACE_OUTER_BOUND('',#27007,.T.) ;
#21145=FACE_OUTER_BOUND('',#27008,.T.) ;
#21146=FACE_OUTER_BOUND('',#27009,.T.) ;
#21147=FACE_OUTER_BOUND('',#27010,.T.) ;
#21148=FACE_OUTER_BOUND('',#27011,.T.) ;
#21149=FACE_OUTER_BOUND('',#27012,.T.) ;
#21150=FACE_OUTER_BOUND('',#27013,.T.) ;
#21151=FACE_OUTER_BOUND('',#27014,.T.) ;
#21152=FACE_OUTER_BOUND('',#27015,.T.) ;
#21153=FACE_OUTER_BOUND('',#27016,.T.) ;
#21154=FACE_OUTER_BOUND('',#27017,.T.) ;
#21155=FACE_OUTER_BOUND('',#27018,.T.) ;
#21156=FACE_OUTER_BOUND('',#27019,.T.) ;
#21157=FACE_OUTER_BOUND('',#27020,.T.) ;
#21158=FACE_OUTER_BOUND('',#27021,.T.) ;
#21159=FACE_OUTER_BOUND('',#27022,.T.) ;
#21160=FACE_OUTER_BOUND('',#27023,.T.) ;
#21161=FACE_OUTER_BOUND('',#27024,.T.) ;
#21162=FACE_OUTER_BOUND('',#27025,.T.) ;
#21163=FACE_OUTER_BOUND('',#27026,.T.) ;
#21164=FACE_OUTER_BOUND('',#27027,.T.) ;
#21165=FACE_OUTER_BOUND('',#27028,.T.) ;
#21166=FACE_OUTER_BOUND('',#27029,.T.) ;
#21167=FACE_OUTER_BOUND('',#27030,.T.) ;
#21168=FACE_OUTER_BOUND('',#27031,.T.) ;
#21169=FACE_OUTER_BOUND('',#27032,.T.) ;
#21170=FACE_OUTER_BOUND('',#27033,.T.) ;
#21171=FACE_OUTER_BOUND('',#27034,.T.) ;
#21172=FACE_OUTER_BOUND('',#27035,.T.) ;
#21173=FACE_OUTER_BOUND('',#27036,.T.) ;
#21174=FACE_OUTER_BOUND('',#27037,.T.) ;
#21175=FACE_OUTER_BOUND('',#27038,.T.) ;
#21176=FACE_OUTER_BOUND('',#27039,.T.) ;
#21177=FACE_OUTER_BOUND('',#27040,.T.) ;
#21178=FACE_OUTER_BOUND('',#27041,.T.) ;
#21179=FACE_OUTER_BOUND('',#27042,.T.) ;
#21180=FACE_OUTER_BOUND('',#27043,.T.) ;
#21181=FACE_OUTER_BOUND('',#27044,.T.) ;
#21182=FACE_OUTER_BOUND('',#27045,.T.) ;
#21183=FACE_OUTER_BOUND('',#27046,.T.) ;
#21184=FACE_OUTER_BOUND('',#27047,.T.) ;
#21185=FACE_OUTER_BOUND('',#27048,.T.) ;
#21186=FACE_OUTER_BOUND('',#27049,.T.) ;
#21187=FACE_OUTER_BOUND('',#27050,.T.) ;
#21188=FACE_OUTER_BOUND('',#27051,.T.) ;
#21189=FACE_OUTER_BOUND('',#27052,.T.) ;
#21190=FACE_OUTER_BOUND('',#27053,.T.) ;
#21191=FACE_OUTER_BOUND('',#27054,.T.) ;
#21192=FACE_OUTER_BOUND('',#27055,.T.) ;
#21193=FACE_OUTER_BOUND('',#27056,.T.) ;
#21194=FACE_OUTER_BOUND('',#27057,.T.) ;
#21195=FACE_OUTER_BOUND('',#27058,.T.) ;
#21196=FACE_OUTER_BOUND('',#27059,.T.) ;
#21197=FACE_OUTER_BOUND('',#27060,.T.) ;
#21198=FACE_OUTER_BOUND('',#27061,.T.) ;
#21199=FACE_OUTER_BOUND('',#27062,.T.) ;
#21200=FACE_OUTER_BOUND('',#27063,.T.) ;
#21201=FACE_OUTER_BOUND('',#27064,.T.) ;
#21202=FACE_OUTER_BOUND('',#27065,.T.) ;
#21203=FACE_OUTER_BOUND('',#27066,.T.) ;
#21204=FACE_OUTER_BOUND('',#27067,.T.) ;
#21205=FACE_OUTER_BOUND('',#27068,.T.) ;
#21206=FACE_OUTER_BOUND('',#27069,.T.) ;
#21207=FACE_OUTER_BOUND('',#27070,.T.) ;
#21208=FACE_OUTER_BOUND('',#27071,.T.) ;
#21209=FACE_OUTER_BOUND('',#27072,.T.) ;
#21210=FACE_OUTER_BOUND('',#27073,.T.) ;
#21211=FACE_OUTER_BOUND('',#27074,.T.) ;
#21212=FACE_OUTER_BOUND('',#27075,.T.) ;
#21213=FACE_OUTER_BOUND('',#27076,.T.) ;
#21214=FACE_OUTER_BOUND('',#27077,.T.) ;
#21215=FACE_OUTER_BOUND('',#27078,.T.) ;
#21216=FACE_OUTER_BOUND('',#27079,.T.) ;
#21217=FACE_OUTER_BOUND('',#27080,.T.) ;
#21218=FACE_OUTER_BOUND('',#27081,.T.) ;
#21219=FACE_OUTER_BOUND('',#27082,.T.) ;
#21220=FACE_OUTER_BOUND('',#27083,.T.) ;
#21221=FACE_OUTER_BOUND('',#27084,.T.) ;
#21222=FACE_OUTER_BOUND('',#27085,.T.) ;
#21223=FACE_OUTER_BOUND('',#27086,.T.) ;
#21224=FACE_OUTER_BOUND('',#27087,.T.) ;
#21225=FACE_OUTER_BOUND('',#27088,.T.) ;
#21226=FACE_OUTER_BOUND('',#27089,.T.) ;
#21227=FACE_OUTER_BOUND('',#27090,.T.) ;
#21228=FACE_OUTER_BOUND('',#27091,.T.) ;
#21229=FACE_OUTER_BOUND('',#27092,.T.) ;
#21230=FACE_OUTER_BOUND('',#27093,.T.) ;
#21231=FACE_OUTER_BOUND('',#27094,.T.) ;
#21232=FACE_OUTER_BOUND('',#27095,.T.) ;
#21233=FACE_OUTER_BOUND('',#27096,.T.) ;
#21234=FACE_OUTER_BOUND('',#27097,.T.) ;
#21235=FACE_OUTER_BOUND('',#27098,.T.) ;
#21236=FACE_OUTER_BOUND('',#27099,.T.) ;
#21237=FACE_OUTER_BOUND('',#27100,.T.) ;
#21238=FACE_OUTER_BOUND('',#27101,.T.) ;
#21239=FACE_OUTER_BOUND('',#27102,.T.) ;
#21240=FACE_OUTER_BOUND('',#27103,.T.) ;
#21241=FACE_OUTER_BOUND('',#27104,.T.) ;
#21242=FACE_OUTER_BOUND('',#27105,.T.) ;
#21243=FACE_OUTER_BOUND('',#27106,.T.) ;
#21244=FACE_OUTER_BOUND('',#27107,.T.) ;
#21245=FACE_OUTER_BOUND('',#27108,.T.) ;
#21246=FACE_OUTER_BOUND('',#27109,.T.) ;
#21247=FACE_OUTER_BOUND('',#27110,.T.) ;
#21248=FACE_OUTER_BOUND('',#27111,.T.) ;
#21249=FACE_OUTER_BOUND('',#27112,.T.) ;
#21250=FACE_OUTER_BOUND('',#27113,.T.) ;
#21251=FACE_OUTER_BOUND('',#27114,.T.) ;
#21252=FACE_OUTER_BOUND('',#27115,.T.) ;
#21253=FACE_OUTER_BOUND('',#27116,.T.) ;
#21254=FACE_OUTER_BOUND('',#27117,.T.) ;
#21255=FACE_OUTER_BOUND('',#27118,.T.) ;
#21256=FACE_OUTER_BOUND('',#27119,.T.) ;
#21257=FACE_OUTER_BOUND('',#27120,.T.) ;
#21258=FACE_OUTER_BOUND('',#27121,.T.) ;
#21259=FACE_OUTER_BOUND('',#27122,.T.) ;
#21260=FACE_OUTER_BOUND('',#27123,.T.) ;
#21261=FACE_OUTER_BOUND('',#27124,.T.) ;
#21262=FACE_OUTER_BOUND('',#27125,.T.) ;
#21263=FACE_OUTER_BOUND('',#27126,.T.) ;
#21264=FACE_OUTER_BOUND('',#27127,.T.) ;
#21265=FACE_OUTER_BOUND('',#27128,.T.) ;
#21266=FACE_OUTER_BOUND('',#27129,.T.) ;
#21267=FACE_OUTER_BOUND('',#27130,.T.) ;
#21268=FACE_OUTER_BOUND('',#27131,.T.) ;
#21269=FACE_OUTER_BOUND('',#27132,.T.) ;
#21270=FACE_OUTER_BOUND('',#27133,.T.) ;
#21271=FACE_OUTER_BOUND('',#27134,.T.) ;
#21272=FACE_OUTER_BOUND('',#27135,.T.) ;
#21273=FACE_OUTER_BOUND('',#27136,.T.) ;
#21274=FACE_OUTER_BOUND('',#27137,.T.) ;
#21275=FACE_OUTER_BOUND('',#27138,.T.) ;
#21276=FACE_OUTER_BOUND('',#27139,.T.) ;
#21277=FACE_OUTER_BOUND('',#27140,.T.) ;
#21278=FACE_OUTER_BOUND('',#27141,.T.) ;
#21279=FACE_OUTER_BOUND('',#27142,.T.) ;
#21280=FACE_OUTER_BOUND('',#27143,.T.) ;
#21281=FACE_OUTER_BOUND('',#27144,.T.) ;
#21282=FACE_OUTER_BOUND('',#27145,.T.) ;
#21283=FACE_OUTER_BOUND('',#27146,.T.) ;
#21284=FACE_OUTER_BOUND('',#27147,.T.) ;
#21285=FACE_OUTER_BOUND('',#27148,.T.) ;
#21286=FACE_OUTER_BOUND('',#27149,.T.) ;
#21287=FACE_OUTER_BOUND('',#27150,.T.) ;
#21288=FACE_OUTER_BOUND('',#27151,.T.) ;
#21289=FACE_OUTER_BOUND('',#27152,.T.) ;
#21290=FACE_OUTER_BOUND('',#27153,.T.) ;
#21291=FACE_OUTER_BOUND('',#27154,.T.) ;
#21292=FACE_OUTER_BOUND('',#27155,.T.) ;
#21293=FACE_OUTER_BOUND('',#27156,.T.) ;
#21294=FACE_OUTER_BOUND('',#27157,.T.) ;
#21295=FACE_OUTER_BOUND('',#27158,.T.) ;
#21296=FACE_OUTER_BOUND('',#27159,.T.) ;
#21297=FACE_OUTER_BOUND('',#27160,.T.) ;
#21298=FACE_OUTER_BOUND('',#27161,.T.) ;
#21299=FACE_OUTER_BOUND('',#27162,.T.) ;
#21300=FACE_OUTER_BOUND('',#27163,.T.) ;
#21301=FACE_OUTER_BOUND('',#27164,.T.) ;
#21302=FACE_OUTER_BOUND('',#27165,.T.) ;
#21303=FACE_OUTER_BOUND('',#27166,.T.) ;
#21304=FACE_OUTER_BOUND('',#27167,.T.) ;
#21305=FACE_OUTER_BOUND('',#27168,.T.) ;
#21306=FACE_OUTER_BOUND('',#27169,.T.) ;
#21307=FACE_OUTER_BOUND('',#27170,.T.) ;
#21308=FACE_OUTER_BOUND('',#27171,.T.) ;
#21309=FACE_OUTER_BOUND('',#27172,.T.) ;
#21310=FACE_OUTER_BOUND('',#27173,.T.) ;
#21311=FACE_OUTER_BOUND('',#27174,.T.) ;
#21312=FACE_OUTER_BOUND('',#27175,.T.) ;
#21313=FACE_OUTER_BOUND('',#27176,.T.) ;
#21314=FACE_OUTER_BOUND('',#27177,.T.) ;
#21315=FACE_OUTER_BOUND('',#27178,.T.) ;
#21316=FACE_OUTER_BOUND('',#27179,.T.) ;
#21317=FACE_OUTER_BOUND('',#27180,.T.) ;
#21318=FACE_OUTER_BOUND('',#27181,.T.) ;
#21319=FACE_OUTER_BOUND('',#27182,.T.) ;
#21320=FACE_OUTER_BOUND('',#27183,.T.) ;
#21321=FACE_OUTER_BOUND('',#27184,.T.) ;
#21322=FACE_OUTER_BOUND('',#27185,.T.) ;
#21323=FACE_OUTER_BOUND('',#27186,.T.) ;
#21324=FACE_OUTER_BOUND('',#27187,.T.) ;
#21325=FACE_OUTER_BOUND('',#27188,.T.) ;
#21326=FACE_OUTER_BOUND('',#27189,.T.) ;
#21327=FACE_OUTER_BOUND('',#27190,.T.) ;
#21328=FACE_OUTER_BOUND('',#27191,.T.) ;
#21329=FACE_OUTER_BOUND('',#27192,.T.) ;
#21330=FACE_OUTER_BOUND('',#27193,.T.) ;
#21331=FACE_OUTER_BOUND('',#27194,.T.) ;
#21332=FACE_OUTER_BOUND('',#27195,.T.) ;
#21333=FACE_OUTER_BOUND('',#27196,.T.) ;
#21334=FACE_OUTER_BOUND('',#27197,.T.) ;
#21335=FACE_OUTER_BOUND('',#27198,.T.) ;
#21336=FACE_OUTER_BOUND('',#27199,.T.) ;
#21337=FACE_OUTER_BOUND('',#27200,.T.) ;
#21338=FACE_OUTER_BOUND('',#27201,.T.) ;
#21339=FACE_OUTER_BOUND('',#27202,.T.) ;
#21340=FACE_OUTER_BOUND('',#27203,.T.) ;
#21341=FACE_OUTER_BOUND('',#27204,.T.) ;
#21342=FACE_OUTER_BOUND('',#27205,.T.) ;
#21343=FACE_OUTER_BOUND('',#27206,.T.) ;
#21344=FACE_OUTER_BOUND('',#27207,.T.) ;
#21345=FACE_OUTER_BOUND('',#27208,.T.) ;
#21346=FACE_OUTER_BOUND('',#27209,.T.) ;
#21347=FACE_OUTER_BOUND('',#27210,.T.) ;
#21348=FACE_OUTER_BOUND('',#27211,.T.) ;
#21349=FACE_OUTER_BOUND('',#27212,.T.) ;
#21350=FACE_OUTER_BOUND('',#27213,.T.) ;
#21351=FACE_OUTER_BOUND('',#27214,.T.) ;
#21352=FACE_OUTER_BOUND('',#27215,.T.) ;
#21353=FACE_OUTER_BOUND('',#27216,.T.) ;
#21354=FACE_OUTER_BOUND('',#27217,.T.) ;
#21355=FACE_OUTER_BOUND('',#27218,.T.) ;
#21356=FACE_OUTER_BOUND('',#27219,.T.) ;
#21357=FACE_OUTER_BOUND('',#27220,.T.) ;
#21358=FACE_OUTER_BOUND('',#27221,.T.) ;
#21359=FACE_OUTER_BOUND('',#27222,.T.) ;
#21360=FACE_OUTER_BOUND('',#27223,.T.) ;
#21361=FACE_OUTER_BOUND('',#27224,.T.) ;
#21362=FACE_OUTER_BOUND('',#27225,.T.) ;
#21363=FACE_OUTER_BOUND('',#27226,.T.) ;
#21364=FACE_OUTER_BOUND('',#27227,.T.) ;
#21365=FACE_OUTER_BOUND('',#27228,.T.) ;
#21366=FACE_OUTER_BOUND('',#27229,.T.) ;
#21367=FACE_OUTER_BOUND('',#27230,.T.) ;
#21368=FACE_OUTER_BOUND('',#27231,.T.) ;
#21369=FACE_OUTER_BOUND('',#27232,.T.) ;
#21370=FACE_OUTER_BOUND('',#27233,.T.) ;
#21371=FACE_OUTER_BOUND('',#27234,.T.) ;
#21372=FACE_OUTER_BOUND('',#27235,.T.) ;
#21373=FACE_OUTER_BOUND('',#27236,.T.) ;
#21374=FACE_OUTER_BOUND('',#27237,.T.) ;
#21375=FACE_OUTER_BOUND('',#27238,.T.) ;
#21376=FACE_OUTER_BOUND('',#27239,.T.) ;
#21377=FACE_OUTER_BOUND('',#27240,.T.) ;
#21378=FACE_OUTER_BOUND('',#27241,.T.) ;
#21379=FACE_OUTER_BOUND('',#27242,.T.) ;
#21380=FACE_OUTER_BOUND('',#27243,.T.) ;
#21381=FACE_OUTER_BOUND('',#27244,.T.) ;
#21382=FACE_OUTER_BOUND('',#27245,.T.) ;
#21383=FACE_OUTER_BOUND('',#27246,.T.) ;
#21384=FACE_OUTER_BOUND('',#27247,.T.) ;
#21385=FACE_OUTER_BOUND('',#27248,.T.) ;
#21386=FACE_OUTER_BOUND('',#27249,.T.) ;
#21387=FACE_OUTER_BOUND('',#27250,.T.) ;
#21388=FACE_OUTER_BOUND('',#27251,.T.) ;
#21389=FACE_OUTER_BOUND('',#27252,.T.) ;
#21390=FACE_OUTER_BOUND('',#27253,.T.) ;
#21391=FACE_OUTER_BOUND('',#27254,.T.) ;
#21392=FACE_OUTER_BOUND('',#27255,.T.) ;
#21393=FACE_OUTER_BOUND('',#27256,.T.) ;
#21394=FACE_OUTER_BOUND('',#27257,.T.) ;
#21395=FACE_OUTER_BOUND('',#27258,.T.) ;
#21396=FACE_OUTER_BOUND('',#27259,.T.) ;
#21397=FACE_OUTER_BOUND('',#27260,.T.) ;
#21398=FACE_OUTER_BOUND('',#27261,.T.) ;
#21399=FACE_OUTER_BOUND('',#27262,.T.) ;
#21400=FACE_OUTER_BOUND('',#27263,.T.) ;
#21401=FACE_OUTER_BOUND('',#27264,.T.) ;
#21402=FACE_OUTER_BOUND('',#27265,.T.) ;
#21403=FACE_OUTER_BOUND('',#27266,.T.) ;
#21404=FACE_OUTER_BOUND('',#27267,.T.) ;
#21405=FACE_OUTER_BOUND('',#27268,.T.) ;
#21406=FACE_OUTER_BOUND('',#27269,.T.) ;
#21407=FACE_OUTER_BOUND('',#27270,.T.) ;
#21408=FACE_OUTER_BOUND('',#27271,.T.) ;
#21409=FACE_OUTER_BOUND('',#27272,.T.) ;
#21410=FACE_OUTER_BOUND('',#27273,.T.) ;
#21411=FACE_OUTER_BOUND('',#27274,.T.) ;
#21412=FACE_OUTER_BOUND('',#27275,.T.) ;
#21413=FACE_OUTER_BOUND('',#27276,.T.) ;
#21414=FACE_OUTER_BOUND('',#27277,.T.) ;
#21415=FACE_OUTER_BOUND('',#27278,.T.) ;
#21416=FACE_OUTER_BOUND('',#27279,.T.) ;
#21417=FACE_OUTER_BOUND('',#27280,.T.) ;
#21418=FACE_OUTER_BOUND('',#27281,.T.) ;
#21419=FACE_OUTER_BOUND('',#27282,.T.) ;
#21420=FACE_OUTER_BOUND('',#27283,.T.) ;
#21421=FACE_OUTER_BOUND('',#27284,.T.) ;
#21422=FACE_OUTER_BOUND('',#27285,.T.) ;
#21423=FACE_OUTER_BOUND('',#27286,.T.) ;
#21424=FACE_OUTER_BOUND('',#27287,.T.) ;
#21425=FACE_OUTER_BOUND('',#27288,.T.) ;
#21426=FACE_OUTER_BOUND('',#27289,.T.) ;
#21427=FACE_OUTER_BOUND('',#27290,.T.) ;
#21428=FACE_OUTER_BOUND('',#27291,.T.) ;
#21429=FACE_OUTER_BOUND('',#27292,.T.) ;
#21430=FACE_OUTER_BOUND('',#27293,.T.) ;
#21431=FACE_OUTER_BOUND('',#27294,.T.) ;
#21432=FACE_OUTER_BOUND('',#27295,.T.) ;
#21433=FACE_OUTER_BOUND('',#27296,.T.) ;
#21434=FACE_OUTER_BOUND('',#27297,.T.) ;
#21435=FACE_OUTER_BOUND('',#27298,.T.) ;
#21436=FACE_OUTER_BOUND('',#27299,.T.) ;
#21437=FACE_OUTER_BOUND('',#27300,.T.) ;
#21438=FACE_OUTER_BOUND('',#27301,.T.) ;
#21439=FACE_OUTER_BOUND('',#27302,.T.) ;
#21440=FACE_OUTER_BOUND('',#27303,.T.) ;
#21441=FACE_OUTER_BOUND('',#27304,.T.) ;
#21442=FACE_OUTER_BOUND('',#27305,.T.) ;
#21443=FACE_OUTER_BOUND('',#27306,.T.) ;
#21444=FACE_OUTER_BOUND('',#27307,.T.) ;
#21445=FACE_OUTER_BOUND('',#27308,.T.) ;
#21446=FACE_OUTER_BOUND('',#27309,.T.) ;
#21447=FACE_OUTER_BOUND('',#27310,.T.) ;
#21448=FACE_OUTER_BOUND('',#27311,.T.) ;
#21449=FACE_OUTER_BOUND('',#27312,.T.) ;
#21450=FACE_OUTER_BOUND('',#27313,.T.) ;
#21451=FACE_OUTER_BOUND('',#27314,.T.) ;
#21452=FACE_OUTER_BOUND('',#27315,.T.) ;
#21453=FACE_OUTER_BOUND('',#27316,.T.) ;
#21454=FACE_OUTER_BOUND('',#27317,.T.) ;
#21455=FACE_OUTER_BOUND('',#27318,.T.) ;
#21456=FACE_OUTER_BOUND('',#27319,.T.) ;
#21457=FACE_OUTER_BOUND('',#27320,.T.) ;
#21458=FACE_OUTER_BOUND('',#27321,.T.) ;
#21459=FACE_OUTER_BOUND('',#27322,.T.) ;
#21460=FACE_OUTER_BOUND('',#27323,.T.) ;
#21461=FACE_OUTER_BOUND('',#27324,.T.) ;
#21462=FACE_OUTER_BOUND('',#27325,.T.) ;
#21463=FACE_OUTER_BOUND('',#27326,.T.) ;
#21464=FACE_OUTER_BOUND('',#27327,.T.) ;
#21465=FACE_OUTER_BOUND('',#27328,.T.) ;
#21466=FACE_OUTER_BOUND('',#27329,.T.) ;
#21467=FACE_OUTER_BOUND('',#27330,.T.) ;
#21468=FACE_OUTER_BOUND('',#27331,.T.) ;
#21469=FACE_OUTER_BOUND('',#27332,.T.) ;
#21470=FACE_OUTER_BOUND('',#27333,.T.) ;
#21471=FACE_OUTER_BOUND('',#27334,.T.) ;
#21472=FACE_OUTER_BOUND('',#27335,.T.) ;
#21473=FACE_OUTER_BOUND('',#27336,.T.) ;
#21474=FACE_OUTER_BOUND('',#27337,.T.) ;
#21475=FACE_OUTER_BOUND('',#27338,.T.) ;
#21476=FACE_OUTER_BOUND('',#27339,.T.) ;
#21477=FACE_OUTER_BOUND('',#27340,.T.) ;
#21478=FACE_OUTER_BOUND('',#27341,.T.) ;
#21479=FACE_OUTER_BOUND('',#27342,.T.) ;
#21480=FACE_OUTER_BOUND('',#27343,.T.) ;
#21481=FACE_OUTER_BOUND('',#27344,.T.) ;
#21482=FACE_OUTER_BOUND('',#27345,.T.) ;
#21483=FACE_OUTER_BOUND('',#27346,.T.) ;
#21484=FACE_OUTER_BOUND('',#27347,.T.) ;
#21485=FACE_OUTER_BOUND('',#27348,.T.) ;
#21486=FACE_OUTER_BOUND('',#27349,.T.) ;
#21487=FACE_OUTER_BOUND('',#27350,.T.) ;
#21488=FACE_OUTER_BOUND('',#27351,.T.) ;
#21489=FACE_OUTER_BOUND('',#27352,.T.) ;
#21490=FACE_OUTER_BOUND('',#27353,.T.) ;
#21491=FACE_OUTER_BOUND('',#27354,.T.) ;
#21492=FACE_OUTER_BOUND('',#27355,.T.) ;
#21493=FACE_OUTER_BOUND('',#27356,.T.) ;
#21494=FACE_OUTER_BOUND('',#27357,.T.) ;
#21495=FACE_OUTER_BOUND('',#27358,.T.) ;
#21496=FACE_OUTER_BOUND('',#27359,.T.) ;
#21497=FACE_OUTER_BOUND('',#27360,.T.) ;
#21498=FACE_OUTER_BOUND('',#27361,.T.) ;
#21499=FACE_OUTER_BOUND('',#27362,.T.) ;
#21500=FACE_OUTER_BOUND('',#27363,.T.) ;
#21501=FACE_OUTER_BOUND('',#27364,.T.) ;
#21502=FACE_OUTER_BOUND('',#27365,.T.) ;
#21503=FACE_OUTER_BOUND('',#27366,.T.) ;
#21504=FACE_OUTER_BOUND('',#27367,.T.) ;
#21505=FACE_OUTER_BOUND('',#27368,.T.) ;
#21506=FACE_OUTER_BOUND('',#27369,.T.) ;
#21507=FACE_OUTER_BOUND('',#27370,.T.) ;
#21508=FACE_OUTER_BOUND('',#27371,.T.) ;
#21509=FACE_OUTER_BOUND('',#27372,.T.) ;
#21510=FACE_OUTER_BOUND('',#27373,.T.) ;
#21511=FACE_OUTER_BOUND('',#27374,.T.) ;
#21512=FACE_OUTER_BOUND('',#27375,.T.) ;
#21513=FACE_OUTER_BOUND('',#27376,.T.) ;
#21514=FACE_OUTER_BOUND('',#27377,.T.) ;
#21515=FACE_OUTER_BOUND('',#27378,.T.) ;
#21516=FACE_OUTER_BOUND('',#27379,.T.) ;
#21517=FACE_OUTER_BOUND('',#27380,.T.) ;
#21518=FACE_OUTER_BOUND('',#27381,.T.) ;
#21519=FACE_OUTER_BOUND('',#27382,.T.) ;
#21520=FACE_OUTER_BOUND('',#27383,.T.) ;
#21521=FACE_OUTER_BOUND('',#27384,.T.) ;
#21522=FACE_OUTER_BOUND('',#27385,.T.) ;
#21523=FACE_OUTER_BOUND('',#27386,.T.) ;
#21524=FACE_OUTER_BOUND('',#27387,.T.) ;
#21525=FACE_OUTER_BOUND('',#27388,.T.) ;
#21526=FACE_OUTER_BOUND('',#27389,.T.) ;
#21527=FACE_OUTER_BOUND('',#27390,.T.) ;
#21528=FACE_OUTER_BOUND('',#27391,.T.) ;
#21529=FACE_OUTER_BOUND('',#27392,.T.) ;
#21530=FACE_OUTER_BOUND('',#27393,.T.) ;
#21531=FACE_OUTER_BOUND('',#27394,.T.) ;
#21532=FACE_OUTER_BOUND('',#27395,.T.) ;
#21533=FACE_OUTER_BOUND('',#27396,.T.) ;
#21534=FACE_OUTER_BOUND('',#27397,.T.) ;
#21535=FACE_OUTER_BOUND('',#27398,.T.) ;
#21536=FACE_OUTER_BOUND('',#27399,.T.) ;
#21537=FACE_OUTER_BOUND('',#27400,.T.) ;
#21538=FACE_OUTER_BOUND('',#27401,.T.) ;
#21539=FACE_OUTER_BOUND('',#27402,.T.) ;
#21540=FACE_OUTER_BOUND('',#27403,.T.) ;
#21541=FACE_OUTER_BOUND('',#27404,.T.) ;
#21542=FACE_OUTER_BOUND('',#27405,.T.) ;
#21543=FACE_OUTER_BOUND('',#27406,.T.) ;
#21544=FACE_OUTER_BOUND('',#27407,.T.) ;
#21545=FACE_OUTER_BOUND('',#27408,.T.) ;
#21546=FACE_OUTER_BOUND('',#27409,.T.) ;
#21547=FACE_OUTER_BOUND('',#27410,.T.) ;
#21548=FACE_OUTER_BOUND('',#27411,.T.) ;
#21549=FACE_OUTER_BOUND('',#27412,.T.) ;
#21550=FACE_OUTER_BOUND('',#27413,.T.) ;
#21551=FACE_OUTER_BOUND('',#27414,.T.) ;
#21552=FACE_OUTER_BOUND('',#27415,.T.) ;
#21553=FACE_OUTER_BOUND('',#27416,.T.) ;
#21554=FACE_OUTER_BOUND('',#27417,.T.) ;
#21555=FACE_OUTER_BOUND('',#27418,.T.) ;
#21556=FACE_OUTER_BOUND('',#27419,.T.) ;
#21557=FACE_OUTER_BOUND('',#27420,.T.) ;
#21558=FACE_OUTER_BOUND('',#27421,.T.) ;
#21559=FACE_OUTER_BOUND('',#27422,.T.) ;
#21560=FACE_OUTER_BOUND('',#27423,.T.) ;
#21561=FACE_OUTER_BOUND('',#27424,.T.) ;
#21562=FACE_OUTER_BOUND('',#27425,.T.) ;
#21563=FACE_OUTER_BOUND('',#27426,.T.) ;
#21564=FACE_OUTER_BOUND('',#27427,.T.) ;
#21565=FACE_OUTER_BOUND('',#27428,.T.) ;
#21566=FACE_OUTER_BOUND('',#27429,.T.) ;
#21567=FACE_OUTER_BOUND('',#27430,.T.) ;
#21568=FACE_OUTER_BOUND('',#27431,.T.) ;
#21569=FACE_OUTER_BOUND('',#27432,.T.) ;
#21570=FACE_OUTER_BOUND('',#27433,.T.) ;
#21571=FACE_OUTER_BOUND('',#27434,.T.) ;
#21572=FACE_OUTER_BOUND('',#27435,.T.) ;
#21573=FACE_OUTER_BOUND('',#27436,.T.) ;
#21574=FACE_OUTER_BOUND('',#27437,.T.) ;
#21575=FACE_OUTER_BOUND('',#27438,.T.) ;
#21576=FACE_OUTER_BOUND('',#27439,.T.) ;
#21577=FACE_OUTER_BOUND('',#27440,.T.) ;
#21578=FACE_OUTER_BOUND('',#27441,.T.) ;
#21579=FACE_OUTER_BOUND('',#27442,.T.) ;
#21580=FACE_OUTER_BOUND('',#27443,.T.) ;
#21581=FACE_OUTER_BOUND('',#27444,.T.) ;
#21582=FACE_OUTER_BOUND('',#27445,.T.) ;
#21583=FACE_OUTER_BOUND('',#27446,.T.) ;
#21584=FACE_OUTER_BOUND('',#27447,.T.) ;
#21585=FACE_OUTER_BOUND('',#27448,.T.) ;
#21586=FACE_OUTER_BOUND('',#27449,.T.) ;
#21587=FACE_OUTER_BOUND('',#27450,.T.) ;
#21588=FACE_OUTER_BOUND('',#27451,.T.) ;
#21589=FACE_OUTER_BOUND('',#27452,.T.) ;
#21590=FACE_OUTER_BOUND('',#27453,.T.) ;
#21591=FACE_OUTER_BOUND('',#27454,.T.) ;
#21592=FACE_OUTER_BOUND('',#27455,.T.) ;
#21593=FACE_OUTER_BOUND('',#27456,.T.) ;
#21594=FACE_OUTER_BOUND('',#27457,.T.) ;
#21595=FACE_OUTER_BOUND('',#27458,.T.) ;
#21596=FACE_OUTER_BOUND('',#27459,.T.) ;
#21597=FACE_OUTER_BOUND('',#27460,.T.) ;
#21598=FACE_OUTER_BOUND('',#27461,.T.) ;
#21599=FACE_OUTER_BOUND('',#27462,.T.) ;
#21600=FACE_OUTER_BOUND('',#27463,.T.) ;
#21601=FACE_OUTER_BOUND('',#27464,.T.) ;
#21602=FACE_OUTER_BOUND('',#27465,.T.) ;
#21603=FACE_OUTER_BOUND('',#27466,.T.) ;
#21604=FACE_OUTER_BOUND('',#27467,.T.) ;
#21605=FACE_OUTER_BOUND('',#27468,.T.) ;
#21606=FACE_OUTER_BOUND('',#27469,.T.) ;
#21607=FACE_OUTER_BOUND('',#27470,.T.) ;
#21608=FACE_OUTER_BOUND('',#27471,.T.) ;
#21609=FACE_OUTER_BOUND('',#27472,.T.) ;
#21610=FACE_OUTER_BOUND('',#27473,.T.) ;
#21611=FACE_OUTER_BOUND('',#27474,.T.) ;
#21612=FACE_OUTER_BOUND('',#27475,.T.) ;
#21613=FACE_OUTER_BOUND('',#27476,.T.) ;
#21614=FACE_OUTER_BOUND('',#27477,.T.) ;
#21615=FACE_OUTER_BOUND('',#27478,.T.) ;
#21616=FACE_OUTER_BOUND('',#27479,.T.) ;
#21617=FACE_OUTER_BOUND('',#27480,.T.) ;
#21618=FACE_OUTER_BOUND('',#27481,.T.) ;
#21619=FACE_OUTER_BOUND('',#27482,.T.) ;
#21620=FACE_OUTER_BOUND('',#27483,.T.) ;
#21621=FACE_OUTER_BOUND('',#27484,.T.) ;
#21622=FACE_OUTER_BOUND('',#27485,.T.) ;
#21623=FACE_OUTER_BOUND('',#27486,.T.) ;
#21624=FACE_OUTER_BOUND('',#27487,.T.) ;
#21625=FACE_OUTER_BOUND('',#27488,.T.) ;
#21626=FACE_OUTER_BOUND('',#27489,.T.) ;
#21627=FACE_OUTER_BOUND('',#27490,.T.) ;
#21628=FACE_OUTER_BOUND('',#27491,.T.) ;
#21629=FACE_OUTER_BOUND('',#27492,.T.) ;
#21630=FACE_OUTER_BOUND('',#27493,.T.) ;
#21631=FACE_OUTER_BOUND('',#27494,.T.) ;
#21632=FACE_OUTER_BOUND('',#27495,.T.) ;
#21633=FACE_OUTER_BOUND('',#27496,.T.) ;
#21634=FACE_OUTER_BOUND('',#27497,.T.) ;
#21635=FACE_OUTER_BOUND('',#27498,.T.) ;
#21636=FACE_OUTER_BOUND('',#27499,.T.) ;
#21637=FACE_OUTER_BOUND('',#27500,.T.) ;
#21638=FACE_OUTER_BOUND('',#27501,.T.) ;
#21639=FACE_OUTER_BOUND('',#27502,.T.) ;
#21640=FACE_OUTER_BOUND('',#27503,.T.) ;
#21641=FACE_OUTER_BOUND('',#27504,.T.) ;
#21642=FACE_OUTER_BOUND('',#27505,.T.) ;
#21643=FACE_OUTER_BOUND('',#27506,.T.) ;
#21644=FACE_OUTER_BOUND('',#27507,.T.) ;
#21645=FACE_OUTER_BOUND('',#27508,.T.) ;
#21646=FACE_OUTER_BOUND('',#27509,.T.) ;
#21647=FACE_OUTER_BOUND('',#27510,.T.) ;
#21648=FACE_OUTER_BOUND('',#27511,.T.) ;
#21649=FACE_OUTER_BOUND('',#27512,.T.) ;
#21650=FACE_OUTER_BOUND('',#27513,.T.) ;
#21651=FACE_OUTER_BOUND('',#27514,.T.) ;
#21652=FACE_OUTER_BOUND('',#27515,.T.) ;
#21653=FACE_OUTER_BOUND('',#27516,.T.) ;
#21654=FACE_OUTER_BOUND('',#27517,.T.) ;
#21655=FACE_OUTER_BOUND('',#27518,.T.) ;
#21656=FACE_OUTER_BOUND('',#27519,.T.) ;
#21657=FACE_OUTER_BOUND('',#27520,.T.) ;
#21658=FACE_OUTER_BOUND('',#27521,.T.) ;
#21659=FACE_OUTER_BOUND('',#27522,.T.) ;
#21660=FACE_OUTER_BOUND('',#27523,.T.) ;
#21661=FACE_OUTER_BOUND('',#27524,.T.) ;
#21662=FACE_OUTER_BOUND('',#27525,.T.) ;
#21663=FACE_OUTER_BOUND('',#27526,.T.) ;
#21664=FACE_OUTER_BOUND('',#27527,.T.) ;
#21665=FACE_OUTER_BOUND('',#27528,.T.) ;
#21666=FACE_OUTER_BOUND('',#27529,.T.) ;
#21667=FACE_OUTER_BOUND('',#27530,.T.) ;
#21668=FACE_OUTER_BOUND('',#27531,.T.) ;
#21669=FACE_OUTER_BOUND('',#27532,.T.) ;
#21670=FACE_OUTER_BOUND('',#27533,.T.) ;
#21671=FACE_OUTER_BOUND('',#27534,.T.) ;
#21672=FACE_OUTER_BOUND('',#27535,.T.) ;
#21673=FACE_OUTER_BOUND('',#27536,.T.) ;
#21674=FACE_OUTER_BOUND('',#27537,.T.) ;
#21675=FACE_OUTER_BOUND('',#27538,.T.) ;
#21676=FACE_OUTER_BOUND('',#27539,.T.) ;
#21677=FACE_OUTER_BOUND('',#27540,.T.) ;
#21678=FACE_OUTER_BOUND('',#27541,.T.) ;
#21679=FACE_OUTER_BOUND('',#27542,.T.) ;
#21680=FACE_OUTER_BOUND('',#27543,.T.) ;
#21681=FACE_OUTER_BOUND('',#27544,.T.) ;
#21682=FACE_OUTER_BOUND('',#27545,.T.) ;
#21683=FACE_OUTER_BOUND('',#27546,.T.) ;
#21684=FACE_OUTER_BOUND('',#27547,.T.) ;
#21685=FACE_OUTER_BOUND('',#27548,.T.) ;
#21686=FACE_OUTER_BOUND('',#27549,.T.) ;
#21687=FACE_OUTER_BOUND('',#27550,.T.) ;
#21688=FACE_OUTER_BOUND('',#27551,.T.) ;
#21689=FACE_OUTER_BOUND('',#27552,.T.) ;
#21690=FACE_OUTER_BOUND('',#27553,.T.) ;
#21691=FACE_OUTER_BOUND('',#27554,.T.) ;
#21692=FACE_OUTER_BOUND('',#27555,.T.) ;
#21693=FACE_OUTER_BOUND('',#27556,.T.) ;
#21694=FACE_OUTER_BOUND('',#27557,.T.) ;
#21695=FACE_OUTER_BOUND('',#27558,.T.) ;
#21696=FACE_OUTER_BOUND('',#27559,.T.) ;
#21697=FACE_OUTER_BOUND('',#27560,.T.) ;
#21698=FACE_OUTER_BOUND('',#27561,.T.) ;
#21699=FACE_OUTER_BOUND('',#27562,.T.) ;
#21700=FACE_OUTER_BOUND('',#27563,.T.) ;
#21701=FACE_OUTER_BOUND('',#27564,.T.) ;
#21702=FACE_OUTER_BOUND('',#27565,.T.) ;
#21703=FACE_OUTER_BOUND('',#27566,.T.) ;
#21704=FACE_OUTER_BOUND('',#27567,.T.) ;
#21705=FACE_OUTER_BOUND('',#27568,.T.) ;
#21706=FACE_OUTER_BOUND('',#27569,.T.) ;
#21707=FACE_OUTER_BOUND('',#27570,.T.) ;
#21708=FACE_OUTER_BOUND('',#27571,.T.) ;
#21709=FACE_OUTER_BOUND('',#27572,.T.) ;
#21710=FACE_OUTER_BOUND('',#27573,.T.) ;
#21711=FACE_OUTER_BOUND('',#27574,.T.) ;
#21712=FACE_OUTER_BOUND('',#27575,.T.) ;
#21713=FACE_OUTER_BOUND('',#27576,.T.) ;
#21714=FACE_OUTER_BOUND('',#27577,.T.) ;
#21715=FACE_OUTER_BOUND('',#27578,.T.) ;
#21716=FACE_OUTER_BOUND('',#27579,.T.) ;
#21717=FACE_OUTER_BOUND('',#27580,.T.) ;
#21718=FACE_OUTER_BOUND('',#27581,.T.) ;
#21719=FACE_OUTER_BOUND('',#27582,.T.) ;
#21720=FACE_OUTER_BOUND('',#27583,.T.) ;
#21721=FACE_OUTER_BOUND('',#27584,.T.) ;
#21722=FACE_OUTER_BOUND('',#27585,.T.) ;
#21723=FACE_OUTER_BOUND('',#27586,.T.) ;
#21724=FACE_OUTER_BOUND('',#27587,.T.) ;
#21725=FACE_OUTER_BOUND('',#27588,.T.) ;
#21726=FACE_OUTER_BOUND('',#27589,.T.) ;
#21727=FACE_OUTER_BOUND('',#27590,.T.) ;
#21728=FACE_OUTER_BOUND('',#27591,.T.) ;
#21729=FACE_OUTER_BOUND('',#27592,.T.) ;
#21730=FACE_OUTER_BOUND('',#27593,.T.) ;
#21731=FACE_OUTER_BOUND('',#27594,.T.) ;
#21732=FACE_OUTER_BOUND('',#27595,.T.) ;
#21733=FACE_OUTER_BOUND('',#27596,.T.) ;
#21734=FACE_OUTER_BOUND('',#27597,.T.) ;
#21735=FACE_OUTER_BOUND('',#27598,.T.) ;
#21736=FACE_OUTER_BOUND('',#27599,.T.) ;
#21737=FACE_OUTER_BOUND('',#27600,.T.) ;
#21738=FACE_OUTER_BOUND('',#27601,.T.) ;
#21739=FACE_OUTER_BOUND('',#27602,.T.) ;
#21740=FACE_OUTER_BOUND('',#27603,.T.) ;
#21741=FACE_OUTER_BOUND('',#27604,.T.) ;
#21742=FACE_OUTER_BOUND('',#27605,.T.) ;
#21743=FACE_OUTER_BOUND('',#27606,.T.) ;
#21744=FACE_OUTER_BOUND('',#27607,.T.) ;
#21745=FACE_OUTER_BOUND('',#27608,.T.) ;
#21746=FACE_OUTER_BOUND('',#27609,.T.) ;
#21747=FACE_OUTER_BOUND('',#27610,.T.) ;
#21748=FACE_OUTER_BOUND('',#27611,.T.) ;
#21749=FACE_OUTER_BOUND('',#27612,.T.) ;
#21750=FACE_OUTER_BOUND('',#27613,.T.) ;
#21751=FACE_OUTER_BOUND('',#27614,.T.) ;
#21752=FACE_OUTER_BOUND('',#27615,.T.) ;
#21753=FACE_OUTER_BOUND('',#27616,.T.) ;
#21754=FACE_OUTER_BOUND('',#27617,.T.) ;
#21755=FACE_OUTER_BOUND('',#27618,.T.) ;
#21756=FACE_OUTER_BOUND('',#27619,.T.) ;
#21757=FACE_OUTER_BOUND('',#27620,.T.) ;
#21758=FACE_OUTER_BOUND('',#27621,.T.) ;
#21759=FACE_OUTER_BOUND('',#27622,.T.) ;
#21760=FACE_OUTER_BOUND('',#27623,.T.) ;
#21761=FACE_OUTER_BOUND('',#27624,.T.) ;
#21762=FACE_OUTER_BOUND('',#27625,.T.) ;
#21763=FACE_OUTER_BOUND('',#27626,.T.) ;
#21764=FACE_OUTER_BOUND('',#27627,.T.) ;
#21765=FACE_OUTER_BOUND('',#27628,.T.) ;
#21766=FACE_OUTER_BOUND('',#27629,.T.) ;
#21767=FACE_OUTER_BOUND('',#27630,.T.) ;
#21768=FACE_OUTER_BOUND('',#27631,.T.) ;
#21769=FACE_OUTER_BOUND('',#27632,.T.) ;
#21770=FACE_OUTER_BOUND('',#27633,.T.) ;
#21771=FACE_OUTER_BOUND('',#27634,.T.) ;
#21772=FACE_OUTER_BOUND('',#27635,.T.) ;
#21773=FACE_OUTER_BOUND('',#27636,.T.) ;
#21774=FACE_OUTER_BOUND('',#27637,.T.) ;
#21775=FACE_OUTER_BOUND('',#27638,.T.) ;
#21776=FACE_OUTER_BOUND('',#27639,.T.) ;
#21777=FACE_OUTER_BOUND('',#27640,.T.) ;
#21778=FACE_OUTER_BOUND('',#27641,.T.) ;
#21779=FACE_OUTER_BOUND('',#27642,.T.) ;
#21780=FACE_OUTER_BOUND('',#27643,.T.) ;
#21781=FACE_OUTER_BOUND('',#27644,.T.) ;
#21782=FACE_OUTER_BOUND('',#27645,.T.) ;
#21783=FACE_OUTER_BOUND('',#27646,.T.) ;
#21784=FACE_OUTER_BOUND('',#27647,.T.) ;
#21785=FACE_OUTER_BOUND('',#27648,.T.) ;
#21786=FACE_OUTER_BOUND('',#27649,.T.) ;
#21787=FACE_OUTER_BOUND('',#27650,.T.) ;
#21788=FACE_OUTER_BOUND('',#27651,.T.) ;
#21789=FACE_OUTER_BOUND('',#27652,.T.) ;
#21790=FACE_OUTER_BOUND('',#27653,.T.) ;
#21791=FACE_OUTER_BOUND('',#27654,.T.) ;
#21792=FACE_OUTER_BOUND('',#27655,.T.) ;
#21793=FACE_OUTER_BOUND('',#27656,.T.) ;
#21794=FACE_OUTER_BOUND('',#27657,.T.) ;
#21795=FACE_OUTER_BOUND('',#27658,.T.) ;
#21796=FACE_OUTER_BOUND('',#27659,.T.) ;
#21797=FACE_OUTER_BOUND('',#27660,.T.) ;
#21798=FACE_OUTER_BOUND('',#27661,.T.) ;
#21799=FACE_OUTER_BOUND('',#27662,.T.) ;
#21800=FACE_OUTER_BOUND('',#27663,.T.) ;
#21801=FACE_OUTER_BOUND('',#27664,.T.) ;
#21802=FACE_OUTER_BOUND('',#27665,.T.) ;
#21803=FACE_OUTER_BOUND('',#27666,.T.) ;
#21804=FACE_OUTER_BOUND('',#27667,.T.) ;
#21805=FACE_OUTER_BOUND('',#27668,.T.) ;
#21806=FACE_OUTER_BOUND('',#27669,.T.) ;
#21807=FACE_OUTER_BOUND('',#27670,.T.) ;
#21808=FACE_OUTER_BOUND('',#27671,.T.) ;
#21809=FACE_OUTER_BOUND('',#27672,.T.) ;
#21810=FACE_OUTER_BOUND('',#27673,.T.) ;
#21811=FACE_OUTER_BOUND('',#27674,.T.) ;
#21812=FACE_OUTER_BOUND('',#27675,.T.) ;
#21813=FACE_OUTER_BOUND('',#27676,.T.) ;
#21814=FACE_OUTER_BOUND('',#27677,.T.) ;
#21815=FACE_OUTER_BOUND('',#27678,.T.) ;
#21816=FACE_OUTER_BOUND('',#27679,.T.) ;
#21817=FACE_OUTER_BOUND('',#27680,.T.) ;
#21818=FACE_OUTER_BOUND('',#27681,.T.) ;
#21819=FACE_OUTER_BOUND('',#27682,.T.) ;
#21820=FACE_OUTER_BOUND('',#27683,.T.) ;
#21821=FACE_OUTER_BOUND('',#27684,.T.) ;
#21822=FACE_OUTER_BOUND('',#27685,.T.) ;
#21823=FACE_OUTER_BOUND('',#27686,.T.) ;
#21824=FACE_OUTER_BOUND('',#27687,.T.) ;
#21825=FACE_OUTER_BOUND('',#27688,.T.) ;
#21826=FACE_OUTER_BOUND('',#27689,.T.) ;
#21827=FACE_OUTER_BOUND('',#27690,.T.) ;
#21828=FACE_OUTER_BOUND('',#27691,.T.) ;
#21829=FACE_OUTER_BOUND('',#27692,.T.) ;
#21830=FACE_OUTER_BOUND('',#27693,.T.) ;
#21831=FACE_OUTER_BOUND('',#27694,.T.) ;
#21832=FACE_OUTER_BOUND('',#27695,.T.) ;
#21833=FACE_OUTER_BOUND('',#27696,.T.) ;
#21834=FACE_OUTER_BOUND('',#27697,.T.) ;
#21835=FACE_OUTER_BOUND('',#27698,.T.) ;
#21836=FACE_OUTER_BOUND('',#27699,.T.) ;
#21837=FACE_OUTER_BOUND('',#27700,.T.) ;
#21838=FACE_OUTER_BOUND('',#27701,.T.) ;
#21839=FACE_OUTER_BOUND('',#27702,.T.) ;
#21840=FACE_OUTER_BOUND('',#27703,.T.) ;
#21841=FACE_OUTER_BOUND('',#27704,.T.) ;
#21842=FACE_OUTER_BOUND('',#27705,.T.) ;
#21843=FACE_OUTER_BOUND('',#27706,.T.) ;
#21844=FACE_OUTER_BOUND('',#27707,.T.) ;
#21845=FACE_OUTER_BOUND('',#27708,.T.) ;
#21846=FACE_OUTER_BOUND('',#27709,.T.) ;
#21847=FACE_OUTER_BOUND('',#27710,.T.) ;
#21848=FACE_OUTER_BOUND('',#27711,.T.) ;
#21849=FACE_OUTER_BOUND('',#27712,.T.) ;
#21850=FACE_OUTER_BOUND('',#27713,.T.) ;
#21851=FACE_OUTER_BOUND('',#27714,.T.) ;
#21852=FACE_OUTER_BOUND('',#27715,.T.) ;
#21853=FACE_OUTER_BOUND('',#27716,.T.) ;
#21854=FACE_OUTER_BOUND('',#27717,.T.) ;
#21855=FACE_OUTER_BOUND('',#27718,.T.) ;
#21856=FACE_OUTER_BOUND('',#27719,.T.) ;
#21857=FACE_OUTER_BOUND('',#27720,.T.) ;
#21858=FACE_OUTER_BOUND('',#27721,.T.) ;
#21859=FACE_OUTER_BOUND('',#27722,.T.) ;
#21860=FACE_OUTER_BOUND('',#27723,.T.) ;
#21861=FACE_OUTER_BOUND('',#27724,.T.) ;
#21862=FACE_OUTER_BOUND('',#27725,.T.) ;
#21863=FACE_OUTER_BOUND('',#27726,.T.) ;
#21864=FACE_OUTER_BOUND('',#27727,.T.) ;
#21865=FACE_OUTER_BOUND('',#27728,.T.) ;
#21866=FACE_OUTER_BOUND('',#27729,.T.) ;
#21867=FACE_OUTER_BOUND('',#27730,.T.) ;
#21868=FACE_OUTER_BOUND('',#27731,.T.) ;
#21869=FACE_OUTER_BOUND('',#27732,.T.) ;
#21870=FACE_OUTER_BOUND('',#27733,.T.) ;
#21871=FACE_OUTER_BOUND('',#27734,.T.) ;
#21872=FACE_OUTER_BOUND('',#27735,.T.) ;
#21873=FACE_OUTER_BOUND('',#27736,.T.) ;
#21874=FACE_OUTER_BOUND('',#27737,.T.) ;
#21875=FACE_OUTER_BOUND('',#27738,.T.) ;
#21876=FACE_OUTER_BOUND('',#27739,.T.) ;
#21877=FACE_OUTER_BOUND('',#27740,.T.) ;
#21878=FACE_OUTER_BOUND('',#27741,.T.) ;
#21879=FACE_OUTER_BOUND('',#27742,.T.) ;
#21880=FACE_OUTER_BOUND('',#27743,.T.) ;
#21881=FACE_OUTER_BOUND('',#27744,.T.) ;
#21882=FACE_OUTER_BOUND('',#27745,.T.) ;
#21883=FACE_OUTER_BOUND('',#27746,.T.) ;
#21884=FACE_OUTER_BOUND('',#27747,.T.) ;
#21885=FACE_OUTER_BOUND('',#27748,.T.) ;
#21886=FACE_OUTER_BOUND('',#27749,.T.) ;
#21887=FACE_OUTER_BOUND('',#27750,.T.) ;
#21888=FACE_OUTER_BOUND('',#27751,.T.) ;
#21889=FACE_OUTER_BOUND('',#27752,.T.) ;
#21890=FACE_OUTER_BOUND('',#27753,.T.) ;
#21891=FACE_OUTER_BOUND('',#27754,.T.) ;
#21892=FACE_OUTER_BOUND('',#27755,.T.) ;
#21893=FACE_OUTER_BOUND('',#27756,.T.) ;
#21894=FACE_OUTER_BOUND('',#27757,.T.) ;
#21895=FACE_OUTER_BOUND('',#27758,.T.) ;
#21896=FACE_OUTER_BOUND('',#27759,.T.) ;
#21897=FACE_OUTER_BOUND('',#27760,.T.) ;
#21898=FACE_OUTER_BOUND('',#27761,.T.) ;
#21899=FACE_OUTER_BOUND('',#27762,.T.) ;
#21900=FACE_OUTER_BOUND('',#27763,.T.) ;
#21901=FACE_OUTER_BOUND('',#27764,.T.) ;
#21902=FACE_OUTER_BOUND('',#27765,.T.) ;
#21903=FACE_OUTER_BOUND('',#27766,.T.) ;
#21904=FACE_OUTER_BOUND('',#27767,.T.) ;
#21905=FACE_OUTER_BOUND('',#27768,.T.) ;
#21906=FACE_OUTER_BOUND('',#27769,.T.) ;
#21907=FACE_OUTER_BOUND('',#27770,.T.) ;
#21908=FACE_OUTER_BOUND('',#27771,.T.) ;
#21909=FACE_OUTER_BOUND('',#27772,.T.) ;
#21910=FACE_OUTER_BOUND('',#27773,.T.) ;
#21911=FACE_OUTER_BOUND('',#27774,.T.) ;
#21912=FACE_OUTER_BOUND('',#27775,.T.) ;
#21913=FACE_OUTER_BOUND('',#27776,.T.) ;
#21914=FACE_OUTER_BOUND('',#27777,.T.) ;
#21915=FACE_OUTER_BOUND('',#27778,.T.) ;
#21916=FACE_OUTER_BOUND('',#27779,.T.) ;
#21917=FACE_OUTER_BOUND('',#27780,.T.) ;
#21918=FACE_OUTER_BOUND('',#27781,.T.) ;
#21919=FACE_OUTER_BOUND('',#27782,.T.) ;
#21920=FACE_OUTER_BOUND('',#27783,.T.) ;
#21921=FACE_OUTER_BOUND('',#27784,.T.) ;
#21922=FACE_OUTER_BOUND('',#27785,.T.) ;
#21923=FACE_OUTER_BOUND('',#27786,.T.) ;
#21924=FACE_OUTER_BOUND('',#27787,.T.) ;
#21925=FACE_OUTER_BOUND('',#27788,.T.) ;
#21926=FACE_OUTER_BOUND('',#27789,.T.) ;
#21927=FACE_OUTER_BOUND('',#27790,.T.) ;
#21928=FACE_OUTER_BOUND('',#27791,.T.) ;
#21929=FACE_OUTER_BOUND('',#27792,.T.) ;
#21930=FACE_OUTER_BOUND('',#27793,.T.) ;
#21931=FACE_OUTER_BOUND('',#27794,.T.) ;
#21932=FACE_OUTER_BOUND('',#27795,.T.) ;
#21933=FACE_OUTER_BOUND('',#27796,.T.) ;
#21934=FACE_OUTER_BOUND('',#27797,.T.) ;
#21935=FACE_OUTER_BOUND('',#27798,.T.) ;
#21936=FACE_OUTER_BOUND('',#27799,.T.) ;
#21937=FACE_OUTER_BOUND('',#27800,.T.) ;
#21938=FACE_OUTER_BOUND('',#27801,.T.) ;
#21939=FACE_OUTER_BOUND('',#27802,.T.) ;
#21940=FACE_OUTER_BOUND('',#27803,.T.) ;
#21941=FACE_OUTER_BOUND('',#27804,.T.) ;
#21942=FACE_OUTER_BOUND('',#27805,.T.) ;
#21943=FACE_OUTER_BOUND('',#27806,.T.) ;
#21944=FACE_OUTER_BOUND('',#27807,.T.) ;
#21945=FACE_OUTER_BOUND('',#27808,.T.) ;
#21946=FACE_OUTER_BOUND('',#27809,.T.) ;
#21947=FACE_OUTER_BOUND('',#27810,.T.) ;
#21948=FACE_OUTER_BOUND('',#27811,.T.) ;
#21949=FACE_OUTER_BOUND('',#27812,.T.) ;
#21950=FACE_OUTER_BOUND('',#27813,.T.) ;
#21951=FACE_OUTER_BOUND('',#27814,.T.) ;
#21952=FACE_OUTER_BOUND('',#27815,.T.) ;
#21953=FACE_OUTER_BOUND('',#27816,.T.) ;
#21954=FACE_OUTER_BOUND('',#27817,.T.) ;
#21955=FACE_OUTER_BOUND('',#27818,.T.) ;
#21956=FACE_OUTER_BOUND('',#27819,.T.) ;
#21957=FACE_OUTER_BOUND('',#27820,.T.) ;
#21958=FACE_OUTER_BOUND('',#27821,.T.) ;
#21959=FACE_OUTER_BOUND('',#27822,.T.) ;
#21960=FACE_OUTER_BOUND('',#27823,.T.) ;
#21961=FACE_OUTER_BOUND('',#27824,.T.) ;
#21962=FACE_OUTER_BOUND('',#27825,.T.) ;
#21963=FACE_OUTER_BOUND('',#27826,.T.) ;
#21964=FACE_OUTER_BOUND('',#27827,.T.) ;
#21965=FACE_OUTER_BOUND('',#27828,.T.) ;
#21966=FACE_OUTER_BOUND('',#27829,.T.) ;
#21967=FACE_OUTER_BOUND('',#27830,.T.) ;
#21968=FACE_OUTER_BOUND('',#27831,.T.) ;
#21969=FACE_OUTER_BOUND('',#27832,.T.) ;
#21970=FACE_OUTER_BOUND('',#27833,.T.) ;
#21971=FACE_OUTER_BOUND('',#27834,.T.) ;
#21972=FACE_OUTER_BOUND('',#27835,.T.) ;
#21973=FACE_OUTER_BOUND('',#27836,.T.) ;
#21974=FACE_OUTER_BOUND('',#27837,.T.) ;
#21975=FACE_OUTER_BOUND('',#27838,.T.) ;
#21976=FACE_OUTER_BOUND('',#27839,.T.) ;
#21977=FACE_OUTER_BOUND('',#27840,.T.) ;
#21978=FACE_OUTER_BOUND('',#27841,.T.) ;
#21979=FACE_OUTER_BOUND('',#27842,.T.) ;
#21980=FACE_OUTER_BOUND('',#27843,.T.) ;
#21981=FACE_OUTER_BOUND('',#27844,.T.) ;
#21982=FACE_OUTER_BOUND('',#27845,.T.) ;
#21983=FACE_OUTER_BOUND('',#27846,.T.) ;
#21984=FACE_OUTER_BOUND('',#27847,.T.) ;
#21985=FACE_OUTER_BOUND('',#27848,.T.) ;
#21986=FACE_OUTER_BOUND('',#27849,.T.) ;
#21987=FACE_OUTER_BOUND('',#27850,.T.) ;
#21988=FACE_OUTER_BOUND('',#27851,.T.) ;
#21989=FACE_OUTER_BOUND('',#27852,.T.) ;
#21990=FACE_OUTER_BOUND('',#27853,.T.) ;
#21991=FACE_OUTER_BOUND('',#27854,.T.) ;
#21992=FACE_OUTER_BOUND('',#27855,.T.) ;
#21993=FACE_OUTER_BOUND('',#27856,.T.) ;
#21994=FACE_OUTER_BOUND('',#27857,.T.) ;
#21995=FACE_OUTER_BOUND('',#27858,.T.) ;
#21996=FACE_OUTER_BOUND('',#27859,.T.) ;
#21997=FACE_OUTER_BOUND('',#27860,.T.) ;
#21998=FACE_OUTER_BOUND('',#27861,.T.) ;
#21999=FACE_OUTER_BOUND('',#27862,.T.) ;
#22000=FACE_OUTER_BOUND('',#27863,.T.) ;
#22001=FACE_OUTER_BOUND('',#27864,.T.) ;
#22002=FACE_OUTER_BOUND('',#27865,.T.) ;
#22003=FACE_OUTER_BOUND('',#27866,.T.) ;
#22004=FACE_OUTER_BOUND('',#27867,.T.) ;
#22005=FACE_OUTER_BOUND('',#27868,.T.) ;
#22006=FACE_OUTER_BOUND('',#27869,.T.) ;
#22007=FACE_OUTER_BOUND('',#27870,.T.) ;
#22008=FACE_OUTER_BOUND('',#27871,.T.) ;
#22009=FACE_OUTER_BOUND('',#27872,.T.) ;
#22010=FACE_OUTER_BOUND('',#27873,.T.) ;
#22011=FACE_OUTER_BOUND('',#27874,.T.) ;
#22012=FACE_OUTER_BOUND('',#27875,.T.) ;
#22013=FACE_OUTER_BOUND('',#27876,.T.) ;
#22014=FACE_OUTER_BOUND('',#27877,.T.) ;
#22015=FACE_OUTER_BOUND('',#27878,.T.) ;
#22016=FACE_OUTER_BOUND('',#27879,.T.) ;
#22017=FACE_OUTER_BOUND('',#27880,.T.) ;
#22018=FACE_OUTER_BOUND('',#27881,.T.) ;
#22019=FACE_OUTER_BOUND('',#27882,.T.) ;
#22020=FACE_OUTER_BOUND('',#27883,.T.) ;
#22021=FACE_OUTER_BOUND('',#27884,.T.) ;
#22022=FACE_OUTER_BOUND('',#27885,.T.) ;
#22023=FACE_OUTER_BOUND('',#27886,.T.) ;
#22024=FACE_OUTER_BOUND('',#27887,.T.) ;
#22025=FACE_OUTER_BOUND('',#27888,.T.) ;
#22026=FACE_OUTER_BOUND('',#27889,.T.) ;
#22027=FACE_OUTER_BOUND('',#27890,.T.) ;
#22028=FACE_OUTER_BOUND('',#27891,.T.) ;
#22029=FACE_OUTER_BOUND('',#27892,.T.) ;
#22030=FACE_OUTER_BOUND('',#27893,.T.) ;
#22031=FACE_OUTER_BOUND('',#27894,.T.) ;
#22032=FACE_OUTER_BOUND('',#27895,.T.) ;
#22033=FACE_OUTER_BOUND('',#27896,.T.) ;
#22034=FACE_OUTER_BOUND('',#27897,.T.) ;
#22035=FACE_OUTER_BOUND('',#27898,.T.) ;
#22036=FACE_OUTER_BOUND('',#27899,.T.) ;
#22037=FACE_OUTER_BOUND('',#27900,.T.) ;
#22038=FACE_OUTER_BOUND('',#27901,.T.) ;
#22039=FACE_OUTER_BOUND('',#27902,.T.) ;
#22040=FACE_OUTER_BOUND('',#27903,.T.) ;
#22041=FACE_OUTER_BOUND('',#27904,.T.) ;
#22042=FACE_OUTER_BOUND('',#27905,.T.) ;
#22043=FACE_OUTER_BOUND('',#27906,.T.) ;
#22044=FACE_OUTER_BOUND('',#27907,.T.) ;
#22045=FACE_OUTER_BOUND('',#27908,.T.) ;
#22046=FACE_OUTER_BOUND('',#27909,.T.) ;
#22047=FACE_OUTER_BOUND('',#27910,.T.) ;
#22048=FACE_OUTER_BOUND('',#27911,.T.) ;
#22049=FACE_OUTER_BOUND('',#27912,.T.) ;
#22050=FACE_OUTER_BOUND('',#27913,.T.) ;
#22051=FACE_OUTER_BOUND('',#27914,.T.) ;
#22052=FACE_OUTER_BOUND('',#27915,.T.) ;
#22053=FACE_OUTER_BOUND('',#27916,.T.) ;
#22054=FACE_OUTER_BOUND('',#27917,.T.) ;
#22055=FACE_OUTER_BOUND('',#27918,.T.) ;
#22056=FACE_OUTER_BOUND('',#27919,.T.) ;
#22057=FACE_OUTER_BOUND('',#27920,.T.) ;
#22058=FACE_OUTER_BOUND('',#27921,.T.) ;
#22059=FACE_OUTER_BOUND('',#27922,.T.) ;
#22060=FACE_OUTER_BOUND('',#27923,.T.) ;
#22061=FACE_OUTER_BOUND('',#27924,.T.) ;
#22062=FACE_OUTER_BOUND('',#27925,.T.) ;
#22063=FACE_OUTER_BOUND('',#27926,.T.) ;
#22064=FACE_OUTER_BOUND('',#27927,.T.) ;
#22065=FACE_OUTER_BOUND('',#27928,.T.) ;
#22066=FACE_OUTER_BOUND('',#27929,.T.) ;
#22067=FACE_OUTER_BOUND('',#27930,.T.) ;
#22068=FACE_OUTER_BOUND('',#27931,.T.) ;
#22069=FACE_OUTER_BOUND('',#27932,.T.) ;
#22070=FACE_OUTER_BOUND('',#27933,.T.) ;
#22071=FACE_OUTER_BOUND('',#27934,.T.) ;
#22072=FACE_OUTER_BOUND('',#27935,.T.) ;
#22073=FACE_OUTER_BOUND('',#27936,.T.) ;
#22074=FACE_OUTER_BOUND('',#27937,.T.) ;
#22075=FACE_OUTER_BOUND('',#27938,.T.) ;
#22076=FACE_OUTER_BOUND('',#27939,.T.) ;
#22077=FACE_OUTER_BOUND('',#27940,.T.) ;
#22078=FACE_OUTER_BOUND('',#27941,.T.) ;
#22079=FACE_OUTER_BOUND('',#27942,.T.) ;
#22080=FACE_OUTER_BOUND('',#27943,.T.) ;
#22081=FACE_OUTER_BOUND('',#27944,.T.) ;
#22082=FACE_OUTER_BOUND('',#27945,.T.) ;
#22083=FACE_OUTER_BOUND('',#27946,.T.) ;
#22084=FACE_OUTER_BOUND('',#27947,.T.) ;
#22085=FACE_OUTER_BOUND('',#27948,.T.) ;
#22086=FACE_OUTER_BOUND('',#27949,.T.) ;
#22087=FACE_OUTER_BOUND('',#27950,.T.) ;
#22088=FACE_OUTER_BOUND('',#27951,.T.) ;
#22089=FACE_OUTER_BOUND('',#27952,.T.) ;
#22090=FACE_OUTER_BOUND('',#27953,.T.) ;
#22091=FACE_OUTER_BOUND('',#27954,.T.) ;
#22092=FACE_OUTER_BOUND('',#27955,.T.) ;
#22093=FACE_OUTER_BOUND('',#27956,.T.) ;
#22094=FACE_OUTER_BOUND('',#27957,.T.) ;
#22095=FACE_OUTER_BOUND('',#27958,.T.) ;
#22096=FACE_OUTER_BOUND('',#27959,.T.) ;
#22097=FACE_OUTER_BOUND('',#27960,.T.) ;
#22098=FACE_OUTER_BOUND('',#27961,.T.) ;
#22099=FACE_OUTER_BOUND('',#27962,.T.) ;
#22100=FACE_OUTER_BOUND('',#27963,.T.) ;
#22101=FACE_OUTER_BOUND('',#27964,.T.) ;
#22102=FACE_OUTER_BOUND('',#27965,.T.) ;
#22103=FACE_OUTER_BOUND('',#27966,.T.) ;
#22104=FACE_OUTER_BOUND('',#27967,.T.) ;
#22105=FACE_OUTER_BOUND('',#27968,.T.) ;
#22106=FACE_OUTER_BOUND('',#27969,.T.) ;
#22107=FACE_OUTER_BOUND('',#27970,.T.) ;
#22108=FACE_OUTER_BOUND('',#27971,.T.) ;
#22109=FACE_OUTER_BOUND('',#27972,.T.) ;
#22110=FACE_OUTER_BOUND('',#27973,.T.) ;
#22111=FACE_OUTER_BOUND('',#27974,.T.) ;
#22112=FACE_OUTER_BOUND('',#27975,.T.) ;
#22113=FACE_OUTER_BOUND('',#27976,.T.) ;
#22114=FACE_OUTER_BOUND('',#27977,.T.) ;
#22115=FACE_OUTER_BOUND('',#27978,.T.) ;
#22116=FACE_OUTER_BOUND('',#27979,.T.) ;
#22117=FACE_OUTER_BOUND('',#27980,.T.) ;
#22118=FACE_OUTER_BOUND('',#27981,.T.) ;
#22119=FACE_OUTER_BOUND('',#27982,.T.) ;
#22120=FACE_OUTER_BOUND('',#27983,.T.) ;
#22121=FACE_OUTER_BOUND('',#27984,.T.) ;
#22122=FACE_OUTER_BOUND('',#27985,.T.) ;
#22123=FACE_OUTER_BOUND('',#27986,.T.) ;
#22124=FACE_OUTER_BOUND('',#27987,.T.) ;
#22125=FACE_OUTER_BOUND('',#27988,.T.) ;
#22126=FACE_OUTER_BOUND('',#27989,.T.) ;
#22127=FACE_OUTER_BOUND('',#27990,.T.) ;
#22128=FACE_OUTER_BOUND('',#27991,.T.) ;
#22129=FACE_OUTER_BOUND('',#27992,.T.) ;
#22130=FACE_OUTER_BOUND('',#27993,.T.) ;
#22131=FACE_OUTER_BOUND('',#27994,.T.) ;
#22132=FACE_OUTER_BOUND('',#27995,.T.) ;
#22133=FACE_OUTER_BOUND('',#27996,.T.) ;
#22134=FACE_OUTER_BOUND('',#27997,.T.) ;
#22135=FACE_OUTER_BOUND('',#27998,.T.) ;
#22136=FACE_OUTER_BOUND('',#27999,.T.) ;
#22137=FACE_OUTER_BOUND('',#28000,.T.) ;
#22138=FACE_OUTER_BOUND('',#28001,.T.) ;
#22139=FACE_OUTER_BOUND('',#28002,.T.) ;
#22140=FACE_OUTER_BOUND('',#28003,.T.) ;
#22141=FACE_OUTER_BOUND('',#28004,.T.) ;
#22142=FACE_OUTER_BOUND('',#28005,.T.) ;
#22143=FACE_OUTER_BOUND('',#28006,.T.) ;
#22144=FACE_OUTER_BOUND('',#28007,.T.) ;
#22145=FACE_OUTER_BOUND('',#28008,.T.) ;
#22146=FACE_OUTER_BOUND('',#28009,.T.) ;
#22147=FACE_OUTER_BOUND('',#28010,.T.) ;
#22148=FACE_OUTER_BOUND('',#28011,.T.) ;
#22149=FACE_OUTER_BOUND('',#28012,.T.) ;
#22150=FACE_OUTER_BOUND('',#28013,.T.) ;
#22151=FACE_OUTER_BOUND('',#28014,.T.) ;
#22152=FACE_OUTER_BOUND('',#28015,.T.) ;
#22153=FACE_OUTER_BOUND('',#28016,.T.) ;
#22154=FACE_OUTER_BOUND('',#28017,.T.) ;
#22155=FACE_OUTER_BOUND('',#28018,.T.) ;
#22156=FACE_OUTER_BOUND('',#28019,.T.) ;
#22157=FACE_OUTER_BOUND('',#28020,.T.) ;
#22158=FACE_OUTER_BOUND('',#28021,.T.) ;
#22159=FACE_OUTER_BOUND('',#28022,.T.) ;
#22160=FACE_OUTER_BOUND('',#28023,.T.) ;
#22161=FACE_OUTER_BOUND('',#28024,.T.) ;
#22162=FACE_OUTER_BOUND('',#28025,.T.) ;
#22163=FACE_OUTER_BOUND('',#28026,.T.) ;
#22164=FACE_OUTER_BOUND('',#28027,.T.) ;
#22165=FACE_OUTER_BOUND('',#28028,.T.) ;
#22166=FACE_OUTER_BOUND('',#28029,.T.) ;
#22167=FACE_OUTER_BOUND('',#28030,.T.) ;
#22168=FACE_OUTER_BOUND('',#28031,.T.) ;
#22169=FACE_OUTER_BOUND('',#28032,.T.) ;
#22170=FACE_OUTER_BOUND('',#28033,.T.) ;
#22171=FACE_OUTER_BOUND('',#28034,.T.) ;
#22172=FACE_OUTER_BOUND('',#28035,.T.) ;
#22173=FACE_OUTER_BOUND('',#28036,.T.) ;
#22174=FACE_OUTER_BOUND('',#28037,.T.) ;
#22175=FACE_OUTER_BOUND('',#28038,.T.) ;
#22176=FACE_OUTER_BOUND('',#28039,.T.) ;
#22177=FACE_OUTER_BOUND('',#28040,.T.) ;
#22178=FACE_OUTER_BOUND('',#28041,.T.) ;
#22179=FACE_OUTER_BOUND('',#28042,.T.) ;
#22180=FACE_OUTER_BOUND('',#28043,.T.) ;
#22181=FACE_OUTER_BOUND('',#28044,.T.) ;
#22182=FACE_OUTER_BOUND('',#28045,.T.) ;
#22183=FACE_OUTER_BOUND('',#28046,.T.) ;
#22184=FACE_OUTER_BOUND('',#28047,.T.) ;
#22185=FACE_OUTER_BOUND('',#28048,.T.) ;
#22186=FACE_OUTER_BOUND('',#28049,.T.) ;
#22187=FACE_OUTER_BOUND('',#28050,.T.) ;
#22188=FACE_OUTER_BOUND('',#28051,.T.) ;
#22189=FACE_OUTER_BOUND('',#28052,.T.) ;
#22190=FACE_OUTER_BOUND('',#28053,.T.) ;
#22191=FACE_OUTER_BOUND('',#28054,.T.) ;
#22192=FACE_OUTER_BOUND('',#28055,.T.) ;
#22193=FACE_OUTER_BOUND('',#28056,.T.) ;
#22194=FACE_OUTER_BOUND('',#28057,.T.) ;
#22195=FACE_OUTER_BOUND('',#28058,.T.) ;
#22196=FACE_OUTER_BOUND('',#28059,.T.) ;
#22197=FACE_OUTER_BOUND('',#28060,.T.) ;
#22198=FACE_OUTER_BOUND('',#28061,.T.) ;
#22199=FACE_OUTER_BOUND('',#28062,.T.) ;
#22200=FACE_OUTER_BOUND('',#28063,.T.) ;
#22201=FACE_OUTER_BOUND('',#28064,.T.) ;
#22202=FACE_OUTER_BOUND('',#28065,.T.) ;
#22203=FACE_OUTER_BOUND('',#28066,.T.) ;
#22204=FACE_OUTER_BOUND('',#28067,.T.) ;
#22205=FACE_OUTER_BOUND('',#28068,.T.) ;
#22206=FACE_OUTER_BOUND('',#28069,.T.) ;
#22207=FACE_OUTER_BOUND('',#28070,.T.) ;
#22208=FACE_OUTER_BOUND('',#28071,.T.) ;
#22209=FACE_OUTER_BOUND('',#28072,.T.) ;
#22210=FACE_OUTER_BOUND('',#28073,.T.) ;
#22211=FACE_OUTER_BOUND('',#28074,.T.) ;
#22212=FACE_OUTER_BOUND('',#28075,.T.) ;
#22213=FACE_OUTER_BOUND('',#28076,.T.) ;
#22214=FACE_OUTER_BOUND('',#28077,.T.) ;
#22215=FACE_OUTER_BOUND('',#28078,.T.) ;
#22216=FACE_OUTER_BOUND('',#28079,.T.) ;
#22217=FACE_OUTER_BOUND('',#28080,.T.) ;
#22218=FACE_OUTER_BOUND('',#28081,.T.) ;
#22219=FACE_OUTER_BOUND('',#28082,.T.) ;
#22220=FACE_OUTER_BOUND('',#28083,.T.) ;
#22221=FACE_OUTER_BOUND('',#28084,.T.) ;
#22222=FACE_OUTER_BOUND('',#28085,.T.) ;
#22223=FACE_OUTER_BOUND('',#28086,.T.) ;
#22224=FACE_OUTER_BOUND('',#28087,.T.) ;
#22225=FACE_OUTER_BOUND('',#28088,.T.) ;
#22226=FACE_OUTER_BOUND('',#28089,.T.) ;
#22227=FACE_OUTER_BOUND('',#28090,.T.) ;
#22228=FACE_OUTER_BOUND('',#28091,.T.) ;
#22229=FACE_OUTER_BOUND('',#28092,.T.) ;
#22230=FACE_OUTER_BOUND('',#28093,.T.) ;
#22231=FACE_OUTER_BOUND('',#28094,.T.) ;
#22232=FACE_OUTER_BOUND('',#28095,.T.) ;
#22233=FACE_OUTER_BOUND('',#28096,.T.) ;
#22234=FACE_OUTER_BOUND('',#28097,.T.) ;
#22235=FACE_OUTER_BOUND('',#28098,.T.) ;
#22236=FACE_OUTER_BOUND('',#28099,.T.) ;
#22237=FACE_OUTER_BOUND('',#28100,.T.) ;
#22238=FACE_OUTER_BOUND('',#28101,.T.) ;
#22239=FACE_OUTER_BOUND('',#28102,.T.) ;
#22240=FACE_OUTER_BOUND('',#28103,.T.) ;
#22241=FACE_OUTER_BOUND('',#28104,.T.) ;
#22242=FACE_OUTER_BOUND('',#28105,.T.) ;
#22243=FACE_OUTER_BOUND('',#28106,.T.) ;
#22244=FACE_OUTER_BOUND('',#28107,.T.) ;
#22245=FACE_OUTER_BOUND('',#28108,.T.) ;
#22246=FACE_OUTER_BOUND('',#28109,.T.) ;
#22247=FACE_OUTER_BOUND('',#28110,.T.) ;
#22248=FACE_OUTER_BOUND('',#28111,.T.) ;
#22249=FACE_OUTER_BOUND('',#28112,.T.) ;
#22250=FACE_OUTER_BOUND('',#28113,.T.) ;
#22251=FACE_OUTER_BOUND('',#28114,.T.) ;
#22252=FACE_OUTER_BOUND('',#28115,.T.) ;
#22253=FACE_OUTER_BOUND('',#28116,.T.) ;
#22254=FACE_OUTER_BOUND('',#28117,.T.) ;
#22255=FACE_OUTER_BOUND('',#28118,.T.) ;
#22256=FACE_OUTER_BOUND('',#28119,.T.) ;
#22257=FACE_OUTER_BOUND('',#28120,.T.) ;
#22258=FACE_OUTER_BOUND('',#28121,.T.) ;
#22259=FACE_OUTER_BOUND('',#28122,.T.) ;
#22260=FACE_OUTER_BOUND('',#28123,.T.) ;
#22261=FACE_OUTER_BOUND('',#28124,.T.) ;
#22262=FACE_OUTER_BOUND('',#28125,.T.) ;
#22263=FACE_OUTER_BOUND('',#28126,.T.) ;
#22264=FACE_OUTER_BOUND('',#28127,.T.) ;
#22265=FACE_OUTER_BOUND('',#28128,.T.) ;
#22266=FACE_OUTER_BOUND('',#28129,.T.) ;
#22267=FACE_OUTER_BOUND('',#28130,.T.) ;
#22268=FACE_OUTER_BOUND('',#28131,.T.) ;
#22269=FACE_OUTER_BOUND('',#28132,.T.) ;
#22270=FACE_OUTER_BOUND('',#28133,.T.) ;
#22271=FACE_OUTER_BOUND('',#28134,.T.) ;
#22272=FACE_OUTER_BOUND('',#28135,.T.) ;
#22273=FACE_OUTER_BOUND('',#28136,.T.) ;
#22274=FACE_OUTER_BOUND('',#28137,.T.) ;
#22275=FACE_OUTER_BOUND('',#28138,.T.) ;
#22276=FACE_OUTER_BOUND('',#28139,.T.) ;
#22277=FACE_OUTER_BOUND('',#28140,.T.) ;
#22278=FACE_OUTER_BOUND('',#28141,.T.) ;
#22279=FACE_OUTER_BOUND('',#28142,.T.) ;
#22280=FACE_OUTER_BOUND('',#28143,.T.) ;
#22281=FACE_OUTER_BOUND('',#28144,.T.) ;
#22282=FACE_OUTER_BOUND('',#28145,.T.) ;
#22283=FACE_OUTER_BOUND('',#28146,.T.) ;
#22284=FACE_OUTER_BOUND('',#28147,.T.) ;
#22285=FACE_OUTER_BOUND('',#28148,.T.) ;
#22286=FACE_OUTER_BOUND('',#28149,.T.) ;
#22287=FACE_OUTER_BOUND('',#28150,.T.) ;
#22288=FACE_OUTER_BOUND('',#28151,.T.) ;
#22289=FACE_OUTER_BOUND('',#28152,.T.) ;
#22290=FACE_OUTER_BOUND('',#28153,.T.) ;
#22291=FACE_OUTER_BOUND('',#28154,.T.) ;
#22292=FACE_OUTER_BOUND('',#28155,.T.) ;
#22293=FACE_OUTER_BOUND('',#28156,.T.) ;
#22294=FACE_OUTER_BOUND('',#28157,.T.) ;
#22295=FACE_OUTER_BOUND('',#28158,.T.) ;
#22296=FACE_OUTER_BOUND('',#28159,.T.) ;
#22297=FACE_OUTER_BOUND('',#28160,.T.) ;
#22298=FACE_OUTER_BOUND('',#28161,.T.) ;
#22299=FACE_OUTER_BOUND('',#28162,.T.) ;
#22300=FACE_OUTER_BOUND('',#28163,.T.) ;
#22301=FACE_OUTER_BOUND('',#28164,.T.) ;
#22302=FACE_OUTER_BOUND('',#28165,.T.) ;
#22303=FACE_OUTER_BOUND('',#28166,.T.) ;
#22304=FACE_OUTER_BOUND('',#28167,.T.) ;
#22305=FACE_OUTER_BOUND('',#28168,.T.) ;
#22306=FACE_OUTER_BOUND('',#28169,.T.) ;
#22307=FACE_OUTER_BOUND('',#28170,.T.) ;
#22308=FACE_OUTER_BOUND('',#28171,.T.) ;
#22309=FACE_OUTER_BOUND('',#28172,.T.) ;
#22310=FACE_OUTER_BOUND('',#28173,.T.) ;
#22311=FACE_OUTER_BOUND('',#28174,.T.) ;
#22312=FACE_OUTER_BOUND('',#28175,.T.) ;
#22313=FACE_OUTER_BOUND('',#28176,.T.) ;
#22314=FACE_OUTER_BOUND('',#28177,.T.) ;
#22315=FACE_OUTER_BOUND('',#28178,.T.) ;
#22316=FACE_OUTER_BOUND('',#28179,.T.) ;
#22317=FACE_OUTER_BOUND('',#28180,.T.) ;
#22318=FACE_OUTER_BOUND('',#28181,.T.) ;
#22319=FACE_OUTER_BOUND('',#28182,.T.) ;
#22320=FACE_OUTER_BOUND('',#28183,.T.) ;
#22321=FACE_OUTER_BOUND('',#28184,.T.) ;
#22322=FACE_OUTER_BOUND('',#28185,.T.) ;
#22323=FACE_OUTER_BOUND('',#28186,.T.) ;
#22324=FACE_OUTER_BOUND('',#28187,.T.) ;
#22325=FACE_OUTER_BOUND('',#28188,.T.) ;
#22326=FACE_OUTER_BOUND('',#28189,.T.) ;
#22327=FACE_OUTER_BOUND('',#28190,.T.) ;
#22328=FACE_OUTER_BOUND('',#28191,.T.) ;
#22329=FACE_OUTER_BOUND('',#28192,.T.) ;
#22330=FACE_OUTER_BOUND('',#28193,.T.) ;
#22331=FACE_OUTER_BOUND('',#28194,.T.) ;
#22332=FACE_OUTER_BOUND('',#28195,.T.) ;
#22333=FACE_OUTER_BOUND('',#28196,.T.) ;
#22334=FACE_OUTER_BOUND('',#28197,.T.) ;
#22335=FACE_OUTER_BOUND('',#28198,.T.) ;
#22336=FACE_OUTER_BOUND('',#28199,.T.) ;
#22337=FACE_OUTER_BOUND('',#28200,.T.) ;
#22338=FACE_OUTER_BOUND('',#28201,.T.) ;
#22339=FACE_OUTER_BOUND('',#28202,.T.) ;
#22340=FACE_OUTER_BOUND('',#28203,.T.) ;
#22341=FACE_OUTER_BOUND('',#28204,.T.) ;
#22342=FACE_OUTER_BOUND('',#28205,.T.) ;
#22343=FACE_OUTER_BOUND('',#28206,.T.) ;
#22344=FACE_OUTER_BOUND('',#28207,.T.) ;
#22345=FACE_OUTER_BOUND('',#28208,.T.) ;
#22346=FACE_OUTER_BOUND('',#28209,.T.) ;
#22347=FACE_OUTER_BOUND('',#28210,.T.) ;
#22348=FACE_OUTER_BOUND('',#28211,.T.) ;
#22349=FACE_OUTER_BOUND('',#28212,.T.) ;
#22350=FACE_OUTER_BOUND('',#28213,.T.) ;
#22351=FACE_OUTER_BOUND('',#28214,.T.) ;
#22352=FACE_OUTER_BOUND('',#28215,.T.) ;
#22353=FACE_OUTER_BOUND('',#28216,.T.) ;
#22354=FACE_OUTER_BOUND('',#28217,.T.) ;
#22355=FACE_OUTER_BOUND('',#28218,.T.) ;
#22356=FACE_OUTER_BOUND('',#28219,.T.) ;
#22357=FACE_OUTER_BOUND('',#28220,.T.) ;
#22358=FACE_OUTER_BOUND('',#28221,.T.) ;
#22359=FACE_OUTER_BOUND('',#28222,.T.) ;
#22360=FACE_OUTER_BOUND('',#28223,.T.) ;
#22361=FACE_OUTER_BOUND('',#28224,.T.) ;
#22362=FACE_OUTER_BOUND('',#28225,.T.) ;
#22363=FACE_OUTER_BOUND('',#28226,.T.) ;
#22364=FACE_OUTER_BOUND('',#28227,.T.) ;
#22365=FACE_OUTER_BOUND('',#28228,.T.) ;
#22366=FACE_OUTER_BOUND('',#28229,.T.) ;
#22367=FACE_OUTER_BOUND('',#28230,.T.) ;
#22368=FACE_OUTER_BOUND('',#28231,.T.) ;
#22369=FACE_OUTER_BOUND('',#28232,.T.) ;
#22370=FACE_OUTER_BOUND('',#28233,.T.) ;
#22371=FACE_OUTER_BOUND('',#28234,.T.) ;
#22372=FACE_OUTER_BOUND('',#28235,.T.) ;
#22373=FACE_OUTER_BOUND('',#28236,.T.) ;
#22374=FACE_OUTER_BOUND('',#28237,.T.) ;
#22375=FACE_OUTER_BOUND('',#28238,.T.) ;
#22376=FACE_OUTER_BOUND('',#28239,.T.) ;
#22377=FACE_OUTER_BOUND('',#28240,.T.) ;
#22378=FACE_OUTER_BOUND('',#28241,.T.) ;
#22379=FACE_OUTER_BOUND('',#28242,.T.) ;
#22380=FACE_OUTER_BOUND('',#28243,.T.) ;
#22381=FACE_OUTER_BOUND('',#28244,.T.) ;
#22382=FACE_OUTER_BOUND('',#28245,.T.) ;
#22383=FACE_OUTER_BOUND('',#28246,.T.) ;
#22384=FACE_OUTER_BOUND('',#28247,.T.) ;
#22385=FACE_OUTER_BOUND('',#28248,.T.) ;
#22386=FACE_OUTER_BOUND('',#28249,.T.) ;
#22387=FACE_OUTER_BOUND('',#28250,.T.) ;
#22388=FACE_OUTER_BOUND('',#28251,.T.) ;
#22389=FACE_OUTER_BOUND('',#28252,.T.) ;
#22390=FACE_OUTER_BOUND('',#28253,.T.) ;
#22391=FACE_OUTER_BOUND('',#28254,.T.) ;
#22392=FACE_OUTER_BOUND('',#28255,.T.) ;
#22393=FACE_OUTER_BOUND('',#28256,.T.) ;
#22394=FACE_OUTER_BOUND('',#28257,.T.) ;
#22395=FACE_OUTER_BOUND('',#28258,.T.) ;
#22396=FACE_OUTER_BOUND('',#28259,.T.) ;
#22397=FACE_OUTER_BOUND('',#28260,.T.) ;
#22398=FACE_OUTER_BOUND('',#28261,.T.) ;
#22399=FACE_OUTER_BOUND('',#28262,.T.) ;
#22400=FACE_OUTER_BOUND('',#28263,.T.) ;
#22401=FACE_OUTER_BOUND('',#28264,.T.) ;
#22402=FACE_OUTER_BOUND('',#28265,.T.) ;
#22403=FACE_OUTER_BOUND('',#28266,.T.) ;
#22404=FACE_OUTER_BOUND('',#28267,.T.) ;
#22405=FACE_OUTER_BOUND('',#28268,.T.) ;
#22406=FACE_OUTER_BOUND('',#28269,.T.) ;
#22407=FACE_OUTER_BOUND('',#28270,.T.) ;
#22408=FACE_OUTER_BOUND('',#28271,.T.) ;
#22409=FACE_OUTER_BOUND('',#28272,.T.) ;
#22410=FACE_OUTER_BOUND('',#28273,.T.) ;
#22411=FACE_OUTER_BOUND('',#28274,.T.) ;
#22412=FACE_OUTER_BOUND('',#28275,.T.) ;
#22413=FACE_OUTER_BOUND('',#28276,.T.) ;
#22414=FACE_OUTER_BOUND('',#28277,.T.) ;
#22415=FACE_OUTER_BOUND('',#28278,.T.) ;
#22416=FACE_OUTER_BOUND('',#28279,.T.) ;
#22417=FACE_OUTER_BOUND('',#28280,.T.) ;
#22418=FACE_OUTER_BOUND('',#28281,.T.) ;
#22419=FACE_OUTER_BOUND('',#28282,.T.) ;
#22420=FACE_OUTER_BOUND('',#28283,.T.) ;
#22421=FACE_OUTER_BOUND('',#28284,.T.) ;
#22422=FACE_OUTER_BOUND('',#28285,.T.) ;
#22423=FACE_OUTER_BOUND('',#28286,.T.) ;
#22424=FACE_OUTER_BOUND('',#28287,.T.) ;
#22425=FACE_OUTER_BOUND('',#28288,.T.) ;
#22426=FACE_OUTER_BOUND('',#28289,.T.) ;
#22427=FACE_OUTER_BOUND('',#28290,.T.) ;
#22428=FACE_OUTER_BOUND('',#28291,.T.) ;
#22429=FACE_OUTER_BOUND('',#28292,.T.) ;
#22430=FACE_OUTER_BOUND('',#28293,.T.) ;
#22431=FACE_OUTER_BOUND('',#28294,.T.) ;
#22432=FACE_OUTER_BOUND('',#28295,.T.) ;
#22433=FACE_OUTER_BOUND('',#28296,.T.) ;
#22434=FACE_OUTER_BOUND('',#28297,.T.) ;
#22435=FACE_OUTER_BOUND('',#28298,.T.) ;
#22436=FACE_OUTER_BOUND('',#28299,.T.) ;
#22437=FACE_OUTER_BOUND('',#28300,.T.) ;
#22438=FACE_OUTER_BOUND('',#28301,.T.) ;
#22439=FACE_OUTER_BOUND('',#28302,.T.) ;
#22440=FACE_OUTER_BOUND('',#28303,.T.) ;
#22441=FACE_OUTER_BOUND('',#28304,.T.) ;
#22442=FACE_OUTER_BOUND('',#28305,.T.) ;
#22443=FACE_OUTER_BOUND('',#28306,.T.) ;
#22444=FACE_OUTER_BOUND('',#28307,.T.) ;
#22445=FACE_OUTER_BOUND('',#28308,.T.) ;
#22446=FACE_OUTER_BOUND('',#28309,.T.) ;
#22447=FACE_OUTER_BOUND('',#28310,.T.) ;
#22448=FACE_OUTER_BOUND('',#28311,.T.) ;
#22449=FACE_OUTER_BOUND('',#28312,.T.) ;
#22450=FACE_OUTER_BOUND('',#28313,.T.) ;
#22451=FACE_OUTER_BOUND('',#28314,.T.) ;
#22452=FACE_OUTER_BOUND('',#28315,.T.) ;
#22453=FACE_OUTER_BOUND('',#28316,.T.) ;
#22454=FACE_OUTER_BOUND('',#28317,.T.) ;
#22455=FACE_OUTER_BOUND('',#28318,.T.) ;
#22456=FACE_OUTER_BOUND('',#28319,.T.) ;
#22457=FACE_OUTER_BOUND('',#28320,.T.) ;
#22458=FACE_OUTER_BOUND('',#28321,.T.) ;
#22459=FACE_OUTER_BOUND('',#28322,.T.) ;
#22460=FACE_OUTER_BOUND('',#28323,.T.) ;
#22461=FACE_OUTER_BOUND('',#28324,.T.) ;
#22462=FACE_OUTER_BOUND('',#28325,.T.) ;
#22463=FACE_OUTER_BOUND('',#28326,.T.) ;
#22464=FACE_OUTER_BOUND('',#28327,.T.) ;
#22465=FACE_OUTER_BOUND('',#28328,.T.) ;
#22466=FACE_OUTER_BOUND('',#28329,.T.) ;
#22467=FACE_OUTER_BOUND('',#28330,.T.) ;
#22468=FACE_OUTER_BOUND('',#28331,.T.) ;
#22469=FACE_OUTER_BOUND('',#28332,.T.) ;
#22470=FACE_OUTER_BOUND('',#28333,.T.) ;
#22471=FACE_OUTER_BOUND('',#28334,.T.) ;
#22472=FACE_OUTER_BOUND('',#28335,.T.) ;
#22473=FACE_OUTER_BOUND('',#28336,.T.) ;
#22474=FACE_OUTER_BOUND('',#28337,.T.) ;
#22475=FACE_OUTER_BOUND('',#28338,.T.) ;
#22476=FACE_OUTER_BOUND('',#28339,.T.) ;
#22477=FACE_OUTER_BOUND('',#28340,.T.) ;
#22478=FACE_OUTER_BOUND('',#28341,.T.) ;
#22479=FACE_OUTER_BOUND('',#28342,.T.) ;
#22480=FACE_OUTER_BOUND('',#28343,.T.) ;
#22481=FACE_OUTER_BOUND('',#28344,.T.) ;
#22482=FACE_OUTER_BOUND('',#28345,.T.) ;
#22483=FACE_OUTER_BOUND('',#28346,.T.) ;
#22484=FACE_OUTER_BOUND('',#28347,.T.) ;
#22485=FACE_OUTER_BOUND('',#28348,.T.) ;
#22486=FACE_OUTER_BOUND('',#28349,.T.) ;
#22487=FACE_OUTER_BOUND('',#28350,.T.) ;
#22488=FACE_OUTER_BOUND('',#28351,.T.) ;
#22489=FACE_OUTER_BOUND('',#28352,.T.) ;
#22490=FACE_OUTER_BOUND('',#28353,.T.) ;
#22491=FACE_OUTER_BOUND('',#28354,.T.) ;
#22492=FACE_OUTER_BOUND('',#28355,.T.) ;
#22493=FACE_OUTER_BOUND('',#28356,.T.) ;
#22494=FACE_OUTER_BOUND('',#28357,.T.) ;
#22495=FACE_OUTER_BOUND('',#28358,.T.) ;
#22496=FACE_OUTER_BOUND('',#28359,.T.) ;
#22497=FACE_OUTER_BOUND('',#28360,.T.) ;
#22498=FACE_OUTER_BOUND('',#28361,.T.) ;
#22499=FACE_OUTER_BOUND('',#28362,.T.) ;
#22500=FACE_OUTER_BOUND('',#28363,.T.) ;
#22501=FACE_OUTER_BOUND('',#28364,.T.) ;
#22502=FACE_OUTER_BOUND('',#28365,.T.) ;
#22503=FACE_OUTER_BOUND('',#28366,.T.) ;
#22504=FACE_OUTER_BOUND('',#28367,.T.) ;
#22505=FACE_OUTER_BOUND('',#28368,.T.) ;
#22506=FACE_OUTER_BOUND('',#28369,.T.) ;
#22507=FACE_OUTER_BOUND('',#28370,.T.) ;
#22508=FACE_OUTER_BOUND('',#28371,.T.) ;
#22509=FACE_OUTER_BOUND('',#28372,.T.) ;
#22510=FACE_OUTER_BOUND('',#28373,.T.) ;
#22511=FACE_OUTER_BOUND('',#28374,.T.) ;
#22512=FACE_OUTER_BOUND('',#28375,.T.) ;
#22513=FACE_OUTER_BOUND('',#28376,.T.) ;
#22514=FACE_OUTER_BOUND('',#28377,.T.) ;
#22515=FACE_OUTER_BOUND('',#28378,.T.) ;
#22516=FACE_OUTER_BOUND('',#28379,.T.) ;
#22517=FACE_OUTER_BOUND('',#28380,.T.) ;
#22518=FACE_OUTER_BOUND('',#28381,.T.) ;
#22519=FACE_OUTER_BOUND('',#28382,.T.) ;
#22520=FACE_OUTER_BOUND('',#28383,.T.) ;
#22521=FACE_OUTER_BOUND('',#28384,.T.) ;
#22522=FACE_OUTER_BOUND('',#28385,.T.) ;
#22523=FACE_OUTER_BOUND('',#28386,.T.) ;
#22524=FACE_OUTER_BOUND('',#28387,.T.) ;
#22525=FACE_OUTER_BOUND('',#28388,.T.) ;
#22526=FACE_OUTER_BOUND('',#28389,.T.) ;
#22527=FACE_OUTER_BOUND('',#28390,.T.) ;
#22528=FACE_OUTER_BOUND('',#28391,.T.) ;
#22529=FACE_OUTER_BOUND('',#28392,.T.) ;
#22530=FACE_OUTER_BOUND('',#28393,.T.) ;
#22531=FACE_OUTER_BOUND('',#28394,.T.) ;
#22532=FACE_OUTER_BOUND('',#28395,.T.) ;
#22533=FACE_OUTER_BOUND('',#28396,.T.) ;
#22534=FACE_OUTER_BOUND('',#28397,.T.) ;
#22535=FACE_OUTER_BOUND('',#28398,.T.) ;
#22536=FACE_OUTER_BOUND('',#28399,.T.) ;
#22537=FACE_OUTER_BOUND('',#28400,.T.) ;
#22538=FACE_OUTER_BOUND('',#28401,.T.) ;
#22539=FACE_OUTER_BOUND('',#28402,.T.) ;
#22540=FACE_OUTER_BOUND('',#28403,.T.) ;
#22541=FACE_OUTER_BOUND('',#28404,.T.) ;
#22542=FACE_OUTER_BOUND('',#28405,.T.) ;
#22543=FACE_OUTER_BOUND('',#28406,.T.) ;
#22544=FACE_OUTER_BOUND('',#28407,.T.) ;
#22545=FACE_OUTER_BOUND('',#28408,.T.) ;
#22546=FACE_OUTER_BOUND('',#28409,.T.) ;
#22547=FACE_OUTER_BOUND('',#28410,.T.) ;
#22548=FACE_OUTER_BOUND('',#28411,.T.) ;
#22549=FACE_OUTER_BOUND('',#28412,.T.) ;
#22550=FACE_OUTER_BOUND('',#28413,.T.) ;
#22551=FACE_OUTER_BOUND('',#28414,.T.) ;
#22552=FACE_OUTER_BOUND('',#28415,.T.) ;
#22553=FACE_OUTER_BOUND('',#28416,.T.) ;
#22554=FACE_OUTER_BOUND('',#28417,.T.) ;
#22555=FACE_OUTER_BOUND('',#28418,.T.) ;
#22556=FACE_OUTER_BOUND('',#28419,.T.) ;
#22557=FACE_OUTER_BOUND('',#28420,.T.) ;
#22558=FACE_OUTER_BOUND('',#28421,.T.) ;
#22559=FACE_OUTER_BOUND('',#28422,.T.) ;
#22560=FACE_OUTER_BOUND('',#28423,.T.) ;
#22561=FACE_OUTER_BOUND('',#28424,.T.) ;
#22562=FACE_OUTER_BOUND('',#28425,.T.) ;
#22563=FACE_OUTER_BOUND('',#28426,.T.) ;
#22564=FACE_OUTER_BOUND('',#28427,.T.) ;
#22565=FACE_OUTER_BOUND('',#28428,.T.) ;
#22566=FACE_OUTER_BOUND('',#28429,.T.) ;
#22567=FACE_OUTER_BOUND('',#28430,.T.) ;
#22568=FACE_OUTER_BOUND('',#28431,.T.) ;
#22569=FACE_OUTER_BOUND('',#28432,.T.) ;
#22570=FACE_OUTER_BOUND('',#28433,.T.) ;
#22571=FACE_OUTER_BOUND('',#28434,.T.) ;
#22572=FACE_OUTER_BOUND('',#28435,.T.) ;
#22573=FACE_OUTER_BOUND('',#28436,.T.) ;
#22574=FACE_OUTER_BOUND('',#28437,.T.) ;
#22575=FACE_OUTER_BOUND('',#28438,.T.) ;
#22576=FACE_OUTER_BOUND('',#28439,.T.) ;
#22577=FACE_OUTER_BOUND('',#28440,.T.) ;
#22578=FACE_OUTER_BOUND('',#28441,.T.) ;
#22579=FACE_OUTER_BOUND('',#28442,.T.) ;
#22580=FACE_OUTER_BOUND('',#28443,.T.) ;
#22581=FACE_OUTER_BOUND('',#28444,.T.) ;
#22582=FACE_OUTER_BOUND('',#28445,.T.) ;
#22583=FACE_OUTER_BOUND('',#28446,.T.) ;
#22584=FACE_OUTER_BOUND('',#28447,.T.) ;
#22585=FACE_OUTER_BOUND('',#28448,.T.) ;
#22586=FACE_OUTER_BOUND('',#28449,.T.) ;
#22587=FACE_OUTER_BOUND('',#28450,.T.) ;
#22588=FACE_OUTER_BOUND('',#28451,.T.) ;
#22589=FACE_OUTER_BOUND('',#28452,.T.) ;
#22590=FACE_OUTER_BOUND('',#28453,.T.) ;
#22591=FACE_OUTER_BOUND('',#28454,.T.) ;
#22592=FACE_OUTER_BOUND('',#28455,.T.) ;
#22593=FACE_OUTER_BOUND('',#28456,.T.) ;
#22594=FACE_OUTER_BOUND('',#28457,.T.) ;
#22595=FACE_OUTER_BOUND('',#28458,.T.) ;
#22596=FACE_OUTER_BOUND('',#28459,.T.) ;
#22597=FACE_OUTER_BOUND('',#28460,.T.) ;
#22598=FACE_OUTER_BOUND('',#28461,.T.) ;
#22599=FACE_OUTER_BOUND('',#28462,.T.) ;
#22600=FACE_OUTER_BOUND('',#28463,.T.) ;
#22601=FACE_OUTER_BOUND('',#28464,.T.) ;
#22602=FACE_OUTER_BOUND('',#28465,.T.) ;
#22603=FACE_OUTER_BOUND('',#28466,.T.) ;
#22604=FACE_OUTER_BOUND('',#28467,.T.) ;
#22605=FACE_OUTER_BOUND('',#28468,.T.) ;
#22606=FACE_OUTER_BOUND('',#28469,.T.) ;
#22607=FACE_OUTER_BOUND('',#28470,.T.) ;
#22608=FACE_OUTER_BOUND('',#28471,.T.) ;
#22609=FACE_OUTER_BOUND('',#28472,.T.) ;
#22610=FACE_OUTER_BOUND('',#28473,.T.) ;
#22611=FACE_OUTER_BOUND('',#28474,.T.) ;
#22612=FACE_OUTER_BOUND('',#28475,.T.) ;
#22613=FACE_OUTER_BOUND('',#28476,.T.) ;
#22614=FACE_OUTER_BOUND('',#28477,.T.) ;
#22615=FACE_OUTER_BOUND('',#28478,.T.) ;
#22616=FACE_OUTER_BOUND('',#28479,.T.) ;
#22617=FACE_OUTER_BOUND('',#28480,.T.) ;
#22618=FACE_OUTER_BOUND('',#28481,.T.) ;
#22619=FACE_OUTER_BOUND('',#28482,.T.) ;
#22620=FACE_OUTER_BOUND('',#28483,.T.) ;
#22621=FACE_OUTER_BOUND('',#28484,.T.) ;
#22622=FACE_OUTER_BOUND('',#28485,.T.) ;
#22623=FACE_OUTER_BOUND('',#28486,.T.) ;
#22624=FACE_OUTER_BOUND('',#28487,.T.) ;
#22625=FACE_OUTER_BOUND('',#28488,.T.) ;
#22626=FACE_OUTER_BOUND('',#28489,.T.) ;
#22627=FACE_OUTER_BOUND('',#28490,.T.) ;
#22628=FACE_OUTER_BOUND('',#28491,.T.) ;
#22629=FACE_OUTER_BOUND('',#28492,.T.) ;
#22630=FACE_OUTER_BOUND('',#28493,.T.) ;
#22631=FACE_OUTER_BOUND('',#28494,.T.) ;
#22632=FACE_OUTER_BOUND('',#28495,.T.) ;
#22633=FACE_OUTER_BOUND('',#28496,.T.) ;
#22634=FACE_OUTER_BOUND('',#28497,.T.) ;
#22635=FACE_OUTER_BOUND('',#28498,.T.) ;
#22636=FACE_OUTER_BOUND('',#28499,.T.) ;
#22637=FACE_OUTER_BOUND('',#28500,.T.) ;
#22638=FACE_OUTER_BOUND('',#28501,.T.) ;
#22639=FACE_OUTER_BOUND('',#28502,.T.) ;
#22640=FACE_OUTER_BOUND('',#28503,.T.) ;
#22641=FACE_OUTER_BOUND('',#28504,.T.) ;
#22642=FACE_OUTER_BOUND('',#28505,.T.) ;
#22643=FACE_OUTER_BOUND('',#28506,.T.) ;
#22644=FACE_OUTER_BOUND('',#28507,.T.) ;
#22645=FACE_OUTER_BOUND('',#28508,.T.) ;
#22646=FACE_OUTER_BOUND('',#28509,.T.) ;
#22647=FACE_OUTER_BOUND('',#28510,.T.) ;
#22648=FACE_OUTER_BOUND('',#28511,.T.) ;
#22649=FACE_OUTER_BOUND('',#28512,.T.) ;
#22650=FACE_OUTER_BOUND('',#28513,.T.) ;
#22651=FACE_OUTER_BOUND('',#28514,.T.) ;
#22652=FACE_OUTER_BOUND('',#28515,.T.) ;
#22653=FACE_OUTER_BOUND('',#28516,.T.) ;
#22654=FACE_OUTER_BOUND('',#28517,.T.) ;
#22655=FACE_OUTER_BOUND('',#28518,.T.) ;
#22656=FACE_OUTER_BOUND('',#28519,.T.) ;
#22657=FACE_OUTER_BOUND('',#28520,.T.) ;
#22658=FACE_OUTER_BOUND('',#28521,.T.) ;
#22659=FACE_OUTER_BOUND('',#28522,.T.) ;
#22660=FACE_OUTER_BOUND('',#28523,.T.) ;
#22661=FACE_OUTER_BOUND('',#28524,.T.) ;
#22662=FACE_OUTER_BOUND('',#28525,.T.) ;
#22663=FACE_OUTER_BOUND('',#28526,.T.) ;
#22664=FACE_OUTER_BOUND('',#28527,.T.) ;
#22665=FACE_OUTER_BOUND('',#28528,.T.) ;
#22666=FACE_OUTER_BOUND('',#28529,.T.) ;
#22667=FACE_OUTER_BOUND('',#28530,.T.) ;
#22668=FACE_OUTER_BOUND('',#28531,.T.) ;
#22669=FACE_OUTER_BOUND('',#28532,.T.) ;
#22670=FACE_OUTER_BOUND('',#28533,.T.) ;
#22671=FACE_OUTER_BOUND('',#28534,.T.) ;
#22672=FACE_OUTER_BOUND('',#28535,.T.) ;
#22673=FACE_OUTER_BOUND('',#28536,.T.) ;
#22674=FACE_OUTER_BOUND('',#28537,.T.) ;
#22675=FACE_OUTER_BOUND('',#28538,.T.) ;
#22676=FACE_OUTER_BOUND('',#28539,.T.) ;
#22677=FACE_OUTER_BOUND('',#28540,.T.) ;
#22678=FACE_OUTER_BOUND('',#28541,.T.) ;
#22679=FACE_OUTER_BOUND('',#28542,.T.) ;
#22680=FACE_OUTER_BOUND('',#28543,.T.) ;
#22681=FACE_OUTER_BOUND('',#28544,.T.) ;
#22682=FACE_OUTER_BOUND('',#28545,.T.) ;
#22683=FACE_OUTER_BOUND('',#28546,.T.) ;
#22684=FACE_OUTER_BOUND('',#28547,.T.) ;
#22685=FACE_OUTER_BOUND('',#28548,.T.) ;
#22686=FACE_OUTER_BOUND('',#28549,.T.) ;
#22687=FACE_OUTER_BOUND('',#28550,.T.) ;
#22688=FACE_OUTER_BOUND('',#28551,.T.) ;
#22689=FACE_OUTER_BOUND('',#28552,.T.) ;
#22690=FACE_OUTER_BOUND('',#28553,.T.) ;
#22691=FACE_OUTER_BOUND('',#28554,.T.) ;
#22692=FACE_OUTER_BOUND('',#28555,.T.) ;
#22693=FACE_OUTER_BOUND('',#28556,.T.) ;
#22694=FACE_OUTER_BOUND('',#28557,.T.) ;
#22695=FACE_OUTER_BOUND('',#28558,.T.) ;
#22696=FACE_OUTER_BOUND('',#28559,.T.) ;
#22697=FACE_OUTER_BOUND('',#28560,.T.) ;
#22698=FACE_OUTER_BOUND('',#28561,.T.) ;
#22699=FACE_OUTER_BOUND('',#28562,.T.) ;
#22700=FACE_OUTER_BOUND('',#28563,.T.) ;
#22701=FACE_OUTER_BOUND('',#28564,.T.) ;
#22702=FACE_OUTER_BOUND('',#28565,.T.) ;
#22703=FACE_OUTER_BOUND('',#28566,.T.) ;
#22704=FACE_OUTER_BOUND('',#28567,.T.) ;
#22705=FACE_OUTER_BOUND('',#28568,.T.) ;
#22706=FACE_OUTER_BOUND('',#28569,.T.) ;
#22707=FACE_OUTER_BOUND('',#28570,.T.) ;
#22708=FACE_OUTER_BOUND('',#28571,.T.) ;
#22709=FACE_OUTER_BOUND('',#28572,.T.) ;
#22710=FACE_OUTER_BOUND('',#28573,.T.) ;
#22711=FACE_OUTER_BOUND('',#28574,.T.) ;
#22712=FACE_OUTER_BOUND('',#28575,.T.) ;
#22713=FACE_OUTER_BOUND('',#28576,.T.) ;
#22714=FACE_OUTER_BOUND('',#28577,.T.) ;
#22715=FACE_OUTER_BOUND('',#28578,.T.) ;
#22716=FACE_OUTER_BOUND('',#28579,.T.) ;
#22717=FACE_OUTER_BOUND('',#28580,.T.) ;
#22718=FACE_OUTER_BOUND('',#28581,.T.) ;
#22719=FACE_OUTER_BOUND('',#28582,.T.) ;
#22720=FACE_OUTER_BOUND('',#28583,.T.) ;
#22721=FACE_OUTER_BOUND('',#28584,.T.) ;
#22722=FACE_OUTER_BOUND('',#28585,.T.) ;
#22723=FACE_OUTER_BOUND('',#28586,.T.) ;
#22724=FACE_OUTER_BOUND('',#28587,.T.) ;
#22725=FACE_OUTER_BOUND('',#28588,.T.) ;
#22726=FACE_OUTER_BOUND('',#28589,.T.) ;
#22727=FACE_OUTER_BOUND('',#28590,.T.) ;
#22728=FACE_OUTER_BOUND('',#28591,.T.) ;
#22729=FACE_OUTER_BOUND('',#28592,.T.) ;
#22730=FACE_OUTER_BOUND('',#28593,.T.) ;
#22731=FACE_OUTER_BOUND('',#28594,.T.) ;
#22732=FACE_OUTER_BOUND('',#28595,.T.) ;
#22733=FACE_OUTER_BOUND('',#28596,.T.) ;
#22734=FACE_OUTER_BOUND('',#28597,.T.) ;
#22735=FACE_OUTER_BOUND('',#28598,.T.) ;
#22736=FACE_OUTER_BOUND('',#28599,.T.) ;
#22737=FACE_OUTER_BOUND('',#28600,.T.) ;
#22738=FACE_OUTER_BOUND('',#28601,.T.) ;
#22739=FACE_OUTER_BOUND('',#28602,.T.) ;
#22740=FACE_OUTER_BOUND('',#28603,.T.) ;
#22741=FACE_OUTER_BOUND('',#28604,.T.) ;
#22742=FACE_OUTER_BOUND('',#28605,.T.) ;
#22743=FACE_OUTER_BOUND('',#28606,.T.) ;
#22744=FACE_OUTER_BOUND('',#28607,.T.) ;
#22745=FACE_OUTER_BOUND('',#28608,.T.) ;
#22746=FACE_OUTER_BOUND('',#28609,.T.) ;
#22747=FACE_OUTER_BOUND('',#28610,.T.) ;
#22748=FACE_OUTER_BOUND('',#28611,.T.) ;
#22749=FACE_OUTER_BOUND('',#28612,.T.) ;
#22750=FACE_OUTER_BOUND('',#28613,.T.) ;
#22751=FACE_OUTER_BOUND('',#28614,.T.) ;
#22752=FACE_OUTER_BOUND('',#28615,.T.) ;
#22753=FACE_OUTER_BOUND('',#28616,.T.) ;
#22754=FACE_OUTER_BOUND('',#28617,.T.) ;
#22755=FACE_OUTER_BOUND('',#28618,.T.) ;
#22756=FACE_OUTER_BOUND('',#28619,.T.) ;
#22757=FACE_OUTER_BOUND('',#28620,.T.) ;
#22758=FACE_OUTER_BOUND('',#28621,.T.) ;
#22759=FACE_OUTER_BOUND('',#28622,.T.) ;
#22760=FACE_OUTER_BOUND('',#28623,.T.) ;
#22761=FACE_OUTER_BOUND('',#28624,.T.) ;
#22762=FACE_OUTER_BOUND('',#28625,.T.) ;
#26181=EDGE_LOOP('',(#68639,#68640,#68641,#68642)) ;
#26182=EDGE_LOOP('',(#68643,#68644,#68645,#68646)) ;
#26183=EDGE_LOOP('',(#68647,#68648,#68649,#68650)) ;
#26184=EDGE_LOOP('',(#68651,#68652,#68653,#68654)) ;
#26185=EDGE_LOOP('',(#68655,#68656,#68657,#68658)) ;
#26186=EDGE_LOOP('',(#68659,#68660,#68661,#68662)) ;
#26187=EDGE_LOOP('',(#68663,#68664,#68665,#68666)) ;
#26188=EDGE_LOOP('',(#68667,#68668,#68669,#68670)) ;
#26189=EDGE_LOOP('',(#68671,#68672,#68673,#68674)) ;
#26190=EDGE_LOOP('',(#68675,#68676,#68677,#68678)) ;
#26191=EDGE_LOOP('',(#68679,#68680,#68681,#68682)) ;
#26192=EDGE_LOOP('',(#68683,#68684,#68685,#68686)) ;
#26193=EDGE_LOOP('',(#68687,#68688,#68689,#68690)) ;
#26194=EDGE_LOOP('',(#68691,#68692,#68693,#68694)) ;
#26195=EDGE_LOOP('',(#68695,#68696,#68697,#68698)) ;
#26196=EDGE_LOOP('',(#68699,#68700,#68701,#68702)) ;
#26197=EDGE_LOOP('',(#68703,#68704,#68705,#68706)) ;
#26198=EDGE_LOOP('',(#68707,#68708,#68709,#68710)) ;
#26199=EDGE_LOOP('',(#68711,#68712,#68713,#68714)) ;
#26200=EDGE_LOOP('',(#68715,#68716,#68717,#68718)) ;
#26201=EDGE_LOOP('',(#68719,#68720,#68721,#68722)) ;
#26202=EDGE_LOOP('',(#68723,#68724,#68725,#68726)) ;
#26203=EDGE_LOOP('',(#68727,#68728,#68729,#68730)) ;
#26204=EDGE_LOOP('',(#68731,#68732,#68733,#68734)) ;
#26205=EDGE_LOOP('',(#68735,#68736,#68737,#68738)) ;
#26206=EDGE_LOOP('',(#68739,#68740,#68741,#68742)) ;
#26207=EDGE_LOOP('',(#68743,#68744,#68745,#68746)) ;
#26208=EDGE_LOOP('',(#68747,#68748,#68749,#68750)) ;
#26209=EDGE_LOOP('',(#68751,#68752,#68753,#68754)) ;
#26210=EDGE_LOOP('',(#68755,#68756,#68757,#68758)) ;
#26211=EDGE_LOOP('',(#68759,#68760,#68761,#68762)) ;
#26212=EDGE_LOOP('',(#68763,#68764,#68765,#68766)) ;
#26213=EDGE_LOOP('',(#68767,#68768,#68769,#68770)) ;
#26214=EDGE_LOOP('',(#68771,#68772,#68773,#68774)) ;
#26215=EDGE_LOOP('',(#68775,#68776,#68777,#68778)) ;
#26216=EDGE_LOOP('',(#68779,#68780,#68781,#68782)) ;
#26217=EDGE_LOOP('',(#68783,#68784,#68785,#68786)) ;
#26218=EDGE_LOOP('',(#68787,#68788,#68789,#68790)) ;
#26219=EDGE_LOOP('',(#68791,#68792,#68793,#68794)) ;
#26220=EDGE_LOOP('',(#68795,#68796,#68797,#68798)) ;
#26221=EDGE_LOOP('',(#68799,#68800,#68801,#68802)) ;
#26222=EDGE_LOOP('',(#68803,#68804,#68805,#68806)) ;
#26223=EDGE_LOOP('',(#68807,#68808,#68809,#68810)) ;
#26224=EDGE_LOOP('',(#68811,#68812,#68813,#68814)) ;
#26225=EDGE_LOOP('',(#68815,#68816,#68817,#68818)) ;
#26226=EDGE_LOOP('',(#68819,#68820,#68821,#68822)) ;
#26227=EDGE_LOOP('',(#68823,#68824,#68825,#68826)) ;
#26228=EDGE_LOOP('',(#68827,#68828,#68829,#68830)) ;
#26229=EDGE_LOOP('',(#68831,#68832,#68833,#68834)) ;
#26230=EDGE_LOOP('',(#68835,#68836,#68837,#68838)) ;
#26231=EDGE_LOOP('',(#68839,#68840,#68841,#68842)) ;
#26232=EDGE_LOOP('',(#68843,#68844,#68845,#68846)) ;
#26233=EDGE_LOOP('',(#68847,#68848,#68849,#68850)) ;
#26234=EDGE_LOOP('',(#68851,#68852,#68853,#68854)) ;
#26235=EDGE_LOOP('',(#68855,#68856,#68857,#68858)) ;
#26236=EDGE_LOOP('',(#68859,#68860,#68861,#68862)) ;
#26237=EDGE_LOOP('',(#68863,#68864,#68865,#68866,#68867,#68868,#68869,#68870,
#68871,#68872,#68873,#68874,#68875,#68876,#68877,#68878,#68879,#68880,#68881,
#68882)) ;
#26238=EDGE_LOOP('',(#68883,#68884,#68885,#68886,#68887,#68888,#68889,#68890,
#68891,#68892,#68893,#68894,#68895,#68896,#68897,#68898,#68899,#68900,#68901,
#68902)) ;
#26239=EDGE_LOOP('',(#68903,#68904,#68905,#68906,#68907,#68908,#68909,#68910,
#68911,#68912,#68913,#68914,#68915,#68916,#68917,#68918,#68919,#68920,#68921,
#68922)) ;
#26240=EDGE_LOOP('',(#68923,#68924,#68925,#68926,#68927,#68928,#68929,#68930,
#68931,#68932,#68933,#68934,#68935,#68936,#68937,#68938,#68939,#68940,#68941,
#68942)) ;
#26241=EDGE_LOOP('',(#68943,#68944,#68945,#68946,#68947,#68948,#68949,#68950,
#68951,#68952,#68953,#68954,#68955,#68956,#68957,#68958,#68959,#68960,#68961,
#68962)) ;
#26242=EDGE_LOOP('',(#68963,#68964,#68965,#68966,#68967,#68968,#68969,#68970,
#68971,#68972,#68973,#68974,#68975,#68976,#68977,#68978,#68979,#68980,#68981,
#68982)) ;
#26243=EDGE_LOOP('',(#68983,#68984,#68985,#68986,#68987,#68988,#68989,#68990,
#68991,#68992,#68993,#68994,#68995,#68996,#68997,#68998,#68999,#69000,#69001,
#69002)) ;
#26244=EDGE_LOOP('',(#69003,#69004,#69005,#69006,#69007,#69008,#69009,#69010,
#69011,#69012,#69013,#69014,#69015,#69016,#69017,#69018,#69019,#69020,#69021,
#69022)) ;
#26245=EDGE_LOOP('',(#69023,#69024,#69025,#69026,#69027,#69028,#69029,#69030,
#69031,#69032,#69033,#69034,#69035,#69036,#69037,#69038,#69039,#69040,#69041,
#69042)) ;
#26246=EDGE_LOOP('',(#69043,#69044,#69045,#69046)) ;
#26247=EDGE_LOOP('',(#69047,#69048,#69049,#69050)) ;
#26248=EDGE_LOOP('',(#69051,#69052,#69053,#69054)) ;
#26249=EDGE_LOOP('',(#69055,#69056,#69057,#69058)) ;
#26250=EDGE_LOOP('',(#69059,#69060,#69061,#69062)) ;
#26251=EDGE_LOOP('',(#69063,#69064,#69065,#69066)) ;
#26252=EDGE_LOOP('',(#69067,#69068,#69069,#69070)) ;
#26253=EDGE_LOOP('',(#69071,#69072,#69073,#69074)) ;
#26254=EDGE_LOOP('',(#69075,#69076,#69077,#69078)) ;
#26255=EDGE_LOOP('',(#69079,#69080,#69081,#69082)) ;
#26256=EDGE_LOOP('',(#69083,#69084,#69085,#69086)) ;
#26257=EDGE_LOOP('',(#69087,#69088,#69089,#69090)) ;
#26258=EDGE_LOOP('',(#69091,#69092,#69093,#69094)) ;
#26259=EDGE_LOOP('',(#69095,#69096,#69097,#69098)) ;
#26260=EDGE_LOOP('',(#69099,#69100,#69101,#69102)) ;
#26261=EDGE_LOOP('',(#69103,#69104,#69105,#69106)) ;
#26262=EDGE_LOOP('',(#69107,#69108,#69109,#69110)) ;
#26263=EDGE_LOOP('',(#69111,#69112,#69113,#69114)) ;
#26264=EDGE_LOOP('',(#69115,#69116,#69117,#69118)) ;
#26265=EDGE_LOOP('',(#69119,#69120,#69121,#69122)) ;
#26266=EDGE_LOOP('',(#69123,#69124,#69125,#69126)) ;
#26267=EDGE_LOOP('',(#69127,#69128,#69129,#69130)) ;
#26268=EDGE_LOOP('',(#69131,#69132,#69133,#69134)) ;
#26269=EDGE_LOOP('',(#69135,#69136,#69137,#69138)) ;
#26270=EDGE_LOOP('',(#69139,#69140,#69141,#69142)) ;
#26271=EDGE_LOOP('',(#69143,#69144,#69145,#69146,#69147,#69148,#69149,#69150,
#69151,#69152,#69153,#69154,#69155,#69156,#69157,#69158,#69159,#69160,#69161,
#69162)) ;
#26272=EDGE_LOOP('',(#69163,#69164,#69165,#69166)) ;
#26273=EDGE_LOOP('',(#69167,#69168,#69169,#69170)) ;
#26274=EDGE_LOOP('',(#69171,#69172,#69173,#69174,#69175,#69176,#69177,#69178,
#69179,#69180,#69181,#69182,#69183,#69184,#69185,#69186,#69187,#69188,#69189,
#69190,#69191,#69192,#69193,#69194,#69195,#69196,#69197,#69198)) ;
#26275=EDGE_LOOP('',(#69199,#69200,#69201,#69202,#69203,#69204,#69205,#69206)) ;
#26276=EDGE_LOOP('',(#69207)) ;
#26277=EDGE_LOOP('',(#69208,#69209,#69210,#69211,#69212,#69213,#69214,#69215)) ;
#26278=EDGE_LOOP('',(#69216)) ;
#26279=EDGE_LOOP('',(#69217,#69218,#69219,#69220,#69221,#69222,#69223,#69224)) ;
#26280=EDGE_LOOP('',(#69225)) ;
#26281=EDGE_LOOP('',(#69226,#69227,#69228,#69229,#69230,#69231,#69232,#69233)) ;
#26282=EDGE_LOOP('',(#69234)) ;
#26283=EDGE_LOOP('',(#69235,#69236,#69237,#69238,#69239,#69240,#69241,#69242)) ;
#26284=EDGE_LOOP('',(#69243)) ;
#26285=EDGE_LOOP('',(#69244)) ;
#26286=EDGE_LOOP('',(#69245,#69246,#69247,#69248,#69249,#69250,#69251,#69252)) ;
#26287=EDGE_LOOP('',(#69253)) ;
#26288=EDGE_LOOP('',(#69254,#69255,#69256,#69257,#69258,#69259,#69260,#69261)) ;
#26289=EDGE_LOOP('',(#69262)) ;
#26290=EDGE_LOOP('',(#69263,#69264,#69265,#69266,#69267,#69268,#69269,#69270)) ;
#26291=EDGE_LOOP('',(#69271)) ;
#26292=EDGE_LOOP('',(#69272,#69273,#69274,#69275,#69276,#69277,#69278,#69279)) ;
#26293=EDGE_LOOP('',(#69280)) ;
#26294=EDGE_LOOP('',(#69281,#69282,#69283,#69284,#69285,#69286,#69287,#69288)) ;
#26295=EDGE_LOOP('',(#69289,#69290,#69291,#69292)) ;
#26296=EDGE_LOOP('',(#69293,#69294,#69295,#69296,#69297,#69298,#69299,#69300)) ;
#26297=EDGE_LOOP('',(#69301,#69302,#69303,#69304)) ;
#26298=EDGE_LOOP('',(#69305,#69306,#69307,#69308,#69309,#69310,#69311,#69312)) ;
#26299=EDGE_LOOP('',(#69313,#69314,#69315,#69316)) ;
#26300=EDGE_LOOP('',(#69317,#69318,#69319,#69320,#69321,#69322,#69323,#69324)) ;
#26301=EDGE_LOOP('',(#69325,#69326,#69327,#69328)) ;
#26302=EDGE_LOOP('',(#69329,#69330,#69331,#69332,#69333,#69334,#69335,#69336)) ;
#26303=EDGE_LOOP('',(#69337,#69338,#69339,#69340)) ;
#26304=EDGE_LOOP('',(#69341,#69342,#69343,#69344,#69345,#69346,#69347,#69348)) ;
#26305=EDGE_LOOP('',(#69349,#69350,#69351,#69352)) ;
#26306=EDGE_LOOP('',(#69353,#69354,#69355,#69356,#69357,#69358,#69359,#69360)) ;
#26307=EDGE_LOOP('',(#69361,#69362,#69363,#69364)) ;
#26308=EDGE_LOOP('',(#69365,#69366,#69367,#69368,#69369,#69370,#69371,#69372)) ;
#26309=EDGE_LOOP('',(#69373,#69374,#69375,#69376)) ;
#26310=EDGE_LOOP('',(#69377,#69378,#69379,#69380,#69381,#69382,#69383,#69384)) ;
#26311=EDGE_LOOP('',(#69385,#69386,#69387,#69388)) ;
#26312=EDGE_LOOP('',(#69389,#69390,#69391,#69392,#69393,#69394,#69395,#69396)) ;
#26313=EDGE_LOOP('',(#69397,#69398)) ;
#26314=EDGE_LOOP('',(#69399,#69400)) ;
#26315=EDGE_LOOP('',(#69401,#69402)) ;
#26316=EDGE_LOOP('',(#69403,#69404)) ;
#26317=EDGE_LOOP('',(#69405,#69406)) ;
#26318=EDGE_LOOP('',(#69407,#69408)) ;
#26319=EDGE_LOOP('',(#69409,#69410)) ;
#26320=EDGE_LOOP('',(#69411,#69412)) ;
#26321=EDGE_LOOP('',(#69413,#69414)) ;
#26322=EDGE_LOOP('',(#69415,#69416,#69417,#69418,#69419,#69420,#69421,#69422,
#69423,#69424,#69425,#69426,#69427,#69428,#69429,#69430,#69431,#69432,#69433,
#69434,#69435,#69436,#69437,#69438,#69439,#69440,#69441,#69442,#69443,#69444,
#69445,#69446,#69447,#69448,#69449,#69450,#69451,#69452,#69453,#69454,#69455,
#69456,#69457,#69458,#69459,#69460,#69461,#69462,#69463,#69464,#69465,#69466,
#69467,#69468,#69469,#69470,#69471,#69472,#69473,#69474,#69475,#69476,#69477,
#69478)) ;
#26323=EDGE_LOOP('',(#69479,#69480,#69481,#69482,#69483,#69484,#69485,#69486)) ;
#26324=EDGE_LOOP('',(#69487,#69488,#69489,#69490,#69491,#69492,#69493,#69494)) ;
#26325=EDGE_LOOP('',(#69495,#69496,#69497,#69498,#69499,#69500,#69501,#69502)) ;
#26326=EDGE_LOOP('',(#69503,#69504,#69505,#69506,#69507,#69508,#69509,#69510)) ;
#26327=EDGE_LOOP('',(#69511,#69512,#69513,#69514,#69515,#69516,#69517,#69518)) ;
#26328=EDGE_LOOP('',(#69519,#69520,#69521,#69522,#69523,#69524,#69525,#69526)) ;
#26329=EDGE_LOOP('',(#69527,#69528,#69529,#69530,#69531,#69532,#69533,#69534)) ;
#26330=EDGE_LOOP('',(#69535,#69536,#69537,#69538,#69539,#69540,#69541,#69542)) ;
#26331=EDGE_LOOP('',(#69543,#69544,#69545,#69546,#69547,#69548,#69549,#69550)) ;
#26332=EDGE_LOOP('',(#69551,#69552,#69553,#69554)) ;
#26333=EDGE_LOOP('',(#69555,#69556,#69557,#69558,#69559,#69560,#69561,#69562,
#69563,#69564,#69565,#69566,#69567,#69568,#69569,#69570,#69571,#69572,#69573,
#69574,#69575,#69576,#69577,#69578,#69579,#69580,#69581,#69582,#69583,#69584,
#69585,#69586,#69587,#69588,#69589,#69590,#69591,#69592,#69593,#69594,#69595,
#69596,#69597,#69598,#69599,#69600,#69601,#69602,#69603,#69604,#69605,#69606,
#69607,#69608,#69609,#69610,#69611,#69612,#69613,#69614,#69615,#69616,#69617,
#69618)) ;
#26334=EDGE_LOOP('',(#69619,#69620,#69621,#69622)) ;
#26335=EDGE_LOOP('',(#69623,#69624,#69625,#69626,#69627,#69628)) ;
#26336=EDGE_LOOP('',(#69629,#69630,#69631,#69632)) ;
#26337=EDGE_LOOP('',(#69633,#69634,#69635,#69636,#69637,#69638,#69639,#69640)) ;
#26338=EDGE_LOOP('',(#69641,#69642,#69643,#69644)) ;
#26339=EDGE_LOOP('',(#69645,#69646,#69647,#69648)) ;
#26340=EDGE_LOOP('',(#69649,#69650,#69651,#69652)) ;
#26341=EDGE_LOOP('',(#69653,#69654,#69655,#69656)) ;
#26342=EDGE_LOOP('',(#69657,#69658,#69659,#69660)) ;
#26343=EDGE_LOOP('',(#69661,#69662,#69663,#69664)) ;
#26344=EDGE_LOOP('',(#69665,#69666,#69667,#69668)) ;
#26345=EDGE_LOOP('',(#69669,#69670,#69671,#69672)) ;
#26346=EDGE_LOOP('',(#69673,#69674,#69675,#69676,#69677,#69678,#69679,#69680)) ;
#26347=EDGE_LOOP('',(#69681,#69682,#69683,#69684)) ;
#26348=EDGE_LOOP('',(#69685,#69686,#69687,#69688,#69689,#69690,#69691,#69692)) ;
#26349=EDGE_LOOP('',(#69693,#69694,#69695,#69696)) ;
#26350=EDGE_LOOP('',(#69697,#69698)) ;
#26351=EDGE_LOOP('',(#69699,#69700,#69701,#69702,#69703,#69704,#69705,#69706)) ;
#26352=EDGE_LOOP('',(#69707,#69708,#69709,#69710)) ;
#26353=EDGE_LOOP('',(#69711,#69712,#69713,#69714)) ;
#26354=EDGE_LOOP('',(#69715,#69716,#69717,#69718)) ;
#26355=EDGE_LOOP('',(#69719,#69720,#69721,#69722)) ;
#26356=EDGE_LOOP('',(#69723,#69724,#69725,#69726)) ;
#26357=EDGE_LOOP('',(#69727,#69728,#69729,#69730)) ;
#26358=EDGE_LOOP('',(#69731,#69732,#69733,#69734)) ;
#26359=EDGE_LOOP('',(#69735,#69736,#69737,#69738)) ;
#26360=EDGE_LOOP('',(#69739,#69740,#69741,#69742)) ;
#26361=EDGE_LOOP('',(#69743,#69744,#69745,#69746)) ;
#26362=EDGE_LOOP('',(#69747,#69748,#69749,#69750)) ;
#26363=EDGE_LOOP('',(#69751,#69752,#69753,#69754)) ;
#26364=EDGE_LOOP('',(#69755,#69756,#69757,#69758,#69759,#69760,#69761,#69762)) ;
#26365=EDGE_LOOP('',(#69763,#69764,#69765,#69766,#69767,#69768,#69769,#69770)) ;
#26366=EDGE_LOOP('',(#69771,#69772,#69773,#69774,#69775,#69776,#69777,#69778,
#69779,#69780,#69781,#69782,#69783,#69784,#69785)) ;
#26367=EDGE_LOOP('',(#69786,#69787,#69788,#69789,#69790,#69791,#69792,#69793,
#69794,#69795,#69796,#69797,#69798,#69799,#69800)) ;
#26368=EDGE_LOOP('',(#69801,#69802,#69803,#69804)) ;
#26369=EDGE_LOOP('',(#69805,#69806,#69807,#69808)) ;
#26370=EDGE_LOOP('',(#69809,#69810,#69811,#69812,#69813,#69814,#69815,#69816)) ;
#26371=EDGE_LOOP('',(#69817,#69818,#69819,#69820)) ;
#26372=EDGE_LOOP('',(#69821,#69822,#69823,#69824)) ;
#26373=EDGE_LOOP('',(#69825,#69826,#69827,#69828,#69829,#69830)) ;
#26374=EDGE_LOOP('',(#69831,#69832,#69833,#69834,#69835,#69836)) ;
#26375=EDGE_LOOP('',(#69837,#69838,#69839,#69840)) ;
#26376=EDGE_LOOP('',(#69841,#69842,#69843,#69844)) ;
#26377=EDGE_LOOP('',(#69845,#69846,#69847,#69848)) ;
#26378=EDGE_LOOP('',(#69849,#69850,#69851,#69852)) ;
#26379=EDGE_LOOP('',(#69853,#69854,#69855,#69856)) ;
#26380=EDGE_LOOP('',(#69857,#69858,#69859,#69860,#69861,#69862,#69863,#69864)) ;
#26381=EDGE_LOOP('',(#69865,#69866,#69867,#69868)) ;
#26382=EDGE_LOOP('',(#69869,#69870,#69871,#69872)) ;
#26383=EDGE_LOOP('',(#69873,#69874,#69875,#69876)) ;
#26384=EDGE_LOOP('',(#69877,#69878,#69879,#69880)) ;
#26385=EDGE_LOOP('',(#69881,#69882,#69883,#69884)) ;
#26386=EDGE_LOOP('',(#69885,#69886,#69887,#69888,#69889,#69890,#69891,#69892,
#69893,#69894,#69895,#69896,#69897,#69898,#69899,#69900,#69901,#69902,#69903)) ;
#26387=EDGE_LOOP('',(#69904,#69905,#69906,#69907)) ;
#26388=EDGE_LOOP('',(#69908,#69909,#69910,#69911,#69912,#69913,#69914,#69915,
#69916,#69917)) ;
#26389=EDGE_LOOP('',(#69918,#69919,#69920,#69921)) ;
#26390=EDGE_LOOP('',(#69922,#69923,#69924,#69925,#69926,#69927,#69928,#69929,
#69930,#69931)) ;
#26391=EDGE_LOOP('',(#69932,#69933,#69934,#69935)) ;
#26392=EDGE_LOOP('',(#69936,#69937,#69938,#69939)) ;
#26393=EDGE_LOOP('',(#69940,#69941,#69942,#69943)) ;
#26394=EDGE_LOOP('',(#69944,#69945,#69946,#69947)) ;
#26395=EDGE_LOOP('',(#69948,#69949,#69950,#69951,#69952,#69953)) ;
#26396=EDGE_LOOP('',(#69954)) ;
#26397=EDGE_LOOP('',(#69955)) ;
#26398=EDGE_LOOP('',(#69956,#69957,#69958,#69959)) ;
#26399=EDGE_LOOP('',(#69960,#69961,#69962,#69963)) ;
#26400=EDGE_LOOP('',(#69964,#69965,#69966,#69967)) ;
#26401=EDGE_LOOP('',(#69968,#69969,#69970,#69971)) ;
#26402=EDGE_LOOP('',(#69972,#69973,#69974,#69975)) ;
#26403=EDGE_LOOP('',(#69976,#69977,#69978,#69979,#69980,#69981,#69982,#69983)) ;
#26404=EDGE_LOOP('',(#69984,#69985,#69986,#69987)) ;
#26405=EDGE_LOOP('',(#69988,#69989,#69990,#69991)) ;
#26406=EDGE_LOOP('',(#69992,#69993,#69994,#69995)) ;
#26407=EDGE_LOOP('',(#69996,#69997,#69998,#69999)) ;
#26408=EDGE_LOOP('',(#70000,#70001,#70002,#70003)) ;
#26409=EDGE_LOOP('',(#70004,#70005,#70006)) ;
#26410=EDGE_LOOP('',(#70007,#70008,#70009,#70010)) ;
#26411=EDGE_LOOP('',(#70011,#70012,#70013,#70014)) ;
#26412=EDGE_LOOP('',(#70015,#70016,#70017,#70018)) ;
#26413=EDGE_LOOP('',(#70019,#70020,#70021,#70022)) ;
#26414=EDGE_LOOP('',(#70023,#70024,#70025,#70026)) ;
#26415=EDGE_LOOP('',(#70027,#70028,#70029,#70030)) ;
#26416=EDGE_LOOP('',(#70031,#70032,#70033,#70034)) ;
#26417=EDGE_LOOP('',(#70035,#70036,#70037,#70038)) ;
#26418=EDGE_LOOP('',(#70039,#70040,#70041,#70042)) ;
#26419=EDGE_LOOP('',(#70043,#70044,#70045,#70046)) ;
#26420=EDGE_LOOP('',(#70047,#70048,#70049,#70050)) ;
#26421=EDGE_LOOP('',(#70051,#70052,#70053,#70054)) ;
#26422=EDGE_LOOP('',(#70055,#70056,#70057,#70058)) ;
#26423=EDGE_LOOP('',(#70059,#70060,#70061,#70062)) ;
#26424=EDGE_LOOP('',(#70063,#70064,#70065,#70066)) ;
#26425=EDGE_LOOP('',(#70067,#70068,#70069,#70070)) ;
#26426=EDGE_LOOP('',(#70071,#70072,#70073,#70074)) ;
#26427=EDGE_LOOP('',(#70075,#70076,#70077,#70078)) ;
#26428=EDGE_LOOP('',(#70079,#70080,#70081,#70082)) ;
#26429=EDGE_LOOP('',(#70083,#70084,#70085)) ;
#26430=EDGE_LOOP('',(#70086,#70087,#70088,#70089)) ;
#26431=EDGE_LOOP('',(#70090,#70091,#70092,#70093)) ;
#26432=EDGE_LOOP('',(#70094,#70095,#70096,#70097)) ;
#26433=EDGE_LOOP('',(#70098,#70099,#70100,#70101)) ;
#26434=EDGE_LOOP('',(#70102,#70103,#70104,#70105)) ;
#26435=EDGE_LOOP('',(#70106,#70107,#70108,#70109)) ;
#26436=EDGE_LOOP('',(#70110,#70111,#70112)) ;
#26437=EDGE_LOOP('',(#70113,#70114,#70115)) ;
#26438=EDGE_LOOP('',(#70116,#70117,#70118,#70119)) ;
#26439=EDGE_LOOP('',(#70120,#70121,#70122,#70123)) ;
#26440=EDGE_LOOP('',(#70124,#70125,#70126,#70127,#70128,#70129)) ;
#26441=EDGE_LOOP('',(#70130,#70131,#70132,#70133)) ;
#26442=EDGE_LOOP('',(#70134,#70135,#70136,#70137)) ;
#26443=EDGE_LOOP('',(#70138,#70139,#70140,#70141)) ;
#26444=EDGE_LOOP('',(#70142,#70143,#70144,#70145)) ;
#26445=EDGE_LOOP('',(#70146,#70147,#70148,#70149)) ;
#26446=EDGE_LOOP('',(#70150,#70151,#70152,#70153)) ;
#26447=EDGE_LOOP('',(#70154,#70155,#70156)) ;
#26448=EDGE_LOOP('',(#70157,#70158,#70159,#70160)) ;
#26449=EDGE_LOOP('',(#70161,#70162,#70163,#70164)) ;
#26450=EDGE_LOOP('',(#70165,#70166,#70167,#70168)) ;
#26451=EDGE_LOOP('',(#70169,#70170,#70171,#70172)) ;
#26452=EDGE_LOOP('',(#70173,#70174,#70175,#70176)) ;
#26453=EDGE_LOOP('',(#70177,#70178,#70179,#70180,#70181,#70182)) ;
#26454=EDGE_LOOP('',(#70183,#70184,#70185)) ;
#26455=EDGE_LOOP('',(#70186,#70187,#70188,#70189)) ;
#26456=EDGE_LOOP('',(#70190,#70191,#70192,#70193)) ;
#26457=EDGE_LOOP('',(#70194,#70195,#70196,#70197)) ;
#26458=EDGE_LOOP('',(#70198,#70199,#70200,#70201)) ;
#26459=EDGE_LOOP('',(#70202,#70203,#70204,#70205)) ;
#26460=EDGE_LOOP('',(#70206,#70207,#70208)) ;
#26461=EDGE_LOOP('',(#70209,#70210,#70211,#70212)) ;
#26462=EDGE_LOOP('',(#70213,#70214,#70215)) ;
#26463=EDGE_LOOP('',(#70216,#70217,#70218,#70219)) ;
#26464=EDGE_LOOP('',(#70220,#70221,#70222,#70223)) ;
#26465=EDGE_LOOP('',(#70224,#70225,#70226,#70227)) ;
#26466=EDGE_LOOP('',(#70228,#70229,#70230,#70231)) ;
#26467=EDGE_LOOP('',(#70232,#70233,#70234,#70235)) ;
#26468=EDGE_LOOP('',(#70236,#70237,#70238,#70239)) ;
#26469=EDGE_LOOP('',(#70240,#70241,#70242)) ;
#26470=EDGE_LOOP('',(#70243,#70244,#70245,#70246)) ;
#26471=EDGE_LOOP('',(#70247,#70248,#70249,#70250)) ;
#26472=EDGE_LOOP('',(#70251,#70252,#70253,#70254)) ;
#26473=EDGE_LOOP('',(#70255,#70256,#70257,#70258)) ;
#26474=EDGE_LOOP('',(#70259,#70260,#70261,#70262)) ;
#26475=EDGE_LOOP('',(#70263,#70264,#70265,#70266)) ;
#26476=EDGE_LOOP('',(#70267,#70268,#70269,#70270)) ;
#26477=EDGE_LOOP('',(#70271,#70272,#70273,#70274)) ;
#26478=EDGE_LOOP('',(#70275,#70276,#70277)) ;
#26479=EDGE_LOOP('',(#70278,#70279,#70280)) ;
#26480=EDGE_LOOP('',(#70281,#70282,#70283,#70284)) ;
#26481=EDGE_LOOP('',(#70285,#70286,#70287,#70288)) ;
#26482=EDGE_LOOP('',(#70289,#70290,#70291,#70292)) ;
#26483=EDGE_LOOP('',(#70293,#70294,#70295,#70296)) ;
#26484=EDGE_LOOP('',(#70297,#70298,#70299)) ;
#26485=EDGE_LOOP('',(#70300,#70301,#70302,#70303)) ;
#26486=EDGE_LOOP('',(#70304,#70305,#70306,#70307)) ;
#26487=EDGE_LOOP('',(#70308,#70309,#70310,#70311)) ;
#26488=EDGE_LOOP('',(#70312,#70313,#70314,#70315)) ;
#26489=EDGE_LOOP('',(#70316,#70317,#70318,#70319)) ;
#26490=EDGE_LOOP('',(#70320,#70321,#70322)) ;
#26491=EDGE_LOOP('',(#70323,#70324,#70325,#70326)) ;
#26492=EDGE_LOOP('',(#70327,#70328,#70329,#70330)) ;
#26493=EDGE_LOOP('',(#70331,#70332,#70333,#70334)) ;
#26494=EDGE_LOOP('',(#70335,#70336,#70337,#70338)) ;
#26495=EDGE_LOOP('',(#70339,#70340,#70341,#70342)) ;
#26496=EDGE_LOOP('',(#70343,#70344,#70345,#70346)) ;
#26497=EDGE_LOOP('',(#70347,#70348,#70349,#70350)) ;
#26498=EDGE_LOOP('',(#70351,#70352,#70353,#70354)) ;
#26499=EDGE_LOOP('',(#70355,#70356,#70357,#70358)) ;
#26500=EDGE_LOOP('',(#70359,#70360,#70361,#70362)) ;
#26501=EDGE_LOOP('',(#70363,#70364,#70365,#70366)) ;
#26502=EDGE_LOOP('',(#70367,#70368,#70369,#70370)) ;
#26503=EDGE_LOOP('',(#70371,#70372,#70373,#70374)) ;
#26504=EDGE_LOOP('',(#70375,#70376,#70377,#70378)) ;
#26505=EDGE_LOOP('',(#70379,#70380,#70381,#70382)) ;
#26506=EDGE_LOOP('',(#70383,#70384,#70385,#70386)) ;
#26507=EDGE_LOOP('',(#70387,#70388,#70389,#70390)) ;
#26508=EDGE_LOOP('',(#70391,#70392,#70393,#70394)) ;
#26509=EDGE_LOOP('',(#70395,#70396,#70397,#70398)) ;
#26510=EDGE_LOOP('',(#70399,#70400,#70401,#70402)) ;
#26511=EDGE_LOOP('',(#70403,#70404,#70405)) ;
#26512=EDGE_LOOP('',(#70406,#70407,#70408)) ;
#26513=EDGE_LOOP('',(#70409,#70410,#70411,#70412)) ;
#26514=EDGE_LOOP('',(#70413,#70414,#70415,#70416)) ;
#26515=EDGE_LOOP('',(#70417,#70418,#70419,#70420)) ;
#26516=EDGE_LOOP('',(#70421,#70422,#70423,#70424)) ;
#26517=EDGE_LOOP('',(#70425,#70426,#70427,#70428)) ;
#26518=EDGE_LOOP('',(#70429,#70430,#70431)) ;
#26519=EDGE_LOOP('',(#70432,#70433,#70434)) ;
#26520=EDGE_LOOP('',(#70435,#70436,#70437,#70438)) ;
#26521=EDGE_LOOP('',(#70439,#70440,#70441,#70442)) ;
#26522=EDGE_LOOP('',(#70443,#70444,#70445,#70446)) ;
#26523=EDGE_LOOP('',(#70447,#70448,#70449,#70450)) ;
#26524=EDGE_LOOP('',(#70451,#70452,#70453)) ;
#26525=EDGE_LOOP('',(#70454,#70455,#70456)) ;
#26526=EDGE_LOOP('',(#70457,#70458,#70459,#70460)) ;
#26527=EDGE_LOOP('',(#70461,#70462,#70463,#70464)) ;
#26528=EDGE_LOOP('',(#70465,#70466,#70467,#70468)) ;
#26529=EDGE_LOOP('',(#70469,#70470,#70471,#70472)) ;
#26530=EDGE_LOOP('',(#70473,#70474,#70475)) ;
#26531=EDGE_LOOP('',(#70476,#70477,#70478)) ;
#26532=EDGE_LOOP('',(#70479,#70480,#70481,#70482)) ;
#26533=EDGE_LOOP('',(#70483,#70484,#70485,#70486)) ;
#26534=EDGE_LOOP('',(#70487,#70488,#70489)) ;
#26535=EDGE_LOOP('',(#70490,#70491,#70492,#70493)) ;
#26536=EDGE_LOOP('',(#70494,#70495,#70496,#70497)) ;
#26537=EDGE_LOOP('',(#70498,#70499,#70500,#70501)) ;
#26538=EDGE_LOOP('',(#70502,#70503,#70504,#70505)) ;
#26539=EDGE_LOOP('',(#70506,#70507,#70508)) ;
#26540=EDGE_LOOP('',(#70509,#70510,#70511,#70512)) ;
#26541=EDGE_LOOP('',(#70513,#70514,#70515,#70516)) ;
#26542=EDGE_LOOP('',(#70517,#70518,#70519,#70520)) ;
#26543=EDGE_LOOP('',(#70521,#70522,#70523,#70524)) ;
#26544=EDGE_LOOP('',(#70525,#70526,#70527,#70528)) ;
#26545=EDGE_LOOP('',(#70529,#70530,#70531)) ;
#26546=EDGE_LOOP('',(#70532,#70533,#70534,#70535)) ;
#26547=EDGE_LOOP('',(#70536,#70537,#70538,#70539)) ;
#26548=EDGE_LOOP('',(#70540,#70541,#70542,#70543)) ;
#26549=EDGE_LOOP('',(#70544,#70545,#70546,#70547)) ;
#26550=EDGE_LOOP('',(#70548,#70549,#70550,#70551)) ;
#26551=EDGE_LOOP('',(#70552,#70553,#70554,#70555)) ;
#26552=EDGE_LOOP('',(#70556,#70557,#70558)) ;
#26553=EDGE_LOOP('',(#70559,#70560,#70561,#70562)) ;
#26554=EDGE_LOOP('',(#70563,#70564,#70565,#70566)) ;
#26555=EDGE_LOOP('',(#70567,#70568,#70569,#70570)) ;
#26556=EDGE_LOOP('',(#70571,#70572,#70573,#70574)) ;
#26557=EDGE_LOOP('',(#70575,#70576,#70577,#70578)) ;
#26558=EDGE_LOOP('',(#70579,#70580,#70581,#70582)) ;
#26559=EDGE_LOOP('',(#70583,#70584,#70585,#70586)) ;
#26560=EDGE_LOOP('',(#70587,#70588,#70589,#70590)) ;
#26561=EDGE_LOOP('',(#70591,#70592,#70593,#70594)) ;
#26562=EDGE_LOOP('',(#70595,#70596,#70597,#70598)) ;
#26563=EDGE_LOOP('',(#70599,#70600,#70601,#70602)) ;
#26564=EDGE_LOOP('',(#70603,#70604,#70605,#70606)) ;
#26565=EDGE_LOOP('',(#70607,#70608,#70609)) ;
#26566=EDGE_LOOP('',(#70610,#70611,#70612)) ;
#26567=EDGE_LOOP('',(#70613,#70614,#70615,#70616)) ;
#26568=EDGE_LOOP('',(#70617,#70618,#70619,#70620)) ;
#26569=EDGE_LOOP('',(#70621,#70622,#70623,#70624)) ;
#26570=EDGE_LOOP('',(#70625,#70626,#70627,#70628)) ;
#26571=EDGE_LOOP('',(#70629,#70630,#70631,#70632)) ;
#26572=EDGE_LOOP('',(#70633,#70634,#70635)) ;
#26573=EDGE_LOOP('',(#70636,#70637,#70638)) ;
#26574=EDGE_LOOP('',(#70639,#70640,#70641,#70642)) ;
#26575=EDGE_LOOP('',(#70643,#70644,#70645,#70646)) ;
#26576=EDGE_LOOP('',(#70647,#70648,#70649,#70650)) ;
#26577=EDGE_LOOP('',(#70651,#70652,#70653,#70654)) ;
#26578=EDGE_LOOP('',(#70655,#70656,#70657)) ;
#26579=EDGE_LOOP('',(#70658,#70659,#70660)) ;
#26580=EDGE_LOOP('',(#70661,#70662,#70663,#70664)) ;
#26581=EDGE_LOOP('',(#70665,#70666,#70667,#70668)) ;
#26582=EDGE_LOOP('',(#70669,#70670,#70671,#70672)) ;
#26583=EDGE_LOOP('',(#70673,#70674,#70675,#70676)) ;
#26584=EDGE_LOOP('',(#70677,#70678,#70679)) ;
#26585=EDGE_LOOP('',(#70680,#70681,#70682)) ;
#26586=EDGE_LOOP('',(#70683,#70684,#70685,#70686)) ;
#26587=EDGE_LOOP('',(#70687,#70688,#70689,#70690)) ;
#26588=EDGE_LOOP('',(#70691,#70692,#70693)) ;
#26589=EDGE_LOOP('',(#70694,#70695,#70696)) ;
#26590=EDGE_LOOP('',(#70697,#70698,#70699,#70700)) ;
#26591=EDGE_LOOP('',(#70701,#70702,#70703,#70704)) ;
#26592=EDGE_LOOP('',(#70705,#70706,#70707)) ;
#26593=EDGE_LOOP('',(#70708,#70709,#70710)) ;
#26594=EDGE_LOOP('',(#70711,#70712,#70713,#70714)) ;
#26595=EDGE_LOOP('',(#70715,#70716,#70717,#70718)) ;
#26596=EDGE_LOOP('',(#70719,#70720,#70721,#70722)) ;
#26597=EDGE_LOOP('',(#70723,#70724,#70725,#70726)) ;
#26598=EDGE_LOOP('',(#70727,#70728,#70729,#70730)) ;
#26599=EDGE_LOOP('',(#70731,#70732,#70733,#70734)) ;
#26600=EDGE_LOOP('',(#70735,#70736,#70737)) ;
#26601=EDGE_LOOP('',(#70738,#70739,#70740,#70741,#70742)) ;
#26602=EDGE_LOOP('',(#70743,#70744,#70745)) ;
#26603=EDGE_LOOP('',(#70746,#70747,#70748)) ;
#26604=EDGE_LOOP('',(#70749,#70750,#70751,#70752,#70753)) ;
#26605=EDGE_LOOP('',(#70754,#70755,#70756)) ;
#26606=EDGE_LOOP('',(#70757,#70758,#70759)) ;
#26607=EDGE_LOOP('',(#70760,#70761,#70762,#70763,#70764)) ;
#26608=EDGE_LOOP('',(#70765,#70766,#70767)) ;
#26609=EDGE_LOOP('',(#70768,#70769,#70770,#70771)) ;
#26610=EDGE_LOOP('',(#70772,#70773,#70774,#70775)) ;
#26611=EDGE_LOOP('',(#70776,#70777,#70778,#70779)) ;
#26612=EDGE_LOOP('',(#70780,#70781,#70782,#70783)) ;
#26613=EDGE_LOOP('',(#70784,#70785,#70786,#70787)) ;
#26614=EDGE_LOOP('',(#70788,#70789,#70790,#70791)) ;
#26615=EDGE_LOOP('',(#70792,#70793,#70794,#70795)) ;
#26616=EDGE_LOOP('',(#70796,#70797,#70798,#70799)) ;
#26617=EDGE_LOOP('',(#70800,#70801,#70802,#70803,#70804,#70805,#70806,#70807)) ;
#26618=EDGE_LOOP('',(#70808,#70809,#70810,#70811)) ;
#26619=EDGE_LOOP('',(#70812,#70813,#70814,#70815)) ;
#26620=EDGE_LOOP('',(#70816,#70817,#70818,#70819)) ;
#26621=EDGE_LOOP('',(#70820,#70821,#70822,#70823)) ;
#26622=EDGE_LOOP('',(#70824,#70825,#70826,#70827,#70828,#70829,#70830,#70831)) ;
#26623=EDGE_LOOP('',(#70832,#70833,#70834,#70835)) ;
#26624=EDGE_LOOP('',(#70836,#70837,#70838,#70839)) ;
#26625=EDGE_LOOP('',(#70840,#70841,#70842,#70843)) ;
#26626=EDGE_LOOP('',(#70844,#70845,#70846,#70847)) ;
#26627=EDGE_LOOP('',(#70848,#70849,#70850,#70851,#70852,#70853,#70854,#70855)) ;
#26628=EDGE_LOOP('',(#70856,#70857,#70858,#70859)) ;
#26629=EDGE_LOOP('',(#70860,#70861,#70862,#70863)) ;
#26630=EDGE_LOOP('',(#70864,#70865,#70866,#70867)) ;
#26631=EDGE_LOOP('',(#70868,#70869,#70870,#70871)) ;
#26632=EDGE_LOOP('',(#70872,#70873,#70874,#70875,#70876,#70877,#70878,#70879)) ;
#26633=EDGE_LOOP('',(#70880,#70881,#70882,#70883)) ;
#26634=EDGE_LOOP('',(#70884,#70885,#70886,#70887)) ;
#26635=EDGE_LOOP('',(#70888,#70889,#70890,#70891)) ;
#26636=EDGE_LOOP('',(#70892,#70893,#70894,#70895)) ;
#26637=EDGE_LOOP('',(#70896,#70897,#70898,#70899,#70900,#70901,#70902,#70903)) ;
#26638=EDGE_LOOP('',(#70904,#70905,#70906,#70907)) ;
#26639=EDGE_LOOP('',(#70908,#70909,#70910,#70911)) ;
#26640=EDGE_LOOP('',(#70912,#70913,#70914,#70915)) ;
#26641=EDGE_LOOP('',(#70916,#70917,#70918,#70919)) ;
#26642=EDGE_LOOP('',(#70920,#70921,#70922,#70923,#70924,#70925,#70926,#70927)) ;
#26643=EDGE_LOOP('',(#70928,#70929,#70930,#70931)) ;
#26644=EDGE_LOOP('',(#70932,#70933,#70934,#70935)) ;
#26645=EDGE_LOOP('',(#70936,#70937,#70938,#70939)) ;
#26646=EDGE_LOOP('',(#70940,#70941,#70942,#70943)) ;
#26647=EDGE_LOOP('',(#70944,#70945,#70946,#70947,#70948,#70949,#70950,#70951)) ;
#26648=EDGE_LOOP('',(#70952,#70953,#70954,#70955)) ;
#26649=EDGE_LOOP('',(#70956,#70957,#70958,#70959)) ;
#26650=EDGE_LOOP('',(#70960,#70961,#70962,#70963)) ;
#26651=EDGE_LOOP('',(#70964,#70965,#70966,#70967)) ;
#26652=EDGE_LOOP('',(#70968,#70969,#70970,#70971,#70972,#70973,#70974,#70975)) ;
#26653=EDGE_LOOP('',(#70976,#70977,#70978,#70979)) ;
#26654=EDGE_LOOP('',(#70980,#70981,#70982,#70983)) ;
#26655=EDGE_LOOP('',(#70984,#70985,#70986,#70987)) ;
#26656=EDGE_LOOP('',(#70988,#70989,#70990,#70991)) ;
#26657=EDGE_LOOP('',(#70992,#70993,#70994,#70995,#70996,#70997,#70998,#70999)) ;
#26658=EDGE_LOOP('',(#71000,#71001,#71002,#71003)) ;
#26659=EDGE_LOOP('',(#71004,#71005,#71006,#71007)) ;
#26660=EDGE_LOOP('',(#71008,#71009,#71010,#71011,#71012,#71013)) ;
#26661=EDGE_LOOP('',(#71014,#71015,#71016,#71017,#71018,#71019,#71020,#71021)) ;
#26662=EDGE_LOOP('',(#71022,#71023,#71024,#71025,#71026,#71027,#71028,#71029)) ;
#26663=EDGE_LOOP('',(#71030,#71031,#71032,#71033,#71034,#71035,#71036,#71037)) ;
#26664=EDGE_LOOP('',(#71038,#71039,#71040,#71041,#71042,#71043,#71044,#71045)) ;
#26665=EDGE_LOOP('',(#71046,#71047,#71048,#71049,#71050,#71051,#71052,#71053)) ;
#26666=EDGE_LOOP('',(#71054,#71055,#71056,#71057,#71058,#71059,#71060,#71061)) ;
#26667=EDGE_LOOP('',(#71062,#71063,#71064,#71065,#71066,#71067,#71068,#71069)) ;
#26668=EDGE_LOOP('',(#71070,#71071,#71072,#71073,#71074,#71075,#71076,#71077)) ;
#26669=EDGE_LOOP('',(#71078,#71079,#71080,#71081,#71082,#71083)) ;
#26670=EDGE_LOOP('',(#71084,#71085,#71086,#71087,#71088,#71089,#71090,#71091)) ;
#26671=EDGE_LOOP('',(#71092,#71093,#71094,#71095,#71096,#71097,#71098,#71099)) ;
#26672=EDGE_LOOP('',(#71100,#71101,#71102,#71103,#71104,#71105,#71106,#71107)) ;
#26673=EDGE_LOOP('',(#71108,#71109,#71110,#71111,#71112,#71113,#71114,#71115)) ;
#26674=EDGE_LOOP('',(#71116,#71117,#71118,#71119,#71120,#71121,#71122,#71123)) ;
#26675=EDGE_LOOP('',(#71124,#71125,#71126,#71127,#71128,#71129,#71130,#71131)) ;
#26676=EDGE_LOOP('',(#71132,#71133,#71134,#71135,#71136,#71137,#71138,#71139)) ;
#26677=EDGE_LOOP('',(#71140,#71141,#71142,#71143,#71144,#71145,#71146,#71147)) ;
#26678=EDGE_LOOP('',(#71148,#71149,#71150,#71151)) ;
#26679=EDGE_LOOP('',(#71152,#71153,#71154,#71155)) ;
#26680=EDGE_LOOP('',(#71156,#71157,#71158,#71159)) ;
#26681=EDGE_LOOP('',(#71160,#71161,#71162,#71163)) ;
#26682=EDGE_LOOP('',(#71164,#71165,#71166,#71167)) ;
#26683=EDGE_LOOP('',(#71168,#71169,#71170,#71171)) ;
#26684=EDGE_LOOP('',(#71172,#71173,#71174,#71175)) ;
#26685=EDGE_LOOP('',(#71176,#71177,#71178,#71179)) ;
#26686=EDGE_LOOP('',(#71180,#71181,#71182,#71183)) ;
#26687=EDGE_LOOP('',(#71184,#71185,#71186,#71187)) ;
#26688=EDGE_LOOP('',(#71188,#71189,#71190,#71191)) ;
#26689=EDGE_LOOP('',(#71192,#71193,#71194,#71195)) ;
#26690=EDGE_LOOP('',(#71196,#71197,#71198,#71199)) ;
#26691=EDGE_LOOP('',(#71200,#71201,#71202,#71203)) ;
#26692=EDGE_LOOP('',(#71204,#71205,#71206,#71207)) ;
#26693=EDGE_LOOP('',(#71208,#71209,#71210,#71211)) ;
#26694=EDGE_LOOP('',(#71212,#71213,#71214,#71215)) ;
#26695=EDGE_LOOP('',(#71216,#71217,#71218,#71219)) ;
#26696=EDGE_LOOP('',(#71220,#71221,#71222,#71223)) ;
#26697=EDGE_LOOP('',(#71224,#71225,#71226,#71227)) ;
#26698=EDGE_LOOP('',(#71228,#71229,#71230,#71231)) ;
#26699=EDGE_LOOP('',(#71232,#71233,#71234,#71235)) ;
#26700=EDGE_LOOP('',(#71236,#71237,#71238,#71239)) ;
#26701=EDGE_LOOP('',(#71240,#71241,#71242,#71243)) ;
#26702=EDGE_LOOP('',(#71244,#71245,#71246,#71247)) ;
#26703=EDGE_LOOP('',(#71248,#71249,#71250,#71251)) ;
#26704=EDGE_LOOP('',(#71252,#71253,#71254,#71255)) ;
#26705=EDGE_LOOP('',(#71256,#71257,#71258,#71259)) ;
#26706=EDGE_LOOP('',(#71260,#71261,#71262,#71263)) ;
#26707=EDGE_LOOP('',(#71264,#71265,#71266,#71267)) ;
#26708=EDGE_LOOP('',(#71268,#71269,#71270,#71271)) ;
#26709=EDGE_LOOP('',(#71272,#71273,#71274,#71275)) ;
#26710=EDGE_LOOP('',(#71276,#71277,#71278,#71279)) ;
#26711=EDGE_LOOP('',(#71280,#71281,#71282,#71283)) ;
#26712=EDGE_LOOP('',(#71284,#71285,#71286,#71287)) ;
#26713=EDGE_LOOP('',(#71288,#71289,#71290,#71291)) ;
#26714=EDGE_LOOP('',(#71292,#71293,#71294,#71295)) ;
#26715=EDGE_LOOP('',(#71296,#71297,#71298,#71299,#71300,#71301,#71302,#71303)) ;
#26716=EDGE_LOOP('',(#71304,#71305,#71306,#71307)) ;
#26717=EDGE_LOOP('',(#71308,#71309,#71310,#71311)) ;
#26718=EDGE_LOOP('',(#71312,#71313,#71314,#71315)) ;
#26719=EDGE_LOOP('',(#71316,#71317,#71318,#71319)) ;
#26720=EDGE_LOOP('',(#71320,#71321,#71322,#71323)) ;
#26721=EDGE_LOOP('',(#71324,#71325,#71326,#71327,#71328,#71329,#71330,#71331)) ;
#26722=EDGE_LOOP('',(#71332,#71333,#71334,#71335)) ;
#26723=EDGE_LOOP('',(#71336,#71337,#71338,#71339)) ;
#26724=EDGE_LOOP('',(#71340,#71341,#71342,#71343)) ;
#26725=EDGE_LOOP('',(#71344,#71345,#71346,#71347)) ;
#26726=EDGE_LOOP('',(#71348,#71349,#71350,#71351)) ;
#26727=EDGE_LOOP('',(#71352,#71353,#71354,#71355,#71356,#71357,#71358,#71359)) ;
#26728=EDGE_LOOP('',(#71360,#71361,#71362,#71363)) ;
#26729=EDGE_LOOP('',(#71364,#71365,#71366,#71367)) ;
#26730=EDGE_LOOP('',(#71368,#71369,#71370,#71371)) ;
#26731=EDGE_LOOP('',(#71372,#71373,#71374,#71375)) ;
#26732=EDGE_LOOP('',(#71376,#71377,#71378,#71379)) ;
#26733=EDGE_LOOP('',(#71380,#71381,#71382,#71383,#71384,#71385,#71386,#71387)) ;
#26734=EDGE_LOOP('',(#71388,#71389,#71390,#71391)) ;
#26735=EDGE_LOOP('',(#71392,#71393,#71394,#71395)) ;
#26736=EDGE_LOOP('',(#71396,#71397,#71398,#71399)) ;
#26737=EDGE_LOOP('',(#71400,#71401,#71402,#71403)) ;
#26738=EDGE_LOOP('',(#71404,#71405,#71406,#71407)) ;
#26739=EDGE_LOOP('',(#71408,#71409,#71410,#71411,#71412,#71413,#71414,#71415)) ;
#26740=EDGE_LOOP('',(#71416,#71417,#71418,#71419)) ;
#26741=EDGE_LOOP('',(#71420,#71421,#71422,#71423)) ;
#26742=EDGE_LOOP('',(#71424,#71425,#71426,#71427)) ;
#26743=EDGE_LOOP('',(#71428,#71429,#71430,#71431)) ;
#26744=EDGE_LOOP('',(#71432,#71433,#71434,#71435)) ;
#26745=EDGE_LOOP('',(#71436,#71437,#71438,#71439,#71440,#71441,#71442,#71443)) ;
#26746=EDGE_LOOP('',(#71444,#71445,#71446,#71447)) ;
#26747=EDGE_LOOP('',(#71448,#71449,#71450,#71451)) ;
#26748=EDGE_LOOP('',(#71452,#71453,#71454,#71455)) ;
#26749=EDGE_LOOP('',(#71456,#71457,#71458,#71459)) ;
#26750=EDGE_LOOP('',(#71460,#71461,#71462,#71463)) ;
#26751=EDGE_LOOP('',(#71464,#71465,#71466,#71467,#71468,#71469,#71470,#71471)) ;
#26752=EDGE_LOOP('',(#71472,#71473,#71474,#71475)) ;
#26753=EDGE_LOOP('',(#71476,#71477,#71478,#71479)) ;
#26754=EDGE_LOOP('',(#71480,#71481,#71482,#71483)) ;
#26755=EDGE_LOOP('',(#71484,#71485,#71486,#71487)) ;
#26756=EDGE_LOOP('',(#71488,#71489,#71490,#71491)) ;
#26757=EDGE_LOOP('',(#71492,#71493,#71494,#71495,#71496,#71497,#71498,#71499)) ;
#26758=EDGE_LOOP('',(#71500,#71501,#71502,#71503)) ;
#26759=EDGE_LOOP('',(#71504,#71505,#71506,#71507)) ;
#26760=EDGE_LOOP('',(#71508,#71509,#71510,#71511)) ;
#26761=EDGE_LOOP('',(#71512,#71513,#71514,#71515)) ;
#26762=EDGE_LOOP('',(#71516,#71517,#71518,#71519)) ;
#26763=EDGE_LOOP('',(#71520,#71521,#71522,#71523,#71524,#71525,#71526,#71527)) ;
#26764=EDGE_LOOP('',(#71528,#71529,#71530,#71531)) ;
#26765=EDGE_LOOP('',(#71532,#71533,#71534,#71535)) ;
#26766=EDGE_LOOP('',(#71536,#71537,#71538,#71539)) ;
#26767=EDGE_LOOP('',(#71540,#71541,#71542,#71543)) ;
#26768=EDGE_LOOP('',(#71544,#71545,#71546,#71547)) ;
#26769=EDGE_LOOP('',(#71548,#71549,#71550,#71551)) ;
#26770=EDGE_LOOP('',(#71552,#71553,#71554,#71555)) ;
#26771=EDGE_LOOP('',(#71556,#71557,#71558,#71559)) ;
#26772=EDGE_LOOP('',(#71560,#71561,#71562,#71563)) ;
#26773=EDGE_LOOP('',(#71564,#71565,#71566,#71567)) ;
#26774=EDGE_LOOP('',(#71568,#71569,#71570,#71571)) ;
#26775=EDGE_LOOP('',(#71572,#71573,#71574,#71575)) ;
#26776=EDGE_LOOP('',(#71576,#71577,#71578,#71579)) ;
#26777=EDGE_LOOP('',(#71580,#71581,#71582,#71583,#71584,#71585,#71586,#71587,
#71588,#71589)) ;
#26778=EDGE_LOOP('',(#71590,#71591,#71592,#71593)) ;
#26779=EDGE_LOOP('',(#71594,#71595,#71596,#71597,#71598,#71599,#71600,#71601,
#71602,#71603)) ;
#26780=EDGE_LOOP('',(#71604,#71605,#71606,#71607)) ;
#26781=EDGE_LOOP('',(#71608,#71609,#71610,#71611,#71612,#71613,#71614,#71615,
#71616,#71617)) ;
#26782=EDGE_LOOP('',(#71618,#71619,#71620,#71621)) ;
#26783=EDGE_LOOP('',(#71622,#71623,#71624,#71625,#71626,#71627,#71628,#71629,
#71630,#71631)) ;
#26784=EDGE_LOOP('',(#71632,#71633,#71634,#71635)) ;
#26785=EDGE_LOOP('',(#71636,#71637,#71638,#71639,#71640,#71641,#71642,#71643,
#71644,#71645)) ;
#26786=EDGE_LOOP('',(#71646,#71647,#71648,#71649)) ;
#26787=EDGE_LOOP('',(#71650,#71651,#71652,#71653,#71654,#71655,#71656,#71657,
#71658,#71659)) ;
#26788=EDGE_LOOP('',(#71660,#71661,#71662,#71663)) ;
#26789=EDGE_LOOP('',(#71664,#71665,#71666,#71667,#71668,#71669,#71670,#71671,
#71672,#71673)) ;
#26790=EDGE_LOOP('',(#71674,#71675,#71676,#71677)) ;
#26791=EDGE_LOOP('',(#71678,#71679,#71680,#71681,#71682,#71683,#71684,#71685,
#71686,#71687)) ;
#26792=EDGE_LOOP('',(#71688,#71689,#71690,#71691)) ;
#26793=EDGE_LOOP('',(#71692,#71693,#71694,#71695,#71696,#71697,#71698,#71699,
#71700,#71701)) ;
#26794=EDGE_LOOP('',(#71702,#71703,#71704,#71705)) ;
#26795=EDGE_LOOP('',(#71706,#71707,#71708,#71709,#71710,#71711,#71712,#71713,
#71714,#71715)) ;
#26796=EDGE_LOOP('',(#71716,#71717,#71718,#71719)) ;
#26797=EDGE_LOOP('',(#71720,#71721,#71722,#71723,#71724,#71725,#71726,#71727,
#71728,#71729)) ;
#26798=EDGE_LOOP('',(#71730,#71731,#71732,#71733)) ;
#26799=EDGE_LOOP('',(#71734,#71735,#71736,#71737,#71738,#71739,#71740,#71741,
#71742,#71743)) ;
#26800=EDGE_LOOP('',(#71744,#71745,#71746,#71747)) ;
#26801=EDGE_LOOP('',(#71748,#71749,#71750,#71751,#71752,#71753,#71754,#71755,
#71756,#71757)) ;
#26802=EDGE_LOOP('',(#71758,#71759,#71760,#71761)) ;
#26803=EDGE_LOOP('',(#71762,#71763,#71764,#71765,#71766,#71767,#71768,#71769,
#71770,#71771)) ;
#26804=EDGE_LOOP('',(#71772,#71773,#71774,#71775)) ;
#26805=EDGE_LOOP('',(#71776,#71777,#71778,#71779,#71780,#71781,#71782,#71783,
#71784,#71785)) ;
#26806=EDGE_LOOP('',(#71786,#71787,#71788,#71789)) ;
#26807=EDGE_LOOP('',(#71790,#71791,#71792,#71793,#71794,#71795,#71796,#71797,
#71798,#71799)) ;
#26808=EDGE_LOOP('',(#71800,#71801,#71802,#71803)) ;
#26809=EDGE_LOOP('',(#71804,#71805,#71806,#71807,#71808,#71809,#71810,#71811,
#71812,#71813)) ;
#26810=EDGE_LOOP('',(#71814,#71815,#71816,#71817)) ;
#26811=EDGE_LOOP('',(#71818,#71819,#71820,#71821,#71822,#71823,#71824,#71825,
#71826,#71827)) ;
#26812=EDGE_LOOP('',(#71828,#71829,#71830,#71831)) ;
#26813=EDGE_LOOP('',(#71832,#71833,#71834,#71835)) ;
#26814=EDGE_LOOP('',(#71836,#71837,#71838,#71839)) ;
#26815=EDGE_LOOP('',(#71840,#71841,#71842,#71843)) ;
#26816=EDGE_LOOP('',(#71844,#71845,#71846,#71847,#71848,#71849)) ;
#26817=EDGE_LOOP('',(#71850)) ;
#26818=EDGE_LOOP('',(#71851,#71852,#71853,#71854)) ;
#26819=EDGE_LOOP('',(#71855,#71856,#71857,#71858)) ;
#26820=EDGE_LOOP('',(#71859,#71860,#71861,#71862)) ;
#26821=EDGE_LOOP('',(#71863,#71864,#71865,#71866,#71867,#71868)) ;
#26822=EDGE_LOOP('',(#71869)) ;
#26823=EDGE_LOOP('',(#71870,#71871,#71872,#71873)) ;
#26824=EDGE_LOOP('',(#71874,#71875,#71876,#71877)) ;
#26825=EDGE_LOOP('',(#71878,#71879,#71880,#71881)) ;
#26826=EDGE_LOOP('',(#71882,#71883,#71884,#71885,#71886,#71887)) ;
#26827=EDGE_LOOP('',(#71888)) ;
#26828=EDGE_LOOP('',(#71889,#71890,#71891,#71892)) ;
#26829=EDGE_LOOP('',(#71893,#71894,#71895,#71896)) ;
#26830=EDGE_LOOP('',(#71897,#71898,#71899,#71900)) ;
#26831=EDGE_LOOP('',(#71901,#71902,#71903,#71904,#71905,#71906)) ;
#26832=EDGE_LOOP('',(#71907)) ;
#26833=EDGE_LOOP('',(#71908,#71909,#71910,#71911)) ;
#26834=EDGE_LOOP('',(#71912,#71913,#71914,#71915)) ;
#26835=EDGE_LOOP('',(#71916,#71917,#71918,#71919)) ;
#26836=EDGE_LOOP('',(#71920,#71921,#71922,#71923,#71924,#71925)) ;
#26837=EDGE_LOOP('',(#71926)) ;
#26838=EDGE_LOOP('',(#71927,#71928,#71929,#71930)) ;
#26839=EDGE_LOOP('',(#71931,#71932,#71933,#71934)) ;
#26840=EDGE_LOOP('',(#71935,#71936,#71937,#71938)) ;
#26841=EDGE_LOOP('',(#71939,#71940,#71941,#71942,#71943,#71944)) ;
#26842=EDGE_LOOP('',(#71945)) ;
#26843=EDGE_LOOP('',(#71946,#71947,#71948,#71949)) ;
#26844=EDGE_LOOP('',(#71950,#71951,#71952,#71953)) ;
#26845=EDGE_LOOP('',(#71954,#71955,#71956,#71957)) ;
#26846=EDGE_LOOP('',(#71958,#71959,#71960,#71961,#71962,#71963)) ;
#26847=EDGE_LOOP('',(#71964)) ;
#26848=EDGE_LOOP('',(#71965,#71966,#71967,#71968)) ;
#26849=EDGE_LOOP('',(#71969,#71970,#71971,#71972)) ;
#26850=EDGE_LOOP('',(#71973,#71974,#71975,#71976)) ;
#26851=EDGE_LOOP('',(#71977,#71978,#71979,#71980,#71981,#71982)) ;
#26852=EDGE_LOOP('',(#71983)) ;
#26853=EDGE_LOOP('',(#71984,#71985,#71986,#71987)) ;
#26854=EDGE_LOOP('',(#71988,#71989,#71990,#71991)) ;
#26855=EDGE_LOOP('',(#71992,#71993,#71994,#71995)) ;
#26856=EDGE_LOOP('',(#71996,#71997,#71998,#71999,#72000,#72001)) ;
#26857=EDGE_LOOP('',(#72002)) ;
#26858=EDGE_LOOP('',(#72003)) ;
#26859=EDGE_LOOP('',(#72004)) ;
#26860=EDGE_LOOP('',(#72005)) ;
#26861=EDGE_LOOP('',(#72006)) ;
#26862=EDGE_LOOP('',(#72007)) ;
#26863=EDGE_LOOP('',(#72008)) ;
#26864=EDGE_LOOP('',(#72009)) ;
#26865=EDGE_LOOP('',(#72010)) ;
#26866=EDGE_LOOP('',(#72011)) ;
#26867=EDGE_LOOP('',(#72012,#72013,#72014,#72015)) ;
#26868=EDGE_LOOP('',(#72016,#72017,#72018,#72019)) ;
#26869=EDGE_LOOP('',(#72020,#72021,#72022,#72023)) ;
#26870=EDGE_LOOP('',(#72024,#72025,#72026,#72027)) ;
#26871=EDGE_LOOP('',(#72028,#72029,#72030,#72031)) ;
#26872=EDGE_LOOP('',(#72032,#72033,#72034,#72035)) ;
#26873=EDGE_LOOP('',(#72036,#72037,#72038,#72039)) ;
#26874=EDGE_LOOP('',(#72040,#72041,#72042,#72043)) ;
#26875=EDGE_LOOP('',(#72044,#72045,#72046,#72047)) ;
#26876=EDGE_LOOP('',(#72048,#72049,#72050,#72051)) ;
#26877=EDGE_LOOP('',(#72052,#72053,#72054,#72055)) ;
#26878=EDGE_LOOP('',(#72056,#72057,#72058,#72059)) ;
#26879=EDGE_LOOP('',(#72060,#72061,#72062,#72063)) ;
#26880=EDGE_LOOP('',(#72064,#72065,#72066,#72067)) ;
#26881=EDGE_LOOP('',(#72068,#72069,#72070,#72071)) ;
#26882=EDGE_LOOP('',(#72072,#72073,#72074,#72075)) ;
#26883=EDGE_LOOP('',(#72076,#72077,#72078,#72079)) ;
#26884=EDGE_LOOP('',(#72080,#72081,#72082,#72083)) ;
#26885=EDGE_LOOP('',(#72084,#72085,#72086,#72087)) ;
#26886=EDGE_LOOP('',(#72088,#72089,#72090,#72091)) ;
#26887=EDGE_LOOP('',(#72092,#72093,#72094,#72095)) ;
#26888=EDGE_LOOP('',(#72096,#72097,#72098,#72099)) ;
#26889=EDGE_LOOP('',(#72100,#72101,#72102,#72103)) ;
#26890=EDGE_LOOP('',(#72104,#72105,#72106,#72107)) ;
#26891=EDGE_LOOP('',(#72108,#72109,#72110,#72111)) ;
#26892=EDGE_LOOP('',(#72112,#72113,#72114,#72115)) ;
#26893=EDGE_LOOP('',(#72116,#72117,#72118,#72119)) ;
#26894=EDGE_LOOP('',(#72120,#72121,#72122,#72123)) ;
#26895=EDGE_LOOP('',(#72124,#72125,#72126,#72127)) ;
#26896=EDGE_LOOP('',(#72128,#72129,#72130,#72131)) ;
#26897=EDGE_LOOP('',(#72132,#72133,#72134,#72135)) ;
#26898=EDGE_LOOP('',(#72136,#72137,#72138,#72139)) ;
#26899=EDGE_LOOP('',(#72140,#72141,#72142,#72143)) ;
#26900=EDGE_LOOP('',(#72144,#72145,#72146,#72147)) ;
#26901=EDGE_LOOP('',(#72148,#72149,#72150,#72151)) ;
#26902=EDGE_LOOP('',(#72152,#72153,#72154,#72155)) ;
#26903=EDGE_LOOP('',(#72156,#72157,#72158,#72159)) ;
#26904=EDGE_LOOP('',(#72160,#72161,#72162,#72163,#72164,#72165,#72166,#72167)) ;
#26905=EDGE_LOOP('',(#72168,#72169,#72170,#72171)) ;
#26906=EDGE_LOOP('',(#72172,#72173,#72174,#72175)) ;
#26907=EDGE_LOOP('',(#72176,#72177,#72178,#72179)) ;
#26908=EDGE_LOOP('',(#72180,#72181,#72182,#72183)) ;
#26909=EDGE_LOOP('',(#72184,#72185,#72186,#72187)) ;
#26910=EDGE_LOOP('',(#72188,#72189,#72190,#72191,#72192,#72193,#72194,#72195)) ;
#26911=EDGE_LOOP('',(#72196,#72197,#72198,#72199)) ;
#26912=EDGE_LOOP('',(#72200,#72201,#72202,#72203)) ;
#26913=EDGE_LOOP('',(#72204,#72205,#72206,#72207)) ;
#26914=EDGE_LOOP('',(#72208,#72209,#72210,#72211)) ;
#26915=EDGE_LOOP('',(#72212,#72213,#72214,#72215)) ;
#26916=EDGE_LOOP('',(#72216,#72217,#72218,#72219,#72220,#72221,#72222,#72223)) ;
#26917=EDGE_LOOP('',(#72224,#72225,#72226,#72227)) ;
#26918=EDGE_LOOP('',(#72228,#72229,#72230,#72231)) ;
#26919=EDGE_LOOP('',(#72232,#72233,#72234,#72235)) ;
#26920=EDGE_LOOP('',(#72236,#72237,#72238,#72239)) ;
#26921=EDGE_LOOP('',(#72240,#72241,#72242,#72243)) ;
#26922=EDGE_LOOP('',(#72244,#72245,#72246,#72247,#72248,#72249,#72250,#72251)) ;
#26923=EDGE_LOOP('',(#72252,#72253,#72254,#72255)) ;
#26924=EDGE_LOOP('',(#72256,#72257,#72258,#72259)) ;
#26925=EDGE_LOOP('',(#72260,#72261,#72262,#72263)) ;
#26926=EDGE_LOOP('',(#72264,#72265,#72266,#72267)) ;
#26927=EDGE_LOOP('',(#72268,#72269,#72270,#72271)) ;
#26928=EDGE_LOOP('',(#72272,#72273,#72274,#72275,#72276,#72277,#72278,#72279)) ;
#26929=EDGE_LOOP('',(#72280,#72281,#72282,#72283)) ;
#26930=EDGE_LOOP('',(#72284,#72285,#72286,#72287)) ;
#26931=EDGE_LOOP('',(#72288,#72289,#72290,#72291)) ;
#26932=EDGE_LOOP('',(#72292,#72293,#72294,#72295)) ;
#26933=EDGE_LOOP('',(#72296,#72297,#72298,#72299)) ;
#26934=EDGE_LOOP('',(#72300,#72301,#72302,#72303,#72304,#72305,#72306,#72307)) ;
#26935=EDGE_LOOP('',(#72308,#72309,#72310,#72311)) ;
#26936=EDGE_LOOP('',(#72312,#72313,#72314,#72315)) ;
#26937=EDGE_LOOP('',(#72316,#72317,#72318,#72319)) ;
#26938=EDGE_LOOP('',(#72320,#72321,#72322,#72323)) ;
#26939=EDGE_LOOP('',(#72324,#72325,#72326,#72327)) ;
#26940=EDGE_LOOP('',(#72328,#72329,#72330,#72331,#72332,#72333,#72334,#72335)) ;
#26941=EDGE_LOOP('',(#72336,#72337,#72338,#72339)) ;
#26942=EDGE_LOOP('',(#72340,#72341,#72342,#72343)) ;
#26943=EDGE_LOOP('',(#72344,#72345,#72346,#72347)) ;
#26944=EDGE_LOOP('',(#72348,#72349,#72350,#72351)) ;
#26945=EDGE_LOOP('',(#72352,#72353,#72354,#72355)) ;
#26946=EDGE_LOOP('',(#72356,#72357,#72358,#72359,#72360,#72361,#72362,#72363)) ;
#26947=EDGE_LOOP('',(#72364,#72365,#72366,#72367)) ;
#26948=EDGE_LOOP('',(#72368,#72369,#72370,#72371)) ;
#26949=EDGE_LOOP('',(#72372,#72373,#72374,#72375)) ;
#26950=EDGE_LOOP('',(#72376,#72377,#72378,#72379)) ;
#26951=EDGE_LOOP('',(#72380,#72381,#72382,#72383)) ;
#26952=EDGE_LOOP('',(#72384,#72385,#72386,#72387,#72388,#72389,#72390,#72391)) ;
#26953=EDGE_LOOP('',(#72392,#72393,#72394,#72395)) ;
#26954=EDGE_LOOP('',(#72396,#72397,#72398,#72399)) ;
#26955=EDGE_LOOP('',(#72400,#72401,#72402,#72403)) ;
#26956=EDGE_LOOP('',(#72404,#72405,#72406,#72407)) ;
#26957=EDGE_LOOP('',(#72408,#72409,#72410,#72411)) ;
#26958=EDGE_LOOP('',(#72412,#72413,#72414,#72415)) ;
#26959=EDGE_LOOP('',(#72416,#72417,#72418,#72419)) ;
#26960=EDGE_LOOP('',(#72420,#72421,#72422,#72423)) ;
#26961=EDGE_LOOP('',(#72424,#72425,#72426,#72427)) ;
#26962=EDGE_LOOP('',(#72428,#72429,#72430,#72431)) ;
#26963=EDGE_LOOP('',(#72432,#72433,#72434,#72435)) ;
#26964=EDGE_LOOP('',(#72436,#72437,#72438,#72439)) ;
#26965=EDGE_LOOP('',(#72440,#72441,#72442,#72443)) ;
#26966=EDGE_LOOP('',(#72444,#72445,#72446)) ;
#26967=EDGE_LOOP('',(#72447,#72448,#72449)) ;
#26968=EDGE_LOOP('',(#72450,#72451,#72452)) ;
#26969=EDGE_LOOP('',(#72453,#72454,#72455)) ;
#26970=EDGE_LOOP('',(#72456,#72457,#72458)) ;
#26971=EDGE_LOOP('',(#72459,#72460,#72461)) ;
#26972=EDGE_LOOP('',(#72462,#72463,#72464)) ;
#26973=EDGE_LOOP('',(#72465,#72466,#72467)) ;
#26974=EDGE_LOOP('',(#72468,#72469,#72470)) ;
#26975=EDGE_LOOP('',(#72471,#72472,#72473,#72474)) ;
#26976=EDGE_LOOP('',(#72475,#72476,#72477,#72478)) ;
#26977=EDGE_LOOP('',(#72479,#72480,#72481,#72482)) ;
#26978=EDGE_LOOP('',(#72483,#72484,#72485,#72486)) ;
#26979=EDGE_LOOP('',(#72487,#72488,#72489,#72490)) ;
#26980=EDGE_LOOP('',(#72491,#72492,#72493,#72494)) ;
#26981=EDGE_LOOP('',(#72495,#72496,#72497,#72498)) ;
#26982=EDGE_LOOP('',(#72499,#72500,#72501,#72502)) ;
#26983=EDGE_LOOP('',(#72503,#72504,#72505,#72506)) ;
#26984=EDGE_LOOP('',(#72507,#72508,#72509,#72510)) ;
#26985=EDGE_LOOP('',(#72511,#72512,#72513,#72514)) ;
#26986=EDGE_LOOP('',(#72515,#72516,#72517,#72518)) ;
#26987=EDGE_LOOP('',(#72519,#72520,#72521,#72522)) ;
#26988=EDGE_LOOP('',(#72523,#72524,#72525,#72526)) ;
#26989=EDGE_LOOP('',(#72527,#72528,#72529,#72530)) ;
#26990=EDGE_LOOP('',(#72531,#72532,#72533,#72534)) ;
#26991=EDGE_LOOP('',(#72535,#72536,#72537,#72538)) ;
#26992=EDGE_LOOP('',(#72539,#72540,#72541,#72542)) ;
#26993=EDGE_LOOP('',(#72543,#72544,#72545,#72546)) ;
#26994=EDGE_LOOP('',(#72547,#72548,#72549,#72550)) ;
#26995=EDGE_LOOP('',(#72551,#72552,#72553,#72554)) ;
#26996=EDGE_LOOP('',(#72555,#72556,#72557,#72558)) ;
#26997=EDGE_LOOP('',(#72559,#72560,#72561,#72562)) ;
#26998=EDGE_LOOP('',(#72563,#72564,#72565,#72566)) ;
#26999=EDGE_LOOP('',(#72567,#72568,#72569,#72570)) ;
#27000=EDGE_LOOP('',(#72571,#72572,#72573,#72574)) ;
#27001=EDGE_LOOP('',(#72575,#72576,#72577,#72578)) ;
#27002=EDGE_LOOP('',(#72579,#72580,#72581,#72582)) ;
#27003=EDGE_LOOP('',(#72583,#72584,#72585,#72586)) ;
#27004=EDGE_LOOP('',(#72587,#72588,#72589,#72590)) ;
#27005=EDGE_LOOP('',(#72591,#72592,#72593,#72594)) ;
#27006=EDGE_LOOP('',(#72595,#72596,#72597,#72598)) ;
#27007=EDGE_LOOP('',(#72599,#72600,#72601,#72602)) ;
#27008=EDGE_LOOP('',(#72603,#72604,#72605,#72606)) ;
#27009=EDGE_LOOP('',(#72607,#72608,#72609,#72610)) ;
#27010=EDGE_LOOP('',(#72611,#72612,#72613,#72614)) ;
#27011=EDGE_LOOP('',(#72615,#72616,#72617,#72618)) ;
#27012=EDGE_LOOP('',(#72619,#72620,#72621,#72622)) ;
#27013=EDGE_LOOP('',(#72623,#72624,#72625,#72626)) ;
#27014=EDGE_LOOP('',(#72627,#72628,#72629,#72630)) ;
#27015=EDGE_LOOP('',(#72631,#72632,#72633,#72634)) ;
#27016=EDGE_LOOP('',(#72635,#72636,#72637,#72638)) ;
#27017=EDGE_LOOP('',(#72639,#72640,#72641,#72642)) ;
#27018=EDGE_LOOP('',(#72643,#72644,#72645,#72646)) ;
#27019=EDGE_LOOP('',(#72647,#72648,#72649,#72650)) ;
#27020=EDGE_LOOP('',(#72651,#72652,#72653,#72654)) ;
#27021=EDGE_LOOP('',(#72655,#72656,#72657,#72658)) ;
#27022=EDGE_LOOP('',(#72659,#72660,#72661,#72662)) ;
#27023=EDGE_LOOP('',(#72663,#72664,#72665,#72666)) ;
#27024=EDGE_LOOP('',(#72667,#72668,#72669,#72670)) ;
#27025=EDGE_LOOP('',(#72671,#72672,#72673,#72674)) ;
#27026=EDGE_LOOP('',(#72675,#72676,#72677,#72678)) ;
#27027=EDGE_LOOP('',(#72679,#72680,#72681,#72682)) ;
#27028=EDGE_LOOP('',(#72683,#72684,#72685,#72686)) ;
#27029=EDGE_LOOP('',(#72687,#72688,#72689,#72690)) ;
#27030=EDGE_LOOP('',(#72691,#72692,#72693,#72694)) ;
#27031=EDGE_LOOP('',(#72695,#72696,#72697,#72698)) ;
#27032=EDGE_LOOP('',(#72699,#72700,#72701,#72702)) ;
#27033=EDGE_LOOP('',(#72703,#72704,#72705,#72706)) ;
#27034=EDGE_LOOP('',(#72707,#72708,#72709,#72710)) ;
#27035=EDGE_LOOP('',(#72711,#72712,#72713,#72714)) ;
#27036=EDGE_LOOP('',(#72715,#72716,#72717,#72718)) ;
#27037=EDGE_LOOP('',(#72719,#72720,#72721,#72722)) ;
#27038=EDGE_LOOP('',(#72723,#72724,#72725,#72726)) ;
#27039=EDGE_LOOP('',(#72727,#72728,#72729,#72730)) ;
#27040=EDGE_LOOP('',(#72731,#72732,#72733,#72734)) ;
#27041=EDGE_LOOP('',(#72735,#72736,#72737,#72738)) ;
#27042=EDGE_LOOP('',(#72739,#72740,#72741,#72742)) ;
#27043=EDGE_LOOP('',(#72743,#72744,#72745,#72746)) ;
#27044=EDGE_LOOP('',(#72747,#72748,#72749,#72750)) ;
#27045=EDGE_LOOP('',(#72751,#72752,#72753,#72754)) ;
#27046=EDGE_LOOP('',(#72755,#72756,#72757,#72758)) ;
#27047=EDGE_LOOP('',(#72759,#72760,#72761,#72762)) ;
#27048=EDGE_LOOP('',(#72763,#72764,#72765,#72766)) ;
#27049=EDGE_LOOP('',(#72767,#72768,#72769,#72770)) ;
#27050=EDGE_LOOP('',(#72771,#72772,#72773,#72774)) ;
#27051=EDGE_LOOP('',(#72775,#72776,#72777,#72778)) ;
#27052=EDGE_LOOP('',(#72779,#72780,#72781,#72782)) ;
#27053=EDGE_LOOP('',(#72783,#72784,#72785,#72786)) ;
#27054=EDGE_LOOP('',(#72787,#72788,#72789,#72790)) ;
#27055=EDGE_LOOP('',(#72791,#72792,#72793,#72794)) ;
#27056=EDGE_LOOP('',(#72795,#72796,#72797,#72798)) ;
#27057=EDGE_LOOP('',(#72799,#72800,#72801,#72802)) ;
#27058=EDGE_LOOP('',(#72803,#72804,#72805,#72806)) ;
#27059=EDGE_LOOP('',(#72807,#72808,#72809,#72810)) ;
#27060=EDGE_LOOP('',(#72811,#72812,#72813,#72814)) ;
#27061=EDGE_LOOP('',(#72815,#72816,#72817,#72818)) ;
#27062=EDGE_LOOP('',(#72819,#72820,#72821,#72822)) ;
#27063=EDGE_LOOP('',(#72823,#72824,#72825,#72826)) ;
#27064=EDGE_LOOP('',(#72827,#72828,#72829,#72830)) ;
#27065=EDGE_LOOP('',(#72831,#72832,#72833,#72834)) ;
#27066=EDGE_LOOP('',(#72835,#72836,#72837,#72838)) ;
#27067=EDGE_LOOP('',(#72839,#72840,#72841,#72842)) ;
#27068=EDGE_LOOP('',(#72843,#72844,#72845,#72846)) ;
#27069=EDGE_LOOP('',(#72847,#72848,#72849,#72850)) ;
#27070=EDGE_LOOP('',(#72851,#72852,#72853,#72854)) ;
#27071=EDGE_LOOP('',(#72855,#72856,#72857,#72858)) ;
#27072=EDGE_LOOP('',(#72859,#72860,#72861,#72862)) ;
#27073=EDGE_LOOP('',(#72863,#72864,#72865,#72866)) ;
#27074=EDGE_LOOP('',(#72867,#72868,#72869,#72870)) ;
#27075=EDGE_LOOP('',(#72871,#72872,#72873,#72874)) ;
#27076=EDGE_LOOP('',(#72875,#72876,#72877,#72878)) ;
#27077=EDGE_LOOP('',(#72879,#72880,#72881,#72882)) ;
#27078=EDGE_LOOP('',(#72883,#72884,#72885,#72886)) ;
#27079=EDGE_LOOP('',(#72887,#72888,#72889,#72890)) ;
#27080=EDGE_LOOP('',(#72891,#72892,#72893,#72894)) ;
#27081=EDGE_LOOP('',(#72895,#72896,#72897,#72898)) ;
#27082=EDGE_LOOP('',(#72899,#72900,#72901,#72902)) ;
#27083=EDGE_LOOP('',(#72903,#72904,#72905)) ;
#27084=EDGE_LOOP('',(#72906,#72907,#72908,#72909)) ;
#27085=EDGE_LOOP('',(#72910,#72911,#72912,#72913)) ;
#27086=EDGE_LOOP('',(#72914,#72915,#72916,#72917)) ;
#27087=EDGE_LOOP('',(#72918,#72919,#72920,#72921)) ;
#27088=EDGE_LOOP('',(#72922,#72923,#72924,#72925)) ;
#27089=EDGE_LOOP('',(#72926,#72927,#72928)) ;
#27090=EDGE_LOOP('',(#72929,#72930,#72931,#72932)) ;
#27091=EDGE_LOOP('',(#72933,#72934,#72935)) ;
#27092=EDGE_LOOP('',(#72936,#72937,#72938,#72939)) ;
#27093=EDGE_LOOP('',(#72940,#72941,#72942,#72943)) ;
#27094=EDGE_LOOP('',(#72944,#72945,#72946,#72947)) ;
#27095=EDGE_LOOP('',(#72948,#72949,#72950,#72951)) ;
#27096=EDGE_LOOP('',(#72952,#72953,#72954,#72955)) ;
#27097=EDGE_LOOP('',(#72956,#72957,#72958,#72959)) ;
#27098=EDGE_LOOP('',(#72960,#72961,#72962)) ;
#27099=EDGE_LOOP('',(#72963,#72964,#72965,#72966)) ;
#27100=EDGE_LOOP('',(#72967,#72968,#72969,#72970)) ;
#27101=EDGE_LOOP('',(#72971,#72972,#72973,#72974)) ;
#27102=EDGE_LOOP('',(#72975,#72976,#72977,#72978)) ;
#27103=EDGE_LOOP('',(#72979,#72980,#72981,#72982)) ;
#27104=EDGE_LOOP('',(#72983,#72984,#72985,#72986)) ;
#27105=EDGE_LOOP('',(#72987,#72988,#72989,#72990)) ;
#27106=EDGE_LOOP('',(#72991,#72992,#72993,#72994)) ;
#27107=EDGE_LOOP('',(#72995,#72996,#72997)) ;
#27108=EDGE_LOOP('',(#72998,#72999,#73000)) ;
#27109=EDGE_LOOP('',(#73001,#73002,#73003,#73004)) ;
#27110=EDGE_LOOP('',(#73005,#73006,#73007,#73008)) ;
#27111=EDGE_LOOP('',(#73009,#73010,#73011,#73012)) ;
#27112=EDGE_LOOP('',(#73013,#73014,#73015,#73016)) ;
#27113=EDGE_LOOP('',(#73017,#73018,#73019)) ;
#27114=EDGE_LOOP('',(#73020,#73021,#73022,#73023)) ;
#27115=EDGE_LOOP('',(#73024,#73025,#73026,#73027)) ;
#27116=EDGE_LOOP('',(#73028,#73029,#73030,#73031)) ;
#27117=EDGE_LOOP('',(#73032,#73033,#73034,#73035)) ;
#27118=EDGE_LOOP('',(#73036,#73037,#73038)) ;
#27119=EDGE_LOOP('',(#73039,#73040,#73041,#73042)) ;
#27120=EDGE_LOOP('',(#73043,#73044,#73045,#73046)) ;
#27121=EDGE_LOOP('',(#73047,#73048,#73049,#73050)) ;
#27122=EDGE_LOOP('',(#73051,#73052,#73053,#73054)) ;
#27123=EDGE_LOOP('',(#73055,#73056,#73057,#73058)) ;
#27124=EDGE_LOOP('',(#73059,#73060,#73061,#73062)) ;
#27125=EDGE_LOOP('',(#73063,#73064,#73065,#73066)) ;
#27126=EDGE_LOOP('',(#73067,#73068,#73069,#73070)) ;
#27127=EDGE_LOOP('',(#73071,#73072,#73073,#73074)) ;
#27128=EDGE_LOOP('',(#73075,#73076,#73077,#73078)) ;
#27129=EDGE_LOOP('',(#73079,#73080,#73081,#73082,#73083,#73084)) ;
#27130=EDGE_LOOP('',(#73085,#73086,#73087,#73088,#73089,#73090)) ;
#27131=EDGE_LOOP('',(#73091,#73092,#73093,#73094,#73095,#73096)) ;
#27132=EDGE_LOOP('',(#73097,#73098,#73099,#73100,#73101,#73102)) ;
#27133=EDGE_LOOP('',(#73103,#73104,#73105,#73106,#73107,#73108)) ;
#27134=EDGE_LOOP('',(#73109,#73110,#73111,#73112,#73113,#73114)) ;
#27135=EDGE_LOOP('',(#73115,#73116,#73117,#73118,#73119,#73120)) ;
#27136=EDGE_LOOP('',(#73121,#73122,#73123,#73124,#73125,#73126)) ;
#27137=EDGE_LOOP('',(#73127,#73128,#73129,#73130,#73131,#73132)) ;
#27138=EDGE_LOOP('',(#73133,#73134,#73135,#73136,#73137,#73138)) ;
#27139=EDGE_LOOP('',(#73139,#73140,#73141,#73142,#73143,#73144)) ;
#27140=EDGE_LOOP('',(#73145,#73146,#73147,#73148,#73149,#73150)) ;
#27141=EDGE_LOOP('',(#73151,#73152,#73153,#73154,#73155,#73156)) ;
#27142=EDGE_LOOP('',(#73157,#73158,#73159,#73160,#73161,#73162)) ;
#27143=EDGE_LOOP('',(#73163,#73164,#73165,#73166,#73167,#73168)) ;
#27144=EDGE_LOOP('',(#73169,#73170,#73171,#73172,#73173,#73174)) ;
#27145=EDGE_LOOP('',(#73175,#73176,#73177,#73178,#73179,#73180)) ;
#27146=EDGE_LOOP('',(#73181,#73182,#73183,#73184,#73185,#73186)) ;
#27147=EDGE_LOOP('',(#73187,#73188,#73189,#73190,#73191,#73192)) ;
#27148=EDGE_LOOP('',(#73193,#73194,#73195,#73196,#73197,#73198)) ;
#27149=EDGE_LOOP('',(#73199,#73200,#73201,#73202,#73203,#73204)) ;
#27150=EDGE_LOOP('',(#73205,#73206,#73207,#73208,#73209,#73210)) ;
#27151=EDGE_LOOP('',(#73211,#73212,#73213,#73214,#73215,#73216)) ;
#27152=EDGE_LOOP('',(#73217,#73218,#73219,#73220,#73221,#73222)) ;
#27153=EDGE_LOOP('',(#73223,#73224,#73225,#73226,#73227,#73228)) ;
#27154=EDGE_LOOP('',(#73229,#73230,#73231,#73232,#73233,#73234)) ;
#27155=EDGE_LOOP('',(#73235,#73236,#73237,#73238,#73239,#73240)) ;
#27156=EDGE_LOOP('',(#73241,#73242,#73243,#73244,#73245,#73246)) ;
#27157=EDGE_LOOP('',(#73247,#73248,#73249,#73250,#73251,#73252)) ;
#27158=EDGE_LOOP('',(#73253,#73254,#73255,#73256,#73257,#73258)) ;
#27159=EDGE_LOOP('',(#73259,#73260,#73261,#73262,#73263,#73264)) ;
#27160=EDGE_LOOP('',(#73265,#73266,#73267,#73268,#73269,#73270)) ;
#27161=EDGE_LOOP('',(#73271,#73272,#73273,#73274)) ;
#27162=EDGE_LOOP('',(#73275,#73276,#73277,#73278)) ;
#27163=EDGE_LOOP('',(#73279,#73280,#73281,#73282)) ;
#27164=EDGE_LOOP('',(#73283,#73284,#73285,#73286)) ;
#27165=EDGE_LOOP('',(#73287,#73288,#73289,#73290)) ;
#27166=EDGE_LOOP('',(#73291,#73292,#73293,#73294)) ;
#27167=EDGE_LOOP('',(#73295,#73296,#73297,#73298)) ;
#27168=EDGE_LOOP('',(#73299,#73300,#73301,#73302)) ;
#27169=EDGE_LOOP('',(#73303,#73304,#73305,#73306)) ;
#27170=EDGE_LOOP('',(#73307,#73308,#73309,#73310)) ;
#27171=EDGE_LOOP('',(#73311,#73312,#73313)) ;
#27172=EDGE_LOOP('',(#73314,#73315,#73316)) ;
#27173=EDGE_LOOP('',(#73317,#73318,#73319,#73320)) ;
#27174=EDGE_LOOP('',(#73321,#73322,#73323,#73324)) ;
#27175=EDGE_LOOP('',(#73325,#73326,#73327,#73328)) ;
#27176=EDGE_LOOP('',(#73329,#73330,#73331,#73332)) ;
#27177=EDGE_LOOP('',(#73333,#73334,#73335,#73336)) ;
#27178=EDGE_LOOP('',(#73337,#73338,#73339)) ;
#27179=EDGE_LOOP('',(#73340,#73341,#73342)) ;
#27180=EDGE_LOOP('',(#73343,#73344,#73345,#73346)) ;
#27181=EDGE_LOOP('',(#73347,#73348,#73349,#73350)) ;
#27182=EDGE_LOOP('',(#73351,#73352,#73353,#73354)) ;
#27183=EDGE_LOOP('',(#73355,#73356,#73357,#73358)) ;
#27184=EDGE_LOOP('',(#73359,#73360,#73361)) ;
#27185=EDGE_LOOP('',(#73362,#73363,#73364)) ;
#27186=EDGE_LOOP('',(#73365,#73366,#73367,#73368)) ;
#27187=EDGE_LOOP('',(#73369,#73370,#73371,#73372)) ;
#27188=EDGE_LOOP('',(#73373,#73374,#73375,#73376)) ;
#27189=EDGE_LOOP('',(#73377,#73378,#73379,#73380)) ;
#27190=EDGE_LOOP('',(#73381,#73382,#73383)) ;
#27191=EDGE_LOOP('',(#73384,#73385,#73386)) ;
#27192=EDGE_LOOP('',(#73387,#73388,#73389,#73390)) ;
#27193=EDGE_LOOP('',(#73391,#73392,#73393,#73394)) ;
#27194=EDGE_LOOP('',(#73395,#73396,#73397)) ;
#27195=EDGE_LOOP('',(#73398,#73399,#73400,#73401)) ;
#27196=EDGE_LOOP('',(#73402,#73403,#73404,#73405)) ;
#27197=EDGE_LOOP('',(#73406,#73407,#73408,#73409)) ;
#27198=EDGE_LOOP('',(#73410,#73411,#73412,#73413)) ;
#27199=EDGE_LOOP('',(#73414,#73415,#73416)) ;
#27200=EDGE_LOOP('',(#73417,#73418,#73419,#73420)) ;
#27201=EDGE_LOOP('',(#73421,#73422,#73423,#73424)) ;
#27202=EDGE_LOOP('',(#73425,#73426,#73427,#73428)) ;
#27203=EDGE_LOOP('',(#73429,#73430,#73431,#73432)) ;
#27204=EDGE_LOOP('',(#73433,#73434,#73435,#73436)) ;
#27205=EDGE_LOOP('',(#73437,#73438,#73439)) ;
#27206=EDGE_LOOP('',(#73440,#73441,#73442,#73443)) ;
#27207=EDGE_LOOP('',(#73444,#73445,#73446,#73447)) ;
#27208=EDGE_LOOP('',(#73448,#73449,#73450,#73451)) ;
#27209=EDGE_LOOP('',(#73452,#73453,#73454,#73455)) ;
#27210=EDGE_LOOP('',(#73456,#73457,#73458,#73459)) ;
#27211=EDGE_LOOP('',(#73460,#73461,#73462,#73463)) ;
#27212=EDGE_LOOP('',(#73464,#73465,#73466)) ;
#27213=EDGE_LOOP('',(#73467,#73468,#73469,#73470)) ;
#27214=EDGE_LOOP('',(#73471,#73472,#73473,#73474)) ;
#27215=EDGE_LOOP('',(#73475,#73476,#73477,#73478,#73479,#73480,#73481)) ;
#27216=EDGE_LOOP('',(#73482,#73483,#73484,#73485,#73486,#73487)) ;
#27217=EDGE_LOOP('',(#73488,#73489,#73490,#73491)) ;
#27218=EDGE_LOOP('',(#73492,#73493,#73494,#73495,#73496,#73497,#73498)) ;
#27219=EDGE_LOOP('',(#73499,#73500,#73501,#73502,#73503,#73504,#73505)) ;
#27220=EDGE_LOOP('',(#73506,#73507,#73508,#73509,#73510,#73511)) ;
#27221=EDGE_LOOP('',(#73512,#73513,#73514,#73515)) ;
#27222=EDGE_LOOP('',(#73516,#73517,#73518,#73519,#73520,#73521,#73522)) ;
#27223=EDGE_LOOP('',(#73523,#73524,#73525,#73526,#73527,#73528,#73529)) ;
#27224=EDGE_LOOP('',(#73530,#73531,#73532,#73533,#73534,#73535)) ;
#27225=EDGE_LOOP('',(#73536,#73537,#73538,#73539)) ;
#27226=EDGE_LOOP('',(#73540,#73541,#73542,#73543,#73544,#73545,#73546)) ;
#27227=EDGE_LOOP('',(#73547,#73548,#73549,#73550,#73551,#73552,#73553)) ;
#27228=EDGE_LOOP('',(#73554,#73555,#73556,#73557,#73558,#73559)) ;
#27229=EDGE_LOOP('',(#73560,#73561,#73562,#73563)) ;
#27230=EDGE_LOOP('',(#73564,#73565,#73566,#73567,#73568,#73569,#73570)) ;
#27231=EDGE_LOOP('',(#73571,#73572,#73573,#73574,#73575,#73576,#73577)) ;
#27232=EDGE_LOOP('',(#73578,#73579,#73580,#73581,#73582,#73583)) ;
#27233=EDGE_LOOP('',(#73584,#73585,#73586,#73587)) ;
#27234=EDGE_LOOP('',(#73588,#73589,#73590,#73591,#73592,#73593,#73594)) ;
#27235=EDGE_LOOP('',(#73595,#73596,#73597,#73598,#73599,#73600,#73601)) ;
#27236=EDGE_LOOP('',(#73602,#73603,#73604,#73605,#73606,#73607)) ;
#27237=EDGE_LOOP('',(#73608,#73609,#73610,#73611)) ;
#27238=EDGE_LOOP('',(#73612,#73613,#73614,#73615,#73616,#73617,#73618)) ;
#27239=EDGE_LOOP('',(#73619,#73620,#73621,#73622,#73623,#73624,#73625)) ;
#27240=EDGE_LOOP('',(#73626,#73627,#73628,#73629,#73630,#73631)) ;
#27241=EDGE_LOOP('',(#73632,#73633,#73634,#73635)) ;
#27242=EDGE_LOOP('',(#73636,#73637,#73638,#73639,#73640,#73641,#73642)) ;
#27243=EDGE_LOOP('',(#73643,#73644,#73645,#73646,#73647,#73648,#73649)) ;
#27244=EDGE_LOOP('',(#73650,#73651,#73652,#73653,#73654,#73655)) ;
#27245=EDGE_LOOP('',(#73656,#73657,#73658,#73659)) ;
#27246=EDGE_LOOP('',(#73660,#73661,#73662,#73663,#73664,#73665,#73666)) ;
#27247=EDGE_LOOP('',(#73667,#73668,#73669,#73670)) ;
#27248=EDGE_LOOP('',(#73671,#73672,#73673,#73674)) ;
#27249=EDGE_LOOP('',(#73675,#73676,#73677,#73678)) ;
#27250=EDGE_LOOP('',(#73679,#73680,#73681,#73682)) ;
#27251=EDGE_LOOP('',(#73683,#73684,#73685,#73686)) ;
#27252=EDGE_LOOP('',(#73687,#73688,#73689,#73690)) ;
#27253=EDGE_LOOP('',(#73691,#73692,#73693,#73694)) ;
#27254=EDGE_LOOP('',(#73695,#73696,#73697,#73698)) ;
#27255=EDGE_LOOP('',(#73699,#73700,#73701,#73702)) ;
#27256=EDGE_LOOP('',(#73703,#73704,#73705,#73706)) ;
#27257=EDGE_LOOP('',(#73707,#73708,#73709)) ;
#27258=EDGE_LOOP('',(#73710,#73711,#73712)) ;
#27259=EDGE_LOOP('',(#73713,#73714,#73715,#73716)) ;
#27260=EDGE_LOOP('',(#73717,#73718,#73719,#73720)) ;
#27261=EDGE_LOOP('',(#73721,#73722,#73723,#73724)) ;
#27262=EDGE_LOOP('',(#73725,#73726,#73727,#73728)) ;
#27263=EDGE_LOOP('',(#73729,#73730,#73731,#73732)) ;
#27264=EDGE_LOOP('',(#73733,#73734,#73735)) ;
#27265=EDGE_LOOP('',(#73736,#73737,#73738)) ;
#27266=EDGE_LOOP('',(#73739,#73740,#73741,#73742)) ;
#27267=EDGE_LOOP('',(#73743,#73744,#73745,#73746)) ;
#27268=EDGE_LOOP('',(#73747,#73748,#73749,#73750)) ;
#27269=EDGE_LOOP('',(#73751,#73752,#73753,#73754)) ;
#27270=EDGE_LOOP('',(#73755,#73756,#73757)) ;
#27271=EDGE_LOOP('',(#73758,#73759,#73760)) ;
#27272=EDGE_LOOP('',(#73761,#73762,#73763,#73764)) ;
#27273=EDGE_LOOP('',(#73765,#73766,#73767,#73768)) ;
#27274=EDGE_LOOP('',(#73769,#73770,#73771,#73772)) ;
#27275=EDGE_LOOP('',(#73773,#73774,#73775,#73776)) ;
#27276=EDGE_LOOP('',(#73777,#73778,#73779)) ;
#27277=EDGE_LOOP('',(#73780,#73781,#73782)) ;
#27278=EDGE_LOOP('',(#73783,#73784,#73785,#73786)) ;
#27279=EDGE_LOOP('',(#73787,#73788,#73789,#73790)) ;
#27280=EDGE_LOOP('',(#73791,#73792,#73793)) ;
#27281=EDGE_LOOP('',(#73794,#73795,#73796)) ;
#27282=EDGE_LOOP('',(#73797,#73798,#73799,#73800)) ;
#27283=EDGE_LOOP('',(#73801,#73802,#73803,#73804)) ;
#27284=EDGE_LOOP('',(#73805,#73806,#73807)) ;
#27285=EDGE_LOOP('',(#73808,#73809,#73810)) ;
#27286=EDGE_LOOP('',(#73811,#73812,#73813,#73814)) ;
#27287=EDGE_LOOP('',(#73815,#73816,#73817,#73818)) ;
#27288=EDGE_LOOP('',(#73819,#73820,#73821,#73822)) ;
#27289=EDGE_LOOP('',(#73823,#73824,#73825,#73826)) ;
#27290=EDGE_LOOP('',(#73827,#73828,#73829,#73830)) ;
#27291=EDGE_LOOP('',(#73831,#73832,#73833)) ;
#27292=EDGE_LOOP('',(#73834,#73835,#73836,#73837)) ;
#27293=EDGE_LOOP('',(#73838,#73839,#73840,#73841)) ;
#27294=EDGE_LOOP('',(#73842,#73843,#73844,#73845)) ;
#27295=EDGE_LOOP('',(#73846,#73847,#73848,#73849)) ;
#27296=EDGE_LOOP('',(#73850,#73851,#73852)) ;
#27297=EDGE_LOOP('',(#73853,#73854,#73855,#73856)) ;
#27298=EDGE_LOOP('',(#73857,#73858,#73859)) ;
#27299=EDGE_LOOP('',(#73860,#73861,#73862,#73863)) ;
#27300=EDGE_LOOP('',(#73864,#73865,#73866,#73867)) ;
#27301=EDGE_LOOP('',(#73868,#73869,#73870,#73871)) ;
#27302=EDGE_LOOP('',(#73872,#73873,#73874,#73875)) ;
#27303=EDGE_LOOP('',(#73876,#73877,#73878,#73879)) ;
#27304=EDGE_LOOP('',(#73880,#73881,#73882,#73883)) ;
#27305=EDGE_LOOP('',(#73884,#73885,#73886,#73887)) ;
#27306=EDGE_LOOP('',(#73888,#73889,#73890,#73891)) ;
#27307=EDGE_LOOP('',(#73892,#73893,#73894,#73895)) ;
#27308=EDGE_LOOP('',(#73896,#73897,#73898)) ;
#27309=EDGE_LOOP('',(#73899,#73900,#73901,#73902)) ;
#27310=EDGE_LOOP('',(#73903,#73904,#73905,#73906)) ;
#27311=EDGE_LOOP('',(#73907,#73908,#73909,#73910)) ;
#27312=EDGE_LOOP('',(#73911,#73912,#73913,#73914)) ;
#27313=EDGE_LOOP('',(#73915,#73916,#73917)) ;
#27314=EDGE_LOOP('',(#73918,#73919,#73920)) ;
#27315=EDGE_LOOP('',(#73921,#73922,#73923,#73924)) ;
#27316=EDGE_LOOP('',(#73925,#73926,#73927,#73928)) ;
#27317=EDGE_LOOP('',(#73929,#73930,#73931,#73932)) ;
#27318=EDGE_LOOP('',(#73933,#73934,#73935,#73936)) ;
#27319=EDGE_LOOP('',(#73937,#73938,#73939,#73940)) ;
#27320=EDGE_LOOP('',(#73941,#73942,#73943,#73944)) ;
#27321=EDGE_LOOP('',(#73945,#73946,#73947)) ;
#27322=EDGE_LOOP('',(#73948,#73949,#73950,#73951)) ;
#27323=EDGE_LOOP('',(#73952,#73953,#73954,#73955)) ;
#27324=EDGE_LOOP('',(#73956,#73957,#73958,#73959)) ;
#27325=EDGE_LOOP('',(#73960,#73961,#73962,#73963)) ;
#27326=EDGE_LOOP('',(#73964,#73965,#73966,#73967)) ;
#27327=EDGE_LOOP('',(#73968,#73969,#73970)) ;
#27328=EDGE_LOOP('',(#73971,#73972,#73973,#73974)) ;
#27329=EDGE_LOOP('',(#73975,#73976,#73977,#73978,#73979)) ;
#27330=EDGE_LOOP('',(#73980,#73981,#73982,#73983)) ;
#27331=EDGE_LOOP('',(#73984,#73985,#73986,#73987,#73988)) ;
#27332=EDGE_LOOP('',(#73989,#73990,#73991)) ;
#27333=EDGE_LOOP('',(#73992,#73993,#73994,#73995,#73996)) ;
#27334=EDGE_LOOP('',(#73997,#73998,#73999,#74000)) ;
#27335=EDGE_LOOP('',(#74001,#74002,#74003,#74004)) ;
#27336=EDGE_LOOP('',(#74005,#74006,#74007,#74008)) ;
#27337=EDGE_LOOP('',(#74009,#74010,#74011,#74012)) ;
#27338=EDGE_LOOP('',(#74013,#74014,#74015)) ;
#27339=EDGE_LOOP('',(#74016,#74017,#74018)) ;
#27340=EDGE_LOOP('',(#74019,#74020,#74021,#74022)) ;
#27341=EDGE_LOOP('',(#74023,#74024,#74025,#74026)) ;
#27342=EDGE_LOOP('',(#74027,#74028,#74029)) ;
#27343=EDGE_LOOP('',(#74030,#74031,#74032,#74033)) ;
#27344=EDGE_LOOP('',(#74034,#74035,#74036,#74037,#74038)) ;
#27345=EDGE_LOOP('',(#74039,#74040,#74041,#74042,#74043)) ;
#27346=EDGE_LOOP('',(#74044,#74045,#74046,#74047)) ;
#27347=EDGE_LOOP('',(#74048,#74049,#74050,#74051)) ;
#27348=EDGE_LOOP('',(#74052,#74053,#74054,#74055)) ;
#27349=EDGE_LOOP('',(#74056,#74057,#74058)) ;
#27350=EDGE_LOOP('',(#74059,#74060,#74061,#74062)) ;
#27351=EDGE_LOOP('',(#74063,#74064,#74065,#74066)) ;
#27352=EDGE_LOOP('',(#74067,#74068,#74069)) ;
#27353=EDGE_LOOP('',(#74070,#74071,#74072,#74073)) ;
#27354=EDGE_LOOP('',(#74074,#74075,#74076,#74077)) ;
#27355=EDGE_LOOP('',(#74078,#74079,#74080)) ;
#27356=EDGE_LOOP('',(#74081,#74082,#74083)) ;
#27357=EDGE_LOOP('',(#74084,#74085,#74086,#74087)) ;
#27358=EDGE_LOOP('',(#74088,#74089,#74090,#74091)) ;
#27359=EDGE_LOOP('',(#74092,#74093,#74094,#74095)) ;
#27360=EDGE_LOOP('',(#74096,#74097,#74098)) ;
#27361=EDGE_LOOP('',(#74099,#74100,#74101,#74102)) ;
#27362=EDGE_LOOP('',(#74103,#74104,#74105,#74106)) ;
#27363=EDGE_LOOP('',(#74107,#74108,#74109)) ;
#27364=EDGE_LOOP('',(#74110,#74111,#74112,#74113)) ;
#27365=EDGE_LOOP('',(#74114,#74115,#74116,#74117)) ;
#27366=EDGE_LOOP('',(#74118,#74119,#74120,#74121,#74122)) ;
#27367=EDGE_LOOP('',(#74123,#74124,#74125,#74126)) ;
#27368=EDGE_LOOP('',(#74127,#74128,#74129,#74130)) ;
#27369=EDGE_LOOP('',(#74131,#74132,#74133,#74134)) ;
#27370=EDGE_LOOP('',(#74135,#74136,#74137,#74138)) ;
#27371=EDGE_LOOP('',(#74139,#74140,#74141,#74142)) ;
#27372=EDGE_LOOP('',(#74143,#74144,#74145,#74146)) ;
#27373=EDGE_LOOP('',(#74147,#74148,#74149,#74150)) ;
#27374=EDGE_LOOP('',(#74151,#74152,#74153,#74154)) ;
#27375=EDGE_LOOP('',(#74155,#74156,#74157,#74158)) ;
#27376=EDGE_LOOP('',(#74159,#74160,#74161,#74162)) ;
#27377=EDGE_LOOP('',(#74163,#74164,#74165,#74166)) ;
#27378=EDGE_LOOP('',(#74167,#74168,#74169)) ;
#27379=EDGE_LOOP('',(#74170,#74171,#74172)) ;
#27380=EDGE_LOOP('',(#74173,#74174,#74175,#74176)) ;
#27381=EDGE_LOOP('',(#74177,#74178,#74179,#74180)) ;
#27382=EDGE_LOOP('',(#74181,#74182,#74183,#74184)) ;
#27383=EDGE_LOOP('',(#74185,#74186,#74187,#74188)) ;
#27384=EDGE_LOOP('',(#74189,#74190,#74191)) ;
#27385=EDGE_LOOP('',(#74192,#74193,#74194)) ;
#27386=EDGE_LOOP('',(#74195,#74196,#74197,#74198)) ;
#27387=EDGE_LOOP('',(#74199,#74200,#74201,#74202)) ;
#27388=EDGE_LOOP('',(#74203,#74204,#74205,#74206)) ;
#27389=EDGE_LOOP('',(#74207,#74208,#74209,#74210)) ;
#27390=EDGE_LOOP('',(#74211,#74212,#74213,#74214)) ;
#27391=EDGE_LOOP('',(#74215,#74216,#74217,#74218)) ;
#27392=EDGE_LOOP('',(#74219,#74220,#74221,#74222)) ;
#27393=EDGE_LOOP('',(#74223,#74224,#74225,#74226)) ;
#27394=EDGE_LOOP('',(#74227,#74228,#74229,#74230)) ;
#27395=EDGE_LOOP('',(#74231,#74232,#74233,#74234)) ;
#27396=EDGE_LOOP('',(#74235,#74236,#74237,#74238)) ;
#27397=EDGE_LOOP('',(#74239,#74240,#74241)) ;
#27398=EDGE_LOOP('',(#74242,#74243,#74244)) ;
#27399=EDGE_LOOP('',(#74245,#74246,#74247,#74248)) ;
#27400=EDGE_LOOP('',(#74249,#74250,#74251,#74252)) ;
#27401=EDGE_LOOP('',(#74253,#74254,#74255,#74256)) ;
#27402=EDGE_LOOP('',(#74257,#74258,#74259,#74260)) ;
#27403=EDGE_LOOP('',(#74261,#74262,#74263,#74264)) ;
#27404=EDGE_LOOP('',(#74265,#74266,#74267)) ;
#27405=EDGE_LOOP('',(#74268,#74269,#74270)) ;
#27406=EDGE_LOOP('',(#74271,#74272,#74273,#74274)) ;
#27407=EDGE_LOOP('',(#74275,#74276,#74277,#74278)) ;
#27408=EDGE_LOOP('',(#74279,#74280,#74281,#74282)) ;
#27409=EDGE_LOOP('',(#74283,#74284,#74285,#74286)) ;
#27410=EDGE_LOOP('',(#74287,#74288,#74289)) ;
#27411=EDGE_LOOP('',(#74290,#74291,#74292)) ;
#27412=EDGE_LOOP('',(#74293,#74294,#74295,#74296)) ;
#27413=EDGE_LOOP('',(#74297,#74298,#74299,#74300)) ;
#27414=EDGE_LOOP('',(#74301,#74302,#74303,#74304)) ;
#27415=EDGE_LOOP('',(#74305,#74306,#74307,#74308)) ;
#27416=EDGE_LOOP('',(#74309,#74310,#74311)) ;
#27417=EDGE_LOOP('',(#74312,#74313,#74314)) ;
#27418=EDGE_LOOP('',(#74315,#74316,#74317,#74318)) ;
#27419=EDGE_LOOP('',(#74319,#74320,#74321,#74322)) ;
#27420=EDGE_LOOP('',(#74323,#74324,#74325)) ;
#27421=EDGE_LOOP('',(#74326,#74327,#74328)) ;
#27422=EDGE_LOOP('',(#74329,#74330,#74331,#74332)) ;
#27423=EDGE_LOOP('',(#74333,#74334,#74335,#74336)) ;
#27424=EDGE_LOOP('',(#74337,#74338,#74339)) ;
#27425=EDGE_LOOP('',(#74340,#74341,#74342)) ;
#27426=EDGE_LOOP('',(#74343,#74344,#74345,#74346)) ;
#27427=EDGE_LOOP('',(#74347,#74348,#74349,#74350)) ;
#27428=EDGE_LOOP('',(#74351,#74352,#74353,#74354)) ;
#27429=EDGE_LOOP('',(#74355,#74356,#74357,#74358)) ;
#27430=EDGE_LOOP('',(#74359,#74360,#74361,#74362)) ;
#27431=EDGE_LOOP('',(#74363,#74364,#74365)) ;
#27432=EDGE_LOOP('',(#74366,#74367,#74368,#74369)) ;
#27433=EDGE_LOOP('',(#74370,#74371,#74372,#74373)) ;
#27434=EDGE_LOOP('',(#74374,#74375,#74376,#74377)) ;
#27435=EDGE_LOOP('',(#74378,#74379,#74380,#74381)) ;
#27436=EDGE_LOOP('',(#74382,#74383,#74384)) ;
#27437=EDGE_LOOP('',(#74385,#74386,#74387,#74388)) ;
#27438=EDGE_LOOP('',(#74389,#74390,#74391)) ;
#27439=EDGE_LOOP('',(#74392,#74393,#74394,#74395)) ;
#27440=EDGE_LOOP('',(#74396,#74397,#74398,#74399)) ;
#27441=EDGE_LOOP('',(#74400,#74401,#74402,#74403)) ;
#27442=EDGE_LOOP('',(#74404,#74405,#74406,#74407)) ;
#27443=EDGE_LOOP('',(#74408,#74409,#74410,#74411)) ;
#27444=EDGE_LOOP('',(#74412,#74413,#74414,#74415)) ;
#27445=EDGE_LOOP('',(#74416,#74417,#74418,#74419)) ;
#27446=EDGE_LOOP('',(#74420,#74421,#74422,#74423)) ;
#27447=EDGE_LOOP('',(#74424,#74425,#74426,#74427)) ;
#27448=EDGE_LOOP('',(#74428,#74429,#74430)) ;
#27449=EDGE_LOOP('',(#74431,#74432,#74433,#74434)) ;
#27450=EDGE_LOOP('',(#74435,#74436,#74437,#74438)) ;
#27451=EDGE_LOOP('',(#74439,#74440,#74441,#74442)) ;
#27452=EDGE_LOOP('',(#74443,#74444,#74445,#74446)) ;
#27453=EDGE_LOOP('',(#74447,#74448,#74449)) ;
#27454=EDGE_LOOP('',(#74450,#74451,#74452)) ;
#27455=EDGE_LOOP('',(#74453,#74454,#74455,#74456)) ;
#27456=EDGE_LOOP('',(#74457,#74458,#74459,#74460)) ;
#27457=EDGE_LOOP('',(#74461,#74462,#74463,#74464)) ;
#27458=EDGE_LOOP('',(#74465,#74466,#74467,#74468)) ;
#27459=EDGE_LOOP('',(#74469,#74470,#74471,#74472)) ;
#27460=EDGE_LOOP('',(#74473,#74474,#74475,#74476)) ;
#27461=EDGE_LOOP('',(#74477,#74478,#74479)) ;
#27462=EDGE_LOOP('',(#74480,#74481,#74482,#74483)) ;
#27463=EDGE_LOOP('',(#74484,#74485,#74486,#74487)) ;
#27464=EDGE_LOOP('',(#74488,#74489,#74490,#74491)) ;
#27465=EDGE_LOOP('',(#74492,#74493,#74494,#74495)) ;
#27466=EDGE_LOOP('',(#74496,#74497,#74498,#74499)) ;
#27467=EDGE_LOOP('',(#74500,#74501,#74502)) ;
#27468=EDGE_LOOP('',(#74503,#74504,#74505,#74506)) ;
#27469=EDGE_LOOP('',(#74507,#74508,#74509,#74510,#74511)) ;
#27470=EDGE_LOOP('',(#74512,#74513,#74514,#74515)) ;
#27471=EDGE_LOOP('',(#74516,#74517,#74518,#74519,#74520)) ;
#27472=EDGE_LOOP('',(#74521,#74522,#74523)) ;
#27473=EDGE_LOOP('',(#74524,#74525,#74526,#74527,#74528)) ;
#27474=EDGE_LOOP('',(#74529,#74530,#74531,#74532)) ;
#27475=EDGE_LOOP('',(#74533,#74534,#74535,#74536)) ;
#27476=EDGE_LOOP('',(#74537,#74538,#74539,#74540)) ;
#27477=EDGE_LOOP('',(#74541,#74542,#74543,#74544)) ;
#27478=EDGE_LOOP('',(#74545,#74546,#74547)) ;
#27479=EDGE_LOOP('',(#74548,#74549,#74550)) ;
#27480=EDGE_LOOP('',(#74551,#74552,#74553,#74554)) ;
#27481=EDGE_LOOP('',(#74555,#74556,#74557,#74558)) ;
#27482=EDGE_LOOP('',(#74559,#74560,#74561)) ;
#27483=EDGE_LOOP('',(#74562,#74563,#74564,#74565)) ;
#27484=EDGE_LOOP('',(#74566,#74567,#74568,#74569,#74570)) ;
#27485=EDGE_LOOP('',(#74571,#74572,#74573,#74574,#74575)) ;
#27486=EDGE_LOOP('',(#74576,#74577,#74578,#74579)) ;
#27487=EDGE_LOOP('',(#74580,#74581,#74582,#74583)) ;
#27488=EDGE_LOOP('',(#74584,#74585,#74586,#74587)) ;
#27489=EDGE_LOOP('',(#74588,#74589,#74590)) ;
#27490=EDGE_LOOP('',(#74591,#74592,#74593,#74594)) ;
#27491=EDGE_LOOP('',(#74595,#74596,#74597,#74598)) ;
#27492=EDGE_LOOP('',(#74599,#74600,#74601)) ;
#27493=EDGE_LOOP('',(#74602,#74603,#74604,#74605)) ;
#27494=EDGE_LOOP('',(#74606,#74607,#74608,#74609)) ;
#27495=EDGE_LOOP('',(#74610,#74611,#74612)) ;
#27496=EDGE_LOOP('',(#74613,#74614,#74615)) ;
#27497=EDGE_LOOP('',(#74616,#74617,#74618,#74619)) ;
#27498=EDGE_LOOP('',(#74620,#74621,#74622,#74623)) ;
#27499=EDGE_LOOP('',(#74624,#74625,#74626,#74627)) ;
#27500=EDGE_LOOP('',(#74628,#74629,#74630)) ;
#27501=EDGE_LOOP('',(#74631,#74632,#74633,#74634)) ;
#27502=EDGE_LOOP('',(#74635,#74636,#74637,#74638)) ;
#27503=EDGE_LOOP('',(#74639,#74640,#74641)) ;
#27504=EDGE_LOOP('',(#74642,#74643,#74644,#74645)) ;
#27505=EDGE_LOOP('',(#74646,#74647,#74648,#74649)) ;
#27506=EDGE_LOOP('',(#74650,#74651,#74652,#74653,#74654)) ;
#27507=EDGE_LOOP('',(#74655,#74656,#74657,#74658)) ;
#27508=EDGE_LOOP('',(#74659,#74660,#74661,#74662)) ;
#27509=EDGE_LOOP('',(#74663,#74664,#74665,#74666)) ;
#27510=EDGE_LOOP('',(#74667,#74668,#74669,#74670)) ;
#27511=EDGE_LOOP('',(#74671,#74672,#74673,#74674)) ;
#27512=EDGE_LOOP('',(#74675,#74676,#74677,#74678)) ;
#27513=EDGE_LOOP('',(#74679,#74680,#74681,#74682)) ;
#27514=EDGE_LOOP('',(#74683,#74684,#74685,#74686)) ;
#27515=EDGE_LOOP('',(#74687,#74688,#74689,#74690)) ;
#27516=EDGE_LOOP('',(#74691,#74692,#74693,#74694)) ;
#27517=EDGE_LOOP('',(#74695,#74696,#74697,#74698)) ;
#27518=EDGE_LOOP('',(#74699,#74700,#74701)) ;
#27519=EDGE_LOOP('',(#74702,#74703,#74704)) ;
#27520=EDGE_LOOP('',(#74705,#74706,#74707,#74708)) ;
#27521=EDGE_LOOP('',(#74709,#74710,#74711,#74712)) ;
#27522=EDGE_LOOP('',(#74713,#74714,#74715,#74716)) ;
#27523=EDGE_LOOP('',(#74717,#74718,#74719,#74720)) ;
#27524=EDGE_LOOP('',(#74721,#74722,#74723)) ;
#27525=EDGE_LOOP('',(#74724,#74725,#74726)) ;
#27526=EDGE_LOOP('',(#74727,#74728,#74729,#74730)) ;
#27527=EDGE_LOOP('',(#74731,#74732,#74733,#74734)) ;
#27528=EDGE_LOOP('',(#74735,#74736,#74737,#74738)) ;
#27529=EDGE_LOOP('',(#74739,#74740,#74741,#74742)) ;
#27530=EDGE_LOOP('',(#74743,#74744,#74745,#74746)) ;
#27531=EDGE_LOOP('',(#74747,#74748,#74749,#74750)) ;
#27532=EDGE_LOOP('',(#74751,#74752,#74753,#74754)) ;
#27533=EDGE_LOOP('',(#74755,#74756,#74757,#74758)) ;
#27534=EDGE_LOOP('',(#74759,#74760,#74761,#74762)) ;
#27535=EDGE_LOOP('',(#74763,#74764,#74765,#74766)) ;
#27536=EDGE_LOOP('',(#74767,#74768,#74769,#74770)) ;
#27537=EDGE_LOOP('',(#74771,#74772,#74773)) ;
#27538=EDGE_LOOP('',(#74774,#74775,#74776)) ;
#27539=EDGE_LOOP('',(#74777,#74778,#74779,#74780)) ;
#27540=EDGE_LOOP('',(#74781,#74782,#74783,#74784)) ;
#27541=EDGE_LOOP('',(#74785,#74786,#74787,#74788)) ;
#27542=EDGE_LOOP('',(#74789,#74790,#74791,#74792)) ;
#27543=EDGE_LOOP('',(#74793,#74794,#74795,#74796)) ;
#27544=EDGE_LOOP('',(#74797,#74798,#74799)) ;
#27545=EDGE_LOOP('',(#74800,#74801,#74802)) ;
#27546=EDGE_LOOP('',(#74803,#74804,#74805,#74806)) ;
#27547=EDGE_LOOP('',(#74807,#74808,#74809,#74810)) ;
#27548=EDGE_LOOP('',(#74811,#74812,#74813,#74814)) ;
#27549=EDGE_LOOP('',(#74815,#74816,#74817,#74818)) ;
#27550=EDGE_LOOP('',(#74819,#74820,#74821)) ;
#27551=EDGE_LOOP('',(#74822,#74823,#74824)) ;
#27552=EDGE_LOOP('',(#74825,#74826,#74827,#74828)) ;
#27553=EDGE_LOOP('',(#74829,#74830,#74831,#74832)) ;
#27554=EDGE_LOOP('',(#74833,#74834,#74835,#74836)) ;
#27555=EDGE_LOOP('',(#74837,#74838,#74839,#74840)) ;
#27556=EDGE_LOOP('',(#74841,#74842,#74843)) ;
#27557=EDGE_LOOP('',(#74844,#74845,#74846)) ;
#27558=EDGE_LOOP('',(#74847,#74848,#74849,#74850)) ;
#27559=EDGE_LOOP('',(#74851,#74852,#74853,#74854)) ;
#27560=EDGE_LOOP('',(#74855,#74856,#74857)) ;
#27561=EDGE_LOOP('',(#74858,#74859,#74860)) ;
#27562=EDGE_LOOP('',(#74861,#74862,#74863,#74864)) ;
#27563=EDGE_LOOP('',(#74865,#74866,#74867,#74868)) ;
#27564=EDGE_LOOP('',(#74869,#74870,#74871)) ;
#27565=EDGE_LOOP('',(#74872,#74873,#74874)) ;
#27566=EDGE_LOOP('',(#74875,#74876,#74877,#74878)) ;
#27567=EDGE_LOOP('',(#74879,#74880,#74881,#74882)) ;
#27568=EDGE_LOOP('',(#74883,#74884,#74885,#74886)) ;
#27569=EDGE_LOOP('',(#74887,#74888,#74889,#74890)) ;
#27570=EDGE_LOOP('',(#74891,#74892,#74893,#74894)) ;
#27571=EDGE_LOOP('',(#74895,#74896,#74897)) ;
#27572=EDGE_LOOP('',(#74898,#74899,#74900,#74901)) ;
#27573=EDGE_LOOP('',(#74902,#74903,#74904,#74905)) ;
#27574=EDGE_LOOP('',(#74906,#74907,#74908,#74909)) ;
#27575=EDGE_LOOP('',(#74910,#74911,#74912,#74913)) ;
#27576=EDGE_LOOP('',(#74914,#74915,#74916)) ;
#27577=EDGE_LOOP('',(#74917,#74918,#74919,#74920)) ;
#27578=EDGE_LOOP('',(#74921,#74922,#74923)) ;
#27579=EDGE_LOOP('',(#74924,#74925,#74926,#74927)) ;
#27580=EDGE_LOOP('',(#74928,#74929,#74930,#74931)) ;
#27581=EDGE_LOOP('',(#74932,#74933,#74934,#74935)) ;
#27582=EDGE_LOOP('',(#74936,#74937,#74938,#74939)) ;
#27583=EDGE_LOOP('',(#74940,#74941,#74942,#74943)) ;
#27584=EDGE_LOOP('',(#74944,#74945,#74946,#74947)) ;
#27585=EDGE_LOOP('',(#74948,#74949,#74950,#74951)) ;
#27586=EDGE_LOOP('',(#74952,#74953,#74954,#74955)) ;
#27587=EDGE_LOOP('',(#74956,#74957,#74958,#74959)) ;
#27588=EDGE_LOOP('',(#74960,#74961,#74962)) ;
#27589=EDGE_LOOP('',(#74963,#74964,#74965,#74966)) ;
#27590=EDGE_LOOP('',(#74967,#74968,#74969,#74970)) ;
#27591=EDGE_LOOP('',(#74971,#74972,#74973,#74974)) ;
#27592=EDGE_LOOP('',(#74975,#74976,#74977,#74978)) ;
#27593=EDGE_LOOP('',(#74979,#74980,#74981)) ;
#27594=EDGE_LOOP('',(#74982,#74983,#74984)) ;
#27595=EDGE_LOOP('',(#74985,#74986,#74987,#74988)) ;
#27596=EDGE_LOOP('',(#74989,#74990,#74991,#74992)) ;
#27597=EDGE_LOOP('',(#74993,#74994,#74995,#74996)) ;
#27598=EDGE_LOOP('',(#74997,#74998,#74999,#75000)) ;
#27599=EDGE_LOOP('',(#75001,#75002,#75003,#75004)) ;
#27600=EDGE_LOOP('',(#75005,#75006,#75007,#75008)) ;
#27601=EDGE_LOOP('',(#75009,#75010,#75011)) ;
#27602=EDGE_LOOP('',(#75012,#75013,#75014,#75015)) ;
#27603=EDGE_LOOP('',(#75016,#75017,#75018,#75019)) ;
#27604=EDGE_LOOP('',(#75020,#75021,#75022,#75023)) ;
#27605=EDGE_LOOP('',(#75024,#75025,#75026,#75027)) ;
#27606=EDGE_LOOP('',(#75028,#75029,#75030,#75031)) ;
#27607=EDGE_LOOP('',(#75032,#75033,#75034)) ;
#27608=EDGE_LOOP('',(#75035,#75036,#75037,#75038)) ;
#27609=EDGE_LOOP('',(#75039,#75040,#75041,#75042,#75043)) ;
#27610=EDGE_LOOP('',(#75044,#75045,#75046,#75047)) ;
#27611=EDGE_LOOP('',(#75048,#75049,#75050,#75051,#75052)) ;
#27612=EDGE_LOOP('',(#75053,#75054,#75055)) ;
#27613=EDGE_LOOP('',(#75056,#75057,#75058,#75059,#75060)) ;
#27614=EDGE_LOOP('',(#75061,#75062,#75063,#75064)) ;
#27615=EDGE_LOOP('',(#75065,#75066,#75067,#75068)) ;
#27616=EDGE_LOOP('',(#75069,#75070,#75071,#75072)) ;
#27617=EDGE_LOOP('',(#75073,#75074,#75075,#75076)) ;
#27618=EDGE_LOOP('',(#75077,#75078,#75079)) ;
#27619=EDGE_LOOP('',(#75080,#75081,#75082)) ;
#27620=EDGE_LOOP('',(#75083,#75084,#75085,#75086)) ;
#27621=EDGE_LOOP('',(#75087,#75088,#75089,#75090)) ;
#27622=EDGE_LOOP('',(#75091,#75092,#75093)) ;
#27623=EDGE_LOOP('',(#75094,#75095,#75096,#75097)) ;
#27624=EDGE_LOOP('',(#75098,#75099,#75100,#75101,#75102)) ;
#27625=EDGE_LOOP('',(#75103,#75104,#75105,#75106,#75107)) ;
#27626=EDGE_LOOP('',(#75108,#75109,#75110,#75111)) ;
#27627=EDGE_LOOP('',(#75112,#75113,#75114,#75115)) ;
#27628=EDGE_LOOP('',(#75116,#75117,#75118,#75119)) ;
#27629=EDGE_LOOP('',(#75120,#75121,#75122)) ;
#27630=EDGE_LOOP('',(#75123,#75124,#75125,#75126)) ;
#27631=EDGE_LOOP('',(#75127,#75128,#75129,#75130)) ;
#27632=EDGE_LOOP('',(#75131,#75132,#75133)) ;
#27633=EDGE_LOOP('',(#75134,#75135,#75136,#75137)) ;
#27634=EDGE_LOOP('',(#75138,#75139,#75140,#75141)) ;
#27635=EDGE_LOOP('',(#75142,#75143,#75144)) ;
#27636=EDGE_LOOP('',(#75145,#75146,#75147)) ;
#27637=EDGE_LOOP('',(#75148,#75149,#75150,#75151)) ;
#27638=EDGE_LOOP('',(#75152,#75153,#75154,#75155)) ;
#27639=EDGE_LOOP('',(#75156,#75157,#75158,#75159)) ;
#27640=EDGE_LOOP('',(#75160,#75161,#75162)) ;
#27641=EDGE_LOOP('',(#75163,#75164,#75165,#75166)) ;
#27642=EDGE_LOOP('',(#75167,#75168,#75169,#75170)) ;
#27643=EDGE_LOOP('',(#75171,#75172,#75173)) ;
#27644=EDGE_LOOP('',(#75174,#75175,#75176,#75177)) ;
#27645=EDGE_LOOP('',(#75178,#75179,#75180,#75181)) ;
#27646=EDGE_LOOP('',(#75182,#75183,#75184,#75185,#75186)) ;
#27647=EDGE_LOOP('',(#75187,#75188,#75189,#75190)) ;
#27648=EDGE_LOOP('',(#75191,#75192,#75193,#75194)) ;
#27649=EDGE_LOOP('',(#75195,#75196,#75197,#75198)) ;
#27650=EDGE_LOOP('',(#75199,#75200,#75201,#75202)) ;
#27651=EDGE_LOOP('',(#75203,#75204,#75205,#75206)) ;
#27652=EDGE_LOOP('',(#75207,#75208,#75209,#75210)) ;
#27653=EDGE_LOOP('',(#75211,#75212,#75213,#75214)) ;
#27654=EDGE_LOOP('',(#75215,#75216,#75217,#75218)) ;
#27655=EDGE_LOOP('',(#75219,#75220,#75221,#75222)) ;
#27656=EDGE_LOOP('',(#75223,#75224,#75225,#75226)) ;
#27657=EDGE_LOOP('',(#75227,#75228,#75229,#75230)) ;
#27658=EDGE_LOOP('',(#75231,#75232,#75233)) ;
#27659=EDGE_LOOP('',(#75234,#75235,#75236)) ;
#27660=EDGE_LOOP('',(#75237,#75238,#75239,#75240)) ;
#27661=EDGE_LOOP('',(#75241,#75242,#75243,#75244)) ;
#27662=EDGE_LOOP('',(#75245,#75246,#75247,#75248)) ;
#27663=EDGE_LOOP('',(#75249,#75250,#75251,#75252)) ;
#27664=EDGE_LOOP('',(#75253,#75254,#75255)) ;
#27665=EDGE_LOOP('',(#75256,#75257,#75258)) ;
#27666=EDGE_LOOP('',(#75259,#75260,#75261,#75262)) ;
#27667=EDGE_LOOP('',(#75263,#75264,#75265,#75266)) ;
#27668=EDGE_LOOP('',(#75267,#75268,#75269,#75270)) ;
#27669=EDGE_LOOP('',(#75271,#75272,#75273,#75274)) ;
#27670=EDGE_LOOP('',(#75275,#75276,#75277,#75278)) ;
#27671=EDGE_LOOP('',(#75279,#75280,#75281,#75282)) ;
#27672=EDGE_LOOP('',(#75283,#75284,#75285,#75286)) ;
#27673=EDGE_LOOP('',(#75287,#75288,#75289,#75290)) ;
#27674=EDGE_LOOP('',(#75291,#75292,#75293,#75294)) ;
#27675=EDGE_LOOP('',(#75295,#75296,#75297,#75298)) ;
#27676=EDGE_LOOP('',(#75299,#75300,#75301,#75302)) ;
#27677=EDGE_LOOP('',(#75303,#75304,#75305)) ;
#27678=EDGE_LOOP('',(#75306,#75307,#75308)) ;
#27679=EDGE_LOOP('',(#75309,#75310,#75311,#75312)) ;
#27680=EDGE_LOOP('',(#75313,#75314,#75315,#75316)) ;
#27681=EDGE_LOOP('',(#75317,#75318,#75319,#75320)) ;
#27682=EDGE_LOOP('',(#75321,#75322,#75323,#75324)) ;
#27683=EDGE_LOOP('',(#75325,#75326,#75327,#75328)) ;
#27684=EDGE_LOOP('',(#75329,#75330,#75331)) ;
#27685=EDGE_LOOP('',(#75332,#75333,#75334)) ;
#27686=EDGE_LOOP('',(#75335,#75336,#75337,#75338)) ;
#27687=EDGE_LOOP('',(#75339,#75340,#75341,#75342)) ;
#27688=EDGE_LOOP('',(#75343,#75344,#75345,#75346)) ;
#27689=EDGE_LOOP('',(#75347,#75348,#75349,#75350)) ;
#27690=EDGE_LOOP('',(#75351,#75352,#75353)) ;
#27691=EDGE_LOOP('',(#75354,#75355,#75356)) ;
#27692=EDGE_LOOP('',(#75357,#75358,#75359,#75360)) ;
#27693=EDGE_LOOP('',(#75361,#75362,#75363,#75364)) ;
#27694=EDGE_LOOP('',(#75365,#75366,#75367,#75368)) ;
#27695=EDGE_LOOP('',(#75369,#75370,#75371,#75372)) ;
#27696=EDGE_LOOP('',(#75373,#75374,#75375)) ;
#27697=EDGE_LOOP('',(#75376,#75377,#75378)) ;
#27698=EDGE_LOOP('',(#75379,#75380,#75381,#75382)) ;
#27699=EDGE_LOOP('',(#75383,#75384,#75385,#75386)) ;
#27700=EDGE_LOOP('',(#75387,#75388,#75389)) ;
#27701=EDGE_LOOP('',(#75390,#75391,#75392)) ;
#27702=EDGE_LOOP('',(#75393,#75394,#75395,#75396)) ;
#27703=EDGE_LOOP('',(#75397,#75398,#75399,#75400)) ;
#27704=EDGE_LOOP('',(#75401,#75402,#75403)) ;
#27705=EDGE_LOOP('',(#75404,#75405,#75406)) ;
#27706=EDGE_LOOP('',(#75407,#75408,#75409,#75410)) ;
#27707=EDGE_LOOP('',(#75411,#75412,#75413,#75414)) ;
#27708=EDGE_LOOP('',(#75415,#75416,#75417,#75418)) ;
#27709=EDGE_LOOP('',(#75419,#75420,#75421,#75422)) ;
#27710=EDGE_LOOP('',(#75423,#75424,#75425,#75426)) ;
#27711=EDGE_LOOP('',(#75427,#75428,#75429)) ;
#27712=EDGE_LOOP('',(#75430,#75431,#75432,#75433)) ;
#27713=EDGE_LOOP('',(#75434,#75435,#75436,#75437)) ;
#27714=EDGE_LOOP('',(#75438,#75439,#75440,#75441)) ;
#27715=EDGE_LOOP('',(#75442,#75443,#75444,#75445)) ;
#27716=EDGE_LOOP('',(#75446,#75447,#75448)) ;
#27717=EDGE_LOOP('',(#75449,#75450,#75451,#75452)) ;
#27718=EDGE_LOOP('',(#75453,#75454,#75455)) ;
#27719=EDGE_LOOP('',(#75456,#75457,#75458,#75459)) ;
#27720=EDGE_LOOP('',(#75460,#75461,#75462,#75463)) ;
#27721=EDGE_LOOP('',(#75464,#75465,#75466,#75467)) ;
#27722=EDGE_LOOP('',(#75468,#75469,#75470,#75471)) ;
#27723=EDGE_LOOP('',(#75472,#75473,#75474,#75475)) ;
#27724=EDGE_LOOP('',(#75476,#75477,#75478,#75479)) ;
#27725=EDGE_LOOP('',(#75480,#75481,#75482,#75483)) ;
#27726=EDGE_LOOP('',(#75484,#75485,#75486,#75487)) ;
#27727=EDGE_LOOP('',(#75488,#75489,#75490,#75491)) ;
#27728=EDGE_LOOP('',(#75492,#75493,#75494)) ;
#27729=EDGE_LOOP('',(#75495,#75496,#75497,#75498)) ;
#27730=EDGE_LOOP('',(#75499,#75500,#75501,#75502)) ;
#27731=EDGE_LOOP('',(#75503,#75504,#75505,#75506)) ;
#27732=EDGE_LOOP('',(#75507,#75508,#75509,#75510)) ;
#27733=EDGE_LOOP('',(#75511,#75512,#75513)) ;
#27734=EDGE_LOOP('',(#75514,#75515,#75516)) ;
#27735=EDGE_LOOP('',(#75517,#75518,#75519,#75520)) ;
#27736=EDGE_LOOP('',(#75521,#75522,#75523,#75524)) ;
#27737=EDGE_LOOP('',(#75525,#75526,#75527,#75528)) ;
#27738=EDGE_LOOP('',(#75529,#75530,#75531,#75532)) ;
#27739=EDGE_LOOP('',(#75533,#75534,#75535,#75536)) ;
#27740=EDGE_LOOP('',(#75537,#75538,#75539,#75540)) ;
#27741=EDGE_LOOP('',(#75541,#75542,#75543)) ;
#27742=EDGE_LOOP('',(#75544,#75545,#75546,#75547)) ;
#27743=EDGE_LOOP('',(#75548,#75549,#75550,#75551)) ;
#27744=EDGE_LOOP('',(#75552,#75553,#75554,#75555)) ;
#27745=EDGE_LOOP('',(#75556,#75557,#75558,#75559)) ;
#27746=EDGE_LOOP('',(#75560,#75561,#75562,#75563)) ;
#27747=EDGE_LOOP('',(#75564,#75565,#75566)) ;
#27748=EDGE_LOOP('',(#75567,#75568,#75569,#75570)) ;
#27749=EDGE_LOOP('',(#75571,#75572,#75573,#75574,#75575)) ;
#27750=EDGE_LOOP('',(#75576,#75577,#75578,#75579)) ;
#27751=EDGE_LOOP('',(#75580,#75581,#75582,#75583,#75584)) ;
#27752=EDGE_LOOP('',(#75585,#75586,#75587)) ;
#27753=EDGE_LOOP('',(#75588,#75589,#75590,#75591,#75592)) ;
#27754=EDGE_LOOP('',(#75593,#75594,#75595,#75596)) ;
#27755=EDGE_LOOP('',(#75597,#75598,#75599,#75600)) ;
#27756=EDGE_LOOP('',(#75601,#75602,#75603,#75604)) ;
#27757=EDGE_LOOP('',(#75605,#75606,#75607,#75608)) ;
#27758=EDGE_LOOP('',(#75609,#75610,#75611)) ;
#27759=EDGE_LOOP('',(#75612,#75613,#75614)) ;
#27760=EDGE_LOOP('',(#75615,#75616,#75617,#75618)) ;
#27761=EDGE_LOOP('',(#75619,#75620,#75621,#75622)) ;
#27762=EDGE_LOOP('',(#75623,#75624,#75625)) ;
#27763=EDGE_LOOP('',(#75626,#75627,#75628,#75629)) ;
#27764=EDGE_LOOP('',(#75630,#75631,#75632,#75633,#75634)) ;
#27765=EDGE_LOOP('',(#75635,#75636,#75637,#75638,#75639)) ;
#27766=EDGE_LOOP('',(#75640,#75641,#75642,#75643)) ;
#27767=EDGE_LOOP('',(#75644,#75645,#75646,#75647)) ;
#27768=EDGE_LOOP('',(#75648,#75649,#75650,#75651)) ;
#27769=EDGE_LOOP('',(#75652,#75653,#75654)) ;
#27770=EDGE_LOOP('',(#75655,#75656,#75657,#75658)) ;
#27771=EDGE_LOOP('',(#75659,#75660,#75661,#75662)) ;
#27772=EDGE_LOOP('',(#75663,#75664,#75665)) ;
#27773=EDGE_LOOP('',(#75666,#75667,#75668,#75669)) ;
#27774=EDGE_LOOP('',(#75670,#75671,#75672,#75673)) ;
#27775=EDGE_LOOP('',(#75674,#75675,#75676)) ;
#27776=EDGE_LOOP('',(#75677,#75678,#75679)) ;
#27777=EDGE_LOOP('',(#75680,#75681,#75682,#75683)) ;
#27778=EDGE_LOOP('',(#75684,#75685,#75686,#75687)) ;
#27779=EDGE_LOOP('',(#75688,#75689,#75690,#75691)) ;
#27780=EDGE_LOOP('',(#75692,#75693,#75694)) ;
#27781=EDGE_LOOP('',(#75695,#75696,#75697,#75698)) ;
#27782=EDGE_LOOP('',(#75699,#75700,#75701,#75702)) ;
#27783=EDGE_LOOP('',(#75703,#75704,#75705)) ;
#27784=EDGE_LOOP('',(#75706,#75707,#75708,#75709)) ;
#27785=EDGE_LOOP('',(#75710,#75711,#75712,#75713)) ;
#27786=EDGE_LOOP('',(#75714,#75715,#75716,#75717,#75718)) ;
#27787=EDGE_LOOP('',(#75719,#75720,#75721,#75722)) ;
#27788=EDGE_LOOP('',(#75723,#75724,#75725,#75726)) ;
#27789=EDGE_LOOP('',(#75727,#75728,#75729,#75730)) ;
#27790=EDGE_LOOP('',(#75731,#75732,#75733,#75734)) ;
#27791=EDGE_LOOP('',(#75735,#75736,#75737,#75738)) ;
#27792=EDGE_LOOP('',(#75739,#75740,#75741,#75742)) ;
#27793=EDGE_LOOP('',(#75743,#75744,#75745,#75746)) ;
#27794=EDGE_LOOP('',(#75747,#75748,#75749,#75750)) ;
#27795=EDGE_LOOP('',(#75751,#75752,#75753,#75754)) ;
#27796=EDGE_LOOP('',(#75755,#75756,#75757,#75758)) ;
#27797=EDGE_LOOP('',(#75759,#75760,#75761,#75762)) ;
#27798=EDGE_LOOP('',(#75763,#75764,#75765)) ;
#27799=EDGE_LOOP('',(#75766,#75767,#75768)) ;
#27800=EDGE_LOOP('',(#75769,#75770,#75771,#75772)) ;
#27801=EDGE_LOOP('',(#75773,#75774,#75775,#75776)) ;
#27802=EDGE_LOOP('',(#75777,#75778,#75779,#75780)) ;
#27803=EDGE_LOOP('',(#75781,#75782,#75783,#75784)) ;
#27804=EDGE_LOOP('',(#75785,#75786,#75787)) ;
#27805=EDGE_LOOP('',(#75788,#75789,#75790)) ;
#27806=EDGE_LOOP('',(#75791,#75792,#75793,#75794)) ;
#27807=EDGE_LOOP('',(#75795,#75796,#75797,#75798)) ;
#27808=EDGE_LOOP('',(#75799,#75800,#75801,#75802)) ;
#27809=EDGE_LOOP('',(#75803,#75804,#75805,#75806)) ;
#27810=EDGE_LOOP('',(#75807,#75808,#75809,#75810)) ;
#27811=EDGE_LOOP('',(#75811,#75812,#75813,#75814)) ;
#27812=EDGE_LOOP('',(#75815,#75816,#75817,#75818)) ;
#27813=EDGE_LOOP('',(#75819,#75820,#75821,#75822)) ;
#27814=EDGE_LOOP('',(#75823,#75824,#75825,#75826)) ;
#27815=EDGE_LOOP('',(#75827,#75828,#75829,#75830)) ;
#27816=EDGE_LOOP('',(#75831,#75832,#75833,#75834)) ;
#27817=EDGE_LOOP('',(#75835,#75836,#75837)) ;
#27818=EDGE_LOOP('',(#75838,#75839,#75840)) ;
#27819=EDGE_LOOP('',(#75841,#75842,#75843,#75844)) ;
#27820=EDGE_LOOP('',(#75845,#75846,#75847,#75848)) ;
#27821=EDGE_LOOP('',(#75849,#75850,#75851,#75852)) ;
#27822=EDGE_LOOP('',(#75853,#75854,#75855,#75856)) ;
#27823=EDGE_LOOP('',(#75857,#75858,#75859,#75860)) ;
#27824=EDGE_LOOP('',(#75861,#75862,#75863)) ;
#27825=EDGE_LOOP('',(#75864,#75865,#75866)) ;
#27826=EDGE_LOOP('',(#75867,#75868,#75869,#75870)) ;
#27827=EDGE_LOOP('',(#75871,#75872,#75873,#75874)) ;
#27828=EDGE_LOOP('',(#75875,#75876,#75877,#75878)) ;
#27829=EDGE_LOOP('',(#75879,#75880,#75881,#75882)) ;
#27830=EDGE_LOOP('',(#75883,#75884,#75885)) ;
#27831=EDGE_LOOP('',(#75886,#75887,#75888)) ;
#27832=EDGE_LOOP('',(#75889,#75890,#75891,#75892)) ;
#27833=EDGE_LOOP('',(#75893,#75894,#75895,#75896)) ;
#27834=EDGE_LOOP('',(#75897,#75898,#75899,#75900)) ;
#27835=EDGE_LOOP('',(#75901,#75902,#75903,#75904)) ;
#27836=EDGE_LOOP('',(#75905,#75906,#75907)) ;
#27837=EDGE_LOOP('',(#75908,#75909,#75910)) ;
#27838=EDGE_LOOP('',(#75911,#75912,#75913,#75914)) ;
#27839=EDGE_LOOP('',(#75915,#75916,#75917,#75918)) ;
#27840=EDGE_LOOP('',(#75919,#75920,#75921)) ;
#27841=EDGE_LOOP('',(#75922,#75923,#75924)) ;
#27842=EDGE_LOOP('',(#75925,#75926,#75927,#75928)) ;
#27843=EDGE_LOOP('',(#75929,#75930,#75931,#75932)) ;
#27844=EDGE_LOOP('',(#75933,#75934,#75935)) ;
#27845=EDGE_LOOP('',(#75936,#75937,#75938)) ;
#27846=EDGE_LOOP('',(#75939,#75940,#75941,#75942)) ;
#27847=EDGE_LOOP('',(#75943,#75944,#75945,#75946)) ;
#27848=EDGE_LOOP('',(#75947,#75948,#75949,#75950)) ;
#27849=EDGE_LOOP('',(#75951,#75952,#75953,#75954)) ;
#27850=EDGE_LOOP('',(#75955,#75956,#75957,#75958)) ;
#27851=EDGE_LOOP('',(#75959,#75960,#75961)) ;
#27852=EDGE_LOOP('',(#75962,#75963,#75964,#75965)) ;
#27853=EDGE_LOOP('',(#75966,#75967,#75968,#75969)) ;
#27854=EDGE_LOOP('',(#75970,#75971,#75972,#75973)) ;
#27855=EDGE_LOOP('',(#75974,#75975,#75976,#75977)) ;
#27856=EDGE_LOOP('',(#75978,#75979,#75980)) ;
#27857=EDGE_LOOP('',(#75981,#75982,#75983,#75984)) ;
#27858=EDGE_LOOP('',(#75985,#75986,#75987)) ;
#27859=EDGE_LOOP('',(#75988,#75989,#75990,#75991)) ;
#27860=EDGE_LOOP('',(#75992,#75993,#75994,#75995)) ;
#27861=EDGE_LOOP('',(#75996,#75997,#75998,#75999)) ;
#27862=EDGE_LOOP('',(#76000,#76001,#76002,#76003)) ;
#27863=EDGE_LOOP('',(#76004,#76005,#76006,#76007)) ;
#27864=EDGE_LOOP('',(#76008,#76009,#76010,#76011)) ;
#27865=EDGE_LOOP('',(#76012,#76013,#76014,#76015)) ;
#27866=EDGE_LOOP('',(#76016,#76017,#76018,#76019)) ;
#27867=EDGE_LOOP('',(#76020,#76021,#76022,#76023)) ;
#27868=EDGE_LOOP('',(#76024,#76025,#76026)) ;
#27869=EDGE_LOOP('',(#76027,#76028,#76029,#76030)) ;
#27870=EDGE_LOOP('',(#76031,#76032,#76033,#76034)) ;
#27871=EDGE_LOOP('',(#76035,#76036,#76037,#76038)) ;
#27872=EDGE_LOOP('',(#76039,#76040,#76041,#76042)) ;
#27873=EDGE_LOOP('',(#76043,#76044,#76045)) ;
#27874=EDGE_LOOP('',(#76046,#76047,#76048)) ;
#27875=EDGE_LOOP('',(#76049,#76050,#76051,#76052)) ;
#27876=EDGE_LOOP('',(#76053,#76054,#76055,#76056)) ;
#27877=EDGE_LOOP('',(#76057,#76058,#76059,#76060)) ;
#27878=EDGE_LOOP('',(#76061,#76062,#76063,#76064)) ;
#27879=EDGE_LOOP('',(#76065,#76066,#76067,#76068)) ;
#27880=EDGE_LOOP('',(#76069,#76070,#76071,#76072)) ;
#27881=EDGE_LOOP('',(#76073,#76074,#76075)) ;
#27882=EDGE_LOOP('',(#76076,#76077,#76078,#76079)) ;
#27883=EDGE_LOOP('',(#76080,#76081,#76082,#76083)) ;
#27884=EDGE_LOOP('',(#76084,#76085,#76086,#76087)) ;
#27885=EDGE_LOOP('',(#76088,#76089,#76090,#76091)) ;
#27886=EDGE_LOOP('',(#76092,#76093,#76094,#76095)) ;
#27887=EDGE_LOOP('',(#76096,#76097,#76098)) ;
#27888=EDGE_LOOP('',(#76099,#76100,#76101,#76102)) ;
#27889=EDGE_LOOP('',(#76103,#76104,#76105,#76106,#76107)) ;
#27890=EDGE_LOOP('',(#76108,#76109,#76110,#76111)) ;
#27891=EDGE_LOOP('',(#76112,#76113,#76114,#76115,#76116)) ;
#27892=EDGE_LOOP('',(#76117,#76118,#76119)) ;
#27893=EDGE_LOOP('',(#76120,#76121,#76122,#76123,#76124)) ;
#27894=EDGE_LOOP('',(#76125,#76126,#76127,#76128)) ;
#27895=EDGE_LOOP('',(#76129,#76130,#76131,#76132)) ;
#27896=EDGE_LOOP('',(#76133,#76134,#76135,#76136)) ;
#27897=EDGE_LOOP('',(#76137,#76138,#76139,#76140)) ;
#27898=EDGE_LOOP('',(#76141,#76142,#76143)) ;
#27899=EDGE_LOOP('',(#76144,#76145,#76146)) ;
#27900=EDGE_LOOP('',(#76147,#76148,#76149,#76150)) ;
#27901=EDGE_LOOP('',(#76151,#76152,#76153,#76154)) ;
#27902=EDGE_LOOP('',(#76155,#76156,#76157)) ;
#27903=EDGE_LOOP('',(#76158,#76159,#76160,#76161)) ;
#27904=EDGE_LOOP('',(#76162,#76163,#76164,#76165,#76166)) ;
#27905=EDGE_LOOP('',(#76167,#76168,#76169,#76170,#76171)) ;
#27906=EDGE_LOOP('',(#76172,#76173,#76174,#76175)) ;
#27907=EDGE_LOOP('',(#76176,#76177,#76178,#76179)) ;
#27908=EDGE_LOOP('',(#76180,#76181,#76182,#76183)) ;
#27909=EDGE_LOOP('',(#76184,#76185,#76186)) ;
#27910=EDGE_LOOP('',(#76187,#76188,#76189,#76190)) ;
#27911=EDGE_LOOP('',(#76191,#76192,#76193,#76194)) ;
#27912=EDGE_LOOP('',(#76195,#76196,#76197)) ;
#27913=EDGE_LOOP('',(#76198,#76199,#76200,#76201)) ;
#27914=EDGE_LOOP('',(#76202,#76203,#76204,#76205)) ;
#27915=EDGE_LOOP('',(#76206,#76207,#76208)) ;
#27916=EDGE_LOOP('',(#76209,#76210,#76211)) ;
#27917=EDGE_LOOP('',(#76212,#76213,#76214,#76215)) ;
#27918=EDGE_LOOP('',(#76216,#76217,#76218,#76219)) ;
#27919=EDGE_LOOP('',(#76220,#76221,#76222,#76223)) ;
#27920=EDGE_LOOP('',(#76224,#76225,#76226)) ;
#27921=EDGE_LOOP('',(#76227,#76228,#76229,#76230)) ;
#27922=EDGE_LOOP('',(#76231,#76232,#76233,#76234)) ;
#27923=EDGE_LOOP('',(#76235,#76236,#76237)) ;
#27924=EDGE_LOOP('',(#76238,#76239,#76240,#76241)) ;
#27925=EDGE_LOOP('',(#76242,#76243,#76244,#76245)) ;
#27926=EDGE_LOOP('',(#76246,#76247,#76248,#76249,#76250)) ;
#27927=EDGE_LOOP('',(#76251,#76252,#76253,#76254)) ;
#27928=EDGE_LOOP('',(#76255,#76256,#76257,#76258)) ;
#27929=EDGE_LOOP('',(#76259,#76260,#76261,#76262)) ;
#27930=EDGE_LOOP('',(#76263,#76264,#76265,#76266)) ;
#27931=EDGE_LOOP('',(#76267,#76268,#76269,#76270)) ;
#27932=EDGE_LOOP('',(#76271,#76272,#76273,#76274)) ;
#27933=EDGE_LOOP('',(#76275,#76276,#76277,#76278)) ;
#27934=EDGE_LOOP('',(#76279,#76280,#76281,#76282)) ;
#27935=EDGE_LOOP('',(#76283,#76284,#76285,#76286)) ;
#27936=EDGE_LOOP('',(#76287,#76288,#76289,#76290)) ;
#27937=EDGE_LOOP('',(#76291,#76292,#76293,#76294)) ;
#27938=EDGE_LOOP('',(#76295,#76296,#76297)) ;
#27939=EDGE_LOOP('',(#76298,#76299,#76300)) ;
#27940=EDGE_LOOP('',(#76301,#76302,#76303,#76304)) ;
#27941=EDGE_LOOP('',(#76305,#76306,#76307,#76308)) ;
#27942=EDGE_LOOP('',(#76309,#76310,#76311,#76312)) ;
#27943=EDGE_LOOP('',(#76313,#76314,#76315,#76316)) ;
#27944=EDGE_LOOP('',(#76317,#76318,#76319)) ;
#27945=EDGE_LOOP('',(#76320,#76321,#76322)) ;
#27946=EDGE_LOOP('',(#76323,#76324,#76325,#76326)) ;
#27947=EDGE_LOOP('',(#76327,#76328,#76329,#76330)) ;
#27948=EDGE_LOOP('',(#76331,#76332,#76333,#76334)) ;
#27949=EDGE_LOOP('',(#76335,#76336,#76337,#76338)) ;
#27950=EDGE_LOOP('',(#76339,#76340,#76341,#76342)) ;
#27951=EDGE_LOOP('',(#76343,#76344,#76345,#76346)) ;
#27952=EDGE_LOOP('',(#76347,#76348,#76349,#76350)) ;
#27953=EDGE_LOOP('',(#76351,#76352,#76353,#76354)) ;
#27954=EDGE_LOOP('',(#76355,#76356,#76357,#76358)) ;
#27955=EDGE_LOOP('',(#76359,#76360,#76361,#76362)) ;
#27956=EDGE_LOOP('',(#76363,#76364,#76365,#76366)) ;
#27957=EDGE_LOOP('',(#76367,#76368,#76369)) ;
#27958=EDGE_LOOP('',(#76370,#76371,#76372)) ;
#27959=EDGE_LOOP('',(#76373,#76374,#76375,#76376)) ;
#27960=EDGE_LOOP('',(#76377,#76378,#76379,#76380)) ;
#27961=EDGE_LOOP('',(#76381,#76382,#76383,#76384)) ;
#27962=EDGE_LOOP('',(#76385,#76386,#76387,#76388)) ;
#27963=EDGE_LOOP('',(#76389,#76390,#76391,#76392)) ;
#27964=EDGE_LOOP('',(#76393,#76394,#76395)) ;
#27965=EDGE_LOOP('',(#76396,#76397,#76398)) ;
#27966=EDGE_LOOP('',(#76399,#76400,#76401,#76402)) ;
#27967=EDGE_LOOP('',(#76403,#76404,#76405,#76406)) ;
#27968=EDGE_LOOP('',(#76407,#76408,#76409,#76410)) ;
#27969=EDGE_LOOP('',(#76411,#76412,#76413,#76414)) ;
#27970=EDGE_LOOP('',(#76415,#76416,#76417)) ;
#27971=EDGE_LOOP('',(#76418,#76419,#76420)) ;
#27972=EDGE_LOOP('',(#76421,#76422,#76423,#76424)) ;
#27973=EDGE_LOOP('',(#76425,#76426,#76427,#76428)) ;
#27974=EDGE_LOOP('',(#76429,#76430,#76431,#76432)) ;
#27975=EDGE_LOOP('',(#76433,#76434,#76435,#76436)) ;
#27976=EDGE_LOOP('',(#76437,#76438,#76439)) ;
#27977=EDGE_LOOP('',(#76440,#76441,#76442)) ;
#27978=EDGE_LOOP('',(#76443,#76444,#76445,#76446)) ;
#27979=EDGE_LOOP('',(#76447,#76448,#76449,#76450)) ;
#27980=EDGE_LOOP('',(#76451,#76452,#76453)) ;
#27981=EDGE_LOOP('',(#76454,#76455,#76456)) ;
#27982=EDGE_LOOP('',(#76457,#76458,#76459,#76460)) ;
#27983=EDGE_LOOP('',(#76461,#76462,#76463,#76464)) ;
#27984=EDGE_LOOP('',(#76465,#76466,#76467)) ;
#27985=EDGE_LOOP('',(#76468,#76469,#76470)) ;
#27986=EDGE_LOOP('',(#76471,#76472,#76473,#76474)) ;
#27987=EDGE_LOOP('',(#76475,#76476,#76477,#76478)) ;
#27988=EDGE_LOOP('',(#76479,#76480,#76481,#76482)) ;
#27989=EDGE_LOOP('',(#76483,#76484,#76485,#76486)) ;
#27990=EDGE_LOOP('',(#76487,#76488,#76489,#76490)) ;
#27991=EDGE_LOOP('',(#76491,#76492,#76493)) ;
#27992=EDGE_LOOP('',(#76494,#76495,#76496,#76497)) ;
#27993=EDGE_LOOP('',(#76498,#76499,#76500,#76501)) ;
#27994=EDGE_LOOP('',(#76502,#76503,#76504,#76505)) ;
#27995=EDGE_LOOP('',(#76506,#76507,#76508,#76509)) ;
#27996=EDGE_LOOP('',(#76510,#76511,#76512)) ;
#27997=EDGE_LOOP('',(#76513,#76514,#76515,#76516)) ;
#27998=EDGE_LOOP('',(#76517,#76518,#76519)) ;
#27999=EDGE_LOOP('',(#76520,#76521,#76522,#76523)) ;
#28000=EDGE_LOOP('',(#76524,#76525,#76526,#76527)) ;
#28001=EDGE_LOOP('',(#76528,#76529,#76530,#76531)) ;
#28002=EDGE_LOOP('',(#76532,#76533,#76534,#76535)) ;
#28003=EDGE_LOOP('',(#76536,#76537,#76538,#76539)) ;
#28004=EDGE_LOOP('',(#76540,#76541,#76542,#76543)) ;
#28005=EDGE_LOOP('',(#76544,#76545,#76546,#76547)) ;
#28006=EDGE_LOOP('',(#76548,#76549,#76550,#76551)) ;
#28007=EDGE_LOOP('',(#76552,#76553,#76554,#76555)) ;
#28008=EDGE_LOOP('',(#76556,#76557,#76558)) ;
#28009=EDGE_LOOP('',(#76559,#76560,#76561,#76562)) ;
#28010=EDGE_LOOP('',(#76563,#76564,#76565,#76566)) ;
#28011=EDGE_LOOP('',(#76567,#76568,#76569,#76570)) ;
#28012=EDGE_LOOP('',(#76571,#76572,#76573,#76574)) ;
#28013=EDGE_LOOP('',(#76575,#76576,#76577)) ;
#28014=EDGE_LOOP('',(#76578,#76579,#76580)) ;
#28015=EDGE_LOOP('',(#76581,#76582,#76583,#76584)) ;
#28016=EDGE_LOOP('',(#76585,#76586,#76587,#76588)) ;
#28017=EDGE_LOOP('',(#76589,#76590,#76591,#76592)) ;
#28018=EDGE_LOOP('',(#76593,#76594,#76595,#76596)) ;
#28019=EDGE_LOOP('',(#76597,#76598,#76599,#76600)) ;
#28020=EDGE_LOOP('',(#76601,#76602,#76603,#76604)) ;
#28021=EDGE_LOOP('',(#76605,#76606,#76607)) ;
#28022=EDGE_LOOP('',(#76608,#76609,#76610,#76611)) ;
#28023=EDGE_LOOP('',(#76612,#76613,#76614,#76615)) ;
#28024=EDGE_LOOP('',(#76616,#76617,#76618,#76619)) ;
#28025=EDGE_LOOP('',(#76620,#76621,#76622,#76623)) ;
#28026=EDGE_LOOP('',(#76624,#76625,#76626,#76627)) ;
#28027=EDGE_LOOP('',(#76628,#76629,#76630)) ;
#28028=EDGE_LOOP('',(#76631,#76632,#76633,#76634)) ;
#28029=EDGE_LOOP('',(#76635,#76636,#76637,#76638,#76639)) ;
#28030=EDGE_LOOP('',(#76640,#76641,#76642,#76643)) ;
#28031=EDGE_LOOP('',(#76644,#76645,#76646,#76647,#76648)) ;
#28032=EDGE_LOOP('',(#76649,#76650,#76651)) ;
#28033=EDGE_LOOP('',(#76652,#76653,#76654,#76655,#76656)) ;
#28034=EDGE_LOOP('',(#76657,#76658,#76659,#76660)) ;
#28035=EDGE_LOOP('',(#76661,#76662,#76663,#76664)) ;
#28036=EDGE_LOOP('',(#76665,#76666,#76667,#76668)) ;
#28037=EDGE_LOOP('',(#76669,#76670,#76671,#76672)) ;
#28038=EDGE_LOOP('',(#76673,#76674,#76675)) ;
#28039=EDGE_LOOP('',(#76676,#76677,#76678)) ;
#28040=EDGE_LOOP('',(#76679,#76680,#76681,#76682)) ;
#28041=EDGE_LOOP('',(#76683,#76684,#76685,#76686)) ;
#28042=EDGE_LOOP('',(#76687,#76688,#76689)) ;
#28043=EDGE_LOOP('',(#76690,#76691,#76692,#76693)) ;
#28044=EDGE_LOOP('',(#76694,#76695,#76696,#76697,#76698)) ;
#28045=EDGE_LOOP('',(#76699,#76700,#76701,#76702,#76703)) ;
#28046=EDGE_LOOP('',(#76704,#76705,#76706,#76707)) ;
#28047=EDGE_LOOP('',(#76708,#76709,#76710,#76711)) ;
#28048=EDGE_LOOP('',(#76712,#76713,#76714,#76715)) ;
#28049=EDGE_LOOP('',(#76716,#76717,#76718)) ;
#28050=EDGE_LOOP('',(#76719,#76720,#76721,#76722)) ;
#28051=EDGE_LOOP('',(#76723,#76724,#76725,#76726)) ;
#28052=EDGE_LOOP('',(#76727,#76728,#76729)) ;
#28053=EDGE_LOOP('',(#76730,#76731,#76732,#76733)) ;
#28054=EDGE_LOOP('',(#76734,#76735,#76736,#76737)) ;
#28055=EDGE_LOOP('',(#76738,#76739,#76740)) ;
#28056=EDGE_LOOP('',(#76741,#76742,#76743)) ;
#28057=EDGE_LOOP('',(#76744,#76745,#76746,#76747)) ;
#28058=EDGE_LOOP('',(#76748,#76749,#76750,#76751)) ;
#28059=EDGE_LOOP('',(#76752,#76753,#76754,#76755)) ;
#28060=EDGE_LOOP('',(#76756,#76757,#76758)) ;
#28061=EDGE_LOOP('',(#76759,#76760,#76761,#76762)) ;
#28062=EDGE_LOOP('',(#76763,#76764,#76765,#76766)) ;
#28063=EDGE_LOOP('',(#76767,#76768,#76769)) ;
#28064=EDGE_LOOP('',(#76770,#76771,#76772,#76773)) ;
#28065=EDGE_LOOP('',(#76774,#76775,#76776,#76777)) ;
#28066=EDGE_LOOP('',(#76778,#76779,#76780,#76781,#76782)) ;
#28067=EDGE_LOOP('',(#76783,#76784,#76785,#76786)) ;
#28068=EDGE_LOOP('',(#76787,#76788,#76789,#76790)) ;
#28069=EDGE_LOOP('',(#76791,#76792,#76793,#76794)) ;
#28070=EDGE_LOOP('',(#76795,#76796,#76797,#76798)) ;
#28071=EDGE_LOOP('',(#76799,#76800,#76801,#76802)) ;
#28072=EDGE_LOOP('',(#76803,#76804,#76805,#76806)) ;
#28073=EDGE_LOOP('',(#76807,#76808,#76809,#76810)) ;
#28074=EDGE_LOOP('',(#76811,#76812,#76813,#76814)) ;
#28075=EDGE_LOOP('',(#76815,#76816,#76817,#76818)) ;
#28076=EDGE_LOOP('',(#76819,#76820,#76821,#76822)) ;
#28077=EDGE_LOOP('',(#76823,#76824,#76825,#76826)) ;
#28078=EDGE_LOOP('',(#76827,#76828,#76829)) ;
#28079=EDGE_LOOP('',(#76830,#76831,#76832)) ;
#28080=EDGE_LOOP('',(#76833,#76834,#76835,#76836)) ;
#28081=EDGE_LOOP('',(#76837,#76838,#76839,#76840)) ;
#28082=EDGE_LOOP('',(#76841,#76842,#76843,#76844)) ;
#28083=EDGE_LOOP('',(#76845,#76846,#76847,#76848)) ;
#28084=EDGE_LOOP('',(#76849,#76850,#76851)) ;
#28085=EDGE_LOOP('',(#76852,#76853,#76854)) ;
#28086=EDGE_LOOP('',(#76855,#76856,#76857,#76858)) ;
#28087=EDGE_LOOP('',(#76859,#76860,#76861,#76862)) ;
#28088=EDGE_LOOP('',(#76863,#76864,#76865,#76866)) ;
#28089=EDGE_LOOP('',(#76867,#76868,#76869,#76870)) ;
#28090=EDGE_LOOP('',(#76871,#76872,#76873,#76874)) ;
#28091=EDGE_LOOP('',(#76875,#76876,#76877,#76878)) ;
#28092=EDGE_LOOP('',(#76879,#76880,#76881,#76882)) ;
#28093=EDGE_LOOP('',(#76883,#76884,#76885,#76886)) ;
#28094=EDGE_LOOP('',(#76887,#76888,#76889,#76890)) ;
#28095=EDGE_LOOP('',(#76891,#76892,#76893,#76894)) ;
#28096=EDGE_LOOP('',(#76895,#76896,#76897,#76898)) ;
#28097=EDGE_LOOP('',(#76899,#76900,#76901)) ;
#28098=EDGE_LOOP('',(#76902,#76903,#76904)) ;
#28099=EDGE_LOOP('',(#76905,#76906,#76907,#76908)) ;
#28100=EDGE_LOOP('',(#76909,#76910,#76911,#76912)) ;
#28101=EDGE_LOOP('',(#76913,#76914,#76915,#76916)) ;
#28102=EDGE_LOOP('',(#76917,#76918,#76919,#76920)) ;
#28103=EDGE_LOOP('',(#76921,#76922,#76923,#76924)) ;
#28104=EDGE_LOOP('',(#76925,#76926,#76927)) ;
#28105=EDGE_LOOP('',(#76928,#76929,#76930)) ;
#28106=EDGE_LOOP('',(#76931,#76932,#76933,#76934)) ;
#28107=EDGE_LOOP('',(#76935,#76936,#76937,#76938)) ;
#28108=EDGE_LOOP('',(#76939,#76940,#76941,#76942)) ;
#28109=EDGE_LOOP('',(#76943,#76944,#76945,#76946)) ;
#28110=EDGE_LOOP('',(#76947,#76948,#76949)) ;
#28111=EDGE_LOOP('',(#76950,#76951,#76952)) ;
#28112=EDGE_LOOP('',(#76953,#76954,#76955,#76956)) ;
#28113=EDGE_LOOP('',(#76957,#76958,#76959,#76960)) ;
#28114=EDGE_LOOP('',(#76961,#76962,#76963,#76964)) ;
#28115=EDGE_LOOP('',(#76965,#76966,#76967,#76968)) ;
#28116=EDGE_LOOP('',(#76969,#76970,#76971)) ;
#28117=EDGE_LOOP('',(#76972,#76973,#76974)) ;
#28118=EDGE_LOOP('',(#76975,#76976,#76977,#76978)) ;
#28119=EDGE_LOOP('',(#76979,#76980,#76981,#76982)) ;
#28120=EDGE_LOOP('',(#76983,#76984,#76985)) ;
#28121=EDGE_LOOP('',(#76986,#76987,#76988)) ;
#28122=EDGE_LOOP('',(#76989,#76990,#76991,#76992)) ;
#28123=EDGE_LOOP('',(#76993,#76994,#76995,#76996)) ;
#28124=EDGE_LOOP('',(#76997,#76998,#76999)) ;
#28125=EDGE_LOOP('',(#77000,#77001,#77002)) ;
#28126=EDGE_LOOP('',(#77003,#77004,#77005,#77006)) ;
#28127=EDGE_LOOP('',(#77007,#77008,#77009,#77010)) ;
#28128=EDGE_LOOP('',(#77011,#77012,#77013,#77014)) ;
#28129=EDGE_LOOP('',(#77015,#77016,#77017,#77018)) ;
#28130=EDGE_LOOP('',(#77019,#77020,#77021,#77022)) ;
#28131=EDGE_LOOP('',(#77023,#77024,#77025)) ;
#28132=EDGE_LOOP('',(#77026,#77027,#77028,#77029)) ;
#28133=EDGE_LOOP('',(#77030,#77031,#77032,#77033)) ;
#28134=EDGE_LOOP('',(#77034,#77035,#77036,#77037)) ;
#28135=EDGE_LOOP('',(#77038,#77039,#77040,#77041)) ;
#28136=EDGE_LOOP('',(#77042,#77043,#77044)) ;
#28137=EDGE_LOOP('',(#77045,#77046,#77047,#77048)) ;
#28138=EDGE_LOOP('',(#77049,#77050,#77051)) ;
#28139=EDGE_LOOP('',(#77052,#77053,#77054,#77055)) ;
#28140=EDGE_LOOP('',(#77056,#77057,#77058,#77059)) ;
#28141=EDGE_LOOP('',(#77060,#77061,#77062,#77063)) ;
#28142=EDGE_LOOP('',(#77064,#77065,#77066,#77067)) ;
#28143=EDGE_LOOP('',(#77068,#77069,#77070,#77071)) ;
#28144=EDGE_LOOP('',(#77072,#77073,#77074,#77075)) ;
#28145=EDGE_LOOP('',(#77076,#77077,#77078,#77079)) ;
#28146=EDGE_LOOP('',(#77080,#77081,#77082,#77083)) ;
#28147=EDGE_LOOP('',(#77084,#77085,#77086,#77087)) ;
#28148=EDGE_LOOP('',(#77088,#77089,#77090)) ;
#28149=EDGE_LOOP('',(#77091,#77092,#77093,#77094)) ;
#28150=EDGE_LOOP('',(#77095,#77096,#77097,#77098)) ;
#28151=EDGE_LOOP('',(#77099,#77100,#77101,#77102)) ;
#28152=EDGE_LOOP('',(#77103,#77104,#77105,#77106)) ;
#28153=EDGE_LOOP('',(#77107,#77108,#77109)) ;
#28154=EDGE_LOOP('',(#77110,#77111,#77112)) ;
#28155=EDGE_LOOP('',(#77113,#77114,#77115,#77116)) ;
#28156=EDGE_LOOP('',(#77117,#77118,#77119,#77120)) ;
#28157=EDGE_LOOP('',(#77121,#77122,#77123,#77124)) ;
#28158=EDGE_LOOP('',(#77125,#77126,#77127,#77128)) ;
#28159=EDGE_LOOP('',(#77129,#77130,#77131,#77132)) ;
#28160=EDGE_LOOP('',(#77133,#77134,#77135,#77136)) ;
#28161=EDGE_LOOP('',(#77137,#77138,#77139)) ;
#28162=EDGE_LOOP('',(#77140,#77141,#77142,#77143)) ;
#28163=EDGE_LOOP('',(#77144,#77145,#77146,#77147)) ;
#28164=EDGE_LOOP('',(#77148,#77149,#77150,#77151)) ;
#28165=EDGE_LOOP('',(#77152,#77153,#77154,#77155)) ;
#28166=EDGE_LOOP('',(#77156,#77157,#77158,#77159)) ;
#28167=EDGE_LOOP('',(#77160,#77161,#77162)) ;
#28168=EDGE_LOOP('',(#77163,#77164,#77165,#77166)) ;
#28169=EDGE_LOOP('',(#77167,#77168,#77169,#77170,#77171)) ;
#28170=EDGE_LOOP('',(#77172,#77173,#77174,#77175)) ;
#28171=EDGE_LOOP('',(#77176,#77177,#77178,#77179,#77180)) ;
#28172=EDGE_LOOP('',(#77181,#77182,#77183)) ;
#28173=EDGE_LOOP('',(#77184,#77185,#77186,#77187,#77188)) ;
#28174=EDGE_LOOP('',(#77189,#77190,#77191,#77192)) ;
#28175=EDGE_LOOP('',(#77193,#77194,#77195,#77196)) ;
#28176=EDGE_LOOP('',(#77197,#77198,#77199,#77200)) ;
#28177=EDGE_LOOP('',(#77201,#77202,#77203,#77204)) ;
#28178=EDGE_LOOP('',(#77205,#77206,#77207)) ;
#28179=EDGE_LOOP('',(#77208,#77209,#77210)) ;
#28180=EDGE_LOOP('',(#77211,#77212,#77213,#77214)) ;
#28181=EDGE_LOOP('',(#77215,#77216,#77217,#77218)) ;
#28182=EDGE_LOOP('',(#77219,#77220,#77221)) ;
#28183=EDGE_LOOP('',(#77222,#77223,#77224,#77225)) ;
#28184=EDGE_LOOP('',(#77226,#77227,#77228,#77229,#77230)) ;
#28185=EDGE_LOOP('',(#77231,#77232,#77233,#77234,#77235)) ;
#28186=EDGE_LOOP('',(#77236,#77237,#77238,#77239)) ;
#28187=EDGE_LOOP('',(#77240,#77241,#77242,#77243)) ;
#28188=EDGE_LOOP('',(#77244,#77245,#77246,#77247)) ;
#28189=EDGE_LOOP('',(#77248,#77249,#77250)) ;
#28190=EDGE_LOOP('',(#77251,#77252,#77253,#77254)) ;
#28191=EDGE_LOOP('',(#77255,#77256,#77257,#77258)) ;
#28192=EDGE_LOOP('',(#77259,#77260,#77261)) ;
#28193=EDGE_LOOP('',(#77262,#77263,#77264,#77265)) ;
#28194=EDGE_LOOP('',(#77266,#77267,#77268,#77269)) ;
#28195=EDGE_LOOP('',(#77270,#77271,#77272)) ;
#28196=EDGE_LOOP('',(#77273,#77274,#77275)) ;
#28197=EDGE_LOOP('',(#77276,#77277,#77278,#77279)) ;
#28198=EDGE_LOOP('',(#77280,#77281,#77282,#77283)) ;
#28199=EDGE_LOOP('',(#77284,#77285,#77286,#77287)) ;
#28200=EDGE_LOOP('',(#77288,#77289,#77290)) ;
#28201=EDGE_LOOP('',(#77291,#77292,#77293,#77294)) ;
#28202=EDGE_LOOP('',(#77295,#77296,#77297,#77298)) ;
#28203=EDGE_LOOP('',(#77299,#77300,#77301)) ;
#28204=EDGE_LOOP('',(#77302,#77303,#77304,#77305)) ;
#28205=EDGE_LOOP('',(#77306,#77307,#77308,#77309)) ;
#28206=EDGE_LOOP('',(#77310,#77311,#77312,#77313,#77314)) ;
#28207=EDGE_LOOP('',(#77315,#77316,#77317,#77318)) ;
#28208=EDGE_LOOP('',(#77319,#77320,#77321,#77322)) ;
#28209=EDGE_LOOP('',(#77323,#77324,#77325,#77326)) ;
#28210=EDGE_LOOP('',(#77327,#77328,#77329,#77330)) ;
#28211=EDGE_LOOP('',(#77331,#77332,#77333,#77334)) ;
#28212=EDGE_LOOP('',(#77335,#77336,#77337,#77338)) ;
#28213=EDGE_LOOP('',(#77339,#77340,#77341,#77342)) ;
#28214=EDGE_LOOP('',(#77343,#77344,#77345,#77346)) ;
#28215=EDGE_LOOP('',(#77347,#77348,#77349,#77350)) ;
#28216=EDGE_LOOP('',(#77351,#77352,#77353,#77354)) ;
#28217=EDGE_LOOP('',(#77355,#77356,#77357,#77358)) ;
#28218=EDGE_LOOP('',(#77359,#77360,#77361)) ;
#28219=EDGE_LOOP('',(#77362,#77363,#77364)) ;
#28220=EDGE_LOOP('',(#77365,#77366,#77367,#77368)) ;
#28221=EDGE_LOOP('',(#77369,#77370,#77371,#77372)) ;
#28222=EDGE_LOOP('',(#77373,#77374,#77375,#77376)) ;
#28223=EDGE_LOOP('',(#77377,#77378,#77379,#77380)) ;
#28224=EDGE_LOOP('',(#77381,#77382,#77383)) ;
#28225=EDGE_LOOP('',(#77384,#77385,#77386)) ;
#28226=EDGE_LOOP('',(#77387,#77388,#77389,#77390)) ;
#28227=EDGE_LOOP('',(#77391,#77392,#77393,#77394)) ;
#28228=EDGE_LOOP('',(#77395,#77396,#77397,#77398)) ;
#28229=EDGE_LOOP('',(#77399,#77400,#77401,#77402)) ;
#28230=EDGE_LOOP('',(#77403,#77404,#77405,#77406)) ;
#28231=EDGE_LOOP('',(#77407,#77408,#77409,#77410)) ;
#28232=EDGE_LOOP('',(#77411,#77412,#77413,#77414)) ;
#28233=EDGE_LOOP('',(#77415,#77416,#77417,#77418)) ;
#28234=EDGE_LOOP('',(#77419,#77420,#77421,#77422)) ;
#28235=EDGE_LOOP('',(#77423,#77424,#77425,#77426)) ;
#28236=EDGE_LOOP('',(#77427,#77428,#77429,#77430)) ;
#28237=EDGE_LOOP('',(#77431,#77432,#77433)) ;
#28238=EDGE_LOOP('',(#77434,#77435,#77436)) ;
#28239=EDGE_LOOP('',(#77437,#77438,#77439,#77440)) ;
#28240=EDGE_LOOP('',(#77441,#77442,#77443,#77444)) ;
#28241=EDGE_LOOP('',(#77445,#77446,#77447,#77448)) ;
#28242=EDGE_LOOP('',(#77449,#77450,#77451,#77452)) ;
#28243=EDGE_LOOP('',(#77453,#77454,#77455,#77456)) ;
#28244=EDGE_LOOP('',(#77457,#77458,#77459)) ;
#28245=EDGE_LOOP('',(#77460,#77461,#77462)) ;
#28246=EDGE_LOOP('',(#77463,#77464,#77465,#77466)) ;
#28247=EDGE_LOOP('',(#77467,#77468,#77469,#77470)) ;
#28248=EDGE_LOOP('',(#77471,#77472,#77473,#77474)) ;
#28249=EDGE_LOOP('',(#77475,#77476,#77477,#77478)) ;
#28250=EDGE_LOOP('',(#77479,#77480,#77481)) ;
#28251=EDGE_LOOP('',(#77482,#77483,#77484)) ;
#28252=EDGE_LOOP('',(#77485,#77486,#77487,#77488)) ;
#28253=EDGE_LOOP('',(#77489,#77490,#77491,#77492)) ;
#28254=EDGE_LOOP('',(#77493,#77494,#77495,#77496)) ;
#28255=EDGE_LOOP('',(#77497,#77498,#77499,#77500)) ;
#28256=EDGE_LOOP('',(#77501,#77502,#77503)) ;
#28257=EDGE_LOOP('',(#77504,#77505,#77506)) ;
#28258=EDGE_LOOP('',(#77507,#77508,#77509,#77510)) ;
#28259=EDGE_LOOP('',(#77511,#77512,#77513,#77514)) ;
#28260=EDGE_LOOP('',(#77515,#77516,#77517)) ;
#28261=EDGE_LOOP('',(#77518,#77519,#77520)) ;
#28262=EDGE_LOOP('',(#77521,#77522,#77523,#77524)) ;
#28263=EDGE_LOOP('',(#77525,#77526,#77527,#77528)) ;
#28264=EDGE_LOOP('',(#77529,#77530,#77531)) ;
#28265=EDGE_LOOP('',(#77532,#77533,#77534)) ;
#28266=EDGE_LOOP('',(#77535,#77536,#77537,#77538)) ;
#28267=EDGE_LOOP('',(#77539,#77540,#77541,#77542)) ;
#28268=EDGE_LOOP('',(#77543,#77544,#77545,#77546)) ;
#28269=EDGE_LOOP('',(#77547,#77548,#77549,#77550)) ;
#28270=EDGE_LOOP('',(#77551,#77552,#77553,#77554)) ;
#28271=EDGE_LOOP('',(#77555,#77556,#77557)) ;
#28272=EDGE_LOOP('',(#77558,#77559,#77560,#77561)) ;
#28273=EDGE_LOOP('',(#77562,#77563,#77564,#77565)) ;
#28274=EDGE_LOOP('',(#77566,#77567,#77568,#77569)) ;
#28275=EDGE_LOOP('',(#77570,#77571,#77572,#77573)) ;
#28276=EDGE_LOOP('',(#77574,#77575,#77576)) ;
#28277=EDGE_LOOP('',(#77577,#77578,#77579,#77580)) ;
#28278=EDGE_LOOP('',(#77581,#77582,#77583)) ;
#28279=EDGE_LOOP('',(#77584,#77585,#77586,#77587)) ;
#28280=EDGE_LOOP('',(#77588,#77589,#77590,#77591)) ;
#28281=EDGE_LOOP('',(#77592,#77593,#77594,#77595)) ;
#28282=EDGE_LOOP('',(#77596,#77597,#77598,#77599)) ;
#28283=EDGE_LOOP('',(#77600,#77601,#77602,#77603)) ;
#28284=EDGE_LOOP('',(#77604,#77605,#77606,#77607)) ;
#28285=EDGE_LOOP('',(#77608,#77609,#77610,#77611)) ;
#28286=EDGE_LOOP('',(#77612,#77613,#77614,#77615)) ;
#28287=EDGE_LOOP('',(#77616,#77617,#77618,#77619)) ;
#28288=EDGE_LOOP('',(#77620,#77621,#77622)) ;
#28289=EDGE_LOOP('',(#77623,#77624,#77625,#77626)) ;
#28290=EDGE_LOOP('',(#77627,#77628,#77629,#77630)) ;
#28291=EDGE_LOOP('',(#77631,#77632,#77633,#77634)) ;
#28292=EDGE_LOOP('',(#77635,#77636,#77637,#77638)) ;
#28293=EDGE_LOOP('',(#77639,#77640,#77641)) ;
#28294=EDGE_LOOP('',(#77642,#77643,#77644)) ;
#28295=EDGE_LOOP('',(#77645,#77646,#77647,#77648)) ;
#28296=EDGE_LOOP('',(#77649,#77650,#77651,#77652)) ;
#28297=EDGE_LOOP('',(#77653,#77654,#77655,#77656)) ;
#28298=EDGE_LOOP('',(#77657,#77658,#77659,#77660)) ;
#28299=EDGE_LOOP('',(#77661,#77662,#77663,#77664)) ;
#28300=EDGE_LOOP('',(#77665,#77666,#77667,#77668)) ;
#28301=EDGE_LOOP('',(#77669,#77670,#77671)) ;
#28302=EDGE_LOOP('',(#77672,#77673,#77674,#77675)) ;
#28303=EDGE_LOOP('',(#77676,#77677,#77678,#77679)) ;
#28304=EDGE_LOOP('',(#77680,#77681,#77682,#77683)) ;
#28305=EDGE_LOOP('',(#77684,#77685,#77686,#77687)) ;
#28306=EDGE_LOOP('',(#77688,#77689,#77690,#77691)) ;
#28307=EDGE_LOOP('',(#77692,#77693,#77694)) ;
#28308=EDGE_LOOP('',(#77695,#77696,#77697,#77698)) ;
#28309=EDGE_LOOP('',(#77699,#77700,#77701,#77702,#77703)) ;
#28310=EDGE_LOOP('',(#77704,#77705,#77706,#77707)) ;
#28311=EDGE_LOOP('',(#77708,#77709,#77710,#77711,#77712)) ;
#28312=EDGE_LOOP('',(#77713,#77714,#77715)) ;
#28313=EDGE_LOOP('',(#77716,#77717,#77718,#77719,#77720)) ;
#28314=EDGE_LOOP('',(#77721,#77722,#77723,#77724)) ;
#28315=EDGE_LOOP('',(#77725,#77726,#77727,#77728)) ;
#28316=EDGE_LOOP('',(#77729,#77730,#77731,#77732)) ;
#28317=EDGE_LOOP('',(#77733,#77734,#77735,#77736)) ;
#28318=EDGE_LOOP('',(#77737,#77738,#77739)) ;
#28319=EDGE_LOOP('',(#77740,#77741,#77742)) ;
#28320=EDGE_LOOP('',(#77743,#77744,#77745,#77746)) ;
#28321=EDGE_LOOP('',(#77747,#77748,#77749,#77750)) ;
#28322=EDGE_LOOP('',(#77751,#77752,#77753)) ;
#28323=EDGE_LOOP('',(#77754,#77755,#77756,#77757)) ;
#28324=EDGE_LOOP('',(#77758,#77759,#77760,#77761,#77762)) ;
#28325=EDGE_LOOP('',(#77763,#77764,#77765,#77766,#77767)) ;
#28326=EDGE_LOOP('',(#77768,#77769,#77770,#77771)) ;
#28327=EDGE_LOOP('',(#77772,#77773,#77774,#77775)) ;
#28328=EDGE_LOOP('',(#77776,#77777,#77778,#77779)) ;
#28329=EDGE_LOOP('',(#77780,#77781,#77782)) ;
#28330=EDGE_LOOP('',(#77783,#77784,#77785,#77786)) ;
#28331=EDGE_LOOP('',(#77787,#77788,#77789,#77790)) ;
#28332=EDGE_LOOP('',(#77791,#77792,#77793)) ;
#28333=EDGE_LOOP('',(#77794,#77795,#77796,#77797)) ;
#28334=EDGE_LOOP('',(#77798,#77799,#77800,#77801)) ;
#28335=EDGE_LOOP('',(#77802,#77803,#77804)) ;
#28336=EDGE_LOOP('',(#77805,#77806,#77807)) ;
#28337=EDGE_LOOP('',(#77808,#77809,#77810,#77811)) ;
#28338=EDGE_LOOP('',(#77812,#77813,#77814,#77815)) ;
#28339=EDGE_LOOP('',(#77816,#77817,#77818,#77819)) ;
#28340=EDGE_LOOP('',(#77820,#77821,#77822)) ;
#28341=EDGE_LOOP('',(#77823,#77824,#77825,#77826)) ;
#28342=EDGE_LOOP('',(#77827,#77828,#77829,#77830)) ;
#28343=EDGE_LOOP('',(#77831,#77832,#77833)) ;
#28344=EDGE_LOOP('',(#77834,#77835,#77836,#77837)) ;
#28345=EDGE_LOOP('',(#77838,#77839,#77840,#77841)) ;
#28346=EDGE_LOOP('',(#77842,#77843,#77844,#77845,#77846)) ;
#28347=EDGE_LOOP('',(#77847,#77848,#77849,#77850)) ;
#28348=EDGE_LOOP('',(#77851,#77852,#77853,#77854)) ;
#28349=EDGE_LOOP('',(#77855,#77856,#77857,#77858)) ;
#28350=EDGE_LOOP('',(#77859,#77860,#77861,#77862)) ;
#28351=EDGE_LOOP('',(#77863,#77864,#77865,#77866)) ;
#28352=EDGE_LOOP('',(#77867,#77868,#77869,#77870)) ;
#28353=EDGE_LOOP('',(#77871,#77872,#77873,#77874)) ;
#28354=EDGE_LOOP('',(#77875,#77876,#77877,#77878)) ;
#28355=EDGE_LOOP('',(#77879,#77880,#77881,#77882)) ;
#28356=EDGE_LOOP('',(#77883,#77884,#77885,#77886)) ;
#28357=EDGE_LOOP('',(#77887,#77888,#77889,#77890)) ;
#28358=EDGE_LOOP('',(#77891,#77892,#77893)) ;
#28359=EDGE_LOOP('',(#77894,#77895,#77896)) ;
#28360=EDGE_LOOP('',(#77897,#77898,#77899,#77900)) ;
#28361=EDGE_LOOP('',(#77901,#77902,#77903,#77904)) ;
#28362=EDGE_LOOP('',(#77905,#77906,#77907,#77908)) ;
#28363=EDGE_LOOP('',(#77909,#77910,#77911,#77912)) ;
#28364=EDGE_LOOP('',(#77913,#77914,#77915)) ;
#28365=EDGE_LOOP('',(#77916,#77917,#77918)) ;
#28366=EDGE_LOOP('',(#77919,#77920,#77921,#77922)) ;
#28367=EDGE_LOOP('',(#77923,#77924,#77925,#77926)) ;
#28368=EDGE_LOOP('',(#77927,#77928,#77929,#77930)) ;
#28369=EDGE_LOOP('',(#77931,#77932,#77933,#77934)) ;
#28370=EDGE_LOOP('',(#77935,#77936,#77937,#77938)) ;
#28371=EDGE_LOOP('',(#77939,#77940,#77941,#77942)) ;
#28372=EDGE_LOOP('',(#77943,#77944,#77945,#77946)) ;
#28373=EDGE_LOOP('',(#77947,#77948,#77949,#77950)) ;
#28374=EDGE_LOOP('',(#77951,#77952,#77953,#77954)) ;
#28375=EDGE_LOOP('',(#77955,#77956,#77957,#77958)) ;
#28376=EDGE_LOOP('',(#77959,#77960,#77961,#77962)) ;
#28377=EDGE_LOOP('',(#77963,#77964,#77965)) ;
#28378=EDGE_LOOP('',(#77966,#77967,#77968)) ;
#28379=EDGE_LOOP('',(#77969,#77970,#77971,#77972)) ;
#28380=EDGE_LOOP('',(#77973,#77974,#77975,#77976)) ;
#28381=EDGE_LOOP('',(#77977,#77978,#77979,#77980)) ;
#28382=EDGE_LOOP('',(#77981,#77982,#77983,#77984)) ;
#28383=EDGE_LOOP('',(#77985,#77986,#77987,#77988)) ;
#28384=EDGE_LOOP('',(#77989,#77990,#77991)) ;
#28385=EDGE_LOOP('',(#77992,#77993,#77994)) ;
#28386=EDGE_LOOP('',(#77995,#77996,#77997,#77998)) ;
#28387=EDGE_LOOP('',(#77999,#78000,#78001,#78002)) ;
#28388=EDGE_LOOP('',(#78003,#78004,#78005,#78006)) ;
#28389=EDGE_LOOP('',(#78007,#78008,#78009,#78010)) ;
#28390=EDGE_LOOP('',(#78011,#78012,#78013)) ;
#28391=EDGE_LOOP('',(#78014,#78015,#78016)) ;
#28392=EDGE_LOOP('',(#78017,#78018,#78019,#78020)) ;
#28393=EDGE_LOOP('',(#78021,#78022,#78023,#78024)) ;
#28394=EDGE_LOOP('',(#78025,#78026,#78027,#78028)) ;
#28395=EDGE_LOOP('',(#78029,#78030,#78031,#78032)) ;
#28396=EDGE_LOOP('',(#78033,#78034,#78035)) ;
#28397=EDGE_LOOP('',(#78036,#78037,#78038)) ;
#28398=EDGE_LOOP('',(#78039,#78040,#78041,#78042)) ;
#28399=EDGE_LOOP('',(#78043,#78044,#78045,#78046)) ;
#28400=EDGE_LOOP('',(#78047,#78048,#78049)) ;
#28401=EDGE_LOOP('',(#78050,#78051,#78052)) ;
#28402=EDGE_LOOP('',(#78053,#78054,#78055,#78056)) ;
#28403=EDGE_LOOP('',(#78057,#78058,#78059,#78060)) ;
#28404=EDGE_LOOP('',(#78061,#78062,#78063)) ;
#28405=EDGE_LOOP('',(#78064,#78065,#78066)) ;
#28406=EDGE_LOOP('',(#78067,#78068,#78069,#78070)) ;
#28407=EDGE_LOOP('',(#78071,#78072,#78073,#78074)) ;
#28408=EDGE_LOOP('',(#78075,#78076,#78077,#78078)) ;
#28409=EDGE_LOOP('',(#78079,#78080,#78081,#78082)) ;
#28410=EDGE_LOOP('',(#78083,#78084,#78085,#78086)) ;
#28411=EDGE_LOOP('',(#78087,#78088,#78089,#78090)) ;
#28412=EDGE_LOOP('',(#78091,#78092,#78093,#78094)) ;
#28413=EDGE_LOOP('',(#78095,#78096,#78097,#78098)) ;
#28414=EDGE_LOOP('',(#78099,#78100,#78101,#78102)) ;
#28415=EDGE_LOOP('',(#78103,#78104,#78105,#78106)) ;
#28416=EDGE_LOOP('',(#78107,#78108,#78109,#78110)) ;
#28417=EDGE_LOOP('',(#78111,#78112,#78113,#78114)) ;
#28418=EDGE_LOOP('',(#78115,#78116,#78117,#78118)) ;
#28419=EDGE_LOOP('',(#78119,#78120,#78121,#78122)) ;
#28420=EDGE_LOOP('',(#78123,#78124,#78125)) ;
#28421=EDGE_LOOP('',(#78126,#78127,#78128,#78129,#78130,#78131)) ;
#28422=EDGE_LOOP('',(#78132,#78133,#78134)) ;
#28423=EDGE_LOOP('',(#78135,#78136,#78137)) ;
#28424=EDGE_LOOP('',(#78138,#78139,#78140)) ;
#28425=EDGE_LOOP('',(#78141,#78142,#78143,#78144,#78145,#78146)) ;
#28426=EDGE_LOOP('',(#78147,#78148,#78149)) ;
#28427=EDGE_LOOP('',(#78150,#78151,#78152)) ;
#28428=EDGE_LOOP('',(#78153,#78154,#78155,#78156,#78157,#78158)) ;
#28429=EDGE_LOOP('',(#78159,#78160,#78161)) ;
#28430=EDGE_LOOP('',(#78162,#78163,#78164)) ;
#28431=EDGE_LOOP('',(#78165,#78166,#78167,#78168,#78169,#78170)) ;
#28432=EDGE_LOOP('',(#78171,#78172,#78173)) ;
#28433=EDGE_LOOP('',(#78174,#78175,#78176)) ;
#28434=EDGE_LOOP('',(#78177,#78178,#78179,#78180,#78181,#78182)) ;
#28435=EDGE_LOOP('',(#78183,#78184,#78185)) ;
#28436=EDGE_LOOP('',(#78186,#78187,#78188)) ;
#28437=EDGE_LOOP('',(#78189,#78190,#78191,#78192,#78193,#78194)) ;
#28438=EDGE_LOOP('',(#78195,#78196,#78197)) ;
#28439=EDGE_LOOP('',(#78198,#78199,#78200)) ;
#28440=EDGE_LOOP('',(#78201,#78202,#78203,#78204,#78205,#78206)) ;
#28441=EDGE_LOOP('',(#78207,#78208,#78209)) ;
#28442=EDGE_LOOP('',(#78210,#78211,#78212)) ;
#28443=EDGE_LOOP('',(#78213,#78214,#78215,#78216,#78217,#78218)) ;
#28444=EDGE_LOOP('',(#78219,#78220,#78221)) ;
#28445=EDGE_LOOP('',(#78222,#78223,#78224,#78225,#78226)) ;
#28446=EDGE_LOOP('',(#78227,#78228,#78229)) ;
#28447=EDGE_LOOP('',(#78230,#78231,#78232)) ;
#28448=EDGE_LOOP('',(#78233,#78234,#78235,#78236,#78237)) ;
#28449=EDGE_LOOP('',(#78238,#78239,#78240)) ;
#28450=EDGE_LOOP('',(#78241,#78242,#78243)) ;
#28451=EDGE_LOOP('',(#78244,#78245,#78246,#78247,#78248)) ;
#28452=EDGE_LOOP('',(#78249,#78250,#78251)) ;
#28453=EDGE_LOOP('',(#78252,#78253,#78254)) ;
#28454=EDGE_LOOP('',(#78255,#78256,#78257,#78258,#78259)) ;
#28455=EDGE_LOOP('',(#78260,#78261,#78262)) ;
#28456=EDGE_LOOP('',(#78263,#78264,#78265)) ;
#28457=EDGE_LOOP('',(#78266,#78267,#78268,#78269,#78270)) ;
#28458=EDGE_LOOP('',(#78271,#78272,#78273)) ;
#28459=EDGE_LOOP('',(#78274,#78275,#78276)) ;
#28460=EDGE_LOOP('',(#78277,#78278,#78279,#78280,#78281)) ;
#28461=EDGE_LOOP('',(#78282,#78283,#78284)) ;
#28462=EDGE_LOOP('',(#78285,#78286,#78287)) ;
#28463=EDGE_LOOP('',(#78288,#78289,#78290,#78291,#78292)) ;
#28464=EDGE_LOOP('',(#78293,#78294,#78295)) ;
#28465=EDGE_LOOP('',(#78296,#78297,#78298)) ;
#28466=EDGE_LOOP('',(#78299,#78300,#78301,#78302,#78303)) ;
#28467=EDGE_LOOP('',(#78304,#78305,#78306)) ;
#28468=EDGE_LOOP('',(#78307,#78308,#78309)) ;
#28469=EDGE_LOOP('',(#78310,#78311,#78312,#78313,#78314)) ;
#28470=EDGE_LOOP('',(#78315,#78316,#78317)) ;
#28471=EDGE_LOOP('',(#78318,#78319,#78320)) ;
#28472=EDGE_LOOP('',(#78321,#78322,#78323,#78324,#78325)) ;
#28473=EDGE_LOOP('',(#78326,#78327,#78328)) ;
#28474=EDGE_LOOP('',(#78329,#78330,#78331)) ;
#28475=EDGE_LOOP('',(#78332,#78333,#78334,#78335,#78336)) ;
#28476=EDGE_LOOP('',(#78337,#78338,#78339)) ;
#28477=EDGE_LOOP('',(#78340,#78341,#78342)) ;
#28478=EDGE_LOOP('',(#78343,#78344,#78345,#78346,#78347)) ;
#28479=EDGE_LOOP('',(#78348,#78349,#78350)) ;
#28480=EDGE_LOOP('',(#78351,#78352,#78353)) ;
#28481=EDGE_LOOP('',(#78354,#78355,#78356,#78357,#78358)) ;
#28482=EDGE_LOOP('',(#78359,#78360,#78361)) ;
#28483=EDGE_LOOP('',(#78362,#78363,#78364)) ;
#28484=EDGE_LOOP('',(#78365,#78366,#78367,#78368,#78369)) ;
#28485=EDGE_LOOP('',(#78370,#78371,#78372)) ;
#28486=EDGE_LOOP('',(#78373,#78374,#78375)) ;
#28487=EDGE_LOOP('',(#78376,#78377,#78378,#78379,#78380)) ;
#28488=EDGE_LOOP('',(#78381,#78382,#78383)) ;
#28489=EDGE_LOOP('',(#78384,#78385,#78386)) ;
#28490=EDGE_LOOP('',(#78387,#78388,#78389,#78390,#78391)) ;
#28491=EDGE_LOOP('',(#78392,#78393,#78394)) ;
#28492=EDGE_LOOP('',(#78395,#78396,#78397)) ;
#28493=EDGE_LOOP('',(#78398,#78399,#78400,#78401,#78402)) ;
#28494=EDGE_LOOP('',(#78403,#78404,#78405)) ;
#28495=EDGE_LOOP('',(#78406,#78407,#78408)) ;
#28496=EDGE_LOOP('',(#78409,#78410,#78411,#78412,#78413)) ;
#28497=EDGE_LOOP('',(#78414,#78415,#78416)) ;
#28498=EDGE_LOOP('',(#78417,#78418,#78419)) ;
#28499=EDGE_LOOP('',(#78420,#78421,#78422,#78423,#78424)) ;
#28500=EDGE_LOOP('',(#78425,#78426,#78427)) ;
#28501=EDGE_LOOP('',(#78428,#78429,#78430,#78431)) ;
#28502=EDGE_LOOP('',(#78432,#78433,#78434,#78435)) ;
#28503=EDGE_LOOP('',(#78436,#78437,#78438,#78439)) ;
#28504=EDGE_LOOP('',(#78440,#78441,#78442,#78443)) ;
#28505=EDGE_LOOP('',(#78444,#78445,#78446,#78447)) ;
#28506=EDGE_LOOP('',(#78448,#78449,#78450,#78451)) ;
#28507=EDGE_LOOP('',(#78452,#78453,#78454,#78455)) ;
#28508=EDGE_LOOP('',(#78456,#78457,#78458,#78459)) ;
#28509=EDGE_LOOP('',(#78460,#78461,#78462,#78463)) ;
#28510=EDGE_LOOP('',(#78464,#78465,#78466,#78467)) ;
#28511=EDGE_LOOP('',(#78468,#78469,#78470,#78471)) ;
#28512=EDGE_LOOP('',(#78472,#78473,#78474,#78475)) ;
#28513=EDGE_LOOP('',(#78476,#78477,#78478,#78479)) ;
#28514=EDGE_LOOP('',(#78480,#78481,#78482,#78483)) ;
#28515=EDGE_LOOP('',(#78484,#78485,#78486,#78487)) ;
#28516=EDGE_LOOP('',(#78488,#78489,#78490,#78491)) ;
#28517=EDGE_LOOP('',(#78492,#78493,#78494,#78495)) ;
#28518=EDGE_LOOP('',(#78496,#78497,#78498,#78499)) ;
#28519=EDGE_LOOP('',(#78500,#78501,#78502,#78503)) ;
#28520=EDGE_LOOP('',(#78504,#78505,#78506,#78507)) ;
#28521=EDGE_LOOP('',(#78508,#78509,#78510,#78511)) ;
#28522=EDGE_LOOP('',(#78512,#78513,#78514,#78515)) ;
#28523=EDGE_LOOP('',(#78516,#78517,#78518,#78519)) ;
#28524=EDGE_LOOP('',(#78520,#78521,#78522,#78523)) ;
#28525=EDGE_LOOP('',(#78524,#78525,#78526,#78527)) ;
#28526=EDGE_LOOP('',(#78528,#78529,#78530,#78531)) ;
#28527=EDGE_LOOP('',(#78532,#78533,#78534,#78535)) ;
#28528=EDGE_LOOP('',(#78536,#78537,#78538,#78539)) ;
#28529=EDGE_LOOP('',(#78540,#78541,#78542,#78543)) ;
#28530=EDGE_LOOP('',(#78544,#78545,#78546,#78547)) ;
#28531=EDGE_LOOP('',(#78548,#78549,#78550,#78551)) ;
#28532=EDGE_LOOP('',(#78552,#78553,#78554,#78555)) ;
#28533=EDGE_LOOP('',(#78556,#78557,#78558,#78559)) ;
#28534=EDGE_LOOP('',(#78560,#78561,#78562,#78563)) ;
#28535=EDGE_LOOP('',(#78564,#78565,#78566,#78567)) ;
#28536=EDGE_LOOP('',(#78568,#78569,#78570,#78571)) ;
#28537=EDGE_LOOP('',(#78572,#78573,#78574,#78575)) ;
#28538=EDGE_LOOP('',(#78576,#78577,#78578,#78579)) ;
#28539=EDGE_LOOP('',(#78580,#78581,#78582,#78583)) ;
#28540=EDGE_LOOP('',(#78584,#78585,#78586,#78587)) ;
#28541=EDGE_LOOP('',(#78588,#78589,#78590,#78591)) ;
#28542=EDGE_LOOP('',(#78592,#78593,#78594,#78595)) ;
#28543=EDGE_LOOP('',(#78596,#78597,#78598,#78599)) ;
#28544=EDGE_LOOP('',(#78600,#78601,#78602,#78603)) ;
#28545=EDGE_LOOP('',(#78604,#78605,#78606,#78607)) ;
#28546=EDGE_LOOP('',(#78608,#78609,#78610,#78611)) ;
#28547=EDGE_LOOP('',(#78612,#78613,#78614,#78615)) ;
#28548=EDGE_LOOP('',(#78616,#78617,#78618,#78619)) ;
#28549=EDGE_LOOP('',(#78620,#78621,#78622,#78623)) ;
#28550=EDGE_LOOP('',(#78624,#78625,#78626,#78627)) ;
#28551=EDGE_LOOP('',(#78628,#78629,#78630,#78631)) ;
#28552=EDGE_LOOP('',(#78632,#78633,#78634,#78635)) ;
#28553=EDGE_LOOP('',(#78636,#78637,#78638,#78639)) ;
#28554=EDGE_LOOP('',(#78640,#78641,#78642,#78643)) ;
#28555=EDGE_LOOP('',(#78644,#78645,#78646,#78647)) ;
#28556=EDGE_LOOP('',(#78648,#78649,#78650,#78651)) ;
#28557=EDGE_LOOP('',(#78652,#78653,#78654,#78655)) ;
#28558=EDGE_LOOP('',(#78656,#78657,#78658,#78659)) ;
#28559=EDGE_LOOP('',(#78660,#78661,#78662,#78663)) ;
#28560=EDGE_LOOP('',(#78664,#78665,#78666,#78667)) ;
#28561=EDGE_LOOP('',(#78668,#78669,#78670)) ;
#28562=EDGE_LOOP('',(#78671,#78672,#78673,#78674)) ;
#28563=EDGE_LOOP('',(#78675,#78676,#78677,#78678)) ;
#28564=EDGE_LOOP('',(#78679,#78680,#78681,#78682)) ;
#28565=EDGE_LOOP('',(#78683,#78684,#78685)) ;
#28566=EDGE_LOOP('',(#78686,#78687,#78688,#78689)) ;
#28567=EDGE_LOOP('',(#78690,#78691,#78692)) ;
#28568=EDGE_LOOP('',(#78693,#78694,#78695,#78696)) ;
#28569=EDGE_LOOP('',(#78697,#78698,#78699)) ;
#28570=EDGE_LOOP('',(#78700,#78701,#78702,#78703)) ;
#28571=EDGE_LOOP('',(#78704,#78705,#78706,#78707)) ;
#28572=EDGE_LOOP('',(#78708,#78709,#78710,#78711)) ;
#28573=EDGE_LOOP('',(#78712,#78713,#78714,#78715)) ;
#28574=EDGE_LOOP('',(#78716,#78717,#78718)) ;
#28575=EDGE_LOOP('',(#78719,#78720,#78721,#78722)) ;
#28576=EDGE_LOOP('',(#78723,#78724,#78725,#78726)) ;
#28577=EDGE_LOOP('',(#78727,#78728,#78729,#78730)) ;
#28578=EDGE_LOOP('',(#78731,#78732,#78733,#78734)) ;
#28579=EDGE_LOOP('',(#78735,#78736,#78737)) ;
#28580=EDGE_LOOP('',(#78738,#78739,#78740)) ;
#28581=EDGE_LOOP('',(#78741,#78742,#78743,#78744)) ;
#28582=EDGE_LOOP('',(#78745,#78746,#78747)) ;
#28583=EDGE_LOOP('',(#78748,#78749,#78750,#78751)) ;
#28584=EDGE_LOOP('',(#78752,#78753,#78754)) ;
#28585=EDGE_LOOP('',(#78755,#78756,#78757,#78758)) ;
#28586=EDGE_LOOP('',(#78759,#78760,#78761)) ;
#28587=EDGE_LOOP('',(#78762,#78763,#78764,#78765)) ;
#28588=EDGE_LOOP('',(#78766,#78767,#78768)) ;
#28589=EDGE_LOOP('',(#78769,#78770,#78771,#78772)) ;
#28590=EDGE_LOOP('',(#78773,#78774,#78775)) ;
#28591=EDGE_LOOP('',(#78776,#78777,#78778,#78779)) ;
#28592=EDGE_LOOP('',(#78780,#78781,#78782)) ;
#28593=EDGE_LOOP('',(#78783,#78784,#78785,#78786)) ;
#28594=EDGE_LOOP('',(#78787,#78788,#78789)) ;
#28595=EDGE_LOOP('',(#78790,#78791,#78792,#78793)) ;
#28596=EDGE_LOOP('',(#78794,#78795,#78796)) ;
#28597=EDGE_LOOP('',(#78797,#78798,#78799)) ;
#28598=EDGE_LOOP('',(#78800,#78801,#78802,#78803)) ;
#28599=EDGE_LOOP('',(#78804,#78805,#78806,#78807)) ;
#28600=EDGE_LOOP('',(#78808,#78809,#78810)) ;
#28601=EDGE_LOOP('',(#78811,#78812,#78813,#78814)) ;
#28602=EDGE_LOOP('',(#78815,#78816,#78817,#78818)) ;
#28603=EDGE_LOOP('',(#78819,#78820,#78821,#78822)) ;
#28604=EDGE_LOOP('',(#78823,#78824,#78825)) ;
#28605=EDGE_LOOP('',(#78826,#78827,#78828)) ;
#28606=EDGE_LOOP('',(#78829,#78830,#78831,#78832)) ;
#28607=EDGE_LOOP('',(#78833,#78834,#78835,#78836)) ;
#28608=EDGE_LOOP('',(#78837,#78838,#78839,#78840)) ;
#28609=EDGE_LOOP('',(#78841,#78842,#78843,#78844)) ;
#28610=EDGE_LOOP('',(#78845,#78846,#78847)) ;
#28611=EDGE_LOOP('',(#78848,#78849,#78850,#78851)) ;
#28612=EDGE_LOOP('',(#78852,#78853,#78854,#78855)) ;
#28613=EDGE_LOOP('',(#78856,#78857,#78858,#78859)) ;
#28614=EDGE_LOOP('',(#78860,#78861,#78862,#78863)) ;
#28615=EDGE_LOOP('',(#78864,#78865,#78866)) ;
#28616=EDGE_LOOP('',(#78867,#78868,#78869,#78870)) ;
#28617=EDGE_LOOP('',(#78871,#78872,#78873,#78874)) ;
#28618=EDGE_LOOP('',(#78875,#78876,#78877,#78878)) ;
#28619=EDGE_LOOP('',(#78879,#78880,#78881)) ;
#28620=EDGE_LOOP('',(#78882,#78883,#78884,#78885)) ;
#28621=EDGE_LOOP('',(#78886,#78887,#78888)) ;
#28622=EDGE_LOOP('',(#78889,#78890,#78891,#78892,#78893)) ;
#28623=EDGE_LOOP('',(#78894,#78895,#78896,#78897)) ;
#28624=EDGE_LOOP('',(#78898,#78899,#78900,#78901,#78902)) ;
#28625=EDGE_LOOP('',(#78903,#78904,#78905,#78906)) ;
#32295=CIRCLE('',#98153,0.0999999999999998) ;
#32296=CIRCLE('',#98154,0.0999999999999998) ;
#32297=CIRCLE('',#98156,0.1645125) ;
#32298=CIRCLE('',#98157,0.1) ;
#32299=CIRCLE('',#98158,0.0645124999999998) ;
#32300=CIRCLE('',#98159,0.1) ;
#32301=CIRCLE('',#98161,0.1645125) ;
#32302=CIRCLE('',#98162,0.0999999999999999) ;
#32303=CIRCLE('',#98163,0.0645125000000003) ;
#32304=CIRCLE('',#98164,0.1) ;
#32305=CIRCLE('',#98166,2.35) ;
#32306=CIRCLE('',#98167,2.25) ;
#32307=CIRCLE('',#98169,0.1645125) ;
#32308=CIRCLE('',#98170,0.1) ;
#32309=CIRCLE('',#98171,0.0645125000000003) ;
#32310=CIRCLE('',#98172,0.1) ;
#32311=CIRCLE('',#98174,2.35) ;
#32312=CIRCLE('',#98175,2.25) ;
#32313=CIRCLE('',#98177,0.1645125) ;
#32314=CIRCLE('',#98178,0.1) ;
#32315=CIRCLE('',#98179,0.0645125000000003) ;
#32316=CIRCLE('',#98180,0.1) ;
#32317=CIRCLE('',#98182,2.35) ;
#32318=CIRCLE('',#98183,2.25) ;
#32319=CIRCLE('',#98185,0.1645125) ;
#32320=CIRCLE('',#98186,0.1) ;
#32321=CIRCLE('',#98187,0.0645125000000003) ;
#32322=CIRCLE('',#98188,0.1) ;
#32323=CIRCLE('',#98190,2.35) ;
#32324=CIRCLE('',#98191,2.25) ;
#32325=CIRCLE('',#98193,0.1645125) ;
#32326=CIRCLE('',#98194,0.0999999999999993) ;
#32327=CIRCLE('',#98195,0.0645125000000003) ;
#32328=CIRCLE('',#98196,0.0999999999999993) ;
#32329=CIRCLE('',#98198,2.35) ;
#32330=CIRCLE('',#98199,2.25) ;
#32331=CIRCLE('',#98201,0.1645125) ;
#32332=CIRCLE('',#98202,0.0999999999999993) ;
#32333=CIRCLE('',#98203,0.0645125000000003) ;
#32334=CIRCLE('',#98204,0.0999999999999993) ;
#32335=CIRCLE('',#98206,2.35) ;
#32336=CIRCLE('',#98207,2.25) ;
#32337=CIRCLE('',#98209,0.1645125) ;
#32338=CIRCLE('',#98210,0.0999999999999993) ;
#32339=CIRCLE('',#98211,0.0645125000000003) ;
#32340=CIRCLE('',#98212,0.0999999999999993) ;
#32341=CIRCLE('',#98214,2.35) ;
#32342=CIRCLE('',#98215,2.25) ;
#32343=CIRCLE('',#98217,0.1645125) ;
#32344=CIRCLE('',#98218,0.0999999999999993) ;
#32345=CIRCLE('',#98219,0.0645125000000003) ;
#32346=CIRCLE('',#98220,0.0999999999999993) ;
#32347=CIRCLE('',#98222,2.35) ;
#32348=CIRCLE('',#98223,2.25) ;
#32349=CIRCLE('',#98225,0.164512500000005) ;
#32350=CIRCLE('',#98226,0.0999999999999999) ;
#32351=CIRCLE('',#98227,0.0645125000000055) ;
#32352=CIRCLE('',#98228,0.100000000000001) ;
#32353=CIRCLE('',#98230,2.35) ;
#32354=CIRCLE('',#98231,2.25) ;
#32355=CIRCLE('',#98233,0.164512500000006) ;
#32356=CIRCLE('',#98234,0.0999999999999992) ;
#32357=CIRCLE('',#98235,0.0645125000000061) ;
#32358=CIRCLE('',#98236,0.100000000000003) ;
#32359=CIRCLE('',#98238,2.35) ;
#32360=CIRCLE('',#98239,2.25) ;
#32361=CIRCLE('',#98241,0.0645124999999989) ;
#32362=CIRCLE('',#98243,0.0645124999999989) ;
#32363=CIRCLE('',#98245,0.0645124999999989) ;
#32364=CIRCLE('',#98247,0.0645124999999989) ;
#32365=CIRCLE('',#98249,0.0645125000000003) ;
#32366=CIRCLE('',#98251,0.0645125000000003) ;
#32367=CIRCLE('',#98253,0.0645124999999998) ;
#32368=CIRCLE('',#98255,0.970710678118651) ;
#32369=CIRCLE('',#98256,0.1) ;
#32370=CIRCLE('',#98257,1.) ;
#32371=CIRCLE('',#98259,1.5) ;
#32372=CIRCLE('',#98260,0.1) ;
#32373=CIRCLE('',#98261,1.6) ;
#32374=CIRCLE('',#98263,1.) ;
#32375=CIRCLE('',#98264,0.1) ;
#32376=CIRCLE('',#98265,1.1) ;
#32377=CIRCLE('',#98267,0.970710678118658) ;
#32378=CIRCLE('',#98268,0.1) ;
#32379=CIRCLE('',#98269,1.) ;
#32380=CIRCLE('',#98271,1.5) ;
#32381=CIRCLE('',#98272,0.1) ;
#32382=CIRCLE('',#98273,1.6) ;
#32383=CIRCLE('',#98275,1.) ;
#32384=CIRCLE('',#98276,0.1) ;
#32385=CIRCLE('',#98277,1.1) ;
#32386=CIRCLE('',#98279,0.970710678118658) ;
#32387=CIRCLE('',#98280,0.1) ;
#32388=CIRCLE('',#98281,1.) ;
#32389=CIRCLE('',#98283,1.5) ;
#32390=CIRCLE('',#98284,0.1) ;
#32391=CIRCLE('',#98285,1.6) ;
#32392=CIRCLE('',#98287,1.) ;
#32393=CIRCLE('',#98288,0.1) ;
#32394=CIRCLE('',#98289,1.1) ;
#32395=CIRCLE('',#98291,0.970710678118658) ;
#32396=CIRCLE('',#98292,0.1) ;
#32397=CIRCLE('',#98293,1.) ;
#32398=CIRCLE('',#98295,1.5) ;
#32399=CIRCLE('',#98296,0.1) ;
#32400=CIRCLE('',#98297,1.6) ;
#32401=CIRCLE('',#98299,1.) ;
#32402=CIRCLE('',#98300,0.1) ;
#32403=CIRCLE('',#98301,1.1) ;
#32404=CIRCLE('',#98303,0.970710678118658) ;
#32405=CIRCLE('',#98304,0.1) ;
#32406=CIRCLE('',#98305,1.) ;
#32407=CIRCLE('',#98307,1.5) ;
#32408=CIRCLE('',#98308,0.1) ;
#32409=CIRCLE('',#98309,1.6) ;
#32410=CIRCLE('',#98311,1.) ;
#32411=CIRCLE('',#98312,0.1) ;
#32412=CIRCLE('',#98313,1.1) ;
#32413=CIRCLE('',#98315,0.970710678118658) ;
#32414=CIRCLE('',#98316,0.1) ;
#32415=CIRCLE('',#98317,1.) ;
#32416=CIRCLE('',#98319,1.5) ;
#32417=CIRCLE('',#98320,0.1) ;
#32418=CIRCLE('',#98321,1.6) ;
#32419=CIRCLE('',#98323,1.) ;
#32420=CIRCLE('',#98324,0.1) ;
#32421=CIRCLE('',#98325,1.1) ;
#32422=CIRCLE('',#98327,0.970710678118658) ;
#32423=CIRCLE('',#98328,0.1) ;
#32424=CIRCLE('',#98329,1.) ;
#32425=CIRCLE('',#98331,1.5) ;
#32426=CIRCLE('',#98332,0.1) ;
#32427=CIRCLE('',#98333,1.6) ;
#32428=CIRCLE('',#98335,1.) ;
#32429=CIRCLE('',#98336,0.1) ;
#32430=CIRCLE('',#98337,1.1) ;
#32431=CIRCLE('',#98339,0.970710678118656) ;
#32432=CIRCLE('',#98340,0.1) ;
#32433=CIRCLE('',#98341,0.999999999999999) ;
#32434=CIRCLE('',#98343,1.5) ;
#32435=CIRCLE('',#98344,0.1) ;
#32436=CIRCLE('',#98345,1.6) ;
#32437=CIRCLE('',#98347,0.999999999999999) ;
#32438=CIRCLE('',#98348,0.1) ;
#32439=CIRCLE('',#98349,1.1) ;
#32440=CIRCLE('',#98351,0.970710678118656) ;
#32441=CIRCLE('',#98352,0.1) ;
#32442=CIRCLE('',#98353,1.) ;
#32443=CIRCLE('',#98355,1.5) ;
#32444=CIRCLE('',#98356,0.1) ;
#32445=CIRCLE('',#98357,1.6) ;
#32446=CIRCLE('',#98359,1.) ;
#32447=CIRCLE('',#98360,0.1) ;
#32448=CIRCLE('',#98361,1.1) ;
#32449=CIRCLE('',#98363,1.5) ;
#32450=CIRCLE('',#98364,1.5) ;
#32451=CIRCLE('',#98365,1.5) ;
#32452=CIRCLE('',#98366,1.5) ;
#32453=CIRCLE('',#98367,1.5) ;
#32454=CIRCLE('',#98369,1.5) ;
#32455=CIRCLE('',#98370,1.5) ;
#32456=CIRCLE('',#98371,1.5) ;
#32457=CIRCLE('',#98372,1.5) ;
#32458=CIRCLE('',#98373,1.5) ;
#32459=CIRCLE('',#98375,1.5) ;
#32460=CIRCLE('',#98376,1.5) ;
#32461=CIRCLE('',#98377,1.5) ;
#32462=CIRCLE('',#98378,1.5) ;
#32463=CIRCLE('',#98379,1.5) ;
#32464=CIRCLE('',#98381,1.5) ;
#32465=CIRCLE('',#98382,1.5) ;
#32466=CIRCLE('',#98383,1.5) ;
#32467=CIRCLE('',#98384,1.5) ;
#32468=CIRCLE('',#98385,1.5) ;
#32469=CIRCLE('',#98387,1.5) ;
#32470=CIRCLE('',#98388,1.5) ;
#32471=CIRCLE('',#98389,1.5) ;
#32472=CIRCLE('',#98390,1.5) ;
#32473=CIRCLE('',#98391,1.5) ;
#32474=CIRCLE('',#98393,1.5) ;
#32475=CIRCLE('',#98394,1.5) ;
#32476=CIRCLE('',#98395,1.5) ;
#32477=CIRCLE('',#98396,1.5) ;
#32478=CIRCLE('',#98397,1.5) ;
#32479=CIRCLE('',#98399,1.5) ;
#32480=CIRCLE('',#98400,1.5) ;
#32481=CIRCLE('',#98401,1.5) ;
#32482=CIRCLE('',#98402,1.5) ;
#32483=CIRCLE('',#98403,1.5) ;
#32484=CIRCLE('',#98405,1.5) ;
#32485=CIRCLE('',#98406,1.5) ;
#32486=CIRCLE('',#98407,1.5) ;
#32487=CIRCLE('',#98408,1.5) ;
#32488=CIRCLE('',#98409,1.5) ;
#32489=CIRCLE('',#98411,1.5) ;
#32490=CIRCLE('',#98412,1.5) ;
#32491=CIRCLE('',#98413,1.5) ;
#32492=CIRCLE('',#98414,1.5) ;
#32493=CIRCLE('',#98415,1.5) ;
#32494=CIRCLE('',#98417,0.5) ;
#32495=CIRCLE('',#98419,0.499999999999997) ;
#32496=CIRCLE('',#98421,0.499999999999997) ;
#32497=CIRCLE('',#98423,0.499999999999997) ;
#32498=CIRCLE('',#98425,0.499999999999997) ;
#32499=CIRCLE('',#98427,0.499999999999997) ;
#32500=CIRCLE('',#98429,0.499999999999997) ;
#32501=CIRCLE('',#98431,0.499999999999997) ;
#32502=CIRCLE('',#98433,0.499999999999998) ;
#32503=CIRCLE('',#98444,0.970710678118656) ;
#32504=CIRCLE('',#98445,0.1) ;
#32505=CIRCLE('',#98446,1.) ;
#32506=CIRCLE('',#98448,1.5) ;
#32507=CIRCLE('',#98449,0.1) ;
#32508=CIRCLE('',#98450,1.6) ;
#32509=CIRCLE('',#98452,1.) ;
#32510=CIRCLE('',#98453,0.1) ;
#32511=CIRCLE('',#98454,1.1) ;
#32512=CIRCLE('',#98456,0.0645125000000024) ;
#32513=CIRCLE('',#98458,0.0645125000000094) ;
#32514=CIRCLE('',#98460,0.0645125) ;
#32515=CIRCLE('',#98462,0.0645125) ;
#32516=CIRCLE('',#98464,1.5) ;
#32517=CIRCLE('',#98465,1.5) ;
#32518=CIRCLE('',#98466,1.5) ;
#32519=CIRCLE('',#98467,1.5) ;
#32520=CIRCLE('',#98468,1.5) ;
#32521=CIRCLE('',#98470,0.499999999999998) ;
#32522=CIRCLE('',#98473,2.15) ;
#32523=CIRCLE('',#98474,2.15) ;
#32524=CIRCLE('',#98475,2.15) ;
#32525=CIRCLE('',#98476,2.15) ;
#32526=CIRCLE('',#98477,2.15) ;
#32527=CIRCLE('',#98478,2.15) ;
#32528=CIRCLE('',#98479,2.15) ;
#32529=CIRCLE('',#98480,2.15) ;
#32530=CIRCLE('',#98481,2.15) ;
#32531=CIRCLE('',#98482,2.15) ;
#32532=CIRCLE('',#98483,0.2) ;
#32533=CIRCLE('',#98484,0.2) ;
#32534=CIRCLE('',#98485,0.2) ;
#32535=CIRCLE('',#98486,0.2) ;
#32536=CIRCLE('',#98487,0.2) ;
#32537=CIRCLE('',#98488,0.2) ;
#32538=CIRCLE('',#98489,0.2) ;
#32539=CIRCLE('',#98490,0.2) ;
#32540=CIRCLE('',#98491,0.2) ;
#32541=CIRCLE('',#98492,0.2) ;
#32542=CIRCLE('',#98493,0.2) ;
#32543=CIRCLE('',#98494,0.2) ;
#32544=CIRCLE('',#98495,0.2) ;
#32545=CIRCLE('',#98496,0.2) ;
#32546=CIRCLE('',#98497,0.2) ;
#32547=CIRCLE('',#98498,0.2) ;
#32548=CIRCLE('',#98499,0.2) ;
#32549=CIRCLE('',#98500,0.2) ;
#32550=CIRCLE('',#98501,0.2) ;
#32551=CIRCLE('',#98502,0.2) ;
#32552=CIRCLE('',#98503,0.2) ;
#32553=CIRCLE('',#98504,0.2) ;
#32554=CIRCLE('',#98505,0.2) ;
#32555=CIRCLE('',#98506,0.2) ;
#32556=CIRCLE('',#98507,0.2) ;
#32557=CIRCLE('',#98508,0.2) ;
#32558=CIRCLE('',#98509,0.2) ;
#32559=CIRCLE('',#98510,0.2) ;
#32560=CIRCLE('',#98511,0.2) ;
#32561=CIRCLE('',#98512,0.2) ;
#32562=CIRCLE('',#98513,0.2) ;
#32563=CIRCLE('',#98514,0.2) ;
#32564=CIRCLE('',#98515,0.2) ;
#32565=CIRCLE('',#98516,0.2) ;
#32566=CIRCLE('',#98517,0.2) ;
#32567=CIRCLE('',#98518,0.2) ;
#32568=CIRCLE('',#98519,0.2) ;
#32569=CIRCLE('',#98520,0.2) ;
#32570=CIRCLE('',#98521,0.2) ;
#32571=CIRCLE('',#98522,0.2) ;
#32572=CIRCLE('',#98524,0.199999999999999) ;
#32573=CIRCLE('',#98525,0.199999999999999) ;
#32574=CIRCLE('',#98526,0.199999999999999) ;
#32575=CIRCLE('',#98527,0.199999999999999) ;
#32576=CIRCLE('',#98529,0.199999999999999) ;
#32577=CIRCLE('',#98530,0.199999999999999) ;
#32578=CIRCLE('',#98531,0.199999999999999) ;
#32579=CIRCLE('',#98532,0.199999999999999) ;
#32580=CIRCLE('',#98534,0.199999999999999) ;
#32581=CIRCLE('',#98535,0.199999999999999) ;
#32582=CIRCLE('',#98536,0.199999999999999) ;
#32583=CIRCLE('',#98537,0.199999999999999) ;
#32584=CIRCLE('',#98539,0.199999999999999) ;
#32585=CIRCLE('',#98540,0.199999999999999) ;
#32586=CIRCLE('',#98541,0.199999999999999) ;
#32587=CIRCLE('',#98542,0.199999999999999) ;
#32588=CIRCLE('',#98544,0.199999999999999) ;
#32589=CIRCLE('',#98545,0.199999999999999) ;
#32590=CIRCLE('',#98546,0.199999999999999) ;
#32591=CIRCLE('',#98547,0.199999999999999) ;
#32592=CIRCLE('',#98549,0.200000000000001) ;
#32593=CIRCLE('',#98550,0.200000000000001) ;
#32594=CIRCLE('',#98551,0.199999999999999) ;
#32595=CIRCLE('',#98552,0.199999999999999) ;
#32596=CIRCLE('',#98554,0.200000000000001) ;
#32597=CIRCLE('',#98555,0.200000000000001) ;
#32598=CIRCLE('',#98556,0.200000000000001) ;
#32599=CIRCLE('',#98557,0.200000000000001) ;
#32600=CIRCLE('',#98559,0.2) ;
#32601=CIRCLE('',#98560,0.200000000000001) ;
#32602=CIRCLE('',#98561,0.200000000000001) ;
#32603=CIRCLE('',#98562,0.200000000000001) ;
#32604=CIRCLE('',#98564,0.2) ;
#32605=CIRCLE('',#98565,0.2) ;
#32606=CIRCLE('',#98566,0.200000000000001) ;
#32607=CIRCLE('',#98567,0.2) ;
#32608=CIRCLE('',#98578,0.2) ;
#32609=CIRCLE('',#98579,0.2) ;
#32610=CIRCLE('',#98580,0.2) ;
#32611=CIRCLE('',#98581,0.2) ;
#32612=CIRCLE('',#98582,0.2) ;
#32613=CIRCLE('',#98583,0.2) ;
#32614=CIRCLE('',#98584,0.2) ;
#32615=CIRCLE('',#98585,0.2) ;
#32616=CIRCLE('',#98586,0.2) ;
#32617=CIRCLE('',#98587,0.2) ;
#32618=CIRCLE('',#98588,0.200000000000001) ;
#32619=CIRCLE('',#98589,0.200000000000001) ;
#32620=CIRCLE('',#98590,0.200000000000001) ;
#32621=CIRCLE('',#98591,0.200000000000001) ;
#32622=CIRCLE('',#98592,0.200000000000001) ;
#32623=CIRCLE('',#98593,0.200000000000001) ;
#32624=CIRCLE('',#98594,0.200000000000001) ;
#32625=CIRCLE('',#98595,0.200000000000001) ;
#32626=CIRCLE('',#98596,0.199999999999999) ;
#32627=CIRCLE('',#98597,0.199999999999999) ;
#32628=CIRCLE('',#98598,0.199999999999999) ;
#32629=CIRCLE('',#98599,0.199999999999999) ;
#32630=CIRCLE('',#98600,0.199999999999999) ;
#32631=CIRCLE('',#98601,0.199999999999999) ;
#32632=CIRCLE('',#98602,0.199999999999999) ;
#32633=CIRCLE('',#98603,0.199999999999999) ;
#32634=CIRCLE('',#98604,0.199999999999999) ;
#32635=CIRCLE('',#98605,0.199999999999999) ;
#32636=CIRCLE('',#98606,0.199999999999999) ;
#32637=CIRCLE('',#98607,0.199999999999999) ;
#32638=CIRCLE('',#98608,0.199999999999999) ;
#32639=CIRCLE('',#98609,0.199999999999999) ;
#32640=CIRCLE('',#98610,0.199999999999999) ;
#32641=CIRCLE('',#98611,0.199999999999999) ;
#32642=CIRCLE('',#98612,0.199999999999999) ;
#32643=CIRCLE('',#98613,0.199999999999999) ;
#32644=CIRCLE('',#98614,0.199999999999999) ;
#32645=CIRCLE('',#98615,0.199999999999999) ;
#32646=CIRCLE('',#98616,0.199999999999999) ;
#32647=CIRCLE('',#98617,0.199999999999999) ;
#32648=CIRCLE('',#98619,0.199999999999999) ;
#32649=CIRCLE('',#98620,0.199999999999999) ;
#32650=CIRCLE('',#98621,1.55625) ;
#32651=CIRCLE('',#98623,0.199999999999999) ;
#32652=CIRCLE('',#98624,0.199999999999999) ;
#32653=CIRCLE('',#98625,1.55625) ;
#32654=CIRCLE('',#98627,0.199999999999999) ;
#32655=CIRCLE('',#98628,0.199999999999999) ;
#32656=CIRCLE('',#98629,1.55625) ;
#32657=CIRCLE('',#98631,0.199999999999999) ;
#32658=CIRCLE('',#98632,0.199999999999999) ;
#32659=CIRCLE('',#98633,1.55625) ;
#32660=CIRCLE('',#98635,0.199999999999999) ;
#32661=CIRCLE('',#98636,0.199999999999999) ;
#32662=CIRCLE('',#98637,1.55625) ;
#32663=CIRCLE('',#98639,0.200000000000001) ;
#32664=CIRCLE('',#98640,0.199999999999999) ;
#32665=CIRCLE('',#98641,1.55625) ;
#32666=CIRCLE('',#98643,0.200000000000001) ;
#32667=CIRCLE('',#98644,0.200000000000001) ;
#32668=CIRCLE('',#98645,1.55625) ;
#32669=CIRCLE('',#98647,0.2) ;
#32670=CIRCLE('',#98648,0.200000000000001) ;
#32671=CIRCLE('',#98649,1.55625) ;
#32672=CIRCLE('',#98651,0.2) ;
#32673=CIRCLE('',#98652,0.2) ;
#32674=CIRCLE('',#98653,1.55625) ;
#32675=CIRCLE('',#98656,0.2) ;
#32676=CIRCLE('',#98657,0.2) ;
#32677=CIRCLE('',#98658,0.2) ;
#32678=CIRCLE('',#98659,0.2) ;
#32679=CIRCLE('',#98660,0.2) ;
#32680=CIRCLE('',#98661,0.2) ;
#32681=CIRCLE('',#98662,0.2) ;
#32682=CIRCLE('',#98663,0.2) ;
#32683=CIRCLE('',#98664,0.2) ;
#32684=CIRCLE('',#98665,0.2) ;
#32685=CIRCLE('',#98666,0.2) ;
#32686=CIRCLE('',#98667,0.2) ;
#32687=CIRCLE('',#98668,0.2) ;
#32688=CIRCLE('',#98669,0.2) ;
#32689=CIRCLE('',#98670,0.2) ;
#32690=CIRCLE('',#98671,0.2) ;
#32691=CIRCLE('',#98672,0.2) ;
#32692=CIRCLE('',#98673,0.2) ;
#32693=CIRCLE('',#98674,0.2) ;
#32694=CIRCLE('',#98675,0.2) ;
#32695=CIRCLE('',#98677,0.0999999999999998) ;
#32696=CIRCLE('',#98678,0.0999999999999998) ;
#32697=CIRCLE('',#98680,0.0999999999999998) ;
#32698=CIRCLE('',#98681,0.0999999999999998) ;
#32699=CIRCLE('',#98682,0.0999999999999998) ;
#32700=CIRCLE('',#98683,0.0999999999999998) ;
#32701=CIRCLE('',#98686,0.2) ;
#32702=CIRCLE('',#98687,0.2) ;
#32703=CIRCLE('',#98688,0.2) ;
#32704=CIRCLE('',#98689,0.2) ;
#32705=CIRCLE('',#98693,0.2) ;
#32706=CIRCLE('',#98694,1.55625) ;
#32707=CIRCLE('',#98695,0.2) ;
#32708=CIRCLE('',#98700,0.2) ;
#32709=CIRCLE('',#98701,0.2) ;
#32710=CIRCLE('',#98702,0.2) ;
#32711=CIRCLE('',#98703,0.2) ;
#32712=CIRCLE('',#98704,0.2) ;
#32713=CIRCLE('',#98705,0.2) ;
#32714=CIRCLE('',#98706,0.2) ;
#32715=CIRCLE('',#98707,0.2) ;
#32716=CIRCLE('',#98709,0.2) ;
#32717=CIRCLE('',#98710,0.2) ;
#32718=CIRCLE('',#98711,0.2) ;
#32719=CIRCLE('',#98713,0.2) ;
#32720=CIRCLE('',#98714,0.2) ;
#32721=CIRCLE('',#98715,0.2) ;
#32722=CIRCLE('',#98732,0.1) ;
#32723=CIRCLE('',#98733,0.1) ;
#32724=CIRCLE('',#98734,0.1) ;
#32725=CIRCLE('',#98735,0.1) ;
#32726=CIRCLE('',#98742,0.2) ;
#32727=CIRCLE('',#98743,0.2) ;
#32728=CIRCLE('',#98746,0.2) ;
#32729=CIRCLE('',#98747,0.2) ;
#32730=CIRCLE('',#98748,0.2) ;
#32731=CIRCLE('',#98751,0.2) ;
#32732=CIRCLE('',#98752,0.2) ;
#32733=CIRCLE('',#98753,0.2) ;
#32734=CIRCLE('',#98758,1.65625) ;
#32735=CIRCLE('',#98759,1.65625) ;
#32736=CIRCLE('',#98761,1.75625) ;
#32737=CIRCLE('',#98768,0.1) ;
#32738=CIRCLE('',#98769,0.1) ;
#32739=CIRCLE('',#98770,0.1) ;
#32740=CIRCLE('',#98771,0.1) ;
#32741=CIRCLE('',#98782,2.25) ;
#32742=CIRCLE('',#98784,2.25) ;
#32743=CIRCLE('',#98788,2.25) ;
#32744=CIRCLE('',#98790,2.25) ;
#32745=CIRCLE('',#98792,0.0999999999999997) ;
#32746=CIRCLE('',#98793,0.0999999999999997) ;
#32747=CIRCLE('',#98796,0.1) ;
#32748=CIRCLE('',#98797,0.1) ;
#32749=CIRCLE('',#98800,0.1) ;
#32750=CIRCLE('',#98801,0.1) ;
#32751=CIRCLE('',#98804,0.0999999999999997) ;
#32752=CIRCLE('',#98805,0.0999999999999997) ;
#32753=CIRCLE('',#98809,0.0999999999999998) ;
#32754=CIRCLE('',#98810,0.0999999999999998) ;
#32755=CIRCLE('',#98812,0.1) ;
#32756=CIRCLE('',#98813,0.0999999999999998) ;
#32757=CIRCLE('',#98815,0.0999999999999998) ;
#32758=CIRCLE('',#98816,0.0999999999999998) ;
#32759=CIRCLE('',#98818,0.0999999999999998) ;
#32760=CIRCLE('',#98820,0.1) ;
#32761=CIRCLE('',#98822,0.100000000000003) ;
#32762=CIRCLE('',#98823,0.100000000000003) ;
#32763=CIRCLE('',#98825,0.0999999999999998) ;
#32764=CIRCLE('',#98826,0.0999999999999998) ;
#32765=CIRCLE('',#98828,0.0999999999999998) ;
#32766=CIRCLE('',#98832,0.1) ;
#32767=CIRCLE('',#98833,0.0999999999999998) ;
#32768=CIRCLE('',#98835,0.100000000000003) ;
#32769=CIRCLE('',#98837,0.0999999999999998) ;
#32770=CIRCLE('',#98838,0.0999999999999998) ;
#32771=CIRCLE('',#98840,0.0999999999999998) ;
#32772=CIRCLE('',#98846,0.1) ;
#32773=CIRCLE('',#98848,0.0999999999999998) ;
#32774=CIRCLE('',#98850,0.1) ;
#32775=CIRCLE('',#98852,0.100000000000003) ;
#32776=CIRCLE('',#98854,0.100000000000003) ;
#32777=CIRCLE('',#98855,0.100000000000003) ;
#32778=CIRCLE('',#98857,0.0999999999999998) ;
#32779=CIRCLE('',#98859,0.1) ;
#32780=CIRCLE('',#98861,0.100000000000003) ;
#32781=CIRCLE('',#98863,0.100000000000003) ;
#32782=CIRCLE('',#98866,0.1) ;
#32783=CIRCLE('',#98868,0.100000000000003) ;
#32784=CIRCLE('',#98873,0.1) ;
#32785=CIRCLE('',#98879,0.0999999999999994) ;
#32786=CIRCLE('',#98880,0.1) ;
#32787=CIRCLE('',#98881,0.1) ;
#32788=CIRCLE('',#98883,0.1) ;
#32789=CIRCLE('',#98885,0.1) ;
#32790=CIRCLE('',#98887,0.0999999999999994) ;
#32791=CIRCLE('',#98889,0.1) ;
#32792=CIRCLE('',#98890,0.1) ;
#32793=CIRCLE('',#98892,0.0999999999999994) ;
#32794=CIRCLE('',#98893,0.0999999999999994) ;
#32795=CIRCLE('',#98895,0.1) ;
#32796=CIRCLE('',#98896,0.0999999999999998) ;
#32797=CIRCLE('',#98898,0.0999999999999998) ;
#32798=CIRCLE('',#98899,0.1) ;
#32799=CIRCLE('',#98901,0.1) ;
#32800=CIRCLE('',#98903,0.1) ;
#32801=CIRCLE('',#98904,0.1) ;
#32802=CIRCLE('',#98906,0.0999999999999994) ;
#32803=CIRCLE('',#98908,0.1) ;
#32804=CIRCLE('',#98910,0.1) ;
#32805=CIRCLE('',#98912,0.0999999999999998) ;
#32806=CIRCLE('',#98914,0.1) ;
#32807=CIRCLE('',#98916,0.1) ;
#32808=CIRCLE('',#98918,0.0999999999999998) ;
#32809=CIRCLE('',#98920,0.1) ;
#32810=CIRCLE('',#98922,0.1) ;
#32811=CIRCLE('',#98924,0.0999999999999998) ;
#32812=CIRCLE('',#98926,0.1) ;
#32813=CIRCLE('',#98928,0.1) ;
#32814=CIRCLE('',#98929,0.1) ;
#32815=CIRCLE('',#98931,0.0999999999999998) ;
#32816=CIRCLE('',#98932,0.0999999999999998) ;
#32817=CIRCLE('',#98934,0.1) ;
#32818=CIRCLE('',#98936,0.1) ;
#32819=CIRCLE('',#98937,0.0999999999999998) ;
#32820=CIRCLE('',#98939,0.1) ;
#32821=CIRCLE('',#98941,0.1) ;
#32822=CIRCLE('',#98943,0.0999999999999998) ;
#32823=CIRCLE('',#98945,0.1) ;
#32824=CIRCLE('',#98947,0.1) ;
#32825=CIRCLE('',#98949,0.1) ;
#32826=CIRCLE('',#98951,0.0999999999999998) ;
#32827=CIRCLE('',#98953,0.0999999999999998) ;
#32828=CIRCLE('',#98954,0.0999999999999998) ;
#32829=CIRCLE('',#98956,0.1) ;
#32830=CIRCLE('',#98957,0.1) ;
#32831=CIRCLE('',#98959,0.1) ;
#32832=CIRCLE('',#98961,0.0999999999999998) ;
#32833=CIRCLE('',#98963,0.1) ;
#32834=CIRCLE('',#98965,0.1) ;
#32835=CIRCLE('',#98968,0.1) ;
#32836=CIRCLE('',#98969,0.0999999999999998) ;
#32837=CIRCLE('',#98971,0.0999999999999998) ;
#32838=CIRCLE('',#98973,0.1) ;
#32839=CIRCLE('',#98975,0.1) ;
#32840=CIRCLE('',#98977,0.0999999999999994) ;
#32841=CIRCLE('',#98979,0.0999999999999998) ;
#32842=CIRCLE('',#98981,0.0999999999999994) ;
#32843=CIRCLE('',#98984,0.1) ;
#32844=CIRCLE('',#98985,0.1) ;
#32845=CIRCLE('',#98987,0.1) ;
#32846=CIRCLE('',#98988,0.1) ;
#32847=CIRCLE('',#98990,0.1) ;
#32848=CIRCLE('',#98991,0.0999999999999998) ;
#32849=CIRCLE('',#98993,0.1) ;
#32850=CIRCLE('',#98995,0.1) ;
#32851=CIRCLE('',#98997,0.1) ;
#32852=CIRCLE('',#98998,0.1) ;
#32853=CIRCLE('',#99000,0.1) ;
#32854=CIRCLE('',#99002,0.0999999999999998) ;
#32855=CIRCLE('',#99004,0.1) ;
#32856=CIRCLE('',#99005,0.1) ;
#32857=CIRCLE('',#99007,0.1) ;
#32858=CIRCLE('',#99009,0.1) ;
#32859=CIRCLE('',#99011,0.1) ;
#32860=CIRCLE('',#99013,0.1) ;
#32861=CIRCLE('',#99015,0.1) ;
#32862=CIRCLE('',#99017,0.1) ;
#32863=CIRCLE('',#99019,0.0999999999999998) ;
#32864=CIRCLE('',#99021,0.1) ;
#32865=CIRCLE('',#99023,0.1) ;
#32866=CIRCLE('',#99025,0.1) ;
#32867=CIRCLE('',#99028,0.1) ;
#32868=CIRCLE('',#99030,0.1) ;
#32869=CIRCLE('',#99031,0.1) ;
#32870=CIRCLE('',#99033,0.1) ;
#32871=CIRCLE('',#99035,0.1) ;
#32872=CIRCLE('',#99037,0.1) ;
#32873=CIRCLE('',#99039,0.1) ;
#32874=CIRCLE('',#99041,0.1) ;
#32875=CIRCLE('',#99043,0.1) ;
#32876=CIRCLE('',#99045,0.1) ;
#32877=CIRCLE('',#99047,0.1) ;
#32878=CIRCLE('',#99049,0.1) ;
#32879=CIRCLE('',#99052,0.0999999999999999) ;
#32880=CIRCLE('',#99054,0.1) ;
#32881=CIRCLE('',#99055,0.1) ;
#32882=CIRCLE('',#99058,0.1) ;
#32883=CIRCLE('',#99060,0.1) ;
#32884=CIRCLE('',#99061,0.1) ;
#32885=CIRCLE('',#99062,0.1) ;
#32886=CIRCLE('',#99064,0.1) ;
#32887=CIRCLE('',#99066,0.1) ;
#32888=CIRCLE('',#99068,0.1) ;
#32889=CIRCLE('',#99070,0.1) ;
#32890=CIRCLE('',#99072,0.1) ;
#32891=CIRCLE('',#99076,0.1) ;
#32892=CIRCLE('',#99077,0.1) ;
#32893=CIRCLE('',#99078,0.1) ;
#32894=CIRCLE('',#99080,0.1) ;
#32895=CIRCLE('',#99082,0.1) ;
#32896=CIRCLE('',#99084,0.1) ;
#32897=CIRCLE('',#99086,0.1) ;
#32898=CIRCLE('',#99088,0.1) ;
#32899=CIRCLE('',#99092,0.1) ;
#32900=CIRCLE('',#99093,0.1) ;
#32901=CIRCLE('',#99095,0.0999999999999998) ;
#32902=CIRCLE('',#99096,0.0999999999999998) ;
#32903=CIRCLE('',#99098,0.0999999999999998) ;
#32904=CIRCLE('',#99099,0.1) ;
#32905=CIRCLE('',#99101,0.0999999999999998) ;
#32906=CIRCLE('',#99103,0.1) ;
#32907=CIRCLE('',#99105,0.1) ;
#32908=CIRCLE('',#99106,0.1) ;
#32909=CIRCLE('',#99108,0.1) ;
#32910=CIRCLE('',#99110,0.1) ;
#32911=CIRCLE('',#99112,0.1) ;
#32912=CIRCLE('',#99113,0.1) ;
#32913=CIRCLE('',#99115,0.0999999999999998) ;
#32914=CIRCLE('',#99117,0.0999999999999998) ;
#32915=CIRCLE('',#99119,0.0999999999999998) ;
#32916=CIRCLE('',#99121,0.0999999999999998) ;
#32917=CIRCLE('',#99123,0.1) ;
#32918=CIRCLE('',#99125,0.0999999999999998) ;
#32919=CIRCLE('',#99127,0.0999999999999998) ;
#32920=CIRCLE('',#99129,0.1) ;
#32921=CIRCLE('',#99131,0.1) ;
#32922=CIRCLE('',#99133,0.1) ;
#32923=CIRCLE('',#99136,0.1) ;
#32924=CIRCLE('',#99138,0.0999999999999998) ;
#32925=CIRCLE('',#99139,0.0999999999999998) ;
#32926=CIRCLE('',#99141,0.1) ;
#32927=CIRCLE('',#99143,0.1) ;
#32928=CIRCLE('',#99145,0.1) ;
#32929=CIRCLE('',#99147,0.1) ;
#32930=CIRCLE('',#99149,0.1) ;
#32931=CIRCLE('',#99151,0.1) ;
#32932=CIRCLE('',#99153,0.1) ;
#32933=CIRCLE('',#99155,0.0999999999999998) ;
#32934=CIRCLE('',#99157,0.0999999999999998) ;
#32935=CIRCLE('',#99160,0.1) ;
#32936=CIRCLE('',#99161,0.0999999999999994) ;
#32937=CIRCLE('',#99163,0.1) ;
#32938=CIRCLE('',#99165,0.1) ;
#32939=CIRCLE('',#99167,0.1) ;
#32940=CIRCLE('',#99169,0.1) ;
#32941=CIRCLE('',#99171,0.0999999999999994) ;
#32942=CIRCLE('',#99173,0.0999999999999994) ;
#32943=CIRCLE('',#99180,0.0999999999999998) ;
#32944=CIRCLE('',#99181,0.0999999999999998) ;
#32945=CIRCLE('',#99184,0.0999999999999998) ;
#32946=CIRCLE('',#99185,0.0999999999999998) ;
#32947=CIRCLE('',#99186,0.0999999999999998) ;
#32948=CIRCLE('',#99189,0.1) ;
#32949=CIRCLE('',#99191,0.1) ;
#32950=CIRCLE('',#99192,0.1) ;
#32951=CIRCLE('',#99195,0.1) ;
#32952=CIRCLE('',#99197,0.1) ;
#32953=CIRCLE('',#99198,0.1) ;
#32954=CIRCLE('',#99201,0.0999999999999998) ;
#32955=CIRCLE('',#99202,0.1) ;
#32956=CIRCLE('',#99205,0.1) ;
#32957=CIRCLE('',#99206,0.0999999999999999) ;
#32958=CIRCLE('',#99376,0.1) ;
#32959=CIRCLE('',#99377,0.0999999999999998) ;
#32960=CIRCLE('',#99378,0.0999999999999998) ;
#32961=CIRCLE('',#99379,0.1) ;
#32962=CIRCLE('',#99385,0.0999999999999994) ;
#32963=CIRCLE('',#99386,0.1) ;
#32964=CIRCLE('',#99387,0.1) ;
#32965=CIRCLE('',#99388,0.0999999999999994) ;
#32966=CIRCLE('',#99394,0.0999999999999994) ;
#32967=CIRCLE('',#99395,0.0999999999999994) ;
#32968=CIRCLE('',#99396,0.0999999999999994) ;
#32969=CIRCLE('',#99397,0.0999999999999994) ;
#32970=CIRCLE('',#99403,0.0999999999999994) ;
#32971=CIRCLE('',#99404,0.0999999999999994) ;
#32972=CIRCLE('',#99405,0.0999999999999994) ;
#32973=CIRCLE('',#99406,0.0999999999999994) ;
#32974=CIRCLE('',#99412,0.0999999999999994) ;
#32975=CIRCLE('',#99413,0.0999999999999994) ;
#32976=CIRCLE('',#99414,0.0999999999999994) ;
#32977=CIRCLE('',#99415,0.0999999999999994) ;
#32978=CIRCLE('',#99421,0.0999999999999994) ;
#32979=CIRCLE('',#99422,0.0999999999999994) ;
#32980=CIRCLE('',#99423,0.0999999999999994) ;
#32981=CIRCLE('',#99424,0.0999999999999994) ;
#32982=CIRCLE('',#99430,0.0999999999999994) ;
#32983=CIRCLE('',#99431,0.0999999999999994) ;
#32984=CIRCLE('',#99432,0.0999999999999994) ;
#32985=CIRCLE('',#99433,0.0999999999999994) ;
#32986=CIRCLE('',#99439,0.0999999999999994) ;
#32987=CIRCLE('',#99440,0.0999999999999994) ;
#32988=CIRCLE('',#99441,0.0999999999999994) ;
#32989=CIRCLE('',#99442,0.0999999999999994) ;
#32990=CIRCLE('',#99448,0.100000000000003) ;
#32991=CIRCLE('',#99449,0.100000000000003) ;
#32992=CIRCLE('',#99450,0.100000000000003) ;
#32993=CIRCLE('',#99451,0.100000000000003) ;
#32994=CIRCLE('',#99466,0.2) ;
#32995=CIRCLE('',#99467,0.2) ;
#32996=CIRCLE('',#99468,0.2) ;
#32997=CIRCLE('',#99471,0.2) ;
#32998=CIRCLE('',#99472,0.2) ;
#32999=CIRCLE('',#99473,0.2) ;
#33000=CIRCLE('',#99476,0.2) ;
#33001=CIRCLE('',#99477,0.2) ;
#33002=CIRCLE('',#99478,0.2) ;
#33003=CIRCLE('',#99481,0.2) ;
#33004=CIRCLE('',#99482,0.2) ;
#33005=CIRCLE('',#99483,0.2) ;
#33006=CIRCLE('',#99486,0.2) ;
#33007=CIRCLE('',#99487,0.2) ;
#33008=CIRCLE('',#99488,0.2) ;
#33009=CIRCLE('',#99491,0.2) ;
#33010=CIRCLE('',#99492,0.2) ;
#33011=CIRCLE('',#99493,0.2) ;
#33012=CIRCLE('',#99496,0.2) ;
#33013=CIRCLE('',#99497,0.2) ;
#33014=CIRCLE('',#99498,0.2) ;
#33015=CIRCLE('',#99501,0.2) ;
#33016=CIRCLE('',#99502,0.2) ;
#33017=CIRCLE('',#99503,0.2) ;
#33018=CIRCLE('',#99506,0.2) ;
#33019=CIRCLE('',#99507,0.2) ;
#33020=CIRCLE('',#99508,0.2) ;
#33021=CIRCLE('',#99511,0.2) ;
#33022=CIRCLE('',#99512,0.2) ;
#33023=CIRCLE('',#99513,0.2) ;
#33024=CIRCLE('',#99516,0.2) ;
#33025=CIRCLE('',#99517,0.2) ;
#33026=CIRCLE('',#99518,0.2) ;
#33027=CIRCLE('',#99521,0.2) ;
#33028=CIRCLE('',#99522,0.2) ;
#33029=CIRCLE('',#99523,0.2) ;
#33030=CIRCLE('',#99526,0.2) ;
#33031=CIRCLE('',#99527,0.2) ;
#33032=CIRCLE('',#99528,0.2) ;
#33033=CIRCLE('',#99531,0.2) ;
#33034=CIRCLE('',#99532,0.2) ;
#33035=CIRCLE('',#99533,0.2) ;
#33036=CIRCLE('',#99536,0.2) ;
#33037=CIRCLE('',#99537,0.2) ;
#33038=CIRCLE('',#99538,0.2) ;
#33039=CIRCLE('',#99541,0.2) ;
#33040=CIRCLE('',#99542,0.2) ;
#33041=CIRCLE('',#99543,0.2) ;
#33042=CIRCLE('',#99546,0.2) ;
#33043=CIRCLE('',#99547,0.2) ;
#33044=CIRCLE('',#99548,0.2) ;
#33045=CIRCLE('',#99551,0.2) ;
#33046=CIRCLE('',#99552,0.2) ;
#33047=CIRCLE('',#99553,0.2) ;
#33048=CIRCLE('',#99558,1.65625) ;
#33049=CIRCLE('',#99559,1.65625) ;
#33050=CIRCLE('',#99561,1.75625) ;
#33051=CIRCLE('',#99565,1.65625) ;
#33052=CIRCLE('',#99566,1.65625) ;
#33053=CIRCLE('',#99568,1.75625) ;
#33054=CIRCLE('',#99572,1.65625) ;
#33055=CIRCLE('',#99573,1.65625) ;
#33056=CIRCLE('',#99575,1.75625) ;
#33057=CIRCLE('',#99579,1.65625) ;
#33058=CIRCLE('',#99580,1.65625) ;
#33059=CIRCLE('',#99582,1.75625) ;
#33060=CIRCLE('',#99586,1.65625) ;
#33061=CIRCLE('',#99587,1.65625) ;
#33062=CIRCLE('',#99589,1.75625) ;
#33063=CIRCLE('',#99593,1.65625) ;
#33064=CIRCLE('',#99594,1.65625) ;
#33065=CIRCLE('',#99596,1.75625) ;
#33066=CIRCLE('',#99600,1.65625) ;
#33067=CIRCLE('',#99601,1.65625) ;
#33068=CIRCLE('',#99603,1.75625) ;
#33069=CIRCLE('',#99607,1.65625) ;
#33070=CIRCLE('',#99608,1.65625) ;
#33071=CIRCLE('',#99610,1.75625) ;
#33072=CIRCLE('',#99614,1.65625) ;
#33073=CIRCLE('',#99615,1.65625) ;
#33074=CIRCLE('',#99617,1.75625) ;
#33075=CIRCLE('',#99664,0.0999999999999998) ;
#33076=CIRCLE('',#99665,0.1) ;
#33077=CIRCLE('',#99666,0.1) ;
#33078=CIRCLE('',#99667,0.0999999999999998) ;
#33079=CIRCLE('',#99673,0.1) ;
#33080=CIRCLE('',#99674,0.0999999999999994) ;
#33081=CIRCLE('',#99675,0.0999999999999994) ;
#33082=CIRCLE('',#99676,0.1) ;
#33083=CIRCLE('',#99682,0.0999999999999994) ;
#33084=CIRCLE('',#99683,0.0999999999999994) ;
#33085=CIRCLE('',#99684,0.0999999999999994) ;
#33086=CIRCLE('',#99685,0.0999999999999994) ;
#33087=CIRCLE('',#99691,0.0999999999999994) ;
#33088=CIRCLE('',#99692,0.0999999999999994) ;
#33089=CIRCLE('',#99693,0.0999999999999994) ;
#33090=CIRCLE('',#99694,0.0999999999999994) ;
#33091=CIRCLE('',#99700,0.0999999999999994) ;
#33092=CIRCLE('',#99701,0.0999999999999994) ;
#33093=CIRCLE('',#99702,0.0999999999999994) ;
#33094=CIRCLE('',#99703,0.0999999999999994) ;
#33095=CIRCLE('',#99709,0.0999999999999994) ;
#33096=CIRCLE('',#99710,0.0999999999999994) ;
#33097=CIRCLE('',#99711,0.0999999999999994) ;
#33098=CIRCLE('',#99712,0.0999999999999994) ;
#33099=CIRCLE('',#99718,0.0999999999999994) ;
#33100=CIRCLE('',#99719,0.0999999999999994) ;
#33101=CIRCLE('',#99720,0.0999999999999994) ;
#33102=CIRCLE('',#99721,0.0999999999999994) ;
#33103=CIRCLE('',#99727,0.0999999999999994) ;
#33104=CIRCLE('',#99728,0.0999999999999994) ;
#33105=CIRCLE('',#99729,0.0999999999999994) ;
#33106=CIRCLE('',#99730,0.0999999999999994) ;
#33107=CIRCLE('',#99736,0.100000000000003) ;
#33108=CIRCLE('',#99737,0.100000000000003) ;
#33109=CIRCLE('',#99738,0.100000000000003) ;
#33110=CIRCLE('',#99739,0.100000000000003) ;
#33111=CIRCLE('',#99790,0.0999999999999994) ;
#33112=CIRCLE('',#99791,0.0999999999999994) ;
#33113=CIRCLE('',#99794,0.1) ;
#33114=CIRCLE('',#99795,0.1) ;
#33115=CIRCLE('',#99798,0.1) ;
#33116=CIRCLE('',#99799,0.1) ;
#33117=CIRCLE('',#99802,0.0999999999999998) ;
#33118=CIRCLE('',#99803,0.0999999999999998) ;
#33119=CIRCLE('',#99807,0.0999999999999994) ;
#33120=CIRCLE('',#99808,0.0999999999999994) ;
#33121=CIRCLE('',#99811,0.0999999999999994) ;
#33122=CIRCLE('',#99812,0.0999999999999994) ;
#33123=CIRCLE('',#99815,0.1) ;
#33124=CIRCLE('',#99816,0.1) ;
#33125=CIRCLE('',#99819,0.0999999999999994) ;
#33126=CIRCLE('',#99820,0.0999999999999994) ;
#33127=CIRCLE('',#99824,0.0999999999999994) ;
#33128=CIRCLE('',#99825,0.0999999999999994) ;
#33129=CIRCLE('',#99828,0.0999999999999994) ;
#33130=CIRCLE('',#99829,0.0999999999999994) ;
#33131=CIRCLE('',#99832,0.0999999999999994) ;
#33132=CIRCLE('',#99833,0.0999999999999994) ;
#33133=CIRCLE('',#99836,0.0999999999999994) ;
#33134=CIRCLE('',#99837,0.0999999999999994) ;
#33135=CIRCLE('',#99841,0.0999999999999994) ;
#33136=CIRCLE('',#99842,0.0999999999999994) ;
#33137=CIRCLE('',#99845,0.0999999999999994) ;
#33138=CIRCLE('',#99846,0.0999999999999994) ;
#33139=CIRCLE('',#99849,0.0999999999999994) ;
#33140=CIRCLE('',#99850,0.0999999999999994) ;
#33141=CIRCLE('',#99853,0.0999999999999994) ;
#33142=CIRCLE('',#99854,0.0999999999999994) ;
#33143=CIRCLE('',#99858,0.0999999999999994) ;
#33144=CIRCLE('',#99859,0.0999999999999994) ;
#33145=CIRCLE('',#99862,0.0999999999999994) ;
#33146=CIRCLE('',#99863,0.0999999999999994) ;
#33147=CIRCLE('',#99866,0.0999999999999994) ;
#33148=CIRCLE('',#99867,0.0999999999999994) ;
#33149=CIRCLE('',#99870,0.0999999999999994) ;
#33150=CIRCLE('',#99871,0.0999999999999994) ;
#33151=CIRCLE('',#99875,0.0999999999999994) ;
#33152=CIRCLE('',#99876,0.0999999999999994) ;
#33153=CIRCLE('',#99879,0.0999999999999994) ;
#33154=CIRCLE('',#99880,0.0999999999999994) ;
#33155=CIRCLE('',#99883,0.0999999999999994) ;
#33156=CIRCLE('',#99884,0.0999999999999994) ;
#33157=CIRCLE('',#99887,0.0999999999999994) ;
#33158=CIRCLE('',#99888,0.0999999999999994) ;
#33159=CIRCLE('',#99892,0.0999999999999994) ;
#33160=CIRCLE('',#99893,0.0999999999999994) ;
#33161=CIRCLE('',#99896,0.0999999999999994) ;
#33162=CIRCLE('',#99897,0.0999999999999994) ;
#33163=CIRCLE('',#99900,0.0999999999999994) ;
#33164=CIRCLE('',#99901,0.0999999999999994) ;
#33165=CIRCLE('',#99904,0.0999999999999994) ;
#33166=CIRCLE('',#99905,0.0999999999999994) ;
#33167=CIRCLE('',#99909,0.0999999999999994) ;
#33168=CIRCLE('',#99910,0.0999999999999994) ;
#33169=CIRCLE('',#99913,0.0999999999999994) ;
#33170=CIRCLE('',#99914,0.0999999999999994) ;
#33171=CIRCLE('',#99917,0.0999999999999994) ;
#33172=CIRCLE('',#99918,0.0999999999999994) ;
#33173=CIRCLE('',#99921,0.0999999999999994) ;
#33174=CIRCLE('',#99922,0.0999999999999994) ;
#33175=CIRCLE('',#99926,0.100000000000003) ;
#33176=CIRCLE('',#99927,0.100000000000003) ;
#33177=CIRCLE('',#99930,0.100000000000003) ;
#33178=CIRCLE('',#99931,0.100000000000003) ;
#33179=CIRCLE('',#99934,0.100000000000003) ;
#33180=CIRCLE('',#99935,0.100000000000003) ;
#33181=CIRCLE('',#99938,0.100000000000003) ;
#33182=CIRCLE('',#99939,0.100000000000003) ;
#33183=CIRCLE('',#99943,0.0999999999999994) ;
#33184=CIRCLE('',#99944,0.0999999999999999) ;
#33185=CIRCLE('',#99945,0.1) ;
#33186=CIRCLE('',#99947,0.1) ;
#33187=CIRCLE('',#99949,0.1) ;
#33188=CIRCLE('',#99951,0.0999999999999998) ;
#33189=CIRCLE('',#99953,0.1) ;
#33190=CIRCLE('',#99954,0.1) ;
#33191=CIRCLE('',#99956,0.0999999999999994) ;
#33192=CIRCLE('',#99957,0.0999999999999994) ;
#33193=CIRCLE('',#99959,0.0999999999999998) ;
#33194=CIRCLE('',#99960,0.0999999999999998) ;
#33195=CIRCLE('',#99962,0.0999999999999998) ;
#33196=CIRCLE('',#99963,0.1) ;
#33197=CIRCLE('',#99965,0.1) ;
#33198=CIRCLE('',#99967,0.0999999999999998) ;
#33199=CIRCLE('',#99968,0.0999999999999998) ;
#33200=CIRCLE('',#99970,0.0999999999999994) ;
#33201=CIRCLE('',#99972,0.0999999999999998) ;
#33202=CIRCLE('',#99974,0.1) ;
#33203=CIRCLE('',#99976,0.0999999999999998) ;
#33204=CIRCLE('',#99978,0.1) ;
#33205=CIRCLE('',#99980,0.0999999999999998) ;
#33206=CIRCLE('',#99982,0.0999999999999998) ;
#33207=CIRCLE('',#99984,0.1) ;
#33208=CIRCLE('',#99986,0.0999999999999998) ;
#33209=CIRCLE('',#99988,0.0999999999999998) ;
#33210=CIRCLE('',#99990,0.1) ;
#33211=CIRCLE('',#99992,0.1) ;
#33212=CIRCLE('',#99993,0.1) ;
#33213=CIRCLE('',#99995,0.1) ;
#33214=CIRCLE('',#99996,0.0999999999999998) ;
#33215=CIRCLE('',#99998,0.0999999999999998) ;
#33216=CIRCLE('',#100000,0.1) ;
#33217=CIRCLE('',#100001,0.1) ;
#33218=CIRCLE('',#100003,0.1) ;
#33219=CIRCLE('',#100005,0.0999999999999998) ;
#33220=CIRCLE('',#100007,0.0999999999999998) ;
#33221=CIRCLE('',#100009,0.1) ;
#33222=CIRCLE('',#100011,0.1) ;
#33223=CIRCLE('',#100013,0.0999999999999998) ;
#33224=CIRCLE('',#100015,0.0999999999999998) ;
#33225=CIRCLE('',#100017,0.0999999999999998) ;
#33226=CIRCLE('',#100018,0.0999999999999998) ;
#33227=CIRCLE('',#100020,0.1) ;
#33228=CIRCLE('',#100022,0.0999999999999998) ;
#33229=CIRCLE('',#100024,0.0999999999999998) ;
#33230=CIRCLE('',#100026,0.0999999999999998) ;
#33231=CIRCLE('',#100029,0.1) ;
#33232=CIRCLE('',#100030,0.0999999999999998) ;
#33233=CIRCLE('',#100032,0.0999999999999998) ;
#33234=CIRCLE('',#100034,0.1) ;
#33235=CIRCLE('',#100036,0.0999999999999998) ;
#33236=CIRCLE('',#100038,0.0999999999999994) ;
#33237=CIRCLE('',#100040,0.0999999999999998) ;
#33238=CIRCLE('',#100042,0.0999999999999994) ;
#33239=CIRCLE('',#100141,0.0999999999999998) ;
#33240=CIRCLE('',#100142,0.0999999999999998) ;
#33241=CIRCLE('',#100144,0.1) ;
#33242=CIRCLE('',#100145,0.0999999999999998) ;
#33243=CIRCLE('',#100147,0.0999999999999998) ;
#33244=CIRCLE('',#100148,0.0999999999999998) ;
#33245=CIRCLE('',#100150,0.1) ;
#33246=CIRCLE('',#100152,0.0999999999999998) ;
#33247=CIRCLE('',#100154,0.0999999999999998) ;
#33248=CIRCLE('',#100155,0.0999999999999998) ;
#33249=CIRCLE('',#100157,0.0999999999999998) ;
#33250=CIRCLE('',#100159,0.0999999999999998) ;
#33251=CIRCLE('',#100161,0.1) ;
#33252=CIRCLE('',#100162,0.1) ;
#33253=CIRCLE('',#100164,0.1) ;
#33254=CIRCLE('',#100166,0.1) ;
#33255=CIRCLE('',#100168,0.1) ;
#33256=CIRCLE('',#100170,0.1) ;
#33257=CIRCLE('',#100172,0.1) ;
#33258=CIRCLE('',#100174,0.1) ;
#33259=CIRCLE('',#100176,0.0999999999999998) ;
#33260=CIRCLE('',#100178,0.1) ;
#33261=CIRCLE('',#100180,0.1) ;
#33262=CIRCLE('',#100182,0.1) ;
#33263=CIRCLE('',#100185,0.0999999999999998) ;
#33264=CIRCLE('',#100187,0.1) ;
#33265=CIRCLE('',#100188,0.1) ;
#33266=CIRCLE('',#100190,0.1) ;
#33267=CIRCLE('',#100192,0.0999999999999998) ;
#33268=CIRCLE('',#100194,0.1) ;
#33269=CIRCLE('',#100196,0.0999999999999998) ;
#33270=CIRCLE('',#100198,0.0999999999999998) ;
#33271=CIRCLE('',#100200,0.1) ;
#33272=CIRCLE('',#100202,0.1) ;
#33273=CIRCLE('',#100204,0.1) ;
#33274=CIRCLE('',#100206,0.1) ;
#33275=CIRCLE('',#100209,0.1) ;
#33276=CIRCLE('',#100211,0.1) ;
#33277=CIRCLE('',#100212,0.1) ;
#33278=CIRCLE('',#100215,0.1) ;
#33279=CIRCLE('',#100217,0.1) ;
#33280=CIRCLE('',#100218,0.1) ;
#33281=CIRCLE('',#100219,0.1) ;
#33282=CIRCLE('',#100221,0.0999999999999996) ;
#33283=CIRCLE('',#100223,0.1) ;
#33284=CIRCLE('',#100225,0.1) ;
#33285=CIRCLE('',#100227,0.1) ;
#33286=CIRCLE('',#100229,0.1) ;
#33287=CIRCLE('',#100233,0.1) ;
#33288=CIRCLE('',#100234,0.0999999999999998) ;
#33289=CIRCLE('',#100235,0.1) ;
#33290=CIRCLE('',#100237,0.0999999999999998) ;
#33291=CIRCLE('',#100239,0.1) ;
#33292=CIRCLE('',#100241,0.0999999999999998) ;
#33293=CIRCLE('',#100243,0.1) ;
#33294=CIRCLE('',#100245,0.0999999999999996) ;
#33295=CIRCLE('',#100409,0.1) ;
#33296=CIRCLE('',#100410,0.1) ;
#33297=CIRCLE('',#100412,0.0999999999999998) ;
#33298=CIRCLE('',#100413,0.0999999999999998) ;
#33299=CIRCLE('',#100415,0.0999999999999998) ;
#33300=CIRCLE('',#100416,0.1) ;
#33301=CIRCLE('',#100418,0.0999999999999998) ;
#33302=CIRCLE('',#100420,0.1) ;
#33303=CIRCLE('',#100422,0.1) ;
#33304=CIRCLE('',#100423,0.1) ;
#33305=CIRCLE('',#100425,0.1) ;
#33306=CIRCLE('',#100427,0.1) ;
#33307=CIRCLE('',#100429,0.0999999999999998) ;
#33308=CIRCLE('',#100430,0.0999999999999998) ;
#33309=CIRCLE('',#100432,0.0999999999999998) ;
#33310=CIRCLE('',#100434,0.0999999999999998) ;
#33311=CIRCLE('',#100436,0.0999999999999998) ;
#33312=CIRCLE('',#100438,0.0999999999999998) ;
#33313=CIRCLE('',#100440,0.0999999999999998) ;
#33314=CIRCLE('',#100442,0.0999999999999998) ;
#33315=CIRCLE('',#100444,0.1) ;
#33316=CIRCLE('',#100446,0.0999999999999998) ;
#33317=CIRCLE('',#100448,0.0999999999999998) ;
#33318=CIRCLE('',#100450,0.0999999999999998) ;
#33319=CIRCLE('',#100453,0.1) ;
#33320=CIRCLE('',#100455,0.0999999999999998) ;
#33321=CIRCLE('',#100456,0.0999999999999998) ;
#33322=CIRCLE('',#100458,0.0999999999999998) ;
#33323=CIRCLE('',#100460,0.1) ;
#33324=CIRCLE('',#100462,0.0999999999999998) ;
#33325=CIRCLE('',#100464,0.1) ;
#33326=CIRCLE('',#100466,0.1) ;
#33327=CIRCLE('',#100468,0.0999999999999998) ;
#33328=CIRCLE('',#100470,0.0999999999999998) ;
#33329=CIRCLE('',#100472,0.0999999999999998) ;
#33330=CIRCLE('',#100474,0.0999999999999998) ;
#33331=CIRCLE('',#100477,0.1) ;
#33332=CIRCLE('',#100478,0.0999999999999994) ;
#33333=CIRCLE('',#100480,0.0999999999999998) ;
#33334=CIRCLE('',#100482,0.1) ;
#33335=CIRCLE('',#100484,0.0999999999999998) ;
#33336=CIRCLE('',#100486,0.1) ;
#33337=CIRCLE('',#100488,0.0999999999999994) ;
#33338=CIRCLE('',#100490,0.0999999999999994) ;
#33339=CIRCLE('',#100497,0.1) ;
#33340=CIRCLE('',#100498,0.0999999999999998) ;
#33341=CIRCLE('',#100499,0.1) ;
#33342=CIRCLE('',#100501,0.0999999999999994) ;
#33343=CIRCLE('',#100503,0.1) ;
#33344=CIRCLE('',#100505,0.1) ;
#33345=CIRCLE('',#100507,0.1) ;
#33346=CIRCLE('',#100508,0.1) ;
#33347=CIRCLE('',#100510,0.1) ;
#33348=CIRCLE('',#100512,0.1) ;
#33349=CIRCLE('',#100513,0.0999999999999998) ;
#33350=CIRCLE('',#100515,0.0999999999999994) ;
#33351=CIRCLE('',#100516,0.0999999999999994) ;
#33352=CIRCLE('',#100518,0.0999999999999994) ;
#33353=CIRCLE('',#100519,0.0999999999999994) ;
#33354=CIRCLE('',#100521,0.1) ;
#33355=CIRCLE('',#100523,0.0999999999999998) ;
#33356=CIRCLE('',#100525,0.1) ;
#33357=CIRCLE('',#100527,0.0999999999999994) ;
#33358=CIRCLE('',#100529,0.0999999999999994) ;
#33359=CIRCLE('',#100531,0.0999999999999994) ;
#33360=CIRCLE('',#100532,0.0999999999999994) ;
#33361=CIRCLE('',#100534,0.1) ;
#33362=CIRCLE('',#100536,0.0999999999999998) ;
#33363=CIRCLE('',#100538,0.0999999999999994) ;
#33364=CIRCLE('',#100540,0.1) ;
#33365=CIRCLE('',#100541,0.1) ;
#33366=CIRCLE('',#100543,0.1) ;
#33367=CIRCLE('',#100545,0.0999999999999998) ;
#33368=CIRCLE('',#100547,0.0999999999999994) ;
#33369=CIRCLE('',#100549,0.0999999999999998) ;
#33370=CIRCLE('',#100551,0.0999999999999998) ;
#33371=CIRCLE('',#100552,0.1) ;
#33372=CIRCLE('',#100554,0.0999999999999994) ;
#33373=CIRCLE('',#100556,0.1) ;
#33374=CIRCLE('',#100558,0.1) ;
#33375=CIRCLE('',#100560,0.0999999999999998) ;
#33376=CIRCLE('',#100562,0.0999999999999994) ;
#33377=CIRCLE('',#100564,0.0999999999999998) ;
#33378=CIRCLE('',#100566,0.0999999999999994) ;
#33379=CIRCLE('',#100568,0.0999999999999998) ;
#33380=CIRCLE('',#100570,0.1) ;
#33381=CIRCLE('',#100572,0.0999999999999994) ;
#33382=CIRCLE('',#100573,0.0999999999999994) ;
#33383=CIRCLE('',#100575,0.1) ;
#33384=CIRCLE('',#100576,0.0999999999999998) ;
#33385=CIRCLE('',#100578,0.0999999999999994) ;
#33386=CIRCLE('',#100580,0.0999999999999994) ;
#33387=CIRCLE('',#100582,0.1) ;
#33388=CIRCLE('',#100584,0.1) ;
#33389=CIRCLE('',#100585,0.1) ;
#33390=CIRCLE('',#100587,0.1) ;
#33391=CIRCLE('',#100588,0.1) ;
#33392=CIRCLE('',#100589,0.0999999999999994) ;
#33393=CIRCLE('',#100591,0.1) ;
#33394=CIRCLE('',#100593,0.1) ;
#33395=CIRCLE('',#100595,0.1) ;
#33396=CIRCLE('',#100597,0.0999999999999994) ;
#33397=CIRCLE('',#100599,0.1) ;
#33398=CIRCLE('',#100601,0.0999999999999994) ;
#33399=CIRCLE('',#100603,0.1) ;
#33400=CIRCLE('',#100605,0.0999999999999994) ;
#33401=CIRCLE('',#100607,0.0999999999999994) ;
#33402=CIRCLE('',#100609,0.0999999999999994) ;
#33403=CIRCLE('',#100610,0.0999999999999996) ;
#33404=CIRCLE('',#100611,0.0999999999999996) ;
#33405=CIRCLE('',#100613,0.1) ;
#33406=CIRCLE('',#100615,0.1) ;
#33407=CIRCLE('',#100617,0.1) ;
#33408=CIRCLE('',#100619,0.1) ;
#33409=CIRCLE('',#100621,0.1) ;
#33410=CIRCLE('',#100623,0.1) ;
#33411=CIRCLE('',#100625,0.1) ;
#33412=CIRCLE('',#100626,0.0999999999999995) ;
#33413=CIRCLE('',#100627,0.0999999999999998) ;
#33414=CIRCLE('',#100628,0.1) ;
#33415=CIRCLE('',#100630,0.1) ;
#33416=CIRCLE('',#100632,0.1) ;
#33417=CIRCLE('',#100634,0.0999999999999994) ;
#33418=CIRCLE('',#100636,0.0999999999999994) ;
#33419=CIRCLE('',#100638,0.1) ;
#33420=CIRCLE('',#100640,0.1) ;
#33421=CIRCLE('',#100642,0.0999999999999996) ;
#33422=CIRCLE('',#100643,0.0999999999999996) ;
#33423=CIRCLE('',#100645,0.0999999999999994) ;
#33424=CIRCLE('',#100646,0.1) ;
#33425=CIRCLE('',#100648,0.0999999999999998) ;
#33426=CIRCLE('',#100650,0.0999999999999994) ;
#33427=CIRCLE('',#100652,0.1) ;
#33428=CIRCLE('',#100654,0.0999999999999994) ;
#33429=CIRCLE('',#100656,0.0999999999999998) ;
#33430=CIRCLE('',#100658,0.0999999999999994) ;
#33431=CIRCLE('',#100661,0.1) ;
#33432=CIRCLE('',#100663,0.1) ;
#33433=CIRCLE('',#100664,0.1) ;
#33434=CIRCLE('',#100666,0.0999999999999994) ;
#33435=CIRCLE('',#100668,0.1) ;
#33436=CIRCLE('',#100670,0.0999999999999994) ;
#33437=CIRCLE('',#100672,0.1) ;
#33438=CIRCLE('',#100674,0.1) ;
#33439=CIRCLE('',#100676,0.0999999999999994) ;
#33440=CIRCLE('',#100678,0.0999999999999994) ;
#33441=CIRCLE('',#100680,0.1) ;
#33442=CIRCLE('',#100682,0.1) ;
#33443=CIRCLE('',#100685,0.0999999999999994) ;
#33444=CIRCLE('',#100686,0.0999999999999994) ;
#33445=CIRCLE('',#100688,0.0999999999999998) ;
#33446=CIRCLE('',#100689,0.0999999999999998) ;
#33447=CIRCLE('',#100691,0.0999999999999998) ;
#33448=CIRCLE('',#100692,0.1) ;
#33449=CIRCLE('',#100694,0.0999999999999998) ;
#33450=CIRCLE('',#100696,0.0999999999999994) ;
#33451=CIRCLE('',#100698,0.0999999999999994) ;
#33452=CIRCLE('',#100699,0.0999999999999994) ;
#33453=CIRCLE('',#100701,0.0999999999999994) ;
#33454=CIRCLE('',#100703,0.1) ;
#33455=CIRCLE('',#100705,0.1) ;
#33456=CIRCLE('',#100706,0.1) ;
#33457=CIRCLE('',#100708,0.0999999999999998) ;
#33458=CIRCLE('',#100710,0.0999999999999998) ;
#33459=CIRCLE('',#100712,0.0999999999999998) ;
#33460=CIRCLE('',#100714,0.0999999999999998) ;
#33461=CIRCLE('',#100716,0.1) ;
#33462=CIRCLE('',#100718,0.0999999999999998) ;
#33463=CIRCLE('',#100720,0.0999999999999998) ;
#33464=CIRCLE('',#100722,0.1) ;
#33465=CIRCLE('',#100724,0.1) ;
#33466=CIRCLE('',#100726,0.1) ;
#33467=CIRCLE('',#100729,0.0999999999999994) ;
#33468=CIRCLE('',#100731,0.0999999999999998) ;
#33469=CIRCLE('',#100732,0.0999999999999998) ;
#33470=CIRCLE('',#100734,0.1) ;
#33471=CIRCLE('',#100736,0.0999999999999994) ;
#33472=CIRCLE('',#100738,0.1) ;
#33473=CIRCLE('',#100740,0.0999999999999994) ;
#33474=CIRCLE('',#100742,0.0999999999999994) ;
#33475=CIRCLE('',#100744,0.1) ;
#33476=CIRCLE('',#100746,0.1) ;
#33477=CIRCLE('',#100748,0.0999999999999998) ;
#33478=CIRCLE('',#100750,0.0999999999999998) ;
#33479=CIRCLE('',#100753,0.1) ;
#33480=CIRCLE('',#100754,0.0999999999999994) ;
#33481=CIRCLE('',#100756,0.1) ;
#33482=CIRCLE('',#100758,0.0999999999999994) ;
#33483=CIRCLE('',#100760,0.1) ;
#33484=CIRCLE('',#100762,0.0999999999999994) ;
#33485=CIRCLE('',#100764,0.0999999999999994) ;
#33486=CIRCLE('',#100766,0.0999999999999994) ;
#33487=CIRCLE('',#100773,0.1) ;
#33488=CIRCLE('',#100774,0.0999999999999998) ;
#33489=CIRCLE('',#100775,0.0999999999999994) ;
#33490=CIRCLE('',#100777,0.0999999999999994) ;
#33491=CIRCLE('',#100779,0.0999999999999994) ;
#33492=CIRCLE('',#100781,0.1) ;
#33493=CIRCLE('',#100783,0.0999999999999994) ;
#33494=CIRCLE('',#100784,0.0999999999999994) ;
#33495=CIRCLE('',#100786,0.0999999999999994) ;
#33496=CIRCLE('',#100788,0.1) ;
#33497=CIRCLE('',#100789,0.0999999999999998) ;
#33498=CIRCLE('',#100791,0.0999999999999994) ;
#33499=CIRCLE('',#100792,0.0999999999999994) ;
#33500=CIRCLE('',#100794,0.0999999999999994) ;
#33501=CIRCLE('',#100795,0.0999999999999994) ;
#33502=CIRCLE('',#100797,0.0999999999999994) ;
#33503=CIRCLE('',#100799,0.0999999999999998) ;
#33504=CIRCLE('',#100801,0.1) ;
#33505=CIRCLE('',#100803,0.0999999999999994) ;
#33506=CIRCLE('',#100805,0.0999999999999994) ;
#33507=CIRCLE('',#100807,0.0999999999999994) ;
#33508=CIRCLE('',#100808,0.0999999999999994) ;
#33509=CIRCLE('',#100810,0.0999999999999994) ;
#33510=CIRCLE('',#100812,0.0999999999999998) ;
#33511=CIRCLE('',#100814,0.0999999999999994) ;
#33512=CIRCLE('',#100816,0.0999999999999994) ;
#33513=CIRCLE('',#100817,0.0999999999999994) ;
#33514=CIRCLE('',#100819,0.0999999999999994) ;
#33515=CIRCLE('',#100821,0.0999999999999998) ;
#33516=CIRCLE('',#100823,0.0999999999999994) ;
#33517=CIRCLE('',#100825,0.0999999999999998) ;
#33518=CIRCLE('',#100827,0.0999999999999998) ;
#33519=CIRCLE('',#100828,0.0999999999999994) ;
#33520=CIRCLE('',#100830,0.0999999999999994) ;
#33521=CIRCLE('',#100832,0.0999999999999994) ;
#33522=CIRCLE('',#100834,0.1) ;
#33523=CIRCLE('',#100836,0.0999999999999998) ;
#33524=CIRCLE('',#100838,0.0999999999999994) ;
#33525=CIRCLE('',#100840,0.0999999999999998) ;
#33526=CIRCLE('',#100842,0.0999999999999994) ;
#33527=CIRCLE('',#100844,0.0999999999999998) ;
#33528=CIRCLE('',#100846,0.1) ;
#33529=CIRCLE('',#100848,0.0999999999999994) ;
#33530=CIRCLE('',#100849,0.0999999999999994) ;
#33531=CIRCLE('',#100851,0.1) ;
#33532=CIRCLE('',#100852,0.0999999999999998) ;
#33533=CIRCLE('',#100854,0.0999999999999994) ;
#33534=CIRCLE('',#100856,0.0999999999999994) ;
#33535=CIRCLE('',#100858,0.0999999999999994) ;
#33536=CIRCLE('',#100860,0.0999999999999994) ;
#33537=CIRCLE('',#100861,0.0999999999999994) ;
#33538=CIRCLE('',#100863,0.1) ;
#33539=CIRCLE('',#100864,0.0999999999999994) ;
#33540=CIRCLE('',#100865,0.0999999999999994) ;
#33541=CIRCLE('',#100867,0.0999999999999994) ;
#33542=CIRCLE('',#100869,0.0999999999999994) ;
#33543=CIRCLE('',#100871,0.1) ;
#33544=CIRCLE('',#100873,0.0999999999999994) ;
#33545=CIRCLE('',#100875,0.1) ;
#33546=CIRCLE('',#100877,0.0999999999999994) ;
#33547=CIRCLE('',#100879,0.1) ;
#33548=CIRCLE('',#100881,0.0999999999999994) ;
#33549=CIRCLE('',#100883,0.0999999999999994) ;
#33550=CIRCLE('',#100885,0.0999999999999994) ;
#33551=CIRCLE('',#100886,0.0999999999999996) ;
#33552=CIRCLE('',#100887,0.0999999999999996) ;
#33553=CIRCLE('',#100889,0.0999999999999996) ;
#33554=CIRCLE('',#100891,0.0999999999999994) ;
#33555=CIRCLE('',#100893,0.1) ;
#33556=CIRCLE('',#100895,0.1) ;
#33557=CIRCLE('',#100897,0.1) ;
#33558=CIRCLE('',#100899,0.1) ;
#33559=CIRCLE('',#100901,0.1) ;
#33560=CIRCLE('',#100902,0.100000000000001) ;
#33561=CIRCLE('',#100903,0.1) ;
#33562=CIRCLE('',#100904,0.1) ;
#33563=CIRCLE('',#100906,0.1) ;
#33564=CIRCLE('',#100908,0.1) ;
#33565=CIRCLE('',#100910,0.1) ;
#33566=CIRCLE('',#100912,0.0999999999999994) ;
#33567=CIRCLE('',#100914,0.1) ;
#33568=CIRCLE('',#100916,0.1) ;
#33569=CIRCLE('',#100918,0.0999999999999996) ;
#33570=CIRCLE('',#100919,0.0999999999999996) ;
#33571=CIRCLE('',#100921,0.0999999999999994) ;
#33572=CIRCLE('',#100922,0.1) ;
#33573=CIRCLE('',#100924,0.1) ;
#33574=CIRCLE('',#100926,0.0999999999999994) ;
#33575=CIRCLE('',#100928,0.0999999999999994) ;
#33576=CIRCLE('',#100930,0.0999999999999994) ;
#33577=CIRCLE('',#100932,0.0999999999999998) ;
#33578=CIRCLE('',#100934,0.0999999999999994) ;
#33579=CIRCLE('',#100937,0.0999999999999994) ;
#33580=CIRCLE('',#100939,0.1) ;
#33581=CIRCLE('',#100940,0.1) ;
#33582=CIRCLE('',#100942,0.0999999999999994) ;
#33583=CIRCLE('',#100944,0.0999999999999994) ;
#33584=CIRCLE('',#100946,0.0999999999999994) ;
#33585=CIRCLE('',#100948,0.0999999999999994) ;
#33586=CIRCLE('',#100950,0.0999999999999994) ;
#33587=CIRCLE('',#100952,0.0999999999999994) ;
#33588=CIRCLE('',#100954,0.0999999999999994) ;
#33589=CIRCLE('',#100956,0.1) ;
#33590=CIRCLE('',#100958,0.1) ;
#33591=CIRCLE('',#100961,0.0999999999999994) ;
#33592=CIRCLE('',#100962,0.0999999999999994) ;
#33593=CIRCLE('',#100964,0.0999999999999998) ;
#33594=CIRCLE('',#100965,0.0999999999999998) ;
#33595=CIRCLE('',#100967,0.0999999999999998) ;
#33596=CIRCLE('',#100968,0.1) ;
#33597=CIRCLE('',#100970,0.0999999999999998) ;
#33598=CIRCLE('',#100972,0.0999999999999994) ;
#33599=CIRCLE('',#100974,0.0999999999999994) ;
#33600=CIRCLE('',#100975,0.0999999999999994) ;
#33601=CIRCLE('',#100977,0.0999999999999994) ;
#33602=CIRCLE('',#100979,0.1) ;
#33603=CIRCLE('',#100981,0.0999999999999994) ;
#33604=CIRCLE('',#100982,0.0999999999999994) ;
#33605=CIRCLE('',#100984,0.0999999999999998) ;
#33606=CIRCLE('',#100986,0.0999999999999998) ;
#33607=CIRCLE('',#100988,0.0999999999999998) ;
#33608=CIRCLE('',#100990,0.0999999999999998) ;
#33609=CIRCLE('',#100992,0.0999999999999994) ;
#33610=CIRCLE('',#100994,0.0999999999999998) ;
#33611=CIRCLE('',#100996,0.0999999999999998) ;
#33612=CIRCLE('',#100998,0.0999999999999994) ;
#33613=CIRCLE('',#101000,0.0999999999999994) ;
#33614=CIRCLE('',#101002,0.0999999999999994) ;
#33615=CIRCLE('',#101005,0.0999999999999994) ;
#33616=CIRCLE('',#101007,0.0999999999999998) ;
#33617=CIRCLE('',#101008,0.0999999999999998) ;
#33618=CIRCLE('',#101010,0.0999999999999994) ;
#33619=CIRCLE('',#101012,0.0999999999999994) ;
#33620=CIRCLE('',#101014,0.0999999999999994) ;
#33621=CIRCLE('',#101016,0.0999999999999994) ;
#33622=CIRCLE('',#101018,0.0999999999999994) ;
#33623=CIRCLE('',#101020,0.0999999999999994) ;
#33624=CIRCLE('',#101022,0.0999999999999994) ;
#33625=CIRCLE('',#101024,0.0999999999999998) ;
#33626=CIRCLE('',#101026,0.0999999999999998) ;
#33627=CIRCLE('',#101029,0.1) ;
#33628=CIRCLE('',#101030,0.0999999999999994) ;
#33629=CIRCLE('',#101032,0.0999999999999994) ;
#33630=CIRCLE('',#101034,0.0999999999999994) ;
#33631=CIRCLE('',#101036,0.0999999999999994) ;
#33632=CIRCLE('',#101038,0.0999999999999994) ;
#33633=CIRCLE('',#101040,0.0999999999999994) ;
#33634=CIRCLE('',#101042,0.0999999999999994) ;
#33635=CIRCLE('',#101049,0.1) ;
#33636=CIRCLE('',#101050,0.0999999999999998) ;
#33637=CIRCLE('',#101051,0.0999999999999994) ;
#33638=CIRCLE('',#101053,0.0999999999999994) ;
#33639=CIRCLE('',#101055,0.0999999999999994) ;
#33640=CIRCLE('',#101057,0.1) ;
#33641=CIRCLE('',#101059,0.0999999999999994) ;
#33642=CIRCLE('',#101060,0.0999999999999994) ;
#33643=CIRCLE('',#101062,0.0999999999999994) ;
#33644=CIRCLE('',#101064,0.1) ;
#33645=CIRCLE('',#101065,0.0999999999999998) ;
#33646=CIRCLE('',#101067,0.0999999999999994) ;
#33647=CIRCLE('',#101068,0.0999999999999994) ;
#33648=CIRCLE('',#101070,0.0999999999999994) ;
#33649=CIRCLE('',#101071,0.0999999999999994) ;
#33650=CIRCLE('',#101073,0.0999999999999994) ;
#33651=CIRCLE('',#101075,0.0999999999999998) ;
#33652=CIRCLE('',#101077,0.1) ;
#33653=CIRCLE('',#101079,0.0999999999999994) ;
#33654=CIRCLE('',#101081,0.0999999999999994) ;
#33655=CIRCLE('',#101083,0.0999999999999994) ;
#33656=CIRCLE('',#101084,0.0999999999999994) ;
#33657=CIRCLE('',#101086,0.0999999999999994) ;
#33658=CIRCLE('',#101088,0.0999999999999998) ;
#33659=CIRCLE('',#101090,0.0999999999999994) ;
#33660=CIRCLE('',#101092,0.0999999999999994) ;
#33661=CIRCLE('',#101093,0.0999999999999994) ;
#33662=CIRCLE('',#101095,0.0999999999999994) ;
#33663=CIRCLE('',#101097,0.0999999999999998) ;
#33664=CIRCLE('',#101099,0.0999999999999994) ;
#33665=CIRCLE('',#101101,0.0999999999999994) ;
#33666=CIRCLE('',#101103,0.0999999999999998) ;
#33667=CIRCLE('',#101104,0.0999999999999994) ;
#33668=CIRCLE('',#101106,0.0999999999999994) ;
#33669=CIRCLE('',#101108,0.0999999999999994) ;
#33670=CIRCLE('',#101110,0.1) ;
#33671=CIRCLE('',#101112,0.0999999999999998) ;
#33672=CIRCLE('',#101114,0.0999999999999994) ;
#33673=CIRCLE('',#101116,0.0999999999999998) ;
#33674=CIRCLE('',#101118,0.0999999999999994) ;
#33675=CIRCLE('',#101120,0.0999999999999998) ;
#33676=CIRCLE('',#101122,0.1) ;
#33677=CIRCLE('',#101124,0.0999999999999994) ;
#33678=CIRCLE('',#101125,0.0999999999999994) ;
#33679=CIRCLE('',#101127,0.1) ;
#33680=CIRCLE('',#101128,0.0999999999999998) ;
#33681=CIRCLE('',#101130,0.0999999999999994) ;
#33682=CIRCLE('',#101132,0.0999999999999994) ;
#33683=CIRCLE('',#101134,0.0999999999999994) ;
#33684=CIRCLE('',#101136,0.0999999999999994) ;
#33685=CIRCLE('',#101137,0.0999999999999994) ;
#33686=CIRCLE('',#101139,0.1) ;
#33687=CIRCLE('',#101140,0.0999999999999994) ;
#33688=CIRCLE('',#101141,0.0999999999999994) ;
#33689=CIRCLE('',#101143,0.0999999999999994) ;
#33690=CIRCLE('',#101145,0.0999999999999994) ;
#33691=CIRCLE('',#101147,0.0999999999999998) ;
#33692=CIRCLE('',#101149,0.0999999999999994) ;
#33693=CIRCLE('',#101151,0.1) ;
#33694=CIRCLE('',#101153,0.0999999999999994) ;
#33695=CIRCLE('',#101155,0.1) ;
#33696=CIRCLE('',#101157,0.0999999999999994) ;
#33697=CIRCLE('',#101159,0.0999999999999994) ;
#33698=CIRCLE('',#101161,0.0999999999999994) ;
#33699=CIRCLE('',#101162,0.0999999999999996) ;
#33700=CIRCLE('',#101163,0.0999999999999996) ;
#33701=CIRCLE('',#101165,0.0999999999999996) ;
#33702=CIRCLE('',#101167,0.0999999999999994) ;
#33703=CIRCLE('',#101169,0.1) ;
#33704=CIRCLE('',#101171,0.1) ;
#33705=CIRCLE('',#101173,0.1) ;
#33706=CIRCLE('',#101175,0.1) ;
#33707=CIRCLE('',#101177,0.1) ;
#33708=CIRCLE('',#101178,0.100000000000001) ;
#33709=CIRCLE('',#101179,0.1) ;
#33710=CIRCLE('',#101180,0.1) ;
#33711=CIRCLE('',#101182,0.1) ;
#33712=CIRCLE('',#101184,0.1) ;
#33713=CIRCLE('',#101186,0.0999999999999994) ;
#33714=CIRCLE('',#101188,0.0999999999999994) ;
#33715=CIRCLE('',#101190,0.100000000000001) ;
#33716=CIRCLE('',#101192,0.0999999999999996) ;
#33717=CIRCLE('',#101194,0.0999999999999996) ;
#33718=CIRCLE('',#101195,0.0999999999999996) ;
#33719=CIRCLE('',#101197,0.0999999999999994) ;
#33720=CIRCLE('',#101198,0.1) ;
#33721=CIRCLE('',#101200,0.1) ;
#33722=CIRCLE('',#101202,0.0999999999999994) ;
#33723=CIRCLE('',#101204,0.0999999999999994) ;
#33724=CIRCLE('',#101206,0.0999999999999994) ;
#33725=CIRCLE('',#101208,0.0999999999999998) ;
#33726=CIRCLE('',#101210,0.0999999999999994) ;
#33727=CIRCLE('',#101213,0.0999999999999994) ;
#33728=CIRCLE('',#101215,0.1) ;
#33729=CIRCLE('',#101216,0.1) ;
#33730=CIRCLE('',#101218,0.0999999999999994) ;
#33731=CIRCLE('',#101220,0.0999999999999994) ;
#33732=CIRCLE('',#101222,0.0999999999999994) ;
#33733=CIRCLE('',#101224,0.0999999999999994) ;
#33734=CIRCLE('',#101226,0.0999999999999994) ;
#33735=CIRCLE('',#101228,0.0999999999999994) ;
#33736=CIRCLE('',#101230,0.0999999999999994) ;
#33737=CIRCLE('',#101232,0.1) ;
#33738=CIRCLE('',#101234,0.1) ;
#33739=CIRCLE('',#101237,0.0999999999999994) ;
#33740=CIRCLE('',#101238,0.0999999999999994) ;
#33741=CIRCLE('',#101240,0.0999999999999998) ;
#33742=CIRCLE('',#101241,0.0999999999999998) ;
#33743=CIRCLE('',#101243,0.0999999999999998) ;
#33744=CIRCLE('',#101244,0.1) ;
#33745=CIRCLE('',#101246,0.0999999999999998) ;
#33746=CIRCLE('',#101248,0.0999999999999994) ;
#33747=CIRCLE('',#101250,0.0999999999999994) ;
#33748=CIRCLE('',#101251,0.0999999999999994) ;
#33749=CIRCLE('',#101253,0.0999999999999994) ;
#33750=CIRCLE('',#101255,0.1) ;
#33751=CIRCLE('',#101257,0.0999999999999994) ;
#33752=CIRCLE('',#101258,0.0999999999999994) ;
#33753=CIRCLE('',#101260,0.0999999999999998) ;
#33754=CIRCLE('',#101262,0.0999999999999998) ;
#33755=CIRCLE('',#101264,0.0999999999999998) ;
#33756=CIRCLE('',#101266,0.0999999999999998) ;
#33757=CIRCLE('',#101268,0.0999999999999994) ;
#33758=CIRCLE('',#101270,0.0999999999999998) ;
#33759=CIRCLE('',#101272,0.0999999999999998) ;
#33760=CIRCLE('',#101274,0.0999999999999994) ;
#33761=CIRCLE('',#101276,0.0999999999999994) ;
#33762=CIRCLE('',#101278,0.0999999999999994) ;
#33763=CIRCLE('',#101281,0.0999999999999994) ;
#33764=CIRCLE('',#101283,0.0999999999999998) ;
#33765=CIRCLE('',#101284,0.0999999999999998) ;
#33766=CIRCLE('',#101286,0.0999999999999994) ;
#33767=CIRCLE('',#101288,0.0999999999999994) ;
#33768=CIRCLE('',#101290,0.0999999999999994) ;
#33769=CIRCLE('',#101292,0.0999999999999994) ;
#33770=CIRCLE('',#101294,0.0999999999999994) ;
#33771=CIRCLE('',#101296,0.0999999999999994) ;
#33772=CIRCLE('',#101298,0.0999999999999994) ;
#33773=CIRCLE('',#101300,0.0999999999999998) ;
#33774=CIRCLE('',#101302,0.0999999999999998) ;
#33775=CIRCLE('',#101305,0.1) ;
#33776=CIRCLE('',#101306,0.0999999999999994) ;
#33777=CIRCLE('',#101308,0.0999999999999994) ;
#33778=CIRCLE('',#101310,0.0999999999999994) ;
#33779=CIRCLE('',#101312,0.0999999999999994) ;
#33780=CIRCLE('',#101314,0.0999999999999994) ;
#33781=CIRCLE('',#101316,0.0999999999999994) ;
#33782=CIRCLE('',#101318,0.0999999999999994) ;
#33783=CIRCLE('',#101325,0.1) ;
#33784=CIRCLE('',#101326,0.0999999999999998) ;
#33785=CIRCLE('',#101327,0.0999999999999994) ;
#33786=CIRCLE('',#101329,0.0999999999999994) ;
#33787=CIRCLE('',#101331,0.0999999999999994) ;
#33788=CIRCLE('',#101333,0.1) ;
#33789=CIRCLE('',#101335,0.0999999999999994) ;
#33790=CIRCLE('',#101336,0.0999999999999994) ;
#33791=CIRCLE('',#101338,0.0999999999999994) ;
#33792=CIRCLE('',#101340,0.1) ;
#33793=CIRCLE('',#101341,0.0999999999999998) ;
#33794=CIRCLE('',#101343,0.0999999999999994) ;
#33795=CIRCLE('',#101344,0.0999999999999994) ;
#33796=CIRCLE('',#101346,0.0999999999999994) ;
#33797=CIRCLE('',#101347,0.0999999999999994) ;
#33798=CIRCLE('',#101349,0.0999999999999994) ;
#33799=CIRCLE('',#101351,0.0999999999999998) ;
#33800=CIRCLE('',#101353,0.1) ;
#33801=CIRCLE('',#101355,0.0999999999999994) ;
#33802=CIRCLE('',#101357,0.0999999999999994) ;
#33803=CIRCLE('',#101359,0.0999999999999994) ;
#33804=CIRCLE('',#101360,0.0999999999999994) ;
#33805=CIRCLE('',#101362,0.0999999999999994) ;
#33806=CIRCLE('',#101364,0.0999999999999998) ;
#33807=CIRCLE('',#101366,0.0999999999999994) ;
#33808=CIRCLE('',#101368,0.0999999999999994) ;
#33809=CIRCLE('',#101369,0.0999999999999994) ;
#33810=CIRCLE('',#101371,0.0999999999999994) ;
#33811=CIRCLE('',#101373,0.0999999999999998) ;
#33812=CIRCLE('',#101375,0.0999999999999994) ;
#33813=CIRCLE('',#101377,0.0999999999999998) ;
#33814=CIRCLE('',#101379,0.0999999999999998) ;
#33815=CIRCLE('',#101380,0.0999999999999994) ;
#33816=CIRCLE('',#101382,0.0999999999999994) ;
#33817=CIRCLE('',#101384,0.0999999999999994) ;
#33818=CIRCLE('',#101386,0.1) ;
#33819=CIRCLE('',#101388,0.0999999999999998) ;
#33820=CIRCLE('',#101390,0.0999999999999994) ;
#33821=CIRCLE('',#101392,0.0999999999999998) ;
#33822=CIRCLE('',#101394,0.0999999999999994) ;
#33823=CIRCLE('',#101396,0.0999999999999998) ;
#33824=CIRCLE('',#101398,0.1) ;
#33825=CIRCLE('',#101400,0.0999999999999994) ;
#33826=CIRCLE('',#101401,0.0999999999999994) ;
#33827=CIRCLE('',#101403,0.1) ;
#33828=CIRCLE('',#101404,0.0999999999999998) ;
#33829=CIRCLE('',#101406,0.0999999999999994) ;
#33830=CIRCLE('',#101408,0.0999999999999994) ;
#33831=CIRCLE('',#101410,0.0999999999999994) ;
#33832=CIRCLE('',#101412,0.0999999999999994) ;
#33833=CIRCLE('',#101413,0.0999999999999994) ;
#33834=CIRCLE('',#101415,0.1) ;
#33835=CIRCLE('',#101416,0.0999999999999994) ;
#33836=CIRCLE('',#101417,0.0999999999999994) ;
#33837=CIRCLE('',#101419,0.0999999999999994) ;
#33838=CIRCLE('',#101421,0.0999999999999994) ;
#33839=CIRCLE('',#101423,0.0999999999999998) ;
#33840=CIRCLE('',#101425,0.0999999999999994) ;
#33841=CIRCLE('',#101427,0.1) ;
#33842=CIRCLE('',#101429,0.0999999999999994) ;
#33843=CIRCLE('',#101431,0.1) ;
#33844=CIRCLE('',#101433,0.0999999999999994) ;
#33845=CIRCLE('',#101435,0.0999999999999994) ;
#33846=CIRCLE('',#101437,0.0999999999999994) ;
#33847=CIRCLE('',#101438,0.0999999999999996) ;
#33848=CIRCLE('',#101439,0.0999999999999996) ;
#33849=CIRCLE('',#101441,0.1) ;
#33850=CIRCLE('',#101443,0.0999999999999994) ;
#33851=CIRCLE('',#101445,0.0999999999999994) ;
#33852=CIRCLE('',#101447,0.1) ;
#33853=CIRCLE('',#101449,0.1) ;
#33854=CIRCLE('',#101451,0.1) ;
#33855=CIRCLE('',#101453,0.1) ;
#33856=CIRCLE('',#101454,0.1) ;
#33857=CIRCLE('',#101455,0.0999999999999998) ;
#33858=CIRCLE('',#101456,0.1) ;
#33859=CIRCLE('',#101458,0.1) ;
#33860=CIRCLE('',#101460,0.1) ;
#33861=CIRCLE('',#101462,0.0999999999999994) ;
#33862=CIRCLE('',#101464,0.0999999999999994) ;
#33863=CIRCLE('',#101466,0.100000000000001) ;
#33864=CIRCLE('',#101468,0.0999999999999996) ;
#33865=CIRCLE('',#101470,0.0999999999999996) ;
#33866=CIRCLE('',#101471,0.0999999999999996) ;
#33867=CIRCLE('',#101473,0.0999999999999994) ;
#33868=CIRCLE('',#101474,0.1) ;
#33869=CIRCLE('',#101476,0.1) ;
#33870=CIRCLE('',#101478,0.0999999999999994) ;
#33871=CIRCLE('',#101480,0.0999999999999994) ;
#33872=CIRCLE('',#101482,0.0999999999999994) ;
#33873=CIRCLE('',#101484,0.0999999999999998) ;
#33874=CIRCLE('',#101486,0.0999999999999994) ;
#33875=CIRCLE('',#101489,0.0999999999999994) ;
#33876=CIRCLE('',#101491,0.1) ;
#33877=CIRCLE('',#101492,0.1) ;
#33878=CIRCLE('',#101494,0.0999999999999994) ;
#33879=CIRCLE('',#101496,0.0999999999999994) ;
#33880=CIRCLE('',#101498,0.0999999999999994) ;
#33881=CIRCLE('',#101500,0.0999999999999994) ;
#33882=CIRCLE('',#101502,0.0999999999999994) ;
#33883=CIRCLE('',#101504,0.0999999999999994) ;
#33884=CIRCLE('',#101506,0.0999999999999994) ;
#33885=CIRCLE('',#101508,0.1) ;
#33886=CIRCLE('',#101510,0.1) ;
#33887=CIRCLE('',#101513,0.0999999999999994) ;
#33888=CIRCLE('',#101514,0.0999999999999994) ;
#33889=CIRCLE('',#101516,0.0999999999999998) ;
#33890=CIRCLE('',#101517,0.0999999999999998) ;
#33891=CIRCLE('',#101519,0.0999999999999998) ;
#33892=CIRCLE('',#101520,0.1) ;
#33893=CIRCLE('',#101522,0.0999999999999998) ;
#33894=CIRCLE('',#101524,0.0999999999999994) ;
#33895=CIRCLE('',#101526,0.0999999999999994) ;
#33896=CIRCLE('',#101527,0.0999999999999994) ;
#33897=CIRCLE('',#101529,0.0999999999999994) ;
#33898=CIRCLE('',#101531,0.1) ;
#33899=CIRCLE('',#101533,0.0999999999999994) ;
#33900=CIRCLE('',#101534,0.0999999999999994) ;
#33901=CIRCLE('',#101536,0.0999999999999998) ;
#33902=CIRCLE('',#101538,0.0999999999999998) ;
#33903=CIRCLE('',#101540,0.0999999999999998) ;
#33904=CIRCLE('',#101542,0.0999999999999998) ;
#33905=CIRCLE('',#101544,0.0999999999999994) ;
#33906=CIRCLE('',#101546,0.0999999999999998) ;
#33907=CIRCLE('',#101548,0.0999999999999998) ;
#33908=CIRCLE('',#101550,0.0999999999999994) ;
#33909=CIRCLE('',#101552,0.0999999999999994) ;
#33910=CIRCLE('',#101554,0.0999999999999994) ;
#33911=CIRCLE('',#101557,0.0999999999999994) ;
#33912=CIRCLE('',#101559,0.0999999999999998) ;
#33913=CIRCLE('',#101560,0.0999999999999998) ;
#33914=CIRCLE('',#101562,0.0999999999999994) ;
#33915=CIRCLE('',#101564,0.0999999999999994) ;
#33916=CIRCLE('',#101566,0.0999999999999994) ;
#33917=CIRCLE('',#101568,0.0999999999999994) ;
#33918=CIRCLE('',#101570,0.0999999999999994) ;
#33919=CIRCLE('',#101572,0.0999999999999994) ;
#33920=CIRCLE('',#101574,0.0999999999999994) ;
#33921=CIRCLE('',#101576,0.0999999999999998) ;
#33922=CIRCLE('',#101578,0.0999999999999998) ;
#33923=CIRCLE('',#101581,0.1) ;
#33924=CIRCLE('',#101582,0.0999999999999994) ;
#33925=CIRCLE('',#101584,0.0999999999999994) ;
#33926=CIRCLE('',#101586,0.0999999999999994) ;
#33927=CIRCLE('',#101588,0.0999999999999994) ;
#33928=CIRCLE('',#101590,0.0999999999999994) ;
#33929=CIRCLE('',#101592,0.0999999999999994) ;
#33930=CIRCLE('',#101594,0.0999999999999994) ;
#33931=CIRCLE('',#101601,0.1) ;
#33932=CIRCLE('',#101602,0.0999999999999998) ;
#33933=CIRCLE('',#101603,0.0999999999999994) ;
#33934=CIRCLE('',#101605,0.0999999999999994) ;
#33935=CIRCLE('',#101607,0.0999999999999994) ;
#33936=CIRCLE('',#101609,0.1) ;
#33937=CIRCLE('',#101611,0.0999999999999994) ;
#33938=CIRCLE('',#101612,0.0999999999999994) ;
#33939=CIRCLE('',#101614,0.0999999999999994) ;
#33940=CIRCLE('',#101616,0.1) ;
#33941=CIRCLE('',#101617,0.0999999999999998) ;
#33942=CIRCLE('',#101619,0.0999999999999994) ;
#33943=CIRCLE('',#101620,0.0999999999999994) ;
#33944=CIRCLE('',#101622,0.0999999999999994) ;
#33945=CIRCLE('',#101623,0.0999999999999994) ;
#33946=CIRCLE('',#101625,0.0999999999999994) ;
#33947=CIRCLE('',#101627,0.0999999999999998) ;
#33948=CIRCLE('',#101629,0.1) ;
#33949=CIRCLE('',#101631,0.0999999999999994) ;
#33950=CIRCLE('',#101633,0.0999999999999994) ;
#33951=CIRCLE('',#101635,0.0999999999999994) ;
#33952=CIRCLE('',#101636,0.0999999999999994) ;
#33953=CIRCLE('',#101638,0.0999999999999994) ;
#33954=CIRCLE('',#101640,0.0999999999999998) ;
#33955=CIRCLE('',#101642,0.0999999999999994) ;
#33956=CIRCLE('',#101644,0.0999999999999994) ;
#33957=CIRCLE('',#101645,0.0999999999999994) ;
#33958=CIRCLE('',#101647,0.0999999999999994) ;
#33959=CIRCLE('',#101649,0.0999999999999998) ;
#33960=CIRCLE('',#101651,0.0999999999999994) ;
#33961=CIRCLE('',#101653,0.0999999999999998) ;
#33962=CIRCLE('',#101655,0.0999999999999998) ;
#33963=CIRCLE('',#101656,0.0999999999999994) ;
#33964=CIRCLE('',#101658,0.0999999999999994) ;
#33965=CIRCLE('',#101660,0.0999999999999994) ;
#33966=CIRCLE('',#101662,0.1) ;
#33967=CIRCLE('',#101664,0.0999999999999998) ;
#33968=CIRCLE('',#101666,0.0999999999999994) ;
#33969=CIRCLE('',#101668,0.0999999999999998) ;
#33970=CIRCLE('',#101670,0.0999999999999994) ;
#33971=CIRCLE('',#101672,0.0999999999999998) ;
#33972=CIRCLE('',#101674,0.1) ;
#33973=CIRCLE('',#101676,0.0999999999999994) ;
#33974=CIRCLE('',#101677,0.0999999999999994) ;
#33975=CIRCLE('',#101679,0.1) ;
#33976=CIRCLE('',#101680,0.0999999999999998) ;
#33977=CIRCLE('',#101682,0.0999999999999994) ;
#33978=CIRCLE('',#101684,0.0999999999999994) ;
#33979=CIRCLE('',#101686,0.0999999999999994) ;
#33980=CIRCLE('',#101688,0.0999999999999994) ;
#33981=CIRCLE('',#101689,0.0999999999999994) ;
#33982=CIRCLE('',#101691,0.1) ;
#33983=CIRCLE('',#101692,0.0999999999999994) ;
#33984=CIRCLE('',#101693,0.0999999999999994) ;
#33985=CIRCLE('',#101695,0.0999999999999994) ;
#33986=CIRCLE('',#101697,0.0999999999999994) ;
#33987=CIRCLE('',#101699,0.0999999999999998) ;
#33988=CIRCLE('',#101701,0.0999999999999994) ;
#33989=CIRCLE('',#101703,0.1) ;
#33990=CIRCLE('',#101705,0.0999999999999994) ;
#33991=CIRCLE('',#101707,0.1) ;
#33992=CIRCLE('',#101709,0.0999999999999994) ;
#33993=CIRCLE('',#101711,0.0999999999999994) ;
#33994=CIRCLE('',#101713,0.0999999999999994) ;
#33995=CIRCLE('',#101714,0.0999999999999996) ;
#33996=CIRCLE('',#101715,0.0999999999999996) ;
#33997=CIRCLE('',#101717,0.1) ;
#33998=CIRCLE('',#101719,0.0999999999999994) ;
#33999=CIRCLE('',#101721,0.0999999999999994) ;
#34000=CIRCLE('',#101723,0.1) ;
#34001=CIRCLE('',#101725,0.1) ;
#34002=CIRCLE('',#101727,0.1) ;
#34003=CIRCLE('',#101729,0.1) ;
#34004=CIRCLE('',#101730,0.1) ;
#34005=CIRCLE('',#101731,0.0999999999999998) ;
#34006=CIRCLE('',#101732,0.1) ;
#34007=CIRCLE('',#101734,0.1) ;
#34008=CIRCLE('',#101736,0.1) ;
#34009=CIRCLE('',#101738,0.0999999999999994) ;
#34010=CIRCLE('',#101740,0.0999999999999994) ;
#34011=CIRCLE('',#101742,0.100000000000001) ;
#34012=CIRCLE('',#101744,0.0999999999999996) ;
#34013=CIRCLE('',#101746,0.0999999999999996) ;
#34014=CIRCLE('',#101747,0.0999999999999996) ;
#34015=CIRCLE('',#101749,0.0999999999999994) ;
#34016=CIRCLE('',#101750,0.1) ;
#34017=CIRCLE('',#101752,0.0999999999999998) ;
#34018=CIRCLE('',#101754,0.0999999999999994) ;
#34019=CIRCLE('',#101756,0.0999999999999994) ;
#34020=CIRCLE('',#101758,0.0999999999999994) ;
#34021=CIRCLE('',#101760,0.0999999999999998) ;
#34022=CIRCLE('',#101762,0.0999999999999994) ;
#34023=CIRCLE('',#101765,0.0999999999999994) ;
#34024=CIRCLE('',#101767,0.1) ;
#34025=CIRCLE('',#101768,0.1) ;
#34026=CIRCLE('',#101770,0.0999999999999994) ;
#34027=CIRCLE('',#101772,0.0999999999999994) ;
#34028=CIRCLE('',#101774,0.0999999999999994) ;
#34029=CIRCLE('',#101776,0.0999999999999994) ;
#34030=CIRCLE('',#101778,0.0999999999999994) ;
#34031=CIRCLE('',#101780,0.0999999999999994) ;
#34032=CIRCLE('',#101782,0.0999999999999994) ;
#34033=CIRCLE('',#101784,0.1) ;
#34034=CIRCLE('',#101786,0.1) ;
#34035=CIRCLE('',#101789,0.0999999999999994) ;
#34036=CIRCLE('',#101790,0.0999999999999994) ;
#34037=CIRCLE('',#101792,0.0999999999999998) ;
#34038=CIRCLE('',#101793,0.0999999999999998) ;
#34039=CIRCLE('',#101795,0.0999999999999998) ;
#34040=CIRCLE('',#101796,0.1) ;
#34041=CIRCLE('',#101798,0.0999999999999998) ;
#34042=CIRCLE('',#101800,0.0999999999999994) ;
#34043=CIRCLE('',#101802,0.0999999999999994) ;
#34044=CIRCLE('',#101803,0.0999999999999994) ;
#34045=CIRCLE('',#101805,0.0999999999999994) ;
#34046=CIRCLE('',#101807,0.1) ;
#34047=CIRCLE('',#101809,0.0999999999999994) ;
#34048=CIRCLE('',#101810,0.0999999999999994) ;
#34049=CIRCLE('',#101812,0.0999999999999998) ;
#34050=CIRCLE('',#101814,0.0999999999999998) ;
#34051=CIRCLE('',#101816,0.0999999999999998) ;
#34052=CIRCLE('',#101818,0.0999999999999998) ;
#34053=CIRCLE('',#101820,0.0999999999999994) ;
#34054=CIRCLE('',#101822,0.0999999999999998) ;
#34055=CIRCLE('',#101824,0.0999999999999998) ;
#34056=CIRCLE('',#101826,0.0999999999999994) ;
#34057=CIRCLE('',#101828,0.0999999999999994) ;
#34058=CIRCLE('',#101830,0.0999999999999994) ;
#34059=CIRCLE('',#101833,0.0999999999999994) ;
#34060=CIRCLE('',#101835,0.0999999999999998) ;
#34061=CIRCLE('',#101836,0.0999999999999998) ;
#34062=CIRCLE('',#101838,0.0999999999999994) ;
#34063=CIRCLE('',#101840,0.0999999999999994) ;
#34064=CIRCLE('',#101842,0.0999999999999994) ;
#34065=CIRCLE('',#101844,0.0999999999999994) ;
#34066=CIRCLE('',#101846,0.0999999999999994) ;
#34067=CIRCLE('',#101848,0.0999999999999994) ;
#34068=CIRCLE('',#101850,0.0999999999999994) ;
#34069=CIRCLE('',#101852,0.0999999999999998) ;
#34070=CIRCLE('',#101854,0.0999999999999998) ;
#34071=CIRCLE('',#101857,0.1) ;
#34072=CIRCLE('',#101858,0.0999999999999994) ;
#34073=CIRCLE('',#101860,0.0999999999999994) ;
#34074=CIRCLE('',#101862,0.0999999999999994) ;
#34075=CIRCLE('',#101864,0.0999999999999994) ;
#34076=CIRCLE('',#101866,0.0999999999999994) ;
#34077=CIRCLE('',#101868,0.0999999999999994) ;
#34078=CIRCLE('',#101870,0.0999999999999994) ;
#34079=CIRCLE('',#101877,0.1) ;
#34080=CIRCLE('',#101878,0.0999999999999998) ;
#34081=CIRCLE('',#101879,0.0999999999999994) ;
#34082=CIRCLE('',#101881,0.0999999999999994) ;
#34083=CIRCLE('',#101883,0.0999999999999994) ;
#34084=CIRCLE('',#101885,0.1) ;
#34085=CIRCLE('',#101887,0.0999999999999994) ;
#34086=CIRCLE('',#101888,0.0999999999999994) ;
#34087=CIRCLE('',#101890,0.0999999999999994) ;
#34088=CIRCLE('',#101892,0.1) ;
#34089=CIRCLE('',#101893,0.0999999999999998) ;
#34090=CIRCLE('',#101895,0.0999999999999994) ;
#34091=CIRCLE('',#101896,0.0999999999999994) ;
#34092=CIRCLE('',#101898,0.0999999999999994) ;
#34093=CIRCLE('',#101899,0.0999999999999994) ;
#34094=CIRCLE('',#101901,0.0999999999999994) ;
#34095=CIRCLE('',#101903,0.0999999999999998) ;
#34096=CIRCLE('',#101905,0.1) ;
#34097=CIRCLE('',#101907,0.0999999999999994) ;
#34098=CIRCLE('',#101909,0.0999999999999994) ;
#34099=CIRCLE('',#101911,0.0999999999999994) ;
#34100=CIRCLE('',#101912,0.0999999999999994) ;
#34101=CIRCLE('',#101914,0.0999999999999994) ;
#34102=CIRCLE('',#101916,0.0999999999999998) ;
#34103=CIRCLE('',#101918,0.0999999999999994) ;
#34104=CIRCLE('',#101920,0.0999999999999994) ;
#34105=CIRCLE('',#101921,0.0999999999999994) ;
#34106=CIRCLE('',#101923,0.0999999999999994) ;
#34107=CIRCLE('',#101925,0.0999999999999998) ;
#34108=CIRCLE('',#101927,0.0999999999999994) ;
#34109=CIRCLE('',#101929,0.0999999999999998) ;
#34110=CIRCLE('',#101931,0.0999999999999998) ;
#34111=CIRCLE('',#101932,0.0999999999999994) ;
#34112=CIRCLE('',#101934,0.0999999999999994) ;
#34113=CIRCLE('',#101936,0.0999999999999994) ;
#34114=CIRCLE('',#101938,0.1) ;
#34115=CIRCLE('',#101940,0.0999999999999998) ;
#34116=CIRCLE('',#101942,0.0999999999999994) ;
#34117=CIRCLE('',#101944,0.0999999999999998) ;
#34118=CIRCLE('',#101946,0.0999999999999994) ;
#34119=CIRCLE('',#101948,0.0999999999999998) ;
#34120=CIRCLE('',#101950,0.1) ;
#34121=CIRCLE('',#101952,0.0999999999999994) ;
#34122=CIRCLE('',#101953,0.0999999999999994) ;
#34123=CIRCLE('',#101955,0.1) ;
#34124=CIRCLE('',#101956,0.0999999999999998) ;
#34125=CIRCLE('',#101958,0.0999999999999994) ;
#34126=CIRCLE('',#101960,0.0999999999999994) ;
#34127=CIRCLE('',#101962,0.0999999999999994) ;
#34128=CIRCLE('',#101964,0.0999999999999994) ;
#34129=CIRCLE('',#101965,0.0999999999999994) ;
#34130=CIRCLE('',#101967,0.1) ;
#34131=CIRCLE('',#101968,0.0999999999999994) ;
#34132=CIRCLE('',#101969,0.0999999999999994) ;
#34133=CIRCLE('',#101971,0.0999999999999994) ;
#34134=CIRCLE('',#101973,0.0999999999999994) ;
#34135=CIRCLE('',#101975,0.0999999999999998) ;
#34136=CIRCLE('',#101977,0.0999999999999994) ;
#34137=CIRCLE('',#101979,0.1) ;
#34138=CIRCLE('',#101981,0.0999999999999994) ;
#34139=CIRCLE('',#101983,0.1) ;
#34140=CIRCLE('',#101985,0.0999999999999994) ;
#34141=CIRCLE('',#101987,0.0999999999999994) ;
#34142=CIRCLE('',#101989,0.0999999999999994) ;
#34143=CIRCLE('',#101990,0.0999999999999996) ;
#34144=CIRCLE('',#101991,0.0999999999999996) ;
#34145=CIRCLE('',#101993,0.1) ;
#34146=CIRCLE('',#101995,0.0999999999999994) ;
#34147=CIRCLE('',#101997,0.0999999999999994) ;
#34148=CIRCLE('',#101999,0.1) ;
#34149=CIRCLE('',#102001,0.1) ;
#34150=CIRCLE('',#102003,0.1) ;
#34151=CIRCLE('',#102005,0.1) ;
#34152=CIRCLE('',#102006,0.1) ;
#34153=CIRCLE('',#102007,0.0999999999999998) ;
#34154=CIRCLE('',#102008,0.1) ;
#34155=CIRCLE('',#102010,0.1) ;
#34156=CIRCLE('',#102012,0.1) ;
#34157=CIRCLE('',#102014,0.0999999999999994) ;
#34158=CIRCLE('',#102016,0.0999999999999994) ;
#34159=CIRCLE('',#102018,0.100000000000001) ;
#34160=CIRCLE('',#102020,0.0999999999999996) ;
#34161=CIRCLE('',#102022,0.0999999999999996) ;
#34162=CIRCLE('',#102023,0.0999999999999996) ;
#34163=CIRCLE('',#102025,0.0999999999999994) ;
#34164=CIRCLE('',#102026,0.1) ;
#34165=CIRCLE('',#102028,0.0999999999999998) ;
#34166=CIRCLE('',#102030,0.0999999999999994) ;
#34167=CIRCLE('',#102032,0.0999999999999994) ;
#34168=CIRCLE('',#102034,0.0999999999999994) ;
#34169=CIRCLE('',#102036,0.0999999999999998) ;
#34170=CIRCLE('',#102038,0.0999999999999994) ;
#34171=CIRCLE('',#102041,0.0999999999999994) ;
#34172=CIRCLE('',#102043,0.1) ;
#34173=CIRCLE('',#102044,0.1) ;
#34174=CIRCLE('',#102046,0.0999999999999994) ;
#34175=CIRCLE('',#102048,0.0999999999999994) ;
#34176=CIRCLE('',#102050,0.0999999999999994) ;
#34177=CIRCLE('',#102052,0.0999999999999994) ;
#34178=CIRCLE('',#102054,0.0999999999999994) ;
#34179=CIRCLE('',#102056,0.0999999999999994) ;
#34180=CIRCLE('',#102058,0.0999999999999994) ;
#34181=CIRCLE('',#102060,0.1) ;
#34182=CIRCLE('',#102062,0.1) ;
#34183=CIRCLE('',#102065,0.0999999999999994) ;
#34184=CIRCLE('',#102066,0.0999999999999994) ;
#34185=CIRCLE('',#102068,0.0999999999999998) ;
#34186=CIRCLE('',#102069,0.0999999999999998) ;
#34187=CIRCLE('',#102071,0.0999999999999998) ;
#34188=CIRCLE('',#102072,0.1) ;
#34189=CIRCLE('',#102074,0.0999999999999998) ;
#34190=CIRCLE('',#102076,0.0999999999999994) ;
#34191=CIRCLE('',#102078,0.0999999999999994) ;
#34192=CIRCLE('',#102079,0.0999999999999994) ;
#34193=CIRCLE('',#102081,0.0999999999999994) ;
#34194=CIRCLE('',#102083,0.1) ;
#34195=CIRCLE('',#102085,0.0999999999999994) ;
#34196=CIRCLE('',#102086,0.0999999999999994) ;
#34197=CIRCLE('',#102088,0.0999999999999998) ;
#34198=CIRCLE('',#102090,0.0999999999999998) ;
#34199=CIRCLE('',#102092,0.0999999999999998) ;
#34200=CIRCLE('',#102094,0.0999999999999998) ;
#34201=CIRCLE('',#102096,0.0999999999999994) ;
#34202=CIRCLE('',#102098,0.0999999999999998) ;
#34203=CIRCLE('',#102100,0.0999999999999998) ;
#34204=CIRCLE('',#102102,0.0999999999999994) ;
#34205=CIRCLE('',#102104,0.0999999999999994) ;
#34206=CIRCLE('',#102106,0.0999999999999994) ;
#34207=CIRCLE('',#102109,0.0999999999999994) ;
#34208=CIRCLE('',#102111,0.0999999999999998) ;
#34209=CIRCLE('',#102112,0.0999999999999998) ;
#34210=CIRCLE('',#102114,0.0999999999999994) ;
#34211=CIRCLE('',#102116,0.0999999999999994) ;
#34212=CIRCLE('',#102118,0.0999999999999994) ;
#34213=CIRCLE('',#102120,0.0999999999999994) ;
#34214=CIRCLE('',#102122,0.0999999999999994) ;
#34215=CIRCLE('',#102124,0.0999999999999994) ;
#34216=CIRCLE('',#102126,0.0999999999999994) ;
#34217=CIRCLE('',#102128,0.0999999999999998) ;
#34218=CIRCLE('',#102130,0.0999999999999998) ;
#34219=CIRCLE('',#102133,0.1) ;
#34220=CIRCLE('',#102134,0.0999999999999994) ;
#34221=CIRCLE('',#102136,0.0999999999999994) ;
#34222=CIRCLE('',#102138,0.0999999999999994) ;
#34223=CIRCLE('',#102140,0.0999999999999994) ;
#34224=CIRCLE('',#102142,0.0999999999999994) ;
#34225=CIRCLE('',#102144,0.0999999999999994) ;
#34226=CIRCLE('',#102146,0.0999999999999994) ;
#34227=CIRCLE('',#102153,0.1) ;
#34228=CIRCLE('',#102154,0.0999999999999998) ;
#34229=CIRCLE('',#102155,0.0999999999999994) ;
#34230=CIRCLE('',#102157,0.0999999999999994) ;
#34231=CIRCLE('',#102159,0.0999999999999994) ;
#34232=CIRCLE('',#102161,0.1) ;
#34233=CIRCLE('',#102163,0.0999999999999994) ;
#34234=CIRCLE('',#102164,0.0999999999999994) ;
#34235=CIRCLE('',#102166,0.0999999999999994) ;
#34236=CIRCLE('',#102168,0.1) ;
#34237=CIRCLE('',#102169,0.0999999999999998) ;
#34238=CIRCLE('',#102171,0.0999999999999994) ;
#34239=CIRCLE('',#102172,0.100000000000003) ;
#34240=CIRCLE('',#102174,0.0999999999999994) ;
#34241=CIRCLE('',#102175,0.0999999999999994) ;
#34242=CIRCLE('',#102177,0.0999999999999994) ;
#34243=CIRCLE('',#102179,0.0999999999999998) ;
#34244=CIRCLE('',#102181,0.1) ;
#34245=CIRCLE('',#102183,0.100000000000003) ;
#34246=CIRCLE('',#102185,0.0999999999999994) ;
#34247=CIRCLE('',#102187,0.100000000000003) ;
#34248=CIRCLE('',#102188,0.100000000000003) ;
#34249=CIRCLE('',#102190,0.0999999999999994) ;
#34250=CIRCLE('',#102192,0.0999999999999998) ;
#34251=CIRCLE('',#102194,0.100000000000003) ;
#34252=CIRCLE('',#102196,0.0999999999999994) ;
#34253=CIRCLE('',#102197,0.0999999999999994) ;
#34254=CIRCLE('',#102199,0.0999999999999994) ;
#34255=CIRCLE('',#102201,0.0999999999999998) ;
#34256=CIRCLE('',#102203,0.100000000000003) ;
#34257=CIRCLE('',#102205,0.0999999999999994) ;
#34258=CIRCLE('',#102207,0.0999999999999998) ;
#34259=CIRCLE('',#102208,0.0999999999999994) ;
#34260=CIRCLE('',#102210,0.100000000000003) ;
#34261=CIRCLE('',#102212,0.0999999999999994) ;
#34262=CIRCLE('',#102214,0.1) ;
#34263=CIRCLE('',#102216,0.0999999999999998) ;
#34264=CIRCLE('',#102218,0.100000000000003) ;
#34265=CIRCLE('',#102220,0.0999999999999998) ;
#34266=CIRCLE('',#102222,0.100000000000003) ;
#34267=CIRCLE('',#102224,0.0999999999999998) ;
#34268=CIRCLE('',#102226,0.1) ;
#34269=CIRCLE('',#102228,0.100000000000003) ;
#34270=CIRCLE('',#102229,0.100000000000003) ;
#34271=CIRCLE('',#102231,0.1) ;
#34272=CIRCLE('',#102232,0.0999999999999998) ;
#34273=CIRCLE('',#102234,0.100000000000003) ;
#34274=CIRCLE('',#102236,0.100000000000003) ;
#34275=CIRCLE('',#102238,0.0999999999999994) ;
#34276=CIRCLE('',#102240,0.0999999999999994) ;
#34277=CIRCLE('',#102241,0.0999999999999994) ;
#34278=CIRCLE('',#102243,0.1) ;
#34279=CIRCLE('',#102244,0.0999999999999994) ;
#34280=CIRCLE('',#102245,0.100000000000003) ;
#34281=CIRCLE('',#102247,0.0999999999999994) ;
#34282=CIRCLE('',#102249,0.0999999999999994) ;
#34283=CIRCLE('',#102251,0.0999999999999998) ;
#34284=CIRCLE('',#102253,0.100000000000003) ;
#34285=CIRCLE('',#102255,0.1) ;
#34286=CIRCLE('',#102257,0.100000000000003) ;
#34287=CIRCLE('',#102259,0.1) ;
#34288=CIRCLE('',#102261,0.100000000000003) ;
#34289=CIRCLE('',#102263,0.100000000000003) ;
#34290=CIRCLE('',#102265,0.100000000000003) ;
#34291=CIRCLE('',#102266,0.0999999999999996) ;
#34292=CIRCLE('',#102267,0.0999999999999996) ;
#34293=CIRCLE('',#102269,0.1) ;
#34294=CIRCLE('',#102271,0.0999999999999994) ;
#34295=CIRCLE('',#102273,0.0999999999999994) ;
#34296=CIRCLE('',#102275,0.1) ;
#34297=CIRCLE('',#102277,0.1) ;
#34298=CIRCLE('',#102279,0.1) ;
#34299=CIRCLE('',#102281,0.1) ;
#34300=CIRCLE('',#102282,0.1) ;
#34301=CIRCLE('',#102283,0.100000000000002) ;
#34302=CIRCLE('',#102284,0.1) ;
#34303=CIRCLE('',#102286,0.1) ;
#34304=CIRCLE('',#102288,0.1) ;
#34305=CIRCLE('',#102290,0.1) ;
#34306=CIRCLE('',#102292,0.100000000000003) ;
#34307=CIRCLE('',#102294,0.0999999999999983) ;
#34308=CIRCLE('',#102296,0.0999999999999996) ;
#34309=CIRCLE('',#102298,0.1) ;
#34310=CIRCLE('',#102299,0.0999999999999969) ;
#34311=CIRCLE('',#102301,0.0999999999999994) ;
#34312=CIRCLE('',#102302,0.1) ;
#34313=CIRCLE('',#102304,0.0999999999999998) ;
#34314=CIRCLE('',#102306,0.0999999999999994) ;
#34315=CIRCLE('',#102308,0.0999999999999994) ;
#34316=CIRCLE('',#102310,0.0999999999999994) ;
#34317=CIRCLE('',#102312,0.0999999999999998) ;
#34318=CIRCLE('',#102314,0.0999999999999994) ;
#34319=CIRCLE('',#102317,0.0999999999999994) ;
#34320=CIRCLE('',#102319,0.1) ;
#34321=CIRCLE('',#102320,0.1) ;
#34322=CIRCLE('',#102322,0.0999999999999994) ;
#34323=CIRCLE('',#102324,0.0999999999999994) ;
#34324=CIRCLE('',#102326,0.0999999999999994) ;
#34325=CIRCLE('',#102328,0.0999999999999994) ;
#34326=CIRCLE('',#102330,0.0999999999999994) ;
#34327=CIRCLE('',#102332,0.0999999999999994) ;
#34328=CIRCLE('',#102334,0.0999999999999994) ;
#34329=CIRCLE('',#102336,0.1) ;
#34330=CIRCLE('',#102338,0.1) ;
#34331=CIRCLE('',#102341,0.100000000000003) ;
#34332=CIRCLE('',#102342,0.100000000000003) ;
#34333=CIRCLE('',#102344,0.0999999999999998) ;
#34334=CIRCLE('',#102345,0.0999999999999998) ;
#34335=CIRCLE('',#102347,0.0999999999999998) ;
#34336=CIRCLE('',#102348,0.1) ;
#34337=CIRCLE('',#102350,0.0999999999999998) ;
#34338=CIRCLE('',#102352,0.100000000000003) ;
#34339=CIRCLE('',#102354,0.100000000000003) ;
#34340=CIRCLE('',#102355,0.100000000000003) ;
#34341=CIRCLE('',#102357,0.100000000000003) ;
#34342=CIRCLE('',#102359,0.1) ;
#34343=CIRCLE('',#102361,0.0999999999999994) ;
#34344=CIRCLE('',#102362,0.0999999999999994) ;
#34345=CIRCLE('',#102364,0.0999999999999998) ;
#34346=CIRCLE('',#102366,0.0999999999999998) ;
#34347=CIRCLE('',#102368,0.0999999999999998) ;
#34348=CIRCLE('',#102370,0.0999999999999998) ;
#34349=CIRCLE('',#102372,0.0999999999999994) ;
#34350=CIRCLE('',#102374,0.0999999999999998) ;
#34351=CIRCLE('',#102376,0.0999999999999998) ;
#34352=CIRCLE('',#102378,0.0999999999999994) ;
#34353=CIRCLE('',#102380,0.0999999999999994) ;
#34354=CIRCLE('',#102382,0.0999999999999994) ;
#34355=CIRCLE('',#102385,0.0999999999999994) ;
#34356=CIRCLE('',#102387,0.0999999999999998) ;
#34357=CIRCLE('',#102388,0.0999999999999998) ;
#34358=CIRCLE('',#102390,0.0999999999999994) ;
#34359=CIRCLE('',#102392,0.0999999999999994) ;
#34360=CIRCLE('',#102394,0.0999999999999994) ;
#34361=CIRCLE('',#102396,0.0999999999999994) ;
#34362=CIRCLE('',#102398,0.0999999999999994) ;
#34363=CIRCLE('',#102400,0.0999999999999994) ;
#34364=CIRCLE('',#102402,0.0999999999999994) ;
#34365=CIRCLE('',#102404,0.0999999999999998) ;
#34366=CIRCLE('',#102406,0.0999999999999998) ;
#34367=CIRCLE('',#102409,0.1) ;
#34368=CIRCLE('',#102410,0.0999999999999994) ;
#34369=CIRCLE('',#102412,0.0999999999999994) ;
#34370=CIRCLE('',#102414,0.0999999999999994) ;
#34371=CIRCLE('',#102416,0.0999999999999994) ;
#34372=CIRCLE('',#102418,0.0999999999999994) ;
#34373=CIRCLE('',#102420,0.0999999999999994) ;
#34374=CIRCLE('',#102422,0.0999999999999994) ;
#34375=CIRCLE('',#102429,0.1) ;
#34376=CIRCLE('',#102430,0.0999999999999998) ;
#34377=CIRCLE('',#102431,0.100000000000003) ;
#34378=CIRCLE('',#102433,0.0999999999999994) ;
#34379=CIRCLE('',#102435,0.100000000000003) ;
#34380=CIRCLE('',#102437,0.1) ;
#34381=CIRCLE('',#102439,0.100000000000003) ;
#34382=CIRCLE('',#102440,0.100000000000003) ;
#34383=CIRCLE('',#102442,0.100000000000003) ;
#34384=CIRCLE('',#102444,0.1) ;
#34385=CIRCLE('',#102445,0.0999999999999998) ;
#34386=CIRCLE('',#102447,0.0999999999999994) ;
#34387=CIRCLE('',#102448,0.100000000000003) ;
#34388=CIRCLE('',#102450,0.0999999999999994) ;
#34389=CIRCLE('',#102451,0.0999999999999994) ;
#34390=CIRCLE('',#102453,0.100000000000003) ;
#34391=CIRCLE('',#102455,0.0999999999999998) ;
#34392=CIRCLE('',#102457,0.1) ;
#34393=CIRCLE('',#102459,0.100000000000003) ;
#34394=CIRCLE('',#102461,0.0999999999999994) ;
#34395=CIRCLE('',#102463,0.100000000000003) ;
#34396=CIRCLE('',#102464,0.100000000000003) ;
#34397=CIRCLE('',#102466,0.100000000000003) ;
#34398=CIRCLE('',#102468,0.0999999999999998) ;
#34399=CIRCLE('',#102470,0.100000000000003) ;
#34400=CIRCLE('',#102472,0.100000000000003) ;
#34401=CIRCLE('',#102473,0.100000000000003) ;
#34402=CIRCLE('',#102475,0.100000000000003) ;
#34403=CIRCLE('',#102477,0.0999999999999998) ;
#34404=CIRCLE('',#102479,0.100000000000003) ;
#34405=CIRCLE('',#102481,0.0999999999999998) ;
#34406=CIRCLE('',#102483,0.0999999999999998) ;
#34407=CIRCLE('',#102484,0.100000000000003) ;
#34408=CIRCLE('',#102486,0.100000000000003) ;
#34409=CIRCLE('',#102488,0.100000000000003) ;
#34410=CIRCLE('',#102490,0.1) ;
#34411=CIRCLE('',#102492,0.0999999999999998) ;
#34412=CIRCLE('',#102494,0.100000000000003) ;
#34413=CIRCLE('',#102496,0.0999999999999998) ;
#34414=CIRCLE('',#102498,0.100000000000003) ;
#34415=CIRCLE('',#102500,0.0999999999999998) ;
#34416=CIRCLE('',#102502,0.1) ;
#34417=CIRCLE('',#102504,0.100000000000003) ;
#34418=CIRCLE('',#102505,0.100000000000003) ;
#34419=CIRCLE('',#102507,0.0999999999999998) ;
#34420=CIRCLE('',#102508,0.0999999999999998) ;
#34421=CIRCLE('',#102510,0.100000000000003) ;
#34422=CIRCLE('',#102512,0.100000000000003) ;
#34423=CIRCLE('',#102514,0.100000000000003) ;
#34424=CIRCLE('',#102516,0.100000000000003) ;
#34425=CIRCLE('',#102517,0.100000000000003) ;
#34426=CIRCLE('',#102519,0.1) ;
#34427=CIRCLE('',#102520,0.100000000000003) ;
#34428=CIRCLE('',#102521,0.100000000000003) ;
#34429=CIRCLE('',#102523,0.100000000000003) ;
#34430=CIRCLE('',#102525,0.100000000000003) ;
#34431=CIRCLE('',#102527,0.0999999999999998) ;
#34432=CIRCLE('',#102529,0.100000000000003) ;
#34433=CIRCLE('',#102531,0.1) ;
#34434=CIRCLE('',#102533,0.100000000000003) ;
#34435=CIRCLE('',#102535,0.1) ;
#34436=CIRCLE('',#102537,0.100000000000003) ;
#34437=CIRCLE('',#102539,0.100000000000003) ;
#34438=CIRCLE('',#102541,0.100000000000003) ;
#34439=CIRCLE('',#102542,0.100000000000003) ;
#34440=CIRCLE('',#102543,0.0999999999999996) ;
#34441=CIRCLE('',#102545,0.1) ;
#34442=CIRCLE('',#102547,0.0999999999999994) ;
#34443=CIRCLE('',#102549,0.1) ;
#34444=CIRCLE('',#102551,0.100000000000003) ;
#34445=CIRCLE('',#102553,0.1) ;
#34446=CIRCLE('',#102555,0.1) ;
#34447=CIRCLE('',#102557,0.1) ;
#34448=CIRCLE('',#102558,0.0999999999999995) ;
#34449=CIRCLE('',#102559,0.100000000000002) ;
#34450=CIRCLE('',#102560,0.1) ;
#34451=CIRCLE('',#102562,0.1) ;
#34452=CIRCLE('',#102564,0.1) ;
#34453=CIRCLE('',#102566,0.1) ;
#34454=CIRCLE('',#102568,0.100000000000003) ;
#34455=CIRCLE('',#102570,0.0999999999999983) ;
#34456=CIRCLE('',#102572,0.0999999999999996) ;
#34457=CIRCLE('',#102574,0.1) ;
#34458=CIRCLE('',#102575,0.0999999999999969) ;
#34459=CIRCLE('',#102577,0.100000000000003) ;
#34460=CIRCLE('',#102578,0.1) ;
#34461=CIRCLE('',#102580,0.1) ;
#34462=CIRCLE('',#102582,0.100000000000003) ;
#34463=CIRCLE('',#102584,0.100000000000003) ;
#34464=CIRCLE('',#102586,0.0999999999999994) ;
#34465=CIRCLE('',#102588,0.0999999999999998) ;
#34466=CIRCLE('',#102590,0.0999999999999994) ;
#34467=CIRCLE('',#102593,0.100000000000003) ;
#34468=CIRCLE('',#102595,0.1) ;
#34469=CIRCLE('',#102596,0.1) ;
#34470=CIRCLE('',#102598,0.100000000000003) ;
#34471=CIRCLE('',#102600,0.100000000000003) ;
#34472=CIRCLE('',#102602,0.100000000000003) ;
#34473=CIRCLE('',#102604,0.100000000000003) ;
#34474=CIRCLE('',#102606,0.100000000000003) ;
#34475=CIRCLE('',#102608,0.100000000000003) ;
#34476=CIRCLE('',#102610,0.100000000000003) ;
#34477=CIRCLE('',#102612,0.1) ;
#34478=CIRCLE('',#102614,0.1) ;
#34479=CIRCLE('',#102617,0.100000000000003) ;
#34480=CIRCLE('',#102618,0.100000000000003) ;
#34481=CIRCLE('',#102620,0.0999999999999998) ;
#34482=CIRCLE('',#102621,0.0999999999999998) ;
#34483=CIRCLE('',#102623,0.0999999999999998) ;
#34484=CIRCLE('',#102624,0.1) ;
#34485=CIRCLE('',#102626,0.0999999999999998) ;
#34486=CIRCLE('',#102628,0.100000000000003) ;
#34487=CIRCLE('',#102630,0.100000000000003) ;
#34488=CIRCLE('',#102631,0.100000000000003) ;
#34489=CIRCLE('',#102633,0.100000000000003) ;
#34490=CIRCLE('',#102635,0.1) ;
#34491=CIRCLE('',#102637,0.100000000000003) ;
#34492=CIRCLE('',#102638,0.100000000000003) ;
#34493=CIRCLE('',#102640,0.0999999999999998) ;
#34494=CIRCLE('',#102642,0.0999999999999998) ;
#34495=CIRCLE('',#102644,0.0999999999999998) ;
#34496=CIRCLE('',#102646,0.0999999999999998) ;
#34497=CIRCLE('',#102648,0.100000000000003) ;
#34498=CIRCLE('',#102650,0.0999999999999998) ;
#34499=CIRCLE('',#102652,0.0999999999999998) ;
#34500=CIRCLE('',#102654,0.100000000000003) ;
#34501=CIRCLE('',#102656,0.100000000000003) ;
#34502=CIRCLE('',#102658,0.100000000000003) ;
#34503=CIRCLE('',#102661,0.100000000000003) ;
#34504=CIRCLE('',#102663,0.0999999999999998) ;
#34505=CIRCLE('',#102664,0.0999999999999998) ;
#34506=CIRCLE('',#102666,0.100000000000003) ;
#34507=CIRCLE('',#102668,0.100000000000003) ;
#34508=CIRCLE('',#102670,0.100000000000003) ;
#34509=CIRCLE('',#102672,0.100000000000003) ;
#34510=CIRCLE('',#102674,0.100000000000003) ;
#34511=CIRCLE('',#102676,0.100000000000003) ;
#34512=CIRCLE('',#102678,0.100000000000003) ;
#34513=CIRCLE('',#102680,0.0999999999999998) ;
#34514=CIRCLE('',#102682,0.0999999999999998) ;
#34515=CIRCLE('',#102685,0.1) ;
#34516=CIRCLE('',#102686,0.0999999999999994) ;
#34517=CIRCLE('',#102688,0.100000000000003) ;
#34518=CIRCLE('',#102690,0.100000000000003) ;
#34519=CIRCLE('',#102692,0.100000000000003) ;
#34520=CIRCLE('',#102694,0.100000000000003) ;
#34521=CIRCLE('',#102696,0.0999999999999994) ;
#34522=CIRCLE('',#102698,0.0999999999999994) ;
#34523=CIRCLE('',#102705,0.0999999999999998) ;
#34524=CIRCLE('',#102706,0.0999999999999998) ;
#34525=CIRCLE('',#102708,0.0999999999999998) ;
#34526=CIRCLE('',#102709,0.0999999999999998) ;
#34527=CIRCLE('',#102711,0.0999999999999998) ;
#34528=CIRCLE('',#102712,0.0999999999999998) ;
#34529=CIRCLE('',#102714,0.0999999999999998) ;
#34530=CIRCLE('',#102715,0.0999999999999998) ;
#34531=CIRCLE('',#102717,0.0999999999999998) ;
#34532=CIRCLE('',#102718,0.0999999999999998) ;
#34533=CIRCLE('',#102720,0.0999999999999998) ;
#34534=CIRCLE('',#102721,0.0999999999999998) ;
#34535=CIRCLE('',#102723,0.0999999999999998) ;
#34536=CIRCLE('',#102724,0.0999999999999998) ;
#34537=CIRCLE('',#102726,0.0999999999999998) ;
#34538=CIRCLE('',#102727,0.0999999999999998) ;
#34539=CIRCLE('',#102729,0.0999999999999998) ;
#34540=CIRCLE('',#102730,0.0999999999999998) ;
#34541=CIRCLE('',#102732,0.0999999999999998) ;
#34542=CIRCLE('',#102734,0.0999999999999998) ;
#34543=CIRCLE('',#102735,0.0999999999999998) ;
#34544=CIRCLE('',#102736,0.0999999999999998) ;
#34545=CIRCLE('',#102740,0.0999999999999998) ;
#34546=CIRCLE('',#102742,0.0999999999999998) ;
#34547=CIRCLE('',#102743,0.0999999999999998) ;
#34548=CIRCLE('',#102744,0.0999999999999998) ;
#34549=CIRCLE('',#102747,0.0999999999999998) ;
#34550=CIRCLE('',#102749,0.0999999999999998) ;
#34551=CIRCLE('',#102750,0.0999999999999998) ;
#34552=CIRCLE('',#102751,0.0999999999999998) ;
#34553=CIRCLE('',#102754,0.0999999999999998) ;
#34554=CIRCLE('',#102756,0.0999999999999998) ;
#34555=CIRCLE('',#102757,0.0999999999999998) ;
#34556=CIRCLE('',#102758,0.0999999999999998) ;
#34557=CIRCLE('',#102761,0.0999999999999998) ;
#34558=CIRCLE('',#102763,0.0999999999999998) ;
#34559=CIRCLE('',#102764,0.0999999999999998) ;
#34560=CIRCLE('',#102765,0.0999999999999998) ;
#34561=CIRCLE('',#102768,0.0999999999999998) ;
#34562=CIRCLE('',#102770,0.0999999999999998) ;
#34563=CIRCLE('',#102771,0.0999999999999998) ;
#34564=CIRCLE('',#102772,0.0999999999999998) ;
#34565=CIRCLE('',#102775,0.0999999999999998) ;
#34566=CIRCLE('',#102777,0.0999999999999998) ;
#34567=CIRCLE('',#102778,0.0999999999999998) ;
#34568=CIRCLE('',#102779,0.0999999999999998) ;
#34569=CIRCLE('',#102782,0.0999999999999998) ;
#34570=CIRCLE('',#102784,0.0999999999999998) ;
#34571=CIRCLE('',#102785,0.0999999999999998) ;
#34572=CIRCLE('',#102786,0.0999999999999998) ;
#34573=CIRCLE('',#102789,0.0999999999999998) ;
#34574=CIRCLE('',#102790,0.0999999999999998) ;
#34575=CIRCLE('',#102791,0.0999999999999998) ;
#34576=CIRCLE('',#102794,0.1) ;
#34577=CIRCLE('',#102796,0.1) ;
#34578=CIRCLE('',#102797,0.1) ;
#34579=CIRCLE('',#102800,0.0999999999999998) ;
#34580=CIRCLE('',#102802,0.0999999999999998) ;
#34581=CIRCLE('',#102803,0.0999999999999998) ;
#34582=CIRCLE('',#102806,0.0999999999999994) ;
#34583=CIRCLE('',#102808,0.0999999999999994) ;
#34584=CIRCLE('',#102809,0.0999999999999994) ;
#34585=CIRCLE('',#102812,0.1) ;
#34586=CIRCLE('',#102814,0.1) ;
#34587=CIRCLE('',#102815,0.1) ;
#34588=CIRCLE('',#102818,0.0999999999999994) ;
#34589=CIRCLE('',#102820,0.0999999999999994) ;
#34590=CIRCLE('',#102821,0.0999999999999994) ;
#34591=CIRCLE('',#102824,0.0999999999999994) ;
#34592=CIRCLE('',#102826,0.0999999999999994) ;
#34593=CIRCLE('',#102827,0.0999999999999994) ;
#34594=CIRCLE('',#102830,0.0999999999999994) ;
#34595=CIRCLE('',#102832,0.0999999999999994) ;
#34596=CIRCLE('',#102833,0.0999999999999994) ;
#34597=CIRCLE('',#102836,0.0999999999999994) ;
#34598=CIRCLE('',#102838,0.0999999999999994) ;
#34599=CIRCLE('',#102839,0.0999999999999994) ;
#34600=CIRCLE('',#102842,0.0999999999999994) ;
#34601=CIRCLE('',#102844,0.0999999999999994) ;
#34602=CIRCLE('',#102845,0.0999999999999994) ;
#34603=CIRCLE('',#102848,0.0999999999999994) ;
#34604=CIRCLE('',#102850,0.0999999999999994) ;
#34605=CIRCLE('',#102851,0.0999999999999994) ;
#34606=CIRCLE('',#102854,0.0999999999999994) ;
#34607=CIRCLE('',#102856,0.0999999999999994) ;
#34608=CIRCLE('',#102857,0.0999999999999994) ;
#34609=CIRCLE('',#102860,0.0999999999999994) ;
#34610=CIRCLE('',#102862,0.0999999999999994) ;
#34611=CIRCLE('',#102863,0.0999999999999994) ;
#34612=CIRCLE('',#102866,0.0999999999999994) ;
#34613=CIRCLE('',#102868,0.0999999999999994) ;
#34614=CIRCLE('',#102869,0.0999999999999994) ;
#34615=CIRCLE('',#102872,0.0999999999999994) ;
#34616=CIRCLE('',#102874,0.0999999999999994) ;
#34617=CIRCLE('',#102875,0.0999999999999994) ;
#34618=CIRCLE('',#102878,0.100000000000003) ;
#34619=CIRCLE('',#102880,0.100000000000003) ;
#34620=CIRCLE('',#102881,0.100000000000003) ;
#34621=CIRCLE('',#102884,0.0999999999999994) ;
#34622=CIRCLE('',#102886,0.0999999999999994) ;
#34623=CIRCLE('',#102887,0.0999999999999994) ;
#34624=CIRCLE('',#102890,0.100000000000003) ;
#34625=CIRCLE('',#102892,0.100000000000003) ;
#34626=CIRCLE('',#102893,0.100000000000003) ;
#34627=CIRCLE('',#102896,0.100000000000003) ;
#34628=CIRCLE('',#102898,0.100000000000003) ;
#34629=CIRCLE('',#102899,0.100000000000003) ;
#34630=CIRCLE('',#102902,0.1) ;
#34631=CIRCLE('',#102903,0.1) ;
#34632=CIRCLE('',#102906,0.0999999999999999) ;
#34633=CIRCLE('',#102907,0.1) ;
#34634=CIRCLE('',#102910,0.0999999999999999) ;
#34635=CIRCLE('',#102911,0.1) ;
#34636=CIRCLE('',#102914,0.1) ;
#34637=CIRCLE('',#102915,0.1) ;
#34638=CIRCLE('',#102918,0.1) ;
#34639=CIRCLE('',#102919,0.1) ;
#34640=CIRCLE('',#102922,0.1) ;
#34641=CIRCLE('',#102923,0.1) ;
#34642=CIRCLE('',#102926,0.1) ;
#34643=CIRCLE('',#102927,0.1) ;
#34644=CIRCLE('',#102930,0.1) ;
#34645=CIRCLE('',#102931,0.1) ;
#34646=CIRCLE('',#102934,0.1) ;
#34647=CIRCLE('',#102935,0.1) ;
#34648=CIRCLE('',#102938,0.1) ;
#34649=CIRCLE('',#102939,0.1) ;
#34650=CIRCLE('',#102942,0.1) ;
#34651=CIRCLE('',#102943,0.1) ;
#34652=CIRCLE('',#102946,0.1) ;
#34653=CIRCLE('',#102947,0.1) ;
#34654=CIRCLE('',#102950,0.1) ;
#34655=CIRCLE('',#102951,0.1) ;
#34656=CIRCLE('',#102954,0.1) ;
#34657=CIRCLE('',#102955,0.1) ;
#34658=CIRCLE('',#102958,0.0999999999999998) ;
#34659=CIRCLE('',#102959,0.1) ;
#34660=CIRCLE('',#102962,0.1) ;
#34661=CIRCLE('',#102963,0.1) ;
#34662=CIRCLE('',#102966,0.0999999999999998) ;
#34663=CIRCLE('',#102967,0.1) ;
#34664=CIRCLE('',#102970,0.1) ;
#34665=CIRCLE('',#102971,0.1) ;
#34666=CIRCLE('',#102974,2.25) ;
#34667=CIRCLE('',#102976,2.25) ;
#34668=CIRCLE('',#102978,2.25) ;
#34669=CIRCLE('',#102980,2.25) ;
#34670=CIRCLE('',#102982,2.25) ;
#34671=CIRCLE('',#102984,2.25) ;
#34672=CIRCLE('',#102986,0.0999999999999998) ;
#34673=CIRCLE('',#102988,0.100000000000003) ;
#34674=CIRCLE('',#102990,0.100000000000003) ;
#34675=CIRCLE('',#102992,0.100000000000003) ;
#34676=CIRCLE('',#102994,0.100000000000003) ;
#34677=CIRCLE('',#102996,0.100000000000003) ;
#34678=CIRCLE('',#102998,0.100000000000003) ;
#34679=CIRCLE('',#103000,0.100000000000003) ;
#34680=CIRCLE('',#103002,0.100000000000003) ;
#34681=CIRCLE('',#103004,0.100000000000003) ;
#34682=CIRCLE('',#103005,0.0999999999999998) ;
#34683=CIRCLE('',#103007,0.100000000000003) ;
#34684=CIRCLE('',#103009,0.100000000000003) ;
#34685=CIRCLE('',#103011,0.0999999999999998) ;
#34686=CIRCLE('',#103013,0.0999999999999998) ;
#34687=CIRCLE('',#103015,0.0999999999999998) ;
#34688=CIRCLE('',#103016,0.100000000000003) ;
#34689=CIRCLE('',#103018,0.0999999999999998) ;
#34690=CIRCLE('',#103020,0.100000000000003) ;
#34691=CIRCLE('',#103023,0.100000000000003) ;
#34692=CIRCLE('',#103033,0.0999999999999998) ;
#34693=CIRCLE('',#103036,0.0999999999999998) ;
#34694=CIRCLE('',#103038,0.0999999999999998) ;
#34695=CIRCLE('',#103041,0.0999999999999998) ;
#34696=CIRCLE('',#103043,0.0999999999999998) ;
#34697=CIRCLE('',#103046,0.1) ;
#34698=CIRCLE('',#103048,0.0999999999999998) ;
#34699=CIRCLE('',#103050,0.0999999999999998) ;
#34700=CIRCLE('',#103051,0.0999999999999998) ;
#34701=CIRCLE('',#103053,0.0999999999999998) ;
#34702=CIRCLE('',#103055,0.1) ;
#34703=CIRCLE('',#103057,0.1) ;
#34704=CIRCLE('',#103059,0.0999999999999998) ;
#34705=CIRCLE('',#103061,0.0999999999999998) ;
#34706=CIRCLE('',#103063,0.0999999999999998) ;
#34707=CIRCLE('',#103065,0.0999999999999998) ;
#34708=CIRCLE('',#103067,0.0999999999999998) ;
#34709=CIRCLE('',#103069,0.0999999999999998) ;
#34710=CIRCLE('',#103071,0.0999999999999998) ;
#34711=CIRCLE('',#103073,0.0999999999999998) ;
#34712=CIRCLE('',#103075,0.1) ;
#34713=CIRCLE('',#103076,0.100000000000001) ;
#38742=VERTEX_POINT('',#152011) ;
#38743=VERTEX_POINT('',#152012) ;
#38744=VERTEX_POINT('',#152014) ;
#38745=VERTEX_POINT('',#152016) ;
#38746=VERTEX_POINT('',#152020) ;
#38747=VERTEX_POINT('',#152021) ;
#38748=VERTEX_POINT('',#152023) ;
#38749=VERTEX_POINT('',#152025) ;
#38750=VERTEX_POINT('',#152029) ;
#38751=VERTEX_POINT('',#152030) ;
#38752=VERTEX_POINT('',#152032) ;
#38753=VERTEX_POINT('',#152034) ;
#38754=VERTEX_POINT('',#152038) ;
#38755=VERTEX_POINT('',#152039) ;
#38756=VERTEX_POINT('',#152041) ;
#38757=VERTEX_POINT('',#152121) ;
#38758=VERTEX_POINT('',#152174) ;
#38759=VERTEX_POINT('',#152175) ;
#38760=VERTEX_POINT('',#152177) ;
#38761=VERTEX_POINT('',#152179) ;
#38762=VERTEX_POINT('',#152183) ;
#38763=VERTEX_POINT('',#152185) ;
#38764=VERTEX_POINT('',#152265) ;
#38765=VERTEX_POINT('',#152349) ;
#38766=VERTEX_POINT('',#152350) ;
#38767=VERTEX_POINT('',#152352) ;
#38768=VERTEX_POINT('',#152354) ;
#38769=VERTEX_POINT('',#152358) ;
#38770=VERTEX_POINT('',#152360) ;
#38771=VERTEX_POINT('',#152443) ;
#38772=VERTEX_POINT('',#152525) ;
#38773=VERTEX_POINT('',#152526) ;
#38774=VERTEX_POINT('',#152528) ;
#38775=VERTEX_POINT('',#152530) ;
#38776=VERTEX_POINT('',#152534) ;
#38777=VERTEX_POINT('',#152536) ;
#38778=VERTEX_POINT('',#152617) ;
#38779=VERTEX_POINT('',#152701) ;
#38780=VERTEX_POINT('',#152702) ;
#38781=VERTEX_POINT('',#152704) ;
#38782=VERTEX_POINT('',#152706) ;
#38783=VERTEX_POINT('',#152710) ;
#38784=VERTEX_POINT('',#152712) ;
#38785=VERTEX_POINT('',#152792) ;
#38786=VERTEX_POINT('',#152876) ;
#38787=VERTEX_POINT('',#152877) ;
#38788=VERTEX_POINT('',#152879) ;
#38789=VERTEX_POINT('',#152881) ;
#38790=VERTEX_POINT('',#152885) ;
#38791=VERTEX_POINT('',#152887) ;
#38792=VERTEX_POINT('',#152967) ;
#38793=VERTEX_POINT('',#153051) ;
#38794=VERTEX_POINT('',#153052) ;
#38795=VERTEX_POINT('',#153054) ;
#38796=VERTEX_POINT('',#153056) ;
#38797=VERTEX_POINT('',#153060) ;
#38798=VERTEX_POINT('',#153062) ;
#38799=VERTEX_POINT('',#153142) ;
#38800=VERTEX_POINT('',#153226) ;
#38801=VERTEX_POINT('',#153227) ;
#38802=VERTEX_POINT('',#153229) ;
#38803=VERTEX_POINT('',#153231) ;
#38804=VERTEX_POINT('',#153235) ;
#38805=VERTEX_POINT('',#153237) ;
#38806=VERTEX_POINT('',#153319) ;
#38807=VERTEX_POINT('',#153402) ;
#38808=VERTEX_POINT('',#153403) ;
#38809=VERTEX_POINT('',#153405) ;
#38810=VERTEX_POINT('',#153407) ;
#38811=VERTEX_POINT('',#153411) ;
#38812=VERTEX_POINT('',#153413) ;
#38813=VERTEX_POINT('',#153494) ;
#38814=VERTEX_POINT('',#153576) ;
#38815=VERTEX_POINT('',#153577) ;
#38816=VERTEX_POINT('',#153579) ;
#38817=VERTEX_POINT('',#153581) ;
#38818=VERTEX_POINT('',#153585) ;
#38819=VERTEX_POINT('',#153587) ;
#38820=VERTEX_POINT('',#153638) ;
#38821=VERTEX_POINT('',#153748) ;
#38822=VERTEX_POINT('',#153750) ;
#38823=VERTEX_POINT('',#153754) ;
#38824=VERTEX_POINT('',#153756) ;
#38825=VERTEX_POINT('',#153760) ;
#38826=VERTEX_POINT('',#153762) ;
#38827=VERTEX_POINT('',#153766) ;
#38828=VERTEX_POINT('',#153768) ;
#38829=VERTEX_POINT('',#153772) ;
#38830=VERTEX_POINT('',#153774) ;
#38831=VERTEX_POINT('',#153778) ;
#38832=VERTEX_POINT('',#153780) ;
#38833=VERTEX_POINT('',#153784) ;
#38834=VERTEX_POINT('',#153786) ;
#38835=VERTEX_POINT('',#153790) ;
#38836=VERTEX_POINT('',#153792) ;
#38837=VERTEX_POINT('',#153796) ;
#38838=VERTEX_POINT('',#153798) ;
#38839=VERTEX_POINT('',#153802) ;
#38840=VERTEX_POINT('',#153804) ;
#38841=VERTEX_POINT('',#153808) ;
#38842=VERTEX_POINT('',#153810) ;
#38843=VERTEX_POINT('',#153814) ;
#38844=VERTEX_POINT('',#153816) ;
#38845=VERTEX_POINT('',#153820) ;
#38846=VERTEX_POINT('',#153822) ;
#38847=VERTEX_POINT('',#153826) ;
#38848=VERTEX_POINT('',#153828) ;
#38849=VERTEX_POINT('',#153832) ;
#38850=VERTEX_POINT('',#153834) ;
#38851=VERTEX_POINT('',#153838) ;
#38852=VERTEX_POINT('',#153840) ;
#38853=VERTEX_POINT('',#153844) ;
#38854=VERTEX_POINT('',#153846) ;
#38855=VERTEX_POINT('',#153850) ;
#38856=VERTEX_POINT('',#153852) ;
#38857=VERTEX_POINT('',#153856) ;
#38858=VERTEX_POINT('',#153858) ;
#38859=VERTEX_POINT('',#153862) ;
#38860=VERTEX_POINT('',#153864) ;
#38861=VERTEX_POINT('',#153868) ;
#38862=VERTEX_POINT('',#153870) ;
#38863=VERTEX_POINT('',#153874) ;
#38864=VERTEX_POINT('',#153876) ;
#38865=VERTEX_POINT('',#153880) ;
#38866=VERTEX_POINT('',#153882) ;
#38867=VERTEX_POINT('',#153886) ;
#38868=VERTEX_POINT('',#153888) ;
#38869=VERTEX_POINT('',#153892) ;
#38870=VERTEX_POINT('',#153894) ;
#38871=VERTEX_POINT('',#153898) ;
#38872=VERTEX_POINT('',#153900) ;
#38873=VERTEX_POINT('',#153904) ;
#38874=VERTEX_POINT('',#153906) ;
#38875=VERTEX_POINT('',#153910) ;
#38876=VERTEX_POINT('',#153911) ;
#38877=VERTEX_POINT('',#153913) ;
#38878=VERTEX_POINT('',#153924) ;
#38879=VERTEX_POINT('',#153926) ;
#38880=VERTEX_POINT('',#153937) ;
#38881=VERTEX_POINT('',#153939) ;
#38882=VERTEX_POINT('',#153950) ;
#38883=VERTEX_POINT('',#153952) ;
#38884=VERTEX_POINT('',#153984) ;
#38885=VERTEX_POINT('',#153986) ;
#38886=VERTEX_POINT('',#153997) ;
#38887=VERTEX_POINT('',#153999) ;
#38888=VERTEX_POINT('',#154010) ;
#38889=VERTEX_POINT('',#154012) ;
#38890=VERTEX_POINT('',#154023) ;
#38891=VERTEX_POINT('',#154025) ;
#38892=VERTEX_POINT('',#154060) ;
#38893=VERTEX_POINT('',#154061) ;
#38894=VERTEX_POINT('',#154063) ;
#38895=VERTEX_POINT('',#154074) ;
#38896=VERTEX_POINT('',#154076) ;
#38897=VERTEX_POINT('',#154087) ;
#38898=VERTEX_POINT('',#154089) ;
#38899=VERTEX_POINT('',#154100) ;
#38900=VERTEX_POINT('',#154102) ;
#38901=VERTEX_POINT('',#154134) ;
#38902=VERTEX_POINT('',#154136) ;
#38903=VERTEX_POINT('',#154147) ;
#38904=VERTEX_POINT('',#154149) ;
#38905=VERTEX_POINT('',#154160) ;
#38906=VERTEX_POINT('',#154162) ;
#38907=VERTEX_POINT('',#154173) ;
#38908=VERTEX_POINT('',#154175) ;
#38909=VERTEX_POINT('',#154210) ;
#38910=VERTEX_POINT('',#154211) ;
#38911=VERTEX_POINT('',#154213) ;
#38912=VERTEX_POINT('',#154224) ;
#38913=VERTEX_POINT('',#154226) ;
#38914=VERTEX_POINT('',#154237) ;
#38915=VERTEX_POINT('',#154239) ;
#38916=VERTEX_POINT('',#154250) ;
#38917=VERTEX_POINT('',#154252) ;
#38918=VERTEX_POINT('',#154284) ;
#38919=VERTEX_POINT('',#154286) ;
#38920=VERTEX_POINT('',#154297) ;
#38921=VERTEX_POINT('',#154299) ;
#38922=VERTEX_POINT('',#154310) ;
#38923=VERTEX_POINT('',#154312) ;
#38924=VERTEX_POINT('',#154323) ;
#38925=VERTEX_POINT('',#154325) ;
#38926=VERTEX_POINT('',#154360) ;
#38927=VERTEX_POINT('',#154361) ;
#38928=VERTEX_POINT('',#154363) ;
#38929=VERTEX_POINT('',#154374) ;
#38930=VERTEX_POINT('',#154376) ;
#38931=VERTEX_POINT('',#154387) ;
#38932=VERTEX_POINT('',#154389) ;
#38933=VERTEX_POINT('',#154400) ;
#38934=VERTEX_POINT('',#154402) ;
#38935=VERTEX_POINT('',#154434) ;
#38936=VERTEX_POINT('',#154436) ;
#38937=VERTEX_POINT('',#154447) ;
#38938=VERTEX_POINT('',#154449) ;
#38939=VERTEX_POINT('',#154460) ;
#38940=VERTEX_POINT('',#154462) ;
#38941=VERTEX_POINT('',#154473) ;
#38942=VERTEX_POINT('',#154475) ;
#38943=VERTEX_POINT('',#154510) ;
#38944=VERTEX_POINT('',#154511) ;
#38945=VERTEX_POINT('',#154513) ;
#38946=VERTEX_POINT('',#154524) ;
#38947=VERTEX_POINT('',#154526) ;
#38948=VERTEX_POINT('',#154537) ;
#38949=VERTEX_POINT('',#154539) ;
#38950=VERTEX_POINT('',#154550) ;
#38951=VERTEX_POINT('',#154552) ;
#38952=VERTEX_POINT('',#154584) ;
#38953=VERTEX_POINT('',#154586) ;
#38954=VERTEX_POINT('',#154597) ;
#38955=VERTEX_POINT('',#154599) ;
#38956=VERTEX_POINT('',#154610) ;
#38957=VERTEX_POINT('',#154612) ;
#38958=VERTEX_POINT('',#154623) ;
#38959=VERTEX_POINT('',#154625) ;
#38960=VERTEX_POINT('',#154660) ;
#38961=VERTEX_POINT('',#154661) ;
#38962=VERTEX_POINT('',#154663) ;
#38963=VERTEX_POINT('',#154674) ;
#38964=VERTEX_POINT('',#154676) ;
#38965=VERTEX_POINT('',#154687) ;
#38966=VERTEX_POINT('',#154689) ;
#38967=VERTEX_POINT('',#154700) ;
#38968=VERTEX_POINT('',#154702) ;
#38969=VERTEX_POINT('',#154734) ;
#38970=VERTEX_POINT('',#154736) ;
#38971=VERTEX_POINT('',#154747) ;
#38972=VERTEX_POINT('',#154749) ;
#38973=VERTEX_POINT('',#154760) ;
#38974=VERTEX_POINT('',#154762) ;
#38975=VERTEX_POINT('',#154773) ;
#38976=VERTEX_POINT('',#154775) ;
#38977=VERTEX_POINT('',#154810) ;
#38978=VERTEX_POINT('',#154811) ;
#38979=VERTEX_POINT('',#154813) ;
#38980=VERTEX_POINT('',#154824) ;
#38981=VERTEX_POINT('',#154826) ;
#38982=VERTEX_POINT('',#154837) ;
#38983=VERTEX_POINT('',#154839) ;
#38984=VERTEX_POINT('',#154850) ;
#38985=VERTEX_POINT('',#154852) ;
#38986=VERTEX_POINT('',#154884) ;
#38987=VERTEX_POINT('',#154886) ;
#38988=VERTEX_POINT('',#154897) ;
#38989=VERTEX_POINT('',#154899) ;
#38990=VERTEX_POINT('',#154910) ;
#38991=VERTEX_POINT('',#154912) ;
#38992=VERTEX_POINT('',#154923) ;
#38993=VERTEX_POINT('',#154925) ;
#38994=VERTEX_POINT('',#154960) ;
#38995=VERTEX_POINT('',#154961) ;
#38996=VERTEX_POINT('',#154963) ;
#38997=VERTEX_POINT('',#154974) ;
#38998=VERTEX_POINT('',#154976) ;
#38999=VERTEX_POINT('',#154987) ;
#39000=VERTEX_POINT('',#154989) ;
#39001=VERTEX_POINT('',#155000) ;
#39002=VERTEX_POINT('',#155002) ;
#39003=VERTEX_POINT('',#155034) ;
#39004=VERTEX_POINT('',#155036) ;
#39005=VERTEX_POINT('',#155047) ;
#39006=VERTEX_POINT('',#155049) ;
#39007=VERTEX_POINT('',#155060) ;
#39008=VERTEX_POINT('',#155062) ;
#39009=VERTEX_POINT('',#155073) ;
#39010=VERTEX_POINT('',#155075) ;
#39011=VERTEX_POINT('',#155110) ;
#39012=VERTEX_POINT('',#155111) ;
#39013=VERTEX_POINT('',#155113) ;
#39014=VERTEX_POINT('',#155124) ;
#39015=VERTEX_POINT('',#155126) ;
#39016=VERTEX_POINT('',#155137) ;
#39017=VERTEX_POINT('',#155139) ;
#39018=VERTEX_POINT('',#155150) ;
#39019=VERTEX_POINT('',#155152) ;
#39020=VERTEX_POINT('',#155184) ;
#39021=VERTEX_POINT('',#155186) ;
#39022=VERTEX_POINT('',#155197) ;
#39023=VERTEX_POINT('',#155199) ;
#39024=VERTEX_POINT('',#155210) ;
#39025=VERTEX_POINT('',#155212) ;
#39026=VERTEX_POINT('',#155223) ;
#39027=VERTEX_POINT('',#155225) ;
#39028=VERTEX_POINT('',#155260) ;
#39029=VERTEX_POINT('',#155264) ;
#39030=VERTEX_POINT('',#155268) ;
#39031=VERTEX_POINT('',#155272) ;
#39032=VERTEX_POINT('',#155276) ;
#39033=VERTEX_POINT('',#155280) ;
#39034=VERTEX_POINT('',#155284) ;
#39035=VERTEX_POINT('',#155288) ;
#39036=VERTEX_POINT('',#155292) ;
#39037=VERTEX_POINT('',#155314) ;
#39038=VERTEX_POINT('',#155316) ;
#39039=VERTEX_POINT('',#155320) ;
#39040=VERTEX_POINT('',#155322) ;
#39041=VERTEX_POINT('',#155326) ;
#39042=VERTEX_POINT('',#155328) ;
#39043=VERTEX_POINT('',#155336) ;
#39044=VERTEX_POINT('',#155341) ;
#39045=VERTEX_POINT('',#155350) ;
#39046=VERTEX_POINT('',#155351) ;
#39047=VERTEX_POINT('',#155353) ;
#39048=VERTEX_POINT('',#155364) ;
#39049=VERTEX_POINT('',#155366) ;
#39050=VERTEX_POINT('',#155377) ;
#39051=VERTEX_POINT('',#155379) ;
#39052=VERTEX_POINT('',#155390) ;
#39053=VERTEX_POINT('',#155392) ;
#39054=VERTEX_POINT('',#155424) ;
#39055=VERTEX_POINT('',#155426) ;
#39056=VERTEX_POINT('',#155437) ;
#39057=VERTEX_POINT('',#155439) ;
#39058=VERTEX_POINT('',#155450) ;
#39059=VERTEX_POINT('',#155452) ;
#39060=VERTEX_POINT('',#155463) ;
#39061=VERTEX_POINT('',#155465) ;
#39062=VERTEX_POINT('',#155500) ;
#39063=VERTEX_POINT('',#155506) ;
#39064=VERTEX_POINT('',#155507) ;
#39065=VERTEX_POINT('',#155509) ;
#39066=VERTEX_POINT('',#155511) ;
#39067=VERTEX_POINT('',#155524) ;
#39068=VERTEX_POINT('',#155526) ;
#39069=VERTEX_POINT('',#155529) ;
#39070=VERTEX_POINT('',#155530) ;
#39071=VERTEX_POINT('',#155532) ;
#39072=VERTEX_POINT('',#155534) ;
#39073=VERTEX_POINT('',#155536) ;
#39074=VERTEX_POINT('',#155538) ;
#39075=VERTEX_POINT('',#155540) ;
#39076=VERTEX_POINT('',#155542) ;
#39077=VERTEX_POINT('',#155545) ;
#39078=VERTEX_POINT('',#155546) ;
#39079=VERTEX_POINT('',#155548) ;
#39080=VERTEX_POINT('',#155550) ;
#39081=VERTEX_POINT('',#155552) ;
#39082=VERTEX_POINT('',#155554) ;
#39083=VERTEX_POINT('',#155556) ;
#39084=VERTEX_POINT('',#155558) ;
#39085=VERTEX_POINT('',#155561) ;
#39086=VERTEX_POINT('',#155562) ;
#39087=VERTEX_POINT('',#155564) ;
#39088=VERTEX_POINT('',#155566) ;
#39089=VERTEX_POINT('',#155568) ;
#39090=VERTEX_POINT('',#155570) ;
#39091=VERTEX_POINT('',#155572) ;
#39092=VERTEX_POINT('',#155574) ;
#39093=VERTEX_POINT('',#155577) ;
#39094=VERTEX_POINT('',#155578) ;
#39095=VERTEX_POINT('',#155580) ;
#39096=VERTEX_POINT('',#155582) ;
#39097=VERTEX_POINT('',#155584) ;
#39098=VERTEX_POINT('',#155586) ;
#39099=VERTEX_POINT('',#155588) ;
#39100=VERTEX_POINT('',#155590) ;
#39101=VERTEX_POINT('',#155593) ;
#39102=VERTEX_POINT('',#155594) ;
#39103=VERTEX_POINT('',#155596) ;
#39104=VERTEX_POINT('',#155598) ;
#39105=VERTEX_POINT('',#155600) ;
#39106=VERTEX_POINT('',#155602) ;
#39107=VERTEX_POINT('',#155604) ;
#39108=VERTEX_POINT('',#155606) ;
#39109=VERTEX_POINT('',#155609) ;
#39110=VERTEX_POINT('',#155610) ;
#39111=VERTEX_POINT('',#155612) ;
#39112=VERTEX_POINT('',#155614) ;
#39113=VERTEX_POINT('',#155616) ;
#39114=VERTEX_POINT('',#155618) ;
#39115=VERTEX_POINT('',#155620) ;
#39116=VERTEX_POINT('',#155622) ;
#39117=VERTEX_POINT('',#155625) ;
#39118=VERTEX_POINT('',#155626) ;
#39119=VERTEX_POINT('',#155628) ;
#39120=VERTEX_POINT('',#155630) ;
#39121=VERTEX_POINT('',#155632) ;
#39122=VERTEX_POINT('',#155634) ;
#39123=VERTEX_POINT('',#155636) ;
#39124=VERTEX_POINT('',#155638) ;
#39125=VERTEX_POINT('',#155641) ;
#39126=VERTEX_POINT('',#155642) ;
#39127=VERTEX_POINT('',#155644) ;
#39128=VERTEX_POINT('',#155646) ;
#39129=VERTEX_POINT('',#155648) ;
#39130=VERTEX_POINT('',#155650) ;
#39131=VERTEX_POINT('',#155652) ;
#39132=VERTEX_POINT('',#155654) ;
#39133=VERTEX_POINT('',#155657) ;
#39134=VERTEX_POINT('',#155658) ;
#39135=VERTEX_POINT('',#155660) ;
#39136=VERTEX_POINT('',#155662) ;
#39137=VERTEX_POINT('',#155664) ;
#39138=VERTEX_POINT('',#155666) ;
#39139=VERTEX_POINT('',#155668) ;
#39140=VERTEX_POINT('',#155670) ;
#39141=VERTEX_POINT('',#155673) ;
#39142=VERTEX_POINT('',#155674) ;
#39143=VERTEX_POINT('',#155676) ;
#39144=VERTEX_POINT('',#155678) ;
#39145=VERTEX_POINT('',#155680) ;
#39146=VERTEX_POINT('',#155682) ;
#39147=VERTEX_POINT('',#155684) ;
#39148=VERTEX_POINT('',#155686) ;
#39149=VERTEX_POINT('',#155690) ;
#39150=VERTEX_POINT('',#155691) ;
#39151=VERTEX_POINT('',#155693) ;
#39152=VERTEX_POINT('',#155695) ;
#39153=VERTEX_POINT('',#155698) ;
#39154=VERTEX_POINT('',#155699) ;
#39155=VERTEX_POINT('',#155701) ;
#39156=VERTEX_POINT('',#155703) ;
#39157=VERTEX_POINT('',#155705) ;
#39158=VERTEX_POINT('',#155707) ;
#39159=VERTEX_POINT('',#155709) ;
#39160=VERTEX_POINT('',#155711) ;
#39161=VERTEX_POINT('',#155715) ;
#39162=VERTEX_POINT('',#155716) ;
#39163=VERTEX_POINT('',#155718) ;
#39164=VERTEX_POINT('',#155720) ;
#39165=VERTEX_POINT('',#155723) ;
#39166=VERTEX_POINT('',#155724) ;
#39167=VERTEX_POINT('',#155726) ;
#39168=VERTEX_POINT('',#155728) ;
#39169=VERTEX_POINT('',#155730) ;
#39170=VERTEX_POINT('',#155732) ;
#39171=VERTEX_POINT('',#155734) ;
#39172=VERTEX_POINT('',#155736) ;
#39173=VERTEX_POINT('',#155740) ;
#39174=VERTEX_POINT('',#155741) ;
#39175=VERTEX_POINT('',#155743) ;
#39176=VERTEX_POINT('',#155745) ;
#39177=VERTEX_POINT('',#155748) ;
#39178=VERTEX_POINT('',#155749) ;
#39179=VERTEX_POINT('',#155751) ;
#39180=VERTEX_POINT('',#155753) ;
#39181=VERTEX_POINT('',#155755) ;
#39182=VERTEX_POINT('',#155757) ;
#39183=VERTEX_POINT('',#155759) ;
#39184=VERTEX_POINT('',#155761) ;
#39185=VERTEX_POINT('',#155765) ;
#39186=VERTEX_POINT('',#155766) ;
#39187=VERTEX_POINT('',#155768) ;
#39188=VERTEX_POINT('',#155770) ;
#39189=VERTEX_POINT('',#155773) ;
#39190=VERTEX_POINT('',#155774) ;
#39191=VERTEX_POINT('',#155776) ;
#39192=VERTEX_POINT('',#155778) ;
#39193=VERTEX_POINT('',#155780) ;
#39194=VERTEX_POINT('',#155782) ;
#39195=VERTEX_POINT('',#155784) ;
#39196=VERTEX_POINT('',#155786) ;
#39197=VERTEX_POINT('',#155790) ;
#39198=VERTEX_POINT('',#155791) ;
#39199=VERTEX_POINT('',#155793) ;
#39200=VERTEX_POINT('',#155795) ;
#39201=VERTEX_POINT('',#155798) ;
#39202=VERTEX_POINT('',#155799) ;
#39203=VERTEX_POINT('',#155801) ;
#39204=VERTEX_POINT('',#155803) ;
#39205=VERTEX_POINT('',#155805) ;
#39206=VERTEX_POINT('',#155807) ;
#39207=VERTEX_POINT('',#155809) ;
#39208=VERTEX_POINT('',#155811) ;
#39209=VERTEX_POINT('',#155815) ;
#39210=VERTEX_POINT('',#155816) ;
#39211=VERTEX_POINT('',#155818) ;
#39212=VERTEX_POINT('',#155820) ;
#39213=VERTEX_POINT('',#155823) ;
#39214=VERTEX_POINT('',#155824) ;
#39215=VERTEX_POINT('',#155826) ;
#39216=VERTEX_POINT('',#155828) ;
#39217=VERTEX_POINT('',#155830) ;
#39218=VERTEX_POINT('',#155832) ;
#39219=VERTEX_POINT('',#155834) ;
#39220=VERTEX_POINT('',#155836) ;
#39221=VERTEX_POINT('',#155840) ;
#39222=VERTEX_POINT('',#155841) ;
#39223=VERTEX_POINT('',#155843) ;
#39224=VERTEX_POINT('',#155845) ;
#39225=VERTEX_POINT('',#155848) ;
#39226=VERTEX_POINT('',#155849) ;
#39227=VERTEX_POINT('',#155851) ;
#39228=VERTEX_POINT('',#155853) ;
#39229=VERTEX_POINT('',#155855) ;
#39230=VERTEX_POINT('',#155857) ;
#39231=VERTEX_POINT('',#155859) ;
#39232=VERTEX_POINT('',#155861) ;
#39233=VERTEX_POINT('',#155865) ;
#39234=VERTEX_POINT('',#155866) ;
#39235=VERTEX_POINT('',#155868) ;
#39236=VERTEX_POINT('',#155870) ;
#39237=VERTEX_POINT('',#155873) ;
#39238=VERTEX_POINT('',#155874) ;
#39239=VERTEX_POINT('',#155876) ;
#39240=VERTEX_POINT('',#155878) ;
#39241=VERTEX_POINT('',#155880) ;
#39242=VERTEX_POINT('',#155882) ;
#39243=VERTEX_POINT('',#155884) ;
#39244=VERTEX_POINT('',#155886) ;
#39245=VERTEX_POINT('',#155890) ;
#39246=VERTEX_POINT('',#155891) ;
#39247=VERTEX_POINT('',#155893) ;
#39248=VERTEX_POINT('',#155895) ;
#39249=VERTEX_POINT('',#155898) ;
#39250=VERTEX_POINT('',#155899) ;
#39251=VERTEX_POINT('',#155901) ;
#39252=VERTEX_POINT('',#155903) ;
#39253=VERTEX_POINT('',#155905) ;
#39254=VERTEX_POINT('',#155907) ;
#39255=VERTEX_POINT('',#155909) ;
#39256=VERTEX_POINT('',#155911) ;
#39257=VERTEX_POINT('',#155933) ;
#39258=VERTEX_POINT('',#155934) ;
#39259=VERTEX_POINT('',#155936) ;
#39260=VERTEX_POINT('',#155938) ;
#39261=VERTEX_POINT('',#155940) ;
#39262=VERTEX_POINT('',#155942) ;
#39263=VERTEX_POINT('',#155944) ;
#39264=VERTEX_POINT('',#155946) ;
#39265=VERTEX_POINT('',#155948) ;
#39266=VERTEX_POINT('',#155950) ;
#39267=VERTEX_POINT('',#155952) ;
#39268=VERTEX_POINT('',#155954) ;
#39269=VERTEX_POINT('',#155956) ;
#39270=VERTEX_POINT('',#155958) ;
#39271=VERTEX_POINT('',#155960) ;
#39272=VERTEX_POINT('',#155962) ;
#39273=VERTEX_POINT('',#155964) ;
#39274=VERTEX_POINT('',#155966) ;
#39275=VERTEX_POINT('',#155968) ;
#39276=VERTEX_POINT('',#155970) ;
#39277=VERTEX_POINT('',#155972) ;
#39278=VERTEX_POINT('',#155974) ;
#39279=VERTEX_POINT('',#155976) ;
#39280=VERTEX_POINT('',#155978) ;
#39281=VERTEX_POINT('',#155980) ;
#39282=VERTEX_POINT('',#155982) ;
#39283=VERTEX_POINT('',#155984) ;
#39284=VERTEX_POINT('',#155986) ;
#39285=VERTEX_POINT('',#155988) ;
#39286=VERTEX_POINT('',#155990) ;
#39287=VERTEX_POINT('',#155992) ;
#39288=VERTEX_POINT('',#155994) ;
#39289=VERTEX_POINT('',#155996) ;
#39290=VERTEX_POINT('',#155998) ;
#39291=VERTEX_POINT('',#156000) ;
#39292=VERTEX_POINT('',#156002) ;
#39293=VERTEX_POINT('',#156004) ;
#39294=VERTEX_POINT('',#156006) ;
#39295=VERTEX_POINT('',#156008) ;
#39296=VERTEX_POINT('',#156010) ;
#39297=VERTEX_POINT('',#156012) ;
#39298=VERTEX_POINT('',#156014) ;
#39299=VERTEX_POINT('',#156016) ;
#39300=VERTEX_POINT('',#156018) ;
#39301=VERTEX_POINT('',#156020) ;
#39302=VERTEX_POINT('',#156022) ;
#39303=VERTEX_POINT('',#156024) ;
#39304=VERTEX_POINT('',#156026) ;
#39305=VERTEX_POINT('',#156028) ;
#39306=VERTEX_POINT('',#156030) ;
#39307=VERTEX_POINT('',#156032) ;
#39308=VERTEX_POINT('',#156034) ;
#39309=VERTEX_POINT('',#156036) ;
#39310=VERTEX_POINT('',#156038) ;
#39311=VERTEX_POINT('',#156040) ;
#39312=VERTEX_POINT('',#156042) ;
#39313=VERTEX_POINT('',#156044) ;
#39314=VERTEX_POINT('',#156046) ;
#39315=VERTEX_POINT('',#156048) ;
#39316=VERTEX_POINT('',#156050) ;
#39317=VERTEX_POINT('',#156052) ;
#39318=VERTEX_POINT('',#156054) ;
#39319=VERTEX_POINT('',#156056) ;
#39320=VERTEX_POINT('',#156058) ;
#39321=VERTEX_POINT('',#156062) ;
#39322=VERTEX_POINT('',#156063) ;
#39323=VERTEX_POINT('',#156065) ;
#39324=VERTEX_POINT('',#156067) ;
#39325=VERTEX_POINT('',#156069) ;
#39326=VERTEX_POINT('',#156071) ;
#39327=VERTEX_POINT('',#156073) ;
#39328=VERTEX_POINT('',#156075) ;
#39329=VERTEX_POINT('',#156079) ;
#39330=VERTEX_POINT('',#156080) ;
#39331=VERTEX_POINT('',#156082) ;
#39332=VERTEX_POINT('',#156084) ;
#39333=VERTEX_POINT('',#156086) ;
#39334=VERTEX_POINT('',#156088) ;
#39335=VERTEX_POINT('',#156090) ;
#39336=VERTEX_POINT('',#156092) ;
#39337=VERTEX_POINT('',#156096) ;
#39338=VERTEX_POINT('',#156097) ;
#39339=VERTEX_POINT('',#156099) ;
#39340=VERTEX_POINT('',#156101) ;
#39341=VERTEX_POINT('',#156103) ;
#39342=VERTEX_POINT('',#156105) ;
#39343=VERTEX_POINT('',#156107) ;
#39344=VERTEX_POINT('',#156109) ;
#39345=VERTEX_POINT('',#156113) ;
#39346=VERTEX_POINT('',#156114) ;
#39347=VERTEX_POINT('',#156116) ;
#39348=VERTEX_POINT('',#156118) ;
#39349=VERTEX_POINT('',#156120) ;
#39350=VERTEX_POINT('',#156122) ;
#39351=VERTEX_POINT('',#156124) ;
#39352=VERTEX_POINT('',#156126) ;
#39353=VERTEX_POINT('',#156130) ;
#39354=VERTEX_POINT('',#156131) ;
#39355=VERTEX_POINT('',#156133) ;
#39356=VERTEX_POINT('',#156135) ;
#39357=VERTEX_POINT('',#156137) ;
#39358=VERTEX_POINT('',#156139) ;
#39359=VERTEX_POINT('',#156141) ;
#39360=VERTEX_POINT('',#156143) ;
#39361=VERTEX_POINT('',#156147) ;
#39362=VERTEX_POINT('',#156148) ;
#39363=VERTEX_POINT('',#156150) ;
#39364=VERTEX_POINT('',#156152) ;
#39365=VERTEX_POINT('',#156154) ;
#39366=VERTEX_POINT('',#156156) ;
#39367=VERTEX_POINT('',#156158) ;
#39368=VERTEX_POINT('',#156160) ;
#39369=VERTEX_POINT('',#156164) ;
#39370=VERTEX_POINT('',#156165) ;
#39371=VERTEX_POINT('',#156167) ;
#39372=VERTEX_POINT('',#156169) ;
#39373=VERTEX_POINT('',#156171) ;
#39374=VERTEX_POINT('',#156173) ;
#39375=VERTEX_POINT('',#156175) ;
#39376=VERTEX_POINT('',#156177) ;
#39377=VERTEX_POINT('',#156181) ;
#39378=VERTEX_POINT('',#156182) ;
#39379=VERTEX_POINT('',#156184) ;
#39380=VERTEX_POINT('',#156186) ;
#39381=VERTEX_POINT('',#156188) ;
#39382=VERTEX_POINT('',#156190) ;
#39383=VERTEX_POINT('',#156192) ;
#39384=VERTEX_POINT('',#156194) ;
#39385=VERTEX_POINT('',#156198) ;
#39386=VERTEX_POINT('',#156199) ;
#39387=VERTEX_POINT('',#156201) ;
#39388=VERTEX_POINT('',#156203) ;
#39389=VERTEX_POINT('',#156205) ;
#39390=VERTEX_POINT('',#156207) ;
#39391=VERTEX_POINT('',#156209) ;
#39392=VERTEX_POINT('',#156211) ;
#39393=VERTEX_POINT('',#156215) ;
#39394=VERTEX_POINT('',#156216) ;
#39395=VERTEX_POINT('',#156218) ;
#39396=VERTEX_POINT('',#156220) ;
#39397=VERTEX_POINT('',#156224) ;
#39398=VERTEX_POINT('',#156225) ;
#39399=VERTEX_POINT('',#156227) ;
#39400=VERTEX_POINT('',#156229) ;
#39401=VERTEX_POINT('',#156231) ;
#39402=VERTEX_POINT('',#156233) ;
#39403=VERTEX_POINT('',#156235) ;
#39404=VERTEX_POINT('',#156237) ;
#39405=VERTEX_POINT('',#156239) ;
#39406=VERTEX_POINT('',#156241) ;
#39407=VERTEX_POINT('',#156243) ;
#39408=VERTEX_POINT('',#156245) ;
#39409=VERTEX_POINT('',#156247) ;
#39410=VERTEX_POINT('',#156249) ;
#39411=VERTEX_POINT('',#156251) ;
#39412=VERTEX_POINT('',#156253) ;
#39413=VERTEX_POINT('',#156255) ;
#39414=VERTEX_POINT('',#156257) ;
#39415=VERTEX_POINT('',#156259) ;
#39416=VERTEX_POINT('',#156261) ;
#39417=VERTEX_POINT('',#156263) ;
#39418=VERTEX_POINT('',#156265) ;
#39419=VERTEX_POINT('',#156267) ;
#39420=VERTEX_POINT('',#156269) ;
#39421=VERTEX_POINT('',#156271) ;
#39422=VERTEX_POINT('',#156273) ;
#39423=VERTEX_POINT('',#156275) ;
#39424=VERTEX_POINT('',#156277) ;
#39425=VERTEX_POINT('',#156279) ;
#39426=VERTEX_POINT('',#156281) ;
#39427=VERTEX_POINT('',#156283) ;
#39428=VERTEX_POINT('',#156285) ;
#39429=VERTEX_POINT('',#156287) ;
#39430=VERTEX_POINT('',#156289) ;
#39431=VERTEX_POINT('',#156291) ;
#39432=VERTEX_POINT('',#156293) ;
#39433=VERTEX_POINT('',#156295) ;
#39434=VERTEX_POINT('',#156297) ;
#39435=VERTEX_POINT('',#156299) ;
#39436=VERTEX_POINT('',#156301) ;
#39437=VERTEX_POINT('',#156303) ;
#39438=VERTEX_POINT('',#156305) ;
#39439=VERTEX_POINT('',#156307) ;
#39440=VERTEX_POINT('',#156309) ;
#39441=VERTEX_POINT('',#156311) ;
#39442=VERTEX_POINT('',#156313) ;
#39443=VERTEX_POINT('',#156315) ;
#39444=VERTEX_POINT('',#156317) ;
#39445=VERTEX_POINT('',#156319) ;
#39446=VERTEX_POINT('',#156321) ;
#39447=VERTEX_POINT('',#156323) ;
#39448=VERTEX_POINT('',#156325) ;
#39449=VERTEX_POINT('',#156327) ;
#39450=VERTEX_POINT('',#156329) ;
#39451=VERTEX_POINT('',#156331) ;
#39452=VERTEX_POINT('',#156333) ;
#39453=VERTEX_POINT('',#156335) ;
#39454=VERTEX_POINT('',#156337) ;
#39455=VERTEX_POINT('',#156339) ;
#39456=VERTEX_POINT('',#156341) ;
#39457=VERTEX_POINT('',#156343) ;
#39458=VERTEX_POINT('',#156345) ;
#39459=VERTEX_POINT('',#156347) ;
#39460=VERTEX_POINT('',#156349) ;
#39461=VERTEX_POINT('',#156353) ;
#39462=VERTEX_POINT('',#156354) ;
#39463=VERTEX_POINT('',#156359) ;
#39464=VERTEX_POINT('',#156360) ;
#39465=VERTEX_POINT('',#156362) ;
#39466=VERTEX_POINT('',#156365) ;
#39467=VERTEX_POINT('',#156369) ;
#39468=VERTEX_POINT('',#156370) ;
#39469=VERTEX_POINT('',#156372) ;
#39470=VERTEX_POINT('',#156374) ;
#39471=VERTEX_POINT('',#156377) ;
#39472=VERTEX_POINT('',#156378) ;
#39473=VERTEX_POINT('',#156385) ;
#39474=VERTEX_POINT('',#156387) ;
#39475=VERTEX_POINT('',#156394) ;
#39476=VERTEX_POINT('',#156396) ;
#39477=VERTEX_POINT('',#156403) ;
#39478=VERTEX_POINT('',#156405) ;
#39479=VERTEX_POINT('',#156413) ;
#39480=VERTEX_POINT('',#156414) ;
#39481=VERTEX_POINT('',#156416) ;
#39482=VERTEX_POINT('',#156418) ;
#39483=VERTEX_POINT('',#156421) ;
#39484=VERTEX_POINT('',#156422) ;
#39485=VERTEX_POINT('',#156424) ;
#39486=VERTEX_POINT('',#156426) ;
#39487=VERTEX_POINT('',#156429) ;
#39488=VERTEX_POINT('',#156430) ;
#39489=VERTEX_POINT('',#156432) ;
#39490=VERTEX_POINT('',#156434) ;
#39491=VERTEX_POINT('',#156437) ;
#39492=VERTEX_POINT('',#156438) ;
#39493=VERTEX_POINT('',#156440) ;
#39494=VERTEX_POINT('',#156442) ;
#39495=VERTEX_POINT('',#156445) ;
#39496=VERTEX_POINT('',#156446) ;
#39497=VERTEX_POINT('',#156448) ;
#39498=VERTEX_POINT('',#156450) ;
#39499=VERTEX_POINT('',#156453) ;
#39500=VERTEX_POINT('',#156454) ;
#39501=VERTEX_POINT('',#156456) ;
#39502=VERTEX_POINT('',#156458) ;
#39503=VERTEX_POINT('',#156461) ;
#39504=VERTEX_POINT('',#156462) ;
#39505=VERTEX_POINT('',#156464) ;
#39506=VERTEX_POINT('',#156466) ;
#39507=VERTEX_POINT('',#156469) ;
#39508=VERTEX_POINT('',#156470) ;
#39509=VERTEX_POINT('',#156472) ;
#39510=VERTEX_POINT('',#156474) ;
#39511=VERTEX_POINT('',#156477) ;
#39512=VERTEX_POINT('',#156478) ;
#39513=VERTEX_POINT('',#156485) ;
#39514=VERTEX_POINT('',#156487) ;
#39515=VERTEX_POINT('',#156494) ;
#39516=VERTEX_POINT('',#156496) ;
#39517=VERTEX_POINT('',#156503) ;
#39518=VERTEX_POINT('',#156505) ;
#39519=VERTEX_POINT('',#156514) ;
#39520=VERTEX_POINT('',#156515) ;
#39521=VERTEX_POINT('',#156517) ;
#39522=VERTEX_POINT('',#156519) ;
#39523=VERTEX_POINT('',#156522) ;
#39524=VERTEX_POINT('',#156523) ;
#39525=VERTEX_POINT('',#156525) ;
#39526=VERTEX_POINT('',#156527) ;
#39527=VERTEX_POINT('',#156529) ;
#39528=VERTEX_POINT('',#156531) ;
#39529=VERTEX_POINT('',#156533) ;
#39530=VERTEX_POINT('',#156535) ;
#39531=VERTEX_POINT('',#156539) ;
#39532=VERTEX_POINT('',#156540) ;
#39533=VERTEX_POINT('',#156542) ;
#39534=VERTEX_POINT('',#156544) ;
#39535=VERTEX_POINT('',#156550) ;
#39536=VERTEX_POINT('',#156551) ;
#39537=VERTEX_POINT('',#156553) ;
#39538=VERTEX_POINT('',#156555) ;
#39539=VERTEX_POINT('',#156557) ;
#39540=VERTEX_POINT('',#156559) ;
#39541=VERTEX_POINT('',#156561) ;
#39542=VERTEX_POINT('',#156563) ;
#39543=VERTEX_POINT('',#156567) ;
#39544=VERTEX_POINT('',#156568) ;
#39545=VERTEX_POINT('',#156570) ;
#39546=VERTEX_POINT('',#156572) ;
#39547=VERTEX_POINT('',#156576) ;
#39548=VERTEX_POINT('',#156578) ;
#39549=VERTEX_POINT('',#156582) ;
#39550=VERTEX_POINT('',#156583) ;
#39551=VERTEX_POINT('',#156585) ;
#39552=VERTEX_POINT('',#156587) ;
#39553=VERTEX_POINT('',#156591) ;
#39554=VERTEX_POINT('',#156592) ;
#39555=VERTEX_POINT('',#156594) ;
#39556=VERTEX_POINT('',#156596) ;
#39557=VERTEX_POINT('',#156599) ;
#39558=VERTEX_POINT('',#156600) ;
#39559=VERTEX_POINT('',#156602) ;
#39560=VERTEX_POINT('',#156604) ;
#39561=VERTEX_POINT('',#156607) ;
#39562=VERTEX_POINT('',#156608) ;
#39563=VERTEX_POINT('',#156610) ;
#39564=VERTEX_POINT('',#156612) ;
#39565=VERTEX_POINT('',#156615) ;
#39566=VERTEX_POINT('',#156616) ;
#39567=VERTEX_POINT('',#156618) ;
#39568=VERTEX_POINT('',#156620) ;
#39569=VERTEX_POINT('',#156623) ;
#39570=VERTEX_POINT('',#156624) ;
#39571=VERTEX_POINT('',#156626) ;
#39572=VERTEX_POINT('',#156628) ;
#39573=VERTEX_POINT('',#156631) ;
#39574=VERTEX_POINT('',#156632) ;
#39575=VERTEX_POINT('',#156634) ;
#39576=VERTEX_POINT('',#156636) ;
#39577=VERTEX_POINT('',#156639) ;
#39578=VERTEX_POINT('',#156640) ;
#39579=VERTEX_POINT('',#156642) ;
#39580=VERTEX_POINT('',#156644) ;
#39581=VERTEX_POINT('',#156647) ;
#39582=VERTEX_POINT('',#156648) ;
#39583=VERTEX_POINT('',#156650) ;
#39584=VERTEX_POINT('',#156652) ;
#39585=VERTEX_POINT('',#156655) ;
#39586=VERTEX_POINT('',#156656) ;
#39587=VERTEX_POINT('',#156658) ;
#39588=VERTEX_POINT('',#156660) ;
#39589=VERTEX_POINT('',#156663) ;
#39590=VERTEX_POINT('',#156664) ;
#39591=VERTEX_POINT('',#156666) ;
#39592=VERTEX_POINT('',#156668) ;
#39593=VERTEX_POINT('',#156670) ;
#39594=VERTEX_POINT('',#156672) ;
#39595=VERTEX_POINT('',#156674) ;
#39596=VERTEX_POINT('',#156676) ;
#39597=VERTEX_POINT('',#156679) ;
#39598=VERTEX_POINT('',#156680) ;
#39599=VERTEX_POINT('',#156682) ;
#39600=VERTEX_POINT('',#156684) ;
#39601=VERTEX_POINT('',#156686) ;
#39602=VERTEX_POINT('',#156688) ;
#39603=VERTEX_POINT('',#156690) ;
#39604=VERTEX_POINT('',#156692) ;
#39605=VERTEX_POINT('',#156696) ;
#39606=VERTEX_POINT('',#156697) ;
#39607=VERTEX_POINT('',#156699) ;
#39608=VERTEX_POINT('',#156701) ;
#39609=VERTEX_POINT('',#156703) ;
#39610=VERTEX_POINT('',#156705) ;
#39611=VERTEX_POINT('',#156707) ;
#39612=VERTEX_POINT('',#156709) ;
#39613=VERTEX_POINT('',#156711) ;
#39614=VERTEX_POINT('',#156713) ;
#39615=VERTEX_POINT('',#156715) ;
#39616=VERTEX_POINT('',#156717) ;
#39617=VERTEX_POINT('',#156719) ;
#39618=VERTEX_POINT('',#156721) ;
#39619=VERTEX_POINT('',#156723) ;
#39620=VERTEX_POINT('',#156727) ;
#39621=VERTEX_POINT('',#156728) ;
#39622=VERTEX_POINT('',#156730) ;
#39623=VERTEX_POINT('',#156732) ;
#39624=VERTEX_POINT('',#156734) ;
#39625=VERTEX_POINT('',#156736) ;
#39626=VERTEX_POINT('',#156738) ;
#39627=VERTEX_POINT('',#156740) ;
#39628=VERTEX_POINT('',#156742) ;
#39629=VERTEX_POINT('',#156744) ;
#39630=VERTEX_POINT('',#156746) ;
#39631=VERTEX_POINT('',#156748) ;
#39632=VERTEX_POINT('',#156750) ;
#39633=VERTEX_POINT('',#156752) ;
#39634=VERTEX_POINT('',#156754) ;
#39635=VERTEX_POINT('',#156758) ;
#39636=VERTEX_POINT('',#156759) ;
#39637=VERTEX_POINT('',#156761) ;
#39638=VERTEX_POINT('',#156763) ;
#39639=VERTEX_POINT('',#156767) ;
#39640=VERTEX_POINT('',#156768) ;
#39641=VERTEX_POINT('',#156770) ;
#39642=VERTEX_POINT('',#156772) ;
#39643=VERTEX_POINT('',#156776) ;
#39644=VERTEX_POINT('',#156777) ;
#39645=VERTEX_POINT('',#156779) ;
#39646=VERTEX_POINT('',#156781) ;
#39647=VERTEX_POINT('',#156783) ;
#39648=VERTEX_POINT('',#156785) ;
#39649=VERTEX_POINT('',#156790) ;
#39650=VERTEX_POINT('',#156792) ;
#39651=VERTEX_POINT('',#156796) ;
#39652=VERTEX_POINT('',#156797) ;
#39653=VERTEX_POINT('',#156799) ;
#39654=VERTEX_POINT('',#156801) ;
#39655=VERTEX_POINT('',#156805) ;
#39656=VERTEX_POINT('',#156806) ;
#39657=VERTEX_POINT('',#156809) ;
#39658=VERTEX_POINT('',#156811) ;
#39659=VERTEX_POINT('',#156815) ;
#39660=VERTEX_POINT('',#156816) ;
#39661=VERTEX_POINT('',#156819) ;
#39662=VERTEX_POINT('',#156821) ;
#39663=VERTEX_POINT('',#156825) ;
#39664=VERTEX_POINT('',#156826) ;
#39665=VERTEX_POINT('',#156828) ;
#39666=VERTEX_POINT('',#156830) ;
#39667=VERTEX_POINT('',#156834) ;
#39668=VERTEX_POINT('',#156835) ;
#39669=VERTEX_POINT('',#156837) ;
#39670=VERTEX_POINT('',#156839) ;
#39671=VERTEX_POINT('',#156843) ;
#39672=VERTEX_POINT('',#156844) ;
#39673=VERTEX_POINT('',#156846) ;
#39674=VERTEX_POINT('',#156848) ;
#39675=VERTEX_POINT('',#156852) ;
#39676=VERTEX_POINT('',#156853) ;
#39677=VERTEX_POINT('',#156855) ;
#39678=VERTEX_POINT('',#156857) ;
#39679=VERTEX_POINT('',#156861) ;
#39680=VERTEX_POINT('',#156862) ;
#39681=VERTEX_POINT('',#156864) ;
#39682=VERTEX_POINT('',#156866) ;
#39683=VERTEX_POINT('',#156869) ;
#39684=VERTEX_POINT('',#156870) ;
#39685=VERTEX_POINT('',#156872) ;
#39686=VERTEX_POINT('',#156874) ;
#39687=VERTEX_POINT('',#156876) ;
#39688=VERTEX_POINT('',#156878) ;
#39689=VERTEX_POINT('',#156880) ;
#39690=VERTEX_POINT('',#156882) ;
#39691=VERTEX_POINT('',#156886) ;
#39692=VERTEX_POINT('',#156888) ;
#39693=VERTEX_POINT('',#156892) ;
#39694=VERTEX_POINT('',#156894) ;
#39695=VERTEX_POINT('',#156898) ;
#39696=VERTEX_POINT('',#156899) ;
#39697=VERTEX_POINT('',#156904) ;
#39698=VERTEX_POINT('',#156906) ;
#39699=VERTEX_POINT('',#156910) ;
#39700=VERTEX_POINT('',#156911) ;
#39701=VERTEX_POINT('',#156913) ;
#39702=VERTEX_POINT('',#156915) ;
#39703=VERTEX_POINT('',#156919) ;
#39704=VERTEX_POINT('',#156921) ;
#39705=VERTEX_POINT('',#156923) ;
#39706=VERTEX_POINT('',#156926) ;
#39707=VERTEX_POINT('',#156928) ;
#39708=VERTEX_POINT('',#156930) ;
#39709=VERTEX_POINT('',#156934) ;
#39710=VERTEX_POINT('',#156935) ;
#39711=VERTEX_POINT('',#156937) ;
#39712=VERTEX_POINT('',#156939) ;
#39713=VERTEX_POINT('',#156943) ;
#39714=VERTEX_POINT('',#156944) ;
#39715=VERTEX_POINT('',#156946) ;
#39716=VERTEX_POINT('',#156948) ;
#39717=VERTEX_POINT('',#156950) ;
#39718=VERTEX_POINT('',#156952) ;
#39719=VERTEX_POINT('',#156954) ;
#39720=VERTEX_POINT('',#156956) ;
#39721=VERTEX_POINT('',#156958) ;
#39722=VERTEX_POINT('',#156960) ;
#39723=VERTEX_POINT('',#156964) ;
#39724=VERTEX_POINT('',#156965) ;
#39725=VERTEX_POINT('',#156967) ;
#39726=VERTEX_POINT('',#156969) ;
#39727=VERTEX_POINT('',#156973) ;
#39728=VERTEX_POINT('',#156974) ;
#39729=VERTEX_POINT('',#156976) ;
#39730=VERTEX_POINT('',#156978) ;
#39731=VERTEX_POINT('',#156980) ;
#39732=VERTEX_POINT('',#156982) ;
#39733=VERTEX_POINT('',#156984) ;
#39734=VERTEX_POINT('',#156986) ;
#39735=VERTEX_POINT('',#156988) ;
#39736=VERTEX_POINT('',#156990) ;
#39737=VERTEX_POINT('',#156994) ;
#39738=VERTEX_POINT('',#156996) ;
#39739=VERTEX_POINT('',#157000) ;
#39740=VERTEX_POINT('',#157001) ;
#39741=VERTEX_POINT('',#157003) ;
#39742=VERTEX_POINT('',#157005) ;
#39743=VERTEX_POINT('',#157009) ;
#39744=VERTEX_POINT('',#157010) ;
#39745=VERTEX_POINT('',#157012) ;
#39746=VERTEX_POINT('',#157014) ;
#39747=VERTEX_POINT('',#157018) ;
#39748=VERTEX_POINT('',#157019) ;
#39749=VERTEX_POINT('',#157021) ;
#39750=VERTEX_POINT('',#157023) ;
#39751=VERTEX_POINT('',#157027) ;
#39752=VERTEX_POINT('',#157028) ;
#39753=VERTEX_POINT('',#157030) ;
#39754=VERTEX_POINT('',#157032) ;
#39755=VERTEX_POINT('',#157034) ;
#39756=VERTEX_POINT('',#157036) ;
#39757=VERTEX_POINT('',#157041) ;
#39758=VERTEX_POINT('',#157042) ;
#39759=VERTEX_POINT('',#157044) ;
#39760=VERTEX_POINT('',#157046) ;
#39761=VERTEX_POINT('',#157050) ;
#39762=VERTEX_POINT('',#157051) ;
#39763=VERTEX_POINT('',#157053) ;
#39764=VERTEX_POINT('',#157055) ;
#39765=VERTEX_POINT('',#157059) ;
#39766=VERTEX_POINT('',#157060) ;
#39767=VERTEX_POINT('',#157062) ;
#39768=VERTEX_POINT('',#157064) ;
#39769=VERTEX_POINT('',#157068) ;
#39770=VERTEX_POINT('',#157069) ;
#39771=VERTEX_POINT('',#157071) ;
#39772=VERTEX_POINT('',#157073) ;
#39773=VERTEX_POINT('',#157077) ;
#39774=VERTEX_POINT('',#157078) ;
#39775=VERTEX_POINT('',#157080) ;
#39776=VERTEX_POINT('',#157082) ;
#39777=VERTEX_POINT('',#157085) ;
#39778=VERTEX_POINT('',#157086) ;
#39779=VERTEX_POINT('',#157088) ;
#39780=VERTEX_POINT('',#157090) ;
#39781=VERTEX_POINT('',#157092) ;
#39782=VERTEX_POINT('',#157094) ;
#39783=VERTEX_POINT('',#157096) ;
#39784=VERTEX_POINT('',#157098) ;
#39785=VERTEX_POINT('',#157102) ;
#39786=VERTEX_POINT('',#157103) ;
#39787=VERTEX_POINT('',#157108) ;
#39788=VERTEX_POINT('',#157109) ;
#39789=VERTEX_POINT('',#157114) ;
#39790=VERTEX_POINT('',#157116) ;
#39791=VERTEX_POINT('',#157120) ;
#39792=VERTEX_POINT('',#157121) ;
#39793=VERTEX_POINT('',#157126) ;
#39794=VERTEX_POINT('',#157127) ;
#39795=VERTEX_POINT('',#157129) ;
#39796=VERTEX_POINT('',#157131) ;
#39797=VERTEX_POINT('',#157150) ;
#39798=VERTEX_POINT('',#157152) ;
#39799=VERTEX_POINT('',#157156) ;
#39800=VERTEX_POINT('',#157157) ;
#39801=VERTEX_POINT('',#157166) ;
#39802=VERTEX_POINT('',#157167) ;
#39803=VERTEX_POINT('',#157169) ;
#39804=VERTEX_POINT('',#157171) ;
#39805=VERTEX_POINT('',#157175) ;
#39806=VERTEX_POINT('',#157177) ;
#39807=VERTEX_POINT('',#157181) ;
#39808=VERTEX_POINT('',#157183) ;
#39809=VERTEX_POINT('',#157187) ;
#39810=VERTEX_POINT('',#157189) ;
#39811=VERTEX_POINT('',#157193) ;
#39812=VERTEX_POINT('',#157195) ;
#39813=VERTEX_POINT('',#157199) ;
#39814=VERTEX_POINT('',#157201) ;
#39815=VERTEX_POINT('',#157205) ;
#39816=VERTEX_POINT('',#157207) ;
#39817=VERTEX_POINT('',#157214) ;
#39818=VERTEX_POINT('',#157215) ;
#39819=VERTEX_POINT('',#157217) ;
#39820=VERTEX_POINT('',#157219) ;
#39821=VERTEX_POINT('',#157242) ;
#39822=VERTEX_POINT('',#157244) ;
#39823=VERTEX_POINT('',#157259) ;
#39824=VERTEX_POINT('',#157261) ;
#39825=VERTEX_POINT('',#157281) ;
#39826=VERTEX_POINT('',#157289) ;
#39827=VERTEX_POINT('',#157295) ;
#39828=VERTEX_POINT('',#157297) ;
#39829=VERTEX_POINT('',#157725) ;
#39830=VERTEX_POINT('',#157756) ;
#39831=VERTEX_POINT('',#157818) ;
#39832=VERTEX_POINT('',#157919) ;
#39833=VERTEX_POINT('',#157920) ;
#39834=VERTEX_POINT('',#157922) ;
#39835=VERTEX_POINT('',#157924) ;
#39836=VERTEX_POINT('',#157928) ;
#39837=VERTEX_POINT('',#157929) ;
#39838=VERTEX_POINT('',#157931) ;
#39839=VERTEX_POINT('',#157933) ;
#39840=VERTEX_POINT('',#157937) ;
#39841=VERTEX_POINT('',#157938) ;
#39842=VERTEX_POINT('',#157940) ;
#39843=VERTEX_POINT('',#157942) ;
#39844=VERTEX_POINT('',#157944) ;
#39845=VERTEX_POINT('',#157946) ;
#39846=VERTEX_POINT('',#157951) ;
#39847=VERTEX_POINT('',#157953) ;
#39848=VERTEX_POINT('',#157957) ;
#39849=VERTEX_POINT('',#157958) ;
#39850=VERTEX_POINT('',#157960) ;
#39851=VERTEX_POINT('',#157962) ;
#39852=VERTEX_POINT('',#157966) ;
#39853=VERTEX_POINT('',#157967) ;
#39854=VERTEX_POINT('',#157969) ;
#39855=VERTEX_POINT('',#157971) ;
#39856=VERTEX_POINT('',#157975) ;
#39857=VERTEX_POINT('',#157976) ;
#39858=VERTEX_POINT('',#157978) ;
#39859=VERTEX_POINT('',#157980) ;
#39860=VERTEX_POINT('',#157984) ;
#39861=VERTEX_POINT('',#157985) ;
#39862=VERTEX_POINT('',#157987) ;
#39863=VERTEX_POINT('',#157989) ;
#39864=VERTEX_POINT('',#157991) ;
#39865=VERTEX_POINT('',#157993) ;
#39866=VERTEX_POINT('',#157998) ;
#39867=VERTEX_POINT('',#158000) ;
#39868=VERTEX_POINT('',#158004) ;
#39869=VERTEX_POINT('',#158005) ;
#39870=VERTEX_POINT('',#158007) ;
#39871=VERTEX_POINT('',#158009) ;
#39872=VERTEX_POINT('',#158013) ;
#39873=VERTEX_POINT('',#158014) ;
#39874=VERTEX_POINT('',#158016) ;
#39875=VERTEX_POINT('',#158018) ;
#39876=VERTEX_POINT('',#158022) ;
#39877=VERTEX_POINT('',#158023) ;
#39878=VERTEX_POINT('',#158025) ;
#39879=VERTEX_POINT('',#158027) ;
#39880=VERTEX_POINT('',#158031) ;
#39881=VERTEX_POINT('',#158032) ;
#39882=VERTEX_POINT('',#158034) ;
#39883=VERTEX_POINT('',#158036) ;
#39884=VERTEX_POINT('',#158038) ;
#39885=VERTEX_POINT('',#158040) ;
#39886=VERTEX_POINT('',#158045) ;
#39887=VERTEX_POINT('',#158047) ;
#39888=VERTEX_POINT('',#158051) ;
#39889=VERTEX_POINT('',#158052) ;
#39890=VERTEX_POINT('',#158054) ;
#39891=VERTEX_POINT('',#158056) ;
#39892=VERTEX_POINT('',#158060) ;
#39893=VERTEX_POINT('',#158061) ;
#39894=VERTEX_POINT('',#158063) ;
#39895=VERTEX_POINT('',#158065) ;
#39896=VERTEX_POINT('',#158069) ;
#39897=VERTEX_POINT('',#158070) ;
#39898=VERTEX_POINT('',#158072) ;
#39899=VERTEX_POINT('',#158074) ;
#39900=VERTEX_POINT('',#158078) ;
#39901=VERTEX_POINT('',#158079) ;
#39902=VERTEX_POINT('',#158081) ;
#39903=VERTEX_POINT('',#158083) ;
#39904=VERTEX_POINT('',#158085) ;
#39905=VERTEX_POINT('',#158087) ;
#39906=VERTEX_POINT('',#158092) ;
#39907=VERTEX_POINT('',#158094) ;
#39908=VERTEX_POINT('',#158098) ;
#39909=VERTEX_POINT('',#158099) ;
#39910=VERTEX_POINT('',#158101) ;
#39911=VERTEX_POINT('',#158103) ;
#39912=VERTEX_POINT('',#158107) ;
#39913=VERTEX_POINT('',#158108) ;
#39914=VERTEX_POINT('',#158110) ;
#39915=VERTEX_POINT('',#158112) ;
#39916=VERTEX_POINT('',#158116) ;
#39917=VERTEX_POINT('',#158117) ;
#39918=VERTEX_POINT('',#158119) ;
#39919=VERTEX_POINT('',#158121) ;
#39920=VERTEX_POINT('',#158125) ;
#39921=VERTEX_POINT('',#158126) ;
#39922=VERTEX_POINT('',#158128) ;
#39923=VERTEX_POINT('',#158130) ;
#39924=VERTEX_POINT('',#158132) ;
#39925=VERTEX_POINT('',#158134) ;
#39926=VERTEX_POINT('',#158139) ;
#39927=VERTEX_POINT('',#158141) ;
#39928=VERTEX_POINT('',#158145) ;
#39929=VERTEX_POINT('',#158146) ;
#39930=VERTEX_POINT('',#158148) ;
#39931=VERTEX_POINT('',#158150) ;
#39932=VERTEX_POINT('',#158154) ;
#39933=VERTEX_POINT('',#158155) ;
#39934=VERTEX_POINT('',#158157) ;
#39935=VERTEX_POINT('',#158159) ;
#39936=VERTEX_POINT('',#158163) ;
#39937=VERTEX_POINT('',#158164) ;
#39938=VERTEX_POINT('',#158166) ;
#39939=VERTEX_POINT('',#158168) ;
#39940=VERTEX_POINT('',#158172) ;
#39941=VERTEX_POINT('',#158173) ;
#39942=VERTEX_POINT('',#158175) ;
#39943=VERTEX_POINT('',#158177) ;
#39944=VERTEX_POINT('',#158179) ;
#39945=VERTEX_POINT('',#158181) ;
#39946=VERTEX_POINT('',#158186) ;
#39947=VERTEX_POINT('',#158188) ;
#39948=VERTEX_POINT('',#158192) ;
#39949=VERTEX_POINT('',#158193) ;
#39950=VERTEX_POINT('',#158195) ;
#39951=VERTEX_POINT('',#158197) ;
#39952=VERTEX_POINT('',#158201) ;
#39953=VERTEX_POINT('',#158202) ;
#39954=VERTEX_POINT('',#158204) ;
#39955=VERTEX_POINT('',#158206) ;
#39956=VERTEX_POINT('',#158210) ;
#39957=VERTEX_POINT('',#158211) ;
#39958=VERTEX_POINT('',#158213) ;
#39959=VERTEX_POINT('',#158215) ;
#39960=VERTEX_POINT('',#158219) ;
#39961=VERTEX_POINT('',#158220) ;
#39962=VERTEX_POINT('',#158222) ;
#39963=VERTEX_POINT('',#158224) ;
#39964=VERTEX_POINT('',#158226) ;
#39965=VERTEX_POINT('',#158228) ;
#39966=VERTEX_POINT('',#158233) ;
#39967=VERTEX_POINT('',#158235) ;
#39968=VERTEX_POINT('',#158239) ;
#39969=VERTEX_POINT('',#158240) ;
#39970=VERTEX_POINT('',#158242) ;
#39971=VERTEX_POINT('',#158244) ;
#39972=VERTEX_POINT('',#158248) ;
#39973=VERTEX_POINT('',#158249) ;
#39974=VERTEX_POINT('',#158251) ;
#39975=VERTEX_POINT('',#158253) ;
#39976=VERTEX_POINT('',#158257) ;
#39977=VERTEX_POINT('',#158258) ;
#39978=VERTEX_POINT('',#158260) ;
#39979=VERTEX_POINT('',#158262) ;
#39980=VERTEX_POINT('',#158266) ;
#39981=VERTEX_POINT('',#158267) ;
#39982=VERTEX_POINT('',#158269) ;
#39983=VERTEX_POINT('',#158271) ;
#39984=VERTEX_POINT('',#158273) ;
#39985=VERTEX_POINT('',#158275) ;
#39986=VERTEX_POINT('',#158280) ;
#39987=VERTEX_POINT('',#158282) ;
#39988=VERTEX_POINT('',#158286) ;
#39989=VERTEX_POINT('',#158287) ;
#39990=VERTEX_POINT('',#158289) ;
#39991=VERTEX_POINT('',#158291) ;
#39992=VERTEX_POINT('',#158295) ;
#39993=VERTEX_POINT('',#158296) ;
#39994=VERTEX_POINT('',#158298) ;
#39995=VERTEX_POINT('',#158300) ;
#39996=VERTEX_POINT('',#158304) ;
#39997=VERTEX_POINT('',#158305) ;
#39998=VERTEX_POINT('',#158307) ;
#39999=VERTEX_POINT('',#158309) ;
#40000=VERTEX_POINT('',#158313) ;
#40001=VERTEX_POINT('',#158314) ;
#40002=VERTEX_POINT('',#158316) ;
#40003=VERTEX_POINT('',#158318) ;
#40004=VERTEX_POINT('',#158320) ;
#40005=VERTEX_POINT('',#158322) ;
#40006=VERTEX_POINT('',#158327) ;
#40007=VERTEX_POINT('',#158329) ;
#40008=VERTEX_POINT('',#158333) ;
#40009=VERTEX_POINT('',#158334) ;
#40010=VERTEX_POINT('',#158336) ;
#40011=VERTEX_POINT('',#158338) ;
#40012=VERTEX_POINT('',#158342) ;
#40013=VERTEX_POINT('',#158343) ;
#40014=VERTEX_POINT('',#158346) ;
#40015=VERTEX_POINT('',#158348) ;
#40016=VERTEX_POINT('',#158352) ;
#40017=VERTEX_POINT('',#158353) ;
#40018=VERTEX_POINT('',#158355) ;
#40019=VERTEX_POINT('',#158357) ;
#40020=VERTEX_POINT('',#158360) ;
#40021=VERTEX_POINT('',#158362) ;
#40022=VERTEX_POINT('',#158366) ;
#40023=VERTEX_POINT('',#158367) ;
#40024=VERTEX_POINT('',#158369) ;
#40025=VERTEX_POINT('',#158371) ;
#40026=VERTEX_POINT('',#158374) ;
#40027=VERTEX_POINT('',#158376) ;
#40028=VERTEX_POINT('',#158380) ;
#40029=VERTEX_POINT('',#158381) ;
#40030=VERTEX_POINT('',#158383) ;
#40031=VERTEX_POINT('',#158385) ;
#40032=VERTEX_POINT('',#158388) ;
#40033=VERTEX_POINT('',#158390) ;
#40034=VERTEX_POINT('',#158394) ;
#40035=VERTEX_POINT('',#158395) ;
#40036=VERTEX_POINT('',#158397) ;
#40037=VERTEX_POINT('',#158399) ;
#40038=VERTEX_POINT('',#158402) ;
#40039=VERTEX_POINT('',#158404) ;
#40040=VERTEX_POINT('',#158408) ;
#40041=VERTEX_POINT('',#158409) ;
#40042=VERTEX_POINT('',#158411) ;
#40043=VERTEX_POINT('',#158413) ;
#40044=VERTEX_POINT('',#158416) ;
#40045=VERTEX_POINT('',#158418) ;
#40046=VERTEX_POINT('',#158422) ;
#40047=VERTEX_POINT('',#158423) ;
#40048=VERTEX_POINT('',#158425) ;
#40049=VERTEX_POINT('',#158427) ;
#40050=VERTEX_POINT('',#158430) ;
#40051=VERTEX_POINT('',#158432) ;
#40052=VERTEX_POINT('',#158436) ;
#40053=VERTEX_POINT('',#158437) ;
#40054=VERTEX_POINT('',#158439) ;
#40055=VERTEX_POINT('',#158441) ;
#40056=VERTEX_POINT('',#158444) ;
#40057=VERTEX_POINT('',#158446) ;
#40058=VERTEX_POINT('',#158450) ;
#40059=VERTEX_POINT('',#158451) ;
#40060=VERTEX_POINT('',#158453) ;
#40061=VERTEX_POINT('',#158455) ;
#40062=VERTEX_POINT('',#158458) ;
#40063=VERTEX_POINT('',#158460) ;
#40064=VERTEX_POINT('',#158464) ;
#40065=VERTEX_POINT('',#158465) ;
#40066=VERTEX_POINT('',#158468) ;
#40067=VERTEX_POINT('',#158470) ;
#40068=VERTEX_POINT('',#158474) ;
#40069=VERTEX_POINT('',#158475) ;
#40070=VERTEX_POINT('',#158477) ;
#40071=VERTEX_POINT('',#158479) ;
#40072=VERTEX_POINT('',#158482) ;
#40073=VERTEX_POINT('',#158484) ;
#40074=VERTEX_POINT('',#158488) ;
#40075=VERTEX_POINT('',#158489) ;
#40076=VERTEX_POINT('',#158491) ;
#40077=VERTEX_POINT('',#158493) ;
#40078=VERTEX_POINT('',#158496) ;
#40079=VERTEX_POINT('',#158498) ;
#40080=VERTEX_POINT('',#158502) ;
#40081=VERTEX_POINT('',#158503) ;
#40082=VERTEX_POINT('',#158505) ;
#40083=VERTEX_POINT('',#158507) ;
#40084=VERTEX_POINT('',#158510) ;
#40085=VERTEX_POINT('',#158512) ;
#40086=VERTEX_POINT('',#158516) ;
#40087=VERTEX_POINT('',#158517) ;
#40088=VERTEX_POINT('',#158519) ;
#40089=VERTEX_POINT('',#158521) ;
#40090=VERTEX_POINT('',#158524) ;
#40091=VERTEX_POINT('',#158526) ;
#40092=VERTEX_POINT('',#158530) ;
#40093=VERTEX_POINT('',#158531) ;
#40094=VERTEX_POINT('',#158533) ;
#40095=VERTEX_POINT('',#158535) ;
#40096=VERTEX_POINT('',#158538) ;
#40097=VERTEX_POINT('',#158540) ;
#40098=VERTEX_POINT('',#158544) ;
#40099=VERTEX_POINT('',#158545) ;
#40100=VERTEX_POINT('',#158547) ;
#40101=VERTEX_POINT('',#158549) ;
#40102=VERTEX_POINT('',#158552) ;
#40103=VERTEX_POINT('',#158554) ;
#40104=VERTEX_POINT('',#158558) ;
#40105=VERTEX_POINT('',#158559) ;
#40106=VERTEX_POINT('',#158561) ;
#40107=VERTEX_POINT('',#158563) ;
#40108=VERTEX_POINT('',#158566) ;
#40109=VERTEX_POINT('',#158568) ;
#40110=VERTEX_POINT('',#158572) ;
#40111=VERTEX_POINT('',#158573) ;
#40112=VERTEX_POINT('',#158575) ;
#40113=VERTEX_POINT('',#158577) ;
#40114=VERTEX_POINT('',#158580) ;
#40115=VERTEX_POINT('',#158582) ;
#40116=VERTEX_POINT('',#158586) ;
#40117=VERTEX_POINT('',#158587) ;
#40118=VERTEX_POINT('',#158589) ;
#40119=VERTEX_POINT('',#158591) ;
#40120=VERTEX_POINT('',#158595) ;
#40121=VERTEX_POINT('',#158596) ;
#40122=VERTEX_POINT('',#158598) ;
#40123=VERTEX_POINT('',#158600) ;
#40124=VERTEX_POINT('',#158604) ;
#40125=VERTEX_POINT('',#158605) ;
#40126=VERTEX_POINT('',#158607) ;
#40127=VERTEX_POINT('',#158609) ;
#40128=VERTEX_POINT('',#158613) ;
#40129=VERTEX_POINT('',#158614) ;
#40130=VERTEX_POINT('',#158616) ;
#40131=VERTEX_POINT('',#158618) ;
#40132=VERTEX_POINT('',#158622) ;
#40133=VERTEX_POINT('',#158623) ;
#40134=VERTEX_POINT('',#158625) ;
#40135=VERTEX_POINT('',#158627) ;
#40136=VERTEX_POINT('',#158631) ;
#40137=VERTEX_POINT('',#158632) ;
#40138=VERTEX_POINT('',#158634) ;
#40139=VERTEX_POINT('',#158636) ;
#40140=VERTEX_POINT('',#158640) ;
#40141=VERTEX_POINT('',#158641) ;
#40142=VERTEX_POINT('',#158643) ;
#40143=VERTEX_POINT('',#158645) ;
#40144=VERTEX_POINT('',#158649) ;
#40145=VERTEX_POINT('',#158650) ;
#40146=VERTEX_POINT('',#158652) ;
#40147=VERTEX_POINT('',#158654) ;
#40148=VERTEX_POINT('',#158658) ;
#40149=VERTEX_POINT('',#158659) ;
#40150=VERTEX_POINT('',#158661) ;
#40151=VERTEX_POINT('',#158663) ;
#40152=VERTEX_POINT('',#158667) ;
#40153=VERTEX_POINT('',#158668) ;
#40154=VERTEX_POINT('',#158670) ;
#40155=VERTEX_POINT('',#158672) ;
#40156=VERTEX_POINT('',#158676) ;
#40157=VERTEX_POINT('',#158677) ;
#40158=VERTEX_POINT('',#158679) ;
#40159=VERTEX_POINT('',#158681) ;
#40160=VERTEX_POINT('',#158685) ;
#40161=VERTEX_POINT('',#158686) ;
#40162=VERTEX_POINT('',#158688) ;
#40163=VERTEX_POINT('',#158690) ;
#40164=VERTEX_POINT('',#158694) ;
#40165=VERTEX_POINT('',#158695) ;
#40166=VERTEX_POINT('',#158697) ;
#40167=VERTEX_POINT('',#158699) ;
#40168=VERTEX_POINT('',#158703) ;
#40169=VERTEX_POINT('',#158704) ;
#40170=VERTEX_POINT('',#158706) ;
#40171=VERTEX_POINT('',#158708) ;
#40172=VERTEX_POINT('',#158712) ;
#40173=VERTEX_POINT('',#158713) ;
#40174=VERTEX_POINT('',#158715) ;
#40175=VERTEX_POINT('',#158717) ;
#40176=VERTEX_POINT('',#158721) ;
#40177=VERTEX_POINT('',#158722) ;
#40178=VERTEX_POINT('',#158724) ;
#40179=VERTEX_POINT('',#158726) ;
#40180=VERTEX_POINT('',#158730) ;
#40181=VERTEX_POINT('',#158731) ;
#40182=VERTEX_POINT('',#158733) ;
#40183=VERTEX_POINT('',#158735) ;
#40184=VERTEX_POINT('',#158739) ;
#40185=VERTEX_POINT('',#158740) ;
#40186=VERTEX_POINT('',#158742) ;
#40187=VERTEX_POINT('',#158744) ;
#40188=VERTEX_POINT('',#158748) ;
#40189=VERTEX_POINT('',#158749) ;
#40190=VERTEX_POINT('',#158751) ;
#40191=VERTEX_POINT('',#158753) ;
#40192=VERTEX_POINT('',#158757) ;
#40193=VERTEX_POINT('',#158758) ;
#40194=VERTEX_POINT('',#158760) ;
#40195=VERTEX_POINT('',#158762) ;
#40196=VERTEX_POINT('',#158766) ;
#40197=VERTEX_POINT('',#158767) ;
#40198=VERTEX_POINT('',#158769) ;
#40199=VERTEX_POINT('',#158771) ;
#40200=VERTEX_POINT('',#158775) ;
#40201=VERTEX_POINT('',#158776) ;
#40202=VERTEX_POINT('',#158778) ;
#40203=VERTEX_POINT('',#158780) ;
#40204=VERTEX_POINT('',#158784) ;
#40205=VERTEX_POINT('',#158785) ;
#40206=VERTEX_POINT('',#158787) ;
#40207=VERTEX_POINT('',#158789) ;
#40208=VERTEX_POINT('',#158793) ;
#40209=VERTEX_POINT('',#158794) ;
#40210=VERTEX_POINT('',#158796) ;
#40211=VERTEX_POINT('',#158798) ;
#40212=VERTEX_POINT('',#158802) ;
#40213=VERTEX_POINT('',#158803) ;
#40214=VERTEX_POINT('',#158805) ;
#40215=VERTEX_POINT('',#158807) ;
#40216=VERTEX_POINT('',#158811) ;
#40217=VERTEX_POINT('',#158812) ;
#40218=VERTEX_POINT('',#158814) ;
#40219=VERTEX_POINT('',#158816) ;
#40220=VERTEX_POINT('',#158820) ;
#40221=VERTEX_POINT('',#158821) ;
#40222=VERTEX_POINT('',#158823) ;
#40223=VERTEX_POINT('',#158825) ;
#40224=VERTEX_POINT('',#158829) ;
#40225=VERTEX_POINT('',#158830) ;
#40226=VERTEX_POINT('',#158832) ;
#40227=VERTEX_POINT('',#158834) ;
#40228=VERTEX_POINT('',#158838) ;
#40229=VERTEX_POINT('',#158839) ;
#40230=VERTEX_POINT('',#158841) ;
#40231=VERTEX_POINT('',#158843) ;
#40232=VERTEX_POINT('',#158847) ;
#40233=VERTEX_POINT('',#158848) ;
#40234=VERTEX_POINT('',#158850) ;
#40235=VERTEX_POINT('',#158852) ;
#40236=VERTEX_POINT('',#158856) ;
#40237=VERTEX_POINT('',#158857) ;
#40238=VERTEX_POINT('',#158859) ;
#40239=VERTEX_POINT('',#158861) ;
#40240=VERTEX_POINT('',#158865) ;
#40241=VERTEX_POINT('',#158866) ;
#40242=VERTEX_POINT('',#158868) ;
#40243=VERTEX_POINT('',#158870) ;
#40244=VERTEX_POINT('',#158874) ;
#40245=VERTEX_POINT('',#158875) ;
#40246=VERTEX_POINT('',#158877) ;
#40247=VERTEX_POINT('',#158879) ;
#40248=VERTEX_POINT('',#158883) ;
#40249=VERTEX_POINT('',#158884) ;
#40250=VERTEX_POINT('',#158886) ;
#40251=VERTEX_POINT('',#158888) ;
#40252=VERTEX_POINT('',#158892) ;
#40253=VERTEX_POINT('',#158893) ;
#40254=VERTEX_POINT('',#158895) ;
#40255=VERTEX_POINT('',#158897) ;
#40256=VERTEX_POINT('',#158901) ;
#40257=VERTEX_POINT('',#158902) ;
#40258=VERTEX_POINT('',#158904) ;
#40259=VERTEX_POINT('',#158906) ;
#40260=VERTEX_POINT('',#158910) ;
#40261=VERTEX_POINT('',#158911) ;
#40262=VERTEX_POINT('',#158913) ;
#40263=VERTEX_POINT('',#158915) ;
#40264=VERTEX_POINT('',#158918) ;
#40265=VERTEX_POINT('',#158919) ;
#40266=VERTEX_POINT('',#158921) ;
#40267=VERTEX_POINT('',#158923) ;
#40268=VERTEX_POINT('',#158925) ;
#40269=VERTEX_POINT('',#158927) ;
#40270=VERTEX_POINT('',#158929) ;
#40271=VERTEX_POINT('',#158931) ;
#40272=VERTEX_POINT('',#158935) ;
#40273=VERTEX_POINT('',#158937) ;
#40274=VERTEX_POINT('',#158941) ;
#40275=VERTEX_POINT('',#158943) ;
#40276=VERTEX_POINT('',#158947) ;
#40277=VERTEX_POINT('',#158948) ;
#40278=VERTEX_POINT('',#158953) ;
#40279=VERTEX_POINT('',#158955) ;
#40280=VERTEX_POINT('',#158959) ;
#40281=VERTEX_POINT('',#158960) ;
#40282=VERTEX_POINT('',#158962) ;
#40283=VERTEX_POINT('',#158964) ;
#40284=VERTEX_POINT('',#158967) ;
#40285=VERTEX_POINT('',#158968) ;
#40286=VERTEX_POINT('',#158970) ;
#40287=VERTEX_POINT('',#158972) ;
#40288=VERTEX_POINT('',#158974) ;
#40289=VERTEX_POINT('',#158976) ;
#40290=VERTEX_POINT('',#158978) ;
#40291=VERTEX_POINT('',#158980) ;
#40292=VERTEX_POINT('',#158984) ;
#40293=VERTEX_POINT('',#158986) ;
#40294=VERTEX_POINT('',#158990) ;
#40295=VERTEX_POINT('',#158992) ;
#40296=VERTEX_POINT('',#158996) ;
#40297=VERTEX_POINT('',#158997) ;
#40298=VERTEX_POINT('',#159002) ;
#40299=VERTEX_POINT('',#159004) ;
#40300=VERTEX_POINT('',#159008) ;
#40301=VERTEX_POINT('',#159009) ;
#40302=VERTEX_POINT('',#159011) ;
#40303=VERTEX_POINT('',#159013) ;
#40304=VERTEX_POINT('',#159016) ;
#40305=VERTEX_POINT('',#159017) ;
#40306=VERTEX_POINT('',#159019) ;
#40307=VERTEX_POINT('',#159021) ;
#40308=VERTEX_POINT('',#159023) ;
#40309=VERTEX_POINT('',#159025) ;
#40310=VERTEX_POINT('',#159027) ;
#40311=VERTEX_POINT('',#159029) ;
#40312=VERTEX_POINT('',#159033) ;
#40313=VERTEX_POINT('',#159035) ;
#40314=VERTEX_POINT('',#159039) ;
#40315=VERTEX_POINT('',#159041) ;
#40316=VERTEX_POINT('',#159045) ;
#40317=VERTEX_POINT('',#159046) ;
#40318=VERTEX_POINT('',#159051) ;
#40319=VERTEX_POINT('',#159053) ;
#40320=VERTEX_POINT('',#159057) ;
#40321=VERTEX_POINT('',#159058) ;
#40322=VERTEX_POINT('',#159060) ;
#40323=VERTEX_POINT('',#159062) ;
#40324=VERTEX_POINT('',#159065) ;
#40325=VERTEX_POINT('',#159066) ;
#40326=VERTEX_POINT('',#159068) ;
#40327=VERTEX_POINT('',#159070) ;
#40328=VERTEX_POINT('',#159072) ;
#40329=VERTEX_POINT('',#159074) ;
#40330=VERTEX_POINT('',#159076) ;
#40331=VERTEX_POINT('',#159078) ;
#40332=VERTEX_POINT('',#159082) ;
#40333=VERTEX_POINT('',#159084) ;
#40334=VERTEX_POINT('',#159088) ;
#40335=VERTEX_POINT('',#159090) ;
#40336=VERTEX_POINT('',#159094) ;
#40337=VERTEX_POINT('',#159095) ;
#40338=VERTEX_POINT('',#159100) ;
#40339=VERTEX_POINT('',#159102) ;
#40340=VERTEX_POINT('',#159106) ;
#40341=VERTEX_POINT('',#159107) ;
#40342=VERTEX_POINT('',#159109) ;
#40343=VERTEX_POINT('',#159111) ;
#40344=VERTEX_POINT('',#159114) ;
#40345=VERTEX_POINT('',#159115) ;
#40346=VERTEX_POINT('',#159117) ;
#40347=VERTEX_POINT('',#159119) ;
#40348=VERTEX_POINT('',#159121) ;
#40349=VERTEX_POINT('',#159123) ;
#40350=VERTEX_POINT('',#159125) ;
#40351=VERTEX_POINT('',#159127) ;
#40352=VERTEX_POINT('',#159131) ;
#40353=VERTEX_POINT('',#159133) ;
#40354=VERTEX_POINT('',#159137) ;
#40355=VERTEX_POINT('',#159139) ;
#40356=VERTEX_POINT('',#159143) ;
#40357=VERTEX_POINT('',#159144) ;
#40358=VERTEX_POINT('',#159149) ;
#40359=VERTEX_POINT('',#159151) ;
#40360=VERTEX_POINT('',#159155) ;
#40361=VERTEX_POINT('',#159156) ;
#40362=VERTEX_POINT('',#159158) ;
#40363=VERTEX_POINT('',#159160) ;
#40364=VERTEX_POINT('',#159163) ;
#40365=VERTEX_POINT('',#159164) ;
#40366=VERTEX_POINT('',#159166) ;
#40367=VERTEX_POINT('',#159168) ;
#40368=VERTEX_POINT('',#159170) ;
#40369=VERTEX_POINT('',#159172) ;
#40370=VERTEX_POINT('',#159174) ;
#40371=VERTEX_POINT('',#159176) ;
#40372=VERTEX_POINT('',#159180) ;
#40373=VERTEX_POINT('',#159182) ;
#40374=VERTEX_POINT('',#159186) ;
#40375=VERTEX_POINT('',#159188) ;
#40376=VERTEX_POINT('',#159192) ;
#40377=VERTEX_POINT('',#159193) ;
#40378=VERTEX_POINT('',#159198) ;
#40379=VERTEX_POINT('',#159200) ;
#40380=VERTEX_POINT('',#159204) ;
#40381=VERTEX_POINT('',#159205) ;
#40382=VERTEX_POINT('',#159207) ;
#40383=VERTEX_POINT('',#159209) ;
#40384=VERTEX_POINT('',#159212) ;
#40385=VERTEX_POINT('',#159213) ;
#40386=VERTEX_POINT('',#159215) ;
#40387=VERTEX_POINT('',#159217) ;
#40388=VERTEX_POINT('',#159219) ;
#40389=VERTEX_POINT('',#159221) ;
#40390=VERTEX_POINT('',#159223) ;
#40391=VERTEX_POINT('',#159225) ;
#40392=VERTEX_POINT('',#159229) ;
#40393=VERTEX_POINT('',#159231) ;
#40394=VERTEX_POINT('',#159235) ;
#40395=VERTEX_POINT('',#159237) ;
#40396=VERTEX_POINT('',#159241) ;
#40397=VERTEX_POINT('',#159242) ;
#40398=VERTEX_POINT('',#159247) ;
#40399=VERTEX_POINT('',#159249) ;
#40400=VERTEX_POINT('',#159253) ;
#40401=VERTEX_POINT('',#159254) ;
#40402=VERTEX_POINT('',#159256) ;
#40403=VERTEX_POINT('',#159258) ;
#40404=VERTEX_POINT('',#159261) ;
#40405=VERTEX_POINT('',#159262) ;
#40406=VERTEX_POINT('',#159264) ;
#40407=VERTEX_POINT('',#159266) ;
#40408=VERTEX_POINT('',#159268) ;
#40409=VERTEX_POINT('',#159270) ;
#40410=VERTEX_POINT('',#159272) ;
#40411=VERTEX_POINT('',#159274) ;
#40412=VERTEX_POINT('',#159278) ;
#40413=VERTEX_POINT('',#159280) ;
#40414=VERTEX_POINT('',#159284) ;
#40415=VERTEX_POINT('',#159286) ;
#40416=VERTEX_POINT('',#159290) ;
#40417=VERTEX_POINT('',#159291) ;
#40418=VERTEX_POINT('',#159296) ;
#40419=VERTEX_POINT('',#159298) ;
#40420=VERTEX_POINT('',#159302) ;
#40421=VERTEX_POINT('',#159303) ;
#40422=VERTEX_POINT('',#159305) ;
#40423=VERTEX_POINT('',#159307) ;
#40424=VERTEX_POINT('',#159310) ;
#40425=VERTEX_POINT('',#159311) ;
#40426=VERTEX_POINT('',#159313) ;
#40427=VERTEX_POINT('',#159315) ;
#40428=VERTEX_POINT('',#159317) ;
#40429=VERTEX_POINT('',#159319) ;
#40430=VERTEX_POINT('',#159321) ;
#40431=VERTEX_POINT('',#159323) ;
#40432=VERTEX_POINT('',#159327) ;
#40433=VERTEX_POINT('',#159329) ;
#40434=VERTEX_POINT('',#159333) ;
#40435=VERTEX_POINT('',#159335) ;
#40436=VERTEX_POINT('',#159339) ;
#40437=VERTEX_POINT('',#159340) ;
#40438=VERTEX_POINT('',#159345) ;
#40439=VERTEX_POINT('',#159347) ;
#40440=VERTEX_POINT('',#159351) ;
#40441=VERTEX_POINT('',#159352) ;
#40442=VERTEX_POINT('',#159354) ;
#40443=VERTEX_POINT('',#159356) ;
#40444=VERTEX_POINT('',#159360) ;
#40445=VERTEX_POINT('',#159361) ;
#40446=VERTEX_POINT('',#159363) ;
#40447=VERTEX_POINT('',#159365) ;
#40448=VERTEX_POINT('',#159369) ;
#40449=VERTEX_POINT('',#159370) ;
#40450=VERTEX_POINT('',#159372) ;
#40451=VERTEX_POINT('',#159374) ;
#40452=VERTEX_POINT('',#159378) ;
#40453=VERTEX_POINT('',#159379) ;
#40454=VERTEX_POINT('',#159381) ;
#40455=VERTEX_POINT('',#159383) ;
#40456=VERTEX_POINT('',#159387) ;
#40457=VERTEX_POINT('',#159388) ;
#40458=VERTEX_POINT('',#159390) ;
#40459=VERTEX_POINT('',#159392) ;
#40460=VERTEX_POINT('',#159396) ;
#40461=VERTEX_POINT('',#159397) ;
#40462=VERTEX_POINT('',#159399) ;
#40463=VERTEX_POINT('',#159401) ;
#40464=VERTEX_POINT('',#159405) ;
#40465=VERTEX_POINT('',#159406) ;
#40466=VERTEX_POINT('',#159408) ;
#40467=VERTEX_POINT('',#159410) ;
#40468=VERTEX_POINT('',#159414) ;
#40469=VERTEX_POINT('',#159415) ;
#40470=VERTEX_POINT('',#159417) ;
#40471=VERTEX_POINT('',#159419) ;
#40472=VERTEX_POINT('',#159423) ;
#40473=VERTEX_POINT('',#159424) ;
#40474=VERTEX_POINT('',#159426) ;
#40475=VERTEX_POINT('',#159428) ;
#40476=VERTEX_POINT('',#159432) ;
#40477=VERTEX_POINT('',#159433) ;
#40478=VERTEX_POINT('',#159435) ;
#40479=VERTEX_POINT('',#159437) ;
#40480=VERTEX_POINT('',#159439) ;
#40481=VERTEX_POINT('',#159441) ;
#40482=VERTEX_POINT('',#159443) ;
#40483=VERTEX_POINT('',#159445) ;
#40484=VERTEX_POINT('',#159447) ;
#40485=VERTEX_POINT('',#159449) ;
#40486=VERTEX_POINT('',#159453) ;
#40487=VERTEX_POINT('',#159454) ;
#40488=VERTEX_POINT('',#159456) ;
#40489=VERTEX_POINT('',#159458) ;
#40490=VERTEX_POINT('',#159462) ;
#40491=VERTEX_POINT('',#159463) ;
#40492=VERTEX_POINT('',#159465) ;
#40493=VERTEX_POINT('',#159467) ;
#40494=VERTEX_POINT('',#159469) ;
#40495=VERTEX_POINT('',#159471) ;
#40496=VERTEX_POINT('',#159473) ;
#40497=VERTEX_POINT('',#159475) ;
#40498=VERTEX_POINT('',#159477) ;
#40499=VERTEX_POINT('',#159479) ;
#40500=VERTEX_POINT('',#159483) ;
#40501=VERTEX_POINT('',#159484) ;
#40502=VERTEX_POINT('',#159486) ;
#40503=VERTEX_POINT('',#159488) ;
#40504=VERTEX_POINT('',#159492) ;
#40505=VERTEX_POINT('',#159493) ;
#40506=VERTEX_POINT('',#159495) ;
#40507=VERTEX_POINT('',#159497) ;
#40508=VERTEX_POINT('',#159499) ;
#40509=VERTEX_POINT('',#159501) ;
#40510=VERTEX_POINT('',#159503) ;
#40511=VERTEX_POINT('',#159505) ;
#40512=VERTEX_POINT('',#159507) ;
#40513=VERTEX_POINT('',#159509) ;
#40514=VERTEX_POINT('',#159513) ;
#40515=VERTEX_POINT('',#159514) ;
#40516=VERTEX_POINT('',#159516) ;
#40517=VERTEX_POINT('',#159518) ;
#40518=VERTEX_POINT('',#159522) ;
#40519=VERTEX_POINT('',#159523) ;
#40520=VERTEX_POINT('',#159525) ;
#40521=VERTEX_POINT('',#159527) ;
#40522=VERTEX_POINT('',#159529) ;
#40523=VERTEX_POINT('',#159531) ;
#40524=VERTEX_POINT('',#159533) ;
#40525=VERTEX_POINT('',#159535) ;
#40526=VERTEX_POINT('',#159537) ;
#40527=VERTEX_POINT('',#159539) ;
#40528=VERTEX_POINT('',#159543) ;
#40529=VERTEX_POINT('',#159544) ;
#40530=VERTEX_POINT('',#159546) ;
#40531=VERTEX_POINT('',#159548) ;
#40532=VERTEX_POINT('',#159552) ;
#40533=VERTEX_POINT('',#159553) ;
#40534=VERTEX_POINT('',#159555) ;
#40535=VERTEX_POINT('',#159557) ;
#40536=VERTEX_POINT('',#159559) ;
#40537=VERTEX_POINT('',#159561) ;
#40538=VERTEX_POINT('',#159563) ;
#40539=VERTEX_POINT('',#159565) ;
#40540=VERTEX_POINT('',#159567) ;
#40541=VERTEX_POINT('',#159569) ;
#40542=VERTEX_POINT('',#159573) ;
#40543=VERTEX_POINT('',#159574) ;
#40544=VERTEX_POINT('',#159576) ;
#40545=VERTEX_POINT('',#159578) ;
#40546=VERTEX_POINT('',#159582) ;
#40547=VERTEX_POINT('',#159583) ;
#40548=VERTEX_POINT('',#159585) ;
#40549=VERTEX_POINT('',#159587) ;
#40550=VERTEX_POINT('',#159589) ;
#40551=VERTEX_POINT('',#159591) ;
#40552=VERTEX_POINT('',#159593) ;
#40553=VERTEX_POINT('',#159595) ;
#40554=VERTEX_POINT('',#159597) ;
#40555=VERTEX_POINT('',#159599) ;
#40556=VERTEX_POINT('',#159603) ;
#40557=VERTEX_POINT('',#159604) ;
#40558=VERTEX_POINT('',#159606) ;
#40559=VERTEX_POINT('',#159608) ;
#40560=VERTEX_POINT('',#159612) ;
#40561=VERTEX_POINT('',#159613) ;
#40562=VERTEX_POINT('',#159615) ;
#40563=VERTEX_POINT('',#159617) ;
#40564=VERTEX_POINT('',#159619) ;
#40565=VERTEX_POINT('',#159621) ;
#40566=VERTEX_POINT('',#159623) ;
#40567=VERTEX_POINT('',#159625) ;
#40568=VERTEX_POINT('',#159627) ;
#40569=VERTEX_POINT('',#159629) ;
#40570=VERTEX_POINT('',#159633) ;
#40571=VERTEX_POINT('',#159634) ;
#40572=VERTEX_POINT('',#159636) ;
#40573=VERTEX_POINT('',#159638) ;
#40574=VERTEX_POINT('',#159642) ;
#40575=VERTEX_POINT('',#159643) ;
#40576=VERTEX_POINT('',#159645) ;
#40577=VERTEX_POINT('',#159647) ;
#40578=VERTEX_POINT('',#159649) ;
#40579=VERTEX_POINT('',#159651) ;
#40580=VERTEX_POINT('',#159653) ;
#40581=VERTEX_POINT('',#159655) ;
#40582=VERTEX_POINT('',#159657) ;
#40583=VERTEX_POINT('',#159659) ;
#40584=VERTEX_POINT('',#159663) ;
#40585=VERTEX_POINT('',#159664) ;
#40586=VERTEX_POINT('',#159666) ;
#40587=VERTEX_POINT('',#159668) ;
#40588=VERTEX_POINT('',#159672) ;
#40589=VERTEX_POINT('',#159673) ;
#40590=VERTEX_POINT('',#159675) ;
#40591=VERTEX_POINT('',#159677) ;
#40592=VERTEX_POINT('',#159679) ;
#40593=VERTEX_POINT('',#159681) ;
#40594=VERTEX_POINT('',#159683) ;
#40595=VERTEX_POINT('',#159685) ;
#40596=VERTEX_POINT('',#159687) ;
#40597=VERTEX_POINT('',#159689) ;
#40598=VERTEX_POINT('',#159693) ;
#40599=VERTEX_POINT('',#159694) ;
#40600=VERTEX_POINT('',#159696) ;
#40601=VERTEX_POINT('',#159698) ;
#40602=VERTEX_POINT('',#159702) ;
#40603=VERTEX_POINT('',#159703) ;
#40604=VERTEX_POINT('',#159705) ;
#40605=VERTEX_POINT('',#159707) ;
#40606=VERTEX_POINT('',#159709) ;
#40607=VERTEX_POINT('',#159711) ;
#40608=VERTEX_POINT('',#159713) ;
#40609=VERTEX_POINT('',#159715) ;
#40610=VERTEX_POINT('',#159717) ;
#40611=VERTEX_POINT('',#159719) ;
#40612=VERTEX_POINT('',#159723) ;
#40613=VERTEX_POINT('',#159724) ;
#40614=VERTEX_POINT('',#159726) ;
#40615=VERTEX_POINT('',#159728) ;
#40616=VERTEX_POINT('',#159732) ;
#40617=VERTEX_POINT('',#159733) ;
#40618=VERTEX_POINT('',#159735) ;
#40619=VERTEX_POINT('',#159737) ;
#40620=VERTEX_POINT('',#159739) ;
#40621=VERTEX_POINT('',#159741) ;
#40622=VERTEX_POINT('',#159743) ;
#40623=VERTEX_POINT('',#159745) ;
#40624=VERTEX_POINT('',#159747) ;
#40625=VERTEX_POINT('',#159749) ;
#40626=VERTEX_POINT('',#159753) ;
#40627=VERTEX_POINT('',#159754) ;
#40628=VERTEX_POINT('',#159756) ;
#40629=VERTEX_POINT('',#159758) ;
#40630=VERTEX_POINT('',#159762) ;
#40631=VERTEX_POINT('',#159763) ;
#40632=VERTEX_POINT('',#159765) ;
#40633=VERTEX_POINT('',#159767) ;
#40634=VERTEX_POINT('',#159769) ;
#40635=VERTEX_POINT('',#159771) ;
#40636=VERTEX_POINT('',#159773) ;
#40637=VERTEX_POINT('',#159775) ;
#40638=VERTEX_POINT('',#159777) ;
#40639=VERTEX_POINT('',#159779) ;
#40640=VERTEX_POINT('',#159783) ;
#40641=VERTEX_POINT('',#159784) ;
#40642=VERTEX_POINT('',#159786) ;
#40643=VERTEX_POINT('',#159788) ;
#40644=VERTEX_POINT('',#159792) ;
#40645=VERTEX_POINT('',#159793) ;
#40646=VERTEX_POINT('',#159795) ;
#40647=VERTEX_POINT('',#159797) ;
#40648=VERTEX_POINT('',#159799) ;
#40649=VERTEX_POINT('',#159801) ;
#40650=VERTEX_POINT('',#159803) ;
#40651=VERTEX_POINT('',#159805) ;
#40652=VERTEX_POINT('',#159807) ;
#40653=VERTEX_POINT('',#159809) ;
#40654=VERTEX_POINT('',#159813) ;
#40655=VERTEX_POINT('',#159814) ;
#40656=VERTEX_POINT('',#159816) ;
#40657=VERTEX_POINT('',#159818) ;
#40658=VERTEX_POINT('',#159822) ;
#40659=VERTEX_POINT('',#159823) ;
#40660=VERTEX_POINT('',#159825) ;
#40661=VERTEX_POINT('',#159827) ;
#40662=VERTEX_POINT('',#159829) ;
#40663=VERTEX_POINT('',#159831) ;
#40664=VERTEX_POINT('',#159833) ;
#40665=VERTEX_POINT('',#159835) ;
#40666=VERTEX_POINT('',#159837) ;
#40667=VERTEX_POINT('',#159839) ;
#40668=VERTEX_POINT('',#159843) ;
#40669=VERTEX_POINT('',#159844) ;
#40670=VERTEX_POINT('',#159846) ;
#40671=VERTEX_POINT('',#159848) ;
#40672=VERTEX_POINT('',#159852) ;
#40673=VERTEX_POINT('',#159853) ;
#40674=VERTEX_POINT('',#159855) ;
#40675=VERTEX_POINT('',#159857) ;
#40676=VERTEX_POINT('',#159859) ;
#40677=VERTEX_POINT('',#159861) ;
#40678=VERTEX_POINT('',#159863) ;
#40679=VERTEX_POINT('',#159865) ;
#40680=VERTEX_POINT('',#159867) ;
#40681=VERTEX_POINT('',#159869) ;
#40682=VERTEX_POINT('',#159873) ;
#40683=VERTEX_POINT('',#159874) ;
#40684=VERTEX_POINT('',#159876) ;
#40685=VERTEX_POINT('',#159878) ;
#40686=VERTEX_POINT('',#159882) ;
#40687=VERTEX_POINT('',#159883) ;
#40688=VERTEX_POINT('',#159885) ;
#40689=VERTEX_POINT('',#159887) ;
#40690=VERTEX_POINT('',#159889) ;
#40691=VERTEX_POINT('',#159891) ;
#40692=VERTEX_POINT('',#159893) ;
#40693=VERTEX_POINT('',#159895) ;
#40694=VERTEX_POINT('',#159897) ;
#40695=VERTEX_POINT('',#159899) ;
#40696=VERTEX_POINT('',#159903) ;
#40697=VERTEX_POINT('',#159904) ;
#40698=VERTEX_POINT('',#159906) ;
#40699=VERTEX_POINT('',#159908) ;
#40700=VERTEX_POINT('',#159912) ;
#40701=VERTEX_POINT('',#159913) ;
#40702=VERTEX_POINT('',#159915) ;
#40703=VERTEX_POINT('',#159917) ;
#40704=VERTEX_POINT('',#159919) ;
#40705=VERTEX_POINT('',#159921) ;
#40706=VERTEX_POINT('',#159923) ;
#40707=VERTEX_POINT('',#159925) ;
#40708=VERTEX_POINT('',#159927) ;
#40709=VERTEX_POINT('',#159929) ;
#40710=VERTEX_POINT('',#159933) ;
#40711=VERTEX_POINT('',#159934) ;
#40712=VERTEX_POINT('',#159936) ;
#40713=VERTEX_POINT('',#159938) ;
#40714=VERTEX_POINT('',#159942) ;
#40715=VERTEX_POINT('',#159943) ;
#40716=VERTEX_POINT('',#159945) ;
#40717=VERTEX_POINT('',#159947) ;
#40718=VERTEX_POINT('',#159949) ;
#40719=VERTEX_POINT('',#159951) ;
#40720=VERTEX_POINT('',#159953) ;
#40721=VERTEX_POINT('',#159955) ;
#40722=VERTEX_POINT('',#159957) ;
#40723=VERTEX_POINT('',#159959) ;
#40724=VERTEX_POINT('',#159963) ;
#40725=VERTEX_POINT('',#159964) ;
#40726=VERTEX_POINT('',#159966) ;
#40727=VERTEX_POINT('',#159968) ;
#40728=VERTEX_POINT('',#159972) ;
#40729=VERTEX_POINT('',#159973) ;
#40730=VERTEX_POINT('',#159975) ;
#40731=VERTEX_POINT('',#159977) ;
#40732=VERTEX_POINT('',#159981) ;
#40733=VERTEX_POINT('',#159982) ;
#40734=VERTEX_POINT('',#159984) ;
#40735=VERTEX_POINT('',#159986) ;
#40736=VERTEX_POINT('',#159990) ;
#40737=VERTEX_POINT('',#159991) ;
#40738=VERTEX_POINT('',#159993) ;
#40739=VERTEX_POINT('',#159995) ;
#40740=VERTEX_POINT('',#159999) ;
#40741=VERTEX_POINT('',#160000) ;
#40742=VERTEX_POINT('',#160002) ;
#40743=VERTEX_POINT('',#160004) ;
#40744=VERTEX_POINT('',#160006) ;
#40745=VERTEX_POINT('',#160008) ;
#40746=VERTEX_POINT('',#160012) ;
#40747=VERTEX_POINT('',#160013) ;
#40748=VERTEX_POINT('',#160015) ;
#40749=VERTEX_POINT('',#160017) ;
#40750=VERTEX_POINT('',#160021) ;
#40751=VERTEX_POINT('',#160022) ;
#40752=VERTEX_POINT('',#160024) ;
#40753=VERTEX_POINT('',#160026) ;
#40754=VERTEX_POINT('',#160030) ;
#40755=VERTEX_POINT('',#160031) ;
#40756=VERTEX_POINT('',#160033) ;
#40757=VERTEX_POINT('',#160035) ;
#40758=VERTEX_POINT('',#160039) ;
#40759=VERTEX_POINT('',#160040) ;
#40760=VERTEX_POINT('',#160042) ;
#40761=VERTEX_POINT('',#160044) ;
#40762=VERTEX_POINT('',#160046) ;
#40763=VERTEX_POINT('',#160048) ;
#40764=VERTEX_POINT('',#160052) ;
#40765=VERTEX_POINT('',#160053) ;
#40766=VERTEX_POINT('',#160055) ;
#40767=VERTEX_POINT('',#160057) ;
#40768=VERTEX_POINT('',#160061) ;
#40769=VERTEX_POINT('',#160062) ;
#40770=VERTEX_POINT('',#160064) ;
#40771=VERTEX_POINT('',#160066) ;
#40772=VERTEX_POINT('',#160070) ;
#40773=VERTEX_POINT('',#160071) ;
#40774=VERTEX_POINT('',#160073) ;
#40775=VERTEX_POINT('',#160075) ;
#40776=VERTEX_POINT('',#160079) ;
#40777=VERTEX_POINT('',#160080) ;
#40778=VERTEX_POINT('',#160082) ;
#40779=VERTEX_POINT('',#160084) ;
#40780=VERTEX_POINT('',#160086) ;
#40781=VERTEX_POINT('',#160088) ;
#40782=VERTEX_POINT('',#160092) ;
#40783=VERTEX_POINT('',#160093) ;
#40784=VERTEX_POINT('',#160095) ;
#40785=VERTEX_POINT('',#160097) ;
#40786=VERTEX_POINT('',#160101) ;
#40787=VERTEX_POINT('',#160102) ;
#40788=VERTEX_POINT('',#160104) ;
#40789=VERTEX_POINT('',#160106) ;
#40790=VERTEX_POINT('',#160110) ;
#40791=VERTEX_POINT('',#160111) ;
#40792=VERTEX_POINT('',#160113) ;
#40793=VERTEX_POINT('',#160115) ;
#40794=VERTEX_POINT('',#160119) ;
#40795=VERTEX_POINT('',#160120) ;
#40796=VERTEX_POINT('',#160122) ;
#40797=VERTEX_POINT('',#160124) ;
#40798=VERTEX_POINT('',#160126) ;
#40799=VERTEX_POINT('',#160128) ;
#40800=VERTEX_POINT('',#160132) ;
#40801=VERTEX_POINT('',#160133) ;
#40802=VERTEX_POINT('',#160135) ;
#40803=VERTEX_POINT('',#160137) ;
#40804=VERTEX_POINT('',#160141) ;
#40805=VERTEX_POINT('',#160142) ;
#40806=VERTEX_POINT('',#160144) ;
#40807=VERTEX_POINT('',#160146) ;
#40808=VERTEX_POINT('',#160150) ;
#40809=VERTEX_POINT('',#160151) ;
#40810=VERTEX_POINT('',#160153) ;
#40811=VERTEX_POINT('',#160155) ;
#40812=VERTEX_POINT('',#160159) ;
#40813=VERTEX_POINT('',#160160) ;
#40814=VERTEX_POINT('',#160162) ;
#40815=VERTEX_POINT('',#160164) ;
#40816=VERTEX_POINT('',#160166) ;
#40817=VERTEX_POINT('',#160168) ;
#40818=VERTEX_POINT('',#160172) ;
#40819=VERTEX_POINT('',#160173) ;
#40820=VERTEX_POINT('',#160175) ;
#40821=VERTEX_POINT('',#160177) ;
#40822=VERTEX_POINT('',#160181) ;
#40823=VERTEX_POINT('',#160182) ;
#40824=VERTEX_POINT('',#160184) ;
#40825=VERTEX_POINT('',#160186) ;
#40826=VERTEX_POINT('',#160190) ;
#40827=VERTEX_POINT('',#160191) ;
#40828=VERTEX_POINT('',#160193) ;
#40829=VERTEX_POINT('',#160195) ;
#40830=VERTEX_POINT('',#160199) ;
#40831=VERTEX_POINT('',#160200) ;
#40832=VERTEX_POINT('',#160202) ;
#40833=VERTEX_POINT('',#160204) ;
#40834=VERTEX_POINT('',#160206) ;
#40835=VERTEX_POINT('',#160208) ;
#40836=VERTEX_POINT('',#160212) ;
#40837=VERTEX_POINT('',#160213) ;
#40838=VERTEX_POINT('',#160215) ;
#40839=VERTEX_POINT('',#160217) ;
#40840=VERTEX_POINT('',#160221) ;
#40841=VERTEX_POINT('',#160222) ;
#40842=VERTEX_POINT('',#160224) ;
#40843=VERTEX_POINT('',#160226) ;
#40844=VERTEX_POINT('',#160230) ;
#40845=VERTEX_POINT('',#160231) ;
#40846=VERTEX_POINT('',#160233) ;
#40847=VERTEX_POINT('',#160235) ;
#40848=VERTEX_POINT('',#160239) ;
#40849=VERTEX_POINT('',#160240) ;
#40850=VERTEX_POINT('',#160242) ;
#40851=VERTEX_POINT('',#160244) ;
#40852=VERTEX_POINT('',#160246) ;
#40853=VERTEX_POINT('',#160248) ;
#40854=VERTEX_POINT('',#160252) ;
#40855=VERTEX_POINT('',#160253) ;
#40856=VERTEX_POINT('',#160255) ;
#40857=VERTEX_POINT('',#160257) ;
#40858=VERTEX_POINT('',#160261) ;
#40859=VERTEX_POINT('',#160262) ;
#40860=VERTEX_POINT('',#160264) ;
#40861=VERTEX_POINT('',#160266) ;
#40862=VERTEX_POINT('',#160270) ;
#40863=VERTEX_POINT('',#160271) ;
#40864=VERTEX_POINT('',#160273) ;
#40865=VERTEX_POINT('',#160275) ;
#40866=VERTEX_POINT('',#160279) ;
#40867=VERTEX_POINT('',#160280) ;
#40868=VERTEX_POINT('',#160282) ;
#40869=VERTEX_POINT('',#160284) ;
#40870=VERTEX_POINT('',#160286) ;
#40871=VERTEX_POINT('',#160288) ;
#40872=VERTEX_POINT('',#160292) ;
#40873=VERTEX_POINT('',#160293) ;
#40874=VERTEX_POINT('',#160295) ;
#40875=VERTEX_POINT('',#160297) ;
#40876=VERTEX_POINT('',#160301) ;
#40877=VERTEX_POINT('',#160302) ;
#40878=VERTEX_POINT('',#160304) ;
#40879=VERTEX_POINT('',#160306) ;
#40880=VERTEX_POINT('',#160310) ;
#40881=VERTEX_POINT('',#160311) ;
#40882=VERTEX_POINT('',#160313) ;
#40883=VERTEX_POINT('',#160315) ;
#40884=VERTEX_POINT('',#160319) ;
#40885=VERTEX_POINT('',#160320) ;
#40886=VERTEX_POINT('',#160322) ;
#40887=VERTEX_POINT('',#160324) ;
#40888=VERTEX_POINT('',#160326) ;
#40889=VERTEX_POINT('',#160328) ;
#40890=VERTEX_POINT('',#160341) ;
#40891=VERTEX_POINT('',#160342) ;
#40892=VERTEX_POINT('',#160344) ;
#40893=VERTEX_POINT('',#160346) ;
#40894=VERTEX_POINT('',#160350) ;
#40895=VERTEX_POINT('',#160351) ;
#40896=VERTEX_POINT('',#160353) ;
#40897=VERTEX_POINT('',#160355) ;
#40898=VERTEX_POINT('',#160359) ;
#40899=VERTEX_POINT('',#160360) ;
#40900=VERTEX_POINT('',#160362) ;
#40901=VERTEX_POINT('',#160364) ;
#40902=VERTEX_POINT('',#160368) ;
#40903=VERTEX_POINT('',#160369) ;
#40904=VERTEX_POINT('',#160371) ;
#40905=VERTEX_POINT('',#160373) ;
#40906=VERTEX_POINT('',#160377) ;
#40907=VERTEX_POINT('',#160378) ;
#40908=VERTEX_POINT('',#160380) ;
#40909=VERTEX_POINT('',#160382) ;
#40910=VERTEX_POINT('',#160386) ;
#40911=VERTEX_POINT('',#160387) ;
#40912=VERTEX_POINT('',#160389) ;
#40913=VERTEX_POINT('',#160391) ;
#40914=VERTEX_POINT('',#160395) ;
#40915=VERTEX_POINT('',#160396) ;
#40916=VERTEX_POINT('',#160398) ;
#40917=VERTEX_POINT('',#160400) ;
#40918=VERTEX_POINT('',#160404) ;
#40919=VERTEX_POINT('',#160405) ;
#40920=VERTEX_POINT('',#160407) ;
#40921=VERTEX_POINT('',#160409) ;
#40922=VERTEX_POINT('',#160413) ;
#40923=VERTEX_POINT('',#160414) ;
#40924=VERTEX_POINT('',#160416) ;
#40925=VERTEX_POINT('',#160418) ;
#40926=VERTEX_POINT('',#160422) ;
#40927=VERTEX_POINT('',#160423) ;
#40928=VERTEX_POINT('',#160425) ;
#40929=VERTEX_POINT('',#160427) ;
#40930=VERTEX_POINT('',#160431) ;
#40931=VERTEX_POINT('',#160432) ;
#40932=VERTEX_POINT('',#160434) ;
#40933=VERTEX_POINT('',#160436) ;
#40934=VERTEX_POINT('',#160440) ;
#40935=VERTEX_POINT('',#160441) ;
#40936=VERTEX_POINT('',#160443) ;
#40937=VERTEX_POINT('',#160445) ;
#40938=VERTEX_POINT('',#160449) ;
#40939=VERTEX_POINT('',#160450) ;
#40940=VERTEX_POINT('',#160452) ;
#40941=VERTEX_POINT('',#160454) ;
#40942=VERTEX_POINT('',#160458) ;
#40943=VERTEX_POINT('',#160459) ;
#40944=VERTEX_POINT('',#160461) ;
#40945=VERTEX_POINT('',#160463) ;
#40946=VERTEX_POINT('',#160467) ;
#40947=VERTEX_POINT('',#160468) ;
#40948=VERTEX_POINT('',#160470) ;
#40949=VERTEX_POINT('',#160472) ;
#40950=VERTEX_POINT('',#160476) ;
#40951=VERTEX_POINT('',#160477) ;
#40952=VERTEX_POINT('',#160479) ;
#40953=VERTEX_POINT('',#160481) ;
#40954=VERTEX_POINT('',#160485) ;
#40955=VERTEX_POINT('',#160486) ;
#40956=VERTEX_POINT('',#160488) ;
#40957=VERTEX_POINT('',#160490) ;
#40958=VERTEX_POINT('',#160494) ;
#40959=VERTEX_POINT('',#160495) ;
#40960=VERTEX_POINT('',#160497) ;
#40961=VERTEX_POINT('',#160499) ;
#40962=VERTEX_POINT('',#160503) ;
#40963=VERTEX_POINT('',#160504) ;
#40964=VERTEX_POINT('',#160506) ;
#40965=VERTEX_POINT('',#160508) ;
#40966=VERTEX_POINT('',#160512) ;
#40967=VERTEX_POINT('',#160513) ;
#40968=VERTEX_POINT('',#160515) ;
#40969=VERTEX_POINT('',#160517) ;
#40970=VERTEX_POINT('',#160521) ;
#40971=VERTEX_POINT('',#160522) ;
#40972=VERTEX_POINT('',#160524) ;
#40973=VERTEX_POINT('',#160526) ;
#40974=VERTEX_POINT('',#160530) ;
#40975=VERTEX_POINT('',#160531) ;
#40976=VERTEX_POINT('',#160533) ;
#40977=VERTEX_POINT('',#160535) ;
#40978=VERTEX_POINT('',#160539) ;
#40979=VERTEX_POINT('',#160540) ;
#40980=VERTEX_POINT('',#160542) ;
#40981=VERTEX_POINT('',#160544) ;
#40982=VERTEX_POINT('',#160548) ;
#40983=VERTEX_POINT('',#160549) ;
#40984=VERTEX_POINT('',#160551) ;
#40985=VERTEX_POINT('',#160553) ;
#40986=VERTEX_POINT('',#160557) ;
#40987=VERTEX_POINT('',#160558) ;
#40988=VERTEX_POINT('',#160560) ;
#40989=VERTEX_POINT('',#160562) ;
#40990=VERTEX_POINT('',#160566) ;
#40991=VERTEX_POINT('',#160567) ;
#40992=VERTEX_POINT('',#160569) ;
#40993=VERTEX_POINT('',#160571) ;
#40994=VERTEX_POINT('',#160575) ;
#40995=VERTEX_POINT('',#160576) ;
#40996=VERTEX_POINT('',#160578) ;
#40997=VERTEX_POINT('',#160580) ;
#40998=VERTEX_POINT('',#160584) ;
#40999=VERTEX_POINT('',#160585) ;
#41000=VERTEX_POINT('',#160587) ;
#41001=VERTEX_POINT('',#160589) ;
#41002=VERTEX_POINT('',#160593) ;
#41003=VERTEX_POINT('',#160594) ;
#41004=VERTEX_POINT('',#160596) ;
#41005=VERTEX_POINT('',#160598) ;
#41006=VERTEX_POINT('',#160602) ;
#41007=VERTEX_POINT('',#160603) ;
#41008=VERTEX_POINT('',#160605) ;
#41009=VERTEX_POINT('',#160607) ;
#41010=VERTEX_POINT('',#160611) ;
#41011=VERTEX_POINT('',#160612) ;
#41012=VERTEX_POINT('',#160614) ;
#41013=VERTEX_POINT('',#160616) ;
#41014=VERTEX_POINT('',#160620) ;
#41015=VERTEX_POINT('',#160621) ;
#41016=VERTEX_POINT('',#160623) ;
#41017=VERTEX_POINT('',#160625) ;
#41018=VERTEX_POINT('',#160629) ;
#41019=VERTEX_POINT('',#160630) ;
#41020=VERTEX_POINT('',#160632) ;
#41021=VERTEX_POINT('',#160634) ;
#41022=VERTEX_POINT('',#160638) ;
#41023=VERTEX_POINT('',#160639) ;
#41024=VERTEX_POINT('',#160641) ;
#41025=VERTEX_POINT('',#160643) ;
#41026=VERTEX_POINT('',#160647) ;
#41027=VERTEX_POINT('',#160648) ;
#41028=VERTEX_POINT('',#160650) ;
#41029=VERTEX_POINT('',#160652) ;
#41030=VERTEX_POINT('',#160656) ;
#41031=VERTEX_POINT('',#160657) ;
#41032=VERTEX_POINT('',#160659) ;
#41033=VERTEX_POINT('',#160661) ;
#41034=VERTEX_POINT('',#160665) ;
#41035=VERTEX_POINT('',#160666) ;
#41036=VERTEX_POINT('',#160668) ;
#41037=VERTEX_POINT('',#160670) ;
#41038=VERTEX_POINT('',#160673) ;
#41039=VERTEX_POINT('',#160674) ;
#41040=VERTEX_POINT('',#160676) ;
#41041=VERTEX_POINT('',#160678) ;
#41042=VERTEX_POINT('',#160680) ;
#41043=VERTEX_POINT('',#160682) ;
#41044=VERTEX_POINT('',#160684) ;
#41045=VERTEX_POINT('',#160686) ;
#41046=VERTEX_POINT('',#160690) ;
#41047=VERTEX_POINT('',#160691) ;
#41048=VERTEX_POINT('',#160696) ;
#41049=VERTEX_POINT('',#160697) ;
#41050=VERTEX_POINT('',#160702) ;
#41051=VERTEX_POINT('',#160704) ;
#41052=VERTEX_POINT('',#160708) ;
#41053=VERTEX_POINT('',#160709) ;
#41054=VERTEX_POINT('',#160714) ;
#41055=VERTEX_POINT('',#160715) ;
#41056=VERTEX_POINT('',#160717) ;
#41057=VERTEX_POINT('',#160719) ;
#41058=VERTEX_POINT('',#160722) ;
#41059=VERTEX_POINT('',#160723) ;
#41060=VERTEX_POINT('',#160725) ;
#41061=VERTEX_POINT('',#160727) ;
#41062=VERTEX_POINT('',#160729) ;
#41063=VERTEX_POINT('',#160731) ;
#41064=VERTEX_POINT('',#160733) ;
#41065=VERTEX_POINT('',#160735) ;
#41066=VERTEX_POINT('',#160739) ;
#41067=VERTEX_POINT('',#160740) ;
#41068=VERTEX_POINT('',#160745) ;
#41069=VERTEX_POINT('',#160746) ;
#41070=VERTEX_POINT('',#160751) ;
#41071=VERTEX_POINT('',#160753) ;
#41072=VERTEX_POINT('',#160757) ;
#41073=VERTEX_POINT('',#160758) ;
#41074=VERTEX_POINT('',#160763) ;
#41075=VERTEX_POINT('',#160764) ;
#41076=VERTEX_POINT('',#160766) ;
#41077=VERTEX_POINT('',#160768) ;
#41078=VERTEX_POINT('',#160771) ;
#41079=VERTEX_POINT('',#160772) ;
#41080=VERTEX_POINT('',#160774) ;
#41081=VERTEX_POINT('',#160776) ;
#41082=VERTEX_POINT('',#160778) ;
#41083=VERTEX_POINT('',#160780) ;
#41084=VERTEX_POINT('',#160782) ;
#41085=VERTEX_POINT('',#160784) ;
#41086=VERTEX_POINT('',#160788) ;
#41087=VERTEX_POINT('',#160789) ;
#41088=VERTEX_POINT('',#160794) ;
#41089=VERTEX_POINT('',#160795) ;
#41090=VERTEX_POINT('',#160800) ;
#41091=VERTEX_POINT('',#160802) ;
#41092=VERTEX_POINT('',#160806) ;
#41093=VERTEX_POINT('',#160807) ;
#41094=VERTEX_POINT('',#160812) ;
#41095=VERTEX_POINT('',#160813) ;
#41096=VERTEX_POINT('',#160815) ;
#41097=VERTEX_POINT('',#160817) ;
#41098=VERTEX_POINT('',#160820) ;
#41099=VERTEX_POINT('',#160821) ;
#41100=VERTEX_POINT('',#160823) ;
#41101=VERTEX_POINT('',#160825) ;
#41102=VERTEX_POINT('',#160827) ;
#41103=VERTEX_POINT('',#160829) ;
#41104=VERTEX_POINT('',#160831) ;
#41105=VERTEX_POINT('',#160833) ;
#41106=VERTEX_POINT('',#160837) ;
#41107=VERTEX_POINT('',#160838) ;
#41108=VERTEX_POINT('',#160843) ;
#41109=VERTEX_POINT('',#160844) ;
#41110=VERTEX_POINT('',#160849) ;
#41111=VERTEX_POINT('',#160851) ;
#41112=VERTEX_POINT('',#160855) ;
#41113=VERTEX_POINT('',#160856) ;
#41114=VERTEX_POINT('',#160861) ;
#41115=VERTEX_POINT('',#160862) ;
#41116=VERTEX_POINT('',#160864) ;
#41117=VERTEX_POINT('',#160866) ;
#41118=VERTEX_POINT('',#160869) ;
#41119=VERTEX_POINT('',#160870) ;
#41120=VERTEX_POINT('',#160872) ;
#41121=VERTEX_POINT('',#160874) ;
#41122=VERTEX_POINT('',#160876) ;
#41123=VERTEX_POINT('',#160878) ;
#41124=VERTEX_POINT('',#160880) ;
#41125=VERTEX_POINT('',#160882) ;
#41126=VERTEX_POINT('',#160886) ;
#41127=VERTEX_POINT('',#160887) ;
#41128=VERTEX_POINT('',#160892) ;
#41129=VERTEX_POINT('',#160893) ;
#41130=VERTEX_POINT('',#160898) ;
#41131=VERTEX_POINT('',#160900) ;
#41132=VERTEX_POINT('',#160904) ;
#41133=VERTEX_POINT('',#160905) ;
#41134=VERTEX_POINT('',#160910) ;
#41135=VERTEX_POINT('',#160911) ;
#41136=VERTEX_POINT('',#160913) ;
#41137=VERTEX_POINT('',#160915) ;
#41138=VERTEX_POINT('',#160918) ;
#41139=VERTEX_POINT('',#160919) ;
#41140=VERTEX_POINT('',#160921) ;
#41141=VERTEX_POINT('',#160923) ;
#41142=VERTEX_POINT('',#160925) ;
#41143=VERTEX_POINT('',#160927) ;
#41144=VERTEX_POINT('',#160929) ;
#41145=VERTEX_POINT('',#160931) ;
#41146=VERTEX_POINT('',#160935) ;
#41147=VERTEX_POINT('',#160936) ;
#41148=VERTEX_POINT('',#160941) ;
#41149=VERTEX_POINT('',#160942) ;
#41150=VERTEX_POINT('',#160947) ;
#41151=VERTEX_POINT('',#160949) ;
#41152=VERTEX_POINT('',#160953) ;
#41153=VERTEX_POINT('',#160954) ;
#41154=VERTEX_POINT('',#160959) ;
#41155=VERTEX_POINT('',#160960) ;
#41156=VERTEX_POINT('',#160962) ;
#41157=VERTEX_POINT('',#160964) ;
#41158=VERTEX_POINT('',#160967) ;
#41159=VERTEX_POINT('',#160968) ;
#41160=VERTEX_POINT('',#160970) ;
#41161=VERTEX_POINT('',#160972) ;
#41162=VERTEX_POINT('',#160974) ;
#41163=VERTEX_POINT('',#160976) ;
#41164=VERTEX_POINT('',#160978) ;
#41165=VERTEX_POINT('',#160980) ;
#41166=VERTEX_POINT('',#160984) ;
#41167=VERTEX_POINT('',#160985) ;
#41168=VERTEX_POINT('',#160990) ;
#41169=VERTEX_POINT('',#160991) ;
#41170=VERTEX_POINT('',#160996) ;
#41171=VERTEX_POINT('',#160998) ;
#41172=VERTEX_POINT('',#161002) ;
#41173=VERTEX_POINT('',#161003) ;
#41174=VERTEX_POINT('',#161008) ;
#41175=VERTEX_POINT('',#161009) ;
#41176=VERTEX_POINT('',#161011) ;
#41177=VERTEX_POINT('',#161013) ;
#41178=VERTEX_POINT('',#161016) ;
#41179=VERTEX_POINT('',#161017) ;
#41180=VERTEX_POINT('',#161019) ;
#41181=VERTEX_POINT('',#161021) ;
#41182=VERTEX_POINT('',#161023) ;
#41183=VERTEX_POINT('',#161025) ;
#41184=VERTEX_POINT('',#161027) ;
#41185=VERTEX_POINT('',#161029) ;
#41186=VERTEX_POINT('',#161033) ;
#41187=VERTEX_POINT('',#161034) ;
#41188=VERTEX_POINT('',#161039) ;
#41189=VERTEX_POINT('',#161040) ;
#41190=VERTEX_POINT('',#161045) ;
#41191=VERTEX_POINT('',#161047) ;
#41192=VERTEX_POINT('',#161051) ;
#41193=VERTEX_POINT('',#161052) ;
#41194=VERTEX_POINT('',#161057) ;
#41195=VERTEX_POINT('',#161058) ;
#41196=VERTEX_POINT('',#161060) ;
#41197=VERTEX_POINT('',#161062) ;
#41198=VERTEX_POINT('',#161065) ;
#41199=VERTEX_POINT('',#161066) ;
#41200=VERTEX_POINT('',#161068) ;
#41201=VERTEX_POINT('',#161070) ;
#41202=VERTEX_POINT('',#161072) ;
#41203=VERTEX_POINT('',#161074) ;
#41204=VERTEX_POINT('',#161076) ;
#41205=VERTEX_POINT('',#161078) ;
#41206=VERTEX_POINT('',#161082) ;
#41207=VERTEX_POINT('',#161083) ;
#41208=VERTEX_POINT('',#161088) ;
#41209=VERTEX_POINT('',#161089) ;
#41210=VERTEX_POINT('',#161094) ;
#41211=VERTEX_POINT('',#161096) ;
#41212=VERTEX_POINT('',#161100) ;
#41213=VERTEX_POINT('',#161101) ;
#41214=VERTEX_POINT('',#161106) ;
#41215=VERTEX_POINT('',#161107) ;
#41216=VERTEX_POINT('',#161109) ;
#41217=VERTEX_POINT('',#161111) ;
#41218=VERTEX_POINT('',#161115) ;
#41219=VERTEX_POINT('',#161116) ;
#41220=VERTEX_POINT('',#161118) ;
#41221=VERTEX_POINT('',#161120) ;
#41222=VERTEX_POINT('',#161124) ;
#41223=VERTEX_POINT('',#161125) ;
#41224=VERTEX_POINT('',#161127) ;
#41225=VERTEX_POINT('',#161129) ;
#41226=VERTEX_POINT('',#161133) ;
#41227=VERTEX_POINT('',#161134) ;
#41228=VERTEX_POINT('',#161136) ;
#41229=VERTEX_POINT('',#161138) ;
#41230=VERTEX_POINT('',#161142) ;
#41231=VERTEX_POINT('',#161143) ;
#41232=VERTEX_POINT('',#161145) ;
#41233=VERTEX_POINT('',#161147) ;
#41234=VERTEX_POINT('',#161151) ;
#41235=VERTEX_POINT('',#161152) ;
#41236=VERTEX_POINT('',#161154) ;
#41237=VERTEX_POINT('',#161156) ;
#41238=VERTEX_POINT('',#161160) ;
#41239=VERTEX_POINT('',#161161) ;
#41240=VERTEX_POINT('',#161163) ;
#41241=VERTEX_POINT('',#161165) ;
#41242=VERTEX_POINT('',#161169) ;
#41243=VERTEX_POINT('',#161170) ;
#41244=VERTEX_POINT('',#161172) ;
#41245=VERTEX_POINT('',#161174) ;
#41246=VERTEX_POINT('',#161178) ;
#41247=VERTEX_POINT('',#161179) ;
#41248=VERTEX_POINT('',#161181) ;
#41249=VERTEX_POINT('',#161183) ;
#41250=VERTEX_POINT('',#161286) ;
#41251=VERTEX_POINT('',#161287) ;
#41252=VERTEX_POINT('',#161289) ;
#41253=VERTEX_POINT('',#161291) ;
#41254=VERTEX_POINT('',#161295) ;
#41255=VERTEX_POINT('',#161297) ;
#41256=VERTEX_POINT('',#161301) ;
#41257=VERTEX_POINT('',#161303) ;
#41258=VERTEX_POINT('',#161307) ;
#41259=VERTEX_POINT('',#161309) ;
#41260=VERTEX_POINT('',#161313) ;
#41261=VERTEX_POINT('',#161315) ;
#41262=VERTEX_POINT('',#161319) ;
#41263=VERTEX_POINT('',#161321) ;
#41264=VERTEX_POINT('',#161325) ;
#41265=VERTEX_POINT('',#161327) ;
#41266=VERTEX_POINT('',#161334) ;
#41267=VERTEX_POINT('',#161335) ;
#41268=VERTEX_POINT('',#161337) ;
#41269=VERTEX_POINT('',#161339) ;
#41270=VERTEX_POINT('',#161343) ;
#41271=VERTEX_POINT('',#161344) ;
#41272=VERTEX_POINT('',#161346) ;
#41273=VERTEX_POINT('',#161348) ;
#41274=VERTEX_POINT('',#161352) ;
#41275=VERTEX_POINT('',#161354) ;
#41276=VERTEX_POINT('',#161358) ;
#41277=VERTEX_POINT('',#161360) ;
#41278=VERTEX_POINT('',#161364) ;
#41279=VERTEX_POINT('',#161366) ;
#41280=VERTEX_POINT('',#161370) ;
#41281=VERTEX_POINT('',#161372) ;
#41282=VERTEX_POINT('',#161376) ;
#41283=VERTEX_POINT('',#161378) ;
#41284=VERTEX_POINT('',#161382) ;
#41285=VERTEX_POINT('',#161384) ;
#41286=VERTEX_POINT('',#161391) ;
#41287=VERTEX_POINT('',#161392) ;
#41288=VERTEX_POINT('',#161394) ;
#41289=VERTEX_POINT('',#161396) ;
#41290=VERTEX_POINT('',#161400) ;
#41291=VERTEX_POINT('',#161401) ;
#41292=VERTEX_POINT('',#161403) ;
#41293=VERTEX_POINT('',#161405) ;
#41294=VERTEX_POINT('',#161409) ;
#41295=VERTEX_POINT('',#161411) ;
#41296=VERTEX_POINT('',#161415) ;
#41297=VERTEX_POINT('',#161417) ;
#41298=VERTEX_POINT('',#161421) ;
#41299=VERTEX_POINT('',#161423) ;
#41300=VERTEX_POINT('',#161427) ;
#41301=VERTEX_POINT('',#161429) ;
#41302=VERTEX_POINT('',#161433) ;
#41303=VERTEX_POINT('',#161435) ;
#41304=VERTEX_POINT('',#161439) ;
#41305=VERTEX_POINT('',#161441) ;
#41306=VERTEX_POINT('',#161448) ;
#41307=VERTEX_POINT('',#161449) ;
#41308=VERTEX_POINT('',#161451) ;
#41309=VERTEX_POINT('',#161453) ;
#41310=VERTEX_POINT('',#161457) ;
#41311=VERTEX_POINT('',#161458) ;
#41312=VERTEX_POINT('',#161460) ;
#41313=VERTEX_POINT('',#161462) ;
#41314=VERTEX_POINT('',#161466) ;
#41315=VERTEX_POINT('',#161468) ;
#41316=VERTEX_POINT('',#161472) ;
#41317=VERTEX_POINT('',#161474) ;
#41318=VERTEX_POINT('',#161478) ;
#41319=VERTEX_POINT('',#161480) ;
#41320=VERTEX_POINT('',#161484) ;
#41321=VERTEX_POINT('',#161486) ;
#41322=VERTEX_POINT('',#161490) ;
#41323=VERTEX_POINT('',#161492) ;
#41324=VERTEX_POINT('',#161496) ;
#41325=VERTEX_POINT('',#161498) ;
#41326=VERTEX_POINT('',#161505) ;
#41327=VERTEX_POINT('',#161506) ;
#41328=VERTEX_POINT('',#161508) ;
#41329=VERTEX_POINT('',#161510) ;
#41330=VERTEX_POINT('',#161514) ;
#41331=VERTEX_POINT('',#161515) ;
#41332=VERTEX_POINT('',#161517) ;
#41333=VERTEX_POINT('',#161519) ;
#41334=VERTEX_POINT('',#161523) ;
#41335=VERTEX_POINT('',#161525) ;
#41336=VERTEX_POINT('',#161529) ;
#41337=VERTEX_POINT('',#161531) ;
#41338=VERTEX_POINT('',#161535) ;
#41339=VERTEX_POINT('',#161537) ;
#41340=VERTEX_POINT('',#161541) ;
#41341=VERTEX_POINT('',#161543) ;
#41342=VERTEX_POINT('',#161547) ;
#41343=VERTEX_POINT('',#161549) ;
#41344=VERTEX_POINT('',#161553) ;
#41345=VERTEX_POINT('',#161555) ;
#41346=VERTEX_POINT('',#161562) ;
#41347=VERTEX_POINT('',#161563) ;
#41348=VERTEX_POINT('',#161565) ;
#41349=VERTEX_POINT('',#161567) ;
#41350=VERTEX_POINT('',#161571) ;
#41351=VERTEX_POINT('',#161572) ;
#41352=VERTEX_POINT('',#161574) ;
#41353=VERTEX_POINT('',#161576) ;
#41354=VERTEX_POINT('',#161580) ;
#41355=VERTEX_POINT('',#161582) ;
#41356=VERTEX_POINT('',#161586) ;
#41357=VERTEX_POINT('',#161588) ;
#41358=VERTEX_POINT('',#161592) ;
#41359=VERTEX_POINT('',#161594) ;
#41360=VERTEX_POINT('',#161598) ;
#41361=VERTEX_POINT('',#161600) ;
#41362=VERTEX_POINT('',#161604) ;
#41363=VERTEX_POINT('',#161606) ;
#41364=VERTEX_POINT('',#161610) ;
#41365=VERTEX_POINT('',#161612) ;
#41366=VERTEX_POINT('',#161619) ;
#41367=VERTEX_POINT('',#161620) ;
#41368=VERTEX_POINT('',#161622) ;
#41369=VERTEX_POINT('',#161624) ;
#41370=VERTEX_POINT('',#161628) ;
#41371=VERTEX_POINT('',#161629) ;
#41372=VERTEX_POINT('',#161631) ;
#41373=VERTEX_POINT('',#161633) ;
#41374=VERTEX_POINT('',#161637) ;
#41375=VERTEX_POINT('',#161639) ;
#41376=VERTEX_POINT('',#161643) ;
#41377=VERTEX_POINT('',#161645) ;
#41378=VERTEX_POINT('',#161649) ;
#41379=VERTEX_POINT('',#161651) ;
#41380=VERTEX_POINT('',#161655) ;
#41381=VERTEX_POINT('',#161657) ;
#41382=VERTEX_POINT('',#161661) ;
#41383=VERTEX_POINT('',#161663) ;
#41384=VERTEX_POINT('',#161667) ;
#41385=VERTEX_POINT('',#161669) ;
#41386=VERTEX_POINT('',#161676) ;
#41387=VERTEX_POINT('',#161677) ;
#41388=VERTEX_POINT('',#161679) ;
#41389=VERTEX_POINT('',#161681) ;
#41390=VERTEX_POINT('',#161685) ;
#41391=VERTEX_POINT('',#161686) ;
#41392=VERTEX_POINT('',#161688) ;
#41393=VERTEX_POINT('',#161690) ;
#41394=VERTEX_POINT('',#161694) ;
#41395=VERTEX_POINT('',#161696) ;
#41396=VERTEX_POINT('',#161700) ;
#41397=VERTEX_POINT('',#161702) ;
#41398=VERTEX_POINT('',#161706) ;
#41399=VERTEX_POINT('',#161708) ;
#41400=VERTEX_POINT('',#161712) ;
#41401=VERTEX_POINT('',#161714) ;
#41402=VERTEX_POINT('',#161718) ;
#41403=VERTEX_POINT('',#161720) ;
#41404=VERTEX_POINT('',#161724) ;
#41405=VERTEX_POINT('',#161726) ;
#41406=VERTEX_POINT('',#161733) ;
#41407=VERTEX_POINT('',#161734) ;
#41408=VERTEX_POINT('',#161736) ;
#41409=VERTEX_POINT('',#161738) ;
#41410=VERTEX_POINT('',#161742) ;
#41411=VERTEX_POINT('',#161743) ;
#41412=VERTEX_POINT('',#161745) ;
#41413=VERTEX_POINT('',#161747) ;
#41414=VERTEX_POINT('',#161751) ;
#41415=VERTEX_POINT('',#161753) ;
#41416=VERTEX_POINT('',#161757) ;
#41417=VERTEX_POINT('',#161759) ;
#41418=VERTEX_POINT('',#161763) ;
#41419=VERTEX_POINT('',#161765) ;
#41420=VERTEX_POINT('',#161769) ;
#41421=VERTEX_POINT('',#161771) ;
#41422=VERTEX_POINT('',#161775) ;
#41423=VERTEX_POINT('',#161777) ;
#41424=VERTEX_POINT('',#161781) ;
#41425=VERTEX_POINT('',#161783) ;
#41426=VERTEX_POINT('',#161790) ;
#41427=VERTEX_POINT('',#161791) ;
#41428=VERTEX_POINT('',#161793) ;
#41429=VERTEX_POINT('',#161795) ;
#41430=VERTEX_POINT('',#161901) ;
#41431=VERTEX_POINT('',#161917) ;
#41432=VERTEX_POINT('',#161934) ;
#41433=VERTEX_POINT('',#161950) ;
#41434=VERTEX_POINT('',#161967) ;
#41435=VERTEX_POINT('',#161983) ;
#41436=VERTEX_POINT('',#162000) ;
#41437=VERTEX_POINT('',#162016) ;
#41438=VERTEX_POINT('',#162033) ;
#41439=VERTEX_POINT('',#162049) ;
#41440=VERTEX_POINT('',#162066) ;
#41441=VERTEX_POINT('',#162082) ;
#41442=VERTEX_POINT('',#162099) ;
#41443=VERTEX_POINT('',#162115) ;
#41444=VERTEX_POINT('',#162132) ;
#41445=VERTEX_POINT('',#162148) ;
#41446=VERTEX_POINT('',#162165) ;
#41447=VERTEX_POINT('',#162181) ;
#41448=VERTEX_POINT('',#162198) ;
#41449=VERTEX_POINT('',#162214) ;
#41450=VERTEX_POINT('',#162231) ;
#41451=VERTEX_POINT('',#162247) ;
#41452=VERTEX_POINT('',#162264) ;
#41453=VERTEX_POINT('',#162280) ;
#41454=VERTEX_POINT('',#162297) ;
#41455=VERTEX_POINT('',#162313) ;
#41456=VERTEX_POINT('',#162330) ;
#41457=VERTEX_POINT('',#162346) ;
#41458=VERTEX_POINT('',#162363) ;
#41459=VERTEX_POINT('',#162379) ;
#41460=VERTEX_POINT('',#162396) ;
#41461=VERTEX_POINT('',#162412) ;
#41462=VERTEX_POINT('',#162429) ;
#41463=VERTEX_POINT('',#162445) ;
#41464=VERTEX_POINT('',#162462) ;
#41465=VERTEX_POINT('',#162478) ;
#41466=VERTEX_POINT('',#162495) ;
#41467=VERTEX_POINT('',#162511) ;
#41468=VERTEX_POINT('',#162528) ;
#41469=VERTEX_POINT('',#162544) ;
#41470=VERTEX_POINT('',#162561) ;
#41471=VERTEX_POINT('',#162577) ;
#41472=VERTEX_POINT('',#162594) ;
#41473=VERTEX_POINT('',#162610) ;
#41474=VERTEX_POINT('',#162627) ;
#41475=VERTEX_POINT('',#162643) ;
#41476=VERTEX_POINT('',#162660) ;
#41477=VERTEX_POINT('',#162676) ;
#41478=VERTEX_POINT('',#162693) ;
#41479=VERTEX_POINT('',#162709) ;
#41480=VERTEX_POINT('',#162726) ;
#41481=VERTEX_POINT('',#162742) ;
#41482=VERTEX_POINT('',#162759) ;
#41483=VERTEX_POINT('',#162775) ;
#41484=VERTEX_POINT('',#162792) ;
#41485=VERTEX_POINT('',#162808) ;
#41486=VERTEX_POINT('',#162825) ;
#41487=VERTEX_POINT('',#162841) ;
#41488=VERTEX_POINT('',#162858) ;
#41489=VERTEX_POINT('',#162874) ;
#41490=VERTEX_POINT('',#162891) ;
#41491=VERTEX_POINT('',#162907) ;
#41492=VERTEX_POINT('',#162924) ;
#41493=VERTEX_POINT('',#162940) ;
#41494=VERTEX_POINT('',#163149) ;
#41495=VERTEX_POINT('',#163152) ;
#41496=VERTEX_POINT('',#163154) ;
#41497=VERTEX_POINT('',#163158) ;
#41498=VERTEX_POINT('',#163161) ;
#41499=VERTEX_POINT('',#163168) ;
#41500=VERTEX_POINT('',#163170) ;
#41501=VERTEX_POINT('',#163173) ;
#41502=VERTEX_POINT('',#163177) ;
#41503=VERTEX_POINT('',#163180) ;
#41504=VERTEX_POINT('',#163182) ;
#41505=VERTEX_POINT('',#163186) ;
#41506=VERTEX_POINT('',#163189) ;
#41507=VERTEX_POINT('',#163196) ;
#41508=VERTEX_POINT('',#163198) ;
#41509=VERTEX_POINT('',#163201) ;
#41510=VERTEX_POINT('',#163205) ;
#41511=VERTEX_POINT('',#163208) ;
#41512=VERTEX_POINT('',#163210) ;
#41513=VERTEX_POINT('',#163214) ;
#41514=VERTEX_POINT('',#163217) ;
#41515=VERTEX_POINT('',#163224) ;
#41516=VERTEX_POINT('',#163226) ;
#41517=VERTEX_POINT('',#163229) ;
#41518=VERTEX_POINT('',#163233) ;
#41519=VERTEX_POINT('',#163236) ;
#41520=VERTEX_POINT('',#163238) ;
#41521=VERTEX_POINT('',#163242) ;
#41522=VERTEX_POINT('',#163245) ;
#41523=VERTEX_POINT('',#163252) ;
#41524=VERTEX_POINT('',#163254) ;
#41525=VERTEX_POINT('',#163257) ;
#41526=VERTEX_POINT('',#163261) ;
#41527=VERTEX_POINT('',#163264) ;
#41528=VERTEX_POINT('',#163266) ;
#41529=VERTEX_POINT('',#163270) ;
#41530=VERTEX_POINT('',#163273) ;
#41531=VERTEX_POINT('',#163280) ;
#41532=VERTEX_POINT('',#163282) ;
#41533=VERTEX_POINT('',#163285) ;
#41534=VERTEX_POINT('',#163289) ;
#41535=VERTEX_POINT('',#163292) ;
#41536=VERTEX_POINT('',#163294) ;
#41537=VERTEX_POINT('',#163298) ;
#41538=VERTEX_POINT('',#163301) ;
#41539=VERTEX_POINT('',#163308) ;
#41540=VERTEX_POINT('',#163310) ;
#41541=VERTEX_POINT('',#163313) ;
#41542=VERTEX_POINT('',#163317) ;
#41543=VERTEX_POINT('',#163320) ;
#41544=VERTEX_POINT('',#163322) ;
#41545=VERTEX_POINT('',#163326) ;
#41546=VERTEX_POINT('',#163329) ;
#41547=VERTEX_POINT('',#163336) ;
#41548=VERTEX_POINT('',#163338) ;
#41549=VERTEX_POINT('',#163341) ;
#41550=VERTEX_POINT('',#163345) ;
#41551=VERTEX_POINT('',#163348) ;
#41552=VERTEX_POINT('',#163350) ;
#41553=VERTEX_POINT('',#163354) ;
#41554=VERTEX_POINT('',#163357) ;
#41555=VERTEX_POINT('',#163364) ;
#41556=VERTEX_POINT('',#163366) ;
#41557=VERTEX_POINT('',#163369) ;
#41558=VERTEX_POINT('',#167424) ;
#41559=VERTEX_POINT('',#167454) ;
#41560=VERTEX_POINT('',#167520) ;
#41561=VERTEX_POINT('',#167550) ;
#41562=VERTEX_POINT('',#167589) ;
#41563=VERTEX_POINT('',#167619) ;
#41564=VERTEX_POINT('',#167658) ;
#41565=VERTEX_POINT('',#167688) ;
#41566=VERTEX_POINT('',#167727) ;
#41567=VERTEX_POINT('',#167757) ;
#41568=VERTEX_POINT('',#167796) ;
#41569=VERTEX_POINT('',#167826) ;
#41570=VERTEX_POINT('',#167865) ;
#41571=VERTEX_POINT('',#167895) ;
#41572=VERTEX_POINT('',#167934) ;
#41573=VERTEX_POINT('',#167964) ;
#41574=VERTEX_POINT('',#168004) ;
#41575=VERTEX_POINT('',#168043) ;
#41576=VERTEX_POINT('',#168105) ;
#41577=VERTEX_POINT('',#168138) ;
#41578=VERTEX_POINT('',#168200) ;
#41579=VERTEX_POINT('',#168233) ;
#41580=VERTEX_POINT('',#168295) ;
#41581=VERTEX_POINT('',#168328) ;
#41582=VERTEX_POINT('',#168390) ;
#41583=VERTEX_POINT('',#168423) ;
#41584=VERTEX_POINT('',#168485) ;
#41585=VERTEX_POINT('',#168518) ;
#41586=VERTEX_POINT('',#168580) ;
#41587=VERTEX_POINT('',#168613) ;
#41588=VERTEX_POINT('',#168675) ;
#41589=VERTEX_POINT('',#168708) ;
#41590=VERTEX_POINT('',#168770) ;
#41591=VERTEX_POINT('',#168803) ;
#41592=VERTEX_POINT('',#168865) ;
#48897=EDGE_CURVE('',#38742,#38743,#32295,.T.) ;
#48898=EDGE_CURVE('',#38744,#38742,#5767,.T.) ;
#48899=EDGE_CURVE('',#38744,#38745,#32296,.T.) ;
#48900=EDGE_CURVE('',#38743,#38745,#5768,.T.) ;
#48901=EDGE_CURVE('',#38746,#38747,#32297,.T.) ;
#48902=EDGE_CURVE('',#38748,#38746,#32298,.T.) ;
#48903=EDGE_CURVE('',#38749,#38748,#32299,.T.) ;
#48904=EDGE_CURVE('',#38749,#38747,#32300,.T.) ;
#48905=EDGE_CURVE('',#38750,#38751,#32301,.T.) ;
#48906=EDGE_CURVE('',#38752,#38750,#32302,.T.) ;
#48907=EDGE_CURVE('',#38753,#38752,#32303,.T.) ;
#48908=EDGE_CURVE('',#38753,#38751,#32304,.T.) ;
#48909=EDGE_CURVE('',#38754,#38755,#32305,.T.) ;
#48910=EDGE_CURVE('',#38754,#38756,#2197,.T.) ;
#48911=EDGE_CURVE('',#38757,#38756,#32306,.T.) ;
#48912=EDGE_CURVE('',#38755,#38757,#2198,.T.) ;
#48913=EDGE_CURVE('',#38758,#38759,#32307,.T.) ;
#48914=EDGE_CURVE('',#38760,#38758,#32308,.T.) ;
#48915=EDGE_CURVE('',#38761,#38760,#32309,.T.) ;
#48916=EDGE_CURVE('',#38761,#38759,#32310,.T.) ;
#48917=EDGE_CURVE('',#38762,#38754,#32311,.T.) ;
#48918=EDGE_CURVE('',#38762,#38763,#2199,.T.) ;
#48919=EDGE_CURVE('',#38764,#38763,#32312,.T.) ;
#48920=EDGE_CURVE('',#38754,#38764,#2200,.T.) ;
#48921=EDGE_CURVE('',#38765,#38766,#32313,.T.) ;
#48922=EDGE_CURVE('',#38767,#38765,#32314,.T.) ;
#48923=EDGE_CURVE('',#38768,#38767,#32315,.T.) ;
#48924=EDGE_CURVE('',#38768,#38766,#32316,.T.) ;
#48925=EDGE_CURVE('',#38769,#38762,#32317,.T.) ;
#48926=EDGE_CURVE('',#38769,#38770,#2201,.T.) ;
#48927=EDGE_CURVE('',#38771,#38770,#32318,.T.) ;
#48928=EDGE_CURVE('',#38762,#38771,#2202,.T.) ;
#48929=EDGE_CURVE('',#38772,#38773,#32319,.T.) ;
#48930=EDGE_CURVE('',#38774,#38772,#32320,.T.) ;
#48931=EDGE_CURVE('',#38775,#38774,#32321,.T.) ;
#48932=EDGE_CURVE('',#38775,#38773,#32322,.T.) ;
#48933=EDGE_CURVE('',#38776,#38769,#32323,.T.) ;
#48934=EDGE_CURVE('',#38776,#38777,#2203,.T.) ;
#48935=EDGE_CURVE('',#38778,#38777,#32324,.T.) ;
#48936=EDGE_CURVE('',#38769,#38778,#2204,.T.) ;
#48937=EDGE_CURVE('',#38779,#38780,#32325,.T.) ;
#48938=EDGE_CURVE('',#38781,#38779,#32326,.T.) ;
#48939=EDGE_CURVE('',#38782,#38781,#32327,.T.) ;
#48940=EDGE_CURVE('',#38782,#38780,#32328,.T.) ;
#48941=EDGE_CURVE('',#38783,#38776,#32329,.T.) ;
#48942=EDGE_CURVE('',#38783,#38784,#2205,.T.) ;
#48943=EDGE_CURVE('',#38785,#38784,#32330,.T.) ;
#48944=EDGE_CURVE('',#38776,#38785,#2206,.T.) ;
#48945=EDGE_CURVE('',#38786,#38787,#32331,.T.) ;
#48946=EDGE_CURVE('',#38788,#38786,#32332,.T.) ;
#48947=EDGE_CURVE('',#38789,#38788,#32333,.T.) ;
#48948=EDGE_CURVE('',#38789,#38787,#32334,.T.) ;
#48949=EDGE_CURVE('',#38790,#38783,#32335,.T.) ;
#48950=EDGE_CURVE('',#38790,#38791,#2207,.T.) ;
#48951=EDGE_CURVE('',#38792,#38791,#32336,.T.) ;
#48952=EDGE_CURVE('',#38783,#38792,#2208,.T.) ;
#48953=EDGE_CURVE('',#38793,#38794,#32337,.T.) ;
#48954=EDGE_CURVE('',#38795,#38793,#32338,.T.) ;
#48955=EDGE_CURVE('',#38796,#38795,#32339,.T.) ;
#48956=EDGE_CURVE('',#38796,#38794,#32340,.T.) ;
#48957=EDGE_CURVE('',#38797,#38790,#32341,.T.) ;
#48958=EDGE_CURVE('',#38797,#38798,#2209,.T.) ;
#48959=EDGE_CURVE('',#38799,#38798,#32342,.T.) ;
#48960=EDGE_CURVE('',#38790,#38799,#2210,.T.) ;
#48961=EDGE_CURVE('',#38800,#38801,#32343,.T.) ;
#48962=EDGE_CURVE('',#38802,#38800,#32344,.T.) ;
#48963=EDGE_CURVE('',#38803,#38802,#32345,.T.) ;
#48964=EDGE_CURVE('',#38803,#38801,#32346,.T.) ;
#48965=EDGE_CURVE('',#38804,#38797,#32347,.T.) ;
#48966=EDGE_CURVE('',#38804,#38805,#2211,.T.) ;
#48967=EDGE_CURVE('',#38806,#38805,#32348,.T.) ;
#48968=EDGE_CURVE('',#38797,#38806,#2212,.T.) ;
#48969=EDGE_CURVE('',#38807,#38808,#32349,.T.) ;
#48970=EDGE_CURVE('',#38809,#38807,#32350,.T.) ;
#48971=EDGE_CURVE('',#38810,#38809,#32351,.T.) ;
#48972=EDGE_CURVE('',#38810,#38808,#32352,.T.) ;
#48973=EDGE_CURVE('',#38811,#38804,#32353,.T.) ;
#48974=EDGE_CURVE('',#38811,#38812,#2213,.T.) ;
#48975=EDGE_CURVE('',#38813,#38812,#32354,.T.) ;
#48976=EDGE_CURVE('',#38804,#38813,#2214,.T.) ;
#48977=EDGE_CURVE('',#38814,#38815,#32355,.T.) ;
#48978=EDGE_CURVE('',#38816,#38814,#32356,.T.) ;
#48979=EDGE_CURVE('',#38817,#38816,#32357,.T.) ;
#48980=EDGE_CURVE('',#38817,#38815,#32358,.T.) ;
#48981=EDGE_CURVE('',#38818,#38811,#32359,.T.) ;
#48982=EDGE_CURVE('',#38818,#38819,#2215,.T.) ;
#48983=EDGE_CURVE('',#38820,#38819,#32360,.T.) ;
#48984=EDGE_CURVE('',#38811,#38820,#2216,.T.) ;
#48985=EDGE_CURVE('',#38805,#38813,#32361,.T.) ;
#48986=EDGE_CURVE('',#38813,#38803,#5769,.T.) ;
#48987=EDGE_CURVE('',#38805,#38802,#5770,.T.) ;
#48988=EDGE_CURVE('',#38798,#38806,#32362,.T.) ;
#48989=EDGE_CURVE('',#38806,#38796,#5771,.T.) ;
#48990=EDGE_CURVE('',#38798,#38795,#5772,.T.) ;
#48991=EDGE_CURVE('',#38791,#38799,#32363,.T.) ;
#48992=EDGE_CURVE('',#38799,#38789,#5773,.T.) ;
#48993=EDGE_CURVE('',#38791,#38788,#5774,.T.) ;
#48994=EDGE_CURVE('',#38784,#38792,#32364,.T.) ;
#48995=EDGE_CURVE('',#38792,#38782,#5775,.T.) ;
#48996=EDGE_CURVE('',#38784,#38781,#5776,.T.) ;
#48997=EDGE_CURVE('',#38777,#38785,#32365,.T.) ;
#48998=EDGE_CURVE('',#38785,#38775,#5777,.T.) ;
#48999=EDGE_CURVE('',#38777,#38774,#5778,.T.) ;
#49000=EDGE_CURVE('',#38770,#38778,#32366,.T.) ;
#49001=EDGE_CURVE('',#38778,#38768,#5779,.T.) ;
#49002=EDGE_CURVE('',#38770,#38767,#5780,.T.) ;
#49003=EDGE_CURVE('',#38763,#38771,#32367,.T.) ;
#49004=EDGE_CURVE('',#38771,#38761,#5781,.T.) ;
#49005=EDGE_CURVE('',#38763,#38760,#5782,.T.) ;
#49006=EDGE_CURVE('',#38821,#38821,#32368,.T.) ;
#49007=EDGE_CURVE('',#38821,#38822,#32369,.T.) ;
#49008=EDGE_CURVE('',#38822,#38822,#32370,.T.) ;
#49009=EDGE_CURVE('',#38823,#38823,#32371,.T.) ;
#49010=EDGE_CURVE('',#38823,#38824,#32372,.T.) ;
#49011=EDGE_CURVE('',#38824,#38824,#32373,.T.) ;
#49012=EDGE_CURVE('',#38825,#38825,#32374,.T.) ;
#49013=EDGE_CURVE('',#38825,#38826,#32375,.T.) ;
#49014=EDGE_CURVE('',#38826,#38826,#32376,.T.) ;
#49015=EDGE_CURVE('',#38827,#38827,#32377,.T.) ;
#49016=EDGE_CURVE('',#38827,#38828,#32378,.T.) ;
#49017=EDGE_CURVE('',#38828,#38828,#32379,.T.) ;
#49018=EDGE_CURVE('',#38829,#38829,#32380,.T.) ;
#49019=EDGE_CURVE('',#38829,#38830,#32381,.T.) ;
#49020=EDGE_CURVE('',#38830,#38830,#32382,.T.) ;
#49021=EDGE_CURVE('',#38831,#38831,#32383,.T.) ;
#49022=EDGE_CURVE('',#38831,#38832,#32384,.T.) ;
#49023=EDGE_CURVE('',#38832,#38832,#32385,.T.) ;
#49024=EDGE_CURVE('',#38833,#38833,#32386,.T.) ;
#49025=EDGE_CURVE('',#38833,#38834,#32387,.T.) ;
#49026=EDGE_CURVE('',#38834,#38834,#32388,.T.) ;
#49027=EDGE_CURVE('',#38835,#38835,#32389,.T.) ;
#49028=EDGE_CURVE('',#38835,#38836,#32390,.T.) ;
#49029=EDGE_CURVE('',#38836,#38836,#32391,.T.) ;
#49030=EDGE_CURVE('',#38837,#38837,#32392,.T.) ;
#49031=EDGE_CURVE('',#38837,#38838,#32393,.T.) ;
#49032=EDGE_CURVE('',#38838,#38838,#32394,.T.) ;
#49033=EDGE_CURVE('',#38839,#38839,#32395,.T.) ;
#49034=EDGE_CURVE('',#38839,#38840,#32396,.T.) ;
#49035=EDGE_CURVE('',#38840,#38840,#32397,.T.) ;
#49036=EDGE_CURVE('',#38841,#38841,#32398,.T.) ;
#49037=EDGE_CURVE('',#38841,#38842,#32399,.T.) ;
#49038=EDGE_CURVE('',#38842,#38842,#32400,.T.) ;
#49039=EDGE_CURVE('',#38843,#38843,#32401,.T.) ;
#49040=EDGE_CURVE('',#38843,#38844,#32402,.T.) ;
#49041=EDGE_CURVE('',#38844,#38844,#32403,.T.) ;
#49042=EDGE_CURVE('',#38845,#38845,#32404,.T.) ;
#49043=EDGE_CURVE('',#38845,#38846,#32405,.T.) ;
#49044=EDGE_CURVE('',#38846,#38846,#32406,.T.) ;
#49045=EDGE_CURVE('',#38847,#38847,#32407,.T.) ;
#49046=EDGE_CURVE('',#38847,#38848,#32408,.T.) ;
#49047=EDGE_CURVE('',#38848,#38848,#32409,.T.) ;
#49048=EDGE_CURVE('',#38849,#38849,#32410,.T.) ;
#49049=EDGE_CURVE('',#38849,#38850,#32411,.T.) ;
#49050=EDGE_CURVE('',#38850,#38850,#32412,.T.) ;
#49051=EDGE_CURVE('',#38851,#38851,#32413,.T.) ;
#49052=EDGE_CURVE('',#38851,#38852,#32414,.T.) ;
#49053=EDGE_CURVE('',#38852,#38852,#32415,.T.) ;
#49054=EDGE_CURVE('',#38853,#38853,#32416,.T.) ;
#49055=EDGE_CURVE('',#38853,#38854,#32417,.T.) ;
#49056=EDGE_CURVE('',#38854,#38854,#32418,.T.) ;
#49057=EDGE_CURVE('',#38855,#38855,#32419,.T.) ;
#49058=EDGE_CURVE('',#38855,#38856,#32420,.T.) ;
#49059=EDGE_CURVE('',#38856,#38856,#32421,.T.) ;
#49060=EDGE_CURVE('',#38857,#38857,#32422,.T.) ;
#49061=EDGE_CURVE('',#38857,#38858,#32423,.T.) ;
#49062=EDGE_CURVE('',#38858,#38858,#32424,.T.) ;
#49063=EDGE_CURVE('',#38859,#38859,#32425,.T.) ;
#49064=EDGE_CURVE('',#38859,#38860,#32426,.T.) ;
#49065=EDGE_CURVE('',#38860,#38860,#32427,.T.) ;
#49066=EDGE_CURVE('',#38861,#38861,#32428,.T.) ;
#49067=EDGE_CURVE('',#38861,#38862,#32429,.T.) ;
#49068=EDGE_CURVE('',#38862,#38862,#32430,.T.) ;
#49069=EDGE_CURVE('',#38863,#38863,#32431,.T.) ;
#49070=EDGE_CURVE('',#38863,#38864,#32432,.T.) ;
#49071=EDGE_CURVE('',#38864,#38864,#32433,.T.) ;
#49072=EDGE_CURVE('',#38865,#38865,#32434,.T.) ;
#49073=EDGE_CURVE('',#38865,#38866,#32435,.T.) ;
#49074=EDGE_CURVE('',#38866,#38866,#32436,.T.) ;
#49075=EDGE_CURVE('',#38867,#38867,#32437,.T.) ;
#49076=EDGE_CURVE('',#38867,#38868,#32438,.T.) ;
#49077=EDGE_CURVE('',#38868,#38868,#32439,.T.) ;
#49078=EDGE_CURVE('',#38869,#38869,#32440,.T.) ;
#49079=EDGE_CURVE('',#38869,#38870,#32441,.T.) ;
#49080=EDGE_CURVE('',#38870,#38870,#32442,.T.) ;
#49081=EDGE_CURVE('',#38871,#38871,#32443,.T.) ;
#49082=EDGE_CURVE('',#38871,#38872,#32444,.T.) ;
#49083=EDGE_CURVE('',#38872,#38872,#32445,.T.) ;
#49084=EDGE_CURVE('',#38873,#38873,#32446,.T.) ;
#49085=EDGE_CURVE('',#38873,#38874,#32447,.T.) ;
#49086=EDGE_CURVE('',#38874,#38874,#32448,.T.) ;
#49087=EDGE_CURVE('',#38875,#38876,#32449,.T.) ;
#49088=EDGE_CURVE('',#38875,#38877,#2217,.T.) ;
#49089=EDGE_CURVE('',#38878,#38877,#5783,.T.) ;
#49090=EDGE_CURVE('',#38878,#38879,#2218,.T.) ;
#49091=EDGE_CURVE('',#38880,#38879,#32450,.T.) ;
#49092=EDGE_CURVE('',#38880,#38881,#2219,.T.) ;
#49093=EDGE_CURVE('',#38881,#38882,#5784,.T.) ;
#49094=EDGE_CURVE('',#38882,#38883,#2220,.T.) ;
#49095=EDGE_CURVE('',#38884,#38883,#32451,.T.) ;
#49096=EDGE_CURVE('',#38884,#38885,#2221,.T.) ;
#49097=EDGE_CURVE('',#38886,#38885,#5785,.T.) ;
#49098=EDGE_CURVE('',#38886,#38887,#2222,.T.) ;
#49099=EDGE_CURVE('',#38888,#38887,#32452,.T.) ;
#49100=EDGE_CURVE('',#38888,#38889,#2223,.T.) ;
#49101=EDGE_CURVE('',#38889,#38890,#5786,.T.) ;
#49102=EDGE_CURVE('',#38890,#38891,#2224,.T.) ;
#49103=EDGE_CURVE('',#38876,#38891,#32453,.T.) ;
#49104=EDGE_CURVE('',#38876,#38871,#5787,.T.) ;
#49105=EDGE_CURVE('',#38892,#38893,#32454,.T.) ;
#49106=EDGE_CURVE('',#38892,#38894,#2225,.T.) ;
#49107=EDGE_CURVE('',#38895,#38894,#5788,.T.) ;
#49108=EDGE_CURVE('',#38895,#38896,#2226,.T.) ;
#49109=EDGE_CURVE('',#38897,#38896,#32455,.T.) ;
#49110=EDGE_CURVE('',#38897,#38898,#2227,.T.) ;
#49111=EDGE_CURVE('',#38898,#38899,#5789,.T.) ;
#49112=EDGE_CURVE('',#38899,#38900,#2228,.T.) ;
#49113=EDGE_CURVE('',#38901,#38900,#32456,.T.) ;
#49114=EDGE_CURVE('',#38901,#38902,#2229,.T.) ;
#49115=EDGE_CURVE('',#38903,#38902,#5790,.T.) ;
#49116=EDGE_CURVE('',#38903,#38904,#2230,.T.) ;
#49117=EDGE_CURVE('',#38905,#38904,#32457,.T.) ;
#49118=EDGE_CURVE('',#38905,#38906,#2231,.T.) ;
#49119=EDGE_CURVE('',#38906,#38907,#5791,.T.) ;
#49120=EDGE_CURVE('',#38907,#38908,#2232,.T.) ;
#49121=EDGE_CURVE('',#38893,#38908,#32458,.T.) ;
#49122=EDGE_CURVE('',#38893,#38865,#5792,.T.) ;
#49123=EDGE_CURVE('',#38909,#38910,#32459,.T.) ;
#49124=EDGE_CURVE('',#38909,#38911,#2233,.T.) ;
#49125=EDGE_CURVE('',#38912,#38911,#5793,.T.) ;
#49126=EDGE_CURVE('',#38912,#38913,#2234,.T.) ;
#49127=EDGE_CURVE('',#38914,#38913,#32460,.T.) ;
#49128=EDGE_CURVE('',#38914,#38915,#2235,.T.) ;
#49129=EDGE_CURVE('',#38915,#38916,#5794,.T.) ;
#49130=EDGE_CURVE('',#38916,#38917,#2236,.T.) ;
#49131=EDGE_CURVE('',#38918,#38917,#32461,.T.) ;
#49132=EDGE_CURVE('',#38918,#38919,#2237,.T.) ;
#49133=EDGE_CURVE('',#38920,#38919,#5795,.T.) ;
#49134=EDGE_CURVE('',#38920,#38921,#2238,.T.) ;
#49135=EDGE_CURVE('',#38922,#38921,#32462,.T.) ;
#49136=EDGE_CURVE('',#38922,#38923,#2239,.T.) ;
#49137=EDGE_CURVE('',#38923,#38924,#5796,.T.) ;
#49138=EDGE_CURVE('',#38924,#38925,#2240,.T.) ;
#49139=EDGE_CURVE('',#38910,#38925,#32463,.T.) ;
#49140=EDGE_CURVE('',#38910,#38859,#5797,.T.) ;
#49141=EDGE_CURVE('',#38926,#38927,#32464,.T.) ;
#49142=EDGE_CURVE('',#38926,#38928,#2241,.T.) ;
#49143=EDGE_CURVE('',#38929,#38928,#5798,.T.) ;
#49144=EDGE_CURVE('',#38929,#38930,#2242,.T.) ;
#49145=EDGE_CURVE('',#38931,#38930,#32465,.T.) ;
#49146=EDGE_CURVE('',#38931,#38932,#2243,.T.) ;
#49147=EDGE_CURVE('',#38932,#38933,#5799,.T.) ;
#49148=EDGE_CURVE('',#38933,#38934,#2244,.T.) ;
#49149=EDGE_CURVE('',#38935,#38934,#32466,.T.) ;
#49150=EDGE_CURVE('',#38935,#38936,#2245,.T.) ;
#49151=EDGE_CURVE('',#38937,#38936,#5800,.T.) ;
#49152=EDGE_CURVE('',#38937,#38938,#2246,.T.) ;
#49153=EDGE_CURVE('',#38939,#38938,#32467,.T.) ;
#49154=EDGE_CURVE('',#38939,#38940,#2247,.T.) ;
#49155=EDGE_CURVE('',#38940,#38941,#5801,.T.) ;
#49156=EDGE_CURVE('',#38941,#38942,#2248,.T.) ;
#49157=EDGE_CURVE('',#38927,#38942,#32468,.T.) ;
#49158=EDGE_CURVE('',#38927,#38853,#5802,.T.) ;
#49159=EDGE_CURVE('',#38943,#38944,#32469,.T.) ;
#49160=EDGE_CURVE('',#38943,#38945,#2249,.T.) ;
#49161=EDGE_CURVE('',#38946,#38945,#5803,.T.) ;
#49162=EDGE_CURVE('',#38946,#38947,#2250,.T.) ;
#49163=EDGE_CURVE('',#38948,#38947,#32470,.T.) ;
#49164=EDGE_CURVE('',#38948,#38949,#2251,.T.) ;
#49165=EDGE_CURVE('',#38949,#38950,#5804,.T.) ;
#49166=EDGE_CURVE('',#38950,#38951,#2252,.T.) ;
#49167=EDGE_CURVE('',#38952,#38951,#32471,.T.) ;
#49168=EDGE_CURVE('',#38952,#38953,#2253,.T.) ;
#49169=EDGE_CURVE('',#38954,#38953,#5805,.T.) ;
#49170=EDGE_CURVE('',#38954,#38955,#2254,.T.) ;
#49171=EDGE_CURVE('',#38956,#38955,#32472,.T.) ;
#49172=EDGE_CURVE('',#38956,#38957,#2255,.T.) ;
#49173=EDGE_CURVE('',#38957,#38958,#5806,.T.) ;
#49174=EDGE_CURVE('',#38958,#38959,#2256,.T.) ;
#49175=EDGE_CURVE('',#38944,#38959,#32473,.T.) ;
#49176=EDGE_CURVE('',#38944,#38847,#5807,.T.) ;
#49177=EDGE_CURVE('',#38960,#38961,#32474,.T.) ;
#49178=EDGE_CURVE('',#38960,#38962,#2257,.T.) ;
#49179=EDGE_CURVE('',#38963,#38962,#5808,.T.) ;
#49180=EDGE_CURVE('',#38963,#38964,#2258,.T.) ;
#49181=EDGE_CURVE('',#38965,#38964,#32475,.T.) ;
#49182=EDGE_CURVE('',#38965,#38966,#2259,.T.) ;
#49183=EDGE_CURVE('',#38966,#38967,#5809,.T.) ;
#49184=EDGE_CURVE('',#38967,#38968,#2260,.T.) ;
#49185=EDGE_CURVE('',#38969,#38968,#32476,.T.) ;
#49186=EDGE_CURVE('',#38969,#38970,#2261,.T.) ;
#49187=EDGE_CURVE('',#38971,#38970,#5810,.T.) ;
#49188=EDGE_CURVE('',#38971,#38972,#2262,.T.) ;
#49189=EDGE_CURVE('',#38973,#38972,#32477,.T.) ;
#49190=EDGE_CURVE('',#38973,#38974,#2263,.T.) ;
#49191=EDGE_CURVE('',#38974,#38975,#5811,.T.) ;
#49192=EDGE_CURVE('',#38975,#38976,#2264,.T.) ;
#49193=EDGE_CURVE('',#38961,#38976,#32478,.T.) ;
#49194=EDGE_CURVE('',#38961,#38841,#5812,.T.) ;
#49195=EDGE_CURVE('',#38977,#38978,#32479,.T.) ;
#49196=EDGE_CURVE('',#38977,#38979,#2265,.T.) ;
#49197=EDGE_CURVE('',#38980,#38979,#5813,.T.) ;
#49198=EDGE_CURVE('',#38980,#38981,#2266,.T.) ;
#49199=EDGE_CURVE('',#38982,#38981,#32480,.T.) ;
#49200=EDGE_CURVE('',#38982,#38983,#2267,.T.) ;
#49201=EDGE_CURVE('',#38983,#38984,#5814,.T.) ;
#49202=EDGE_CURVE('',#38984,#38985,#2268,.T.) ;
#49203=EDGE_CURVE('',#38986,#38985,#32481,.T.) ;
#49204=EDGE_CURVE('',#38986,#38987,#2269,.T.) ;
#49205=EDGE_CURVE('',#38988,#38987,#5815,.T.) ;
#49206=EDGE_CURVE('',#38988,#38989,#2270,.T.) ;
#49207=EDGE_CURVE('',#38990,#38989,#32482,.T.) ;
#49208=EDGE_CURVE('',#38990,#38991,#2271,.T.) ;
#49209=EDGE_CURVE('',#38991,#38992,#5816,.T.) ;
#49210=EDGE_CURVE('',#38992,#38993,#2272,.T.) ;
#49211=EDGE_CURVE('',#38978,#38993,#32483,.T.) ;
#49212=EDGE_CURVE('',#38978,#38835,#5817,.T.) ;
#49213=EDGE_CURVE('',#38994,#38995,#32484,.T.) ;
#49214=EDGE_CURVE('',#38994,#38996,#2273,.T.) ;
#49215=EDGE_CURVE('',#38997,#38996,#5818,.T.) ;
#49216=EDGE_CURVE('',#38997,#38998,#2274,.T.) ;
#49217=EDGE_CURVE('',#38999,#38998,#32485,.T.) ;
#49218=EDGE_CURVE('',#38999,#39000,#2275,.T.) ;
#49219=EDGE_CURVE('',#39000,#39001,#5819,.T.) ;
#49220=EDGE_CURVE('',#39001,#39002,#2276,.T.) ;
#49221=EDGE_CURVE('',#39003,#39002,#32486,.T.) ;
#49222=EDGE_CURVE('',#39003,#39004,#2277,.T.) ;
#49223=EDGE_CURVE('',#39005,#39004,#5820,.T.) ;
#49224=EDGE_CURVE('',#39005,#39006,#2278,.T.) ;
#49225=EDGE_CURVE('',#39007,#39006,#32487,.T.) ;
#49226=EDGE_CURVE('',#39007,#39008,#2279,.T.) ;
#49227=EDGE_CURVE('',#39008,#39009,#5821,.T.) ;
#49228=EDGE_CURVE('',#39009,#39010,#2280,.T.) ;
#49229=EDGE_CURVE('',#38995,#39010,#32488,.T.) ;
#49230=EDGE_CURVE('',#38995,#38829,#5822,.T.) ;
#49231=EDGE_CURVE('',#39011,#39012,#32489,.T.) ;
#49232=EDGE_CURVE('',#39011,#39013,#2281,.T.) ;
#49233=EDGE_CURVE('',#39014,#39013,#5823,.T.) ;
#49234=EDGE_CURVE('',#39014,#39015,#2282,.T.) ;
#49235=EDGE_CURVE('',#39016,#39015,#32490,.T.) ;
#49236=EDGE_CURVE('',#39016,#39017,#2283,.T.) ;
#49237=EDGE_CURVE('',#39017,#39018,#5824,.T.) ;
#49238=EDGE_CURVE('',#39018,#39019,#2284,.T.) ;
#49239=EDGE_CURVE('',#39020,#39019,#32491,.T.) ;
#49240=EDGE_CURVE('',#39020,#39021,#2285,.T.) ;
#49241=EDGE_CURVE('',#39022,#39021,#5825,.T.) ;
#49242=EDGE_CURVE('',#39022,#39023,#2286,.T.) ;
#49243=EDGE_CURVE('',#39024,#39023,#32492,.T.) ;
#49244=EDGE_CURVE('',#39024,#39025,#2287,.T.) ;
#49245=EDGE_CURVE('',#39025,#39026,#5826,.T.) ;
#49246=EDGE_CURVE('',#39026,#39027,#2288,.T.) ;
#49247=EDGE_CURVE('',#39012,#39027,#32493,.T.) ;
#49248=EDGE_CURVE('',#39012,#38823,#5827,.T.) ;
#49249=EDGE_CURVE('',#39028,#39028,#32494,.T.) ;
#49250=EDGE_CURVE('',#39028,#38821,#5828,.T.) ;
#49251=EDGE_CURVE('',#39029,#39029,#32495,.T.) ;
#49252=EDGE_CURVE('',#39029,#38827,#5829,.T.) ;
#49253=EDGE_CURVE('',#39030,#39030,#32496,.T.) ;
#49254=EDGE_CURVE('',#39030,#38833,#5830,.T.) ;
#49255=EDGE_CURVE('',#39031,#39031,#32497,.T.) ;
#49256=EDGE_CURVE('',#39031,#38839,#5831,.T.) ;
#49257=EDGE_CURVE('',#39032,#39032,#32498,.T.) ;
#49258=EDGE_CURVE('',#39032,#38845,#5832,.T.) ;
#49259=EDGE_CURVE('',#39033,#39033,#32499,.T.) ;
#49260=EDGE_CURVE('',#39033,#38851,#5833,.T.) ;
#49261=EDGE_CURVE('',#39034,#39034,#32500,.T.) ;
#49262=EDGE_CURVE('',#39034,#38857,#5834,.T.) ;
#49263=EDGE_CURVE('',#39035,#39035,#32501,.T.) ;
#49264=EDGE_CURVE('',#39035,#38863,#5835,.T.) ;
#49265=EDGE_CURVE('',#39036,#39036,#32502,.T.) ;
#49266=EDGE_CURVE('',#39036,#38869,#5836,.T.) ;
#49267=EDGE_CURVE('',#38870,#38873,#5837,.T.) ;
#49268=EDGE_CURVE('',#38864,#38867,#5838,.T.) ;
#49269=EDGE_CURVE('',#38858,#38861,#5839,.T.) ;
#49270=EDGE_CURVE('',#38852,#38855,#5840,.T.) ;
#49271=EDGE_CURVE('',#38846,#38849,#5841,.T.) ;
#49272=EDGE_CURVE('',#38840,#38843,#5842,.T.) ;
#49273=EDGE_CURVE('',#38834,#38837,#5843,.T.) ;
#49274=EDGE_CURVE('',#38828,#38831,#5844,.T.) ;
#49275=EDGE_CURVE('',#38822,#38825,#5845,.T.) ;
#49276=EDGE_CURVE('',#39037,#39037,#32503,.T.) ;
#49277=EDGE_CURVE('',#39037,#39038,#32504,.T.) ;
#49278=EDGE_CURVE('',#39038,#39038,#32505,.T.) ;
#49279=EDGE_CURVE('',#39039,#39039,#32506,.T.) ;
#49280=EDGE_CURVE('',#39039,#39040,#32507,.T.) ;
#49281=EDGE_CURVE('',#39040,#39040,#32508,.T.) ;
#49282=EDGE_CURVE('',#39041,#39041,#32509,.T.) ;
#49283=EDGE_CURVE('',#39041,#39042,#32510,.T.) ;
#49284=EDGE_CURVE('',#39042,#39042,#32511,.T.) ;
#49285=EDGE_CURVE('',#38812,#38820,#32512,.T.) ;
#49286=EDGE_CURVE('',#38820,#38810,#5846,.T.) ;
#49287=EDGE_CURVE('',#38812,#38809,#5847,.T.) ;
#49288=EDGE_CURVE('',#38819,#39043,#32513,.T.) ;
#49289=EDGE_CURVE('',#39043,#38817,#5848,.T.) ;
#49290=EDGE_CURVE('',#38819,#38816,#5849,.T.) ;
#49291=EDGE_CURVE('',#39044,#38757,#32514,.T.) ;
#49292=EDGE_CURVE('',#38757,#38749,#5850,.T.) ;
#49293=EDGE_CURVE('',#39044,#38748,#5851,.T.) ;
#49294=EDGE_CURVE('',#38756,#38764,#32515,.T.) ;
#49295=EDGE_CURVE('',#38764,#38753,#5852,.T.) ;
#49296=EDGE_CURVE('',#38756,#38752,#5853,.T.) ;
#49297=EDGE_CURVE('',#39045,#39046,#32516,.T.) ;
#49298=EDGE_CURVE('',#39045,#39047,#2289,.T.) ;
#49299=EDGE_CURVE('',#39048,#39047,#5854,.T.) ;
#49300=EDGE_CURVE('',#39048,#39049,#2290,.T.) ;
#49301=EDGE_CURVE('',#39050,#39049,#32517,.T.) ;
#49302=EDGE_CURVE('',#39050,#39051,#2291,.T.) ;
#49303=EDGE_CURVE('',#39051,#39052,#5855,.T.) ;
#49304=EDGE_CURVE('',#39052,#39053,#2292,.T.) ;
#49305=EDGE_CURVE('',#39054,#39053,#32518,.T.) ;
#49306=EDGE_CURVE('',#39054,#39055,#2293,.T.) ;
#49307=EDGE_CURVE('',#39056,#39055,#5856,.T.) ;
#49308=EDGE_CURVE('',#39056,#39057,#2294,.T.) ;
#49309=EDGE_CURVE('',#39058,#39057,#32519,.T.) ;
#49310=EDGE_CURVE('',#39058,#39059,#2295,.T.) ;
#49311=EDGE_CURVE('',#39059,#39060,#5857,.T.) ;
#49312=EDGE_CURVE('',#39060,#39061,#2296,.T.) ;
#49313=EDGE_CURVE('',#39046,#39061,#32520,.T.) ;
#49314=EDGE_CURVE('',#39046,#39039,#5858,.T.) ;
#49315=EDGE_CURVE('',#39062,#39062,#32521,.T.) ;
#49316=EDGE_CURVE('',#39062,#39037,#5859,.T.) ;
#49317=EDGE_CURVE('',#39038,#39041,#5860,.T.) ;
#49318=EDGE_CURVE('',#39063,#39064,#5861,.T.) ;
#49319=EDGE_CURVE('',#39064,#39065,#5862,.T.) ;
#49320=EDGE_CURVE('',#39065,#39066,#5863,.T.) ;
#49321=EDGE_CURVE('',#39066,#38746,#5864,.T.) ;
#49322=EDGE_CURVE('',#38747,#38750,#32522,.T.) ;
#49323=EDGE_CURVE('',#38751,#38758,#32523,.T.) ;
#49324=EDGE_CURVE('',#38759,#38765,#32524,.T.) ;
#49325=EDGE_CURVE('',#38766,#38772,#32525,.T.) ;
#49326=EDGE_CURVE('',#38773,#38779,#32526,.T.) ;
#49327=EDGE_CURVE('',#38780,#38786,#32527,.T.) ;
#49328=EDGE_CURVE('',#38787,#38793,#32528,.T.) ;
#49329=EDGE_CURVE('',#38794,#38800,#32529,.T.) ;
#49330=EDGE_CURVE('',#38801,#38807,#32530,.T.) ;
#49331=EDGE_CURVE('',#38808,#38814,#32531,.T.) ;
#49332=EDGE_CURVE('',#38815,#39067,#5865,.T.) ;
#49333=EDGE_CURVE('',#39067,#39068,#5866,.T.) ;
#49334=EDGE_CURVE('',#39068,#39063,#5867,.T.) ;
#49335=EDGE_CURVE('',#39069,#39070,#32532,.T.) ;
#49336=EDGE_CURVE('',#39069,#39071,#5868,.T.) ;
#49337=EDGE_CURVE('',#39072,#39071,#32533,.T.) ;
#49338=EDGE_CURVE('',#39072,#39073,#5869,.T.) ;
#49339=EDGE_CURVE('',#39074,#39073,#32534,.T.) ;
#49340=EDGE_CURVE('',#39074,#39075,#5870,.T.) ;
#49341=EDGE_CURVE('',#39076,#39075,#32535,.T.) ;
#49342=EDGE_CURVE('',#39076,#39070,#5871,.T.) ;
#49343=EDGE_CURVE('',#39077,#39078,#32536,.T.) ;
#49344=EDGE_CURVE('',#39077,#39079,#5872,.T.) ;
#49345=EDGE_CURVE('',#39080,#39079,#32537,.T.) ;
#49346=EDGE_CURVE('',#39080,#39081,#5873,.T.) ;
#49347=EDGE_CURVE('',#39082,#39081,#32538,.T.) ;
#49348=EDGE_CURVE('',#39082,#39083,#5874,.T.) ;
#49349=EDGE_CURVE('',#39084,#39083,#32539,.T.) ;
#49350=EDGE_CURVE('',#39084,#39078,#5875,.T.) ;
#49351=EDGE_CURVE('',#39085,#39086,#32540,.T.) ;
#49352=EDGE_CURVE('',#39085,#39087,#5876,.T.) ;
#49353=EDGE_CURVE('',#39088,#39087,#32541,.T.) ;
#49354=EDGE_CURVE('',#39088,#39089,#5877,.T.) ;
#49355=EDGE_CURVE('',#39090,#39089,#32542,.T.) ;
#49356=EDGE_CURVE('',#39090,#39091,#5878,.T.) ;
#49357=EDGE_CURVE('',#39092,#39091,#32543,.T.) ;
#49358=EDGE_CURVE('',#39092,#39086,#5879,.T.) ;
#49359=EDGE_CURVE('',#39093,#39094,#32544,.T.) ;
#49360=EDGE_CURVE('',#39093,#39095,#5880,.T.) ;
#49361=EDGE_CURVE('',#39096,#39095,#32545,.T.) ;
#49362=EDGE_CURVE('',#39096,#39097,#5881,.T.) ;
#49363=EDGE_CURVE('',#39098,#39097,#32546,.T.) ;
#49364=EDGE_CURVE('',#39098,#39099,#5882,.T.) ;
#49365=EDGE_CURVE('',#39100,#39099,#32547,.T.) ;
#49366=EDGE_CURVE('',#39100,#39094,#5883,.T.) ;
#49367=EDGE_CURVE('',#39101,#39102,#32548,.T.) ;
#49368=EDGE_CURVE('',#39101,#39103,#5884,.T.) ;
#49369=EDGE_CURVE('',#39104,#39103,#32549,.T.) ;
#49370=EDGE_CURVE('',#39104,#39105,#5885,.T.) ;
#49371=EDGE_CURVE('',#39106,#39105,#32550,.T.) ;
#49372=EDGE_CURVE('',#39106,#39107,#5886,.T.) ;
#49373=EDGE_CURVE('',#39108,#39107,#32551,.T.) ;
#49374=EDGE_CURVE('',#39108,#39102,#5887,.T.) ;
#49375=EDGE_CURVE('',#39109,#39110,#32552,.T.) ;
#49376=EDGE_CURVE('',#39109,#39111,#5888,.T.) ;
#49377=EDGE_CURVE('',#39112,#39111,#32553,.T.) ;
#49378=EDGE_CURVE('',#39112,#39113,#5889,.T.) ;
#49379=EDGE_CURVE('',#39114,#39113,#32554,.T.) ;
#49380=EDGE_CURVE('',#39114,#39115,#5890,.T.) ;
#49381=EDGE_CURVE('',#39116,#39115,#32555,.T.) ;
#49382=EDGE_CURVE('',#39116,#39110,#5891,.T.) ;
#49383=EDGE_CURVE('',#39117,#39118,#32556,.T.) ;
#49384=EDGE_CURVE('',#39117,#39119,#5892,.T.) ;
#49385=EDGE_CURVE('',#39120,#39119,#32557,.T.) ;
#49386=EDGE_CURVE('',#39120,#39121,#5893,.T.) ;
#49387=EDGE_CURVE('',#39122,#39121,#32558,.T.) ;
#49388=EDGE_CURVE('',#39122,#39123,#5894,.T.) ;
#49389=EDGE_CURVE('',#39124,#39123,#32559,.T.) ;
#49390=EDGE_CURVE('',#39124,#39118,#5895,.T.) ;
#49391=EDGE_CURVE('',#39125,#39126,#32560,.T.) ;
#49392=EDGE_CURVE('',#39125,#39127,#5896,.T.) ;
#49393=EDGE_CURVE('',#39128,#39127,#32561,.T.) ;
#49394=EDGE_CURVE('',#39128,#39129,#5897,.T.) ;
#49395=EDGE_CURVE('',#39130,#39129,#32562,.T.) ;
#49396=EDGE_CURVE('',#39130,#39131,#5898,.T.) ;
#49397=EDGE_CURVE('',#39132,#39131,#32563,.T.) ;
#49398=EDGE_CURVE('',#39132,#39126,#5899,.T.) ;
#49399=EDGE_CURVE('',#39133,#39134,#32564,.T.) ;
#49400=EDGE_CURVE('',#39133,#39135,#5900,.T.) ;
#49401=EDGE_CURVE('',#39136,#39135,#32565,.T.) ;
#49402=EDGE_CURVE('',#39136,#39137,#5901,.T.) ;
#49403=EDGE_CURVE('',#39138,#39137,#32566,.T.) ;
#49404=EDGE_CURVE('',#39138,#39139,#5902,.T.) ;
#49405=EDGE_CURVE('',#39140,#39139,#32567,.T.) ;
#49406=EDGE_CURVE('',#39140,#39134,#5903,.T.) ;
#49407=EDGE_CURVE('',#39141,#39142,#32568,.T.) ;
#49408=EDGE_CURVE('',#39141,#39143,#5904,.T.) ;
#49409=EDGE_CURVE('',#39144,#39143,#32569,.T.) ;
#49410=EDGE_CURVE('',#39144,#39145,#5905,.T.) ;
#49411=EDGE_CURVE('',#39146,#39145,#32570,.T.) ;
#49412=EDGE_CURVE('',#39146,#39147,#5906,.T.) ;
#49413=EDGE_CURVE('',#39148,#39147,#32571,.T.) ;
#49414=EDGE_CURVE('',#39148,#39142,#5907,.T.) ;
#49415=EDGE_CURVE('',#39149,#39150,#5908,.T.) ;
#49416=EDGE_CURVE('',#39150,#39151,#5909,.T.) ;
#49417=EDGE_CURVE('',#39151,#39152,#5910,.T.) ;
#49418=EDGE_CURVE('',#39152,#39149,#5911,.T.) ;
#49419=EDGE_CURVE('',#39153,#39154,#5912,.T.) ;
#49420=EDGE_CURVE('',#39154,#39155,#32572,.T.) ;
#49421=EDGE_CURVE('',#39155,#39156,#5913,.T.) ;
#49422=EDGE_CURVE('',#39156,#39157,#32573,.T.) ;
#49423=EDGE_CURVE('',#39157,#39158,#5914,.T.) ;
#49424=EDGE_CURVE('',#39158,#39159,#32574,.T.) ;
#49425=EDGE_CURVE('',#39159,#39160,#5915,.T.) ;
#49426=EDGE_CURVE('',#39160,#39153,#32575,.T.) ;
#49427=EDGE_CURVE('',#39161,#39162,#5916,.T.) ;
#49428=EDGE_CURVE('',#39162,#39163,#5917,.T.) ;
#49429=EDGE_CURVE('',#39163,#39164,#5918,.T.) ;
#49430=EDGE_CURVE('',#39164,#39161,#5919,.T.) ;
#49431=EDGE_CURVE('',#39165,#39166,#5920,.T.) ;
#49432=EDGE_CURVE('',#39166,#39167,#32576,.T.) ;
#49433=EDGE_CURVE('',#39167,#39168,#5921,.T.) ;
#49434=EDGE_CURVE('',#39168,#39169,#32577,.T.) ;
#49435=EDGE_CURVE('',#39169,#39170,#5922,.T.) ;
#49436=EDGE_CURVE('',#39170,#39171,#32578,.T.) ;
#49437=EDGE_CURVE('',#39171,#39172,#5923,.T.) ;
#49438=EDGE_CURVE('',#39172,#39165,#32579,.T.) ;
#49439=EDGE_CURVE('',#39173,#39174,#5924,.T.) ;
#49440=EDGE_CURVE('',#39174,#39175,#5925,.T.) ;
#49441=EDGE_CURVE('',#39175,#39176,#5926,.T.) ;
#49442=EDGE_CURVE('',#39176,#39173,#5927,.T.) ;
#49443=EDGE_CURVE('',#39177,#39178,#5928,.T.) ;
#49444=EDGE_CURVE('',#39178,#39179,#32580,.T.) ;
#49445=EDGE_CURVE('',#39179,#39180,#5929,.T.) ;
#49446=EDGE_CURVE('',#39180,#39181,#32581,.T.) ;
#49447=EDGE_CURVE('',#39181,#39182,#5930,.T.) ;
#49448=EDGE_CURVE('',#39182,#39183,#32582,.T.) ;
#49449=EDGE_CURVE('',#39183,#39184,#5931,.T.) ;
#49450=EDGE_CURVE('',#39184,#39177,#32583,.T.) ;
#49451=EDGE_CURVE('',#39185,#39186,#5932,.T.) ;
#49452=EDGE_CURVE('',#39186,#39187,#5933,.T.) ;
#49453=EDGE_CURVE('',#39187,#39188,#5934,.T.) ;
#49454=EDGE_CURVE('',#39188,#39185,#5935,.T.) ;
#49455=EDGE_CURVE('',#39189,#39190,#5936,.T.) ;
#49456=EDGE_CURVE('',#39190,#39191,#32584,.T.) ;
#49457=EDGE_CURVE('',#39191,#39192,#5937,.T.) ;
#49458=EDGE_CURVE('',#39192,#39193,#32585,.T.) ;
#49459=EDGE_CURVE('',#39193,#39194,#5938,.T.) ;
#49460=EDGE_CURVE('',#39194,#39195,#32586,.T.) ;
#49461=EDGE_CURVE('',#39195,#39196,#5939,.T.) ;
#49462=EDGE_CURVE('',#39196,#39189,#32587,.T.) ;
#49463=EDGE_CURVE('',#39197,#39198,#5940,.T.) ;
#49464=EDGE_CURVE('',#39198,#39199,#5941,.T.) ;
#49465=EDGE_CURVE('',#39199,#39200,#5942,.T.) ;
#49466=EDGE_CURVE('',#39200,#39197,#5943,.T.) ;
#49467=EDGE_CURVE('',#39201,#39202,#5944,.T.) ;
#49468=EDGE_CURVE('',#39202,#39203,#32588,.T.) ;
#49469=EDGE_CURVE('',#39203,#39204,#5945,.T.) ;
#49470=EDGE_CURVE('',#39204,#39205,#32589,.T.) ;
#49471=EDGE_CURVE('',#39205,#39206,#5946,.T.) ;
#49472=EDGE_CURVE('',#39206,#39207,#32590,.T.) ;
#49473=EDGE_CURVE('',#39207,#39208,#5947,.T.) ;
#49474=EDGE_CURVE('',#39208,#39201,#32591,.T.) ;
#49475=EDGE_CURVE('',#39209,#39210,#5948,.T.) ;
#49476=EDGE_CURVE('',#39210,#39211,#5949,.T.) ;
#49477=EDGE_CURVE('',#39211,#39212,#5950,.T.) ;
#49478=EDGE_CURVE('',#39212,#39209,#5951,.T.) ;
#49479=EDGE_CURVE('',#39213,#39214,#5952,.T.) ;
#49480=EDGE_CURVE('',#39214,#39215,#32592,.T.) ;
#49481=EDGE_CURVE('',#39215,#39216,#5953,.T.) ;
#49482=EDGE_CURVE('',#39216,#39217,#32593,.T.) ;
#49483=EDGE_CURVE('',#39217,#39218,#5954,.T.) ;
#49484=EDGE_CURVE('',#39218,#39219,#32594,.T.) ;
#49485=EDGE_CURVE('',#39219,#39220,#5955,.T.) ;
#49486=EDGE_CURVE('',#39220,#39213,#32595,.T.) ;
#49487=EDGE_CURVE('',#39221,#39222,#5956,.T.) ;
#49488=EDGE_CURVE('',#39222,#39223,#5957,.T.) ;
#49489=EDGE_CURVE('',#39223,#39224,#5958,.T.) ;
#49490=EDGE_CURVE('',#39224,#39221,#5959,.T.) ;
#49491=EDGE_CURVE('',#39225,#39226,#5960,.T.) ;
#49492=EDGE_CURVE('',#39226,#39227,#32596,.T.) ;
#49493=EDGE_CURVE('',#39227,#39228,#5961,.T.) ;
#49494=EDGE_CURVE('',#39228,#39229,#32597,.T.) ;
#49495=EDGE_CURVE('',#39229,#39230,#5962,.T.) ;
#49496=EDGE_CURVE('',#39230,#39231,#32598,.T.) ;
#49497=EDGE_CURVE('',#39231,#39232,#5963,.T.) ;
#49498=EDGE_CURVE('',#39232,#39225,#32599,.T.) ;
#49499=EDGE_CURVE('',#39233,#39234,#5964,.T.) ;
#49500=EDGE_CURVE('',#39234,#39235,#5965,.T.) ;
#49501=EDGE_CURVE('',#39235,#39236,#5966,.T.) ;
#49502=EDGE_CURVE('',#39236,#39233,#5967,.T.) ;
#49503=EDGE_CURVE('',#39237,#39238,#5968,.T.) ;
#49504=EDGE_CURVE('',#39238,#39239,#32600,.T.) ;
#49505=EDGE_CURVE('',#39239,#39240,#5969,.T.) ;
#49506=EDGE_CURVE('',#39240,#39241,#32601,.T.) ;
#49507=EDGE_CURVE('',#39241,#39242,#5970,.T.) ;
#49508=EDGE_CURVE('',#39242,#39243,#32602,.T.) ;
#49509=EDGE_CURVE('',#39243,#39244,#5971,.T.) ;
#49510=EDGE_CURVE('',#39244,#39237,#32603,.T.) ;
#49511=EDGE_CURVE('',#39245,#39246,#5972,.T.) ;
#49512=EDGE_CURVE('',#39246,#39247,#5973,.T.) ;
#49513=EDGE_CURVE('',#39247,#39248,#5974,.T.) ;
#49514=EDGE_CURVE('',#39248,#39245,#5975,.T.) ;
#49515=EDGE_CURVE('',#39249,#39250,#5976,.T.) ;
#49516=EDGE_CURVE('',#39250,#39251,#32604,.T.) ;
#49517=EDGE_CURVE('',#39251,#39252,#5977,.T.) ;
#49518=EDGE_CURVE('',#39252,#39253,#32605,.T.) ;
#49519=EDGE_CURVE('',#39253,#39254,#5978,.T.) ;
#49520=EDGE_CURVE('',#39254,#39255,#32606,.T.) ;
#49521=EDGE_CURVE('',#39255,#39256,#5979,.T.) ;
#49522=EDGE_CURVE('',#39256,#39249,#32607,.T.) ;
#49523=EDGE_CURVE('',#39019,#39020,#5980,.T.) ;
#49524=EDGE_CURVE('',#39002,#39003,#5981,.T.) ;
#49525=EDGE_CURVE('',#38985,#38986,#5982,.T.) ;
#49526=EDGE_CURVE('',#38968,#38969,#5983,.T.) ;
#49527=EDGE_CURVE('',#38951,#38952,#5984,.T.) ;
#49528=EDGE_CURVE('',#38934,#38935,#5985,.T.) ;
#49529=EDGE_CURVE('',#38917,#38918,#5986,.T.) ;
#49530=EDGE_CURVE('',#38900,#38901,#5987,.T.) ;
#49531=EDGE_CURVE('',#38883,#38884,#5988,.T.) ;
#49532=EDGE_CURVE('',#39257,#39258,#5989,.T.) ;
#49533=EDGE_CURVE('',#39258,#39259,#5990,.T.) ;
#49534=EDGE_CURVE('',#39259,#39260,#5991,.T.) ;
#49535=EDGE_CURVE('',#39260,#39261,#5992,.T.) ;
#49536=EDGE_CURVE('',#39261,#39262,#5993,.T.) ;
#49537=EDGE_CURVE('',#39262,#39263,#32608,.T.) ;
#49538=EDGE_CURVE('',#39263,#39264,#32609,.T.) ;
#49539=EDGE_CURVE('',#39264,#39265,#5994,.T.) ;
#49540=EDGE_CURVE('',#39265,#39266,#32610,.T.) ;
#49541=EDGE_CURVE('',#39266,#39267,#32611,.T.) ;
#49542=EDGE_CURVE('',#39267,#39268,#5995,.T.) ;
#49543=EDGE_CURVE('',#39268,#39269,#32612,.T.) ;
#49544=EDGE_CURVE('',#39269,#39270,#32613,.T.) ;
#49545=EDGE_CURVE('',#39270,#39271,#5996,.T.) ;
#49546=EDGE_CURVE('',#39271,#39272,#32614,.T.) ;
#49547=EDGE_CURVE('',#39272,#39273,#32615,.T.) ;
#49548=EDGE_CURVE('',#39273,#39274,#5997,.T.) ;
#49549=EDGE_CURVE('',#39274,#39275,#32616,.T.) ;
#49550=EDGE_CURVE('',#39275,#39276,#32617,.T.) ;
#49551=EDGE_CURVE('',#39276,#39277,#5998,.T.) ;
#49552=EDGE_CURVE('',#39277,#39278,#32618,.T.) ;
#49553=EDGE_CURVE('',#39278,#39279,#32619,.T.) ;
#49554=EDGE_CURVE('',#39279,#39280,#5999,.T.) ;
#49555=EDGE_CURVE('',#39280,#39281,#32620,.T.) ;
#49556=EDGE_CURVE('',#39281,#39282,#32621,.T.) ;
#49557=EDGE_CURVE('',#39282,#39283,#6000,.T.) ;
#49558=EDGE_CURVE('',#39283,#39284,#32622,.T.) ;
#49559=EDGE_CURVE('',#39284,#39285,#32623,.T.) ;
#49560=EDGE_CURVE('',#39285,#39286,#6001,.T.) ;
#49561=EDGE_CURVE('',#39286,#39287,#32624,.T.) ;
#49562=EDGE_CURVE('',#39287,#39288,#32625,.T.) ;
#49563=EDGE_CURVE('',#39288,#39289,#6002,.T.) ;
#49564=EDGE_CURVE('',#39289,#39290,#32626,.T.) ;
#49565=EDGE_CURVE('',#39290,#39291,#32627,.T.) ;
#49566=EDGE_CURVE('',#39291,#39292,#6003,.T.) ;
#49567=EDGE_CURVE('',#39292,#39293,#32628,.T.) ;
#49568=EDGE_CURVE('',#39293,#39294,#32629,.T.) ;
#49569=EDGE_CURVE('',#39294,#39295,#6004,.T.) ;
#49570=EDGE_CURVE('',#39295,#39296,#32630,.T.) ;
#49571=EDGE_CURVE('',#39296,#39297,#32631,.T.) ;
#49572=EDGE_CURVE('',#39297,#39298,#6005,.T.) ;
#49573=EDGE_CURVE('',#39298,#39299,#32632,.T.) ;
#49574=EDGE_CURVE('',#39299,#39300,#32633,.T.) ;
#49575=EDGE_CURVE('',#39300,#39301,#6006,.T.) ;
#49576=EDGE_CURVE('',#39301,#39302,#32634,.T.) ;
#49577=EDGE_CURVE('',#39302,#39303,#32635,.T.) ;
#49578=EDGE_CURVE('',#39303,#39304,#6007,.T.) ;
#49579=EDGE_CURVE('',#39304,#39305,#32636,.T.) ;
#49580=EDGE_CURVE('',#39305,#39306,#32637,.T.) ;
#49581=EDGE_CURVE('',#39306,#39307,#6008,.T.) ;
#49582=EDGE_CURVE('',#39307,#39308,#32638,.T.) ;
#49583=EDGE_CURVE('',#39308,#39309,#32639,.T.) ;
#49584=EDGE_CURVE('',#39309,#39310,#6009,.T.) ;
#49585=EDGE_CURVE('',#39310,#39311,#32640,.T.) ;
#49586=EDGE_CURVE('',#39311,#39312,#32641,.T.) ;
#49587=EDGE_CURVE('',#39312,#39313,#6010,.T.) ;
#49588=EDGE_CURVE('',#39313,#39314,#32642,.T.) ;
#49589=EDGE_CURVE('',#39314,#39315,#32643,.T.) ;
#49590=EDGE_CURVE('',#39315,#39316,#6011,.T.) ;
#49591=EDGE_CURVE('',#39316,#39317,#32644,.T.) ;
#49592=EDGE_CURVE('',#39317,#39318,#32645,.T.) ;
#49593=EDGE_CURVE('',#39318,#39319,#6012,.T.) ;
#49594=EDGE_CURVE('',#39319,#39320,#32646,.T.) ;
#49595=EDGE_CURVE('',#39320,#39257,#32647,.T.) ;
#49596=EDGE_CURVE('',#39321,#39322,#32648,.T.) ;
#49597=EDGE_CURVE('',#39321,#39323,#6013,.T.) ;
#49598=EDGE_CURVE('',#39323,#39324,#6014,.T.) ;
#49599=EDGE_CURVE('',#39324,#39325,#6015,.T.) ;
#49600=EDGE_CURVE('',#39325,#39326,#6016,.T.) ;
#49601=EDGE_CURVE('',#39326,#39327,#6017,.T.) ;
#49602=EDGE_CURVE('',#39328,#39327,#32649,.T.) ;
#49603=EDGE_CURVE('',#39328,#39322,#32650,.T.) ;
#49604=EDGE_CURVE('',#39329,#39330,#32651,.T.) ;
#49605=EDGE_CURVE('',#39329,#39331,#6018,.T.) ;
#49606=EDGE_CURVE('',#39331,#39332,#6019,.T.) ;
#49607=EDGE_CURVE('',#39332,#39333,#6020,.T.) ;
#49608=EDGE_CURVE('',#39333,#39334,#6021,.T.) ;
#49609=EDGE_CURVE('',#39334,#39335,#6022,.T.) ;
#49610=EDGE_CURVE('',#39336,#39335,#32652,.T.) ;
#49611=EDGE_CURVE('',#39336,#39330,#32653,.T.) ;
#49612=EDGE_CURVE('',#39337,#39338,#32654,.T.) ;
#49613=EDGE_CURVE('',#39337,#39339,#6023,.T.) ;
#49614=EDGE_CURVE('',#39339,#39340,#6024,.T.) ;
#49615=EDGE_CURVE('',#39340,#39341,#6025,.T.) ;
#49616=EDGE_CURVE('',#39341,#39342,#6026,.T.) ;
#49617=EDGE_CURVE('',#39342,#39343,#6027,.T.) ;
#49618=EDGE_CURVE('',#39344,#39343,#32655,.T.) ;
#49619=EDGE_CURVE('',#39344,#39338,#32656,.T.) ;
#49620=EDGE_CURVE('',#39345,#39346,#32657,.T.) ;
#49621=EDGE_CURVE('',#39345,#39347,#6028,.T.) ;
#49622=EDGE_CURVE('',#39347,#39348,#6029,.T.) ;
#49623=EDGE_CURVE('',#39348,#39349,#6030,.T.) ;
#49624=EDGE_CURVE('',#39349,#39350,#6031,.T.) ;
#49625=EDGE_CURVE('',#39350,#39351,#6032,.T.) ;
#49626=EDGE_CURVE('',#39352,#39351,#32658,.T.) ;
#49627=EDGE_CURVE('',#39352,#39346,#32659,.T.) ;
#49628=EDGE_CURVE('',#39353,#39354,#32660,.T.) ;
#49629=EDGE_CURVE('',#39353,#39355,#6033,.T.) ;
#49630=EDGE_CURVE('',#39355,#39356,#6034,.T.) ;
#49631=EDGE_CURVE('',#39356,#39357,#6035,.T.) ;
#49632=EDGE_CURVE('',#39357,#39358,#6036,.T.) ;
#49633=EDGE_CURVE('',#39358,#39359,#6037,.T.) ;
#49634=EDGE_CURVE('',#39360,#39359,#32661,.T.) ;
#49635=EDGE_CURVE('',#39360,#39354,#32662,.T.) ;
#49636=EDGE_CURVE('',#39361,#39362,#32663,.T.) ;
#49637=EDGE_CURVE('',#39361,#39363,#6038,.T.) ;
#49638=EDGE_CURVE('',#39363,#39364,#6039,.T.) ;
#49639=EDGE_CURVE('',#39364,#39365,#6040,.T.) ;
#49640=EDGE_CURVE('',#39365,#39366,#6041,.T.) ;
#49641=EDGE_CURVE('',#39366,#39367,#6042,.T.) ;
#49642=EDGE_CURVE('',#39368,#39367,#32664,.T.) ;
#49643=EDGE_CURVE('',#39368,#39362,#32665,.T.) ;
#49644=EDGE_CURVE('',#39369,#39370,#32666,.T.) ;
#49645=EDGE_CURVE('',#39369,#39371,#6043,.T.) ;
#49646=EDGE_CURVE('',#39371,#39372,#6044,.T.) ;
#49647=EDGE_CURVE('',#39372,#39373,#6045,.T.) ;
#49648=EDGE_CURVE('',#39373,#39374,#6046,.T.) ;
#49649=EDGE_CURVE('',#39374,#39375,#6047,.T.) ;
#49650=EDGE_CURVE('',#39376,#39375,#32667,.T.) ;
#49651=EDGE_CURVE('',#39376,#39370,#32668,.T.) ;
#49652=EDGE_CURVE('',#39377,#39378,#32669,.T.) ;
#49653=EDGE_CURVE('',#39377,#39379,#6048,.T.) ;
#49654=EDGE_CURVE('',#39379,#39380,#6049,.T.) ;
#49655=EDGE_CURVE('',#39380,#39381,#6050,.T.) ;
#49656=EDGE_CURVE('',#39381,#39382,#6051,.T.) ;
#49657=EDGE_CURVE('',#39382,#39383,#6052,.T.) ;
#49658=EDGE_CURVE('',#39384,#39383,#32670,.T.) ;
#49659=EDGE_CURVE('',#39384,#39378,#32671,.T.) ;
#49660=EDGE_CURVE('',#39385,#39386,#32672,.T.) ;
#49661=EDGE_CURVE('',#39385,#39387,#6053,.T.) ;
#49662=EDGE_CURVE('',#39387,#39388,#6054,.T.) ;
#49663=EDGE_CURVE('',#39388,#39389,#6055,.T.) ;
#49664=EDGE_CURVE('',#39389,#39390,#6056,.T.) ;
#49665=EDGE_CURVE('',#39390,#39391,#6057,.T.) ;
#49666=EDGE_CURVE('',#39392,#39391,#32673,.T.) ;
#49667=EDGE_CURVE('',#39392,#39386,#32674,.T.) ;
#49668=EDGE_CURVE('',#39393,#39394,#6058,.T.) ;
#49669=EDGE_CURVE('',#39394,#39395,#6059,.T.) ;
#49670=EDGE_CURVE('',#39395,#39396,#6060,.T.) ;
#49671=EDGE_CURVE('',#39396,#39393,#6061,.T.) ;
#49672=EDGE_CURVE('',#39397,#39398,#6062,.T.) ;
#49673=EDGE_CURVE('',#39398,#39399,#6063,.T.) ;
#49674=EDGE_CURVE('',#39399,#39400,#6064,.T.) ;
#49675=EDGE_CURVE('',#39400,#39401,#6065,.T.) ;
#49676=EDGE_CURVE('',#39402,#39401,#32675,.T.) ;
#49677=EDGE_CURVE('',#39402,#39403,#6066,.T.) ;
#49678=EDGE_CURVE('',#39404,#39403,#32676,.T.) ;
#49679=EDGE_CURVE('',#39404,#39405,#6067,.T.) ;
#49680=EDGE_CURVE('',#39405,#39406,#6068,.T.) ;
#49681=EDGE_CURVE('',#39406,#39407,#6069,.T.) ;
#49682=EDGE_CURVE('',#39408,#39407,#32677,.T.) ;
#49683=EDGE_CURVE('',#39408,#39409,#6070,.T.) ;
#49684=EDGE_CURVE('',#39410,#39409,#32678,.T.) ;
#49685=EDGE_CURVE('',#39410,#39411,#6071,.T.) ;
#49686=EDGE_CURVE('',#39411,#39412,#6072,.T.) ;
#49687=EDGE_CURVE('',#39412,#39413,#6073,.T.) ;
#49688=EDGE_CURVE('',#39414,#39413,#32679,.T.) ;
#49689=EDGE_CURVE('',#39414,#39415,#6074,.T.) ;
#49690=EDGE_CURVE('',#39416,#39415,#32680,.T.) ;
#49691=EDGE_CURVE('',#39416,#39417,#6075,.T.) ;
#49692=EDGE_CURVE('',#39417,#39418,#6076,.T.) ;
#49693=EDGE_CURVE('',#39418,#39419,#6077,.T.) ;
#49694=EDGE_CURVE('',#39420,#39419,#32681,.T.) ;
#49695=EDGE_CURVE('',#39420,#39421,#6078,.T.) ;
#49696=EDGE_CURVE('',#39422,#39421,#32682,.T.) ;
#49697=EDGE_CURVE('',#39422,#39423,#6079,.T.) ;
#49698=EDGE_CURVE('',#39423,#39424,#6080,.T.) ;
#49699=EDGE_CURVE('',#39424,#39425,#6081,.T.) ;
#49700=EDGE_CURVE('',#39426,#39425,#32683,.T.) ;
#49701=EDGE_CURVE('',#39426,#39427,#6082,.T.) ;
#49702=EDGE_CURVE('',#39428,#39427,#32684,.T.) ;
#49703=EDGE_CURVE('',#39428,#39429,#6083,.T.) ;
#49704=EDGE_CURVE('',#39429,#39430,#6084,.T.) ;
#49705=EDGE_CURVE('',#39430,#39431,#6085,.T.) ;
#49706=EDGE_CURVE('',#39432,#39431,#32685,.T.) ;
#49707=EDGE_CURVE('',#39432,#39433,#6086,.T.) ;
#49708=EDGE_CURVE('',#39434,#39433,#32686,.T.) ;
#49709=EDGE_CURVE('',#39434,#39435,#6087,.T.) ;
#49710=EDGE_CURVE('',#39435,#39436,#6088,.T.) ;
#49711=EDGE_CURVE('',#39436,#39437,#6089,.T.) ;
#49712=EDGE_CURVE('',#39438,#39437,#32687,.T.) ;
#49713=EDGE_CURVE('',#39438,#39439,#6090,.T.) ;
#49714=EDGE_CURVE('',#39440,#39439,#32688,.T.) ;
#49715=EDGE_CURVE('',#39440,#39441,#6091,.T.) ;
#49716=EDGE_CURVE('',#39441,#39442,#6092,.T.) ;
#49717=EDGE_CURVE('',#39442,#39443,#6093,.T.) ;
#49718=EDGE_CURVE('',#39444,#39443,#32689,.T.) ;
#49719=EDGE_CURVE('',#39444,#39445,#6094,.T.) ;
#49720=EDGE_CURVE('',#39446,#39445,#32690,.T.) ;
#49721=EDGE_CURVE('',#39446,#39447,#6095,.T.) ;
#49722=EDGE_CURVE('',#39447,#39448,#6096,.T.) ;
#49723=EDGE_CURVE('',#39448,#39449,#6097,.T.) ;
#49724=EDGE_CURVE('',#39450,#39449,#32691,.T.) ;
#49725=EDGE_CURVE('',#39450,#39451,#6098,.T.) ;
#49726=EDGE_CURVE('',#39452,#39451,#32692,.T.) ;
#49727=EDGE_CURVE('',#39452,#39453,#6099,.T.) ;
#49728=EDGE_CURVE('',#39453,#39454,#6100,.T.) ;
#49729=EDGE_CURVE('',#39454,#39455,#6101,.T.) ;
#49730=EDGE_CURVE('',#39456,#39455,#32693,.T.) ;
#49731=EDGE_CURVE('',#39456,#39457,#6102,.T.) ;
#49732=EDGE_CURVE('',#39458,#39457,#32694,.T.) ;
#49733=EDGE_CURVE('',#39458,#39459,#6103,.T.) ;
#49734=EDGE_CURVE('',#39459,#39460,#6104,.T.) ;
#49735=EDGE_CURVE('',#39460,#39397,#6105,.T.) ;
#49736=EDGE_CURVE('',#39461,#39462,#6106,.T.) ;
#49737=EDGE_CURVE('',#39461,#39260,#32695,.T.) ;
#49738=EDGE_CURVE('',#39259,#39462,#32696,.T.) ;
#49739=EDGE_CURVE('',#39463,#39464,#6107,.T.) ;
#49740=EDGE_CURVE('',#39465,#39463,#32697,.T.) ;
#49741=EDGE_CURVE('',#39268,#39465,#32698,.T.) ;
#49742=EDGE_CURVE('',#39466,#39267,#32699,.T.) ;
#49743=EDGE_CURVE('',#39464,#39466,#32700,.T.) ;
#49744=EDGE_CURVE('',#39467,#39468,#6108,.T.) ;
#49745=EDGE_CURVE('',#39468,#39469,#6109,.T.) ;
#49746=EDGE_CURVE('',#39469,#39470,#6110,.T.) ;
#49747=EDGE_CURVE('',#39470,#39467,#6111,.T.) ;
#49748=EDGE_CURVE('',#39471,#39472,#2297,.T.) ;
#49749=EDGE_CURVE('',#39471,#39473,#6112,.T.) ;
#49750=EDGE_CURVE('',#39474,#39473,#2298,.T.) ;
#49751=EDGE_CURVE('',#39474,#39475,#6113,.T.) ;
#49752=EDGE_CURVE('',#39476,#39475,#2299,.T.) ;
#49753=EDGE_CURVE('',#39476,#39477,#6114,.T.) ;
#49754=EDGE_CURVE('',#39478,#39477,#2300,.T.) ;
#49755=EDGE_CURVE('',#39478,#39472,#6115,.T.) ;
#49756=EDGE_CURVE('',#39479,#39480,#6116,.T.) ;
#49757=EDGE_CURVE('',#39480,#39481,#6117,.T.) ;
#49758=EDGE_CURVE('',#39481,#39482,#6118,.T.) ;
#49759=EDGE_CURVE('',#39482,#39479,#6119,.T.) ;
#49760=EDGE_CURVE('',#39483,#39484,#6120,.T.) ;
#49761=EDGE_CURVE('',#39484,#39485,#6121,.T.) ;
#49762=EDGE_CURVE('',#39485,#39486,#6122,.T.) ;
#49763=EDGE_CURVE('',#39486,#39483,#6123,.T.) ;
#49764=EDGE_CURVE('',#39487,#39488,#6124,.T.) ;
#49765=EDGE_CURVE('',#39488,#39489,#6125,.T.) ;
#49766=EDGE_CURVE('',#39489,#39490,#6126,.T.) ;
#49767=EDGE_CURVE('',#39490,#39487,#6127,.T.) ;
#49768=EDGE_CURVE('',#39491,#39492,#6128,.T.) ;
#49769=EDGE_CURVE('',#39492,#39493,#6129,.T.) ;
#49770=EDGE_CURVE('',#39493,#39494,#6130,.T.) ;
#49771=EDGE_CURVE('',#39494,#39491,#6131,.T.) ;
#49772=EDGE_CURVE('',#39495,#39496,#6132,.T.) ;
#49773=EDGE_CURVE('',#39496,#39497,#6133,.T.) ;
#49774=EDGE_CURVE('',#39497,#39498,#6134,.T.) ;
#49775=EDGE_CURVE('',#39498,#39495,#6135,.T.) ;
#49776=EDGE_CURVE('',#39499,#39500,#6136,.T.) ;
#49777=EDGE_CURVE('',#39500,#39501,#6137,.T.) ;
#49778=EDGE_CURVE('',#39501,#39502,#6138,.T.) ;
#49779=EDGE_CURVE('',#39502,#39499,#6139,.T.) ;
#49780=EDGE_CURVE('',#39503,#39504,#6140,.T.) ;
#49781=EDGE_CURVE('',#39504,#39505,#6141,.T.) ;
#49782=EDGE_CURVE('',#39505,#39506,#6142,.T.) ;
#49783=EDGE_CURVE('',#39506,#39503,#6143,.T.) ;
#49784=EDGE_CURVE('',#39507,#39508,#6144,.T.) ;
#49785=EDGE_CURVE('',#39508,#39509,#6145,.T.) ;
#49786=EDGE_CURVE('',#39509,#39510,#6146,.T.) ;
#49787=EDGE_CURVE('',#39510,#39507,#6147,.T.) ;
#49788=EDGE_CURVE('',#39511,#39512,#2301,.T.) ;
#49789=EDGE_CURVE('',#39511,#39513,#6148,.T.) ;
#49790=EDGE_CURVE('',#39514,#39513,#2302,.T.) ;
#49791=EDGE_CURVE('',#39514,#39515,#6149,.T.) ;
#49792=EDGE_CURVE('',#39516,#39515,#2303,.T.) ;
#49793=EDGE_CURVE('',#39516,#39517,#6150,.T.) ;
#49794=EDGE_CURVE('',#39518,#39517,#2304,.T.) ;
#49795=EDGE_CURVE('',#39518,#39512,#6151,.T.) ;
#49796=EDGE_CURVE('',#39519,#39520,#6152,.T.) ;
#49797=EDGE_CURVE('',#39520,#39521,#6153,.T.) ;
#49798=EDGE_CURVE('',#39521,#39522,#6154,.T.) ;
#49799=EDGE_CURVE('',#39522,#39519,#6155,.T.) ;
#49800=EDGE_CURVE('',#39523,#39524,#6156,.T.) ;
#49801=EDGE_CURVE('',#39524,#39525,#32701,.T.) ;
#49802=EDGE_CURVE('',#39525,#39526,#6157,.T.) ;
#49803=EDGE_CURVE('',#39526,#39527,#32702,.T.) ;
#49804=EDGE_CURVE('',#39527,#39528,#6158,.T.) ;
#49805=EDGE_CURVE('',#39528,#39529,#32703,.T.) ;
#49806=EDGE_CURVE('',#39529,#39530,#6159,.T.) ;
#49807=EDGE_CURVE('',#39530,#39523,#32704,.T.) ;
#49808=EDGE_CURVE('',#39531,#39532,#6160,.T.) ;
#49809=EDGE_CURVE('',#39532,#39533,#6161,.T.) ;
#49810=EDGE_CURVE('',#39533,#39534,#6162,.T.) ;
#49811=EDGE_CURVE('',#39534,#39531,#6163,.T.) ;
#49812=EDGE_CURVE('',#39053,#39054,#6164,.T.) ;
#49813=EDGE_CURVE('',#39535,#39536,#6165,.T.) ;
#49814=EDGE_CURVE('',#39536,#39537,#6166,.T.) ;
#49815=EDGE_CURVE('',#39537,#39538,#6167,.T.) ;
#49816=EDGE_CURVE('',#39538,#39539,#6168,.T.) ;
#49817=EDGE_CURVE('',#39540,#39539,#32705,.T.) ;
#49818=EDGE_CURVE('',#39540,#39541,#32706,.T.) ;
#49819=EDGE_CURVE('',#39542,#39541,#32707,.T.) ;
#49820=EDGE_CURVE('',#39542,#39535,#6169,.T.) ;
#49821=EDGE_CURVE('',#39543,#39544,#6170,.T.) ;
#49822=EDGE_CURVE('',#39544,#39545,#6171,.T.) ;
#49823=EDGE_CURVE('',#39545,#39546,#6172,.T.) ;
#49824=EDGE_CURVE('',#39546,#39543,#6173,.T.) ;
#49825=EDGE_CURVE('',#39547,#38744,#6174,.T.) ;
#49826=EDGE_CURVE('',#38742,#39548,#6175,.T.) ;
#49827=EDGE_CURVE('',#39548,#39547,#6176,.T.) ;
#49828=EDGE_CURVE('',#39549,#39550,#6177,.T.) ;
#49829=EDGE_CURVE('',#39550,#39551,#6178,.T.) ;
#49830=EDGE_CURVE('',#39551,#39552,#6179,.T.) ;
#49831=EDGE_CURVE('',#39552,#39549,#6180,.T.) ;
#49832=EDGE_CURVE('',#39553,#39554,#6181,.T.) ;
#49833=EDGE_CURVE('',#39554,#39555,#6182,.T.) ;
#49834=EDGE_CURVE('',#39555,#39556,#6183,.T.) ;
#49835=EDGE_CURVE('',#39556,#39553,#6184,.T.) ;
#49836=EDGE_CURVE('',#39557,#39558,#6185,.T.) ;
#49837=EDGE_CURVE('',#39558,#39559,#6186,.T.) ;
#49838=EDGE_CURVE('',#39559,#39560,#6187,.T.) ;
#49839=EDGE_CURVE('',#39560,#39557,#6188,.T.) ;
#49840=EDGE_CURVE('',#39561,#39562,#6189,.T.) ;
#49841=EDGE_CURVE('',#39562,#39563,#6190,.T.) ;
#49842=EDGE_CURVE('',#39563,#39564,#6191,.T.) ;
#49843=EDGE_CURVE('',#39564,#39561,#6192,.T.) ;
#49844=EDGE_CURVE('',#39565,#39566,#6193,.T.) ;
#49845=EDGE_CURVE('',#39566,#39567,#6194,.T.) ;
#49846=EDGE_CURVE('',#39567,#39568,#6195,.T.) ;
#49847=EDGE_CURVE('',#39568,#39565,#6196,.T.) ;
#49848=EDGE_CURVE('',#39569,#39570,#6197,.T.) ;
#49849=EDGE_CURVE('',#39570,#39571,#6198,.T.) ;
#49850=EDGE_CURVE('',#39571,#39572,#6199,.T.) ;
#49851=EDGE_CURVE('',#39572,#39569,#6200,.T.) ;
#49852=EDGE_CURVE('',#39573,#39574,#6201,.T.) ;
#49853=EDGE_CURVE('',#39574,#39575,#6202,.T.) ;
#49854=EDGE_CURVE('',#39575,#39576,#6203,.T.) ;
#49855=EDGE_CURVE('',#39576,#39573,#6204,.T.) ;
#49856=EDGE_CURVE('',#39577,#39578,#6205,.T.) ;
#49857=EDGE_CURVE('',#39578,#39579,#6206,.T.) ;
#49858=EDGE_CURVE('',#39579,#39580,#6207,.T.) ;
#49859=EDGE_CURVE('',#39580,#39577,#6208,.T.) ;
#49860=EDGE_CURVE('',#39581,#39582,#6209,.T.) ;
#49861=EDGE_CURVE('',#39582,#39583,#6210,.T.) ;
#49862=EDGE_CURVE('',#39583,#39584,#6211,.T.) ;
#49863=EDGE_CURVE('',#39584,#39581,#6212,.T.) ;
#49864=EDGE_CURVE('',#39585,#39586,#6213,.T.) ;
#49865=EDGE_CURVE('',#39586,#39587,#6214,.T.) ;
#49866=EDGE_CURVE('',#39587,#39588,#6215,.T.) ;
#49867=EDGE_CURVE('',#39588,#39585,#6216,.T.) ;
#49868=EDGE_CURVE('',#39589,#39590,#32708,.T.) ;
#49869=EDGE_CURVE('',#39589,#39591,#6217,.T.) ;
#49870=EDGE_CURVE('',#39592,#39591,#32709,.T.) ;
#49871=EDGE_CURVE('',#39592,#39593,#6218,.T.) ;
#49872=EDGE_CURVE('',#39594,#39593,#32710,.T.) ;
#49873=EDGE_CURVE('',#39594,#39595,#6219,.T.) ;
#49874=EDGE_CURVE('',#39596,#39595,#32711,.T.) ;
#49875=EDGE_CURVE('',#39596,#39590,#6220,.T.) ;
#49876=EDGE_CURVE('',#39597,#39598,#32712,.T.) ;
#49877=EDGE_CURVE('',#39597,#39599,#6221,.T.) ;
#49878=EDGE_CURVE('',#39600,#39599,#32713,.T.) ;
#49879=EDGE_CURVE('',#39600,#39601,#6222,.T.) ;
#49880=EDGE_CURVE('',#39602,#39601,#32714,.T.) ;
#49881=EDGE_CURVE('',#39602,#39603,#6223,.T.) ;
#49882=EDGE_CURVE('',#39604,#39603,#32715,.T.) ;
#49883=EDGE_CURVE('',#39604,#39598,#6224,.T.) ;
#49884=EDGE_CURVE('',#39605,#39606,#6225,.T.) ;
#49885=EDGE_CURVE('',#39606,#39607,#6226,.T.) ;
#49886=EDGE_CURVE('',#39607,#39608,#6227,.T.) ;
#49887=EDGE_CURVE('',#39609,#39608,#32716,.T.) ;
#49888=EDGE_CURVE('',#39609,#39610,#6228,.T.) ;
#49889=EDGE_CURVE('',#39610,#39611,#6229,.T.) ;
#49890=EDGE_CURVE('',#39611,#39612,#6230,.T.) ;
#49891=EDGE_CURVE('',#39612,#39613,#32717,.T.) ;
#49892=EDGE_CURVE('',#39613,#39614,#6231,.T.) ;
#49893=EDGE_CURVE('',#39614,#39615,#6232,.T.) ;
#49894=EDGE_CURVE('',#39615,#39616,#6233,.T.) ;
#49895=EDGE_CURVE('',#39616,#39617,#6234,.T.) ;
#49896=EDGE_CURVE('',#39618,#39617,#32718,.T.) ;
#49897=EDGE_CURVE('',#39618,#39619,#6235,.T.) ;
#49898=EDGE_CURVE('',#39619,#39605,#6236,.T.) ;
#49899=EDGE_CURVE('',#39620,#39621,#6237,.T.) ;
#49900=EDGE_CURVE('',#39621,#39622,#6238,.T.) ;
#49901=EDGE_CURVE('',#39622,#39623,#6239,.T.) ;
#49902=EDGE_CURVE('',#39623,#39624,#6240,.T.) ;
#49903=EDGE_CURVE('',#39624,#39625,#6241,.T.) ;
#49904=EDGE_CURVE('',#39626,#39625,#32719,.T.) ;
#49905=EDGE_CURVE('',#39626,#39627,#6242,.T.) ;
#49906=EDGE_CURVE('',#39627,#39628,#6243,.T.) ;
#49907=EDGE_CURVE('',#39628,#39629,#6244,.T.) ;
#49908=EDGE_CURVE('',#39629,#39630,#6245,.T.) ;
#49909=EDGE_CURVE('',#39630,#39631,#32720,.T.) ;
#49910=EDGE_CURVE('',#39631,#39632,#6246,.T.) ;
#49911=EDGE_CURVE('',#39632,#39633,#6247,.T.) ;
#49912=EDGE_CURVE('',#39633,#39634,#6248,.T.) ;
#49913=EDGE_CURVE('',#39620,#39634,#32721,.T.) ;
#49914=EDGE_CURVE('',#39635,#39636,#6249,.T.) ;
#49915=EDGE_CURVE('',#39636,#39637,#6250,.T.) ;
#49916=EDGE_CURVE('',#39637,#39638,#6251,.T.) ;
#49917=EDGE_CURVE('',#39638,#39635,#6252,.T.) ;
#49918=EDGE_CURVE('',#39639,#39640,#6253,.T.) ;
#49919=EDGE_CURVE('',#39640,#39641,#6254,.T.) ;
#49920=EDGE_CURVE('',#39641,#39642,#6255,.T.) ;
#49921=EDGE_CURVE('',#39642,#39639,#6256,.T.) ;
#49922=EDGE_CURVE('',#39643,#39644,#6257,.T.) ;
#49923=EDGE_CURVE('',#39643,#39645,#367,.T.) ;
#49924=EDGE_CURVE('',#39645,#39646,#6258,.T.) ;
#49925=EDGE_CURVE('',#39646,#39647,#368,.T.) ;
#49926=EDGE_CURVE('',#39647,#39648,#6259,.T.) ;
#49927=EDGE_CURVE('',#39648,#39642,#369,.T.) ;
#49928=EDGE_CURVE('',#39641,#39644,#370,.T.) ;
#49929=EDGE_CURVE('',#39645,#39649,#6260,.T.) ;
#49930=EDGE_CURVE('',#39649,#39650,#6261,.T.) ;
#49931=EDGE_CURVE('',#39650,#39646,#6262,.T.) ;
#49932=EDGE_CURVE('',#39651,#39652,#6263,.T.) ;
#49933=EDGE_CURVE('',#39652,#39653,#6264,.T.) ;
#49934=EDGE_CURVE('',#39653,#39654,#6265,.T.) ;
#49935=EDGE_CURVE('',#39654,#39651,#6266,.T.) ;
#49936=EDGE_CURVE('',#39655,#39656,#6267,.T.) ;
#49937=EDGE_CURVE('',#39656,#39643,#6268,.T.) ;
#49938=EDGE_CURVE('',#39644,#39657,#6269,.T.) ;
#49939=EDGE_CURVE('',#39657,#39658,#6270,.T.) ;
#49940=EDGE_CURVE('',#39658,#39655,#6271,.T.) ;
#49941=EDGE_CURVE('',#39659,#39660,#6272,.T.) ;
#49942=EDGE_CURVE('',#39660,#39648,#6273,.T.) ;
#49943=EDGE_CURVE('',#39647,#39661,#6274,.T.) ;
#49944=EDGE_CURVE('',#39661,#39662,#6275,.T.) ;
#49945=EDGE_CURVE('',#39662,#39659,#6276,.T.) ;
#49946=EDGE_CURVE('',#39663,#39664,#6277,.T.) ;
#49947=EDGE_CURVE('',#39664,#39665,#6278,.T.) ;
#49948=EDGE_CURVE('',#39665,#39666,#6279,.T.) ;
#49949=EDGE_CURVE('',#39666,#39663,#6280,.T.) ;
#49950=EDGE_CURVE('',#39667,#39668,#6281,.T.) ;
#49951=EDGE_CURVE('',#39668,#39669,#6282,.T.) ;
#49952=EDGE_CURVE('',#39669,#39670,#6283,.T.) ;
#49953=EDGE_CURVE('',#39670,#39667,#6284,.T.) ;
#49954=EDGE_CURVE('',#39671,#39672,#6285,.T.) ;
#49955=EDGE_CURVE('',#39672,#39673,#6286,.T.) ;
#49956=EDGE_CURVE('',#39673,#39674,#6287,.T.) ;
#49957=EDGE_CURVE('',#39674,#39671,#6288,.T.) ;
#49958=EDGE_CURVE('',#39675,#39676,#6289,.T.) ;
#49959=EDGE_CURVE('',#39676,#39677,#6290,.T.) ;
#49960=EDGE_CURVE('',#39677,#39678,#6291,.T.) ;
#49961=EDGE_CURVE('',#39678,#39675,#6292,.T.) ;
#49962=EDGE_CURVE('',#39679,#39680,#6293,.T.) ;
#49963=EDGE_CURVE('',#39680,#39681,#6294,.T.) ;
#49964=EDGE_CURVE('',#39681,#39682,#6295,.T.) ;
#49965=EDGE_CURVE('',#39682,#39679,#6296,.T.) ;
#49966=EDGE_CURVE('',#39683,#39684,#6297,.T.) ;
#49967=EDGE_CURVE('',#39683,#39685,#32722,.T.) ;
#49968=EDGE_CURVE('',#39686,#39685,#6298,.T.) ;
#49969=EDGE_CURVE('',#39686,#39687,#32723,.T.) ;
#49970=EDGE_CURVE('',#39688,#39687,#6299,.T.) ;
#49971=EDGE_CURVE('',#39688,#39689,#32724,.T.) ;
#49972=EDGE_CURVE('',#39690,#39689,#6300,.T.) ;
#49973=EDGE_CURVE('',#39690,#39684,#32725,.T.) ;
#49974=EDGE_CURVE('',#39689,#39691,#6301,.T.) ;
#49975=EDGE_CURVE('',#39691,#39692,#6302,.T.) ;
#49976=EDGE_CURVE('',#39692,#39690,#6303,.T.) ;
#49977=EDGE_CURVE('',#39684,#39693,#6304,.T.) ;
#49978=EDGE_CURVE('',#39693,#39694,#6305,.T.) ;
#49979=EDGE_CURVE('',#39694,#39683,#6306,.T.) ;
#49980=EDGE_CURVE('',#39695,#39696,#6307,.T.) ;
#49981=EDGE_CURVE('',#39696,#39686,#6308,.T.) ;
#49982=EDGE_CURVE('',#39685,#39695,#6309,.T.) ;
#49983=EDGE_CURVE('',#39687,#39697,#6310,.T.) ;
#49984=EDGE_CURVE('',#39697,#39698,#6311,.T.) ;
#49985=EDGE_CURVE('',#39698,#39688,#6312,.T.) ;
#49986=EDGE_CURVE('',#39699,#39700,#6313,.T.) ;
#49987=EDGE_CURVE('',#39700,#39701,#6314,.T.) ;
#49988=EDGE_CURVE('',#39701,#39702,#6315,.T.) ;
#49989=EDGE_CURVE('',#39702,#39699,#6316,.T.) ;
#49990=EDGE_CURVE('',#39462,#39703,#6317,.T.) ;
#49991=EDGE_CURVE('',#39703,#39704,#6318,.T.) ;
#49992=EDGE_CURVE('',#39705,#39704,#32726,.T.) ;
#49993=EDGE_CURVE('',#39705,#38818,#6319,.T.) ;
#49994=EDGE_CURVE('',#38755,#39706,#6320,.T.) ;
#49995=EDGE_CURVE('',#39707,#39706,#32727,.T.) ;
#49996=EDGE_CURVE('',#39707,#39708,#6321,.T.) ;
#49997=EDGE_CURVE('',#39708,#39461,#6322,.T.) ;
#49998=EDGE_CURVE('',#39709,#39710,#6323,.T.) ;
#49999=EDGE_CURVE('',#39710,#39711,#6324,.T.) ;
#50000=EDGE_CURVE('',#39711,#39712,#6325,.T.) ;
#50001=EDGE_CURVE('',#39712,#39709,#6326,.T.) ;
#50002=EDGE_CURVE('',#39713,#39714,#32728,.T.) ;
#50003=EDGE_CURVE('',#39714,#39715,#32729,.T.) ;
#50004=EDGE_CURVE('',#39715,#39716,#6327,.T.) ;
#50005=EDGE_CURVE('',#39716,#39717,#6328,.T.) ;
#50006=EDGE_CURVE('',#39717,#39718,#6329,.T.) ;
#50007=EDGE_CURVE('',#39718,#39719,#6330,.T.) ;
#50008=EDGE_CURVE('',#39720,#39719,#32730,.T.) ;
#50009=EDGE_CURVE('',#39720,#39721,#6331,.T.) ;
#50010=EDGE_CURVE('',#39721,#39722,#6332,.T.) ;
#50011=EDGE_CURVE('',#39722,#39713,#6333,.T.) ;
#50012=EDGE_CURVE('',#39723,#39724,#6334,.T.) ;
#50013=EDGE_CURVE('',#39724,#39725,#6335,.T.) ;
#50014=EDGE_CURVE('',#39725,#39726,#6336,.T.) ;
#50015=EDGE_CURVE('',#39726,#39723,#6337,.T.) ;
#50016=EDGE_CURVE('',#39727,#39728,#6338,.T.) ;
#50017=EDGE_CURVE('',#39728,#39729,#32731,.T.) ;
#50018=EDGE_CURVE('',#39729,#39730,#32732,.T.) ;
#50019=EDGE_CURVE('',#39730,#39731,#6339,.T.) ;
#50020=EDGE_CURVE('',#39731,#39732,#6340,.T.) ;
#50021=EDGE_CURVE('',#39732,#39733,#6341,.T.) ;
#50022=EDGE_CURVE('',#39734,#39733,#32733,.T.) ;
#50023=EDGE_CURVE('',#39734,#39735,#6342,.T.) ;
#50024=EDGE_CURVE('',#39735,#39736,#6343,.T.) ;
#50025=EDGE_CURVE('',#39736,#39727,#6344,.T.) ;
#50026=EDGE_CURVE('',#39737,#39463,#6345,.T.) ;
#50027=EDGE_CURVE('',#39464,#39738,#6346,.T.) ;
#50028=EDGE_CURVE('',#39738,#39737,#6347,.T.) ;
#50029=EDGE_CURVE('',#39739,#39740,#6348,.T.) ;
#50030=EDGE_CURVE('',#39740,#39741,#6349,.T.) ;
#50031=EDGE_CURVE('',#39741,#39742,#6350,.T.) ;
#50032=EDGE_CURVE('',#39742,#39739,#6351,.T.) ;
#50033=EDGE_CURVE('',#39743,#39744,#6352,.T.) ;
#50034=EDGE_CURVE('',#39744,#39745,#6353,.T.) ;
#50035=EDGE_CURVE('',#39745,#39746,#6354,.T.) ;
#50036=EDGE_CURVE('',#39746,#39743,#6355,.T.) ;
#50037=EDGE_CURVE('',#39747,#39748,#6356,.T.) ;
#50038=EDGE_CURVE('',#39748,#39749,#32734,.T.) ;
#50039=EDGE_CURVE('',#39749,#39750,#6357,.T.) ;
#50040=EDGE_CURVE('',#39750,#39747,#32735,.T.) ;
#50041=EDGE_CURVE('',#39751,#39752,#6358,.T.) ;
#50042=EDGE_CURVE('',#39752,#39753,#32736,.T.) ;
#50043=EDGE_CURVE('',#39753,#39754,#6359,.T.) ;
#50044=EDGE_CURVE('',#39754,#39755,#6360,.T.) ;
#50045=EDGE_CURVE('',#39755,#39756,#6361,.T.) ;
#50046=EDGE_CURVE('',#39756,#39751,#6362,.T.) ;
#50047=EDGE_CURVE('',#39757,#39758,#6363,.T.) ;
#50048=EDGE_CURVE('',#39758,#39759,#6364,.T.) ;
#50049=EDGE_CURVE('',#39759,#39760,#6365,.T.) ;
#50050=EDGE_CURVE('',#39760,#39757,#6366,.T.) ;
#50051=EDGE_CURVE('',#39761,#39762,#6367,.T.) ;
#50052=EDGE_CURVE('',#39762,#39763,#6368,.T.) ;
#50053=EDGE_CURVE('',#39763,#39764,#6369,.T.) ;
#50054=EDGE_CURVE('',#39764,#39761,#6370,.T.) ;
#50055=EDGE_CURVE('',#39765,#39766,#6371,.T.) ;
#50056=EDGE_CURVE('',#39766,#39767,#6372,.T.) ;
#50057=EDGE_CURVE('',#39767,#39768,#6373,.T.) ;
#50058=EDGE_CURVE('',#39768,#39765,#6374,.T.) ;
#50059=EDGE_CURVE('',#39769,#39770,#6375,.T.) ;
#50060=EDGE_CURVE('',#39770,#39771,#6376,.T.) ;
#50061=EDGE_CURVE('',#39771,#39772,#6377,.T.) ;
#50062=EDGE_CURVE('',#39772,#39769,#6378,.T.) ;
#50063=EDGE_CURVE('',#39773,#39774,#6379,.T.) ;
#50064=EDGE_CURVE('',#39774,#39775,#6380,.T.) ;
#50065=EDGE_CURVE('',#39775,#39776,#6381,.T.) ;
#50066=EDGE_CURVE('',#39776,#39773,#6382,.T.) ;
#50067=EDGE_CURVE('',#39777,#39778,#6383,.T.) ;
#50068=EDGE_CURVE('',#39777,#39779,#32737,.T.) ;
#50069=EDGE_CURVE('',#39780,#39779,#6384,.T.) ;
#50070=EDGE_CURVE('',#39780,#39781,#32738,.T.) ;
#50071=EDGE_CURVE('',#39782,#39781,#6385,.T.) ;
#50072=EDGE_CURVE('',#39782,#39783,#32739,.T.) ;
#50073=EDGE_CURVE('',#39784,#39783,#6386,.T.) ;
#50074=EDGE_CURVE('',#39784,#39778,#32740,.T.) ;
#50075=EDGE_CURVE('',#39785,#39786,#6387,.T.) ;
#50076=EDGE_CURVE('',#39786,#39784,#6388,.T.) ;
#50077=EDGE_CURVE('',#39783,#39785,#6389,.T.) ;
#50078=EDGE_CURVE('',#39787,#39788,#6390,.T.) ;
#50079=EDGE_CURVE('',#39788,#39777,#6391,.T.) ;
#50080=EDGE_CURVE('',#39778,#39787,#6392,.T.) ;
#50081=EDGE_CURVE('',#39779,#39789,#6393,.T.) ;
#50082=EDGE_CURVE('',#39789,#39790,#6394,.T.) ;
#50083=EDGE_CURVE('',#39790,#39780,#6395,.T.) ;
#50084=EDGE_CURVE('',#39791,#39792,#6396,.T.) ;
#50085=EDGE_CURVE('',#39792,#39782,#6397,.T.) ;
#50086=EDGE_CURVE('',#39781,#39791,#6398,.T.) ;
#50087=EDGE_CURVE('',#39793,#39794,#6399,.T.) ;
#50088=EDGE_CURVE('',#39794,#39795,#6400,.T.) ;
#50089=EDGE_CURVE('',#39795,#39796,#6401,.T.) ;
#50090=EDGE_CURVE('',#39796,#39793,#6402,.T.) ;
#50091=EDGE_CURVE('',#39061,#39045,#6403,.T.) ;
#50092=EDGE_CURVE('',#39047,#39060,#6404,.T.) ;
#50093=EDGE_CURVE('',#39059,#39048,#6405,.T.) ;
#50094=EDGE_CURVE('',#39051,#39056,#6406,.T.) ;
#50095=EDGE_CURVE('',#39055,#39052,#6407,.T.) ;
#50096=EDGE_CURVE('',#39049,#39058,#6408,.T.) ;
#50097=EDGE_CURVE('',#39057,#39050,#6409,.T.) ;
#50098=EDGE_CURVE('',#38760,#38753,#32741,.T.) ;
#50099=EDGE_CURVE('',#38752,#38749,#32742,.T.) ;
#50100=EDGE_CURVE('',#38748,#39797,#6410,.T.) ;
#50101=EDGE_CURVE('',#39797,#39798,#6411,.T.) ;
#50102=EDGE_CURVE('',#39798,#39044,#6412,.T.) ;
#50103=EDGE_CURVE('',#39799,#39800,#6413,.T.) ;
#50104=EDGE_CURVE('',#39800,#38817,#6414,.T.) ;
#50105=EDGE_CURVE('',#39043,#39799,#6415,.T.) ;
#50106=EDGE_CURVE('',#38816,#38810,#32743,.T.) ;
#50107=EDGE_CURVE('',#38809,#38803,#32744,.T.) ;
#50108=EDGE_CURVE('',#39801,#39802,#6416,.T.) ;
#50109=EDGE_CURVE('',#39802,#39803,#32745,.T.) ;
#50110=EDGE_CURVE('',#39804,#39803,#6417,.T.) ;
#50111=EDGE_CURVE('',#39804,#39801,#32746,.T.) ;
#50112=EDGE_CURVE('',#39803,#39805,#6418,.T.) ;
#50113=EDGE_CURVE('',#39806,#39805,#6419,.T.) ;
#50114=EDGE_CURVE('',#39806,#39804,#6420,.T.) ;
#50115=EDGE_CURVE('',#39805,#39807,#32747,.T.) ;
#50116=EDGE_CURVE('',#39808,#39807,#6421,.T.) ;
#50117=EDGE_CURVE('',#39808,#39806,#32748,.T.) ;
#50118=EDGE_CURVE('',#39807,#39809,#6422,.T.) ;
#50119=EDGE_CURVE('',#39810,#39809,#6423,.T.) ;
#50120=EDGE_CURVE('',#39810,#39808,#6424,.T.) ;
#50121=EDGE_CURVE('',#39809,#39811,#32749,.T.) ;
#50122=EDGE_CURVE('',#39812,#39811,#6425,.T.) ;
#50123=EDGE_CURVE('',#39812,#39810,#32750,.T.) ;
#50124=EDGE_CURVE('',#39811,#39813,#6426,.T.) ;
#50125=EDGE_CURVE('',#39814,#39813,#6427,.T.) ;
#50126=EDGE_CURVE('',#39814,#39812,#6428,.T.) ;
#50127=EDGE_CURVE('',#39813,#39815,#32751,.T.) ;
#50128=EDGE_CURVE('',#39816,#39815,#6429,.T.) ;
#50129=EDGE_CURVE('',#39816,#39814,#32752,.T.) ;
#50130=EDGE_CURVE('',#39801,#39816,#6430,.T.) ;
#50131=EDGE_CURVE('',#39815,#39802,#6431,.T.) ;
#50132=EDGE_CURVE('',#39817,#39818,#6432,.T.) ;
#50133=EDGE_CURVE('',#39818,#39819,#6433,.T.) ;
#50134=EDGE_CURVE('',#39819,#39820,#6434,.T.) ;
#50135=EDGE_CURVE('',#39820,#39817,#6435,.T.) ;
#50136=EDGE_CURVE('',#39555,#39629,#32753,.T.) ;
#50137=EDGE_CURVE('',#39556,#39628,#32754,.T.) ;
#50138=EDGE_CURVE('',#39556,#39469,#32755,.T.) ;
#50139=EDGE_CURVE('',#39469,#39628,#32756,.T.) ;
#50140=EDGE_CURVE('',#39554,#39398,#32757,.T.) ;
#50141=EDGE_CURVE('',#39397,#39555,#32758,.T.) ;
#50142=EDGE_CURVE('',#39470,#39627,#32759,.T.) ;
#50143=EDGE_CURVE('',#39553,#39468,#32760,.T.) ;
#50144=EDGE_CURVE('',#39614,#39554,#32761,.T.) ;
#50145=EDGE_CURVE('',#39615,#39553,#32762,.T.) ;
#50146=EDGE_CURVE('',#39622,#39552,#32763,.T.) ;
#50147=EDGE_CURVE('',#39623,#39551,#32764,.T.) ;
#50148=EDGE_CURVE('',#39821,#39623,#32765,.T.) ;
#50149=EDGE_CURVE('',#39821,#39822,#371,.T.) ;
#50150=EDGE_CURVE('',#39822,#39624,#372,.T.) ;
#50151=EDGE_CURVE('',#39470,#39546,#32766,.T.) ;
#50152=EDGE_CURVE('',#39546,#39627,#32767,.T.) ;
#50153=EDGE_CURVE('',#39615,#39468,#32768,.T.) ;
#50154=EDGE_CURVE('',#39552,#39064,#32769,.T.) ;
#50155=EDGE_CURVE('',#39063,#39549,#32770,.T.) ;
#50156=EDGE_CURVE('',#38745,#39551,#32771,.T.) ;
#50157=EDGE_CURVE('',#38745,#39821,#373,.T.) ;
#50158=EDGE_CURVE('',#39624,#39823,#374,.T.) ;
#50159=EDGE_CURVE('',#39823,#39824,#375,.T.) ;
#50160=EDGE_CURVE('',#39824,#38744,#376,.T.) ;
#50161=EDGE_CURVE('',#39625,#39547,#32772,.T.) ;
#50162=EDGE_CURVE('',#39543,#39626,#32773,.T.) ;
#50163=EDGE_CURVE('',#39467,#39545,#32774,.T.) ;
#50164=EDGE_CURVE('',#39616,#39467,#32775,.T.) ;
#50165=EDGE_CURVE('',#39549,#39606,#32776,.T.) ;
#50166=EDGE_CURVE('',#39550,#39605,#32777,.T.) ;
#50167=EDGE_CURVE('',#38743,#39550,#32778,.T.) ;
#50168=EDGE_CURVE('',#39543,#39547,#32779,.T.) ;
#50169=EDGE_CURVE('',#39616,#39545,#32780,.T.) ;
#50170=EDGE_CURVE('',#39825,#39605,#32781,.T.) ;
#50171=EDGE_CURVE('',#39825,#38743,#377,.T.) ;
#50172=EDGE_CURVE('',#39544,#39548,#32782,.T.) ;
#50173=EDGE_CURVE('',#39617,#39544,#32783,.T.) ;
#50174=EDGE_CURVE('',#39619,#39826,#378,.T.) ;
#50175=EDGE_CURVE('',#39826,#39825,#379,.T.) ;
#50176=EDGE_CURVE('',#39618,#39548,#32784,.T.) ;
#50177=EDGE_CURVE('',#38742,#39827,#380,.T.) ;
#50178=EDGE_CURVE('',#39827,#39828,#381,.T.) ;
#50179=EDGE_CURVE('',#39828,#39619,#382,.T.) ;
#50180=EDGE_CURVE('',#39753,#39739,#32785,.T.) ;
#50181=EDGE_CURVE('',#39750,#39753,#32786,.T.) ;
#50182=EDGE_CURVE('',#39739,#39750,#32787,.T.) ;
#50183=EDGE_CURVE('',#39747,#39752,#32788,.T.) ;
#50184=EDGE_CURVE('',#39740,#39749,#32789,.T.) ;
#50185=EDGE_CURVE('',#39754,#39742,#32790,.T.) ;
#50186=EDGE_CURVE('',#39731,#39755,#32791,.T.) ;
#50187=EDGE_CURVE('',#39732,#39754,#32792,.T.) ;
#50188=EDGE_CURVE('',#39755,#39520,#32793,.T.) ;
#50189=EDGE_CURVE('',#39519,#39756,#32794,.T.) ;
#50190=EDGE_CURVE('',#39747,#39746,#32795,.T.) ;
#50191=EDGE_CURVE('',#39746,#39752,#32796,.T.) ;
#50192=EDGE_CURVE('',#39740,#39539,#32797,.T.) ;
#50193=EDGE_CURVE('',#39540,#39749,#32798,.T.) ;
#50194=EDGE_CURVE('',#39732,#39742,#32799,.T.) ;
#50195=EDGE_CURVE('',#39756,#39722,#32800,.T.) ;
#50196=EDGE_CURVE('',#39751,#39721,#32801,.T.) ;
#50197=EDGE_CURVE('',#39743,#39751,#32802,.T.) ;
#50198=EDGE_CURVE('',#39748,#39745,#32803,.T.) ;
#50199=EDGE_CURVE('',#39541,#39748,#32804,.T.) ;
#50200=EDGE_CURVE('',#39741,#39538,#32805,.T.) ;
#50201=EDGE_CURVE('',#39733,#39741,#32806,.T.) ;
#50202=EDGE_CURVE('',#39743,#39721,#32807,.T.) ;
#50203=EDGE_CURVE('',#39542,#39745,#32808,.T.) ;
#50204=EDGE_CURVE('',#39734,#39538,#32809,.T.) ;
#50205=EDGE_CURVE('',#39744,#39720,#32810,.T.) ;
#50206=EDGE_CURVE('',#39535,#39744,#32811,.T.) ;
#50207=EDGE_CURVE('',#39735,#39537,#32812,.T.) ;
#50208=EDGE_CURVE('',#39464,#39728,#32813,.T.) ;
#50209=EDGE_CURVE('',#39738,#39727,#32814,.T.) ;
#50210=EDGE_CURVE('',#39454,#39738,#32815,.T.) ;
#50211=EDGE_CURVE('',#39737,#39453,#32816,.T.) ;
#50212=EDGE_CURVE('',#39535,#39719,#32817,.T.) ;
#50213=EDGE_CURVE('',#39735,#39726,#32818,.T.) ;
#50214=EDGE_CURVE('',#39726,#39537,#32819,.T.) ;
#50215=EDGE_CURVE('',#39454,#39727,#32820,.T.) ;
#50216=EDGE_CURVE('',#39536,#39718,#32821,.T.) ;
#50217=EDGE_CURVE('',#39723,#39536,#32822,.T.) ;
#50218=EDGE_CURVE('',#39736,#39725,#32823,.T.) ;
#50219=EDGE_CURVE('',#39455,#39736,#32824,.T.) ;
#50220=EDGE_CURVE('',#39723,#39718,#32825,.T.) ;
#50221=EDGE_CURVE('',#39456,#39725,#32826,.T.) ;
#50222=EDGE_CURVE('',#39711,#39460,#32827,.T.) ;
#50223=EDGE_CURVE('',#39712,#39459,#32828,.T.) ;
#50224=EDGE_CURVE('',#39715,#39709,#32829,.T.) ;
#50225=EDGE_CURVE('',#39716,#39712,#32830,.T.) ;
#50226=EDGE_CURVE('',#39724,#39717,#32831,.T.) ;
#50227=EDGE_CURVE('',#39457,#39724,#32832,.T.) ;
#50228=EDGE_CURVE('',#39716,#39459,#32833,.T.) ;
#50229=EDGE_CURVE('',#39458,#39717,#32834,.T.) ;
#50230=EDGE_CURVE('',#39529,#39805,#32835,.T.) ;
#50231=EDGE_CURVE('',#39807,#39528,#32836,.T.) ;
#50232=EDGE_CURVE('',#39809,#39527,#32837,.T.) ;
#50233=EDGE_CURVE('',#39530,#39803,#32838,.T.) ;
#50234=EDGE_CURVE('',#39811,#39526,#32839,.T.) ;
#50235=EDGE_CURVE('',#39523,#39802,#32840,.T.) ;
#50236=EDGE_CURVE('',#39813,#39525,#32841,.T.) ;
#50237=EDGE_CURVE('',#39524,#39815,#32842,.T.) ;
#50238=EDGE_CURVE('',#39603,#39678,#32843,.T.) ;
#50239=EDGE_CURVE('',#39675,#39602,#32844,.T.) ;
#50240=EDGE_CURVE('',#39674,#39601,#32845,.T.) ;
#50241=EDGE_CURVE('',#39675,#39674,#32846,.T.) ;
#50242=EDGE_CURVE('',#39666,#39678,#32847,.T.) ;
#50243=EDGE_CURVE('',#39604,#39666,#32848,.T.) ;
#50244=EDGE_CURVE('',#39671,#39600,#32849,.T.) ;
#50245=EDGE_CURVE('',#39676,#39673,#32850,.T.) ;
#50246=EDGE_CURVE('',#39677,#39682,#32851,.T.) ;
#50247=EDGE_CURVE('',#39679,#39676,#32852,.T.) ;
#50248=EDGE_CURVE('',#39663,#39677,#32853,.T.) ;
#50249=EDGE_CURVE('',#39598,#39665,#32854,.T.) ;
#50250=EDGE_CURVE('',#39599,#39669,#32855,.T.) ;
#50251=EDGE_CURVE('',#39670,#39597,#32856,.T.) ;
#50252=EDGE_CURVE('',#39671,#39669,#32857,.T.) ;
#50253=EDGE_CURVE('',#39679,#39673,#32858,.T.) ;
#50254=EDGE_CURVE('',#39663,#39682,#32859,.T.) ;
#50255=EDGE_CURVE('',#39670,#39665,#32860,.T.) ;
#50256=EDGE_CURVE('',#39672,#39668,#32861,.T.) ;
#50257=EDGE_CURVE('',#39680,#39672,#32862,.T.) ;
#50258=EDGE_CURVE('',#39664,#39681,#32863,.T.) ;
#50259=EDGE_CURVE('',#39667,#39664,#32864,.T.) ;
#50260=EDGE_CURVE('',#39680,#39668,#32865,.T.) ;
#50261=EDGE_CURVE('',#39667,#39681,#32866,.T.) ;
#50262=EDGE_CURVE('',#39691,#39698,#32867,.T.) ;
#50263=EDGE_CURVE('',#39692,#39702,#32868,.T.) ;
#50264=EDGE_CURVE('',#39699,#39691,#32869,.T.) ;
#50265=EDGE_CURVE('',#39693,#39692,#32870,.T.) ;
#50266=EDGE_CURVE('',#39699,#39698,#32871,.T.) ;
#50267=EDGE_CURVE('',#39693,#39702,#32872,.T.) ;
#50268=EDGE_CURVE('',#39697,#39696,#32873,.T.) ;
#50269=EDGE_CURVE('',#39700,#39697,#32874,.T.) ;
#50270=EDGE_CURVE('',#39694,#39701,#32875,.T.) ;
#50271=EDGE_CURVE('',#39695,#39694,#32876,.T.) ;
#50272=EDGE_CURVE('',#39700,#39696,#32877,.T.) ;
#50273=EDGE_CURVE('',#39695,#39701,#32878,.T.) ;
#50274=EDGE_CURVE('',#39639,#39660,#32879,.T.) ;
#50275=EDGE_CURVE('',#39639,#39637,#32880,.T.) ;
#50276=EDGE_CURVE('',#39637,#39660,#32881,.T.) ;
#50277=EDGE_CURVE('',#39638,#39659,#2305,.T.) ;
#50278=EDGE_CURVE('',#39640,#39636,#32882,.T.) ;
#50279=EDGE_CURVE('',#39657,#39640,#32883,.T.) ;
#50280=EDGE_CURVE('',#39638,#39515,#32884,.T.) ;
#50281=EDGE_CURVE('',#39516,#39659,#32885,.T.) ;
#50282=EDGE_CURVE('',#39657,#39636,#32886,.T.) ;
#50283=EDGE_CURVE('',#39661,#39650,#32887,.T.) ;
#50284=EDGE_CURVE('',#39662,#39654,#2306,.T.) ;
#50285=EDGE_CURVE('',#39651,#39661,#32888,.T.) ;
#50286=EDGE_CURVE('',#39517,#39662,#32889,.T.) ;
#50287=EDGE_CURVE('',#39635,#39514,#32890,.T.) ;
#50288=EDGE_CURVE('',#39658,#39635,#383,.T.) ;
#50289=EDGE_CURVE('',#39651,#39650,#32891,.T.) ;
#50290=EDGE_CURVE('',#39518,#39654,#32892,.T.) ;
#50291=EDGE_CURVE('',#39658,#39513,#32893,.T.) ;
#50292=EDGE_CURVE('',#39649,#39656,#32894,.T.) ;
#50293=EDGE_CURVE('',#39652,#39649,#32895,.T.) ;
#50294=EDGE_CURVE('',#39512,#39653,#32896,.T.) ;
#50295=EDGE_CURVE('',#39655,#39511,#32897,.T.) ;
#50296=EDGE_CURVE('',#39652,#39656,#32898,.T.) ;
#50297=EDGE_CURVE('',#39655,#39653,#384,.T.) ;
#50298=EDGE_CURVE('',#39107,#39771,#32899,.T.) ;
#50299=EDGE_CURVE('',#39772,#39106,#32900,.T.) ;
#50300=EDGE_CURVE('',#39768,#39105,#32901,.T.) ;
#50301=EDGE_CURVE('',#39772,#39768,#32902,.T.) ;
#50302=EDGE_CURVE('',#39760,#39771,#32903,.T.) ;
#50303=EDGE_CURVE('',#39108,#39760,#32904,.T.) ;
#50304=EDGE_CURVE('',#39765,#39104,#32905,.T.) ;
#50305=EDGE_CURVE('',#39769,#39767,#32906,.T.) ;
#50306=EDGE_CURVE('',#39770,#39776,#32907,.T.) ;
#50307=EDGE_CURVE('',#39773,#39769,#32908,.T.) ;
#50308=EDGE_CURVE('',#39757,#39770,#32909,.T.) ;
#50309=EDGE_CURVE('',#39102,#39759,#32910,.T.) ;
#50310=EDGE_CURVE('',#39103,#39761,#32911,.T.) ;
#50311=EDGE_CURVE('',#39762,#39101,#32912,.T.) ;
#50312=EDGE_CURVE('',#39765,#39761,#32913,.T.) ;
#50313=EDGE_CURVE('',#39773,#39767,#32914,.T.) ;
#50314=EDGE_CURVE('',#39757,#39776,#32915,.T.) ;
#50315=EDGE_CURVE('',#39762,#39759,#32916,.T.) ;
#50316=EDGE_CURVE('',#39766,#39764,#32917,.T.) ;
#50317=EDGE_CURVE('',#39774,#39766,#32918,.T.) ;
#50318=EDGE_CURVE('',#39758,#39775,#32919,.T.) ;
#50319=EDGE_CURVE('',#39763,#39758,#32920,.T.) ;
#50320=EDGE_CURVE('',#39774,#39764,#32921,.T.) ;
#50321=EDGE_CURVE('',#39763,#39775,#32922,.T.) ;
#50322=EDGE_CURVE('',#39785,#39792,#32923,.T.) ;
#50323=EDGE_CURVE('',#39786,#39796,#32924,.T.) ;
#50324=EDGE_CURVE('',#39793,#39785,#32925,.T.) ;
#50325=EDGE_CURVE('',#39787,#39786,#32926,.T.) ;
#50326=EDGE_CURVE('',#39793,#39792,#32927,.T.) ;
#50327=EDGE_CURVE('',#39787,#39796,#32928,.T.) ;
#50328=EDGE_CURVE('',#39791,#39790,#32929,.T.) ;
#50329=EDGE_CURVE('',#39794,#39791,#32930,.T.) ;
#50330=EDGE_CURVE('',#39788,#39795,#32931,.T.) ;
#50331=EDGE_CURVE('',#39789,#39788,#32932,.T.) ;
#50332=EDGE_CURVE('',#39794,#39790,#32933,.T.) ;
#50333=EDGE_CURVE('',#39789,#39795,#32934,.T.) ;
#50334=EDGE_CURVE('',#39808,#39820,#32935,.T.) ;
#50335=EDGE_CURVE('',#39817,#39810,#32936,.T.) ;
#50336=EDGE_CURVE('',#39817,#39812,#32937,.T.) ;
#50337=EDGE_CURVE('',#39806,#39820,#32938,.T.) ;
#50338=EDGE_CURVE('',#39818,#39814,#32939,.T.) ;
#50339=EDGE_CURVE('',#39804,#39819,#32940,.T.) ;
#50340=EDGE_CURVE('',#39818,#39816,#32941,.T.) ;
#50341=EDGE_CURVE('',#39801,#39819,#32942,.T.) ;
#50342=EDGE_CURVE('',#39521,#39265,#32943,.T.) ;
#50343=EDGE_CURVE('',#39264,#39522,#32944,.T.) ;
#50344=EDGE_CURVE('',#39266,#39466,#2307,.T.) ;
#50345=EDGE_CURVE('',#39261,#39710,#32945,.T.) ;
#50346=EDGE_CURVE('',#39829,#39709,#32946,.T.) ;
#50347=EDGE_CURVE('',#39262,#39829,#32947,.T.) ;
#50348=EDGE_CURVE('',#39829,#39263,#2308,.T.) ;
#50349=EDGE_CURVE('',#39729,#39830,#2309,.T.) ;
#50350=EDGE_CURVE('',#39730,#39830,#32948,.T.) ;
#50351=EDGE_CURVE('',#39830,#39521,#32949,.T.) ;
#50352=EDGE_CURVE('',#39731,#39520,#32950,.T.) ;
#50353=EDGE_CURVE('',#39831,#39713,#32951,.T.) ;
#50354=EDGE_CURVE('',#39831,#39714,#2310,.T.) ;
#50355=EDGE_CURVE('',#39522,#39831,#32952,.T.) ;
#50356=EDGE_CURVE('',#39519,#39722,#32953,.T.) ;
#50357=EDGE_CURVE('',#39266,#39830,#32954,.T.) ;
#50358=EDGE_CURVE('',#39466,#39729,#32955,.T.) ;
#50359=EDGE_CURVE('',#39831,#39263,#32956,.T.) ;
#50360=EDGE_CURVE('',#39714,#39829,#32957,.T.) ;
#50361=EDGE_CURVE('',#39832,#39833,#6436,.T.) ;
#50362=EDGE_CURVE('',#39833,#39834,#6437,.T.) ;
#50363=EDGE_CURVE('',#39834,#39835,#6438,.T.) ;
#50364=EDGE_CURVE('',#39835,#39832,#6439,.T.) ;
#50365=EDGE_CURVE('',#39836,#39837,#6440,.T.) ;
#50366=EDGE_CURVE('',#39837,#39838,#6441,.T.) ;
#50367=EDGE_CURVE('',#39838,#39839,#6442,.T.) ;
#50368=EDGE_CURVE('',#39839,#39836,#6443,.T.) ;
#50369=EDGE_CURVE('',#39840,#39841,#6444,.T.) ;
#50370=EDGE_CURVE('',#39840,#39842,#385,.T.) ;
#50371=EDGE_CURVE('',#39842,#39843,#6445,.T.) ;
#50372=EDGE_CURVE('',#39843,#39844,#386,.T.) ;
#50373=EDGE_CURVE('',#39844,#39845,#6446,.T.) ;
#50374=EDGE_CURVE('',#39845,#39839,#387,.T.) ;
#50375=EDGE_CURVE('',#39838,#39841,#388,.T.) ;
#50376=EDGE_CURVE('',#39842,#39846,#6447,.T.) ;
#50377=EDGE_CURVE('',#39846,#39847,#6448,.T.) ;
#50378=EDGE_CURVE('',#39847,#39843,#6449,.T.) ;
#50379=EDGE_CURVE('',#39848,#39849,#6450,.T.) ;
#50380=EDGE_CURVE('',#39849,#39850,#6451,.T.) ;
#50381=EDGE_CURVE('',#39850,#39851,#6452,.T.) ;
#50382=EDGE_CURVE('',#39851,#39848,#6453,.T.) ;
#50383=EDGE_CURVE('',#39852,#39853,#6454,.T.) ;
#50384=EDGE_CURVE('',#39853,#39854,#6455,.T.) ;
#50385=EDGE_CURVE('',#39854,#39855,#6456,.T.) ;
#50386=EDGE_CURVE('',#39855,#39852,#6457,.T.) ;
#50387=EDGE_CURVE('',#39856,#39857,#6458,.T.) ;
#50388=EDGE_CURVE('',#39857,#39858,#6459,.T.) ;
#50389=EDGE_CURVE('',#39858,#39859,#6460,.T.) ;
#50390=EDGE_CURVE('',#39859,#39856,#6461,.T.) ;
#50391=EDGE_CURVE('',#39860,#39861,#6462,.T.) ;
#50392=EDGE_CURVE('',#39860,#39862,#389,.T.) ;
#50393=EDGE_CURVE('',#39862,#39863,#6463,.T.) ;
#50394=EDGE_CURVE('',#39863,#39864,#390,.T.) ;
#50395=EDGE_CURVE('',#39864,#39865,#6464,.T.) ;
#50396=EDGE_CURVE('',#39865,#39859,#391,.T.) ;
#50397=EDGE_CURVE('',#39858,#39861,#392,.T.) ;
#50398=EDGE_CURVE('',#39862,#39866,#6465,.T.) ;
#50399=EDGE_CURVE('',#39866,#39867,#6466,.T.) ;
#50400=EDGE_CURVE('',#39867,#39863,#6467,.T.) ;
#50401=EDGE_CURVE('',#39868,#39869,#6468,.T.) ;
#50402=EDGE_CURVE('',#39869,#39870,#6469,.T.) ;
#50403=EDGE_CURVE('',#39870,#39871,#6470,.T.) ;
#50404=EDGE_CURVE('',#39871,#39868,#6471,.T.) ;
#50405=EDGE_CURVE('',#39872,#39873,#6472,.T.) ;
#50406=EDGE_CURVE('',#39873,#39874,#6473,.T.) ;
#50407=EDGE_CURVE('',#39874,#39875,#6474,.T.) ;
#50408=EDGE_CURVE('',#39875,#39872,#6475,.T.) ;
#50409=EDGE_CURVE('',#39876,#39877,#6476,.T.) ;
#50410=EDGE_CURVE('',#39877,#39878,#6477,.T.) ;
#50411=EDGE_CURVE('',#39878,#39879,#6478,.T.) ;
#50412=EDGE_CURVE('',#39879,#39876,#6479,.T.) ;
#50413=EDGE_CURVE('',#39880,#39881,#6480,.T.) ;
#50414=EDGE_CURVE('',#39880,#39882,#393,.T.) ;
#50415=EDGE_CURVE('',#39882,#39883,#6481,.T.) ;
#50416=EDGE_CURVE('',#39883,#39884,#394,.T.) ;
#50417=EDGE_CURVE('',#39884,#39885,#6482,.T.) ;
#50418=EDGE_CURVE('',#39885,#39879,#395,.T.) ;
#50419=EDGE_CURVE('',#39878,#39881,#396,.T.) ;
#50420=EDGE_CURVE('',#39882,#39886,#6483,.T.) ;
#50421=EDGE_CURVE('',#39886,#39887,#6484,.T.) ;
#50422=EDGE_CURVE('',#39887,#39883,#6485,.T.) ;
#50423=EDGE_CURVE('',#39888,#39889,#6486,.T.) ;
#50424=EDGE_CURVE('',#39889,#39890,#6487,.T.) ;
#50425=EDGE_CURVE('',#39890,#39891,#6488,.T.) ;
#50426=EDGE_CURVE('',#39891,#39888,#6489,.T.) ;
#50427=EDGE_CURVE('',#39892,#39893,#6490,.T.) ;
#50428=EDGE_CURVE('',#39893,#39894,#6491,.T.) ;
#50429=EDGE_CURVE('',#39894,#39895,#6492,.T.) ;
#50430=EDGE_CURVE('',#39895,#39892,#6493,.T.) ;
#50431=EDGE_CURVE('',#39896,#39897,#6494,.T.) ;
#50432=EDGE_CURVE('',#39897,#39898,#6495,.T.) ;
#50433=EDGE_CURVE('',#39898,#39899,#6496,.T.) ;
#50434=EDGE_CURVE('',#39899,#39896,#6497,.T.) ;
#50435=EDGE_CURVE('',#39900,#39901,#6498,.T.) ;
#50436=EDGE_CURVE('',#39900,#39902,#397,.T.) ;
#50437=EDGE_CURVE('',#39902,#39903,#6499,.T.) ;
#50438=EDGE_CURVE('',#39903,#39904,#398,.T.) ;
#50439=EDGE_CURVE('',#39904,#39905,#6500,.T.) ;
#50440=EDGE_CURVE('',#39905,#39899,#399,.T.) ;
#50441=EDGE_CURVE('',#39898,#39901,#400,.T.) ;
#50442=EDGE_CURVE('',#39902,#39906,#6501,.T.) ;
#50443=EDGE_CURVE('',#39906,#39907,#6502,.T.) ;
#50444=EDGE_CURVE('',#39907,#39903,#6503,.T.) ;
#50445=EDGE_CURVE('',#39908,#39909,#6504,.T.) ;
#50446=EDGE_CURVE('',#39909,#39910,#6505,.T.) ;
#50447=EDGE_CURVE('',#39910,#39911,#6506,.T.) ;
#50448=EDGE_CURVE('',#39911,#39908,#6507,.T.) ;
#50449=EDGE_CURVE('',#39912,#39913,#6508,.T.) ;
#50450=EDGE_CURVE('',#39913,#39914,#6509,.T.) ;
#50451=EDGE_CURVE('',#39914,#39915,#6510,.T.) ;
#50452=EDGE_CURVE('',#39915,#39912,#6511,.T.) ;
#50453=EDGE_CURVE('',#39916,#39917,#6512,.T.) ;
#50454=EDGE_CURVE('',#39917,#39918,#6513,.T.) ;
#50455=EDGE_CURVE('',#39918,#39919,#6514,.T.) ;
#50456=EDGE_CURVE('',#39919,#39916,#6515,.T.) ;
#50457=EDGE_CURVE('',#39920,#39921,#6516,.T.) ;
#50458=EDGE_CURVE('',#39920,#39922,#401,.T.) ;
#50459=EDGE_CURVE('',#39922,#39923,#6517,.T.) ;
#50460=EDGE_CURVE('',#39923,#39924,#402,.T.) ;
#50461=EDGE_CURVE('',#39924,#39925,#6518,.T.) ;
#50462=EDGE_CURVE('',#39925,#39919,#403,.T.) ;
#50463=EDGE_CURVE('',#39918,#39921,#404,.T.) ;
#50464=EDGE_CURVE('',#39922,#39926,#6519,.T.) ;
#50465=EDGE_CURVE('',#39926,#39927,#6520,.T.) ;
#50466=EDGE_CURVE('',#39927,#39923,#6521,.T.) ;
#50467=EDGE_CURVE('',#39928,#39929,#6522,.T.) ;
#50468=EDGE_CURVE('',#39929,#39930,#6523,.T.) ;
#50469=EDGE_CURVE('',#39930,#39931,#6524,.T.) ;
#50470=EDGE_CURVE('',#39931,#39928,#6525,.T.) ;
#50471=EDGE_CURVE('',#39932,#39933,#6526,.T.) ;
#50472=EDGE_CURVE('',#39933,#39934,#6527,.T.) ;
#50473=EDGE_CURVE('',#39934,#39935,#6528,.T.) ;
#50474=EDGE_CURVE('',#39935,#39932,#6529,.T.) ;
#50475=EDGE_CURVE('',#39936,#39937,#6530,.T.) ;
#50476=EDGE_CURVE('',#39937,#39938,#6531,.T.) ;
#50477=EDGE_CURVE('',#39938,#39939,#6532,.T.) ;
#50478=EDGE_CURVE('',#39939,#39936,#6533,.T.) ;
#50479=EDGE_CURVE('',#39940,#39941,#6534,.T.) ;
#50480=EDGE_CURVE('',#39940,#39942,#405,.T.) ;
#50481=EDGE_CURVE('',#39942,#39943,#6535,.T.) ;
#50482=EDGE_CURVE('',#39943,#39944,#406,.T.) ;
#50483=EDGE_CURVE('',#39944,#39945,#6536,.T.) ;
#50484=EDGE_CURVE('',#39945,#39939,#407,.T.) ;
#50485=EDGE_CURVE('',#39938,#39941,#408,.T.) ;
#50486=EDGE_CURVE('',#39942,#39946,#6537,.T.) ;
#50487=EDGE_CURVE('',#39946,#39947,#6538,.T.) ;
#50488=EDGE_CURVE('',#39947,#39943,#6539,.T.) ;
#50489=EDGE_CURVE('',#39948,#39949,#6540,.T.) ;
#50490=EDGE_CURVE('',#39949,#39950,#6541,.T.) ;
#50491=EDGE_CURVE('',#39950,#39951,#6542,.T.) ;
#50492=EDGE_CURVE('',#39951,#39948,#6543,.T.) ;
#50493=EDGE_CURVE('',#39952,#39953,#6544,.T.) ;
#50494=EDGE_CURVE('',#39953,#39954,#6545,.T.) ;
#50495=EDGE_CURVE('',#39954,#39955,#6546,.T.) ;
#50496=EDGE_CURVE('',#39955,#39952,#6547,.T.) ;
#50497=EDGE_CURVE('',#39956,#39957,#6548,.T.) ;
#50498=EDGE_CURVE('',#39957,#39958,#6549,.T.) ;
#50499=EDGE_CURVE('',#39958,#39959,#6550,.T.) ;
#50500=EDGE_CURVE('',#39959,#39956,#6551,.T.) ;
#50501=EDGE_CURVE('',#39960,#39961,#6552,.T.) ;
#50502=EDGE_CURVE('',#39960,#39962,#409,.T.) ;
#50503=EDGE_CURVE('',#39962,#39963,#6553,.T.) ;
#50504=EDGE_CURVE('',#39963,#39964,#410,.T.) ;
#50505=EDGE_CURVE('',#39964,#39965,#6554,.T.) ;
#50506=EDGE_CURVE('',#39965,#39959,#411,.T.) ;
#50507=EDGE_CURVE('',#39958,#39961,#412,.T.) ;
#50508=EDGE_CURVE('',#39962,#39966,#6555,.T.) ;
#50509=EDGE_CURVE('',#39966,#39967,#6556,.T.) ;
#50510=EDGE_CURVE('',#39967,#39963,#6557,.T.) ;
#50511=EDGE_CURVE('',#39968,#39969,#6558,.T.) ;
#50512=EDGE_CURVE('',#39969,#39970,#6559,.T.) ;
#50513=EDGE_CURVE('',#39970,#39971,#6560,.T.) ;
#50514=EDGE_CURVE('',#39971,#39968,#6561,.T.) ;
#50515=EDGE_CURVE('',#39972,#39973,#6562,.T.) ;
#50516=EDGE_CURVE('',#39973,#39974,#6563,.T.) ;
#50517=EDGE_CURVE('',#39974,#39975,#6564,.T.) ;
#50518=EDGE_CURVE('',#39975,#39972,#6565,.T.) ;
#50519=EDGE_CURVE('',#39976,#39977,#6566,.T.) ;
#50520=EDGE_CURVE('',#39977,#39978,#6567,.T.) ;
#50521=EDGE_CURVE('',#39978,#39979,#6568,.T.) ;
#50522=EDGE_CURVE('',#39979,#39976,#6569,.T.) ;
#50523=EDGE_CURVE('',#39980,#39981,#6570,.T.) ;
#50524=EDGE_CURVE('',#39980,#39982,#413,.T.) ;
#50525=EDGE_CURVE('',#39982,#39983,#6571,.T.) ;
#50526=EDGE_CURVE('',#39983,#39984,#414,.T.) ;
#50527=EDGE_CURVE('',#39984,#39985,#6572,.T.) ;
#50528=EDGE_CURVE('',#39985,#39979,#415,.T.) ;
#50529=EDGE_CURVE('',#39978,#39981,#416,.T.) ;
#50530=EDGE_CURVE('',#39982,#39986,#6573,.T.) ;
#50531=EDGE_CURVE('',#39986,#39987,#6574,.T.) ;
#50532=EDGE_CURVE('',#39987,#39983,#6575,.T.) ;
#50533=EDGE_CURVE('',#39988,#39989,#6576,.T.) ;
#50534=EDGE_CURVE('',#39989,#39990,#6577,.T.) ;
#50535=EDGE_CURVE('',#39990,#39991,#6578,.T.) ;
#50536=EDGE_CURVE('',#39991,#39988,#6579,.T.) ;
#50537=EDGE_CURVE('',#39992,#39993,#6580,.T.) ;
#50538=EDGE_CURVE('',#39993,#39994,#6581,.T.) ;
#50539=EDGE_CURVE('',#39994,#39995,#6582,.T.) ;
#50540=EDGE_CURVE('',#39995,#39992,#6583,.T.) ;
#50541=EDGE_CURVE('',#39996,#39997,#6584,.T.) ;
#50542=EDGE_CURVE('',#39997,#39998,#6585,.T.) ;
#50543=EDGE_CURVE('',#39998,#39999,#6586,.T.) ;
#50544=EDGE_CURVE('',#39999,#39996,#6587,.T.) ;
#50545=EDGE_CURVE('',#40000,#40001,#6588,.T.) ;
#50546=EDGE_CURVE('',#40000,#40002,#417,.T.) ;
#50547=EDGE_CURVE('',#40002,#40003,#6589,.T.) ;
#50548=EDGE_CURVE('',#40003,#40004,#418,.T.) ;
#50549=EDGE_CURVE('',#40004,#40005,#6590,.T.) ;
#50550=EDGE_CURVE('',#40005,#39999,#419,.T.) ;
#50551=EDGE_CURVE('',#39998,#40001,#420,.T.) ;
#50552=EDGE_CURVE('',#40002,#40006,#6591,.T.) ;
#50553=EDGE_CURVE('',#40006,#40007,#6592,.T.) ;
#50554=EDGE_CURVE('',#40007,#40003,#6593,.T.) ;
#50555=EDGE_CURVE('',#40008,#40009,#6594,.T.) ;
#50556=EDGE_CURVE('',#40009,#40010,#6595,.T.) ;
#50557=EDGE_CURVE('',#40010,#40011,#6596,.T.) ;
#50558=EDGE_CURVE('',#40011,#40008,#6597,.T.) ;
#50559=EDGE_CURVE('',#40012,#40013,#6598,.T.) ;
#50560=EDGE_CURVE('',#40013,#40000,#6599,.T.) ;
#50561=EDGE_CURVE('',#40001,#40014,#6600,.T.) ;
#50562=EDGE_CURVE('',#40014,#40015,#6601,.T.) ;
#50563=EDGE_CURVE('',#40015,#40012,#6602,.T.) ;
#50564=EDGE_CURVE('',#40016,#40017,#6603,.T.) ;
#50565=EDGE_CURVE('',#40017,#40018,#421,.T.) ;
#50566=EDGE_CURVE('',#40018,#40019,#6604,.T.) ;
#50567=EDGE_CURVE('',#40019,#39980,#6605,.T.) ;
#50568=EDGE_CURVE('',#39981,#40020,#6606,.T.) ;
#50569=EDGE_CURVE('',#40020,#40021,#6607,.T.) ;
#50570=EDGE_CURVE('',#40021,#40016,#422,.T.) ;
#50571=EDGE_CURVE('',#40022,#40023,#6608,.T.) ;
#50572=EDGE_CURVE('',#40023,#40024,#423,.T.) ;
#50573=EDGE_CURVE('',#40024,#40025,#6609,.T.) ;
#50574=EDGE_CURVE('',#40025,#39960,#6610,.T.) ;
#50575=EDGE_CURVE('',#39961,#40026,#6611,.T.) ;
#50576=EDGE_CURVE('',#40026,#40027,#6612,.T.) ;
#50577=EDGE_CURVE('',#40027,#40022,#424,.T.) ;
#50578=EDGE_CURVE('',#40028,#40029,#6613,.T.) ;
#50579=EDGE_CURVE('',#40029,#40030,#425,.T.) ;
#50580=EDGE_CURVE('',#40030,#40031,#6614,.T.) ;
#50581=EDGE_CURVE('',#40031,#39940,#6615,.T.) ;
#50582=EDGE_CURVE('',#39941,#40032,#6616,.T.) ;
#50583=EDGE_CURVE('',#40032,#40033,#6617,.T.) ;
#50584=EDGE_CURVE('',#40033,#40028,#426,.T.) ;
#50585=EDGE_CURVE('',#40034,#40035,#6618,.T.) ;
#50586=EDGE_CURVE('',#40035,#40036,#427,.T.) ;
#50587=EDGE_CURVE('',#40036,#40037,#6619,.T.) ;
#50588=EDGE_CURVE('',#40037,#39920,#6620,.T.) ;
#50589=EDGE_CURVE('',#39921,#40038,#6621,.T.) ;
#50590=EDGE_CURVE('',#40038,#40039,#6622,.T.) ;
#50591=EDGE_CURVE('',#40039,#40034,#428,.T.) ;
#50592=EDGE_CURVE('',#40040,#40041,#6623,.T.) ;
#50593=EDGE_CURVE('',#40041,#40042,#429,.T.) ;
#50594=EDGE_CURVE('',#40042,#40043,#6624,.T.) ;
#50595=EDGE_CURVE('',#40043,#39900,#6625,.T.) ;
#50596=EDGE_CURVE('',#39901,#40044,#6626,.T.) ;
#50597=EDGE_CURVE('',#40044,#40045,#6627,.T.) ;
#50598=EDGE_CURVE('',#40045,#40040,#430,.T.) ;
#50599=EDGE_CURVE('',#40046,#40047,#6628,.T.) ;
#50600=EDGE_CURVE('',#40047,#40048,#431,.T.) ;
#50601=EDGE_CURVE('',#40048,#40049,#6629,.T.) ;
#50602=EDGE_CURVE('',#40049,#39880,#6630,.T.) ;
#50603=EDGE_CURVE('',#39881,#40050,#6631,.T.) ;
#50604=EDGE_CURVE('',#40050,#40051,#6632,.T.) ;
#50605=EDGE_CURVE('',#40051,#40046,#432,.T.) ;
#50606=EDGE_CURVE('',#40052,#40053,#6633,.T.) ;
#50607=EDGE_CURVE('',#40053,#40054,#433,.T.) ;
#50608=EDGE_CURVE('',#40054,#40055,#6634,.T.) ;
#50609=EDGE_CURVE('',#40055,#39860,#6635,.T.) ;
#50610=EDGE_CURVE('',#39861,#40056,#6636,.T.) ;
#50611=EDGE_CURVE('',#40056,#40057,#6637,.T.) ;
#50612=EDGE_CURVE('',#40057,#40052,#434,.T.) ;
#50613=EDGE_CURVE('',#40058,#40059,#6638,.T.) ;
#50614=EDGE_CURVE('',#40059,#40060,#435,.T.) ;
#50615=EDGE_CURVE('',#40060,#40061,#6639,.T.) ;
#50616=EDGE_CURVE('',#40061,#39840,#6640,.T.) ;
#50617=EDGE_CURVE('',#39841,#40062,#6641,.T.) ;
#50618=EDGE_CURVE('',#40062,#40063,#6642,.T.) ;
#50619=EDGE_CURVE('',#40063,#40058,#436,.T.) ;
#50620=EDGE_CURVE('',#40064,#40065,#6643,.T.) ;
#50621=EDGE_CURVE('',#40065,#40005,#6644,.T.) ;
#50622=EDGE_CURVE('',#40004,#40066,#6645,.T.) ;
#50623=EDGE_CURVE('',#40066,#40067,#6646,.T.) ;
#50624=EDGE_CURVE('',#40067,#40064,#6647,.T.) ;
#50625=EDGE_CURVE('',#40068,#40069,#6648,.T.) ;
#50626=EDGE_CURVE('',#40069,#40070,#437,.T.) ;
#50627=EDGE_CURVE('',#40070,#40071,#6649,.T.) ;
#50628=EDGE_CURVE('',#40071,#39985,#6650,.T.) ;
#50629=EDGE_CURVE('',#39984,#40072,#6651,.T.) ;
#50630=EDGE_CURVE('',#40072,#40073,#6652,.T.) ;
#50631=EDGE_CURVE('',#40073,#40068,#438,.T.) ;
#50632=EDGE_CURVE('',#40074,#40075,#6653,.T.) ;
#50633=EDGE_CURVE('',#40075,#40076,#439,.T.) ;
#50634=EDGE_CURVE('',#40076,#40077,#6654,.T.) ;
#50635=EDGE_CURVE('',#40077,#39965,#6655,.T.) ;
#50636=EDGE_CURVE('',#39964,#40078,#6656,.T.) ;
#50637=EDGE_CURVE('',#40078,#40079,#6657,.T.) ;
#50638=EDGE_CURVE('',#40079,#40074,#440,.T.) ;
#50639=EDGE_CURVE('',#40080,#40081,#6658,.T.) ;
#50640=EDGE_CURVE('',#40081,#40082,#441,.T.) ;
#50641=EDGE_CURVE('',#40082,#40083,#6659,.T.) ;
#50642=EDGE_CURVE('',#40083,#39945,#6660,.T.) ;
#50643=EDGE_CURVE('',#39944,#40084,#6661,.T.) ;
#50644=EDGE_CURVE('',#40084,#40085,#6662,.T.) ;
#50645=EDGE_CURVE('',#40085,#40080,#442,.T.) ;
#50646=EDGE_CURVE('',#40086,#40087,#6663,.T.) ;
#50647=EDGE_CURVE('',#40087,#40088,#443,.T.) ;
#50648=EDGE_CURVE('',#40088,#40089,#6664,.T.) ;
#50649=EDGE_CURVE('',#40089,#39925,#6665,.T.) ;
#50650=EDGE_CURVE('',#39924,#40090,#6666,.T.) ;
#50651=EDGE_CURVE('',#40090,#40091,#6667,.T.) ;
#50652=EDGE_CURVE('',#40091,#40086,#444,.T.) ;
#50653=EDGE_CURVE('',#40092,#40093,#6668,.T.) ;
#50654=EDGE_CURVE('',#40093,#40094,#445,.T.) ;
#50655=EDGE_CURVE('',#40094,#40095,#6669,.T.) ;
#50656=EDGE_CURVE('',#40095,#39905,#6670,.T.) ;
#50657=EDGE_CURVE('',#39904,#40096,#6671,.T.) ;
#50658=EDGE_CURVE('',#40096,#40097,#6672,.T.) ;
#50659=EDGE_CURVE('',#40097,#40092,#446,.T.) ;
#50660=EDGE_CURVE('',#40098,#40099,#6673,.T.) ;
#50661=EDGE_CURVE('',#40099,#40100,#447,.T.) ;
#50662=EDGE_CURVE('',#40100,#40101,#6674,.T.) ;
#50663=EDGE_CURVE('',#40101,#39885,#6675,.T.) ;
#50664=EDGE_CURVE('',#39884,#40102,#6676,.T.) ;
#50665=EDGE_CURVE('',#40102,#40103,#6677,.T.) ;
#50666=EDGE_CURVE('',#40103,#40098,#448,.T.) ;
#50667=EDGE_CURVE('',#40104,#40105,#6678,.T.) ;
#50668=EDGE_CURVE('',#40105,#40106,#449,.T.) ;
#50669=EDGE_CURVE('',#40106,#40107,#6679,.T.) ;
#50670=EDGE_CURVE('',#40107,#39865,#6680,.T.) ;
#50671=EDGE_CURVE('',#39864,#40108,#6681,.T.) ;
#50672=EDGE_CURVE('',#40108,#40109,#6682,.T.) ;
#50673=EDGE_CURVE('',#40109,#40104,#450,.T.) ;
#50674=EDGE_CURVE('',#40110,#40111,#6683,.T.) ;
#50675=EDGE_CURVE('',#40111,#40112,#451,.T.) ;
#50676=EDGE_CURVE('',#40112,#40113,#6684,.T.) ;
#50677=EDGE_CURVE('',#40113,#39845,#6685,.T.) ;
#50678=EDGE_CURVE('',#39844,#40114,#6686,.T.) ;
#50679=EDGE_CURVE('',#40114,#40115,#6687,.T.) ;
#50680=EDGE_CURVE('',#40115,#40110,#452,.T.) ;
#50681=EDGE_CURVE('',#40116,#40117,#6688,.T.) ;
#50682=EDGE_CURVE('',#40117,#40118,#6689,.T.) ;
#50683=EDGE_CURVE('',#40118,#40119,#6690,.T.) ;
#50684=EDGE_CURVE('',#40119,#40116,#6691,.T.) ;
#50685=EDGE_CURVE('',#40120,#40121,#6692,.T.) ;
#50686=EDGE_CURVE('',#40121,#40122,#6693,.T.) ;
#50687=EDGE_CURVE('',#40122,#40123,#6694,.T.) ;
#50688=EDGE_CURVE('',#40123,#40120,#6695,.T.) ;
#50689=EDGE_CURVE('',#40124,#40125,#6696,.T.) ;
#50690=EDGE_CURVE('',#40125,#40126,#6697,.T.) ;
#50691=EDGE_CURVE('',#40126,#40127,#6698,.T.) ;
#50692=EDGE_CURVE('',#40127,#40124,#6699,.T.) ;
#50693=EDGE_CURVE('',#40128,#40129,#6700,.T.) ;
#50694=EDGE_CURVE('',#40129,#40130,#6701,.T.) ;
#50695=EDGE_CURVE('',#40130,#40131,#6702,.T.) ;
#50696=EDGE_CURVE('',#40131,#40128,#6703,.T.) ;
#50697=EDGE_CURVE('',#40132,#40133,#6704,.T.) ;
#50698=EDGE_CURVE('',#40133,#40134,#6705,.T.) ;
#50699=EDGE_CURVE('',#40134,#40135,#6706,.T.) ;
#50700=EDGE_CURVE('',#40135,#40132,#6707,.T.) ;
#50701=EDGE_CURVE('',#40136,#40137,#6708,.T.) ;
#50702=EDGE_CURVE('',#40137,#40138,#6709,.T.) ;
#50703=EDGE_CURVE('',#40138,#40139,#6710,.T.) ;
#50704=EDGE_CURVE('',#40139,#40136,#6711,.T.) ;
#50705=EDGE_CURVE('',#40140,#40141,#6712,.T.) ;
#50706=EDGE_CURVE('',#40141,#40142,#6713,.T.) ;
#50707=EDGE_CURVE('',#40142,#40143,#6714,.T.) ;
#50708=EDGE_CURVE('',#40143,#40140,#6715,.T.) ;
#50709=EDGE_CURVE('',#40144,#40145,#6716,.T.) ;
#50710=EDGE_CURVE('',#40145,#40146,#6717,.T.) ;
#50711=EDGE_CURVE('',#40146,#40147,#6718,.T.) ;
#50712=EDGE_CURVE('',#40147,#40144,#6719,.T.) ;
#50713=EDGE_CURVE('',#40148,#40149,#6720,.T.) ;
#50714=EDGE_CURVE('',#40149,#40150,#6721,.T.) ;
#50715=EDGE_CURVE('',#40150,#40151,#6722,.T.) ;
#50716=EDGE_CURVE('',#40151,#40148,#6723,.T.) ;
#50717=EDGE_CURVE('',#40152,#40153,#6724,.T.) ;
#50718=EDGE_CURVE('',#40153,#40154,#6725,.T.) ;
#50719=EDGE_CURVE('',#40154,#40155,#6726,.T.) ;
#50720=EDGE_CURVE('',#40155,#40152,#6727,.T.) ;
#50721=EDGE_CURVE('',#40156,#40157,#6728,.T.) ;
#50722=EDGE_CURVE('',#40157,#40158,#6729,.T.) ;
#50723=EDGE_CURVE('',#40158,#40159,#6730,.T.) ;
#50724=EDGE_CURVE('',#40159,#40156,#6731,.T.) ;
#50725=EDGE_CURVE('',#40160,#40161,#6732,.T.) ;
#50726=EDGE_CURVE('',#40161,#40162,#6733,.T.) ;
#50727=EDGE_CURVE('',#40162,#40163,#6734,.T.) ;
#50728=EDGE_CURVE('',#40163,#40160,#6735,.T.) ;
#50729=EDGE_CURVE('',#40164,#40165,#6736,.T.) ;
#50730=EDGE_CURVE('',#40165,#40166,#6737,.T.) ;
#50731=EDGE_CURVE('',#40166,#40167,#6738,.T.) ;
#50732=EDGE_CURVE('',#40167,#40164,#6739,.T.) ;
#50733=EDGE_CURVE('',#40168,#40169,#6740,.T.) ;
#50734=EDGE_CURVE('',#40169,#40170,#6741,.T.) ;
#50735=EDGE_CURVE('',#40170,#40171,#6742,.T.) ;
#50736=EDGE_CURVE('',#40171,#40168,#6743,.T.) ;
#50737=EDGE_CURVE('',#40172,#40173,#6744,.T.) ;
#50738=EDGE_CURVE('',#40173,#40174,#6745,.T.) ;
#50739=EDGE_CURVE('',#40174,#40175,#6746,.T.) ;
#50740=EDGE_CURVE('',#40175,#40172,#6747,.T.) ;
#50741=EDGE_CURVE('',#40176,#40177,#6748,.T.) ;
#50742=EDGE_CURVE('',#40177,#40178,#6749,.T.) ;
#50743=EDGE_CURVE('',#40178,#40179,#6750,.T.) ;
#50744=EDGE_CURVE('',#40179,#40176,#6751,.T.) ;
#50745=EDGE_CURVE('',#40180,#40181,#6752,.T.) ;
#50746=EDGE_CURVE('',#40181,#40182,#6753,.T.) ;
#50747=EDGE_CURVE('',#40182,#40183,#6754,.T.) ;
#50748=EDGE_CURVE('',#40183,#40180,#6755,.T.) ;
#50749=EDGE_CURVE('',#40184,#40185,#6756,.T.) ;
#50750=EDGE_CURVE('',#40185,#40186,#6757,.T.) ;
#50751=EDGE_CURVE('',#40186,#40187,#6758,.T.) ;
#50752=EDGE_CURVE('',#40187,#40184,#6759,.T.) ;
#50753=EDGE_CURVE('',#40188,#40189,#6760,.T.) ;
#50754=EDGE_CURVE('',#40189,#40190,#6761,.T.) ;
#50755=EDGE_CURVE('',#40190,#40191,#6762,.T.) ;
#50756=EDGE_CURVE('',#40191,#40188,#6763,.T.) ;
#50757=EDGE_CURVE('',#40192,#40193,#6764,.T.) ;
#50758=EDGE_CURVE('',#40193,#40194,#6765,.T.) ;
#50759=EDGE_CURVE('',#40194,#40195,#6766,.T.) ;
#50760=EDGE_CURVE('',#40195,#40192,#6767,.T.) ;
#50761=EDGE_CURVE('',#40196,#40197,#6768,.T.) ;
#50762=EDGE_CURVE('',#40197,#40198,#6769,.T.) ;
#50763=EDGE_CURVE('',#40198,#40199,#6770,.T.) ;
#50764=EDGE_CURVE('',#40199,#40196,#6771,.T.) ;
#50765=EDGE_CURVE('',#40200,#40201,#6772,.T.) ;
#50766=EDGE_CURVE('',#40201,#40202,#6773,.T.) ;
#50767=EDGE_CURVE('',#40202,#40203,#6774,.T.) ;
#50768=EDGE_CURVE('',#40203,#40200,#6775,.T.) ;
#50769=EDGE_CURVE('',#40204,#40205,#6776,.T.) ;
#50770=EDGE_CURVE('',#40205,#40206,#6777,.T.) ;
#50771=EDGE_CURVE('',#40206,#40207,#6778,.T.) ;
#50772=EDGE_CURVE('',#40207,#40204,#6779,.T.) ;
#50773=EDGE_CURVE('',#40208,#40209,#6780,.T.) ;
#50774=EDGE_CURVE('',#40209,#40210,#6781,.T.) ;
#50775=EDGE_CURVE('',#40210,#40211,#6782,.T.) ;
#50776=EDGE_CURVE('',#40211,#40208,#6783,.T.) ;
#50777=EDGE_CURVE('',#40212,#40213,#6784,.T.) ;
#50778=EDGE_CURVE('',#40213,#40214,#6785,.T.) ;
#50779=EDGE_CURVE('',#40214,#40215,#6786,.T.) ;
#50780=EDGE_CURVE('',#40215,#40212,#6787,.T.) ;
#50781=EDGE_CURVE('',#40216,#40217,#6788,.T.) ;
#50782=EDGE_CURVE('',#40217,#40218,#6789,.T.) ;
#50783=EDGE_CURVE('',#40218,#40219,#6790,.T.) ;
#50784=EDGE_CURVE('',#40219,#40216,#6791,.T.) ;
#50785=EDGE_CURVE('',#40220,#40221,#6792,.T.) ;
#50786=EDGE_CURVE('',#40221,#40222,#6793,.T.) ;
#50787=EDGE_CURVE('',#40222,#40223,#6794,.T.) ;
#50788=EDGE_CURVE('',#40223,#40220,#6795,.T.) ;
#50789=EDGE_CURVE('',#40224,#40225,#6796,.T.) ;
#50790=EDGE_CURVE('',#40225,#40226,#6797,.T.) ;
#50791=EDGE_CURVE('',#40226,#40227,#6798,.T.) ;
#50792=EDGE_CURVE('',#40227,#40224,#6799,.T.) ;
#50793=EDGE_CURVE('',#40228,#40229,#6800,.T.) ;
#50794=EDGE_CURVE('',#40229,#40230,#6801,.T.) ;
#50795=EDGE_CURVE('',#40230,#40231,#6802,.T.) ;
#50796=EDGE_CURVE('',#40231,#40228,#6803,.T.) ;
#50797=EDGE_CURVE('',#40232,#40233,#6804,.T.) ;
#50798=EDGE_CURVE('',#40233,#40234,#6805,.T.) ;
#50799=EDGE_CURVE('',#40234,#40235,#6806,.T.) ;
#50800=EDGE_CURVE('',#40235,#40232,#6807,.T.) ;
#50801=EDGE_CURVE('',#40236,#40237,#6808,.T.) ;
#50802=EDGE_CURVE('',#40237,#40238,#6809,.T.) ;
#50803=EDGE_CURVE('',#40238,#40239,#6810,.T.) ;
#50804=EDGE_CURVE('',#40239,#40236,#6811,.T.) ;
#50805=EDGE_CURVE('',#40240,#40241,#6812,.T.) ;
#50806=EDGE_CURVE('',#40241,#40242,#6813,.T.) ;
#50807=EDGE_CURVE('',#40242,#40243,#6814,.T.) ;
#50808=EDGE_CURVE('',#40243,#40240,#6815,.T.) ;
#50809=EDGE_CURVE('',#40244,#40245,#6816,.T.) ;
#50810=EDGE_CURVE('',#40245,#40246,#6817,.T.) ;
#50811=EDGE_CURVE('',#40246,#40247,#6818,.T.) ;
#50812=EDGE_CURVE('',#40247,#40244,#6819,.T.) ;
#50813=EDGE_CURVE('',#40248,#40249,#6820,.T.) ;
#50814=EDGE_CURVE('',#40249,#40250,#6821,.T.) ;
#50815=EDGE_CURVE('',#40250,#40251,#6822,.T.) ;
#50816=EDGE_CURVE('',#40251,#40248,#6823,.T.) ;
#50817=EDGE_CURVE('',#40252,#40253,#6824,.T.) ;
#50818=EDGE_CURVE('',#40253,#40254,#6825,.T.) ;
#50819=EDGE_CURVE('',#40254,#40255,#6826,.T.) ;
#50820=EDGE_CURVE('',#40255,#40252,#6827,.T.) ;
#50821=EDGE_CURVE('',#40256,#40257,#6828,.T.) ;
#50822=EDGE_CURVE('',#40257,#40258,#6829,.T.) ;
#50823=EDGE_CURVE('',#40258,#40259,#6830,.T.) ;
#50824=EDGE_CURVE('',#40259,#40256,#6831,.T.) ;
#50825=EDGE_CURVE('',#40260,#40261,#6832,.T.) ;
#50826=EDGE_CURVE('',#40261,#40262,#6833,.T.) ;
#50827=EDGE_CURVE('',#40262,#40263,#6834,.T.) ;
#50828=EDGE_CURVE('',#40263,#40260,#6835,.T.) ;
#50829=EDGE_CURVE('',#40264,#40265,#6836,.T.) ;
#50830=EDGE_CURVE('',#40264,#40266,#32958,.T.) ;
#50831=EDGE_CURVE('',#40267,#40266,#6837,.T.) ;
#50832=EDGE_CURVE('',#40267,#40268,#32959,.T.) ;
#50833=EDGE_CURVE('',#40269,#40268,#6838,.T.) ;
#50834=EDGE_CURVE('',#40269,#40270,#32960,.T.) ;
#50835=EDGE_CURVE('',#40271,#40270,#6839,.T.) ;
#50836=EDGE_CURVE('',#40271,#40265,#32961,.T.) ;
#50837=EDGE_CURVE('',#40270,#40272,#6840,.T.) ;
#50838=EDGE_CURVE('',#40272,#40273,#6841,.T.) ;
#50839=EDGE_CURVE('',#40273,#40271,#6842,.T.) ;
#50840=EDGE_CURVE('',#40265,#40274,#6843,.T.) ;
#50841=EDGE_CURVE('',#40274,#40275,#6844,.T.) ;
#50842=EDGE_CURVE('',#40275,#40264,#6845,.T.) ;
#50843=EDGE_CURVE('',#40276,#40277,#6846,.T.) ;
#50844=EDGE_CURVE('',#40277,#40267,#6847,.T.) ;
#50845=EDGE_CURVE('',#40266,#40276,#6848,.T.) ;
#50846=EDGE_CURVE('',#40268,#40278,#6849,.T.) ;
#50847=EDGE_CURVE('',#40278,#40279,#6850,.T.) ;
#50848=EDGE_CURVE('',#40279,#40269,#6851,.T.) ;
#50849=EDGE_CURVE('',#40280,#40281,#6852,.T.) ;
#50850=EDGE_CURVE('',#40281,#40282,#6853,.T.) ;
#50851=EDGE_CURVE('',#40282,#40283,#6854,.T.) ;
#50852=EDGE_CURVE('',#40283,#40280,#6855,.T.) ;
#50853=EDGE_CURVE('',#40284,#40285,#6856,.T.) ;
#50854=EDGE_CURVE('',#40284,#40286,#32962,.T.) ;
#50855=EDGE_CURVE('',#40287,#40286,#6857,.T.) ;
#50856=EDGE_CURVE('',#40287,#40288,#32963,.T.) ;
#50857=EDGE_CURVE('',#40289,#40288,#6858,.T.) ;
#50858=EDGE_CURVE('',#40289,#40290,#32964,.T.) ;
#50859=EDGE_CURVE('',#40291,#40290,#6859,.T.) ;
#50860=EDGE_CURVE('',#40291,#40285,#32965,.T.) ;
#50861=EDGE_CURVE('',#40290,#40292,#6860,.T.) ;
#50862=EDGE_CURVE('',#40292,#40293,#6861,.T.) ;
#50863=EDGE_CURVE('',#40293,#40291,#6862,.T.) ;
#50864=EDGE_CURVE('',#40285,#40294,#6863,.T.) ;
#50865=EDGE_CURVE('',#40294,#40295,#6864,.T.) ;
#50866=EDGE_CURVE('',#40295,#40284,#6865,.T.) ;
#50867=EDGE_CURVE('',#40296,#40297,#6866,.T.) ;
#50868=EDGE_CURVE('',#40297,#40287,#6867,.T.) ;
#50869=EDGE_CURVE('',#40286,#40296,#6868,.T.) ;
#50870=EDGE_CURVE('',#40288,#40298,#6869,.T.) ;
#50871=EDGE_CURVE('',#40298,#40299,#6870,.T.) ;
#50872=EDGE_CURVE('',#40299,#40289,#6871,.T.) ;
#50873=EDGE_CURVE('',#40300,#40301,#6872,.T.) ;
#50874=EDGE_CURVE('',#40301,#40302,#6873,.T.) ;
#50875=EDGE_CURVE('',#40302,#40303,#6874,.T.) ;
#50876=EDGE_CURVE('',#40303,#40300,#6875,.T.) ;
#50877=EDGE_CURVE('',#40304,#40305,#6876,.T.) ;
#50878=EDGE_CURVE('',#40304,#40306,#32966,.T.) ;
#50879=EDGE_CURVE('',#40307,#40306,#6877,.T.) ;
#50880=EDGE_CURVE('',#40307,#40308,#32967,.T.) ;
#50881=EDGE_CURVE('',#40309,#40308,#6878,.T.) ;
#50882=EDGE_CURVE('',#40309,#40310,#32968,.T.) ;
#50883=EDGE_CURVE('',#40311,#40310,#6879,.T.) ;
#50884=EDGE_CURVE('',#40311,#40305,#32969,.T.) ;
#50885=EDGE_CURVE('',#40310,#40312,#6880,.T.) ;
#50886=EDGE_CURVE('',#40312,#40313,#6881,.T.) ;
#50887=EDGE_CURVE('',#40313,#40311,#6882,.T.) ;
#50888=EDGE_CURVE('',#40305,#40314,#6883,.T.) ;
#50889=EDGE_CURVE('',#40314,#40315,#6884,.T.) ;
#50890=EDGE_CURVE('',#40315,#40304,#6885,.T.) ;
#50891=EDGE_CURVE('',#40316,#40317,#6886,.T.) ;
#50892=EDGE_CURVE('',#40317,#40307,#6887,.T.) ;
#50893=EDGE_CURVE('',#40306,#40316,#6888,.T.) ;
#50894=EDGE_CURVE('',#40308,#40318,#6889,.T.) ;
#50895=EDGE_CURVE('',#40318,#40319,#6890,.T.) ;
#50896=EDGE_CURVE('',#40319,#40309,#6891,.T.) ;
#50897=EDGE_CURVE('',#40320,#40321,#6892,.T.) ;
#50898=EDGE_CURVE('',#40321,#40322,#6893,.T.) ;
#50899=EDGE_CURVE('',#40322,#40323,#6894,.T.) ;
#50900=EDGE_CURVE('',#40323,#40320,#6895,.T.) ;
#50901=EDGE_CURVE('',#40324,#40325,#6896,.T.) ;
#50902=EDGE_CURVE('',#40324,#40326,#32970,.T.) ;
#50903=EDGE_CURVE('',#40327,#40326,#6897,.T.) ;
#50904=EDGE_CURVE('',#40327,#40328,#32971,.T.) ;
#50905=EDGE_CURVE('',#40329,#40328,#6898,.T.) ;
#50906=EDGE_CURVE('',#40329,#40330,#32972,.T.) ;
#50907=EDGE_CURVE('',#40331,#40330,#6899,.T.) ;
#50908=EDGE_CURVE('',#40331,#40325,#32973,.T.) ;
#50909=EDGE_CURVE('',#40330,#40332,#6900,.T.) ;
#50910=EDGE_CURVE('',#40332,#40333,#6901,.T.) ;
#50911=EDGE_CURVE('',#40333,#40331,#6902,.T.) ;
#50912=EDGE_CURVE('',#40325,#40334,#6903,.T.) ;
#50913=EDGE_CURVE('',#40334,#40335,#6904,.T.) ;
#50914=EDGE_CURVE('',#40335,#40324,#6905,.T.) ;
#50915=EDGE_CURVE('',#40336,#40337,#6906,.T.) ;
#50916=EDGE_CURVE('',#40337,#40327,#6907,.T.) ;
#50917=EDGE_CURVE('',#40326,#40336,#6908,.T.) ;
#50918=EDGE_CURVE('',#40328,#40338,#6909,.T.) ;
#50919=EDGE_CURVE('',#40338,#40339,#6910,.T.) ;
#50920=EDGE_CURVE('',#40339,#40329,#6911,.T.) ;
#50921=EDGE_CURVE('',#40340,#40341,#6912,.T.) ;
#50922=EDGE_CURVE('',#40341,#40342,#6913,.T.) ;
#50923=EDGE_CURVE('',#40342,#40343,#6914,.T.) ;
#50924=EDGE_CURVE('',#40343,#40340,#6915,.T.) ;
#50925=EDGE_CURVE('',#40344,#40345,#6916,.T.) ;
#50926=EDGE_CURVE('',#40344,#40346,#32974,.T.) ;
#50927=EDGE_CURVE('',#40347,#40346,#6917,.T.) ;
#50928=EDGE_CURVE('',#40347,#40348,#32975,.T.) ;
#50929=EDGE_CURVE('',#40349,#40348,#6918,.T.) ;
#50930=EDGE_CURVE('',#40349,#40350,#32976,.T.) ;
#50931=EDGE_CURVE('',#40351,#40350,#6919,.T.) ;
#50932=EDGE_CURVE('',#40351,#40345,#32977,.T.) ;
#50933=EDGE_CURVE('',#40350,#40352,#6920,.T.) ;
#50934=EDGE_CURVE('',#40352,#40353,#6921,.T.) ;
#50935=EDGE_CURVE('',#40353,#40351,#6922,.T.) ;
#50936=EDGE_CURVE('',#40345,#40354,#6923,.T.) ;
#50937=EDGE_CURVE('',#40354,#40355,#6924,.T.) ;
#50938=EDGE_CURVE('',#40355,#40344,#6925,.T.) ;
#50939=EDGE_CURVE('',#40356,#40357,#6926,.T.) ;
#50940=EDGE_CURVE('',#40357,#40347,#6927,.T.) ;
#50941=EDGE_CURVE('',#40346,#40356,#6928,.T.) ;
#50942=EDGE_CURVE('',#40348,#40358,#6929,.T.) ;
#50943=EDGE_CURVE('',#40358,#40359,#6930,.T.) ;
#50944=EDGE_CURVE('',#40359,#40349,#6931,.T.) ;
#50945=EDGE_CURVE('',#40360,#40361,#6932,.T.) ;
#50946=EDGE_CURVE('',#40361,#40362,#6933,.T.) ;
#50947=EDGE_CURVE('',#40362,#40363,#6934,.T.) ;
#50948=EDGE_CURVE('',#40363,#40360,#6935,.T.) ;
#50949=EDGE_CURVE('',#40364,#40365,#6936,.T.) ;
#50950=EDGE_CURVE('',#40364,#40366,#32978,.T.) ;
#50951=EDGE_CURVE('',#40367,#40366,#6937,.T.) ;
#50952=EDGE_CURVE('',#40367,#40368,#32979,.T.) ;
#50953=EDGE_CURVE('',#40369,#40368,#6938,.T.) ;
#50954=EDGE_CURVE('',#40369,#40370,#32980,.T.) ;
#50955=EDGE_CURVE('',#40371,#40370,#6939,.T.) ;
#50956=EDGE_CURVE('',#40371,#40365,#32981,.T.) ;
#50957=EDGE_CURVE('',#40370,#40372,#6940,.T.) ;
#50958=EDGE_CURVE('',#40372,#40373,#6941,.T.) ;
#50959=EDGE_CURVE('',#40373,#40371,#6942,.T.) ;
#50960=EDGE_CURVE('',#40365,#40374,#6943,.T.) ;
#50961=EDGE_CURVE('',#40374,#40375,#6944,.T.) ;
#50962=EDGE_CURVE('',#40375,#40364,#6945,.T.) ;
#50963=EDGE_CURVE('',#40376,#40377,#6946,.T.) ;
#50964=EDGE_CURVE('',#40377,#40367,#6947,.T.) ;
#50965=EDGE_CURVE('',#40366,#40376,#6948,.T.) ;
#50966=EDGE_CURVE('',#40368,#40378,#6949,.T.) ;
#50967=EDGE_CURVE('',#40378,#40379,#6950,.T.) ;
#50968=EDGE_CURVE('',#40379,#40369,#6951,.T.) ;
#50969=EDGE_CURVE('',#40380,#40381,#6952,.T.) ;
#50970=EDGE_CURVE('',#40381,#40382,#6953,.T.) ;
#50971=EDGE_CURVE('',#40382,#40383,#6954,.T.) ;
#50972=EDGE_CURVE('',#40383,#40380,#6955,.T.) ;
#50973=EDGE_CURVE('',#40384,#40385,#6956,.T.) ;
#50974=EDGE_CURVE('',#40384,#40386,#32982,.T.) ;
#50975=EDGE_CURVE('',#40387,#40386,#6957,.T.) ;
#50976=EDGE_CURVE('',#40387,#40388,#32983,.T.) ;
#50977=EDGE_CURVE('',#40389,#40388,#6958,.T.) ;
#50978=EDGE_CURVE('',#40389,#40390,#32984,.T.) ;
#50979=EDGE_CURVE('',#40391,#40390,#6959,.T.) ;
#50980=EDGE_CURVE('',#40391,#40385,#32985,.T.) ;
#50981=EDGE_CURVE('',#40390,#40392,#6960,.T.) ;
#50982=EDGE_CURVE('',#40392,#40393,#6961,.T.) ;
#50983=EDGE_CURVE('',#40393,#40391,#6962,.T.) ;
#50984=EDGE_CURVE('',#40385,#40394,#6963,.T.) ;
#50985=EDGE_CURVE('',#40394,#40395,#6964,.T.) ;
#50986=EDGE_CURVE('',#40395,#40384,#6965,.T.) ;
#50987=EDGE_CURVE('',#40396,#40397,#6966,.T.) ;
#50988=EDGE_CURVE('',#40397,#40387,#6967,.T.) ;
#50989=EDGE_CURVE('',#40386,#40396,#6968,.T.) ;
#50990=EDGE_CURVE('',#40388,#40398,#6969,.T.) ;
#50991=EDGE_CURVE('',#40398,#40399,#6970,.T.) ;
#50992=EDGE_CURVE('',#40399,#40389,#6971,.T.) ;
#50993=EDGE_CURVE('',#40400,#40401,#6972,.T.) ;
#50994=EDGE_CURVE('',#40401,#40402,#6973,.T.) ;
#50995=EDGE_CURVE('',#40402,#40403,#6974,.T.) ;
#50996=EDGE_CURVE('',#40403,#40400,#6975,.T.) ;
#50997=EDGE_CURVE('',#40404,#40405,#6976,.T.) ;
#50998=EDGE_CURVE('',#40404,#40406,#32986,.T.) ;
#50999=EDGE_CURVE('',#40407,#40406,#6977,.T.) ;
#51000=EDGE_CURVE('',#40407,#40408,#32987,.T.) ;
#51001=EDGE_CURVE('',#40409,#40408,#6978,.T.) ;
#51002=EDGE_CURVE('',#40409,#40410,#32988,.T.) ;
#51003=EDGE_CURVE('',#40411,#40410,#6979,.T.) ;
#51004=EDGE_CURVE('',#40411,#40405,#32989,.T.) ;
#51005=EDGE_CURVE('',#40410,#40412,#6980,.T.) ;
#51006=EDGE_CURVE('',#40412,#40413,#6981,.T.) ;
#51007=EDGE_CURVE('',#40413,#40411,#6982,.T.) ;
#51008=EDGE_CURVE('',#40405,#40414,#6983,.T.) ;
#51009=EDGE_CURVE('',#40414,#40415,#6984,.T.) ;
#51010=EDGE_CURVE('',#40415,#40404,#6985,.T.) ;
#51011=EDGE_CURVE('',#40416,#40417,#6986,.T.) ;
#51012=EDGE_CURVE('',#40417,#40407,#6987,.T.) ;
#51013=EDGE_CURVE('',#40406,#40416,#6988,.T.) ;
#51014=EDGE_CURVE('',#40408,#40418,#6989,.T.) ;
#51015=EDGE_CURVE('',#40418,#40419,#6990,.T.) ;
#51016=EDGE_CURVE('',#40419,#40409,#6991,.T.) ;
#51017=EDGE_CURVE('',#40420,#40421,#6992,.T.) ;
#51018=EDGE_CURVE('',#40421,#40422,#6993,.T.) ;
#51019=EDGE_CURVE('',#40422,#40423,#6994,.T.) ;
#51020=EDGE_CURVE('',#40423,#40420,#6995,.T.) ;
#51021=EDGE_CURVE('',#40424,#40425,#6996,.T.) ;
#51022=EDGE_CURVE('',#40424,#40426,#32990,.T.) ;
#51023=EDGE_CURVE('',#40427,#40426,#6997,.T.) ;
#51024=EDGE_CURVE('',#40427,#40428,#32991,.T.) ;
#51025=EDGE_CURVE('',#40429,#40428,#6998,.T.) ;
#51026=EDGE_CURVE('',#40429,#40430,#32992,.T.) ;
#51027=EDGE_CURVE('',#40431,#40430,#6999,.T.) ;
#51028=EDGE_CURVE('',#40431,#40425,#32993,.T.) ;
#51029=EDGE_CURVE('',#40430,#40432,#7000,.T.) ;
#51030=EDGE_CURVE('',#40432,#40433,#7001,.T.) ;
#51031=EDGE_CURVE('',#40433,#40431,#7002,.T.) ;
#51032=EDGE_CURVE('',#40425,#40434,#7003,.T.) ;
#51033=EDGE_CURVE('',#40434,#40435,#7004,.T.) ;
#51034=EDGE_CURVE('',#40435,#40424,#7005,.T.) ;
#51035=EDGE_CURVE('',#40436,#40437,#7006,.T.) ;
#51036=EDGE_CURVE('',#40437,#40427,#7007,.T.) ;
#51037=EDGE_CURVE('',#40426,#40436,#7008,.T.) ;
#51038=EDGE_CURVE('',#40428,#40438,#7009,.T.) ;
#51039=EDGE_CURVE('',#40438,#40439,#7010,.T.) ;
#51040=EDGE_CURVE('',#40439,#40429,#7011,.T.) ;
#51041=EDGE_CURVE('',#40440,#40441,#7012,.T.) ;
#51042=EDGE_CURVE('',#40441,#40442,#7013,.T.) ;
#51043=EDGE_CURVE('',#40442,#40443,#7014,.T.) ;
#51044=EDGE_CURVE('',#40443,#40440,#7015,.T.) ;
#51045=EDGE_CURVE('',#40444,#40445,#7016,.T.) ;
#51046=EDGE_CURVE('',#40445,#40446,#7017,.T.) ;
#51047=EDGE_CURVE('',#40446,#40447,#7018,.T.) ;
#51048=EDGE_CURVE('',#40447,#40444,#7019,.T.) ;
#51049=EDGE_CURVE('',#40448,#40449,#7020,.T.) ;
#51050=EDGE_CURVE('',#40449,#40450,#7021,.T.) ;
#51051=EDGE_CURVE('',#40450,#40451,#7022,.T.) ;
#51052=EDGE_CURVE('',#40451,#40448,#7023,.T.) ;
#51053=EDGE_CURVE('',#40452,#40453,#7024,.T.) ;
#51054=EDGE_CURVE('',#40453,#40454,#7025,.T.) ;
#51055=EDGE_CURVE('',#40454,#40455,#7026,.T.) ;
#51056=EDGE_CURVE('',#40455,#40452,#7027,.T.) ;
#51057=EDGE_CURVE('',#40456,#40457,#7028,.T.) ;
#51058=EDGE_CURVE('',#40457,#40458,#7029,.T.) ;
#51059=EDGE_CURVE('',#40458,#40459,#7030,.T.) ;
#51060=EDGE_CURVE('',#40459,#40456,#7031,.T.) ;
#51061=EDGE_CURVE('',#40460,#40461,#7032,.T.) ;
#51062=EDGE_CURVE('',#40461,#40462,#7033,.T.) ;
#51063=EDGE_CURVE('',#40462,#40463,#7034,.T.) ;
#51064=EDGE_CURVE('',#40463,#40460,#7035,.T.) ;
#51065=EDGE_CURVE('',#40464,#40465,#7036,.T.) ;
#51066=EDGE_CURVE('',#40465,#40466,#7037,.T.) ;
#51067=EDGE_CURVE('',#40466,#40467,#7038,.T.) ;
#51068=EDGE_CURVE('',#40467,#40464,#7039,.T.) ;
#51069=EDGE_CURVE('',#40468,#40469,#7040,.T.) ;
#51070=EDGE_CURVE('',#40469,#40470,#7041,.T.) ;
#51071=EDGE_CURVE('',#40470,#40471,#7042,.T.) ;
#51072=EDGE_CURVE('',#40471,#40468,#7043,.T.) ;
#51073=EDGE_CURVE('',#40472,#40473,#7044,.T.) ;
#51074=EDGE_CURVE('',#40473,#40474,#7045,.T.) ;
#51075=EDGE_CURVE('',#40474,#40475,#7046,.T.) ;
#51076=EDGE_CURVE('',#40475,#40472,#7047,.T.) ;
#51077=EDGE_CURVE('',#40476,#40477,#32994,.T.) ;
#51078=EDGE_CURVE('',#40477,#40478,#32995,.T.) ;
#51079=EDGE_CURVE('',#40478,#40479,#7048,.T.) ;
#51080=EDGE_CURVE('',#40479,#40480,#7049,.T.) ;
#51081=EDGE_CURVE('',#40480,#40481,#7050,.T.) ;
#51082=EDGE_CURVE('',#40481,#40482,#7051,.T.) ;
#51083=EDGE_CURVE('',#40483,#40482,#32996,.T.) ;
#51084=EDGE_CURVE('',#40483,#40484,#7052,.T.) ;
#51085=EDGE_CURVE('',#40484,#40485,#7053,.T.) ;
#51086=EDGE_CURVE('',#40485,#40476,#7054,.T.) ;
#51087=EDGE_CURVE('',#40486,#40487,#7055,.T.) ;
#51088=EDGE_CURVE('',#40487,#40488,#7056,.T.) ;
#51089=EDGE_CURVE('',#40488,#40489,#7057,.T.) ;
#51090=EDGE_CURVE('',#40489,#40486,#7058,.T.) ;
#51091=EDGE_CURVE('',#40490,#40491,#7059,.T.) ;
#51092=EDGE_CURVE('',#40491,#40492,#32997,.T.) ;
#51093=EDGE_CURVE('',#40492,#40493,#32998,.T.) ;
#51094=EDGE_CURVE('',#40493,#40494,#7060,.T.) ;
#51095=EDGE_CURVE('',#40494,#40495,#7061,.T.) ;
#51096=EDGE_CURVE('',#40495,#40496,#7062,.T.) ;
#51097=EDGE_CURVE('',#40497,#40496,#32999,.T.) ;
#51098=EDGE_CURVE('',#40497,#40498,#7063,.T.) ;
#51099=EDGE_CURVE('',#40498,#40499,#7064,.T.) ;
#51100=EDGE_CURVE('',#40499,#40490,#7065,.T.) ;
#51101=EDGE_CURVE('',#40500,#40501,#7066,.T.) ;
#51102=EDGE_CURVE('',#40501,#40502,#7067,.T.) ;
#51103=EDGE_CURVE('',#40502,#40503,#7068,.T.) ;
#51104=EDGE_CURVE('',#40503,#40500,#7069,.T.) ;
#51105=EDGE_CURVE('',#40504,#40505,#33000,.T.) ;
#51106=EDGE_CURVE('',#40505,#40506,#33001,.T.) ;
#51107=EDGE_CURVE('',#40506,#40507,#7070,.T.) ;
#51108=EDGE_CURVE('',#40507,#40508,#7071,.T.) ;
#51109=EDGE_CURVE('',#40508,#40509,#7072,.T.) ;
#51110=EDGE_CURVE('',#40509,#40510,#7073,.T.) ;
#51111=EDGE_CURVE('',#40511,#40510,#33002,.T.) ;
#51112=EDGE_CURVE('',#40511,#40512,#7074,.T.) ;
#51113=EDGE_CURVE('',#40512,#40513,#7075,.T.) ;
#51114=EDGE_CURVE('',#40513,#40504,#7076,.T.) ;
#51115=EDGE_CURVE('',#40514,#40515,#7077,.T.) ;
#51116=EDGE_CURVE('',#40515,#40516,#7078,.T.) ;
#51117=EDGE_CURVE('',#40516,#40517,#7079,.T.) ;
#51118=EDGE_CURVE('',#40517,#40514,#7080,.T.) ;
#51119=EDGE_CURVE('',#40518,#40519,#7081,.T.) ;
#51120=EDGE_CURVE('',#40519,#40520,#33003,.T.) ;
#51121=EDGE_CURVE('',#40520,#40521,#33004,.T.) ;
#51122=EDGE_CURVE('',#40521,#40522,#7082,.T.) ;
#51123=EDGE_CURVE('',#40522,#40523,#7083,.T.) ;
#51124=EDGE_CURVE('',#40523,#40524,#7084,.T.) ;
#51125=EDGE_CURVE('',#40525,#40524,#33005,.T.) ;
#51126=EDGE_CURVE('',#40525,#40526,#7085,.T.) ;
#51127=EDGE_CURVE('',#40526,#40527,#7086,.T.) ;
#51128=EDGE_CURVE('',#40527,#40518,#7087,.T.) ;
#51129=EDGE_CURVE('',#40528,#40529,#7088,.T.) ;
#51130=EDGE_CURVE('',#40529,#40530,#7089,.T.) ;
#51131=EDGE_CURVE('',#40530,#40531,#7090,.T.) ;
#51132=EDGE_CURVE('',#40531,#40528,#7091,.T.) ;
#51133=EDGE_CURVE('',#40532,#40533,#33006,.T.) ;
#51134=EDGE_CURVE('',#40533,#40534,#33007,.T.) ;
#51135=EDGE_CURVE('',#40534,#40535,#7092,.T.) ;
#51136=EDGE_CURVE('',#40535,#40536,#7093,.T.) ;
#51137=EDGE_CURVE('',#40536,#40537,#7094,.T.) ;
#51138=EDGE_CURVE('',#40537,#40538,#7095,.T.) ;
#51139=EDGE_CURVE('',#40539,#40538,#33008,.T.) ;
#51140=EDGE_CURVE('',#40539,#40540,#7096,.T.) ;
#51141=EDGE_CURVE('',#40540,#40541,#7097,.T.) ;
#51142=EDGE_CURVE('',#40541,#40532,#7098,.T.) ;
#51143=EDGE_CURVE('',#40542,#40543,#7099,.T.) ;
#51144=EDGE_CURVE('',#40543,#40544,#7100,.T.) ;
#51145=EDGE_CURVE('',#40544,#40545,#7101,.T.) ;
#51146=EDGE_CURVE('',#40545,#40542,#7102,.T.) ;
#51147=EDGE_CURVE('',#40546,#40547,#7103,.T.) ;
#51148=EDGE_CURVE('',#40547,#40548,#33009,.T.) ;
#51149=EDGE_CURVE('',#40548,#40549,#33010,.T.) ;
#51150=EDGE_CURVE('',#40549,#40550,#7104,.T.) ;
#51151=EDGE_CURVE('',#40550,#40551,#7105,.T.) ;
#51152=EDGE_CURVE('',#40551,#40552,#7106,.T.) ;
#51153=EDGE_CURVE('',#40553,#40552,#33011,.T.) ;
#51154=EDGE_CURVE('',#40553,#40554,#7107,.T.) ;
#51155=EDGE_CURVE('',#40554,#40555,#7108,.T.) ;
#51156=EDGE_CURVE('',#40555,#40546,#7109,.T.) ;
#51157=EDGE_CURVE('',#40556,#40557,#7110,.T.) ;
#51158=EDGE_CURVE('',#40557,#40558,#7111,.T.) ;
#51159=EDGE_CURVE('',#40558,#40559,#7112,.T.) ;
#51160=EDGE_CURVE('',#40559,#40556,#7113,.T.) ;
#51161=EDGE_CURVE('',#40560,#40561,#33012,.T.) ;
#51162=EDGE_CURVE('',#40561,#40562,#33013,.T.) ;
#51163=EDGE_CURVE('',#40562,#40563,#7114,.T.) ;
#51164=EDGE_CURVE('',#40563,#40564,#7115,.T.) ;
#51165=EDGE_CURVE('',#40564,#40565,#7116,.T.) ;
#51166=EDGE_CURVE('',#40565,#40566,#7117,.T.) ;
#51167=EDGE_CURVE('',#40567,#40566,#33014,.T.) ;
#51168=EDGE_CURVE('',#40567,#40568,#7118,.T.) ;
#51169=EDGE_CURVE('',#40568,#40569,#7119,.T.) ;
#51170=EDGE_CURVE('',#40569,#40560,#7120,.T.) ;
#51171=EDGE_CURVE('',#40570,#40571,#7121,.T.) ;
#51172=EDGE_CURVE('',#40571,#40572,#7122,.T.) ;
#51173=EDGE_CURVE('',#40572,#40573,#7123,.T.) ;
#51174=EDGE_CURVE('',#40573,#40570,#7124,.T.) ;
#51175=EDGE_CURVE('',#40574,#40575,#7125,.T.) ;
#51176=EDGE_CURVE('',#40575,#40576,#33015,.T.) ;
#51177=EDGE_CURVE('',#40576,#40577,#33016,.T.) ;
#51178=EDGE_CURVE('',#40577,#40578,#7126,.T.) ;
#51179=EDGE_CURVE('',#40578,#40579,#7127,.T.) ;
#51180=EDGE_CURVE('',#40579,#40580,#7128,.T.) ;
#51181=EDGE_CURVE('',#40581,#40580,#33017,.T.) ;
#51182=EDGE_CURVE('',#40581,#40582,#7129,.T.) ;
#51183=EDGE_CURVE('',#40582,#40583,#7130,.T.) ;
#51184=EDGE_CURVE('',#40583,#40574,#7131,.T.) ;
#51185=EDGE_CURVE('',#40584,#40585,#7132,.T.) ;
#51186=EDGE_CURVE('',#40585,#40586,#7133,.T.) ;
#51187=EDGE_CURVE('',#40586,#40587,#7134,.T.) ;
#51188=EDGE_CURVE('',#40587,#40584,#7135,.T.) ;
#51189=EDGE_CURVE('',#40588,#40589,#33018,.T.) ;
#51190=EDGE_CURVE('',#40589,#40590,#33019,.T.) ;
#51191=EDGE_CURVE('',#40590,#40591,#7136,.T.) ;
#51192=EDGE_CURVE('',#40591,#40592,#7137,.T.) ;
#51193=EDGE_CURVE('',#40592,#40593,#7138,.T.) ;
#51194=EDGE_CURVE('',#40593,#40594,#7139,.T.) ;
#51195=EDGE_CURVE('',#40595,#40594,#33020,.T.) ;
#51196=EDGE_CURVE('',#40595,#40596,#7140,.T.) ;
#51197=EDGE_CURVE('',#40596,#40597,#7141,.T.) ;
#51198=EDGE_CURVE('',#40597,#40588,#7142,.T.) ;
#51199=EDGE_CURVE('',#40598,#40599,#7143,.T.) ;
#51200=EDGE_CURVE('',#40599,#40600,#7144,.T.) ;
#51201=EDGE_CURVE('',#40600,#40601,#7145,.T.) ;
#51202=EDGE_CURVE('',#40601,#40598,#7146,.T.) ;
#51203=EDGE_CURVE('',#40602,#40603,#7147,.T.) ;
#51204=EDGE_CURVE('',#40603,#40604,#33021,.T.) ;
#51205=EDGE_CURVE('',#40604,#40605,#33022,.T.) ;
#51206=EDGE_CURVE('',#40605,#40606,#7148,.T.) ;
#51207=EDGE_CURVE('',#40606,#40607,#7149,.T.) ;
#51208=EDGE_CURVE('',#40607,#40608,#7150,.T.) ;
#51209=EDGE_CURVE('',#40609,#40608,#33023,.T.) ;
#51210=EDGE_CURVE('',#40609,#40610,#7151,.T.) ;
#51211=EDGE_CURVE('',#40610,#40611,#7152,.T.) ;
#51212=EDGE_CURVE('',#40611,#40602,#7153,.T.) ;
#51213=EDGE_CURVE('',#40612,#40613,#7154,.T.) ;
#51214=EDGE_CURVE('',#40613,#40614,#7155,.T.) ;
#51215=EDGE_CURVE('',#40614,#40615,#7156,.T.) ;
#51216=EDGE_CURVE('',#40615,#40612,#7157,.T.) ;
#51217=EDGE_CURVE('',#40616,#40617,#33024,.T.) ;
#51218=EDGE_CURVE('',#40617,#40618,#33025,.T.) ;
#51219=EDGE_CURVE('',#40618,#40619,#7158,.T.) ;
#51220=EDGE_CURVE('',#40619,#40620,#7159,.T.) ;
#51221=EDGE_CURVE('',#40620,#40621,#7160,.T.) ;
#51222=EDGE_CURVE('',#40621,#40622,#7161,.T.) ;
#51223=EDGE_CURVE('',#40623,#40622,#33026,.T.) ;
#51224=EDGE_CURVE('',#40623,#40624,#7162,.T.) ;
#51225=EDGE_CURVE('',#40624,#40625,#7163,.T.) ;
#51226=EDGE_CURVE('',#40625,#40616,#7164,.T.) ;
#51227=EDGE_CURVE('',#40626,#40627,#7165,.T.) ;
#51228=EDGE_CURVE('',#40627,#40628,#7166,.T.) ;
#51229=EDGE_CURVE('',#40628,#40629,#7167,.T.) ;
#51230=EDGE_CURVE('',#40629,#40626,#7168,.T.) ;
#51231=EDGE_CURVE('',#40630,#40631,#7169,.T.) ;
#51232=EDGE_CURVE('',#40631,#40632,#33027,.T.) ;
#51233=EDGE_CURVE('',#40632,#40633,#33028,.T.) ;
#51234=EDGE_CURVE('',#40633,#40634,#7170,.T.) ;
#51235=EDGE_CURVE('',#40634,#40635,#7171,.T.) ;
#51236=EDGE_CURVE('',#40635,#40636,#7172,.T.) ;
#51237=EDGE_CURVE('',#40637,#40636,#33029,.T.) ;
#51238=EDGE_CURVE('',#40637,#40638,#7173,.T.) ;
#51239=EDGE_CURVE('',#40638,#40639,#7174,.T.) ;
#51240=EDGE_CURVE('',#40639,#40630,#7175,.T.) ;
#51241=EDGE_CURVE('',#40640,#40641,#7176,.T.) ;
#51242=EDGE_CURVE('',#40641,#40642,#7177,.T.) ;
#51243=EDGE_CURVE('',#40642,#40643,#7178,.T.) ;
#51244=EDGE_CURVE('',#40643,#40640,#7179,.T.) ;
#51245=EDGE_CURVE('',#40644,#40645,#33030,.T.) ;
#51246=EDGE_CURVE('',#40645,#40646,#33031,.T.) ;
#51247=EDGE_CURVE('',#40646,#40647,#7180,.T.) ;
#51248=EDGE_CURVE('',#40647,#40648,#7181,.T.) ;
#51249=EDGE_CURVE('',#40648,#40649,#7182,.T.) ;
#51250=EDGE_CURVE('',#40649,#40650,#7183,.T.) ;
#51251=EDGE_CURVE('',#40651,#40650,#33032,.T.) ;
#51252=EDGE_CURVE('',#40651,#40652,#7184,.T.) ;
#51253=EDGE_CURVE('',#40652,#40653,#7185,.T.) ;
#51254=EDGE_CURVE('',#40653,#40644,#7186,.T.) ;
#51255=EDGE_CURVE('',#40654,#40655,#7187,.T.) ;
#51256=EDGE_CURVE('',#40655,#40656,#7188,.T.) ;
#51257=EDGE_CURVE('',#40656,#40657,#7189,.T.) ;
#51258=EDGE_CURVE('',#40657,#40654,#7190,.T.) ;
#51259=EDGE_CURVE('',#40658,#40659,#7191,.T.) ;
#51260=EDGE_CURVE('',#40659,#40660,#33033,.T.) ;
#51261=EDGE_CURVE('',#40660,#40661,#33034,.T.) ;
#51262=EDGE_CURVE('',#40661,#40662,#7192,.T.) ;
#51263=EDGE_CURVE('',#40662,#40663,#7193,.T.) ;
#51264=EDGE_CURVE('',#40663,#40664,#7194,.T.) ;
#51265=EDGE_CURVE('',#40665,#40664,#33035,.T.) ;
#51266=EDGE_CURVE('',#40665,#40666,#7195,.T.) ;
#51267=EDGE_CURVE('',#40666,#40667,#7196,.T.) ;
#51268=EDGE_CURVE('',#40667,#40658,#7197,.T.) ;
#51269=EDGE_CURVE('',#40668,#40669,#7198,.T.) ;
#51270=EDGE_CURVE('',#40669,#40670,#7199,.T.) ;
#51271=EDGE_CURVE('',#40670,#40671,#7200,.T.) ;
#51272=EDGE_CURVE('',#40671,#40668,#7201,.T.) ;
#51273=EDGE_CURVE('',#40672,#40673,#33036,.T.) ;
#51274=EDGE_CURVE('',#40673,#40674,#33037,.T.) ;
#51275=EDGE_CURVE('',#40674,#40675,#7202,.T.) ;
#51276=EDGE_CURVE('',#40675,#40676,#7203,.T.) ;
#51277=EDGE_CURVE('',#40676,#40677,#7204,.T.) ;
#51278=EDGE_CURVE('',#40677,#40678,#7205,.T.) ;
#51279=EDGE_CURVE('',#40679,#40678,#33038,.T.) ;
#51280=EDGE_CURVE('',#40679,#40680,#7206,.T.) ;
#51281=EDGE_CURVE('',#40680,#40681,#7207,.T.) ;
#51282=EDGE_CURVE('',#40681,#40672,#7208,.T.) ;
#51283=EDGE_CURVE('',#40682,#40683,#7209,.T.) ;
#51284=EDGE_CURVE('',#40683,#40684,#7210,.T.) ;
#51285=EDGE_CURVE('',#40684,#40685,#7211,.T.) ;
#51286=EDGE_CURVE('',#40685,#40682,#7212,.T.) ;
#51287=EDGE_CURVE('',#40686,#40687,#7213,.T.) ;
#51288=EDGE_CURVE('',#40687,#40688,#33039,.T.) ;
#51289=EDGE_CURVE('',#40688,#40689,#33040,.T.) ;
#51290=EDGE_CURVE('',#40689,#40690,#7214,.T.) ;
#51291=EDGE_CURVE('',#40690,#40691,#7215,.T.) ;
#51292=EDGE_CURVE('',#40691,#40692,#7216,.T.) ;
#51293=EDGE_CURVE('',#40693,#40692,#33041,.T.) ;
#51294=EDGE_CURVE('',#40693,#40694,#7217,.T.) ;
#51295=EDGE_CURVE('',#40694,#40695,#7218,.T.) ;
#51296=EDGE_CURVE('',#40695,#40686,#7219,.T.) ;
#51297=EDGE_CURVE('',#40696,#40697,#7220,.T.) ;
#51298=EDGE_CURVE('',#40697,#40698,#7221,.T.) ;
#51299=EDGE_CURVE('',#40698,#40699,#7222,.T.) ;
#51300=EDGE_CURVE('',#40699,#40696,#7223,.T.) ;
#51301=EDGE_CURVE('',#40700,#40701,#33042,.T.) ;
#51302=EDGE_CURVE('',#40701,#40702,#33043,.T.) ;
#51303=EDGE_CURVE('',#40702,#40703,#7224,.T.) ;
#51304=EDGE_CURVE('',#40703,#40704,#7225,.T.) ;
#51305=EDGE_CURVE('',#40704,#40705,#7226,.T.) ;
#51306=EDGE_CURVE('',#40705,#40706,#7227,.T.) ;
#51307=EDGE_CURVE('',#40707,#40706,#33044,.T.) ;
#51308=EDGE_CURVE('',#40707,#40708,#7228,.T.) ;
#51309=EDGE_CURVE('',#40708,#40709,#7229,.T.) ;
#51310=EDGE_CURVE('',#40709,#40700,#7230,.T.) ;
#51311=EDGE_CURVE('',#40710,#40711,#7231,.T.) ;
#51312=EDGE_CURVE('',#40711,#40712,#7232,.T.) ;
#51313=EDGE_CURVE('',#40712,#40713,#7233,.T.) ;
#51314=EDGE_CURVE('',#40713,#40710,#7234,.T.) ;
#51315=EDGE_CURVE('',#40714,#40715,#7235,.T.) ;
#51316=EDGE_CURVE('',#40715,#40716,#33045,.T.) ;
#51317=EDGE_CURVE('',#40716,#40717,#33046,.T.) ;
#51318=EDGE_CURVE('',#40717,#40718,#7236,.T.) ;
#51319=EDGE_CURVE('',#40718,#40719,#7237,.T.) ;
#51320=EDGE_CURVE('',#40719,#40720,#7238,.T.) ;
#51321=EDGE_CURVE('',#40721,#40720,#33047,.T.) ;
#51322=EDGE_CURVE('',#40721,#40722,#7239,.T.) ;
#51323=EDGE_CURVE('',#40722,#40723,#7240,.T.) ;
#51324=EDGE_CURVE('',#40723,#40714,#7241,.T.) ;
#51325=EDGE_CURVE('',#40724,#40725,#7242,.T.) ;
#51326=EDGE_CURVE('',#40725,#40726,#7243,.T.) ;
#51327=EDGE_CURVE('',#40726,#40727,#7244,.T.) ;
#51328=EDGE_CURVE('',#40727,#40724,#7245,.T.) ;
#51329=EDGE_CURVE('',#40728,#40729,#7246,.T.) ;
#51330=EDGE_CURVE('',#40729,#40730,#7247,.T.) ;
#51331=EDGE_CURVE('',#40730,#40731,#7248,.T.) ;
#51332=EDGE_CURVE('',#40731,#40728,#7249,.T.) ;
#51333=EDGE_CURVE('',#40732,#40733,#7250,.T.) ;
#51334=EDGE_CURVE('',#40733,#40734,#7251,.T.) ;
#51335=EDGE_CURVE('',#40734,#40735,#7252,.T.) ;
#51336=EDGE_CURVE('',#40735,#40732,#7253,.T.) ;
#51337=EDGE_CURVE('',#40736,#40737,#7254,.T.) ;
#51338=EDGE_CURVE('',#40737,#40738,#33048,.T.) ;
#51339=EDGE_CURVE('',#40738,#40739,#7255,.T.) ;
#51340=EDGE_CURVE('',#40739,#40736,#33049,.T.) ;
#51341=EDGE_CURVE('',#40740,#40741,#7256,.T.) ;
#51342=EDGE_CURVE('',#40741,#40742,#33050,.T.) ;
#51343=EDGE_CURVE('',#40742,#40743,#7257,.T.) ;
#51344=EDGE_CURVE('',#40743,#40744,#7258,.T.) ;
#51345=EDGE_CURVE('',#40744,#40745,#7259,.T.) ;
#51346=EDGE_CURVE('',#40745,#40740,#7260,.T.) ;
#51347=EDGE_CURVE('',#40746,#40747,#7261,.T.) ;
#51348=EDGE_CURVE('',#40747,#40748,#7262,.T.) ;
#51349=EDGE_CURVE('',#40748,#40749,#7263,.T.) ;
#51350=EDGE_CURVE('',#40749,#40746,#7264,.T.) ;
#51351=EDGE_CURVE('',#40750,#40751,#7265,.T.) ;
#51352=EDGE_CURVE('',#40751,#40752,#7266,.T.) ;
#51353=EDGE_CURVE('',#40752,#40753,#7267,.T.) ;
#51354=EDGE_CURVE('',#40753,#40750,#7268,.T.) ;
#51355=EDGE_CURVE('',#40754,#40755,#7269,.T.) ;
#51356=EDGE_CURVE('',#40755,#40756,#33051,.T.) ;
#51357=EDGE_CURVE('',#40756,#40757,#7270,.T.) ;
#51358=EDGE_CURVE('',#40757,#40754,#33052,.T.) ;
#51359=EDGE_CURVE('',#40758,#40759,#7271,.T.) ;
#51360=EDGE_CURVE('',#40759,#40760,#33053,.T.) ;
#51361=EDGE_CURVE('',#40760,#40761,#7272,.T.) ;
#51362=EDGE_CURVE('',#40761,#40762,#7273,.T.) ;
#51363=EDGE_CURVE('',#40762,#40763,#7274,.T.) ;
#51364=EDGE_CURVE('',#40763,#40758,#7275,.T.) ;
#51365=EDGE_CURVE('',#40764,#40765,#7276,.T.) ;
#51366=EDGE_CURVE('',#40765,#40766,#7277,.T.) ;
#51367=EDGE_CURVE('',#40766,#40767,#7278,.T.) ;
#51368=EDGE_CURVE('',#40767,#40764,#7279,.T.) ;
#51369=EDGE_CURVE('',#40768,#40769,#7280,.T.) ;
#51370=EDGE_CURVE('',#40769,#40770,#7281,.T.) ;
#51371=EDGE_CURVE('',#40770,#40771,#7282,.T.) ;
#51372=EDGE_CURVE('',#40771,#40768,#7283,.T.) ;
#51373=EDGE_CURVE('',#40772,#40773,#7284,.T.) ;
#51374=EDGE_CURVE('',#40773,#40774,#33054,.T.) ;
#51375=EDGE_CURVE('',#40774,#40775,#7285,.T.) ;
#51376=EDGE_CURVE('',#40775,#40772,#33055,.T.) ;
#51377=EDGE_CURVE('',#40776,#40777,#7286,.T.) ;
#51378=EDGE_CURVE('',#40777,#40778,#33056,.T.) ;
#51379=EDGE_CURVE('',#40778,#40779,#7287,.T.) ;
#51380=EDGE_CURVE('',#40779,#40780,#7288,.T.) ;
#51381=EDGE_CURVE('',#40780,#40781,#7289,.T.) ;
#51382=EDGE_CURVE('',#40781,#40776,#7290,.T.) ;
#51383=EDGE_CURVE('',#40782,#40783,#7291,.T.) ;
#51384=EDGE_CURVE('',#40783,#40784,#7292,.T.) ;
#51385=EDGE_CURVE('',#40784,#40785,#7293,.T.) ;
#51386=EDGE_CURVE('',#40785,#40782,#7294,.T.) ;
#51387=EDGE_CURVE('',#40786,#40787,#7295,.T.) ;
#51388=EDGE_CURVE('',#40787,#40788,#7296,.T.) ;
#51389=EDGE_CURVE('',#40788,#40789,#7297,.T.) ;
#51390=EDGE_CURVE('',#40789,#40786,#7298,.T.) ;
#51391=EDGE_CURVE('',#40790,#40791,#7299,.T.) ;
#51392=EDGE_CURVE('',#40791,#40792,#33057,.T.) ;
#51393=EDGE_CURVE('',#40792,#40793,#7300,.T.) ;
#51394=EDGE_CURVE('',#40793,#40790,#33058,.T.) ;
#51395=EDGE_CURVE('',#40794,#40795,#7301,.T.) ;
#51396=EDGE_CURVE('',#40795,#40796,#33059,.T.) ;
#51397=EDGE_CURVE('',#40796,#40797,#7302,.T.) ;
#51398=EDGE_CURVE('',#40797,#40798,#7303,.T.) ;
#51399=EDGE_CURVE('',#40798,#40799,#7304,.T.) ;
#51400=EDGE_CURVE('',#40799,#40794,#7305,.T.) ;
#51401=EDGE_CURVE('',#40800,#40801,#7306,.T.) ;
#51402=EDGE_CURVE('',#40801,#40802,#7307,.T.) ;
#51403=EDGE_CURVE('',#40802,#40803,#7308,.T.) ;
#51404=EDGE_CURVE('',#40803,#40800,#7309,.T.) ;
#51405=EDGE_CURVE('',#40804,#40805,#7310,.T.) ;
#51406=EDGE_CURVE('',#40805,#40806,#7311,.T.) ;
#51407=EDGE_CURVE('',#40806,#40807,#7312,.T.) ;
#51408=EDGE_CURVE('',#40807,#40804,#7313,.T.) ;
#51409=EDGE_CURVE('',#40808,#40809,#7314,.T.) ;
#51410=EDGE_CURVE('',#40809,#40810,#33060,.T.) ;
#51411=EDGE_CURVE('',#40810,#40811,#7315,.T.) ;
#51412=EDGE_CURVE('',#40811,#40808,#33061,.T.) ;
#51413=EDGE_CURVE('',#40812,#40813,#7316,.T.) ;
#51414=EDGE_CURVE('',#40813,#40814,#33062,.T.) ;
#51415=EDGE_CURVE('',#40814,#40815,#7317,.T.) ;
#51416=EDGE_CURVE('',#40815,#40816,#7318,.T.) ;
#51417=EDGE_CURVE('',#40816,#40817,#7319,.T.) ;
#51418=EDGE_CURVE('',#40817,#40812,#7320,.T.) ;
#51419=EDGE_CURVE('',#40818,#40819,#7321,.T.) ;
#51420=EDGE_CURVE('',#40819,#40820,#7322,.T.) ;
#51421=EDGE_CURVE('',#40820,#40821,#7323,.T.) ;
#51422=EDGE_CURVE('',#40821,#40818,#7324,.T.) ;
#51423=EDGE_CURVE('',#40822,#40823,#7325,.T.) ;
#51424=EDGE_CURVE('',#40823,#40824,#7326,.T.) ;
#51425=EDGE_CURVE('',#40824,#40825,#7327,.T.) ;
#51426=EDGE_CURVE('',#40825,#40822,#7328,.T.) ;
#51427=EDGE_CURVE('',#40826,#40827,#7329,.T.) ;
#51428=EDGE_CURVE('',#40827,#40828,#33063,.T.) ;
#51429=EDGE_CURVE('',#40828,#40829,#7330,.T.) ;
#51430=EDGE_CURVE('',#40829,#40826,#33064,.T.) ;
#51431=EDGE_CURVE('',#40830,#40831,#7331,.T.) ;
#51432=EDGE_CURVE('',#40831,#40832,#33065,.T.) ;
#51433=EDGE_CURVE('',#40832,#40833,#7332,.T.) ;
#51434=EDGE_CURVE('',#40833,#40834,#7333,.T.) ;
#51435=EDGE_CURVE('',#40834,#40835,#7334,.T.) ;
#51436=EDGE_CURVE('',#40835,#40830,#7335,.T.) ;
#51437=EDGE_CURVE('',#40836,#40837,#7336,.T.) ;
#51438=EDGE_CURVE('',#40837,#40838,#7337,.T.) ;
#51439=EDGE_CURVE('',#40838,#40839,#7338,.T.) ;
#51440=EDGE_CURVE('',#40839,#40836,#7339,.T.) ;
#51441=EDGE_CURVE('',#40840,#40841,#7340,.T.) ;
#51442=EDGE_CURVE('',#40841,#40842,#7341,.T.) ;
#51443=EDGE_CURVE('',#40842,#40843,#7342,.T.) ;
#51444=EDGE_CURVE('',#40843,#40840,#7343,.T.) ;
#51445=EDGE_CURVE('',#40844,#40845,#7344,.T.) ;
#51446=EDGE_CURVE('',#40845,#40846,#33066,.T.) ;
#51447=EDGE_CURVE('',#40846,#40847,#7345,.T.) ;
#51448=EDGE_CURVE('',#40847,#40844,#33067,.T.) ;
#51449=EDGE_CURVE('',#40848,#40849,#7346,.T.) ;
#51450=EDGE_CURVE('',#40849,#40850,#33068,.T.) ;
#51451=EDGE_CURVE('',#40850,#40851,#7347,.T.) ;
#51452=EDGE_CURVE('',#40851,#40852,#7348,.T.) ;
#51453=EDGE_CURVE('',#40852,#40853,#7349,.T.) ;
#51454=EDGE_CURVE('',#40853,#40848,#7350,.T.) ;
#51455=EDGE_CURVE('',#40854,#40855,#7351,.T.) ;
#51456=EDGE_CURVE('',#40855,#40856,#7352,.T.) ;
#51457=EDGE_CURVE('',#40856,#40857,#7353,.T.) ;
#51458=EDGE_CURVE('',#40857,#40854,#7354,.T.) ;
#51459=EDGE_CURVE('',#40858,#40859,#7355,.T.) ;
#51460=EDGE_CURVE('',#40859,#40860,#7356,.T.) ;
#51461=EDGE_CURVE('',#40860,#40861,#7357,.T.) ;
#51462=EDGE_CURVE('',#40861,#40858,#7358,.T.) ;
#51463=EDGE_CURVE('',#40862,#40863,#7359,.T.) ;
#51464=EDGE_CURVE('',#40863,#40864,#33069,.T.) ;
#51465=EDGE_CURVE('',#40864,#40865,#7360,.T.) ;
#51466=EDGE_CURVE('',#40865,#40862,#33070,.T.) ;
#51467=EDGE_CURVE('',#40866,#40867,#7361,.T.) ;
#51468=EDGE_CURVE('',#40867,#40868,#33071,.T.) ;
#51469=EDGE_CURVE('',#40868,#40869,#7362,.T.) ;
#51470=EDGE_CURVE('',#40869,#40870,#7363,.T.) ;
#51471=EDGE_CURVE('',#40870,#40871,#7364,.T.) ;
#51472=EDGE_CURVE('',#40871,#40866,#7365,.T.) ;
#51473=EDGE_CURVE('',#40872,#40873,#7366,.T.) ;
#51474=EDGE_CURVE('',#40873,#40874,#7367,.T.) ;
#51475=EDGE_CURVE('',#40874,#40875,#7368,.T.) ;
#51476=EDGE_CURVE('',#40875,#40872,#7369,.T.) ;
#51477=EDGE_CURVE('',#40876,#40877,#7370,.T.) ;
#51478=EDGE_CURVE('',#40877,#40878,#7371,.T.) ;
#51479=EDGE_CURVE('',#40878,#40879,#7372,.T.) ;
#51480=EDGE_CURVE('',#40879,#40876,#7373,.T.) ;
#51481=EDGE_CURVE('',#40880,#40881,#7374,.T.) ;
#51482=EDGE_CURVE('',#40881,#40882,#33072,.T.) ;
#51483=EDGE_CURVE('',#40882,#40883,#7375,.T.) ;
#51484=EDGE_CURVE('',#40883,#40880,#33073,.T.) ;
#51485=EDGE_CURVE('',#40884,#40885,#7376,.T.) ;
#51486=EDGE_CURVE('',#40885,#40886,#33074,.T.) ;
#51487=EDGE_CURVE('',#40886,#40887,#7377,.T.) ;
#51488=EDGE_CURVE('',#40887,#40888,#7378,.T.) ;
#51489=EDGE_CURVE('',#40888,#40889,#7379,.T.) ;
#51490=EDGE_CURVE('',#40889,#40884,#7380,.T.) ;
#51491=EDGE_CURVE('',#40890,#40891,#7381,.T.) ;
#51492=EDGE_CURVE('',#40891,#40892,#7382,.T.) ;
#51493=EDGE_CURVE('',#40892,#40893,#7383,.T.) ;
#51494=EDGE_CURVE('',#40893,#40890,#7384,.T.) ;
#51495=EDGE_CURVE('',#40894,#40895,#7385,.T.) ;
#51496=EDGE_CURVE('',#40895,#40896,#7386,.T.) ;
#51497=EDGE_CURVE('',#40896,#40897,#7387,.T.) ;
#51498=EDGE_CURVE('',#40897,#40894,#7388,.T.) ;
#51499=EDGE_CURVE('',#40898,#40899,#7389,.T.) ;
#51500=EDGE_CURVE('',#40899,#40900,#7390,.T.) ;
#51501=EDGE_CURVE('',#40900,#40901,#7391,.T.) ;
#51502=EDGE_CURVE('',#40901,#40898,#7392,.T.) ;
#51503=EDGE_CURVE('',#40902,#40903,#7393,.T.) ;
#51504=EDGE_CURVE('',#40903,#40904,#7394,.T.) ;
#51505=EDGE_CURVE('',#40904,#40905,#7395,.T.) ;
#51506=EDGE_CURVE('',#40905,#40902,#7396,.T.) ;
#51507=EDGE_CURVE('',#40906,#40907,#7397,.T.) ;
#51508=EDGE_CURVE('',#40907,#40908,#7398,.T.) ;
#51509=EDGE_CURVE('',#40908,#40909,#7399,.T.) ;
#51510=EDGE_CURVE('',#40909,#40906,#7400,.T.) ;
#51511=EDGE_CURVE('',#40910,#40911,#7401,.T.) ;
#51512=EDGE_CURVE('',#40911,#40912,#7402,.T.) ;
#51513=EDGE_CURVE('',#40912,#40913,#7403,.T.) ;
#51514=EDGE_CURVE('',#40913,#40910,#7404,.T.) ;
#51515=EDGE_CURVE('',#40914,#40915,#7405,.T.) ;
#51516=EDGE_CURVE('',#40915,#40916,#7406,.T.) ;
#51517=EDGE_CURVE('',#40916,#40917,#7407,.T.) ;
#51518=EDGE_CURVE('',#40917,#40914,#7408,.T.) ;
#51519=EDGE_CURVE('',#40918,#40919,#7409,.T.) ;
#51520=EDGE_CURVE('',#40919,#40920,#7410,.T.) ;
#51521=EDGE_CURVE('',#40920,#40921,#7411,.T.) ;
#51522=EDGE_CURVE('',#40921,#40918,#7412,.T.) ;
#51523=EDGE_CURVE('',#40922,#40923,#7413,.T.) ;
#51524=EDGE_CURVE('',#40923,#40924,#7414,.T.) ;
#51525=EDGE_CURVE('',#40924,#40925,#7415,.T.) ;
#51526=EDGE_CURVE('',#40925,#40922,#7416,.T.) ;
#51527=EDGE_CURVE('',#40926,#40927,#7417,.T.) ;
#51528=EDGE_CURVE('',#40927,#40928,#7418,.T.) ;
#51529=EDGE_CURVE('',#40928,#40929,#7419,.T.) ;
#51530=EDGE_CURVE('',#40929,#40926,#7420,.T.) ;
#51531=EDGE_CURVE('',#40930,#40931,#7421,.T.) ;
#51532=EDGE_CURVE('',#40931,#40932,#7422,.T.) ;
#51533=EDGE_CURVE('',#40932,#40933,#7423,.T.) ;
#51534=EDGE_CURVE('',#40933,#40930,#7424,.T.) ;
#51535=EDGE_CURVE('',#40934,#40935,#7425,.T.) ;
#51536=EDGE_CURVE('',#40935,#40936,#7426,.T.) ;
#51537=EDGE_CURVE('',#40936,#40937,#7427,.T.) ;
#51538=EDGE_CURVE('',#40937,#40934,#7428,.T.) ;
#51539=EDGE_CURVE('',#40938,#40939,#7429,.T.) ;
#51540=EDGE_CURVE('',#40939,#40940,#7430,.T.) ;
#51541=EDGE_CURVE('',#40940,#40941,#7431,.T.) ;
#51542=EDGE_CURVE('',#40941,#40938,#7432,.T.) ;
#51543=EDGE_CURVE('',#40942,#40943,#7433,.T.) ;
#51544=EDGE_CURVE('',#40943,#40944,#7434,.T.) ;
#51545=EDGE_CURVE('',#40944,#40945,#7435,.T.) ;
#51546=EDGE_CURVE('',#40945,#40942,#7436,.T.) ;
#51547=EDGE_CURVE('',#40946,#40947,#7437,.T.) ;
#51548=EDGE_CURVE('',#40947,#40948,#7438,.T.) ;
#51549=EDGE_CURVE('',#40948,#40949,#7439,.T.) ;
#51550=EDGE_CURVE('',#40949,#40946,#7440,.T.) ;
#51551=EDGE_CURVE('',#40950,#40951,#7441,.T.) ;
#51552=EDGE_CURVE('',#40951,#40952,#7442,.T.) ;
#51553=EDGE_CURVE('',#40952,#40953,#7443,.T.) ;
#51554=EDGE_CURVE('',#40953,#40950,#7444,.T.) ;
#51555=EDGE_CURVE('',#40954,#40955,#7445,.T.) ;
#51556=EDGE_CURVE('',#40955,#40956,#7446,.T.) ;
#51557=EDGE_CURVE('',#40956,#40957,#7447,.T.) ;
#51558=EDGE_CURVE('',#40957,#40954,#7448,.T.) ;
#51559=EDGE_CURVE('',#40958,#40959,#7449,.T.) ;
#51560=EDGE_CURVE('',#40959,#40960,#7450,.T.) ;
#51561=EDGE_CURVE('',#40960,#40961,#7451,.T.) ;
#51562=EDGE_CURVE('',#40961,#40958,#7452,.T.) ;
#51563=EDGE_CURVE('',#40962,#40963,#7453,.T.) ;
#51564=EDGE_CURVE('',#40963,#40964,#7454,.T.) ;
#51565=EDGE_CURVE('',#40964,#40965,#7455,.T.) ;
#51566=EDGE_CURVE('',#40965,#40962,#7456,.T.) ;
#51567=EDGE_CURVE('',#40966,#40967,#7457,.T.) ;
#51568=EDGE_CURVE('',#40967,#40968,#7458,.T.) ;
#51569=EDGE_CURVE('',#40968,#40969,#7459,.T.) ;
#51570=EDGE_CURVE('',#40969,#40966,#7460,.T.) ;
#51571=EDGE_CURVE('',#40970,#40971,#7461,.T.) ;
#51572=EDGE_CURVE('',#40971,#40972,#7462,.T.) ;
#51573=EDGE_CURVE('',#40972,#40973,#7463,.T.) ;
#51574=EDGE_CURVE('',#40973,#40970,#7464,.T.) ;
#51575=EDGE_CURVE('',#40974,#40975,#7465,.T.) ;
#51576=EDGE_CURVE('',#40975,#40976,#7466,.T.) ;
#51577=EDGE_CURVE('',#40976,#40977,#7467,.T.) ;
#51578=EDGE_CURVE('',#40977,#40974,#7468,.T.) ;
#51579=EDGE_CURVE('',#40978,#40979,#7469,.T.) ;
#51580=EDGE_CURVE('',#40979,#40980,#7470,.T.) ;
#51581=EDGE_CURVE('',#40980,#40981,#7471,.T.) ;
#51582=EDGE_CURVE('',#40981,#40978,#7472,.T.) ;
#51583=EDGE_CURVE('',#40982,#40983,#7473,.T.) ;
#51584=EDGE_CURVE('',#40983,#40984,#7474,.T.) ;
#51585=EDGE_CURVE('',#40984,#40985,#7475,.T.) ;
#51586=EDGE_CURVE('',#40985,#40982,#7476,.T.) ;
#51587=EDGE_CURVE('',#40986,#40987,#7477,.T.) ;
#51588=EDGE_CURVE('',#40987,#40988,#7478,.T.) ;
#51589=EDGE_CURVE('',#40988,#40989,#7479,.T.) ;
#51590=EDGE_CURVE('',#40989,#40986,#7480,.T.) ;
#51591=EDGE_CURVE('',#40990,#40991,#7481,.T.) ;
#51592=EDGE_CURVE('',#40991,#40992,#7482,.T.) ;
#51593=EDGE_CURVE('',#40992,#40993,#7483,.T.) ;
#51594=EDGE_CURVE('',#40993,#40990,#7484,.T.) ;
#51595=EDGE_CURVE('',#40994,#40995,#7485,.T.) ;
#51596=EDGE_CURVE('',#40995,#40996,#7486,.T.) ;
#51597=EDGE_CURVE('',#40996,#40997,#7487,.T.) ;
#51598=EDGE_CURVE('',#40997,#40994,#7488,.T.) ;
#51599=EDGE_CURVE('',#40998,#40999,#7489,.T.) ;
#51600=EDGE_CURVE('',#40999,#41000,#7490,.T.) ;
#51601=EDGE_CURVE('',#41000,#41001,#7491,.T.) ;
#51602=EDGE_CURVE('',#41001,#40998,#7492,.T.) ;
#51603=EDGE_CURVE('',#41002,#41003,#7493,.T.) ;
#51604=EDGE_CURVE('',#41003,#41004,#7494,.T.) ;
#51605=EDGE_CURVE('',#41004,#41005,#7495,.T.) ;
#51606=EDGE_CURVE('',#41005,#41002,#7496,.T.) ;
#51607=EDGE_CURVE('',#41006,#41007,#7497,.T.) ;
#51608=EDGE_CURVE('',#41007,#41008,#7498,.T.) ;
#51609=EDGE_CURVE('',#41008,#41009,#7499,.T.) ;
#51610=EDGE_CURVE('',#41009,#41006,#7500,.T.) ;
#51611=EDGE_CURVE('',#41010,#41011,#7501,.T.) ;
#51612=EDGE_CURVE('',#41011,#41012,#7502,.T.) ;
#51613=EDGE_CURVE('',#41012,#41013,#7503,.T.) ;
#51614=EDGE_CURVE('',#41013,#41010,#7504,.T.) ;
#51615=EDGE_CURVE('',#41014,#41015,#7505,.T.) ;
#51616=EDGE_CURVE('',#41015,#41016,#7506,.T.) ;
#51617=EDGE_CURVE('',#41016,#41017,#7507,.T.) ;
#51618=EDGE_CURVE('',#41017,#41014,#7508,.T.) ;
#51619=EDGE_CURVE('',#41018,#41019,#7509,.T.) ;
#51620=EDGE_CURVE('',#41019,#41020,#7510,.T.) ;
#51621=EDGE_CURVE('',#41020,#41021,#7511,.T.) ;
#51622=EDGE_CURVE('',#41021,#41018,#7512,.T.) ;
#51623=EDGE_CURVE('',#41022,#41023,#7513,.T.) ;
#51624=EDGE_CURVE('',#41023,#41024,#7514,.T.) ;
#51625=EDGE_CURVE('',#41024,#41025,#7515,.T.) ;
#51626=EDGE_CURVE('',#41025,#41022,#7516,.T.) ;
#51627=EDGE_CURVE('',#41026,#41027,#7517,.T.) ;
#51628=EDGE_CURVE('',#41027,#41028,#7518,.T.) ;
#51629=EDGE_CURVE('',#41028,#41029,#7519,.T.) ;
#51630=EDGE_CURVE('',#41029,#41026,#7520,.T.) ;
#51631=EDGE_CURVE('',#41030,#41031,#7521,.T.) ;
#51632=EDGE_CURVE('',#41031,#41032,#7522,.T.) ;
#51633=EDGE_CURVE('',#41032,#41033,#7523,.T.) ;
#51634=EDGE_CURVE('',#41033,#41030,#7524,.T.) ;
#51635=EDGE_CURVE('',#41034,#41035,#7525,.T.) ;
#51636=EDGE_CURVE('',#41035,#41036,#7526,.T.) ;
#51637=EDGE_CURVE('',#41036,#41037,#7527,.T.) ;
#51638=EDGE_CURVE('',#41037,#41034,#7528,.T.) ;
#51639=EDGE_CURVE('',#41038,#41039,#7529,.T.) ;
#51640=EDGE_CURVE('',#41038,#41040,#33075,.T.) ;
#51641=EDGE_CURVE('',#41041,#41040,#7530,.T.) ;
#51642=EDGE_CURVE('',#41041,#41042,#33076,.T.) ;
#51643=EDGE_CURVE('',#41043,#41042,#7531,.T.) ;
#51644=EDGE_CURVE('',#41043,#41044,#33077,.T.) ;
#51645=EDGE_CURVE('',#41045,#41044,#7532,.T.) ;
#51646=EDGE_CURVE('',#41045,#41039,#33078,.T.) ;
#51647=EDGE_CURVE('',#41046,#41047,#7533,.T.) ;
#51648=EDGE_CURVE('',#41047,#41045,#7534,.T.) ;
#51649=EDGE_CURVE('',#41044,#41046,#7535,.T.) ;
#51650=EDGE_CURVE('',#41048,#41049,#7536,.T.) ;
#51651=EDGE_CURVE('',#41049,#41038,#7537,.T.) ;
#51652=EDGE_CURVE('',#41039,#41048,#7538,.T.) ;
#51653=EDGE_CURVE('',#41040,#41050,#7539,.T.) ;
#51654=EDGE_CURVE('',#41050,#41051,#7540,.T.) ;
#51655=EDGE_CURVE('',#41051,#41041,#7541,.T.) ;
#51656=EDGE_CURVE('',#41052,#41053,#7542,.T.) ;
#51657=EDGE_CURVE('',#41053,#41043,#7543,.T.) ;
#51658=EDGE_CURVE('',#41042,#41052,#7544,.T.) ;
#51659=EDGE_CURVE('',#41054,#41055,#7545,.T.) ;
#51660=EDGE_CURVE('',#41055,#41056,#7546,.T.) ;
#51661=EDGE_CURVE('',#41056,#41057,#7547,.T.) ;
#51662=EDGE_CURVE('',#41057,#41054,#7548,.T.) ;
#51663=EDGE_CURVE('',#41058,#41059,#7549,.T.) ;
#51664=EDGE_CURVE('',#41058,#41060,#33079,.T.) ;
#51665=EDGE_CURVE('',#41061,#41060,#7550,.T.) ;
#51666=EDGE_CURVE('',#41061,#41062,#33080,.T.) ;
#51667=EDGE_CURVE('',#41063,#41062,#7551,.T.) ;
#51668=EDGE_CURVE('',#41063,#41064,#33081,.T.) ;
#51669=EDGE_CURVE('',#41065,#41064,#7552,.T.) ;
#51670=EDGE_CURVE('',#41065,#41059,#33082,.T.) ;
#51671=EDGE_CURVE('',#41066,#41067,#7553,.T.) ;
#51672=EDGE_CURVE('',#41067,#41065,#7554,.T.) ;
#51673=EDGE_CURVE('',#41064,#41066,#7555,.T.) ;
#51674=EDGE_CURVE('',#41068,#41069,#7556,.T.) ;
#51675=EDGE_CURVE('',#41069,#41058,#7557,.T.) ;
#51676=EDGE_CURVE('',#41059,#41068,#7558,.T.) ;
#51677=EDGE_CURVE('',#41060,#41070,#7559,.T.) ;
#51678=EDGE_CURVE('',#41070,#41071,#7560,.T.) ;
#51679=EDGE_CURVE('',#41071,#41061,#7561,.T.) ;
#51680=EDGE_CURVE('',#41072,#41073,#7562,.T.) ;
#51681=EDGE_CURVE('',#41073,#41063,#7563,.T.) ;
#51682=EDGE_CURVE('',#41062,#41072,#7564,.T.) ;
#51683=EDGE_CURVE('',#41074,#41075,#7565,.T.) ;
#51684=EDGE_CURVE('',#41075,#41076,#7566,.T.) ;
#51685=EDGE_CURVE('',#41076,#41077,#7567,.T.) ;
#51686=EDGE_CURVE('',#41077,#41074,#7568,.T.) ;
#51687=EDGE_CURVE('',#41078,#41079,#7569,.T.) ;
#51688=EDGE_CURVE('',#41078,#41080,#33083,.T.) ;
#51689=EDGE_CURVE('',#41081,#41080,#7570,.T.) ;
#51690=EDGE_CURVE('',#41081,#41082,#33084,.T.) ;
#51691=EDGE_CURVE('',#41083,#41082,#7571,.T.) ;
#51692=EDGE_CURVE('',#41083,#41084,#33085,.T.) ;
#51693=EDGE_CURVE('',#41085,#41084,#7572,.T.) ;
#51694=EDGE_CURVE('',#41085,#41079,#33086,.T.) ;
#51695=EDGE_CURVE('',#41086,#41087,#7573,.T.) ;
#51696=EDGE_CURVE('',#41087,#41085,#7574,.T.) ;
#51697=EDGE_CURVE('',#41084,#41086,#7575,.T.) ;
#51698=EDGE_CURVE('',#41088,#41089,#7576,.T.) ;
#51699=EDGE_CURVE('',#41089,#41078,#7577,.T.) ;
#51700=EDGE_CURVE('',#41079,#41088,#7578,.T.) ;
#51701=EDGE_CURVE('',#41080,#41090,#7579,.T.) ;
#51702=EDGE_CURVE('',#41090,#41091,#7580,.T.) ;
#51703=EDGE_CURVE('',#41091,#41081,#7581,.T.) ;
#51704=EDGE_CURVE('',#41092,#41093,#7582,.T.) ;
#51705=EDGE_CURVE('',#41093,#41083,#7583,.T.) ;
#51706=EDGE_CURVE('',#41082,#41092,#7584,.T.) ;
#51707=EDGE_CURVE('',#41094,#41095,#7585,.T.) ;
#51708=EDGE_CURVE('',#41095,#41096,#7586,.T.) ;
#51709=EDGE_CURVE('',#41096,#41097,#7587,.T.) ;
#51710=EDGE_CURVE('',#41097,#41094,#7588,.T.) ;
#51711=EDGE_CURVE('',#41098,#41099,#7589,.T.) ;
#51712=EDGE_CURVE('',#41098,#41100,#33087,.T.) ;
#51713=EDGE_CURVE('',#41101,#41100,#7590,.T.) ;
#51714=EDGE_CURVE('',#41101,#41102,#33088,.T.) ;
#51715=EDGE_CURVE('',#41103,#41102,#7591,.T.) ;
#51716=EDGE_CURVE('',#41103,#41104,#33089,.T.) ;
#51717=EDGE_CURVE('',#41105,#41104,#7592,.T.) ;
#51718=EDGE_CURVE('',#41105,#41099,#33090,.T.) ;
#51719=EDGE_CURVE('',#41106,#41107,#7593,.T.) ;
#51720=EDGE_CURVE('',#41107,#41105,#7594,.T.) ;
#51721=EDGE_CURVE('',#41104,#41106,#7595,.T.) ;
#51722=EDGE_CURVE('',#41108,#41109,#7596,.T.) ;
#51723=EDGE_CURVE('',#41109,#41098,#7597,.T.) ;
#51724=EDGE_CURVE('',#41099,#41108,#7598,.T.) ;
#51725=EDGE_CURVE('',#41100,#41110,#7599,.T.) ;
#51726=EDGE_CURVE('',#41110,#41111,#7600,.T.) ;
#51727=EDGE_CURVE('',#41111,#41101,#7601,.T.) ;
#51728=EDGE_CURVE('',#41112,#41113,#7602,.T.) ;
#51729=EDGE_CURVE('',#41113,#41103,#7603,.T.) ;
#51730=EDGE_CURVE('',#41102,#41112,#7604,.T.) ;
#51731=EDGE_CURVE('',#41114,#41115,#7605,.T.) ;
#51732=EDGE_CURVE('',#41115,#41116,#7606,.T.) ;
#51733=EDGE_CURVE('',#41116,#41117,#7607,.T.) ;
#51734=EDGE_CURVE('',#41117,#41114,#7608,.T.) ;
#51735=EDGE_CURVE('',#41118,#41119,#7609,.T.) ;
#51736=EDGE_CURVE('',#41118,#41120,#33091,.T.) ;
#51737=EDGE_CURVE('',#41121,#41120,#7610,.T.) ;
#51738=EDGE_CURVE('',#41121,#41122,#33092,.T.) ;
#51739=EDGE_CURVE('',#41123,#41122,#7611,.T.) ;
#51740=EDGE_CURVE('',#41123,#41124,#33093,.T.) ;
#51741=EDGE_CURVE('',#41125,#41124,#7612,.T.) ;
#51742=EDGE_CURVE('',#41125,#41119,#33094,.T.) ;
#51743=EDGE_CURVE('',#41126,#41127,#7613,.T.) ;
#51744=EDGE_CURVE('',#41127,#41125,#7614,.T.) ;
#51745=EDGE_CURVE('',#41124,#41126,#7615,.T.) ;
#51746=EDGE_CURVE('',#41128,#41129,#7616,.T.) ;
#51747=EDGE_CURVE('',#41129,#41118,#7617,.T.) ;
#51748=EDGE_CURVE('',#41119,#41128,#7618,.T.) ;
#51749=EDGE_CURVE('',#41120,#41130,#7619,.T.) ;
#51750=EDGE_CURVE('',#41130,#41131,#7620,.T.) ;
#51751=EDGE_CURVE('',#41131,#41121,#7621,.T.) ;
#51752=EDGE_CURVE('',#41132,#41133,#7622,.T.) ;
#51753=EDGE_CURVE('',#41133,#41123,#7623,.T.) ;
#51754=EDGE_CURVE('',#41122,#41132,#7624,.T.) ;
#51755=EDGE_CURVE('',#41134,#41135,#7625,.T.) ;
#51756=EDGE_CURVE('',#41135,#41136,#7626,.T.) ;
#51757=EDGE_CURVE('',#41136,#41137,#7627,.T.) ;
#51758=EDGE_CURVE('',#41137,#41134,#7628,.T.) ;
#51759=EDGE_CURVE('',#41138,#41139,#7629,.T.) ;
#51760=EDGE_CURVE('',#41138,#41140,#33095,.T.) ;
#51761=EDGE_CURVE('',#41141,#41140,#7630,.T.) ;
#51762=EDGE_CURVE('',#41141,#41142,#33096,.T.) ;
#51763=EDGE_CURVE('',#41143,#41142,#7631,.T.) ;
#51764=EDGE_CURVE('',#41143,#41144,#33097,.T.) ;
#51765=EDGE_CURVE('',#41145,#41144,#7632,.T.) ;
#51766=EDGE_CURVE('',#41145,#41139,#33098,.T.) ;
#51767=EDGE_CURVE('',#41146,#41147,#7633,.T.) ;
#51768=EDGE_CURVE('',#41147,#41145,#7634,.T.) ;
#51769=EDGE_CURVE('',#41144,#41146,#7635,.T.) ;
#51770=EDGE_CURVE('',#41148,#41149,#7636,.T.) ;
#51771=EDGE_CURVE('',#41149,#41138,#7637,.T.) ;
#51772=EDGE_CURVE('',#41139,#41148,#7638,.T.) ;
#51773=EDGE_CURVE('',#41140,#41150,#7639,.T.) ;
#51774=EDGE_CURVE('',#41150,#41151,#7640,.T.) ;
#51775=EDGE_CURVE('',#41151,#41141,#7641,.T.) ;
#51776=EDGE_CURVE('',#41152,#41153,#7642,.T.) ;
#51777=EDGE_CURVE('',#41153,#41143,#7643,.T.) ;
#51778=EDGE_CURVE('',#41142,#41152,#7644,.T.) ;
#51779=EDGE_CURVE('',#41154,#41155,#7645,.T.) ;
#51780=EDGE_CURVE('',#41155,#41156,#7646,.T.) ;
#51781=EDGE_CURVE('',#41156,#41157,#7647,.T.) ;
#51782=EDGE_CURVE('',#41157,#41154,#7648,.T.) ;
#51783=EDGE_CURVE('',#41158,#41159,#7649,.T.) ;
#51784=EDGE_CURVE('',#41158,#41160,#33099,.T.) ;
#51785=EDGE_CURVE('',#41161,#41160,#7650,.T.) ;
#51786=EDGE_CURVE('',#41161,#41162,#33100,.T.) ;
#51787=EDGE_CURVE('',#41163,#41162,#7651,.T.) ;
#51788=EDGE_CURVE('',#41163,#41164,#33101,.T.) ;
#51789=EDGE_CURVE('',#41165,#41164,#7652,.T.) ;
#51790=EDGE_CURVE('',#41165,#41159,#33102,.T.) ;
#51791=EDGE_CURVE('',#41166,#41167,#7653,.T.) ;
#51792=EDGE_CURVE('',#41167,#41165,#7654,.T.) ;
#51793=EDGE_CURVE('',#41164,#41166,#7655,.T.) ;
#51794=EDGE_CURVE('',#41168,#41169,#7656,.T.) ;
#51795=EDGE_CURVE('',#41169,#41158,#7657,.T.) ;
#51796=EDGE_CURVE('',#41159,#41168,#7658,.T.) ;
#51797=EDGE_CURVE('',#41160,#41170,#7659,.T.) ;
#51798=EDGE_CURVE('',#41170,#41171,#7660,.T.) ;
#51799=EDGE_CURVE('',#41171,#41161,#7661,.T.) ;
#51800=EDGE_CURVE('',#41172,#41173,#7662,.T.) ;
#51801=EDGE_CURVE('',#41173,#41163,#7663,.T.) ;
#51802=EDGE_CURVE('',#41162,#41172,#7664,.T.) ;
#51803=EDGE_CURVE('',#41174,#41175,#7665,.T.) ;
#51804=EDGE_CURVE('',#41175,#41176,#7666,.T.) ;
#51805=EDGE_CURVE('',#41176,#41177,#7667,.T.) ;
#51806=EDGE_CURVE('',#41177,#41174,#7668,.T.) ;
#51807=EDGE_CURVE('',#41178,#41179,#7669,.T.) ;
#51808=EDGE_CURVE('',#41178,#41180,#33103,.T.) ;
#51809=EDGE_CURVE('',#41181,#41180,#7670,.T.) ;
#51810=EDGE_CURVE('',#41181,#41182,#33104,.T.) ;
#51811=EDGE_CURVE('',#41183,#41182,#7671,.T.) ;
#51812=EDGE_CURVE('',#41183,#41184,#33105,.T.) ;
#51813=EDGE_CURVE('',#41185,#41184,#7672,.T.) ;
#51814=EDGE_CURVE('',#41185,#41179,#33106,.T.) ;
#51815=EDGE_CURVE('',#41186,#41187,#7673,.T.) ;
#51816=EDGE_CURVE('',#41187,#41185,#7674,.T.) ;
#51817=EDGE_CURVE('',#41184,#41186,#7675,.T.) ;
#51818=EDGE_CURVE('',#41188,#41189,#7676,.T.) ;
#51819=EDGE_CURVE('',#41189,#41178,#7677,.T.) ;
#51820=EDGE_CURVE('',#41179,#41188,#7678,.T.) ;
#51821=EDGE_CURVE('',#41180,#41190,#7679,.T.) ;
#51822=EDGE_CURVE('',#41190,#41191,#7680,.T.) ;
#51823=EDGE_CURVE('',#41191,#41181,#7681,.T.) ;
#51824=EDGE_CURVE('',#41192,#41193,#7682,.T.) ;
#51825=EDGE_CURVE('',#41193,#41183,#7683,.T.) ;
#51826=EDGE_CURVE('',#41182,#41192,#7684,.T.) ;
#51827=EDGE_CURVE('',#41194,#41195,#7685,.T.) ;
#51828=EDGE_CURVE('',#41195,#41196,#7686,.T.) ;
#51829=EDGE_CURVE('',#41196,#41197,#7687,.T.) ;
#51830=EDGE_CURVE('',#41197,#41194,#7688,.T.) ;
#51831=EDGE_CURVE('',#41198,#41199,#7689,.T.) ;
#51832=EDGE_CURVE('',#41198,#41200,#33107,.T.) ;
#51833=EDGE_CURVE('',#41201,#41200,#7690,.T.) ;
#51834=EDGE_CURVE('',#41201,#41202,#33108,.T.) ;
#51835=EDGE_CURVE('',#41203,#41202,#7691,.T.) ;
#51836=EDGE_CURVE('',#41203,#41204,#33109,.T.) ;
#51837=EDGE_CURVE('',#41205,#41204,#7692,.T.) ;
#51838=EDGE_CURVE('',#41205,#41199,#33110,.T.) ;
#51839=EDGE_CURVE('',#41206,#41207,#7693,.T.) ;
#51840=EDGE_CURVE('',#41207,#41205,#7694,.T.) ;
#51841=EDGE_CURVE('',#41204,#41206,#7695,.T.) ;
#51842=EDGE_CURVE('',#41208,#41209,#7696,.T.) ;
#51843=EDGE_CURVE('',#41209,#41198,#7697,.T.) ;
#51844=EDGE_CURVE('',#41199,#41208,#7698,.T.) ;
#51845=EDGE_CURVE('',#41200,#41210,#7699,.T.) ;
#51846=EDGE_CURVE('',#41210,#41211,#7700,.T.) ;
#51847=EDGE_CURVE('',#41211,#41201,#7701,.T.) ;
#51848=EDGE_CURVE('',#41212,#41213,#7702,.T.) ;
#51849=EDGE_CURVE('',#41213,#41203,#7703,.T.) ;
#51850=EDGE_CURVE('',#41202,#41212,#7704,.T.) ;
#51851=EDGE_CURVE('',#41214,#41215,#7705,.T.) ;
#51852=EDGE_CURVE('',#41215,#41216,#7706,.T.) ;
#51853=EDGE_CURVE('',#41216,#41217,#7707,.T.) ;
#51854=EDGE_CURVE('',#41217,#41214,#7708,.T.) ;
#51855=EDGE_CURVE('',#41218,#41219,#7709,.T.) ;
#51856=EDGE_CURVE('',#41219,#41220,#7710,.T.) ;
#51857=EDGE_CURVE('',#41220,#41221,#7711,.T.) ;
#51858=EDGE_CURVE('',#41221,#41218,#7712,.T.) ;
#51859=EDGE_CURVE('',#41222,#41223,#7713,.T.) ;
#51860=EDGE_CURVE('',#41223,#41224,#7714,.T.) ;
#51861=EDGE_CURVE('',#41224,#41225,#7715,.T.) ;
#51862=EDGE_CURVE('',#41225,#41222,#7716,.T.) ;
#51863=EDGE_CURVE('',#41226,#41227,#7717,.T.) ;
#51864=EDGE_CURVE('',#41227,#41228,#7718,.T.) ;
#51865=EDGE_CURVE('',#41228,#41229,#7719,.T.) ;
#51866=EDGE_CURVE('',#41229,#41226,#7720,.T.) ;
#51867=EDGE_CURVE('',#41230,#41231,#7721,.T.) ;
#51868=EDGE_CURVE('',#41231,#41232,#7722,.T.) ;
#51869=EDGE_CURVE('',#41232,#41233,#7723,.T.) ;
#51870=EDGE_CURVE('',#41233,#41230,#7724,.T.) ;
#51871=EDGE_CURVE('',#41234,#41235,#7725,.T.) ;
#51872=EDGE_CURVE('',#41235,#41236,#7726,.T.) ;
#51873=EDGE_CURVE('',#41236,#41237,#7727,.T.) ;
#51874=EDGE_CURVE('',#41237,#41234,#7728,.T.) ;
#51875=EDGE_CURVE('',#41238,#41239,#7729,.T.) ;
#51876=EDGE_CURVE('',#41239,#41240,#7730,.T.) ;
#51877=EDGE_CURVE('',#41240,#41241,#7731,.T.) ;
#51878=EDGE_CURVE('',#41241,#41238,#7732,.T.) ;
#51879=EDGE_CURVE('',#41242,#41243,#7733,.T.) ;
#51880=EDGE_CURVE('',#41243,#41244,#7734,.T.) ;
#51881=EDGE_CURVE('',#41244,#41245,#7735,.T.) ;
#51882=EDGE_CURVE('',#41245,#41242,#7736,.T.) ;
#51883=EDGE_CURVE('',#41246,#41247,#7737,.T.) ;
#51884=EDGE_CURVE('',#41247,#41248,#7738,.T.) ;
#51885=EDGE_CURVE('',#41248,#41249,#7739,.T.) ;
#51886=EDGE_CURVE('',#41249,#41246,#7740,.T.) ;
#51887=EDGE_CURVE('',#39027,#39011,#7741,.T.) ;
#51888=EDGE_CURVE('',#39010,#38994,#7742,.T.) ;
#51889=EDGE_CURVE('',#38993,#38977,#7743,.T.) ;
#51890=EDGE_CURVE('',#38976,#38960,#7744,.T.) ;
#51891=EDGE_CURVE('',#38959,#38943,#7745,.T.) ;
#51892=EDGE_CURVE('',#38942,#38926,#7746,.T.) ;
#51893=EDGE_CURVE('',#38925,#38909,#7747,.T.) ;
#51894=EDGE_CURVE('',#38908,#38892,#7748,.T.) ;
#51895=EDGE_CURVE('',#38891,#38875,#7749,.T.) ;
#51896=EDGE_CURVE('',#38877,#38890,#7750,.T.) ;
#51897=EDGE_CURVE('',#38889,#38878,#7751,.T.) ;
#51898=EDGE_CURVE('',#38881,#38886,#7752,.T.) ;
#51899=EDGE_CURVE('',#38885,#38882,#7753,.T.) ;
#51900=EDGE_CURVE('',#38879,#38888,#7754,.T.) ;
#51901=EDGE_CURVE('',#38887,#38880,#7755,.T.) ;
#51902=EDGE_CURVE('',#38894,#38907,#7756,.T.) ;
#51903=EDGE_CURVE('',#38906,#38895,#7757,.T.) ;
#51904=EDGE_CURVE('',#38898,#38903,#7758,.T.) ;
#51905=EDGE_CURVE('',#38902,#38899,#7759,.T.) ;
#51906=EDGE_CURVE('',#38896,#38905,#7760,.T.) ;
#51907=EDGE_CURVE('',#38904,#38897,#7761,.T.) ;
#51908=EDGE_CURVE('',#38911,#38924,#7762,.T.) ;
#51909=EDGE_CURVE('',#38923,#38912,#7763,.T.) ;
#51910=EDGE_CURVE('',#38915,#38920,#7764,.T.) ;
#51911=EDGE_CURVE('',#38919,#38916,#7765,.T.) ;
#51912=EDGE_CURVE('',#38913,#38922,#7766,.T.) ;
#51913=EDGE_CURVE('',#38921,#38914,#7767,.T.) ;
#51914=EDGE_CURVE('',#38928,#38941,#7768,.T.) ;
#51915=EDGE_CURVE('',#38940,#38929,#7769,.T.) ;
#51916=EDGE_CURVE('',#38932,#38937,#7770,.T.) ;
#51917=EDGE_CURVE('',#38936,#38933,#7771,.T.) ;
#51918=EDGE_CURVE('',#38930,#38939,#7772,.T.) ;
#51919=EDGE_CURVE('',#38938,#38931,#7773,.T.) ;
#51920=EDGE_CURVE('',#38945,#38958,#7774,.T.) ;
#51921=EDGE_CURVE('',#38957,#38946,#7775,.T.) ;
#51922=EDGE_CURVE('',#38949,#38954,#7776,.T.) ;
#51923=EDGE_CURVE('',#38953,#38950,#7777,.T.) ;
#51924=EDGE_CURVE('',#38947,#38956,#7778,.T.) ;
#51925=EDGE_CURVE('',#38955,#38948,#7779,.T.) ;
#51926=EDGE_CURVE('',#38962,#38975,#7780,.T.) ;
#51927=EDGE_CURVE('',#38974,#38963,#7781,.T.) ;
#51928=EDGE_CURVE('',#38966,#38971,#7782,.T.) ;
#51929=EDGE_CURVE('',#38970,#38967,#7783,.T.) ;
#51930=EDGE_CURVE('',#38964,#38973,#7784,.T.) ;
#51931=EDGE_CURVE('',#38972,#38965,#7785,.T.) ;
#51932=EDGE_CURVE('',#38979,#38992,#7786,.T.) ;
#51933=EDGE_CURVE('',#38991,#38980,#7787,.T.) ;
#51934=EDGE_CURVE('',#38983,#38988,#7788,.T.) ;
#51935=EDGE_CURVE('',#38987,#38984,#7789,.T.) ;
#51936=EDGE_CURVE('',#38981,#38990,#7790,.T.) ;
#51937=EDGE_CURVE('',#38989,#38982,#7791,.T.) ;
#51938=EDGE_CURVE('',#38996,#39009,#7792,.T.) ;
#51939=EDGE_CURVE('',#39008,#38997,#7793,.T.) ;
#51940=EDGE_CURVE('',#39000,#39005,#7794,.T.) ;
#51941=EDGE_CURVE('',#39004,#39001,#7795,.T.) ;
#51942=EDGE_CURVE('',#38998,#39007,#7796,.T.) ;
#51943=EDGE_CURVE('',#39006,#38999,#7797,.T.) ;
#51944=EDGE_CURVE('',#39013,#39026,#7798,.T.) ;
#51945=EDGE_CURVE('',#39025,#39014,#7799,.T.) ;
#51946=EDGE_CURVE('',#39017,#39022,#7800,.T.) ;
#51947=EDGE_CURVE('',#39021,#39018,#7801,.T.) ;
#51948=EDGE_CURVE('',#39015,#39024,#7802,.T.) ;
#51949=EDGE_CURVE('',#39023,#39016,#7803,.T.) ;
#51950=EDGE_CURVE('',#41250,#41251,#7804,.T.) ;
#51951=EDGE_CURVE('',#41251,#41252,#33111,.T.) ;
#51952=EDGE_CURVE('',#41253,#41252,#7805,.T.) ;
#51953=EDGE_CURVE('',#41253,#41250,#33112,.T.) ;
#51954=EDGE_CURVE('',#41252,#41254,#7806,.T.) ;
#51955=EDGE_CURVE('',#41255,#41254,#7807,.T.) ;
#51956=EDGE_CURVE('',#41255,#41253,#7808,.T.) ;
#51957=EDGE_CURVE('',#41254,#41256,#33113,.T.) ;
#51958=EDGE_CURVE('',#41257,#41256,#7809,.T.) ;
#51959=EDGE_CURVE('',#41257,#41255,#33114,.T.) ;
#51960=EDGE_CURVE('',#41256,#41258,#7810,.T.) ;
#51961=EDGE_CURVE('',#41259,#41258,#7811,.T.) ;
#51962=EDGE_CURVE('',#41259,#41257,#7812,.T.) ;
#51963=EDGE_CURVE('',#41258,#41260,#33115,.T.) ;
#51964=EDGE_CURVE('',#41261,#41260,#7813,.T.) ;
#51965=EDGE_CURVE('',#41261,#41259,#33116,.T.) ;
#51966=EDGE_CURVE('',#41260,#41262,#7814,.T.) ;
#51967=EDGE_CURVE('',#41263,#41262,#7815,.T.) ;
#51968=EDGE_CURVE('',#41263,#41261,#7816,.T.) ;
#51969=EDGE_CURVE('',#41262,#41264,#33117,.T.) ;
#51970=EDGE_CURVE('',#41265,#41264,#7817,.T.) ;
#51971=EDGE_CURVE('',#41265,#41263,#33118,.T.) ;
#51972=EDGE_CURVE('',#41250,#41265,#7818,.T.) ;
#51973=EDGE_CURVE('',#41264,#41251,#7819,.T.) ;
#51974=EDGE_CURVE('',#41266,#41267,#7820,.T.) ;
#51975=EDGE_CURVE('',#41267,#41268,#7821,.T.) ;
#51976=EDGE_CURVE('',#41268,#41269,#7822,.T.) ;
#51977=EDGE_CURVE('',#41269,#41266,#7823,.T.) ;
#51978=EDGE_CURVE('',#41270,#41271,#7824,.T.) ;
#51979=EDGE_CURVE('',#41271,#41272,#33119,.T.) ;
#51980=EDGE_CURVE('',#41273,#41272,#7825,.T.) ;
#51981=EDGE_CURVE('',#41273,#41270,#33120,.T.) ;
#51982=EDGE_CURVE('',#41272,#41274,#7826,.T.) ;
#51983=EDGE_CURVE('',#41275,#41274,#7827,.T.) ;
#51984=EDGE_CURVE('',#41275,#41273,#7828,.T.) ;
#51985=EDGE_CURVE('',#41274,#41276,#33121,.T.) ;
#51986=EDGE_CURVE('',#41277,#41276,#7829,.T.) ;
#51987=EDGE_CURVE('',#41277,#41275,#33122,.T.) ;
#51988=EDGE_CURVE('',#41276,#41278,#7830,.T.) ;
#51989=EDGE_CURVE('',#41279,#41278,#7831,.T.) ;
#51990=EDGE_CURVE('',#41279,#41277,#7832,.T.) ;
#51991=EDGE_CURVE('',#41278,#41280,#33123,.T.) ;
#51992=EDGE_CURVE('',#41281,#41280,#7833,.T.) ;
#51993=EDGE_CURVE('',#41281,#41279,#33124,.T.) ;
#51994=EDGE_CURVE('',#41280,#41282,#7834,.T.) ;
#51995=EDGE_CURVE('',#41283,#41282,#7835,.T.) ;
#51996=EDGE_CURVE('',#41283,#41281,#7836,.T.) ;
#51997=EDGE_CURVE('',#41282,#41284,#33125,.T.) ;
#51998=EDGE_CURVE('',#41285,#41284,#7837,.T.) ;
#51999=EDGE_CURVE('',#41285,#41283,#33126,.T.) ;
#52000=EDGE_CURVE('',#41270,#41285,#7838,.T.) ;
#52001=EDGE_CURVE('',#41284,#41271,#7839,.T.) ;
#52002=EDGE_CURVE('',#41286,#41287,#7840,.T.) ;
#52003=EDGE_CURVE('',#41287,#41288,#7841,.T.) ;
#52004=EDGE_CURVE('',#41288,#41289,#7842,.T.) ;
#52005=EDGE_CURVE('',#41289,#41286,#7843,.T.) ;
#52006=EDGE_CURVE('',#41290,#41291,#7844,.T.) ;
#52007=EDGE_CURVE('',#41291,#41292,#33127,.T.) ;
#52008=EDGE_CURVE('',#41293,#41292,#7845,.T.) ;
#52009=EDGE_CURVE('',#41293,#41290,#33128,.T.) ;
#52010=EDGE_CURVE('',#41292,#41294,#7846,.T.) ;
#52011=EDGE_CURVE('',#41295,#41294,#7847,.T.) ;
#52012=EDGE_CURVE('',#41295,#41293,#7848,.T.) ;
#52013=EDGE_CURVE('',#41294,#41296,#33129,.T.) ;
#52014=EDGE_CURVE('',#41297,#41296,#7849,.T.) ;
#52015=EDGE_CURVE('',#41297,#41295,#33130,.T.) ;
#52016=EDGE_CURVE('',#41296,#41298,#7850,.T.) ;
#52017=EDGE_CURVE('',#41299,#41298,#7851,.T.) ;
#52018=EDGE_CURVE('',#41299,#41297,#7852,.T.) ;
#52019=EDGE_CURVE('',#41298,#41300,#33131,.T.) ;
#52020=EDGE_CURVE('',#41301,#41300,#7853,.T.) ;
#52021=EDGE_CURVE('',#41301,#41299,#33132,.T.) ;
#52022=EDGE_CURVE('',#41300,#41302,#7854,.T.) ;
#52023=EDGE_CURVE('',#41303,#41302,#7855,.T.) ;
#52024=EDGE_CURVE('',#41303,#41301,#7856,.T.) ;
#52025=EDGE_CURVE('',#41302,#41304,#33133,.T.) ;
#52026=EDGE_CURVE('',#41305,#41304,#7857,.T.) ;
#52027=EDGE_CURVE('',#41305,#41303,#33134,.T.) ;
#52028=EDGE_CURVE('',#41290,#41305,#7858,.T.) ;
#52029=EDGE_CURVE('',#41304,#41291,#7859,.T.) ;
#52030=EDGE_CURVE('',#41306,#41307,#7860,.T.) ;
#52031=EDGE_CURVE('',#41307,#41308,#7861,.T.) ;
#52032=EDGE_CURVE('',#41308,#41309,#7862,.T.) ;
#52033=EDGE_CURVE('',#41309,#41306,#7863,.T.) ;
#52034=EDGE_CURVE('',#41310,#41311,#7864,.T.) ;
#52035=EDGE_CURVE('',#41311,#41312,#33135,.T.) ;
#52036=EDGE_CURVE('',#41313,#41312,#7865,.T.) ;
#52037=EDGE_CURVE('',#41313,#41310,#33136,.T.) ;
#52038=EDGE_CURVE('',#41312,#41314,#7866,.T.) ;
#52039=EDGE_CURVE('',#41315,#41314,#7867,.T.) ;
#52040=EDGE_CURVE('',#41315,#41313,#7868,.T.) ;
#52041=EDGE_CURVE('',#41314,#41316,#33137,.T.) ;
#52042=EDGE_CURVE('',#41317,#41316,#7869,.T.) ;
#52043=EDGE_CURVE('',#41317,#41315,#33138,.T.) ;
#52044=EDGE_CURVE('',#41316,#41318,#7870,.T.) ;
#52045=EDGE_CURVE('',#41319,#41318,#7871,.T.) ;
#52046=EDGE_CURVE('',#41319,#41317,#7872,.T.) ;
#52047=EDGE_CURVE('',#41318,#41320,#33139,.T.) ;
#52048=EDGE_CURVE('',#41321,#41320,#7873,.T.) ;
#52049=EDGE_CURVE('',#41321,#41319,#33140,.T.) ;
#52050=EDGE_CURVE('',#41320,#41322,#7874,.T.) ;
#52051=EDGE_CURVE('',#41323,#41322,#7875,.T.) ;
#52052=EDGE_CURVE('',#41323,#41321,#7876,.T.) ;
#52053=EDGE_CURVE('',#41322,#41324,#33141,.T.) ;
#52054=EDGE_CURVE('',#41325,#41324,#7877,.T.) ;
#52055=EDGE_CURVE('',#41325,#41323,#33142,.T.) ;
#52056=EDGE_CURVE('',#41310,#41325,#7878,.T.) ;
#52057=EDGE_CURVE('',#41324,#41311,#7879,.T.) ;
#52058=EDGE_CURVE('',#41326,#41327,#7880,.T.) ;
#52059=EDGE_CURVE('',#41327,#41328,#7881,.T.) ;
#52060=EDGE_CURVE('',#41328,#41329,#7882,.T.) ;
#52061=EDGE_CURVE('',#41329,#41326,#7883,.T.) ;
#52062=EDGE_CURVE('',#41330,#41331,#7884,.T.) ;
#52063=EDGE_CURVE('',#41331,#41332,#33143,.T.) ;
#52064=EDGE_CURVE('',#41333,#41332,#7885,.T.) ;
#52065=EDGE_CURVE('',#41333,#41330,#33144,.T.) ;
#52066=EDGE_CURVE('',#41332,#41334,#7886,.T.) ;
#52067=EDGE_CURVE('',#41335,#41334,#7887,.T.) ;
#52068=EDGE_CURVE('',#41335,#41333,#7888,.T.) ;
#52069=EDGE_CURVE('',#41334,#41336,#33145,.T.) ;
#52070=EDGE_CURVE('',#41337,#41336,#7889,.T.) ;
#52071=EDGE_CURVE('',#41337,#41335,#33146,.T.) ;
#52072=EDGE_CURVE('',#41336,#41338,#7890,.T.) ;
#52073=EDGE_CURVE('',#41339,#41338,#7891,.T.) ;
#52074=EDGE_CURVE('',#41339,#41337,#7892,.T.) ;
#52075=EDGE_CURVE('',#41338,#41340,#33147,.T.) ;
#52076=EDGE_CURVE('',#41341,#41340,#7893,.T.) ;
#52077=EDGE_CURVE('',#41341,#41339,#33148,.T.) ;
#52078=EDGE_CURVE('',#41340,#41342,#7894,.T.) ;
#52079=EDGE_CURVE('',#41343,#41342,#7895,.T.) ;
#52080=EDGE_CURVE('',#41343,#41341,#7896,.T.) ;
#52081=EDGE_CURVE('',#41342,#41344,#33149,.T.) ;
#52082=EDGE_CURVE('',#41345,#41344,#7897,.T.) ;
#52083=EDGE_CURVE('',#41345,#41343,#33150,.T.) ;
#52084=EDGE_CURVE('',#41330,#41345,#7898,.T.) ;
#52085=EDGE_CURVE('',#41344,#41331,#7899,.T.) ;
#52086=EDGE_CURVE('',#41346,#41347,#7900,.T.) ;
#52087=EDGE_CURVE('',#41347,#41348,#7901,.T.) ;
#52088=EDGE_CURVE('',#41348,#41349,#7902,.T.) ;
#52089=EDGE_CURVE('',#41349,#41346,#7903,.T.) ;
#52090=EDGE_CURVE('',#41350,#41351,#7904,.T.) ;
#52091=EDGE_CURVE('',#41351,#41352,#33151,.T.) ;
#52092=EDGE_CURVE('',#41353,#41352,#7905,.T.) ;
#52093=EDGE_CURVE('',#41353,#41350,#33152,.T.) ;
#52094=EDGE_CURVE('',#41352,#41354,#7906,.T.) ;
#52095=EDGE_CURVE('',#41355,#41354,#7907,.T.) ;
#52096=EDGE_CURVE('',#41355,#41353,#7908,.T.) ;
#52097=EDGE_CURVE('',#41354,#41356,#33153,.T.) ;
#52098=EDGE_CURVE('',#41357,#41356,#7909,.T.) ;
#52099=EDGE_CURVE('',#41357,#41355,#33154,.T.) ;
#52100=EDGE_CURVE('',#41356,#41358,#7910,.T.) ;
#52101=EDGE_CURVE('',#41359,#41358,#7911,.T.) ;
#52102=EDGE_CURVE('',#41359,#41357,#7912,.T.) ;
#52103=EDGE_CURVE('',#41358,#41360,#33155,.T.) ;
#52104=EDGE_CURVE('',#41361,#41360,#7913,.T.) ;
#52105=EDGE_CURVE('',#41361,#41359,#33156,.T.) ;
#52106=EDGE_CURVE('',#41360,#41362,#7914,.T.) ;
#52107=EDGE_CURVE('',#41363,#41362,#7915,.T.) ;
#52108=EDGE_CURVE('',#41363,#41361,#7916,.T.) ;
#52109=EDGE_CURVE('',#41362,#41364,#33157,.T.) ;
#52110=EDGE_CURVE('',#41365,#41364,#7917,.T.) ;
#52111=EDGE_CURVE('',#41365,#41363,#33158,.T.) ;
#52112=EDGE_CURVE('',#41350,#41365,#7918,.T.) ;
#52113=EDGE_CURVE('',#41364,#41351,#7919,.T.) ;
#52114=EDGE_CURVE('',#41366,#41367,#7920,.T.) ;
#52115=EDGE_CURVE('',#41367,#41368,#7921,.T.) ;
#52116=EDGE_CURVE('',#41368,#41369,#7922,.T.) ;
#52117=EDGE_CURVE('',#41369,#41366,#7923,.T.) ;
#52118=EDGE_CURVE('',#41370,#41371,#7924,.T.) ;
#52119=EDGE_CURVE('',#41371,#41372,#33159,.T.) ;
#52120=EDGE_CURVE('',#41373,#41372,#7925,.T.) ;
#52121=EDGE_CURVE('',#41373,#41370,#33160,.T.) ;
#52122=EDGE_CURVE('',#41372,#41374,#7926,.T.) ;
#52123=EDGE_CURVE('',#41375,#41374,#7927,.T.) ;
#52124=EDGE_CURVE('',#41375,#41373,#7928,.T.) ;
#52125=EDGE_CURVE('',#41374,#41376,#33161,.T.) ;
#52126=EDGE_CURVE('',#41377,#41376,#7929,.T.) ;
#52127=EDGE_CURVE('',#41377,#41375,#33162,.T.) ;
#52128=EDGE_CURVE('',#41376,#41378,#7930,.T.) ;
#52129=EDGE_CURVE('',#41379,#41378,#7931,.T.) ;
#52130=EDGE_CURVE('',#41379,#41377,#7932,.T.) ;
#52131=EDGE_CURVE('',#41378,#41380,#33163,.T.) ;
#52132=EDGE_CURVE('',#41381,#41380,#7933,.T.) ;
#52133=EDGE_CURVE('',#41381,#41379,#33164,.T.) ;
#52134=EDGE_CURVE('',#41380,#41382,#7934,.T.) ;
#52135=EDGE_CURVE('',#41383,#41382,#7935,.T.) ;
#52136=EDGE_CURVE('',#41383,#41381,#7936,.T.) ;
#52137=EDGE_CURVE('',#41382,#41384,#33165,.T.) ;
#52138=EDGE_CURVE('',#41385,#41384,#7937,.T.) ;
#52139=EDGE_CURVE('',#41385,#41383,#33166,.T.) ;
#52140=EDGE_CURVE('',#41370,#41385,#7938,.T.) ;
#52141=EDGE_CURVE('',#41384,#41371,#7939,.T.) ;
#52142=EDGE_CURVE('',#41386,#41387,#7940,.T.) ;
#52143=EDGE_CURVE('',#41387,#41388,#7941,.T.) ;
#52144=EDGE_CURVE('',#41388,#41389,#7942,.T.) ;
#52145=EDGE_CURVE('',#41389,#41386,#7943,.T.) ;
#52146=EDGE_CURVE('',#41390,#41391,#7944,.T.) ;
#52147=EDGE_CURVE('',#41391,#41392,#33167,.T.) ;
#52148=EDGE_CURVE('',#41393,#41392,#7945,.T.) ;
#52149=EDGE_CURVE('',#41393,#41390,#33168,.T.) ;
#52150=EDGE_CURVE('',#41392,#41394,#7946,.T.) ;
#52151=EDGE_CURVE('',#41395,#41394,#7947,.T.) ;
#52152=EDGE_CURVE('',#41395,#41393,#7948,.T.) ;
#52153=EDGE_CURVE('',#41394,#41396,#33169,.T.) ;
#52154=EDGE_CURVE('',#41397,#41396,#7949,.T.) ;
#52155=EDGE_CURVE('',#41397,#41395,#33170,.T.) ;
#52156=EDGE_CURVE('',#41396,#41398,#7950,.T.) ;
#52157=EDGE_CURVE('',#41399,#41398,#7951,.T.) ;
#52158=EDGE_CURVE('',#41399,#41397,#7952,.T.) ;
#52159=EDGE_CURVE('',#41398,#41400,#33171,.T.) ;
#52160=EDGE_CURVE('',#41401,#41400,#7953,.T.) ;
#52161=EDGE_CURVE('',#41401,#41399,#33172,.T.) ;
#52162=EDGE_CURVE('',#41400,#41402,#7954,.T.) ;
#52163=EDGE_CURVE('',#41403,#41402,#7955,.T.) ;
#52164=EDGE_CURVE('',#41403,#41401,#7956,.T.) ;
#52165=EDGE_CURVE('',#41402,#41404,#33173,.T.) ;
#52166=EDGE_CURVE('',#41405,#41404,#7957,.T.) ;
#52167=EDGE_CURVE('',#41405,#41403,#33174,.T.) ;
#52168=EDGE_CURVE('',#41390,#41405,#7958,.T.) ;
#52169=EDGE_CURVE('',#41404,#41391,#7959,.T.) ;
#52170=EDGE_CURVE('',#41406,#41407,#7960,.T.) ;
#52171=EDGE_CURVE('',#41407,#41408,#7961,.T.) ;
#52172=EDGE_CURVE('',#41408,#41409,#7962,.T.) ;
#52173=EDGE_CURVE('',#41409,#41406,#7963,.T.) ;
#52174=EDGE_CURVE('',#41410,#41411,#7964,.T.) ;
#52175=EDGE_CURVE('',#41411,#41412,#33175,.T.) ;
#52176=EDGE_CURVE('',#41413,#41412,#7965,.T.) ;
#52177=EDGE_CURVE('',#41413,#41410,#33176,.T.) ;
#52178=EDGE_CURVE('',#41412,#41414,#7966,.T.) ;
#52179=EDGE_CURVE('',#41415,#41414,#7967,.T.) ;
#52180=EDGE_CURVE('',#41415,#41413,#7968,.T.) ;
#52181=EDGE_CURVE('',#41414,#41416,#33177,.T.) ;
#52182=EDGE_CURVE('',#41417,#41416,#7969,.T.) ;
#52183=EDGE_CURVE('',#41417,#41415,#33178,.T.) ;
#52184=EDGE_CURVE('',#41416,#41418,#7970,.T.) ;
#52185=EDGE_CURVE('',#41419,#41418,#7971,.T.) ;
#52186=EDGE_CURVE('',#41419,#41417,#7972,.T.) ;
#52187=EDGE_CURVE('',#41418,#41420,#33179,.T.) ;
#52188=EDGE_CURVE('',#41421,#41420,#7973,.T.) ;
#52189=EDGE_CURVE('',#41421,#41419,#33180,.T.) ;
#52190=EDGE_CURVE('',#41420,#41422,#7974,.T.) ;
#52191=EDGE_CURVE('',#41423,#41422,#7975,.T.) ;
#52192=EDGE_CURVE('',#41423,#41421,#7976,.T.) ;
#52193=EDGE_CURVE('',#41422,#41424,#33181,.T.) ;
#52194=EDGE_CURVE('',#41425,#41424,#7977,.T.) ;
#52195=EDGE_CURVE('',#41425,#41423,#33182,.T.) ;
#52196=EDGE_CURVE('',#41410,#41425,#7978,.T.) ;
#52197=EDGE_CURVE('',#41424,#41411,#7979,.T.) ;
#52198=EDGE_CURVE('',#41426,#41427,#7980,.T.) ;
#52199=EDGE_CURVE('',#41427,#41428,#7981,.T.) ;
#52200=EDGE_CURVE('',#41428,#41429,#7982,.T.) ;
#52201=EDGE_CURVE('',#41429,#41426,#7983,.T.) ;
#52202=EDGE_CURVE('',#40742,#40728,#33183,.T.) ;
#52203=EDGE_CURVE('',#40739,#40742,#33184,.T.) ;
#52204=EDGE_CURVE('',#40728,#40739,#33185,.T.) ;
#52205=EDGE_CURVE('',#40736,#40741,#33186,.T.) ;
#52206=EDGE_CURVE('',#40729,#40738,#33187,.T.) ;
#52207=EDGE_CURVE('',#40743,#40731,#33188,.T.) ;
#52208=EDGE_CURVE('',#40494,#40744,#33189,.T.) ;
#52209=EDGE_CURVE('',#40495,#40743,#33190,.T.) ;
#52210=EDGE_CURVE('',#40744,#39246,#33191,.T.) ;
#52211=EDGE_CURVE('',#39245,#40745,#33192,.T.) ;
#52212=EDGE_CURVE('',#40736,#40735,#33193,.T.) ;
#52213=EDGE_CURVE('',#40735,#40741,#33194,.T.) ;
#52214=EDGE_CURVE('',#40729,#39391,#33195,.T.) ;
#52215=EDGE_CURVE('',#39392,#40738,#33196,.T.) ;
#52216=EDGE_CURVE('',#40495,#40731,#33197,.T.) ;
#52217=EDGE_CURVE('',#40745,#40485,#33198,.T.) ;
#52218=EDGE_CURVE('',#40740,#40484,#33199,.T.) ;
#52219=EDGE_CURVE('',#40732,#40740,#33200,.T.) ;
#52220=EDGE_CURVE('',#40737,#40734,#33201,.T.) ;
#52221=EDGE_CURVE('',#39386,#40737,#33202,.T.) ;
#52222=EDGE_CURVE('',#40730,#39390,#33203,.T.) ;
#52223=EDGE_CURVE('',#40496,#40730,#33204,.T.) ;
#52224=EDGE_CURVE('',#40732,#40484,#33205,.T.) ;
#52225=EDGE_CURVE('',#39385,#40734,#33206,.T.) ;
#52226=EDGE_CURVE('',#40497,#39390,#33207,.T.) ;
#52227=EDGE_CURVE('',#40733,#40483,#33208,.T.) ;
#52228=EDGE_CURVE('',#39387,#40733,#33209,.T.) ;
#52229=EDGE_CURVE('',#40498,#39389,#33210,.T.) ;
#52230=EDGE_CURVE('',#40502,#40491,#33211,.T.) ;
#52231=EDGE_CURVE('',#40503,#40490,#33212,.T.) ;
#52232=EDGE_CURVE('',#39447,#40500,#33213,.T.) ;
#52233=EDGE_CURVE('',#39448,#40503,#33214,.T.) ;
#52234=EDGE_CURVE('',#39387,#40482,#33215,.T.) ;
#52235=EDGE_CURVE('',#40498,#40489,#33216,.T.) ;
#52236=EDGE_CURVE('',#40489,#39389,#33217,.T.) ;
#52237=EDGE_CURVE('',#39448,#40490,#33218,.T.) ;
#52238=EDGE_CURVE('',#39388,#40481,#33219,.T.) ;
#52239=EDGE_CURVE('',#40486,#39388,#33220,.T.) ;
#52240=EDGE_CURVE('',#40499,#40488,#33221,.T.) ;
#52241=EDGE_CURVE('',#39449,#40499,#33222,.T.) ;
#52242=EDGE_CURVE('',#40486,#40481,#33223,.T.) ;
#52243=EDGE_CURVE('',#39450,#40488,#33224,.T.) ;
#52244=EDGE_CURVE('',#40478,#39463,#33225,.T.) ;
#52245=EDGE_CURVE('',#40479,#39737,#33226,.T.) ;
#52246=EDGE_CURVE('',#40487,#40480,#33227,.T.) ;
#52247=EDGE_CURVE('',#39451,#40487,#33228,.T.) ;
#52248=EDGE_CURVE('',#40479,#39453,#33229,.T.) ;
#52249=EDGE_CURVE('',#39452,#40480,#33230,.T.) ;
#52250=EDGE_CURVE('',#39255,#41254,#33231,.T.) ;
#52251=EDGE_CURVE('',#41256,#39254,#33232,.T.) ;
#52252=EDGE_CURVE('',#41258,#39253,#33233,.T.) ;
#52253=EDGE_CURVE('',#39256,#41252,#33234,.T.) ;
#52254=EDGE_CURVE('',#41260,#39252,#33235,.T.) ;
#52255=EDGE_CURVE('',#39249,#41251,#33236,.T.) ;
#52256=EDGE_CURVE('',#41262,#39251,#33237,.T.) ;
#52257=EDGE_CURVE('',#39250,#41264,#33238,.T.) ;
#52258=EDGE_CURVE('',#40122,#41430,#453,.T.) ;
#52259=EDGE_CURVE('',#41430,#39557,#2311,.T.) ;
#52260=EDGE_CURVE('',#39560,#41431,#2312,.T.) ;
#52261=EDGE_CURVE('',#41431,#40123,#454,.T.) ;
#52262=EDGE_CURVE('',#39559,#41432,#2313,.T.) ;
#52263=EDGE_CURVE('',#41432,#40117,#455,.T.) ;
#52264=EDGE_CURVE('',#40116,#41433,#456,.T.) ;
#52265=EDGE_CURVE('',#41433,#39560,#2314,.T.) ;
#52266=EDGE_CURVE('',#39557,#41434,#2315,.T.) ;
#52267=EDGE_CURVE('',#41434,#40125,#457,.T.) ;
#52268=EDGE_CURVE('',#40124,#41435,#458,.T.) ;
#52269=EDGE_CURVE('',#41435,#39558,#2316,.T.) ;
#52270=EDGE_CURVE('',#39558,#41436,#2317,.T.) ;
#52271=EDGE_CURVE('',#41436,#40129,#459,.T.) ;
#52272=EDGE_CURVE('',#40128,#41437,#460,.T.) ;
#52273=EDGE_CURVE('',#41437,#39559,#2318,.T.) ;
#52274=EDGE_CURVE('',#40138,#41438,#461,.T.) ;
#52275=EDGE_CURVE('',#41438,#39561,#2319,.T.) ;
#52276=EDGE_CURVE('',#39564,#41439,#2320,.T.) ;
#52277=EDGE_CURVE('',#41439,#40139,#462,.T.) ;
#52278=EDGE_CURVE('',#39563,#41440,#2321,.T.) ;
#52279=EDGE_CURVE('',#41440,#40133,#463,.T.) ;
#52280=EDGE_CURVE('',#40132,#41441,#464,.T.) ;
#52281=EDGE_CURVE('',#41441,#39564,#2322,.T.) ;
#52282=EDGE_CURVE('',#39561,#41442,#2323,.T.) ;
#52283=EDGE_CURVE('',#41442,#40141,#465,.T.) ;
#52284=EDGE_CURVE('',#40140,#41443,#466,.T.) ;
#52285=EDGE_CURVE('',#41443,#39562,#2324,.T.) ;
#52286=EDGE_CURVE('',#39562,#41444,#2325,.T.) ;
#52287=EDGE_CURVE('',#41444,#40145,#467,.T.) ;
#52288=EDGE_CURVE('',#40144,#41445,#468,.T.) ;
#52289=EDGE_CURVE('',#41445,#39563,#2326,.T.) ;
#52290=EDGE_CURVE('',#40154,#41446,#469,.T.) ;
#52291=EDGE_CURVE('',#41446,#39565,#2327,.T.) ;
#52292=EDGE_CURVE('',#39568,#41447,#2328,.T.) ;
#52293=EDGE_CURVE('',#41447,#40155,#470,.T.) ;
#52294=EDGE_CURVE('',#39567,#41448,#2329,.T.) ;
#52295=EDGE_CURVE('',#41448,#40149,#471,.T.) ;
#52296=EDGE_CURVE('',#40148,#41449,#472,.T.) ;
#52297=EDGE_CURVE('',#41449,#39568,#2330,.T.) ;
#52298=EDGE_CURVE('',#39565,#41450,#2331,.T.) ;
#52299=EDGE_CURVE('',#41450,#40157,#473,.T.) ;
#52300=EDGE_CURVE('',#40156,#41451,#474,.T.) ;
#52301=EDGE_CURVE('',#41451,#39566,#2332,.T.) ;
#52302=EDGE_CURVE('',#39566,#41452,#2333,.T.) ;
#52303=EDGE_CURVE('',#41452,#40161,#475,.T.) ;
#52304=EDGE_CURVE('',#40160,#41453,#476,.T.) ;
#52305=EDGE_CURVE('',#41453,#39567,#2334,.T.) ;
#52306=EDGE_CURVE('',#40170,#41454,#477,.T.) ;
#52307=EDGE_CURVE('',#41454,#39569,#2335,.T.) ;
#52308=EDGE_CURVE('',#39572,#41455,#2336,.T.) ;
#52309=EDGE_CURVE('',#41455,#40171,#478,.T.) ;
#52310=EDGE_CURVE('',#39571,#41456,#2337,.T.) ;
#52311=EDGE_CURVE('',#41456,#40165,#479,.T.) ;
#52312=EDGE_CURVE('',#40164,#41457,#480,.T.) ;
#52313=EDGE_CURVE('',#41457,#39572,#2338,.T.) ;
#52314=EDGE_CURVE('',#39569,#41458,#2339,.T.) ;
#52315=EDGE_CURVE('',#41458,#40173,#481,.T.) ;
#52316=EDGE_CURVE('',#40172,#41459,#482,.T.) ;
#52317=EDGE_CURVE('',#41459,#39570,#2340,.T.) ;
#52318=EDGE_CURVE('',#39570,#41460,#2341,.T.) ;
#52319=EDGE_CURVE('',#41460,#40177,#483,.T.) ;
#52320=EDGE_CURVE('',#40176,#41461,#484,.T.) ;
#52321=EDGE_CURVE('',#41461,#39571,#2342,.T.) ;
#52322=EDGE_CURVE('',#40186,#41462,#485,.T.) ;
#52323=EDGE_CURVE('',#41462,#39573,#2343,.T.) ;
#52324=EDGE_CURVE('',#39576,#41463,#2344,.T.) ;
#52325=EDGE_CURVE('',#41463,#40187,#486,.T.) ;
#52326=EDGE_CURVE('',#39575,#41464,#2345,.T.) ;
#52327=EDGE_CURVE('',#41464,#40181,#487,.T.) ;
#52328=EDGE_CURVE('',#40180,#41465,#488,.T.) ;
#52329=EDGE_CURVE('',#41465,#39576,#2346,.T.) ;
#52330=EDGE_CURVE('',#39573,#41466,#2347,.T.) ;
#52331=EDGE_CURVE('',#41466,#40189,#489,.T.) ;
#52332=EDGE_CURVE('',#40188,#41467,#490,.T.) ;
#52333=EDGE_CURVE('',#41467,#39574,#2348,.T.) ;
#52334=EDGE_CURVE('',#39574,#41468,#2349,.T.) ;
#52335=EDGE_CURVE('',#41468,#40193,#491,.T.) ;
#52336=EDGE_CURVE('',#40192,#41469,#492,.T.) ;
#52337=EDGE_CURVE('',#41469,#39575,#2350,.T.) ;
#52338=EDGE_CURVE('',#40202,#41470,#493,.T.) ;
#52339=EDGE_CURVE('',#41470,#39577,#2351,.T.) ;
#52340=EDGE_CURVE('',#39580,#41471,#2352,.T.) ;
#52341=EDGE_CURVE('',#41471,#40203,#494,.T.) ;
#52342=EDGE_CURVE('',#39579,#41472,#2353,.T.) ;
#52343=EDGE_CURVE('',#41472,#40197,#495,.T.) ;
#52344=EDGE_CURVE('',#40196,#41473,#496,.T.) ;
#52345=EDGE_CURVE('',#41473,#39580,#2354,.T.) ;
#52346=EDGE_CURVE('',#39577,#41474,#2355,.T.) ;
#52347=EDGE_CURVE('',#41474,#40205,#497,.T.) ;
#52348=EDGE_CURVE('',#40204,#41475,#498,.T.) ;
#52349=EDGE_CURVE('',#41475,#39578,#2356,.T.) ;
#52350=EDGE_CURVE('',#39578,#41476,#2357,.T.) ;
#52351=EDGE_CURVE('',#41476,#40209,#499,.T.) ;
#52352=EDGE_CURVE('',#40208,#41477,#500,.T.) ;
#52353=EDGE_CURVE('',#41477,#39579,#2358,.T.) ;
#52354=EDGE_CURVE('',#40218,#41478,#501,.T.) ;
#52355=EDGE_CURVE('',#41478,#39581,#2359,.T.) ;
#52356=EDGE_CURVE('',#39584,#41479,#2360,.T.) ;
#52357=EDGE_CURVE('',#41479,#40219,#502,.T.) ;
#52358=EDGE_CURVE('',#39583,#41480,#2361,.T.) ;
#52359=EDGE_CURVE('',#41480,#40213,#503,.T.) ;
#52360=EDGE_CURVE('',#40212,#41481,#504,.T.) ;
#52361=EDGE_CURVE('',#41481,#39584,#2362,.T.) ;
#52362=EDGE_CURVE('',#39581,#41482,#2363,.T.) ;
#52363=EDGE_CURVE('',#41482,#40221,#505,.T.) ;
#52364=EDGE_CURVE('',#40220,#41483,#506,.T.) ;
#52365=EDGE_CURVE('',#41483,#39582,#2364,.T.) ;
#52366=EDGE_CURVE('',#39582,#41484,#2365,.T.) ;
#52367=EDGE_CURVE('',#41484,#40225,#507,.T.) ;
#52368=EDGE_CURVE('',#40224,#41485,#508,.T.) ;
#52369=EDGE_CURVE('',#41485,#39583,#2366,.T.) ;
#52370=EDGE_CURVE('',#40234,#41486,#509,.T.) ;
#52371=EDGE_CURVE('',#41486,#39585,#2367,.T.) ;
#52372=EDGE_CURVE('',#39588,#41487,#2368,.T.) ;
#52373=EDGE_CURVE('',#41487,#40235,#510,.T.) ;
#52374=EDGE_CURVE('',#39587,#41488,#2369,.T.) ;
#52375=EDGE_CURVE('',#41488,#40229,#511,.T.) ;
#52376=EDGE_CURVE('',#40228,#41489,#512,.T.) ;
#52377=EDGE_CURVE('',#41489,#39588,#2370,.T.) ;
#52378=EDGE_CURVE('',#39585,#41490,#2371,.T.) ;
#52379=EDGE_CURVE('',#41490,#40237,#513,.T.) ;
#52380=EDGE_CURVE('',#40236,#41491,#514,.T.) ;
#52381=EDGE_CURVE('',#41491,#39586,#2372,.T.) ;
#52382=EDGE_CURVE('',#39586,#41492,#2373,.T.) ;
#52383=EDGE_CURVE('',#41492,#40241,#515,.T.) ;
#52384=EDGE_CURVE('',#40240,#41493,#516,.T.) ;
#52385=EDGE_CURVE('',#41493,#39587,#2374,.T.) ;
#52386=EDGE_CURVE('',#39595,#40259,#33239,.T.) ;
#52387=EDGE_CURVE('',#40256,#39594,#33240,.T.) ;
#52388=EDGE_CURVE('',#40255,#39593,#33241,.T.) ;
#52389=EDGE_CURVE('',#40256,#40255,#33242,.T.) ;
#52390=EDGE_CURVE('',#40247,#40259,#33243,.T.) ;
#52391=EDGE_CURVE('',#39596,#40247,#33244,.T.) ;
#52392=EDGE_CURVE('',#40252,#39592,#33245,.T.) ;
#52393=EDGE_CURVE('',#40257,#40254,#33246,.T.) ;
#52394=EDGE_CURVE('',#40258,#40263,#33247,.T.) ;
#52395=EDGE_CURVE('',#40260,#40257,#33248,.T.) ;
#52396=EDGE_CURVE('',#40244,#40258,#33249,.T.) ;
#52397=EDGE_CURVE('',#39590,#40246,#33250,.T.) ;
#52398=EDGE_CURVE('',#39591,#40250,#33251,.T.) ;
#52399=EDGE_CURVE('',#40251,#39589,#33252,.T.) ;
#52400=EDGE_CURVE('',#40252,#40250,#33253,.T.) ;
#52401=EDGE_CURVE('',#40260,#40254,#33254,.T.) ;
#52402=EDGE_CURVE('',#40244,#40263,#33255,.T.) ;
#52403=EDGE_CURVE('',#40251,#40246,#33256,.T.) ;
#52404=EDGE_CURVE('',#40253,#40249,#33257,.T.) ;
#52405=EDGE_CURVE('',#40261,#40253,#33258,.T.) ;
#52406=EDGE_CURVE('',#40245,#40262,#33259,.T.) ;
#52407=EDGE_CURVE('',#40248,#40245,#33260,.T.) ;
#52408=EDGE_CURVE('',#40261,#40249,#33261,.T.) ;
#52409=EDGE_CURVE('',#40248,#40262,#33262,.T.) ;
#52410=EDGE_CURVE('',#40272,#40279,#33263,.T.) ;
#52411=EDGE_CURVE('',#40273,#40443,#33264,.T.) ;
#52412=EDGE_CURVE('',#40440,#40272,#33265,.T.) ;
#52413=EDGE_CURVE('',#40274,#40273,#33266,.T.) ;
#52414=EDGE_CURVE('',#40440,#40279,#33267,.T.) ;
#52415=EDGE_CURVE('',#40274,#40443,#33268,.T.) ;
#52416=EDGE_CURVE('',#40278,#40277,#33269,.T.) ;
#52417=EDGE_CURVE('',#40441,#40278,#33270,.T.) ;
#52418=EDGE_CURVE('',#40275,#40442,#33271,.T.) ;
#52419=EDGE_CURVE('',#40276,#40275,#33272,.T.) ;
#52420=EDGE_CURVE('',#40441,#40277,#33273,.T.) ;
#52421=EDGE_CURVE('',#40276,#40442,#33274,.T.) ;
#52422=EDGE_CURVE('',#39996,#40065,#33275,.T.) ;
#52423=EDGE_CURVE('',#39996,#39994,#33276,.T.) ;
#52424=EDGE_CURVE('',#39994,#40065,#33277,.T.) ;
#52425=EDGE_CURVE('',#39995,#40064,#2375,.T.) ;
#52426=EDGE_CURVE('',#39997,#39993,#33278,.T.) ;
#52427=EDGE_CURVE('',#40014,#39997,#33279,.T.) ;
#52428=EDGE_CURVE('',#39995,#39475,#33280,.T.) ;
#52429=EDGE_CURVE('',#39476,#40064,#33281,.T.) ;
#52430=EDGE_CURVE('',#40014,#39993,#33282,.T.) ;
#52431=EDGE_CURVE('',#40066,#40007,#33283,.T.) ;
#52432=EDGE_CURVE('',#40067,#40011,#2376,.T.) ;
#52433=EDGE_CURVE('',#40008,#40066,#33284,.T.) ;
#52434=EDGE_CURVE('',#39477,#40067,#33285,.T.) ;
#52435=EDGE_CURVE('',#39992,#39474,#33286,.T.) ;
#52436=EDGE_CURVE('',#40015,#39992,#517,.T.) ;
#52437=EDGE_CURVE('',#40008,#40007,#33287,.T.) ;
#52438=EDGE_CURVE('',#39478,#40011,#33288,.T.) ;
#52439=EDGE_CURVE('',#40015,#39473,#33289,.T.) ;
#52440=EDGE_CURVE('',#40006,#40013,#33290,.T.) ;
#52441=EDGE_CURVE('',#40009,#40006,#33291,.T.) ;
#52442=EDGE_CURVE('',#39472,#40010,#33292,.T.) ;
#52443=EDGE_CURVE('',#40012,#39471,#33293,.T.) ;
#52444=EDGE_CURVE('',#40009,#40013,#33294,.T.) ;
#52445=EDGE_CURVE('',#40012,#40010,#518,.T.) ;
#52446=EDGE_CURVE('',#39482,#41494,#519,.T.) ;
#52447=EDGE_CURVE('',#41494,#39989,#520,.T.) ;
#52448=EDGE_CURVE('',#39988,#41495,#521,.T.) ;
#52449=EDGE_CURVE('',#41495,#41496,#522,.T.) ;
#52450=EDGE_CURVE('',#41496,#39479,#523,.T.) ;
#52451=EDGE_CURVE('',#39479,#41497,#524,.T.) ;
#52452=EDGE_CURVE('',#41497,#40017,#525,.T.) ;
#52453=EDGE_CURVE('',#40016,#41498,#526,.T.) ;
#52454=EDGE_CURVE('',#41498,#39480,#527,.T.) ;
#52455=EDGE_CURVE('',#40068,#39482,#528,.T.) ;
#52456=EDGE_CURVE('',#39481,#40069,#529,.T.) ;
#52457=EDGE_CURVE('',#39480,#41499,#530,.T.) ;
#52458=EDGE_CURVE('',#41499,#41500,#531,.T.) ;
#52459=EDGE_CURVE('',#41500,#39973,#532,.T.) ;
#52460=EDGE_CURVE('',#39972,#41501,#533,.T.) ;
#52461=EDGE_CURVE('',#41501,#39481,#534,.T.) ;
#52462=EDGE_CURVE('',#39486,#41502,#535,.T.) ;
#52463=EDGE_CURVE('',#41502,#39969,#536,.T.) ;
#52464=EDGE_CURVE('',#39968,#41503,#537,.T.) ;
#52465=EDGE_CURVE('',#41503,#41504,#538,.T.) ;
#52466=EDGE_CURVE('',#41504,#39483,#539,.T.) ;
#52467=EDGE_CURVE('',#39483,#41505,#540,.T.) ;
#52468=EDGE_CURVE('',#41505,#40023,#541,.T.) ;
#52469=EDGE_CURVE('',#40022,#41506,#542,.T.) ;
#52470=EDGE_CURVE('',#41506,#39484,#543,.T.) ;
#52471=EDGE_CURVE('',#40074,#39486,#544,.T.) ;
#52472=EDGE_CURVE('',#39485,#40075,#545,.T.) ;
#52473=EDGE_CURVE('',#39484,#41507,#546,.T.) ;
#52474=EDGE_CURVE('',#41507,#41508,#547,.T.) ;
#52475=EDGE_CURVE('',#41508,#39953,#548,.T.) ;
#52476=EDGE_CURVE('',#39952,#41509,#549,.T.) ;
#52477=EDGE_CURVE('',#41509,#39485,#550,.T.) ;
#52478=EDGE_CURVE('',#39490,#41510,#551,.T.) ;
#52479=EDGE_CURVE('',#41510,#39949,#552,.T.) ;
#52480=EDGE_CURVE('',#39948,#41511,#553,.T.) ;
#52481=EDGE_CURVE('',#41511,#41512,#554,.T.) ;
#52482=EDGE_CURVE('',#41512,#39487,#555,.T.) ;
#52483=EDGE_CURVE('',#39487,#41513,#556,.T.) ;
#52484=EDGE_CURVE('',#41513,#40029,#557,.T.) ;
#52485=EDGE_CURVE('',#40028,#41514,#558,.T.) ;
#52486=EDGE_CURVE('',#41514,#39488,#559,.T.) ;
#52487=EDGE_CURVE('',#40080,#39490,#560,.T.) ;
#52488=EDGE_CURVE('',#39489,#40081,#561,.T.) ;
#52489=EDGE_CURVE('',#39488,#41515,#562,.T.) ;
#52490=EDGE_CURVE('',#41515,#41516,#563,.T.) ;
#52491=EDGE_CURVE('',#41516,#39933,#564,.T.) ;
#52492=EDGE_CURVE('',#39932,#41517,#565,.T.) ;
#52493=EDGE_CURVE('',#41517,#39489,#566,.T.) ;
#52494=EDGE_CURVE('',#39494,#41518,#567,.T.) ;
#52495=EDGE_CURVE('',#41518,#39929,#568,.T.) ;
#52496=EDGE_CURVE('',#39928,#41519,#569,.T.) ;
#52497=EDGE_CURVE('',#41519,#41520,#570,.T.) ;
#52498=EDGE_CURVE('',#41520,#39491,#571,.T.) ;
#52499=EDGE_CURVE('',#39491,#41521,#572,.T.) ;
#52500=EDGE_CURVE('',#41521,#40035,#573,.T.) ;
#52501=EDGE_CURVE('',#40034,#41522,#574,.T.) ;
#52502=EDGE_CURVE('',#41522,#39492,#575,.T.) ;
#52503=EDGE_CURVE('',#40086,#39494,#576,.T.) ;
#52504=EDGE_CURVE('',#39493,#40087,#577,.T.) ;
#52505=EDGE_CURVE('',#39492,#41523,#578,.T.) ;
#52506=EDGE_CURVE('',#41523,#41524,#579,.T.) ;
#52507=EDGE_CURVE('',#41524,#39913,#580,.T.) ;
#52508=EDGE_CURVE('',#39912,#41525,#581,.T.) ;
#52509=EDGE_CURVE('',#41525,#39493,#582,.T.) ;
#52510=EDGE_CURVE('',#39498,#41526,#583,.T.) ;
#52511=EDGE_CURVE('',#41526,#39909,#584,.T.) ;
#52512=EDGE_CURVE('',#39908,#41527,#585,.T.) ;
#52513=EDGE_CURVE('',#41527,#41528,#586,.T.) ;
#52514=EDGE_CURVE('',#41528,#39495,#587,.T.) ;
#52515=EDGE_CURVE('',#39495,#41529,#588,.T.) ;
#52516=EDGE_CURVE('',#41529,#40041,#589,.T.) ;
#52517=EDGE_CURVE('',#40040,#41530,#590,.T.) ;
#52518=EDGE_CURVE('',#41530,#39496,#591,.T.) ;
#52519=EDGE_CURVE('',#40092,#39498,#592,.T.) ;
#52520=EDGE_CURVE('',#39497,#40093,#593,.T.) ;
#52521=EDGE_CURVE('',#39496,#41531,#594,.T.) ;
#52522=EDGE_CURVE('',#41531,#41532,#595,.T.) ;
#52523=EDGE_CURVE('',#41532,#39893,#596,.T.) ;
#52524=EDGE_CURVE('',#39892,#41533,#597,.T.) ;
#52525=EDGE_CURVE('',#41533,#39497,#598,.T.) ;
#52526=EDGE_CURVE('',#39502,#41534,#599,.T.) ;
#52527=EDGE_CURVE('',#41534,#39889,#600,.T.) ;
#52528=EDGE_CURVE('',#39888,#41535,#601,.T.) ;
#52529=EDGE_CURVE('',#41535,#41536,#602,.T.) ;
#52530=EDGE_CURVE('',#41536,#39499,#603,.T.) ;
#52531=EDGE_CURVE('',#39499,#41537,#604,.T.) ;
#52532=EDGE_CURVE('',#41537,#40047,#605,.T.) ;
#52533=EDGE_CURVE('',#40046,#41538,#606,.T.) ;
#52534=EDGE_CURVE('',#41538,#39500,#607,.T.) ;
#52535=EDGE_CURVE('',#40098,#39502,#608,.T.) ;
#52536=EDGE_CURVE('',#39501,#40099,#609,.T.) ;
#52537=EDGE_CURVE('',#39500,#41539,#610,.T.) ;
#52538=EDGE_CURVE('',#41539,#41540,#611,.T.) ;
#52539=EDGE_CURVE('',#41540,#39873,#612,.T.) ;
#52540=EDGE_CURVE('',#39872,#41541,#613,.T.) ;
#52541=EDGE_CURVE('',#41541,#39501,#614,.T.) ;
#52542=EDGE_CURVE('',#39506,#41542,#615,.T.) ;
#52543=EDGE_CURVE('',#41542,#39869,#616,.T.) ;
#52544=EDGE_CURVE('',#39868,#41543,#617,.T.) ;
#52545=EDGE_CURVE('',#41543,#41544,#618,.T.) ;
#52546=EDGE_CURVE('',#41544,#39503,#619,.T.) ;
#52547=EDGE_CURVE('',#39503,#41545,#620,.T.) ;
#52548=EDGE_CURVE('',#41545,#40053,#621,.T.) ;
#52549=EDGE_CURVE('',#40052,#41546,#622,.T.) ;
#52550=EDGE_CURVE('',#41546,#39504,#623,.T.) ;
#52551=EDGE_CURVE('',#40104,#39506,#624,.T.) ;
#52552=EDGE_CURVE('',#39505,#40105,#625,.T.) ;
#52553=EDGE_CURVE('',#39504,#41547,#626,.T.) ;
#52554=EDGE_CURVE('',#41547,#41548,#627,.T.) ;
#52555=EDGE_CURVE('',#41548,#39853,#628,.T.) ;
#52556=EDGE_CURVE('',#39852,#41549,#629,.T.) ;
#52557=EDGE_CURVE('',#41549,#39505,#630,.T.) ;
#52558=EDGE_CURVE('',#39510,#41550,#631,.T.) ;
#52559=EDGE_CURVE('',#41550,#39849,#632,.T.) ;
#52560=EDGE_CURVE('',#39848,#41551,#633,.T.) ;
#52561=EDGE_CURVE('',#41551,#41552,#634,.T.) ;
#52562=EDGE_CURVE('',#41552,#39507,#635,.T.) ;
#52563=EDGE_CURVE('',#39507,#41553,#636,.T.) ;
#52564=EDGE_CURVE('',#41553,#40059,#637,.T.) ;
#52565=EDGE_CURVE('',#40058,#41554,#638,.T.) ;
#52566=EDGE_CURVE('',#41554,#39508,#639,.T.) ;
#52567=EDGE_CURVE('',#40110,#39510,#640,.T.) ;
#52568=EDGE_CURVE('',#39509,#40111,#641,.T.) ;
#52569=EDGE_CURVE('',#39508,#41555,#642,.T.) ;
#52570=EDGE_CURVE('',#41555,#41556,#643,.T.) ;
#52571=EDGE_CURVE('',#41556,#39833,#644,.T.) ;
#52572=EDGE_CURVE('',#39832,#41557,#645,.T.) ;
#52573=EDGE_CURVE('',#41557,#39509,#646,.T.) ;
#52574=EDGE_CURVE('',#39115,#41032,#33295,.T.) ;
#52575=EDGE_CURVE('',#41033,#39114,#33296,.T.) ;
#52576=EDGE_CURVE('',#41029,#39113,#33297,.T.) ;
#52577=EDGE_CURVE('',#41033,#41029,#33298,.T.) ;
#52578=EDGE_CURVE('',#41021,#41032,#33299,.T.) ;
#52579=EDGE_CURVE('',#39116,#41021,#33300,.T.) ;
#52580=EDGE_CURVE('',#41026,#39112,#33301,.T.) ;
#52581=EDGE_CURVE('',#41030,#41028,#33302,.T.) ;
#52582=EDGE_CURVE('',#41031,#41037,#33303,.T.) ;
#52583=EDGE_CURVE('',#41034,#41030,#33304,.T.) ;
#52584=EDGE_CURVE('',#41018,#41031,#33305,.T.) ;
#52585=EDGE_CURVE('',#39110,#41020,#33306,.T.) ;
#52586=EDGE_CURVE('',#39111,#41022,#33307,.T.) ;
#52587=EDGE_CURVE('',#41023,#39109,#33308,.T.) ;
#52588=EDGE_CURVE('',#41026,#41022,#33309,.T.) ;
#52589=EDGE_CURVE('',#41034,#41028,#33310,.T.) ;
#52590=EDGE_CURVE('',#41018,#41037,#33311,.T.) ;
#52591=EDGE_CURVE('',#41023,#41020,#33312,.T.) ;
#52592=EDGE_CURVE('',#41027,#41025,#33313,.T.) ;
#52593=EDGE_CURVE('',#41035,#41027,#33314,.T.) ;
#52594=EDGE_CURVE('',#41019,#41036,#33315,.T.) ;
#52595=EDGE_CURVE('',#41024,#41019,#33316,.T.) ;
#52596=EDGE_CURVE('',#41035,#41025,#33317,.T.) ;
#52597=EDGE_CURVE('',#41024,#41036,#33318,.T.) ;
#52598=EDGE_CURVE('',#41046,#41053,#33319,.T.) ;
#52599=EDGE_CURVE('',#41047,#41217,#33320,.T.) ;
#52600=EDGE_CURVE('',#41214,#41046,#33321,.T.) ;
#52601=EDGE_CURVE('',#41048,#41047,#33322,.T.) ;
#52602=EDGE_CURVE('',#41214,#41053,#33323,.T.) ;
#52603=EDGE_CURVE('',#41048,#41217,#33324,.T.) ;
#52604=EDGE_CURVE('',#41052,#41051,#33325,.T.) ;
#52605=EDGE_CURVE('',#41215,#41052,#33326,.T.) ;
#52606=EDGE_CURVE('',#41049,#41216,#33327,.T.) ;
#52607=EDGE_CURVE('',#41050,#41049,#33328,.T.) ;
#52608=EDGE_CURVE('',#41215,#41051,#33329,.T.) ;
#52609=EDGE_CURVE('',#41050,#41216,#33330,.T.) ;
#52610=EDGE_CURVE('',#41257,#41269,#33331,.T.) ;
#52611=EDGE_CURVE('',#41266,#41259,#33332,.T.) ;
#52612=EDGE_CURVE('',#41266,#41261,#33333,.T.) ;
#52613=EDGE_CURVE('',#41255,#41269,#33334,.T.) ;
#52614=EDGE_CURVE('',#41267,#41263,#33335,.T.) ;
#52615=EDGE_CURVE('',#41253,#41268,#33336,.T.) ;
#52616=EDGE_CURVE('',#41267,#41265,#33337,.T.) ;
#52617=EDGE_CURVE('',#41250,#41268,#33338,.T.) ;
#52618=EDGE_CURVE('',#40759,#40754,#33339,.T.) ;
#52619=EDGE_CURVE('',#40753,#40759,#33340,.T.) ;
#52620=EDGE_CURVE('',#40754,#40753,#33341,.T.) ;
#52621=EDGE_CURVE('',#40750,#40758,#33342,.T.) ;
#52622=EDGE_CURVE('',#40755,#40752,#33343,.T.) ;
#52623=EDGE_CURVE('',#40760,#40757,#33344,.T.) ;
#52624=EDGE_CURVE('',#40763,#40513,#33345,.T.) ;
#52625=EDGE_CURVE('',#40758,#40512,#33346,.T.) ;
#52626=EDGE_CURVE('',#40750,#40512,#33347,.T.) ;
#52627=EDGE_CURVE('',#40755,#39378,#33348,.T.) ;
#52628=EDGE_CURVE('',#39377,#40752,#33349,.T.) ;
#52629=EDGE_CURVE('',#40760,#40746,#33350,.T.) ;
#52630=EDGE_CURVE('',#40746,#40757,#33351,.T.) ;
#52631=EDGE_CURVE('',#40762,#39234,#33352,.T.) ;
#52632=EDGE_CURVE('',#39233,#40763,#33353,.T.) ;
#52633=EDGE_CURVE('',#40751,#40511,#33354,.T.) ;
#52634=EDGE_CURVE('',#39379,#40751,#33355,.T.) ;
#52635=EDGE_CURVE('',#40756,#39384,#33356,.T.) ;
#52636=EDGE_CURVE('',#40747,#40756,#33357,.T.) ;
#52637=EDGE_CURVE('',#40761,#40749,#33358,.T.) ;
#52638=EDGE_CURVE('',#40522,#40762,#33359,.T.) ;
#52639=EDGE_CURVE('',#40523,#40761,#33360,.T.) ;
#52640=EDGE_CURVE('',#39379,#40510,#33361,.T.) ;
#52641=EDGE_CURVE('',#40747,#39383,#33362,.T.) ;
#52642=EDGE_CURVE('',#40523,#40749,#33363,.T.) ;
#52643=EDGE_CURVE('',#40506,#40501,#33364,.T.) ;
#52644=EDGE_CURVE('',#40507,#40500,#33365,.T.) ;
#52645=EDGE_CURVE('',#39380,#40509,#33366,.T.) ;
#52646=EDGE_CURVE('',#40748,#39382,#33367,.T.) ;
#52647=EDGE_CURVE('',#40524,#40748,#33368,.T.) ;
#52648=EDGE_CURVE('',#40507,#39447,#33369,.T.) ;
#52649=EDGE_CURVE('',#39380,#40514,#33370,.T.) ;
#52650=EDGE_CURVE('',#40514,#40509,#33371,.T.) ;
#52651=EDGE_CURVE('',#40525,#39382,#33372,.T.) ;
#52652=EDGE_CURVE('',#40508,#39446,#33373,.T.) ;
#52653=EDGE_CURVE('',#40515,#40508,#33374,.T.) ;
#52654=EDGE_CURVE('',#39381,#40517,#33375,.T.) ;
#52655=EDGE_CURVE('',#40526,#39381,#33376,.T.) ;
#52656=EDGE_CURVE('',#40515,#39445,#33377,.T.) ;
#52657=EDGE_CURVE('',#40526,#40517,#33378,.T.) ;
#52658=EDGE_CURVE('',#40516,#39444,#33379,.T.) ;
#52659=EDGE_CURVE('',#40527,#40516,#33380,.T.) ;
#52660=EDGE_CURVE('',#40530,#40519,#33381,.T.) ;
#52661=EDGE_CURVE('',#40531,#40518,#33382,.T.) ;
#52662=EDGE_CURVE('',#39441,#40528,#33383,.T.) ;
#52663=EDGE_CURVE('',#39442,#40531,#33384,.T.) ;
#52664=EDGE_CURVE('',#40527,#39443,#33385,.T.) ;
#52665=EDGE_CURVE('',#39442,#40518,#33386,.T.) ;
#52666=EDGE_CURVE('',#40229,#40240,#33387,.T.) ;
#52667=EDGE_CURVE('',#40230,#40243,#33388,.T.) ;
#52668=EDGE_CURVE('',#40241,#40236,#33389,.T.) ;
#52669=EDGE_CURVE('',#40230,#40283,#33390,.T.) ;
#52670=EDGE_CURVE('',#40283,#40243,#33391,.T.) ;
#52671=EDGE_CURVE('',#40235,#40228,#33392,.T.) ;
#52672=EDGE_CURVE('',#40242,#40239,#33393,.T.) ;
#52673=EDGE_CURVE('',#40280,#40242,#33394,.T.) ;
#52674=EDGE_CURVE('',#40231,#40282,#33395,.T.) ;
#52675=EDGE_CURVE('',#40232,#40231,#33396,.T.) ;
#52676=EDGE_CURVE('',#40280,#40239,#33397,.T.) ;
#52677=EDGE_CURVE('',#40232,#40282,#33398,.T.) ;
#52678=EDGE_CURVE('',#40281,#40238,#33399,.T.) ;
#52679=EDGE_CURVE('',#40233,#40281,#33400,.T.) ;
#52680=EDGE_CURVE('',#40233,#40238,#33401,.T.) ;
#52681=EDGE_CURVE('',#40234,#40237,#33402,.T.) ;
#52682=EDGE_CURVE('',#40017,#41495,#33403,.T.) ;
#52683=EDGE_CURVE('',#40018,#39988,#33404,.T.) ;
#52684=EDGE_CURVE('',#40019,#39991,#33405,.T.) ;
#52685=EDGE_CURVE('',#39986,#40019,#33406,.T.) ;
#52686=EDGE_CURVE('',#39986,#39991,#33407,.T.) ;
#52687=EDGE_CURVE('',#39987,#39990,#33408,.T.) ;
#52688=EDGE_CURVE('',#40072,#39987,#33409,.T.) ;
#52689=EDGE_CURVE('',#40072,#39990,#33410,.T.) ;
#52690=EDGE_CURVE('',#40073,#39989,#33411,.T.) ;
#52691=EDGE_CURVE('',#40068,#41494,#33412,.T.) ;
#52692=EDGE_CURVE('',#40069,#41501,#33413,.T.) ;
#52693=EDGE_CURVE('',#40070,#39972,#33414,.T.) ;
#52694=EDGE_CURVE('',#40071,#39975,#33415,.T.) ;
#52695=EDGE_CURVE('',#39976,#40071,#33416,.T.) ;
#52696=EDGE_CURVE('',#39976,#39975,#33417,.T.) ;
#52697=EDGE_CURVE('',#39977,#39974,#33418,.T.) ;
#52698=EDGE_CURVE('',#40020,#39977,#33419,.T.) ;
#52699=EDGE_CURVE('',#40020,#39974,#33420,.T.) ;
#52700=EDGE_CURVE('',#40021,#39973,#33421,.T.) ;
#52701=EDGE_CURVE('',#40016,#41500,#33422,.T.) ;
#52702=EDGE_CURVE('',#39243,#41274,#33423,.T.) ;
#52703=EDGE_CURVE('',#41276,#39242,#33424,.T.) ;
#52704=EDGE_CURVE('',#41278,#39241,#33425,.T.) ;
#52705=EDGE_CURVE('',#39244,#41272,#33426,.T.) ;
#52706=EDGE_CURVE('',#41280,#39240,#33427,.T.) ;
#52707=EDGE_CURVE('',#39237,#41271,#33428,.T.) ;
#52708=EDGE_CURVE('',#41282,#39239,#33429,.T.) ;
#52709=EDGE_CURVE('',#39238,#41284,#33430,.T.) ;
#52710=EDGE_CURVE('',#40292,#40299,#33431,.T.) ;
#52711=EDGE_CURVE('',#40293,#40447,#33432,.T.) ;
#52712=EDGE_CURVE('',#40444,#40292,#33433,.T.) ;
#52713=EDGE_CURVE('',#40294,#40293,#33434,.T.) ;
#52714=EDGE_CURVE('',#40444,#40299,#33435,.T.) ;
#52715=EDGE_CURVE('',#40294,#40447,#33436,.T.) ;
#52716=EDGE_CURVE('',#40298,#40297,#33437,.T.) ;
#52717=EDGE_CURVE('',#40445,#40298,#33438,.T.) ;
#52718=EDGE_CURVE('',#40295,#40446,#33439,.T.) ;
#52719=EDGE_CURVE('',#40296,#40295,#33440,.T.) ;
#52720=EDGE_CURVE('',#40445,#40297,#33441,.T.) ;
#52721=EDGE_CURVE('',#40296,#40446,#33442,.T.) ;
#52722=EDGE_CURVE('',#39099,#41016,#33443,.T.) ;
#52723=EDGE_CURVE('',#41017,#39098,#33444,.T.) ;
#52724=EDGE_CURVE('',#41013,#39097,#33445,.T.) ;
#52725=EDGE_CURVE('',#41017,#41013,#33446,.T.) ;
#52726=EDGE_CURVE('',#41005,#41016,#33447,.T.) ;
#52727=EDGE_CURVE('',#39100,#41005,#33448,.T.) ;
#52728=EDGE_CURVE('',#41010,#39096,#33449,.T.) ;
#52729=EDGE_CURVE('',#41014,#41012,#33450,.T.) ;
#52730=EDGE_CURVE('',#41015,#41057,#33451,.T.) ;
#52731=EDGE_CURVE('',#41054,#41014,#33452,.T.) ;
#52732=EDGE_CURVE('',#41002,#41015,#33453,.T.) ;
#52733=EDGE_CURVE('',#39094,#41004,#33454,.T.) ;
#52734=EDGE_CURVE('',#39095,#41006,#33455,.T.) ;
#52735=EDGE_CURVE('',#41007,#39093,#33456,.T.) ;
#52736=EDGE_CURVE('',#41010,#41006,#33457,.T.) ;
#52737=EDGE_CURVE('',#41054,#41012,#33458,.T.) ;
#52738=EDGE_CURVE('',#41002,#41057,#33459,.T.) ;
#52739=EDGE_CURVE('',#41007,#41004,#33460,.T.) ;
#52740=EDGE_CURVE('',#41011,#41009,#33461,.T.) ;
#52741=EDGE_CURVE('',#41055,#41011,#33462,.T.) ;
#52742=EDGE_CURVE('',#41003,#41056,#33463,.T.) ;
#52743=EDGE_CURVE('',#41008,#41003,#33464,.T.) ;
#52744=EDGE_CURVE('',#41055,#41009,#33465,.T.) ;
#52745=EDGE_CURVE('',#41008,#41056,#33466,.T.) ;
#52746=EDGE_CURVE('',#41066,#41073,#33467,.T.) ;
#52747=EDGE_CURVE('',#41067,#41221,#33468,.T.) ;
#52748=EDGE_CURVE('',#41218,#41066,#33469,.T.) ;
#52749=EDGE_CURVE('',#41068,#41067,#33470,.T.) ;
#52750=EDGE_CURVE('',#41218,#41073,#33471,.T.) ;
#52751=EDGE_CURVE('',#41068,#41221,#33472,.T.) ;
#52752=EDGE_CURVE('',#41072,#41071,#33473,.T.) ;
#52753=EDGE_CURVE('',#41219,#41072,#33474,.T.) ;
#52754=EDGE_CURVE('',#41069,#41220,#33475,.T.) ;
#52755=EDGE_CURVE('',#41070,#41069,#33476,.T.) ;
#52756=EDGE_CURVE('',#41219,#41071,#33477,.T.) ;
#52757=EDGE_CURVE('',#41070,#41220,#33478,.T.) ;
#52758=EDGE_CURVE('',#41277,#41289,#33479,.T.) ;
#52759=EDGE_CURVE('',#41286,#41279,#33480,.T.) ;
#52760=EDGE_CURVE('',#41286,#41281,#33481,.T.) ;
#52761=EDGE_CURVE('',#41275,#41289,#33482,.T.) ;
#52762=EDGE_CURVE('',#41287,#41283,#33483,.T.) ;
#52763=EDGE_CURVE('',#41273,#41288,#33484,.T.) ;
#52764=EDGE_CURVE('',#41287,#41285,#33485,.T.) ;
#52765=EDGE_CURVE('',#41270,#41288,#33486,.T.) ;
#52766=EDGE_CURVE('',#40777,#40772,#33487,.T.) ;
#52767=EDGE_CURVE('',#40771,#40777,#33488,.T.) ;
#52768=EDGE_CURVE('',#40772,#40771,#33489,.T.) ;
#52769=EDGE_CURVE('',#40768,#40776,#33490,.T.) ;
#52770=EDGE_CURVE('',#40773,#40770,#33491,.T.) ;
#52771=EDGE_CURVE('',#40778,#40775,#33492,.T.) ;
#52772=EDGE_CURVE('',#40781,#40541,#33493,.T.) ;
#52773=EDGE_CURVE('',#40776,#40540,#33494,.T.) ;
#52774=EDGE_CURVE('',#40768,#40540,#33495,.T.) ;
#52775=EDGE_CURVE('',#40773,#39370,#33496,.T.) ;
#52776=EDGE_CURVE('',#39369,#40770,#33497,.T.) ;
#52777=EDGE_CURVE('',#40778,#40764,#33498,.T.) ;
#52778=EDGE_CURVE('',#40764,#40775,#33499,.T.) ;
#52779=EDGE_CURVE('',#40780,#39222,#33500,.T.) ;
#52780=EDGE_CURVE('',#39221,#40781,#33501,.T.) ;
#52781=EDGE_CURVE('',#40769,#40539,#33502,.T.) ;
#52782=EDGE_CURVE('',#39371,#40769,#33503,.T.) ;
#52783=EDGE_CURVE('',#40774,#39376,#33504,.T.) ;
#52784=EDGE_CURVE('',#40765,#40774,#33505,.T.) ;
#52785=EDGE_CURVE('',#40779,#40767,#33506,.T.) ;
#52786=EDGE_CURVE('',#40550,#40780,#33507,.T.) ;
#52787=EDGE_CURVE('',#40551,#40779,#33508,.T.) ;
#52788=EDGE_CURVE('',#39371,#40538,#33509,.T.) ;
#52789=EDGE_CURVE('',#40765,#39375,#33510,.T.) ;
#52790=EDGE_CURVE('',#40551,#40767,#33511,.T.) ;
#52791=EDGE_CURVE('',#40534,#40529,#33512,.T.) ;
#52792=EDGE_CURVE('',#40535,#40528,#33513,.T.) ;
#52793=EDGE_CURVE('',#39372,#40537,#33514,.T.) ;
#52794=EDGE_CURVE('',#40766,#39374,#33515,.T.) ;
#52795=EDGE_CURVE('',#40552,#40766,#33516,.T.) ;
#52796=EDGE_CURVE('',#40535,#39441,#33517,.T.) ;
#52797=EDGE_CURVE('',#39372,#40542,#33518,.T.) ;
#52798=EDGE_CURVE('',#40542,#40537,#33519,.T.) ;
#52799=EDGE_CURVE('',#40553,#39374,#33520,.T.) ;
#52800=EDGE_CURVE('',#40536,#39440,#33521,.T.) ;
#52801=EDGE_CURVE('',#40543,#40536,#33522,.T.) ;
#52802=EDGE_CURVE('',#39373,#40545,#33523,.T.) ;
#52803=EDGE_CURVE('',#40554,#39373,#33524,.T.) ;
#52804=EDGE_CURVE('',#40543,#39439,#33525,.T.) ;
#52805=EDGE_CURVE('',#40554,#40545,#33526,.T.) ;
#52806=EDGE_CURVE('',#40544,#39438,#33527,.T.) ;
#52807=EDGE_CURVE('',#40555,#40544,#33528,.T.) ;
#52808=EDGE_CURVE('',#40558,#40547,#33529,.T.) ;
#52809=EDGE_CURVE('',#40559,#40546,#33530,.T.) ;
#52810=EDGE_CURVE('',#39435,#40556,#33531,.T.) ;
#52811=EDGE_CURVE('',#39436,#40559,#33532,.T.) ;
#52812=EDGE_CURVE('',#40555,#39437,#33533,.T.) ;
#52813=EDGE_CURVE('',#39436,#40546,#33534,.T.) ;
#52814=EDGE_CURVE('',#40213,#40224,#33535,.T.) ;
#52815=EDGE_CURVE('',#40214,#40227,#33536,.T.) ;
#52816=EDGE_CURVE('',#40225,#40220,#33537,.T.) ;
#52817=EDGE_CURVE('',#40214,#40303,#33538,.T.) ;
#52818=EDGE_CURVE('',#40303,#40227,#33539,.T.) ;
#52819=EDGE_CURVE('',#40219,#40212,#33540,.T.) ;
#52820=EDGE_CURVE('',#40226,#40223,#33541,.T.) ;
#52821=EDGE_CURVE('',#40300,#40226,#33542,.T.) ;
#52822=EDGE_CURVE('',#40215,#40302,#33543,.T.) ;
#52823=EDGE_CURVE('',#40216,#40215,#33544,.T.) ;
#52824=EDGE_CURVE('',#40300,#40223,#33545,.T.) ;
#52825=EDGE_CURVE('',#40216,#40302,#33546,.T.) ;
#52826=EDGE_CURVE('',#40301,#40222,#33547,.T.) ;
#52827=EDGE_CURVE('',#40217,#40301,#33548,.T.) ;
#52828=EDGE_CURVE('',#40217,#40222,#33549,.T.) ;
#52829=EDGE_CURVE('',#40218,#40221,#33550,.T.) ;
#52830=EDGE_CURVE('',#40023,#41503,#33551,.T.) ;
#52831=EDGE_CURVE('',#40024,#39968,#33552,.T.) ;
#52832=EDGE_CURVE('',#40025,#39971,#33553,.T.) ;
#52833=EDGE_CURVE('',#39966,#40025,#33554,.T.) ;
#52834=EDGE_CURVE('',#39966,#39971,#33555,.T.) ;
#52835=EDGE_CURVE('',#39967,#39970,#33556,.T.) ;
#52836=EDGE_CURVE('',#40078,#39967,#33557,.T.) ;
#52837=EDGE_CURVE('',#40078,#39970,#33558,.T.) ;
#52838=EDGE_CURVE('',#40079,#39969,#33559,.T.) ;
#52839=EDGE_CURVE('',#40074,#41502,#33560,.T.) ;
#52840=EDGE_CURVE('',#40075,#41509,#33561,.T.) ;
#52841=EDGE_CURVE('',#40076,#39952,#33562,.T.) ;
#52842=EDGE_CURVE('',#40077,#39955,#33563,.T.) ;
#52843=EDGE_CURVE('',#39956,#40077,#33564,.T.) ;
#52844=EDGE_CURVE('',#39956,#39955,#33565,.T.) ;
#52845=EDGE_CURVE('',#39957,#39954,#33566,.T.) ;
#52846=EDGE_CURVE('',#40026,#39957,#33567,.T.) ;
#52847=EDGE_CURVE('',#40026,#39954,#33568,.T.) ;
#52848=EDGE_CURVE('',#40027,#39953,#33569,.T.) ;
#52849=EDGE_CURVE('',#40022,#41508,#33570,.T.) ;
#52850=EDGE_CURVE('',#39231,#41294,#33571,.T.) ;
#52851=EDGE_CURVE('',#41296,#39230,#33572,.T.) ;
#52852=EDGE_CURVE('',#41298,#39229,#33573,.T.) ;
#52853=EDGE_CURVE('',#39232,#41292,#33574,.T.) ;
#52854=EDGE_CURVE('',#41300,#39228,#33575,.T.) ;
#52855=EDGE_CURVE('',#39225,#41291,#33576,.T.) ;
#52856=EDGE_CURVE('',#41302,#39227,#33577,.T.) ;
#52857=EDGE_CURVE('',#39226,#41304,#33578,.T.) ;
#52858=EDGE_CURVE('',#40312,#40319,#33579,.T.) ;
#52859=EDGE_CURVE('',#40313,#40451,#33580,.T.) ;
#52860=EDGE_CURVE('',#40448,#40312,#33581,.T.) ;
#52861=EDGE_CURVE('',#40314,#40313,#33582,.T.) ;
#52862=EDGE_CURVE('',#40448,#40319,#33583,.T.) ;
#52863=EDGE_CURVE('',#40314,#40451,#33584,.T.) ;
#52864=EDGE_CURVE('',#40318,#40317,#33585,.T.) ;
#52865=EDGE_CURVE('',#40449,#40318,#33586,.T.) ;
#52866=EDGE_CURVE('',#40315,#40450,#33587,.T.) ;
#52867=EDGE_CURVE('',#40316,#40315,#33588,.T.) ;
#52868=EDGE_CURVE('',#40449,#40317,#33589,.T.) ;
#52869=EDGE_CURVE('',#40316,#40450,#33590,.T.) ;
#52870=EDGE_CURVE('',#39123,#41000,#33591,.T.) ;
#52871=EDGE_CURVE('',#41001,#39122,#33592,.T.) ;
#52872=EDGE_CURVE('',#40997,#39121,#33593,.T.) ;
#52873=EDGE_CURVE('',#41001,#40997,#33594,.T.) ;
#52874=EDGE_CURVE('',#40989,#41000,#33595,.T.) ;
#52875=EDGE_CURVE('',#39124,#40989,#33596,.T.) ;
#52876=EDGE_CURVE('',#40994,#39120,#33597,.T.) ;
#52877=EDGE_CURVE('',#40998,#40996,#33598,.T.) ;
#52878=EDGE_CURVE('',#40999,#41077,#33599,.T.) ;
#52879=EDGE_CURVE('',#41074,#40998,#33600,.T.) ;
#52880=EDGE_CURVE('',#40986,#40999,#33601,.T.) ;
#52881=EDGE_CURVE('',#39118,#40988,#33602,.T.) ;
#52882=EDGE_CURVE('',#39119,#40990,#33603,.T.) ;
#52883=EDGE_CURVE('',#40991,#39117,#33604,.T.) ;
#52884=EDGE_CURVE('',#40994,#40990,#33605,.T.) ;
#52885=EDGE_CURVE('',#41074,#40996,#33606,.T.) ;
#52886=EDGE_CURVE('',#40986,#41077,#33607,.T.) ;
#52887=EDGE_CURVE('',#40991,#40988,#33608,.T.) ;
#52888=EDGE_CURVE('',#40995,#40993,#33609,.T.) ;
#52889=EDGE_CURVE('',#41075,#40995,#33610,.T.) ;
#52890=EDGE_CURVE('',#40987,#41076,#33611,.T.) ;
#52891=EDGE_CURVE('',#40992,#40987,#33612,.T.) ;
#52892=EDGE_CURVE('',#41075,#40993,#33613,.T.) ;
#52893=EDGE_CURVE('',#40992,#41076,#33614,.T.) ;
#52894=EDGE_CURVE('',#41086,#41093,#33615,.T.) ;
#52895=EDGE_CURVE('',#41087,#41225,#33616,.T.) ;
#52896=EDGE_CURVE('',#41222,#41086,#33617,.T.) ;
#52897=EDGE_CURVE('',#41088,#41087,#33618,.T.) ;
#52898=EDGE_CURVE('',#41222,#41093,#33619,.T.) ;
#52899=EDGE_CURVE('',#41088,#41225,#33620,.T.) ;
#52900=EDGE_CURVE('',#41092,#41091,#33621,.T.) ;
#52901=EDGE_CURVE('',#41223,#41092,#33622,.T.) ;
#52902=EDGE_CURVE('',#41089,#41224,#33623,.T.) ;
#52903=EDGE_CURVE('',#41090,#41089,#33624,.T.) ;
#52904=EDGE_CURVE('',#41223,#41091,#33625,.T.) ;
#52905=EDGE_CURVE('',#41090,#41224,#33626,.T.) ;
#52906=EDGE_CURVE('',#41297,#41309,#33627,.T.) ;
#52907=EDGE_CURVE('',#41306,#41299,#33628,.T.) ;
#52908=EDGE_CURVE('',#41306,#41301,#33629,.T.) ;
#52909=EDGE_CURVE('',#41295,#41309,#33630,.T.) ;
#52910=EDGE_CURVE('',#41307,#41303,#33631,.T.) ;
#52911=EDGE_CURVE('',#41293,#41308,#33632,.T.) ;
#52912=EDGE_CURVE('',#41307,#41305,#33633,.T.) ;
#52913=EDGE_CURVE('',#41290,#41308,#33634,.T.) ;
#52914=EDGE_CURVE('',#40795,#40790,#33635,.T.) ;
#52915=EDGE_CURVE('',#40789,#40795,#33636,.T.) ;
#52916=EDGE_CURVE('',#40790,#40789,#33637,.T.) ;
#52917=EDGE_CURVE('',#40786,#40794,#33638,.T.) ;
#52918=EDGE_CURVE('',#40791,#40788,#33639,.T.) ;
#52919=EDGE_CURVE('',#40796,#40793,#33640,.T.) ;
#52920=EDGE_CURVE('',#40799,#40569,#33641,.T.) ;
#52921=EDGE_CURVE('',#40794,#40568,#33642,.T.) ;
#52922=EDGE_CURVE('',#40786,#40568,#33643,.T.) ;
#52923=EDGE_CURVE('',#40791,#39362,#33644,.T.) ;
#52924=EDGE_CURVE('',#39361,#40788,#33645,.T.) ;
#52925=EDGE_CURVE('',#40796,#40782,#33646,.T.) ;
#52926=EDGE_CURVE('',#40782,#40793,#33647,.T.) ;
#52927=EDGE_CURVE('',#40798,#39210,#33648,.T.) ;
#52928=EDGE_CURVE('',#39209,#40799,#33649,.T.) ;
#52929=EDGE_CURVE('',#40787,#40567,#33650,.T.) ;
#52930=EDGE_CURVE('',#39363,#40787,#33651,.T.) ;
#52931=EDGE_CURVE('',#40792,#39368,#33652,.T.) ;
#52932=EDGE_CURVE('',#40783,#40792,#33653,.T.) ;
#52933=EDGE_CURVE('',#40797,#40785,#33654,.T.) ;
#52934=EDGE_CURVE('',#40578,#40798,#33655,.T.) ;
#52935=EDGE_CURVE('',#40579,#40797,#33656,.T.) ;
#52936=EDGE_CURVE('',#39363,#40566,#33657,.T.) ;
#52937=EDGE_CURVE('',#40783,#39367,#33658,.T.) ;
#52938=EDGE_CURVE('',#40579,#40785,#33659,.T.) ;
#52939=EDGE_CURVE('',#40562,#40557,#33660,.T.) ;
#52940=EDGE_CURVE('',#40563,#40556,#33661,.T.) ;
#52941=EDGE_CURVE('',#39364,#40565,#33662,.T.) ;
#52942=EDGE_CURVE('',#40784,#39366,#33663,.T.) ;
#52943=EDGE_CURVE('',#40580,#40784,#33664,.T.) ;
#52944=EDGE_CURVE('',#40563,#39435,#33665,.T.) ;
#52945=EDGE_CURVE('',#39364,#40570,#33666,.T.) ;
#52946=EDGE_CURVE('',#40570,#40565,#33667,.T.) ;
#52947=EDGE_CURVE('',#40581,#39366,#33668,.T.) ;
#52948=EDGE_CURVE('',#40564,#39434,#33669,.T.) ;
#52949=EDGE_CURVE('',#40571,#40564,#33670,.T.) ;
#52950=EDGE_CURVE('',#39365,#40573,#33671,.T.) ;
#52951=EDGE_CURVE('',#40582,#39365,#33672,.T.) ;
#52952=EDGE_CURVE('',#40571,#39433,#33673,.T.) ;
#52953=EDGE_CURVE('',#40582,#40573,#33674,.T.) ;
#52954=EDGE_CURVE('',#40572,#39432,#33675,.T.) ;
#52955=EDGE_CURVE('',#40583,#40572,#33676,.T.) ;
#52956=EDGE_CURVE('',#40586,#40575,#33677,.T.) ;
#52957=EDGE_CURVE('',#40587,#40574,#33678,.T.) ;
#52958=EDGE_CURVE('',#39429,#40584,#33679,.T.) ;
#52959=EDGE_CURVE('',#39430,#40587,#33680,.T.) ;
#52960=EDGE_CURVE('',#40583,#39431,#33681,.T.) ;
#52961=EDGE_CURVE('',#39430,#40574,#33682,.T.) ;
#52962=EDGE_CURVE('',#40197,#40208,#33683,.T.) ;
#52963=EDGE_CURVE('',#40198,#40211,#33684,.T.) ;
#52964=EDGE_CURVE('',#40209,#40204,#33685,.T.) ;
#52965=EDGE_CURVE('',#40198,#40323,#33686,.T.) ;
#52966=EDGE_CURVE('',#40323,#40211,#33687,.T.) ;
#52967=EDGE_CURVE('',#40203,#40196,#33688,.T.) ;
#52968=EDGE_CURVE('',#40210,#40207,#33689,.T.) ;
#52969=EDGE_CURVE('',#40320,#40210,#33690,.T.) ;
#52970=EDGE_CURVE('',#40199,#40322,#33691,.T.) ;
#52971=EDGE_CURVE('',#40200,#40199,#33692,.T.) ;
#52972=EDGE_CURVE('',#40320,#40207,#33693,.T.) ;
#52973=EDGE_CURVE('',#40200,#40322,#33694,.T.) ;
#52974=EDGE_CURVE('',#40321,#40206,#33695,.T.) ;
#52975=EDGE_CURVE('',#40201,#40321,#33696,.T.) ;
#52976=EDGE_CURVE('',#40201,#40206,#33697,.T.) ;
#52977=EDGE_CURVE('',#40202,#40205,#33698,.T.) ;
#52978=EDGE_CURVE('',#40029,#41511,#33699,.T.) ;
#52979=EDGE_CURVE('',#40030,#39948,#33700,.T.) ;
#52980=EDGE_CURVE('',#40031,#39951,#33701,.T.) ;
#52981=EDGE_CURVE('',#39946,#40031,#33702,.T.) ;
#52982=EDGE_CURVE('',#39946,#39951,#33703,.T.) ;
#52983=EDGE_CURVE('',#39947,#39950,#33704,.T.) ;
#52984=EDGE_CURVE('',#40084,#39947,#33705,.T.) ;
#52985=EDGE_CURVE('',#40084,#39950,#33706,.T.) ;
#52986=EDGE_CURVE('',#40085,#39949,#33707,.T.) ;
#52987=EDGE_CURVE('',#40080,#41510,#33708,.T.) ;
#52988=EDGE_CURVE('',#40081,#41517,#33709,.T.) ;
#52989=EDGE_CURVE('',#40082,#39932,#33710,.T.) ;
#52990=EDGE_CURVE('',#40083,#39935,#33711,.T.) ;
#52991=EDGE_CURVE('',#39936,#40083,#33712,.T.) ;
#52992=EDGE_CURVE('',#39936,#39935,#33713,.T.) ;
#52993=EDGE_CURVE('',#39937,#39934,#33714,.T.) ;
#52994=EDGE_CURVE('',#40032,#39937,#33715,.T.) ;
#52995=EDGE_CURVE('',#40032,#39934,#33716,.T.) ;
#52996=EDGE_CURVE('',#40033,#39933,#33717,.T.) ;
#52997=EDGE_CURVE('',#40028,#41516,#33718,.T.) ;
#52998=EDGE_CURVE('',#39219,#41314,#33719,.T.) ;
#52999=EDGE_CURVE('',#41316,#39218,#33720,.T.) ;
#53000=EDGE_CURVE('',#41318,#39217,#33721,.T.) ;
#53001=EDGE_CURVE('',#39220,#41312,#33722,.T.) ;
#53002=EDGE_CURVE('',#41320,#39216,#33723,.T.) ;
#53003=EDGE_CURVE('',#39213,#41311,#33724,.T.) ;
#53004=EDGE_CURVE('',#41322,#39215,#33725,.T.) ;
#53005=EDGE_CURVE('',#39214,#41324,#33726,.T.) ;
#53006=EDGE_CURVE('',#40332,#40339,#33727,.T.) ;
#53007=EDGE_CURVE('',#40333,#40455,#33728,.T.) ;
#53008=EDGE_CURVE('',#40452,#40332,#33729,.T.) ;
#53009=EDGE_CURVE('',#40334,#40333,#33730,.T.) ;
#53010=EDGE_CURVE('',#40452,#40339,#33731,.T.) ;
#53011=EDGE_CURVE('',#40334,#40455,#33732,.T.) ;
#53012=EDGE_CURVE('',#40338,#40337,#33733,.T.) ;
#53013=EDGE_CURVE('',#40453,#40338,#33734,.T.) ;
#53014=EDGE_CURVE('',#40335,#40454,#33735,.T.) ;
#53015=EDGE_CURVE('',#40336,#40335,#33736,.T.) ;
#53016=EDGE_CURVE('',#40453,#40337,#33737,.T.) ;
#53017=EDGE_CURVE('',#40336,#40454,#33738,.T.) ;
#53018=EDGE_CURVE('',#39091,#40984,#33739,.T.) ;
#53019=EDGE_CURVE('',#40985,#39090,#33740,.T.) ;
#53020=EDGE_CURVE('',#40981,#39089,#33741,.T.) ;
#53021=EDGE_CURVE('',#40985,#40981,#33742,.T.) ;
#53022=EDGE_CURVE('',#40973,#40984,#33743,.T.) ;
#53023=EDGE_CURVE('',#39092,#40973,#33744,.T.) ;
#53024=EDGE_CURVE('',#40978,#39088,#33745,.T.) ;
#53025=EDGE_CURVE('',#40982,#40980,#33746,.T.) ;
#53026=EDGE_CURVE('',#40983,#41097,#33747,.T.) ;
#53027=EDGE_CURVE('',#41094,#40982,#33748,.T.) ;
#53028=EDGE_CURVE('',#40970,#40983,#33749,.T.) ;
#53029=EDGE_CURVE('',#39086,#40972,#33750,.T.) ;
#53030=EDGE_CURVE('',#39087,#40974,#33751,.T.) ;
#53031=EDGE_CURVE('',#40975,#39085,#33752,.T.) ;
#53032=EDGE_CURVE('',#40978,#40974,#33753,.T.) ;
#53033=EDGE_CURVE('',#41094,#40980,#33754,.T.) ;
#53034=EDGE_CURVE('',#40970,#41097,#33755,.T.) ;
#53035=EDGE_CURVE('',#40975,#40972,#33756,.T.) ;
#53036=EDGE_CURVE('',#40979,#40977,#33757,.T.) ;
#53037=EDGE_CURVE('',#41095,#40979,#33758,.T.) ;
#53038=EDGE_CURVE('',#40971,#41096,#33759,.T.) ;
#53039=EDGE_CURVE('',#40976,#40971,#33760,.T.) ;
#53040=EDGE_CURVE('',#41095,#40977,#33761,.T.) ;
#53041=EDGE_CURVE('',#40976,#41096,#33762,.T.) ;
#53042=EDGE_CURVE('',#41106,#41113,#33763,.T.) ;
#53043=EDGE_CURVE('',#41107,#41229,#33764,.T.) ;
#53044=EDGE_CURVE('',#41226,#41106,#33765,.T.) ;
#53045=EDGE_CURVE('',#41108,#41107,#33766,.T.) ;
#53046=EDGE_CURVE('',#41226,#41113,#33767,.T.) ;
#53047=EDGE_CURVE('',#41108,#41229,#33768,.T.) ;
#53048=EDGE_CURVE('',#41112,#41111,#33769,.T.) ;
#53049=EDGE_CURVE('',#41227,#41112,#33770,.T.) ;
#53050=EDGE_CURVE('',#41109,#41228,#33771,.T.) ;
#53051=EDGE_CURVE('',#41110,#41109,#33772,.T.) ;
#53052=EDGE_CURVE('',#41227,#41111,#33773,.T.) ;
#53053=EDGE_CURVE('',#41110,#41228,#33774,.T.) ;
#53054=EDGE_CURVE('',#41317,#41329,#33775,.T.) ;
#53055=EDGE_CURVE('',#41326,#41319,#33776,.T.) ;
#53056=EDGE_CURVE('',#41326,#41321,#33777,.T.) ;
#53057=EDGE_CURVE('',#41315,#41329,#33778,.T.) ;
#53058=EDGE_CURVE('',#41327,#41323,#33779,.T.) ;
#53059=EDGE_CURVE('',#41313,#41328,#33780,.T.) ;
#53060=EDGE_CURVE('',#41327,#41325,#33781,.T.) ;
#53061=EDGE_CURVE('',#41310,#41328,#33782,.T.) ;
#53062=EDGE_CURVE('',#40813,#40808,#33783,.T.) ;
#53063=EDGE_CURVE('',#40807,#40813,#33784,.T.) ;
#53064=EDGE_CURVE('',#40808,#40807,#33785,.T.) ;
#53065=EDGE_CURVE('',#40804,#40812,#33786,.T.) ;
#53066=EDGE_CURVE('',#40809,#40806,#33787,.T.) ;
#53067=EDGE_CURVE('',#40814,#40811,#33788,.T.) ;
#53068=EDGE_CURVE('',#40817,#40597,#33789,.T.) ;
#53069=EDGE_CURVE('',#40812,#40596,#33790,.T.) ;
#53070=EDGE_CURVE('',#40804,#40596,#33791,.T.) ;
#53071=EDGE_CURVE('',#40809,#39354,#33792,.T.) ;
#53072=EDGE_CURVE('',#39353,#40806,#33793,.T.) ;
#53073=EDGE_CURVE('',#40814,#40800,#33794,.T.) ;
#53074=EDGE_CURVE('',#40800,#40811,#33795,.T.) ;
#53075=EDGE_CURVE('',#40816,#39198,#33796,.T.) ;
#53076=EDGE_CURVE('',#39197,#40817,#33797,.T.) ;
#53077=EDGE_CURVE('',#40805,#40595,#33798,.T.) ;
#53078=EDGE_CURVE('',#39355,#40805,#33799,.T.) ;
#53079=EDGE_CURVE('',#40810,#39360,#33800,.T.) ;
#53080=EDGE_CURVE('',#40801,#40810,#33801,.T.) ;
#53081=EDGE_CURVE('',#40815,#40803,#33802,.T.) ;
#53082=EDGE_CURVE('',#40606,#40816,#33803,.T.) ;
#53083=EDGE_CURVE('',#40607,#40815,#33804,.T.) ;
#53084=EDGE_CURVE('',#39355,#40594,#33805,.T.) ;
#53085=EDGE_CURVE('',#40801,#39359,#33806,.T.) ;
#53086=EDGE_CURVE('',#40607,#40803,#33807,.T.) ;
#53087=EDGE_CURVE('',#40590,#40585,#33808,.T.) ;
#53088=EDGE_CURVE('',#40591,#40584,#33809,.T.) ;
#53089=EDGE_CURVE('',#39356,#40593,#33810,.T.) ;
#53090=EDGE_CURVE('',#40802,#39358,#33811,.T.) ;
#53091=EDGE_CURVE('',#40608,#40802,#33812,.T.) ;
#53092=EDGE_CURVE('',#40591,#39429,#33813,.T.) ;
#53093=EDGE_CURVE('',#39356,#40598,#33814,.T.) ;
#53094=EDGE_CURVE('',#40598,#40593,#33815,.T.) ;
#53095=EDGE_CURVE('',#40609,#39358,#33816,.T.) ;
#53096=EDGE_CURVE('',#40592,#39428,#33817,.T.) ;
#53097=EDGE_CURVE('',#40599,#40592,#33818,.T.) ;
#53098=EDGE_CURVE('',#39357,#40601,#33819,.T.) ;
#53099=EDGE_CURVE('',#40610,#39357,#33820,.T.) ;
#53100=EDGE_CURVE('',#40599,#39427,#33821,.T.) ;
#53101=EDGE_CURVE('',#40610,#40601,#33822,.T.) ;
#53102=EDGE_CURVE('',#40600,#39426,#33823,.T.) ;
#53103=EDGE_CURVE('',#40611,#40600,#33824,.T.) ;
#53104=EDGE_CURVE('',#40614,#40603,#33825,.T.) ;
#53105=EDGE_CURVE('',#40615,#40602,#33826,.T.) ;
#53106=EDGE_CURVE('',#39423,#40612,#33827,.T.) ;
#53107=EDGE_CURVE('',#39424,#40615,#33828,.T.) ;
#53108=EDGE_CURVE('',#40611,#39425,#33829,.T.) ;
#53109=EDGE_CURVE('',#39424,#40602,#33830,.T.) ;
#53110=EDGE_CURVE('',#40181,#40192,#33831,.T.) ;
#53111=EDGE_CURVE('',#40182,#40195,#33832,.T.) ;
#53112=EDGE_CURVE('',#40193,#40188,#33833,.T.) ;
#53113=EDGE_CURVE('',#40182,#40343,#33834,.T.) ;
#53114=EDGE_CURVE('',#40343,#40195,#33835,.T.) ;
#53115=EDGE_CURVE('',#40187,#40180,#33836,.T.) ;
#53116=EDGE_CURVE('',#40194,#40191,#33837,.T.) ;
#53117=EDGE_CURVE('',#40340,#40194,#33838,.T.) ;
#53118=EDGE_CURVE('',#40183,#40342,#33839,.T.) ;
#53119=EDGE_CURVE('',#40184,#40183,#33840,.T.) ;
#53120=EDGE_CURVE('',#40340,#40191,#33841,.T.) ;
#53121=EDGE_CURVE('',#40184,#40342,#33842,.T.) ;
#53122=EDGE_CURVE('',#40341,#40190,#33843,.T.) ;
#53123=EDGE_CURVE('',#40185,#40341,#33844,.T.) ;
#53124=EDGE_CURVE('',#40185,#40190,#33845,.T.) ;
#53125=EDGE_CURVE('',#40186,#40189,#33846,.T.) ;
#53126=EDGE_CURVE('',#40035,#41519,#33847,.T.) ;
#53127=EDGE_CURVE('',#40036,#39928,#33848,.T.) ;
#53128=EDGE_CURVE('',#40037,#39931,#33849,.T.) ;
#53129=EDGE_CURVE('',#39926,#40037,#33850,.T.) ;
#53130=EDGE_CURVE('',#39926,#39931,#33851,.T.) ;
#53131=EDGE_CURVE('',#39927,#39930,#33852,.T.) ;
#53132=EDGE_CURVE('',#40090,#39927,#33853,.T.) ;
#53133=EDGE_CURVE('',#40090,#39930,#33854,.T.) ;
#53134=EDGE_CURVE('',#40091,#39929,#33855,.T.) ;
#53135=EDGE_CURVE('',#40086,#41518,#33856,.T.) ;
#53136=EDGE_CURVE('',#40087,#41525,#33857,.T.) ;
#53137=EDGE_CURVE('',#40088,#39912,#33858,.T.) ;
#53138=EDGE_CURVE('',#40089,#39915,#33859,.T.) ;
#53139=EDGE_CURVE('',#39916,#40089,#33860,.T.) ;
#53140=EDGE_CURVE('',#39916,#39915,#33861,.T.) ;
#53141=EDGE_CURVE('',#39917,#39914,#33862,.T.) ;
#53142=EDGE_CURVE('',#40038,#39917,#33863,.T.) ;
#53143=EDGE_CURVE('',#40038,#39914,#33864,.T.) ;
#53144=EDGE_CURVE('',#40039,#39913,#33865,.T.) ;
#53145=EDGE_CURVE('',#40034,#41524,#33866,.T.) ;
#53146=EDGE_CURVE('',#39207,#41334,#33867,.T.) ;
#53147=EDGE_CURVE('',#41336,#39206,#33868,.T.) ;
#53148=EDGE_CURVE('',#41338,#39205,#33869,.T.) ;
#53149=EDGE_CURVE('',#39208,#41332,#33870,.T.) ;
#53150=EDGE_CURVE('',#41340,#39204,#33871,.T.) ;
#53151=EDGE_CURVE('',#39201,#41331,#33872,.T.) ;
#53152=EDGE_CURVE('',#41342,#39203,#33873,.T.) ;
#53153=EDGE_CURVE('',#39202,#41344,#33874,.T.) ;
#53154=EDGE_CURVE('',#40352,#40359,#33875,.T.) ;
#53155=EDGE_CURVE('',#40353,#40459,#33876,.T.) ;
#53156=EDGE_CURVE('',#40456,#40352,#33877,.T.) ;
#53157=EDGE_CURVE('',#40354,#40353,#33878,.T.) ;
#53158=EDGE_CURVE('',#40456,#40359,#33879,.T.) ;
#53159=EDGE_CURVE('',#40354,#40459,#33880,.T.) ;
#53160=EDGE_CURVE('',#40358,#40357,#33881,.T.) ;
#53161=EDGE_CURVE('',#40457,#40358,#33882,.T.) ;
#53162=EDGE_CURVE('',#40355,#40458,#33883,.T.) ;
#53163=EDGE_CURVE('',#40356,#40355,#33884,.T.) ;
#53164=EDGE_CURVE('',#40457,#40357,#33885,.T.) ;
#53165=EDGE_CURVE('',#40356,#40458,#33886,.T.) ;
#53166=EDGE_CURVE('',#39131,#40968,#33887,.T.) ;
#53167=EDGE_CURVE('',#40969,#39130,#33888,.T.) ;
#53168=EDGE_CURVE('',#40965,#39129,#33889,.T.) ;
#53169=EDGE_CURVE('',#40969,#40965,#33890,.T.) ;
#53170=EDGE_CURVE('',#40957,#40968,#33891,.T.) ;
#53171=EDGE_CURVE('',#39132,#40957,#33892,.T.) ;
#53172=EDGE_CURVE('',#40962,#39128,#33893,.T.) ;
#53173=EDGE_CURVE('',#40966,#40964,#33894,.T.) ;
#53174=EDGE_CURVE('',#40967,#41117,#33895,.T.) ;
#53175=EDGE_CURVE('',#41114,#40966,#33896,.T.) ;
#53176=EDGE_CURVE('',#40954,#40967,#33897,.T.) ;
#53177=EDGE_CURVE('',#39126,#40956,#33898,.T.) ;
#53178=EDGE_CURVE('',#39127,#40958,#33899,.T.) ;
#53179=EDGE_CURVE('',#40959,#39125,#33900,.T.) ;
#53180=EDGE_CURVE('',#40962,#40958,#33901,.T.) ;
#53181=EDGE_CURVE('',#41114,#40964,#33902,.T.) ;
#53182=EDGE_CURVE('',#40954,#41117,#33903,.T.) ;
#53183=EDGE_CURVE('',#40959,#40956,#33904,.T.) ;
#53184=EDGE_CURVE('',#40963,#40961,#33905,.T.) ;
#53185=EDGE_CURVE('',#41115,#40963,#33906,.T.) ;
#53186=EDGE_CURVE('',#40955,#41116,#33907,.T.) ;
#53187=EDGE_CURVE('',#40960,#40955,#33908,.T.) ;
#53188=EDGE_CURVE('',#41115,#40961,#33909,.T.) ;
#53189=EDGE_CURVE('',#40960,#41116,#33910,.T.) ;
#53190=EDGE_CURVE('',#41126,#41133,#33911,.T.) ;
#53191=EDGE_CURVE('',#41127,#41233,#33912,.T.) ;
#53192=EDGE_CURVE('',#41230,#41126,#33913,.T.) ;
#53193=EDGE_CURVE('',#41128,#41127,#33914,.T.) ;
#53194=EDGE_CURVE('',#41230,#41133,#33915,.T.) ;
#53195=EDGE_CURVE('',#41128,#41233,#33916,.T.) ;
#53196=EDGE_CURVE('',#41132,#41131,#33917,.T.) ;
#53197=EDGE_CURVE('',#41231,#41132,#33918,.T.) ;
#53198=EDGE_CURVE('',#41129,#41232,#33919,.T.) ;
#53199=EDGE_CURVE('',#41130,#41129,#33920,.T.) ;
#53200=EDGE_CURVE('',#41231,#41131,#33921,.T.) ;
#53201=EDGE_CURVE('',#41130,#41232,#33922,.T.) ;
#53202=EDGE_CURVE('',#41337,#41349,#33923,.T.) ;
#53203=EDGE_CURVE('',#41346,#41339,#33924,.T.) ;
#53204=EDGE_CURVE('',#41346,#41341,#33925,.T.) ;
#53205=EDGE_CURVE('',#41335,#41349,#33926,.T.) ;
#53206=EDGE_CURVE('',#41347,#41343,#33927,.T.) ;
#53207=EDGE_CURVE('',#41333,#41348,#33928,.T.) ;
#53208=EDGE_CURVE('',#41347,#41345,#33929,.T.) ;
#53209=EDGE_CURVE('',#41330,#41348,#33930,.T.) ;
#53210=EDGE_CURVE('',#40831,#40826,#33931,.T.) ;
#53211=EDGE_CURVE('',#40825,#40831,#33932,.T.) ;
#53212=EDGE_CURVE('',#40826,#40825,#33933,.T.) ;
#53213=EDGE_CURVE('',#40822,#40830,#33934,.T.) ;
#53214=EDGE_CURVE('',#40827,#40824,#33935,.T.) ;
#53215=EDGE_CURVE('',#40832,#40829,#33936,.T.) ;
#53216=EDGE_CURVE('',#40835,#40625,#33937,.T.) ;
#53217=EDGE_CURVE('',#40830,#40624,#33938,.T.) ;
#53218=EDGE_CURVE('',#40822,#40624,#33939,.T.) ;
#53219=EDGE_CURVE('',#40827,#39346,#33940,.T.) ;
#53220=EDGE_CURVE('',#39345,#40824,#33941,.T.) ;
#53221=EDGE_CURVE('',#40832,#40818,#33942,.T.) ;
#53222=EDGE_CURVE('',#40818,#40829,#33943,.T.) ;
#53223=EDGE_CURVE('',#40834,#39186,#33944,.T.) ;
#53224=EDGE_CURVE('',#39185,#40835,#33945,.T.) ;
#53225=EDGE_CURVE('',#40823,#40623,#33946,.T.) ;
#53226=EDGE_CURVE('',#39347,#40823,#33947,.T.) ;
#53227=EDGE_CURVE('',#40828,#39352,#33948,.T.) ;
#53228=EDGE_CURVE('',#40819,#40828,#33949,.T.) ;
#53229=EDGE_CURVE('',#40833,#40821,#33950,.T.) ;
#53230=EDGE_CURVE('',#40634,#40834,#33951,.T.) ;
#53231=EDGE_CURVE('',#40635,#40833,#33952,.T.) ;
#53232=EDGE_CURVE('',#39347,#40622,#33953,.T.) ;
#53233=EDGE_CURVE('',#40819,#39351,#33954,.T.) ;
#53234=EDGE_CURVE('',#40635,#40821,#33955,.T.) ;
#53235=EDGE_CURVE('',#40618,#40613,#33956,.T.) ;
#53236=EDGE_CURVE('',#40619,#40612,#33957,.T.) ;
#53237=EDGE_CURVE('',#39348,#40621,#33958,.T.) ;
#53238=EDGE_CURVE('',#40820,#39350,#33959,.T.) ;
#53239=EDGE_CURVE('',#40636,#40820,#33960,.T.) ;
#53240=EDGE_CURVE('',#40619,#39423,#33961,.T.) ;
#53241=EDGE_CURVE('',#39348,#40626,#33962,.T.) ;
#53242=EDGE_CURVE('',#40626,#40621,#33963,.T.) ;
#53243=EDGE_CURVE('',#40637,#39350,#33964,.T.) ;
#53244=EDGE_CURVE('',#40620,#39422,#33965,.T.) ;
#53245=EDGE_CURVE('',#40627,#40620,#33966,.T.) ;
#53246=EDGE_CURVE('',#39349,#40629,#33967,.T.) ;
#53247=EDGE_CURVE('',#40638,#39349,#33968,.T.) ;
#53248=EDGE_CURVE('',#40627,#39421,#33969,.T.) ;
#53249=EDGE_CURVE('',#40638,#40629,#33970,.T.) ;
#53250=EDGE_CURVE('',#40628,#39420,#33971,.T.) ;
#53251=EDGE_CURVE('',#40639,#40628,#33972,.T.) ;
#53252=EDGE_CURVE('',#40642,#40631,#33973,.T.) ;
#53253=EDGE_CURVE('',#40643,#40630,#33974,.T.) ;
#53254=EDGE_CURVE('',#39417,#40640,#33975,.T.) ;
#53255=EDGE_CURVE('',#39418,#40643,#33976,.T.) ;
#53256=EDGE_CURVE('',#40639,#39419,#33977,.T.) ;
#53257=EDGE_CURVE('',#39418,#40630,#33978,.T.) ;
#53258=EDGE_CURVE('',#40165,#40176,#33979,.T.) ;
#53259=EDGE_CURVE('',#40166,#40179,#33980,.T.) ;
#53260=EDGE_CURVE('',#40177,#40172,#33981,.T.) ;
#53261=EDGE_CURVE('',#40166,#40363,#33982,.T.) ;
#53262=EDGE_CURVE('',#40363,#40179,#33983,.T.) ;
#53263=EDGE_CURVE('',#40171,#40164,#33984,.T.) ;
#53264=EDGE_CURVE('',#40178,#40175,#33985,.T.) ;
#53265=EDGE_CURVE('',#40360,#40178,#33986,.T.) ;
#53266=EDGE_CURVE('',#40167,#40362,#33987,.T.) ;
#53267=EDGE_CURVE('',#40168,#40167,#33988,.T.) ;
#53268=EDGE_CURVE('',#40360,#40175,#33989,.T.) ;
#53269=EDGE_CURVE('',#40168,#40362,#33990,.T.) ;
#53270=EDGE_CURVE('',#40361,#40174,#33991,.T.) ;
#53271=EDGE_CURVE('',#40169,#40361,#33992,.T.) ;
#53272=EDGE_CURVE('',#40169,#40174,#33993,.T.) ;
#53273=EDGE_CURVE('',#40170,#40173,#33994,.T.) ;
#53274=EDGE_CURVE('',#40041,#41527,#33995,.T.) ;
#53275=EDGE_CURVE('',#40042,#39908,#33996,.T.) ;
#53276=EDGE_CURVE('',#40043,#39911,#33997,.T.) ;
#53277=EDGE_CURVE('',#39906,#40043,#33998,.T.) ;
#53278=EDGE_CURVE('',#39906,#39911,#33999,.T.) ;
#53279=EDGE_CURVE('',#39907,#39910,#34000,.T.) ;
#53280=EDGE_CURVE('',#40096,#39907,#34001,.T.) ;
#53281=EDGE_CURVE('',#40096,#39910,#34002,.T.) ;
#53282=EDGE_CURVE('',#40097,#39909,#34003,.T.) ;
#53283=EDGE_CURVE('',#40092,#41526,#34004,.T.) ;
#53284=EDGE_CURVE('',#40093,#41533,#34005,.T.) ;
#53285=EDGE_CURVE('',#40094,#39892,#34006,.T.) ;
#53286=EDGE_CURVE('',#40095,#39895,#34007,.T.) ;
#53287=EDGE_CURVE('',#39896,#40095,#34008,.T.) ;
#53288=EDGE_CURVE('',#39896,#39895,#34009,.T.) ;
#53289=EDGE_CURVE('',#39897,#39894,#34010,.T.) ;
#53290=EDGE_CURVE('',#40044,#39897,#34011,.T.) ;
#53291=EDGE_CURVE('',#40044,#39894,#34012,.T.) ;
#53292=EDGE_CURVE('',#40045,#39893,#34013,.T.) ;
#53293=EDGE_CURVE('',#40040,#41532,#34014,.T.) ;
#53294=EDGE_CURVE('',#39195,#41354,#34015,.T.) ;
#53295=EDGE_CURVE('',#41356,#39194,#34016,.T.) ;
#53296=EDGE_CURVE('',#41358,#39193,#34017,.T.) ;
#53297=EDGE_CURVE('',#39196,#41352,#34018,.T.) ;
#53298=EDGE_CURVE('',#41360,#39192,#34019,.T.) ;
#53299=EDGE_CURVE('',#39189,#41351,#34020,.T.) ;
#53300=EDGE_CURVE('',#41362,#39191,#34021,.T.) ;
#53301=EDGE_CURVE('',#39190,#41364,#34022,.T.) ;
#53302=EDGE_CURVE('',#40372,#40379,#34023,.T.) ;
#53303=EDGE_CURVE('',#40373,#40463,#34024,.T.) ;
#53304=EDGE_CURVE('',#40460,#40372,#34025,.T.) ;
#53305=EDGE_CURVE('',#40374,#40373,#34026,.T.) ;
#53306=EDGE_CURVE('',#40460,#40379,#34027,.T.) ;
#53307=EDGE_CURVE('',#40374,#40463,#34028,.T.) ;
#53308=EDGE_CURVE('',#40378,#40377,#34029,.T.) ;
#53309=EDGE_CURVE('',#40461,#40378,#34030,.T.) ;
#53310=EDGE_CURVE('',#40375,#40462,#34031,.T.) ;
#53311=EDGE_CURVE('',#40376,#40375,#34032,.T.) ;
#53312=EDGE_CURVE('',#40461,#40377,#34033,.T.) ;
#53313=EDGE_CURVE('',#40376,#40462,#34034,.T.) ;
#53314=EDGE_CURVE('',#39083,#40952,#34035,.T.) ;
#53315=EDGE_CURVE('',#40953,#39082,#34036,.T.) ;
#53316=EDGE_CURVE('',#40949,#39081,#34037,.T.) ;
#53317=EDGE_CURVE('',#40953,#40949,#34038,.T.) ;
#53318=EDGE_CURVE('',#40941,#40952,#34039,.T.) ;
#53319=EDGE_CURVE('',#39084,#40941,#34040,.T.) ;
#53320=EDGE_CURVE('',#40946,#39080,#34041,.T.) ;
#53321=EDGE_CURVE('',#40950,#40948,#34042,.T.) ;
#53322=EDGE_CURVE('',#40951,#41137,#34043,.T.) ;
#53323=EDGE_CURVE('',#41134,#40950,#34044,.T.) ;
#53324=EDGE_CURVE('',#40938,#40951,#34045,.T.) ;
#53325=EDGE_CURVE('',#39078,#40940,#34046,.T.) ;
#53326=EDGE_CURVE('',#39079,#40942,#34047,.T.) ;
#53327=EDGE_CURVE('',#40943,#39077,#34048,.T.) ;
#53328=EDGE_CURVE('',#40946,#40942,#34049,.T.) ;
#53329=EDGE_CURVE('',#41134,#40948,#34050,.T.) ;
#53330=EDGE_CURVE('',#40938,#41137,#34051,.T.) ;
#53331=EDGE_CURVE('',#40943,#40940,#34052,.T.) ;
#53332=EDGE_CURVE('',#40947,#40945,#34053,.T.) ;
#53333=EDGE_CURVE('',#41135,#40947,#34054,.T.) ;
#53334=EDGE_CURVE('',#40939,#41136,#34055,.T.) ;
#53335=EDGE_CURVE('',#40944,#40939,#34056,.T.) ;
#53336=EDGE_CURVE('',#41135,#40945,#34057,.T.) ;
#53337=EDGE_CURVE('',#40944,#41136,#34058,.T.) ;
#53338=EDGE_CURVE('',#41146,#41153,#34059,.T.) ;
#53339=EDGE_CURVE('',#41147,#41237,#34060,.T.) ;
#53340=EDGE_CURVE('',#41234,#41146,#34061,.T.) ;
#53341=EDGE_CURVE('',#41148,#41147,#34062,.T.) ;
#53342=EDGE_CURVE('',#41234,#41153,#34063,.T.) ;
#53343=EDGE_CURVE('',#41148,#41237,#34064,.T.) ;
#53344=EDGE_CURVE('',#41152,#41151,#34065,.T.) ;
#53345=EDGE_CURVE('',#41235,#41152,#34066,.T.) ;
#53346=EDGE_CURVE('',#41149,#41236,#34067,.T.) ;
#53347=EDGE_CURVE('',#41150,#41149,#34068,.T.) ;
#53348=EDGE_CURVE('',#41235,#41151,#34069,.T.) ;
#53349=EDGE_CURVE('',#41150,#41236,#34070,.T.) ;
#53350=EDGE_CURVE('',#41357,#41369,#34071,.T.) ;
#53351=EDGE_CURVE('',#41366,#41359,#34072,.T.) ;
#53352=EDGE_CURVE('',#41366,#41361,#34073,.T.) ;
#53353=EDGE_CURVE('',#41355,#41369,#34074,.T.) ;
#53354=EDGE_CURVE('',#41367,#41363,#34075,.T.) ;
#53355=EDGE_CURVE('',#41353,#41368,#34076,.T.) ;
#53356=EDGE_CURVE('',#41367,#41365,#34077,.T.) ;
#53357=EDGE_CURVE('',#41350,#41368,#34078,.T.) ;
#53358=EDGE_CURVE('',#40849,#40844,#34079,.T.) ;
#53359=EDGE_CURVE('',#40843,#40849,#34080,.T.) ;
#53360=EDGE_CURVE('',#40844,#40843,#34081,.T.) ;
#53361=EDGE_CURVE('',#40840,#40848,#34082,.T.) ;
#53362=EDGE_CURVE('',#40845,#40842,#34083,.T.) ;
#53363=EDGE_CURVE('',#40850,#40847,#34084,.T.) ;
#53364=EDGE_CURVE('',#40853,#40653,#34085,.T.) ;
#53365=EDGE_CURVE('',#40848,#40652,#34086,.T.) ;
#53366=EDGE_CURVE('',#40840,#40652,#34087,.T.) ;
#53367=EDGE_CURVE('',#40845,#39338,#34088,.T.) ;
#53368=EDGE_CURVE('',#39337,#40842,#34089,.T.) ;
#53369=EDGE_CURVE('',#40850,#40836,#34090,.T.) ;
#53370=EDGE_CURVE('',#40836,#40847,#34091,.T.) ;
#53371=EDGE_CURVE('',#40852,#39174,#34092,.T.) ;
#53372=EDGE_CURVE('',#39173,#40853,#34093,.T.) ;
#53373=EDGE_CURVE('',#40841,#40651,#34094,.T.) ;
#53374=EDGE_CURVE('',#39339,#40841,#34095,.T.) ;
#53375=EDGE_CURVE('',#40846,#39344,#34096,.T.) ;
#53376=EDGE_CURVE('',#40837,#40846,#34097,.T.) ;
#53377=EDGE_CURVE('',#40851,#40839,#34098,.T.) ;
#53378=EDGE_CURVE('',#40662,#40852,#34099,.T.) ;
#53379=EDGE_CURVE('',#40663,#40851,#34100,.T.) ;
#53380=EDGE_CURVE('',#39339,#40650,#34101,.T.) ;
#53381=EDGE_CURVE('',#40837,#39343,#34102,.T.) ;
#53382=EDGE_CURVE('',#40663,#40839,#34103,.T.) ;
#53383=EDGE_CURVE('',#40646,#40641,#34104,.T.) ;
#53384=EDGE_CURVE('',#40647,#40640,#34105,.T.) ;
#53385=EDGE_CURVE('',#39340,#40649,#34106,.T.) ;
#53386=EDGE_CURVE('',#40838,#39342,#34107,.T.) ;
#53387=EDGE_CURVE('',#40664,#40838,#34108,.T.) ;
#53388=EDGE_CURVE('',#40647,#39417,#34109,.T.) ;
#53389=EDGE_CURVE('',#39340,#40654,#34110,.T.) ;
#53390=EDGE_CURVE('',#40654,#40649,#34111,.T.) ;
#53391=EDGE_CURVE('',#40665,#39342,#34112,.T.) ;
#53392=EDGE_CURVE('',#40648,#39416,#34113,.T.) ;
#53393=EDGE_CURVE('',#40655,#40648,#34114,.T.) ;
#53394=EDGE_CURVE('',#39341,#40657,#34115,.T.) ;
#53395=EDGE_CURVE('',#40666,#39341,#34116,.T.) ;
#53396=EDGE_CURVE('',#40655,#39415,#34117,.T.) ;
#53397=EDGE_CURVE('',#40666,#40657,#34118,.T.) ;
#53398=EDGE_CURVE('',#40656,#39414,#34119,.T.) ;
#53399=EDGE_CURVE('',#40667,#40656,#34120,.T.) ;
#53400=EDGE_CURVE('',#40670,#40659,#34121,.T.) ;
#53401=EDGE_CURVE('',#40671,#40658,#34122,.T.) ;
#53402=EDGE_CURVE('',#39411,#40668,#34123,.T.) ;
#53403=EDGE_CURVE('',#39412,#40671,#34124,.T.) ;
#53404=EDGE_CURVE('',#40667,#39413,#34125,.T.) ;
#53405=EDGE_CURVE('',#39412,#40658,#34126,.T.) ;
#53406=EDGE_CURVE('',#40149,#40160,#34127,.T.) ;
#53407=EDGE_CURVE('',#40150,#40163,#34128,.T.) ;
#53408=EDGE_CURVE('',#40161,#40156,#34129,.T.) ;
#53409=EDGE_CURVE('',#40150,#40383,#34130,.T.) ;
#53410=EDGE_CURVE('',#40383,#40163,#34131,.T.) ;
#53411=EDGE_CURVE('',#40155,#40148,#34132,.T.) ;
#53412=EDGE_CURVE('',#40162,#40159,#34133,.T.) ;
#53413=EDGE_CURVE('',#40380,#40162,#34134,.T.) ;
#53414=EDGE_CURVE('',#40151,#40382,#34135,.T.) ;
#53415=EDGE_CURVE('',#40152,#40151,#34136,.T.) ;
#53416=EDGE_CURVE('',#40380,#40159,#34137,.T.) ;
#53417=EDGE_CURVE('',#40152,#40382,#34138,.T.) ;
#53418=EDGE_CURVE('',#40381,#40158,#34139,.T.) ;
#53419=EDGE_CURVE('',#40153,#40381,#34140,.T.) ;
#53420=EDGE_CURVE('',#40153,#40158,#34141,.T.) ;
#53421=EDGE_CURVE('',#40154,#40157,#34142,.T.) ;
#53422=EDGE_CURVE('',#40047,#41535,#34143,.T.) ;
#53423=EDGE_CURVE('',#40048,#39888,#34144,.T.) ;
#53424=EDGE_CURVE('',#40049,#39891,#34145,.T.) ;
#53425=EDGE_CURVE('',#39886,#40049,#34146,.T.) ;
#53426=EDGE_CURVE('',#39886,#39891,#34147,.T.) ;
#53427=EDGE_CURVE('',#39887,#39890,#34148,.T.) ;
#53428=EDGE_CURVE('',#40102,#39887,#34149,.T.) ;
#53429=EDGE_CURVE('',#40102,#39890,#34150,.T.) ;
#53430=EDGE_CURVE('',#40103,#39889,#34151,.T.) ;
#53431=EDGE_CURVE('',#40098,#41534,#34152,.T.) ;
#53432=EDGE_CURVE('',#40099,#41541,#34153,.T.) ;
#53433=EDGE_CURVE('',#40100,#39872,#34154,.T.) ;
#53434=EDGE_CURVE('',#40101,#39875,#34155,.T.) ;
#53435=EDGE_CURVE('',#39876,#40101,#34156,.T.) ;
#53436=EDGE_CURVE('',#39876,#39875,#34157,.T.) ;
#53437=EDGE_CURVE('',#39877,#39874,#34158,.T.) ;
#53438=EDGE_CURVE('',#40050,#39877,#34159,.T.) ;
#53439=EDGE_CURVE('',#40050,#39874,#34160,.T.) ;
#53440=EDGE_CURVE('',#40051,#39873,#34161,.T.) ;
#53441=EDGE_CURVE('',#40046,#41540,#34162,.T.) ;
#53442=EDGE_CURVE('',#39183,#41374,#34163,.T.) ;
#53443=EDGE_CURVE('',#41376,#39182,#34164,.T.) ;
#53444=EDGE_CURVE('',#41378,#39181,#34165,.T.) ;
#53445=EDGE_CURVE('',#39184,#41372,#34166,.T.) ;
#53446=EDGE_CURVE('',#41380,#39180,#34167,.T.) ;
#53447=EDGE_CURVE('',#39177,#41371,#34168,.T.) ;
#53448=EDGE_CURVE('',#41382,#39179,#34169,.T.) ;
#53449=EDGE_CURVE('',#39178,#41384,#34170,.T.) ;
#53450=EDGE_CURVE('',#40392,#40399,#34171,.T.) ;
#53451=EDGE_CURVE('',#40393,#40467,#34172,.T.) ;
#53452=EDGE_CURVE('',#40464,#40392,#34173,.T.) ;
#53453=EDGE_CURVE('',#40394,#40393,#34174,.T.) ;
#53454=EDGE_CURVE('',#40464,#40399,#34175,.T.) ;
#53455=EDGE_CURVE('',#40394,#40467,#34176,.T.) ;
#53456=EDGE_CURVE('',#40398,#40397,#34177,.T.) ;
#53457=EDGE_CURVE('',#40465,#40398,#34178,.T.) ;
#53458=EDGE_CURVE('',#40395,#40466,#34179,.T.) ;
#53459=EDGE_CURVE('',#40396,#40395,#34180,.T.) ;
#53460=EDGE_CURVE('',#40465,#40397,#34181,.T.) ;
#53461=EDGE_CURVE('',#40396,#40466,#34182,.T.) ;
#53462=EDGE_CURVE('',#39139,#40936,#34183,.T.) ;
#53463=EDGE_CURVE('',#40937,#39138,#34184,.T.) ;
#53464=EDGE_CURVE('',#40933,#39137,#34185,.T.) ;
#53465=EDGE_CURVE('',#40937,#40933,#34186,.T.) ;
#53466=EDGE_CURVE('',#40925,#40936,#34187,.T.) ;
#53467=EDGE_CURVE('',#39140,#40925,#34188,.T.) ;
#53468=EDGE_CURVE('',#40930,#39136,#34189,.T.) ;
#53469=EDGE_CURVE('',#40934,#40932,#34190,.T.) ;
#53470=EDGE_CURVE('',#40935,#41157,#34191,.T.) ;
#53471=EDGE_CURVE('',#41154,#40934,#34192,.T.) ;
#53472=EDGE_CURVE('',#40922,#40935,#34193,.T.) ;
#53473=EDGE_CURVE('',#39134,#40924,#34194,.T.) ;
#53474=EDGE_CURVE('',#39135,#40926,#34195,.T.) ;
#53475=EDGE_CURVE('',#40927,#39133,#34196,.T.) ;
#53476=EDGE_CURVE('',#40930,#40926,#34197,.T.) ;
#53477=EDGE_CURVE('',#41154,#40932,#34198,.T.) ;
#53478=EDGE_CURVE('',#40922,#41157,#34199,.T.) ;
#53479=EDGE_CURVE('',#40927,#40924,#34200,.T.) ;
#53480=EDGE_CURVE('',#40931,#40929,#34201,.T.) ;
#53481=EDGE_CURVE('',#41155,#40931,#34202,.T.) ;
#53482=EDGE_CURVE('',#40923,#41156,#34203,.T.) ;
#53483=EDGE_CURVE('',#40928,#40923,#34204,.T.) ;
#53484=EDGE_CURVE('',#41155,#40929,#34205,.T.) ;
#53485=EDGE_CURVE('',#40928,#41156,#34206,.T.) ;
#53486=EDGE_CURVE('',#41166,#41173,#34207,.T.) ;
#53487=EDGE_CURVE('',#41167,#41241,#34208,.T.) ;
#53488=EDGE_CURVE('',#41238,#41166,#34209,.T.) ;
#53489=EDGE_CURVE('',#41168,#41167,#34210,.T.) ;
#53490=EDGE_CURVE('',#41238,#41173,#34211,.T.) ;
#53491=EDGE_CURVE('',#41168,#41241,#34212,.T.) ;
#53492=EDGE_CURVE('',#41172,#41171,#34213,.T.) ;
#53493=EDGE_CURVE('',#41239,#41172,#34214,.T.) ;
#53494=EDGE_CURVE('',#41169,#41240,#34215,.T.) ;
#53495=EDGE_CURVE('',#41170,#41169,#34216,.T.) ;
#53496=EDGE_CURVE('',#41239,#41171,#34217,.T.) ;
#53497=EDGE_CURVE('',#41170,#41240,#34218,.T.) ;
#53498=EDGE_CURVE('',#41377,#41389,#34219,.T.) ;
#53499=EDGE_CURVE('',#41386,#41379,#34220,.T.) ;
#53500=EDGE_CURVE('',#41386,#41381,#34221,.T.) ;
#53501=EDGE_CURVE('',#41375,#41389,#34222,.T.) ;
#53502=EDGE_CURVE('',#41387,#41383,#34223,.T.) ;
#53503=EDGE_CURVE('',#41373,#41388,#34224,.T.) ;
#53504=EDGE_CURVE('',#41387,#41385,#34225,.T.) ;
#53505=EDGE_CURVE('',#41370,#41388,#34226,.T.) ;
#53506=EDGE_CURVE('',#40867,#40862,#34227,.T.) ;
#53507=EDGE_CURVE('',#40861,#40867,#34228,.T.) ;
#53508=EDGE_CURVE('',#40862,#40861,#34229,.T.) ;
#53509=EDGE_CURVE('',#40858,#40866,#34230,.T.) ;
#53510=EDGE_CURVE('',#40863,#40860,#34231,.T.) ;
#53511=EDGE_CURVE('',#40868,#40865,#34232,.T.) ;
#53512=EDGE_CURVE('',#40871,#40681,#34233,.T.) ;
#53513=EDGE_CURVE('',#40866,#40680,#34234,.T.) ;
#53514=EDGE_CURVE('',#40858,#40680,#34235,.T.) ;
#53515=EDGE_CURVE('',#40863,#39330,#34236,.T.) ;
#53516=EDGE_CURVE('',#39329,#40860,#34237,.T.) ;
#53517=EDGE_CURVE('',#40868,#40854,#34238,.T.) ;
#53518=EDGE_CURVE('',#40854,#40865,#34239,.T.) ;
#53519=EDGE_CURVE('',#40870,#39162,#34240,.T.) ;
#53520=EDGE_CURVE('',#39161,#40871,#34241,.T.) ;
#53521=EDGE_CURVE('',#40859,#40679,#34242,.T.) ;
#53522=EDGE_CURVE('',#39331,#40859,#34243,.T.) ;
#53523=EDGE_CURVE('',#40864,#39336,#34244,.T.) ;
#53524=EDGE_CURVE('',#40855,#40864,#34245,.T.) ;
#53525=EDGE_CURVE('',#40869,#40857,#34246,.T.) ;
#53526=EDGE_CURVE('',#40690,#40870,#34247,.T.) ;
#53527=EDGE_CURVE('',#40691,#40869,#34248,.T.) ;
#53528=EDGE_CURVE('',#39331,#40678,#34249,.T.) ;
#53529=EDGE_CURVE('',#40855,#39335,#34250,.T.) ;
#53530=EDGE_CURVE('',#40691,#40857,#34251,.T.) ;
#53531=EDGE_CURVE('',#40674,#40669,#34252,.T.) ;
#53532=EDGE_CURVE('',#40675,#40668,#34253,.T.) ;
#53533=EDGE_CURVE('',#39332,#40677,#34254,.T.) ;
#53534=EDGE_CURVE('',#40856,#39334,#34255,.T.) ;
#53535=EDGE_CURVE('',#40692,#40856,#34256,.T.) ;
#53536=EDGE_CURVE('',#40675,#39411,#34257,.T.) ;
#53537=EDGE_CURVE('',#39332,#40682,#34258,.T.) ;
#53538=EDGE_CURVE('',#40682,#40677,#34259,.T.) ;
#53539=EDGE_CURVE('',#40693,#39334,#34260,.T.) ;
#53540=EDGE_CURVE('',#40676,#39410,#34261,.T.) ;
#53541=EDGE_CURVE('',#40683,#40676,#34262,.T.) ;
#53542=EDGE_CURVE('',#39333,#40685,#34263,.T.) ;
#53543=EDGE_CURVE('',#40694,#39333,#34264,.T.) ;
#53544=EDGE_CURVE('',#40683,#39409,#34265,.T.) ;
#53545=EDGE_CURVE('',#40694,#40685,#34266,.T.) ;
#53546=EDGE_CURVE('',#40684,#39408,#34267,.T.) ;
#53547=EDGE_CURVE('',#40695,#40684,#34268,.T.) ;
#53548=EDGE_CURVE('',#40698,#40687,#34269,.T.) ;
#53549=EDGE_CURVE('',#40699,#40686,#34270,.T.) ;
#53550=EDGE_CURVE('',#39405,#40696,#34271,.T.) ;
#53551=EDGE_CURVE('',#39406,#40699,#34272,.T.) ;
#53552=EDGE_CURVE('',#40695,#39407,#34273,.T.) ;
#53553=EDGE_CURVE('',#39406,#40686,#34274,.T.) ;
#53554=EDGE_CURVE('',#40133,#40144,#34275,.T.) ;
#53555=EDGE_CURVE('',#40134,#40147,#34276,.T.) ;
#53556=EDGE_CURVE('',#40145,#40140,#34277,.T.) ;
#53557=EDGE_CURVE('',#40134,#40403,#34278,.T.) ;
#53558=EDGE_CURVE('',#40403,#40147,#34279,.T.) ;
#53559=EDGE_CURVE('',#40139,#40132,#34280,.T.) ;
#53560=EDGE_CURVE('',#40146,#40143,#34281,.T.) ;
#53561=EDGE_CURVE('',#40400,#40146,#34282,.T.) ;
#53562=EDGE_CURVE('',#40135,#40402,#34283,.T.) ;
#53563=EDGE_CURVE('',#40136,#40135,#34284,.T.) ;
#53564=EDGE_CURVE('',#40400,#40143,#34285,.T.) ;
#53565=EDGE_CURVE('',#40136,#40402,#34286,.T.) ;
#53566=EDGE_CURVE('',#40401,#40142,#34287,.T.) ;
#53567=EDGE_CURVE('',#40137,#40401,#34288,.T.) ;
#53568=EDGE_CURVE('',#40137,#40142,#34289,.T.) ;
#53569=EDGE_CURVE('',#40138,#40141,#34290,.T.) ;
#53570=EDGE_CURVE('',#40053,#41543,#34291,.T.) ;
#53571=EDGE_CURVE('',#40054,#39868,#34292,.T.) ;
#53572=EDGE_CURVE('',#40055,#39871,#34293,.T.) ;
#53573=EDGE_CURVE('',#39866,#40055,#34294,.T.) ;
#53574=EDGE_CURVE('',#39866,#39871,#34295,.T.) ;
#53575=EDGE_CURVE('',#39867,#39870,#34296,.T.) ;
#53576=EDGE_CURVE('',#40108,#39867,#34297,.T.) ;
#53577=EDGE_CURVE('',#40108,#39870,#34298,.T.) ;
#53578=EDGE_CURVE('',#40109,#39869,#34299,.T.) ;
#53579=EDGE_CURVE('',#40104,#41542,#34300,.T.) ;
#53580=EDGE_CURVE('',#40105,#41549,#34301,.T.) ;
#53581=EDGE_CURVE('',#40106,#39852,#34302,.T.) ;
#53582=EDGE_CURVE('',#40107,#39855,#34303,.T.) ;
#53583=EDGE_CURVE('',#39856,#40107,#34304,.T.) ;
#53584=EDGE_CURVE('',#39856,#39855,#34305,.T.) ;
#53585=EDGE_CURVE('',#39857,#39854,#34306,.T.) ;
#53586=EDGE_CURVE('',#40056,#39857,#34307,.T.) ;
#53587=EDGE_CURVE('',#40056,#39854,#34308,.T.) ;
#53588=EDGE_CURVE('',#40057,#39853,#34309,.T.) ;
#53589=EDGE_CURVE('',#40052,#41548,#34310,.T.) ;
#53590=EDGE_CURVE('',#39171,#41394,#34311,.T.) ;
#53591=EDGE_CURVE('',#41396,#39170,#34312,.T.) ;
#53592=EDGE_CURVE('',#41398,#39169,#34313,.T.) ;
#53593=EDGE_CURVE('',#39172,#41392,#34314,.T.) ;
#53594=EDGE_CURVE('',#41400,#39168,#34315,.T.) ;
#53595=EDGE_CURVE('',#39165,#41391,#34316,.T.) ;
#53596=EDGE_CURVE('',#41402,#39167,#34317,.T.) ;
#53597=EDGE_CURVE('',#39166,#41404,#34318,.T.) ;
#53598=EDGE_CURVE('',#40412,#40419,#34319,.T.) ;
#53599=EDGE_CURVE('',#40413,#40471,#34320,.T.) ;
#53600=EDGE_CURVE('',#40468,#40412,#34321,.T.) ;
#53601=EDGE_CURVE('',#40414,#40413,#34322,.T.) ;
#53602=EDGE_CURVE('',#40468,#40419,#34323,.T.) ;
#53603=EDGE_CURVE('',#40414,#40471,#34324,.T.) ;
#53604=EDGE_CURVE('',#40418,#40417,#34325,.T.) ;
#53605=EDGE_CURVE('',#40469,#40418,#34326,.T.) ;
#53606=EDGE_CURVE('',#40415,#40470,#34327,.T.) ;
#53607=EDGE_CURVE('',#40416,#40415,#34328,.T.) ;
#53608=EDGE_CURVE('',#40469,#40417,#34329,.T.) ;
#53609=EDGE_CURVE('',#40416,#40470,#34330,.T.) ;
#53610=EDGE_CURVE('',#39075,#40920,#34331,.T.) ;
#53611=EDGE_CURVE('',#40921,#39074,#34332,.T.) ;
#53612=EDGE_CURVE('',#40917,#39073,#34333,.T.) ;
#53613=EDGE_CURVE('',#40921,#40917,#34334,.T.) ;
#53614=EDGE_CURVE('',#40909,#40920,#34335,.T.) ;
#53615=EDGE_CURVE('',#39076,#40909,#34336,.T.) ;
#53616=EDGE_CURVE('',#40914,#39072,#34337,.T.) ;
#53617=EDGE_CURVE('',#40918,#40916,#34338,.T.) ;
#53618=EDGE_CURVE('',#40919,#41177,#34339,.T.) ;
#53619=EDGE_CURVE('',#41174,#40918,#34340,.T.) ;
#53620=EDGE_CURVE('',#40906,#40919,#34341,.T.) ;
#53621=EDGE_CURVE('',#39070,#40908,#34342,.T.) ;
#53622=EDGE_CURVE('',#39071,#40910,#34343,.T.) ;
#53623=EDGE_CURVE('',#40911,#39069,#34344,.T.) ;
#53624=EDGE_CURVE('',#40914,#40910,#34345,.T.) ;
#53625=EDGE_CURVE('',#41174,#40916,#34346,.T.) ;
#53626=EDGE_CURVE('',#40906,#41177,#34347,.T.) ;
#53627=EDGE_CURVE('',#40911,#40908,#34348,.T.) ;
#53628=EDGE_CURVE('',#40915,#40913,#34349,.T.) ;
#53629=EDGE_CURVE('',#41175,#40915,#34350,.T.) ;
#53630=EDGE_CURVE('',#40907,#41176,#34351,.T.) ;
#53631=EDGE_CURVE('',#40912,#40907,#34352,.T.) ;
#53632=EDGE_CURVE('',#41175,#40913,#34353,.T.) ;
#53633=EDGE_CURVE('',#40912,#41176,#34354,.T.) ;
#53634=EDGE_CURVE('',#41186,#41193,#34355,.T.) ;
#53635=EDGE_CURVE('',#41187,#41245,#34356,.T.) ;
#53636=EDGE_CURVE('',#41242,#41186,#34357,.T.) ;
#53637=EDGE_CURVE('',#41188,#41187,#34358,.T.) ;
#53638=EDGE_CURVE('',#41242,#41193,#34359,.T.) ;
#53639=EDGE_CURVE('',#41188,#41245,#34360,.T.) ;
#53640=EDGE_CURVE('',#41192,#41191,#34361,.T.) ;
#53641=EDGE_CURVE('',#41243,#41192,#34362,.T.) ;
#53642=EDGE_CURVE('',#41189,#41244,#34363,.T.) ;
#53643=EDGE_CURVE('',#41190,#41189,#34364,.T.) ;
#53644=EDGE_CURVE('',#41243,#41191,#34365,.T.) ;
#53645=EDGE_CURVE('',#41190,#41244,#34366,.T.) ;
#53646=EDGE_CURVE('',#41397,#41409,#34367,.T.) ;
#53647=EDGE_CURVE('',#41406,#41399,#34368,.T.) ;
#53648=EDGE_CURVE('',#41406,#41401,#34369,.T.) ;
#53649=EDGE_CURVE('',#41395,#41409,#34370,.T.) ;
#53650=EDGE_CURVE('',#41407,#41403,#34371,.T.) ;
#53651=EDGE_CURVE('',#41393,#41408,#34372,.T.) ;
#53652=EDGE_CURVE('',#41407,#41405,#34373,.T.) ;
#53653=EDGE_CURVE('',#41390,#41408,#34374,.T.) ;
#53654=EDGE_CURVE('',#40885,#40880,#34375,.T.) ;
#53655=EDGE_CURVE('',#40879,#40885,#34376,.T.) ;
#53656=EDGE_CURVE('',#40880,#40879,#34377,.T.) ;
#53657=EDGE_CURVE('',#40876,#40884,#34378,.T.) ;
#53658=EDGE_CURVE('',#40881,#40878,#34379,.T.) ;
#53659=EDGE_CURVE('',#40886,#40883,#34380,.T.) ;
#53660=EDGE_CURVE('',#40889,#40709,#34381,.T.) ;
#53661=EDGE_CURVE('',#40884,#40708,#34382,.T.) ;
#53662=EDGE_CURVE('',#40876,#40708,#34383,.T.) ;
#53663=EDGE_CURVE('',#40881,#39322,#34384,.T.) ;
#53664=EDGE_CURVE('',#39321,#40878,#34385,.T.) ;
#53665=EDGE_CURVE('',#40886,#40872,#34386,.T.) ;
#53666=EDGE_CURVE('',#40872,#40883,#34387,.T.) ;
#53667=EDGE_CURVE('',#40888,#39150,#34388,.T.) ;
#53668=EDGE_CURVE('',#39149,#40889,#34389,.T.) ;
#53669=EDGE_CURVE('',#40877,#40707,#34390,.T.) ;
#53670=EDGE_CURVE('',#39323,#40877,#34391,.T.) ;
#53671=EDGE_CURVE('',#40882,#39328,#34392,.T.) ;
#53672=EDGE_CURVE('',#40873,#40882,#34393,.T.) ;
#53673=EDGE_CURVE('',#40887,#40875,#34394,.T.) ;
#53674=EDGE_CURVE('',#40718,#40888,#34395,.T.) ;
#53675=EDGE_CURVE('',#40719,#40887,#34396,.T.) ;
#53676=EDGE_CURVE('',#39323,#40706,#34397,.T.) ;
#53677=EDGE_CURVE('',#40873,#39327,#34398,.T.) ;
#53678=EDGE_CURVE('',#40719,#40875,#34399,.T.) ;
#53679=EDGE_CURVE('',#40702,#40697,#34400,.T.) ;
#53680=EDGE_CURVE('',#40703,#40696,#34401,.T.) ;
#53681=EDGE_CURVE('',#39324,#40705,#34402,.T.) ;
#53682=EDGE_CURVE('',#40874,#39326,#34403,.T.) ;
#53683=EDGE_CURVE('',#40720,#40874,#34404,.T.) ;
#53684=EDGE_CURVE('',#40703,#39405,#34405,.T.) ;
#53685=EDGE_CURVE('',#39324,#40710,#34406,.T.) ;
#53686=EDGE_CURVE('',#40710,#40705,#34407,.T.) ;
#53687=EDGE_CURVE('',#40721,#39326,#34408,.T.) ;
#53688=EDGE_CURVE('',#40704,#39404,#34409,.T.) ;
#53689=EDGE_CURVE('',#40711,#40704,#34410,.T.) ;
#53690=EDGE_CURVE('',#39325,#40713,#34411,.T.) ;
#53691=EDGE_CURVE('',#40722,#39325,#34412,.T.) ;
#53692=EDGE_CURVE('',#40711,#39403,#34413,.T.) ;
#53693=EDGE_CURVE('',#40722,#40713,#34414,.T.) ;
#53694=EDGE_CURVE('',#40712,#39402,#34415,.T.) ;
#53695=EDGE_CURVE('',#40723,#40712,#34416,.T.) ;
#53696=EDGE_CURVE('',#40727,#40715,#34417,.T.) ;
#53697=EDGE_CURVE('',#40724,#40714,#34418,.T.) ;
#53698=EDGE_CURVE('',#39399,#40725,#34419,.T.) ;
#53699=EDGE_CURVE('',#39400,#40724,#34420,.T.) ;
#53700=EDGE_CURVE('',#40723,#39401,#34421,.T.) ;
#53701=EDGE_CURVE('',#39400,#40714,#34422,.T.) ;
#53702=EDGE_CURVE('',#40117,#40128,#34423,.T.) ;
#53703=EDGE_CURVE('',#40118,#40131,#34424,.T.) ;
#53704=EDGE_CURVE('',#40129,#40124,#34425,.T.) ;
#53705=EDGE_CURVE('',#40118,#40423,#34426,.T.) ;
#53706=EDGE_CURVE('',#40423,#40131,#34427,.T.) ;
#53707=EDGE_CURVE('',#40123,#40116,#34428,.T.) ;
#53708=EDGE_CURVE('',#40130,#40127,#34429,.T.) ;
#53709=EDGE_CURVE('',#40420,#40130,#34430,.T.) ;
#53710=EDGE_CURVE('',#40119,#40422,#34431,.T.) ;
#53711=EDGE_CURVE('',#40120,#40119,#34432,.T.) ;
#53712=EDGE_CURVE('',#40420,#40127,#34433,.T.) ;
#53713=EDGE_CURVE('',#40120,#40422,#34434,.T.) ;
#53714=EDGE_CURVE('',#40421,#40126,#34435,.T.) ;
#53715=EDGE_CURVE('',#40121,#40421,#34436,.T.) ;
#53716=EDGE_CURVE('',#40121,#40126,#34437,.T.) ;
#53717=EDGE_CURVE('',#40122,#40125,#34438,.T.) ;
#53718=EDGE_CURVE('',#40059,#41551,#34439,.T.) ;
#53719=EDGE_CURVE('',#40060,#39848,#34440,.T.) ;
#53720=EDGE_CURVE('',#40061,#39851,#34441,.T.) ;
#53721=EDGE_CURVE('',#39846,#40061,#34442,.T.) ;
#53722=EDGE_CURVE('',#39846,#39851,#34443,.T.) ;
#53723=EDGE_CURVE('',#39847,#39850,#34444,.T.) ;
#53724=EDGE_CURVE('',#40114,#39847,#34445,.T.) ;
#53725=EDGE_CURVE('',#40114,#39850,#34446,.T.) ;
#53726=EDGE_CURVE('',#40115,#39849,#34447,.T.) ;
#53727=EDGE_CURVE('',#40110,#41550,#34448,.T.) ;
#53728=EDGE_CURVE('',#40111,#41557,#34449,.T.) ;
#53729=EDGE_CURVE('',#40112,#39832,#34450,.T.) ;
#53730=EDGE_CURVE('',#40113,#39835,#34451,.T.) ;
#53731=EDGE_CURVE('',#39836,#40113,#34452,.T.) ;
#53732=EDGE_CURVE('',#39836,#39835,#34453,.T.) ;
#53733=EDGE_CURVE('',#39837,#39834,#34454,.T.) ;
#53734=EDGE_CURVE('',#40062,#39837,#34455,.T.) ;
#53735=EDGE_CURVE('',#40062,#39834,#34456,.T.) ;
#53736=EDGE_CURVE('',#40063,#39833,#34457,.T.) ;
#53737=EDGE_CURVE('',#40058,#41556,#34458,.T.) ;
#53738=EDGE_CURVE('',#39159,#41414,#34459,.T.) ;
#53739=EDGE_CURVE('',#41416,#39158,#34460,.T.) ;
#53740=EDGE_CURVE('',#41418,#39157,#34461,.T.) ;
#53741=EDGE_CURVE('',#39160,#41412,#34462,.T.) ;
#53742=EDGE_CURVE('',#41420,#39156,#34463,.T.) ;
#53743=EDGE_CURVE('',#39153,#41411,#34464,.T.) ;
#53744=EDGE_CURVE('',#41422,#39155,#34465,.T.) ;
#53745=EDGE_CURVE('',#39154,#41424,#34466,.T.) ;
#53746=EDGE_CURVE('',#40432,#40439,#34467,.T.) ;
#53747=EDGE_CURVE('',#40433,#40475,#34468,.T.) ;
#53748=EDGE_CURVE('',#40472,#40432,#34469,.T.) ;
#53749=EDGE_CURVE('',#40434,#40433,#34470,.T.) ;
#53750=EDGE_CURVE('',#40472,#40439,#34471,.T.) ;
#53751=EDGE_CURVE('',#40434,#40475,#34472,.T.) ;
#53752=EDGE_CURVE('',#40438,#40437,#34473,.T.) ;
#53753=EDGE_CURVE('',#40473,#40438,#34474,.T.) ;
#53754=EDGE_CURVE('',#40435,#40474,#34475,.T.) ;
#53755=EDGE_CURVE('',#40436,#40435,#34476,.T.) ;
#53756=EDGE_CURVE('',#40473,#40437,#34477,.T.) ;
#53757=EDGE_CURVE('',#40436,#40474,#34478,.T.) ;
#53758=EDGE_CURVE('',#39147,#40904,#34479,.T.) ;
#53759=EDGE_CURVE('',#40905,#39146,#34480,.T.) ;
#53760=EDGE_CURVE('',#40901,#39145,#34481,.T.) ;
#53761=EDGE_CURVE('',#40905,#40901,#34482,.T.) ;
#53762=EDGE_CURVE('',#40893,#40904,#34483,.T.) ;
#53763=EDGE_CURVE('',#39148,#40893,#34484,.T.) ;
#53764=EDGE_CURVE('',#40898,#39144,#34485,.T.) ;
#53765=EDGE_CURVE('',#40902,#40900,#34486,.T.) ;
#53766=EDGE_CURVE('',#40903,#41197,#34487,.T.) ;
#53767=EDGE_CURVE('',#41194,#40902,#34488,.T.) ;
#53768=EDGE_CURVE('',#40890,#40903,#34489,.T.) ;
#53769=EDGE_CURVE('',#39142,#40892,#34490,.T.) ;
#53770=EDGE_CURVE('',#39143,#40894,#34491,.T.) ;
#53771=EDGE_CURVE('',#40895,#39141,#34492,.T.) ;
#53772=EDGE_CURVE('',#40898,#40894,#34493,.T.) ;
#53773=EDGE_CURVE('',#41194,#40900,#34494,.T.) ;
#53774=EDGE_CURVE('',#40890,#41197,#34495,.T.) ;
#53775=EDGE_CURVE('',#40895,#40892,#34496,.T.) ;
#53776=EDGE_CURVE('',#40899,#40897,#34497,.T.) ;
#53777=EDGE_CURVE('',#41195,#40899,#34498,.T.) ;
#53778=EDGE_CURVE('',#40891,#41196,#34499,.T.) ;
#53779=EDGE_CURVE('',#40896,#40891,#34500,.T.) ;
#53780=EDGE_CURVE('',#41195,#40897,#34501,.T.) ;
#53781=EDGE_CURVE('',#40896,#41196,#34502,.T.) ;
#53782=EDGE_CURVE('',#41206,#41213,#34503,.T.) ;
#53783=EDGE_CURVE('',#41207,#41249,#34504,.T.) ;
#53784=EDGE_CURVE('',#41246,#41206,#34505,.T.) ;
#53785=EDGE_CURVE('',#41208,#41207,#34506,.T.) ;
#53786=EDGE_CURVE('',#41246,#41213,#34507,.T.) ;
#53787=EDGE_CURVE('',#41208,#41249,#34508,.T.) ;
#53788=EDGE_CURVE('',#41212,#41211,#34509,.T.) ;
#53789=EDGE_CURVE('',#41247,#41212,#34510,.T.) ;
#53790=EDGE_CURVE('',#41209,#41248,#34511,.T.) ;
#53791=EDGE_CURVE('',#41210,#41209,#34512,.T.) ;
#53792=EDGE_CURVE('',#41247,#41211,#34513,.T.) ;
#53793=EDGE_CURVE('',#41210,#41248,#34514,.T.) ;
#53794=EDGE_CURVE('',#41417,#41429,#34515,.T.) ;
#53795=EDGE_CURVE('',#41426,#41419,#34516,.T.) ;
#53796=EDGE_CURVE('',#41426,#41421,#34517,.T.) ;
#53797=EDGE_CURVE('',#41415,#41429,#34518,.T.) ;
#53798=EDGE_CURVE('',#41427,#41423,#34519,.T.) ;
#53799=EDGE_CURVE('',#41413,#41428,#34520,.T.) ;
#53800=EDGE_CURVE('',#41427,#41425,#34521,.T.) ;
#53801=EDGE_CURVE('',#41410,#41428,#34522,.T.) ;
#53802=EDGE_CURVE('',#39247,#39271,#34523,.T.) ;
#53803=EDGE_CURVE('',#39270,#39248,#34524,.T.) ;
#53804=EDGE_CURVE('',#39235,#39277,#34525,.T.) ;
#53805=EDGE_CURVE('',#39276,#39236,#34526,.T.) ;
#53806=EDGE_CURVE('',#39223,#39283,#34527,.T.) ;
#53807=EDGE_CURVE('',#39282,#39224,#34528,.T.) ;
#53808=EDGE_CURVE('',#39211,#39289,#34529,.T.) ;
#53809=EDGE_CURVE('',#39288,#39212,#34530,.T.) ;
#53810=EDGE_CURVE('',#39199,#39295,#34531,.T.) ;
#53811=EDGE_CURVE('',#39294,#39200,#34532,.T.) ;
#53812=EDGE_CURVE('',#39187,#39301,#34533,.T.) ;
#53813=EDGE_CURVE('',#39300,#39188,#34534,.T.) ;
#53814=EDGE_CURVE('',#39175,#39307,#34535,.T.) ;
#53815=EDGE_CURVE('',#39306,#39176,#34536,.T.) ;
#53816=EDGE_CURVE('',#39163,#39313,#34537,.T.) ;
#53817=EDGE_CURVE('',#39312,#39164,#34538,.T.) ;
#53818=EDGE_CURVE('',#39151,#39319,#34539,.T.) ;
#53819=EDGE_CURVE('',#39318,#39152,#34540,.T.) ;
#53820=EDGE_CURVE('',#41558,#39274,#34541,.T.) ;
#53821=EDGE_CURVE('',#41558,#39275,#2377,.T.) ;
#53822=EDGE_CURVE('',#40501,#41558,#34542,.T.) ;
#53823=EDGE_CURVE('',#41559,#39273,#34543,.T.) ;
#53824=EDGE_CURVE('',#40502,#41559,#34544,.T.) ;
#53825=EDGE_CURVE('',#39272,#41559,#2378,.T.) ;
#53826=EDGE_CURVE('',#39465,#39269,#2379,.T.) ;
#53827=EDGE_CURVE('',#41560,#39280,#34545,.T.) ;
#53828=EDGE_CURVE('',#41560,#39281,#2380,.T.) ;
#53829=EDGE_CURVE('',#40529,#41560,#34546,.T.) ;
#53830=EDGE_CURVE('',#41561,#39279,#34547,.T.) ;
#53831=EDGE_CURVE('',#40530,#41561,#34548,.T.) ;
#53832=EDGE_CURVE('',#39278,#41561,#2381,.T.) ;
#53833=EDGE_CURVE('',#41562,#39286,#34549,.T.) ;
#53834=EDGE_CURVE('',#41562,#39287,#2382,.T.) ;
#53835=EDGE_CURVE('',#40557,#41562,#34550,.T.) ;
#53836=EDGE_CURVE('',#41563,#39285,#34551,.T.) ;
#53837=EDGE_CURVE('',#40558,#41563,#34552,.T.) ;
#53838=EDGE_CURVE('',#39284,#41563,#2383,.T.) ;
#53839=EDGE_CURVE('',#41564,#39292,#34553,.T.) ;
#53840=EDGE_CURVE('',#41564,#39293,#2384,.T.) ;
#53841=EDGE_CURVE('',#40585,#41564,#34554,.T.) ;
#53842=EDGE_CURVE('',#41565,#39291,#34555,.T.) ;
#53843=EDGE_CURVE('',#40586,#41565,#34556,.T.) ;
#53844=EDGE_CURVE('',#39290,#41565,#2385,.T.) ;
#53845=EDGE_CURVE('',#41566,#39298,#34557,.T.) ;
#53846=EDGE_CURVE('',#41566,#39299,#2386,.T.) ;
#53847=EDGE_CURVE('',#40613,#41566,#34558,.T.) ;
#53848=EDGE_CURVE('',#41567,#39297,#34559,.T.) ;
#53849=EDGE_CURVE('',#40614,#41567,#34560,.T.) ;
#53850=EDGE_CURVE('',#39296,#41567,#2387,.T.) ;
#53851=EDGE_CURVE('',#41568,#39304,#34561,.T.) ;
#53852=EDGE_CURVE('',#41568,#39305,#2388,.T.) ;
#53853=EDGE_CURVE('',#40641,#41568,#34562,.T.) ;
#53854=EDGE_CURVE('',#41569,#39303,#34563,.T.) ;
#53855=EDGE_CURVE('',#40642,#41569,#34564,.T.) ;
#53856=EDGE_CURVE('',#39302,#41569,#2389,.T.) ;
#53857=EDGE_CURVE('',#41570,#39310,#34565,.T.) ;
#53858=EDGE_CURVE('',#41570,#39311,#2390,.T.) ;
#53859=EDGE_CURVE('',#40669,#41570,#34566,.T.) ;
#53860=EDGE_CURVE('',#41571,#39309,#34567,.T.) ;
#53861=EDGE_CURVE('',#40670,#41571,#34568,.T.) ;
#53862=EDGE_CURVE('',#39308,#41571,#2391,.T.) ;
#53863=EDGE_CURVE('',#41572,#39316,#34569,.T.) ;
#53864=EDGE_CURVE('',#41572,#39317,#2392,.T.) ;
#53865=EDGE_CURVE('',#40697,#41572,#34570,.T.) ;
#53866=EDGE_CURVE('',#41573,#39315,#34571,.T.) ;
#53867=EDGE_CURVE('',#40698,#41573,#34572,.T.) ;
#53868=EDGE_CURVE('',#39314,#41573,#2393,.T.) ;
#53869=EDGE_CURVE('',#40726,#39258,#34573,.T.) ;
#53870=EDGE_CURVE('',#41574,#39257,#34574,.T.) ;
#53871=EDGE_CURVE('',#40727,#41574,#34575,.T.) ;
#53872=EDGE_CURVE('',#39320,#41574,#2394,.T.) ;
#53873=EDGE_CURVE('',#40492,#41575,#2395,.T.) ;
#53874=EDGE_CURVE('',#40493,#41575,#34576,.T.) ;
#53875=EDGE_CURVE('',#41575,#39247,#34577,.T.) ;
#53876=EDGE_CURVE('',#40494,#39246,#34578,.T.) ;
#53877=EDGE_CURVE('',#41576,#40476,#34579,.T.) ;
#53878=EDGE_CURVE('',#41576,#40477,#2396,.T.) ;
#53879=EDGE_CURVE('',#39248,#41576,#34580,.T.) ;
#53880=EDGE_CURVE('',#39245,#40485,#34581,.T.) ;
#53881=EDGE_CURVE('',#40520,#41577,#2397,.T.) ;
#53882=EDGE_CURVE('',#40521,#41577,#34582,.T.) ;
#53883=EDGE_CURVE('',#41577,#39235,#34583,.T.) ;
#53884=EDGE_CURVE('',#40522,#39234,#34584,.T.) ;
#53885=EDGE_CURVE('',#41578,#40504,#34585,.T.) ;
#53886=EDGE_CURVE('',#41578,#40505,#2398,.T.) ;
#53887=EDGE_CURVE('',#39236,#41578,#34586,.T.) ;
#53888=EDGE_CURVE('',#39233,#40513,#34587,.T.) ;
#53889=EDGE_CURVE('',#40548,#41579,#2399,.T.) ;
#53890=EDGE_CURVE('',#40549,#41579,#34588,.T.) ;
#53891=EDGE_CURVE('',#41579,#39223,#34589,.T.) ;
#53892=EDGE_CURVE('',#40550,#39222,#34590,.T.) ;
#53893=EDGE_CURVE('',#41580,#40532,#34591,.T.) ;
#53894=EDGE_CURVE('',#41580,#40533,#2400,.T.) ;
#53895=EDGE_CURVE('',#39224,#41580,#34592,.T.) ;
#53896=EDGE_CURVE('',#39221,#40541,#34593,.T.) ;
#53897=EDGE_CURVE('',#40576,#41581,#2401,.T.) ;
#53898=EDGE_CURVE('',#40577,#41581,#34594,.T.) ;
#53899=EDGE_CURVE('',#41581,#39211,#34595,.T.) ;
#53900=EDGE_CURVE('',#40578,#39210,#34596,.T.) ;
#53901=EDGE_CURVE('',#41582,#40560,#34597,.T.) ;
#53902=EDGE_CURVE('',#41582,#40561,#2402,.T.) ;
#53903=EDGE_CURVE('',#39212,#41582,#34598,.T.) ;
#53904=EDGE_CURVE('',#39209,#40569,#34599,.T.) ;
#53905=EDGE_CURVE('',#40604,#41583,#2403,.T.) ;
#53906=EDGE_CURVE('',#40605,#41583,#34600,.T.) ;
#53907=EDGE_CURVE('',#41583,#39199,#34601,.T.) ;
#53908=EDGE_CURVE('',#40606,#39198,#34602,.T.) ;
#53909=EDGE_CURVE('',#41584,#40588,#34603,.T.) ;
#53910=EDGE_CURVE('',#41584,#40589,#2404,.T.) ;
#53911=EDGE_CURVE('',#39200,#41584,#34604,.T.) ;
#53912=EDGE_CURVE('',#39197,#40597,#34605,.T.) ;
#53913=EDGE_CURVE('',#40632,#41585,#2405,.T.) ;
#53914=EDGE_CURVE('',#40633,#41585,#34606,.T.) ;
#53915=EDGE_CURVE('',#41585,#39187,#34607,.T.) ;
#53916=EDGE_CURVE('',#40634,#39186,#34608,.T.) ;
#53917=EDGE_CURVE('',#41586,#40616,#34609,.T.) ;
#53918=EDGE_CURVE('',#41586,#40617,#2406,.T.) ;
#53919=EDGE_CURVE('',#39188,#41586,#34610,.T.) ;
#53920=EDGE_CURVE('',#39185,#40625,#34611,.T.) ;
#53921=EDGE_CURVE('',#40660,#41587,#2407,.T.) ;
#53922=EDGE_CURVE('',#40661,#41587,#34612,.T.) ;
#53923=EDGE_CURVE('',#41587,#39175,#34613,.T.) ;
#53924=EDGE_CURVE('',#40662,#39174,#34614,.T.) ;
#53925=EDGE_CURVE('',#41588,#40644,#34615,.T.) ;
#53926=EDGE_CURVE('',#41588,#40645,#2408,.T.) ;
#53927=EDGE_CURVE('',#39176,#41588,#34616,.T.) ;
#53928=EDGE_CURVE('',#39173,#40653,#34617,.T.) ;
#53929=EDGE_CURVE('',#40688,#41589,#2409,.T.) ;
#53930=EDGE_CURVE('',#40689,#41589,#34618,.T.) ;
#53931=EDGE_CURVE('',#41589,#39163,#34619,.T.) ;
#53932=EDGE_CURVE('',#40690,#39162,#34620,.T.) ;
#53933=EDGE_CURVE('',#41590,#40672,#34621,.T.) ;
#53934=EDGE_CURVE('',#41590,#40673,#2410,.T.) ;
#53935=EDGE_CURVE('',#39164,#41590,#34622,.T.) ;
#53936=EDGE_CURVE('',#39161,#40681,#34623,.T.) ;
#53937=EDGE_CURVE('',#40716,#41591,#2411,.T.) ;
#53938=EDGE_CURVE('',#40717,#41591,#34624,.T.) ;
#53939=EDGE_CURVE('',#41591,#39151,#34625,.T.) ;
#53940=EDGE_CURVE('',#40718,#39150,#34626,.T.) ;
#53941=EDGE_CURVE('',#41592,#40700,#34627,.T.) ;
#53942=EDGE_CURVE('',#41592,#40701,#2412,.T.) ;
#53943=EDGE_CURVE('',#39152,#41592,#34628,.T.) ;
#53944=EDGE_CURVE('',#39149,#40709,#34629,.T.) ;
#53945=EDGE_CURVE('',#39272,#41575,#34630,.T.) ;
#53946=EDGE_CURVE('',#41559,#40492,#34631,.T.) ;
#53947=EDGE_CURVE('',#41576,#39269,#34632,.T.) ;
#53948=EDGE_CURVE('',#40477,#39465,#34633,.T.) ;
#53949=EDGE_CURVE('',#39278,#41577,#34634,.T.) ;
#53950=EDGE_CURVE('',#41561,#40520,#34635,.T.) ;
#53951=EDGE_CURVE('',#41578,#39275,#34636,.T.) ;
#53952=EDGE_CURVE('',#40505,#41558,#34637,.T.) ;
#53953=EDGE_CURVE('',#39284,#41579,#34638,.T.) ;
#53954=EDGE_CURVE('',#41563,#40548,#34639,.T.) ;
#53955=EDGE_CURVE('',#41580,#39281,#34640,.T.) ;
#53956=EDGE_CURVE('',#40533,#41560,#34641,.T.) ;
#53957=EDGE_CURVE('',#39290,#41581,#34642,.T.) ;
#53958=EDGE_CURVE('',#41565,#40576,#34643,.T.) ;
#53959=EDGE_CURVE('',#41582,#39287,#34644,.T.) ;
#53960=EDGE_CURVE('',#40561,#41562,#34645,.T.) ;
#53961=EDGE_CURVE('',#39296,#41583,#34646,.T.) ;
#53962=EDGE_CURVE('',#41567,#40604,#34647,.T.) ;
#53963=EDGE_CURVE('',#41584,#39293,#34648,.T.) ;
#53964=EDGE_CURVE('',#40589,#41564,#34649,.T.) ;
#53965=EDGE_CURVE('',#39302,#41585,#34650,.T.) ;
#53966=EDGE_CURVE('',#41569,#40632,#34651,.T.) ;
#53967=EDGE_CURVE('',#41586,#39299,#34652,.T.) ;
#53968=EDGE_CURVE('',#40617,#41566,#34653,.T.) ;
#53969=EDGE_CURVE('',#39308,#41587,#34654,.T.) ;
#53970=EDGE_CURVE('',#41571,#40660,#34655,.T.) ;
#53971=EDGE_CURVE('',#41588,#39305,#34656,.T.) ;
#53972=EDGE_CURVE('',#40645,#41568,#34657,.T.) ;
#53973=EDGE_CURVE('',#39314,#41589,#34658,.T.) ;
#53974=EDGE_CURVE('',#41573,#40688,#34659,.T.) ;
#53975=EDGE_CURVE('',#41590,#39311,#34660,.T.) ;
#53976=EDGE_CURVE('',#40673,#41570,#34661,.T.) ;
#53977=EDGE_CURVE('',#39320,#41591,#34662,.T.) ;
#53978=EDGE_CURVE('',#41574,#40716,#34663,.T.) ;
#53979=EDGE_CURVE('',#41592,#39317,#34664,.T.) ;
#53980=EDGE_CURVE('',#40701,#41572,#34665,.T.) ;
#53981=EDGE_CURVE('',#38767,#38761,#34666,.T.) ;
#53982=EDGE_CURVE('',#38774,#38768,#34667,.T.) ;
#53983=EDGE_CURVE('',#38781,#38775,#34668,.T.) ;
#53984=EDGE_CURVE('',#38788,#38782,#34669,.T.) ;
#53985=EDGE_CURVE('',#38795,#38789,#34670,.T.) ;
#53986=EDGE_CURVE('',#38802,#38796,#34671,.T.) ;
#53987=EDGE_CURVE('',#39398,#39614,#34672,.T.) ;
#53988=EDGE_CURVE('',#39399,#39613,#34673,.T.) ;
#53989=EDGE_CURVE('',#40725,#39612,#34674,.T.) ;
#53990=EDGE_CURVE('',#40726,#39611,#34675,.T.) ;
#53991=EDGE_CURVE('',#39258,#39611,#34676,.T.) ;
#53992=EDGE_CURVE('',#39259,#39610,#34677,.T.) ;
#53993=EDGE_CURVE('',#39462,#39610,#34678,.T.) ;
#53994=EDGE_CURVE('',#39703,#39609,#34679,.T.) ;
#53995=EDGE_CURVE('',#39606,#39063,#34680,.T.) ;
#53996=EDGE_CURVE('',#39393,#39608,#34681,.T.) ;
#53997=EDGE_CURVE('',#39703,#39393,#34682,.T.) ;
#53998=EDGE_CURVE('',#39607,#39068,#34683,.T.) ;
#53999=EDGE_CURVE('',#39394,#39607,#34684,.T.) ;
#54000=EDGE_CURVE('',#39704,#39396,#34685,.T.) ;
#54001=EDGE_CURVE('',#39394,#39068,#34686,.T.) ;
#54002=EDGE_CURVE('',#39799,#39396,#34687,.T.) ;
#54003=EDGE_CURVE('',#39705,#39799,#34688,.T.) ;
#54004=EDGE_CURVE('',#39395,#39067,#34689,.T.) ;
#54005=EDGE_CURVE('',#39800,#39395,#34690,.T.) ;
#54006=EDGE_CURVE('',#38818,#39043,#2413,.T.) ;
#54007=EDGE_CURVE('',#39800,#39067,#34691,.T.) ;
#54008=EDGE_CURVE('',#39629,#39397,#34692,.T.) ;
#54009=EDGE_CURVE('',#39630,#39460,#34693,.T.) ;
#54010=EDGE_CURVE('',#39631,#39711,#34694,.T.) ;
#54011=EDGE_CURVE('',#39632,#39710,#34695,.T.) ;
#54012=EDGE_CURVE('',#38755,#39044,#2414,.T.) ;
#54013=EDGE_CURVE('',#39632,#39261,#34696,.T.) ;
#54014=EDGE_CURVE('',#39706,#39798,#34697,.T.) ;
#54015=EDGE_CURVE('',#39633,#39260,#34698,.T.) ;
#54016=EDGE_CURVE('',#39531,#39798,#34699,.T.) ;
#54017=EDGE_CURVE('',#39707,#39531,#34700,.T.) ;
#54018=EDGE_CURVE('',#39633,#39461,#34701,.T.) ;
#54019=EDGE_CURVE('',#39797,#39066,#34702,.T.) ;
#54020=EDGE_CURVE('',#39532,#39797,#34703,.T.) ;
#54021=EDGE_CURVE('',#39708,#39534,#34704,.T.) ;
#54022=EDGE_CURVE('',#39634,#39708,#34705,.T.) ;
#54023=EDGE_CURVE('',#39532,#39066,#34706,.T.) ;
#54024=EDGE_CURVE('',#39620,#39534,#34707,.T.) ;
#54025=EDGE_CURVE('',#39533,#39065,#34708,.T.) ;
#54026=EDGE_CURVE('',#39621,#39533,#34709,.T.) ;
#54027=EDGE_CURVE('',#39621,#39065,#34710,.T.) ;
#54028=EDGE_CURVE('',#39622,#39064,#34711,.T.) ;
#54029=EDGE_CURVE('',#39824,#39821,#34712,.T.) ;
#54030=EDGE_CURVE('',#39825,#39827,#34713,.T.) ;
#68639=ORIENTED_EDGE('',*,*,#48897,.F.) ;
#68640=ORIENTED_EDGE('',*,*,#48898,.F.) ;
#68641=ORIENTED_EDGE('',*,*,#48899,.T.) ;
#68642=ORIENTED_EDGE('',*,*,#48900,.F.) ;
#68643=ORIENTED_EDGE('',*,*,#48901,.F.) ;
#68644=ORIENTED_EDGE('',*,*,#48902,.F.) ;
#68645=ORIENTED_EDGE('',*,*,#48903,.F.) ;
#68646=ORIENTED_EDGE('',*,*,#48904,.T.) ;
#68647=ORIENTED_EDGE('',*,*,#48905,.F.) ;
#68648=ORIENTED_EDGE('',*,*,#48906,.F.) ;
#68649=ORIENTED_EDGE('',*,*,#48907,.F.) ;
#68650=ORIENTED_EDGE('',*,*,#48908,.T.) ;
#68651=ORIENTED_EDGE('',*,*,#48909,.F.) ;
#68652=ORIENTED_EDGE('',*,*,#48910,.T.) ;
#68653=ORIENTED_EDGE('',*,*,#48911,.F.) ;
#68654=ORIENTED_EDGE('',*,*,#48912,.F.) ;
#68655=ORIENTED_EDGE('',*,*,#48913,.F.) ;
#68656=ORIENTED_EDGE('',*,*,#48914,.F.) ;
#68657=ORIENTED_EDGE('',*,*,#48915,.F.) ;
#68658=ORIENTED_EDGE('',*,*,#48916,.T.) ;
#68659=ORIENTED_EDGE('',*,*,#48917,.F.) ;
#68660=ORIENTED_EDGE('',*,*,#48918,.T.) ;
#68661=ORIENTED_EDGE('',*,*,#48919,.F.) ;
#68662=ORIENTED_EDGE('',*,*,#48920,.F.) ;
#68663=ORIENTED_EDGE('',*,*,#48921,.F.) ;
#68664=ORIENTED_EDGE('',*,*,#48922,.F.) ;
#68665=ORIENTED_EDGE('',*,*,#48923,.F.) ;
#68666=ORIENTED_EDGE('',*,*,#48924,.T.) ;
#68667=ORIENTED_EDGE('',*,*,#48925,.F.) ;
#68668=ORIENTED_EDGE('',*,*,#48926,.T.) ;
#68669=ORIENTED_EDGE('',*,*,#48927,.F.) ;
#68670=ORIENTED_EDGE('',*,*,#48928,.F.) ;
#68671=ORIENTED_EDGE('',*,*,#48929,.F.) ;
#68672=ORIENTED_EDGE('',*,*,#48930,.F.) ;
#68673=ORIENTED_EDGE('',*,*,#48931,.F.) ;
#68674=ORIENTED_EDGE('',*,*,#48932,.T.) ;
#68675=ORIENTED_EDGE('',*,*,#48933,.F.) ;
#68676=ORIENTED_EDGE('',*,*,#48934,.T.) ;
#68677=ORIENTED_EDGE('',*,*,#48935,.F.) ;
#68678=ORIENTED_EDGE('',*,*,#48936,.F.) ;
#68679=ORIENTED_EDGE('',*,*,#48937,.F.) ;
#68680=ORIENTED_EDGE('',*,*,#48938,.F.) ;
#68681=ORIENTED_EDGE('',*,*,#48939,.F.) ;
#68682=ORIENTED_EDGE('',*,*,#48940,.T.) ;
#68683=ORIENTED_EDGE('',*,*,#48941,.F.) ;
#68684=ORIENTED_EDGE('',*,*,#48942,.T.) ;
#68685=ORIENTED_EDGE('',*,*,#48943,.F.) ;
#68686=ORIENTED_EDGE('',*,*,#48944,.F.) ;
#68687=ORIENTED_EDGE('',*,*,#48945,.F.) ;
#68688=ORIENTED_EDGE('',*,*,#48946,.F.) ;
#68689=ORIENTED_EDGE('',*,*,#48947,.F.) ;
#68690=ORIENTED_EDGE('',*,*,#48948,.T.) ;
#68691=ORIENTED_EDGE('',*,*,#48949,.F.) ;
#68692=ORIENTED_EDGE('',*,*,#48950,.T.) ;
#68693=ORIENTED_EDGE('',*,*,#48951,.F.) ;
#68694=ORIENTED_EDGE('',*,*,#48952,.F.) ;
#68695=ORIENTED_EDGE('',*,*,#48953,.F.) ;
#68696=ORIENTED_EDGE('',*,*,#48954,.F.) ;
#68697=ORIENTED_EDGE('',*,*,#48955,.F.) ;
#68698=ORIENTED_EDGE('',*,*,#48956,.T.) ;
#68699=ORIENTED_EDGE('',*,*,#48957,.F.) ;
#68700=ORIENTED_EDGE('',*,*,#48958,.T.) ;
#68701=ORIENTED_EDGE('',*,*,#48959,.F.) ;
#68702=ORIENTED_EDGE('',*,*,#48960,.F.) ;
#68703=ORIENTED_EDGE('',*,*,#48961,.F.) ;
#68704=ORIENTED_EDGE('',*,*,#48962,.F.) ;
#68705=ORIENTED_EDGE('',*,*,#48963,.F.) ;
#68706=ORIENTED_EDGE('',*,*,#48964,.T.) ;
#68707=ORIENTED_EDGE('',*,*,#48965,.F.) ;
#68708=ORIENTED_EDGE('',*,*,#48966,.T.) ;
#68709=ORIENTED_EDGE('',*,*,#48967,.F.) ;
#68710=ORIENTED_EDGE('',*,*,#48968,.F.) ;
#68711=ORIENTED_EDGE('',*,*,#48969,.F.) ;
#68712=ORIENTED_EDGE('',*,*,#48970,.F.) ;
#68713=ORIENTED_EDGE('',*,*,#48971,.F.) ;
#68714=ORIENTED_EDGE('',*,*,#48972,.T.) ;
#68715=ORIENTED_EDGE('',*,*,#48973,.F.) ;
#68716=ORIENTED_EDGE('',*,*,#48974,.T.) ;
#68717=ORIENTED_EDGE('',*,*,#48975,.F.) ;
#68718=ORIENTED_EDGE('',*,*,#48976,.F.) ;
#68719=ORIENTED_EDGE('',*,*,#48977,.F.) ;
#68720=ORIENTED_EDGE('',*,*,#48978,.F.) ;
#68721=ORIENTED_EDGE('',*,*,#48979,.F.) ;
#68722=ORIENTED_EDGE('',*,*,#48980,.T.) ;
#68723=ORIENTED_EDGE('',*,*,#48981,.F.) ;
#68724=ORIENTED_EDGE('',*,*,#48982,.T.) ;
#68725=ORIENTED_EDGE('',*,*,#48983,.F.) ;
#68726=ORIENTED_EDGE('',*,*,#48984,.F.) ;
#68727=ORIENTED_EDGE('',*,*,#48985,.T.) ;
#68728=ORIENTED_EDGE('',*,*,#48986,.T.) ;
#68729=ORIENTED_EDGE('',*,*,#48963,.T.) ;
#68730=ORIENTED_EDGE('',*,*,#48987,.F.) ;
#68731=ORIENTED_EDGE('',*,*,#48988,.T.) ;
#68732=ORIENTED_EDGE('',*,*,#48989,.T.) ;
#68733=ORIENTED_EDGE('',*,*,#48955,.T.) ;
#68734=ORIENTED_EDGE('',*,*,#48990,.F.) ;
#68735=ORIENTED_EDGE('',*,*,#48991,.T.) ;
#68736=ORIENTED_EDGE('',*,*,#48992,.T.) ;
#68737=ORIENTED_EDGE('',*,*,#48947,.T.) ;
#68738=ORIENTED_EDGE('',*,*,#48993,.F.) ;
#68739=ORIENTED_EDGE('',*,*,#48994,.T.) ;
#68740=ORIENTED_EDGE('',*,*,#48995,.T.) ;
#68741=ORIENTED_EDGE('',*,*,#48939,.T.) ;
#68742=ORIENTED_EDGE('',*,*,#48996,.F.) ;
#68743=ORIENTED_EDGE('',*,*,#48997,.T.) ;
#68744=ORIENTED_EDGE('',*,*,#48998,.T.) ;
#68745=ORIENTED_EDGE('',*,*,#48931,.T.) ;
#68746=ORIENTED_EDGE('',*,*,#48999,.F.) ;
#68747=ORIENTED_EDGE('',*,*,#49000,.T.) ;
#68748=ORIENTED_EDGE('',*,*,#49001,.T.) ;
#68749=ORIENTED_EDGE('',*,*,#48923,.T.) ;
#68750=ORIENTED_EDGE('',*,*,#49002,.F.) ;
#68751=ORIENTED_EDGE('',*,*,#49003,.T.) ;
#68752=ORIENTED_EDGE('',*,*,#49004,.T.) ;
#68753=ORIENTED_EDGE('',*,*,#48915,.T.) ;
#68754=ORIENTED_EDGE('',*,*,#49005,.F.) ;
#68755=ORIENTED_EDGE('',*,*,#49006,.F.) ;
#68756=ORIENTED_EDGE('',*,*,#49007,.T.) ;
#68757=ORIENTED_EDGE('',*,*,#49008,.F.) ;
#68758=ORIENTED_EDGE('',*,*,#49007,.F.) ;
#68759=ORIENTED_EDGE('',*,*,#49009,.F.) ;
#68760=ORIENTED_EDGE('',*,*,#49010,.T.) ;
#68761=ORIENTED_EDGE('',*,*,#49011,.F.) ;
#68762=ORIENTED_EDGE('',*,*,#49010,.F.) ;
#68763=ORIENTED_EDGE('',*,*,#49012,.F.) ;
#68764=ORIENTED_EDGE('',*,*,#49013,.T.) ;
#68765=ORIENTED_EDGE('',*,*,#49014,.F.) ;
#68766=ORIENTED_EDGE('',*,*,#49013,.F.) ;
#68767=ORIENTED_EDGE('',*,*,#49015,.F.) ;
#68768=ORIENTED_EDGE('',*,*,#49016,.T.) ;
#68769=ORIENTED_EDGE('',*,*,#49017,.F.) ;
#68770=ORIENTED_EDGE('',*,*,#49016,.F.) ;
#68771=ORIENTED_EDGE('',*,*,#49018,.F.) ;
#68772=ORIENTED_EDGE('',*,*,#49019,.T.) ;
#68773=ORIENTED_EDGE('',*,*,#49020,.F.) ;
#68774=ORIENTED_EDGE('',*,*,#49019,.F.) ;
#68775=ORIENTED_EDGE('',*,*,#49021,.F.) ;
#68776=ORIENTED_EDGE('',*,*,#49022,.T.) ;
#68777=ORIENTED_EDGE('',*,*,#49023,.F.) ;
#68778=ORIENTED_EDGE('',*,*,#49022,.F.) ;
#68779=ORIENTED_EDGE('',*,*,#49024,.F.) ;
#68780=ORIENTED_EDGE('',*,*,#49025,.T.) ;
#68781=ORIENTED_EDGE('',*,*,#49026,.F.) ;
#68782=ORIENTED_EDGE('',*,*,#49025,.F.) ;
#68783=ORIENTED_EDGE('',*,*,#49027,.F.) ;
#68784=ORIENTED_EDGE('',*,*,#49028,.T.) ;
#68785=ORIENTED_EDGE('',*,*,#49029,.F.) ;
#68786=ORIENTED_EDGE('',*,*,#49028,.F.) ;
#68787=ORIENTED_EDGE('',*,*,#49030,.F.) ;
#68788=ORIENTED_EDGE('',*,*,#49031,.T.) ;
#68789=ORIENTED_EDGE('',*,*,#49032,.F.) ;
#68790=ORIENTED_EDGE('',*,*,#49031,.F.) ;
#68791=ORIENTED_EDGE('',*,*,#49033,.F.) ;
#68792=ORIENTED_EDGE('',*,*,#49034,.T.) ;
#68793=ORIENTED_EDGE('',*,*,#49035,.F.) ;
#68794=ORIENTED_EDGE('',*,*,#49034,.F.) ;
#68795=ORIENTED_EDGE('',*,*,#49036,.F.) ;
#68796=ORIENTED_EDGE('',*,*,#49037,.T.) ;
#68797=ORIENTED_EDGE('',*,*,#49038,.F.) ;
#68798=ORIENTED_EDGE('',*,*,#49037,.F.) ;
#68799=ORIENTED_EDGE('',*,*,#49039,.F.) ;
#68800=ORIENTED_EDGE('',*,*,#49040,.T.) ;
#68801=ORIENTED_EDGE('',*,*,#49041,.F.) ;
#68802=ORIENTED_EDGE('',*,*,#49040,.F.) ;
#68803=ORIENTED_EDGE('',*,*,#49042,.F.) ;
#68804=ORIENTED_EDGE('',*,*,#49043,.T.) ;
#68805=ORIENTED_EDGE('',*,*,#49044,.F.) ;
#68806=ORIENTED_EDGE('',*,*,#49043,.F.) ;
#68807=ORIENTED_EDGE('',*,*,#49045,.F.) ;
#68808=ORIENTED_EDGE('',*,*,#49046,.T.) ;
#68809=ORIENTED_EDGE('',*,*,#49047,.F.) ;
#68810=ORIENTED_EDGE('',*,*,#49046,.F.) ;
#68811=ORIENTED_EDGE('',*,*,#49048,.F.) ;
#68812=ORIENTED_EDGE('',*,*,#49049,.T.) ;
#68813=ORIENTED_EDGE('',*,*,#49050,.F.) ;
#68814=ORIENTED_EDGE('',*,*,#49049,.F.) ;
#68815=ORIENTED_EDGE('',*,*,#49051,.F.) ;
#68816=ORIENTED_EDGE('',*,*,#49052,.T.) ;
#68817=ORIENTED_EDGE('',*,*,#49053,.F.) ;
#68818=ORIENTED_EDGE('',*,*,#49052,.F.) ;
#68819=ORIENTED_EDGE('',*,*,#49054,.F.) ;
#68820=ORIENTED_EDGE('',*,*,#49055,.T.) ;
#68821=ORIENTED_EDGE('',*,*,#49056,.F.) ;
#68822=ORIENTED_EDGE('',*,*,#49055,.F.) ;
#68823=ORIENTED_EDGE('',*,*,#49057,.F.) ;
#68824=ORIENTED_EDGE('',*,*,#49058,.T.) ;
#68825=ORIENTED_EDGE('',*,*,#49059,.F.) ;
#68826=ORIENTED_EDGE('',*,*,#49058,.F.) ;
#68827=ORIENTED_EDGE('',*,*,#49060,.F.) ;
#68828=ORIENTED_EDGE('',*,*,#49061,.T.) ;
#68829=ORIENTED_EDGE('',*,*,#49062,.F.) ;
#68830=ORIENTED_EDGE('',*,*,#49061,.F.) ;
#68831=ORIENTED_EDGE('',*,*,#49063,.F.) ;
#68832=ORIENTED_EDGE('',*,*,#49064,.T.) ;
#68833=ORIENTED_EDGE('',*,*,#49065,.F.) ;
#68834=ORIENTED_EDGE('',*,*,#49064,.F.) ;
#68835=ORIENTED_EDGE('',*,*,#49066,.F.) ;
#68836=ORIENTED_EDGE('',*,*,#49067,.T.) ;
#68837=ORIENTED_EDGE('',*,*,#49068,.F.) ;
#68838=ORIENTED_EDGE('',*,*,#49067,.F.) ;
#68839=ORIENTED_EDGE('',*,*,#49069,.F.) ;
#68840=ORIENTED_EDGE('',*,*,#49070,.T.) ;
#68841=ORIENTED_EDGE('',*,*,#49071,.F.) ;
#68842=ORIENTED_EDGE('',*,*,#49070,.F.) ;
#68843=ORIENTED_EDGE('',*,*,#49072,.F.) ;
#68844=ORIENTED_EDGE('',*,*,#49073,.T.) ;
#68845=ORIENTED_EDGE('',*,*,#49074,.F.) ;
#68846=ORIENTED_EDGE('',*,*,#49073,.F.) ;
#68847=ORIENTED_EDGE('',*,*,#49075,.F.) ;
#68848=ORIENTED_EDGE('',*,*,#49076,.T.) ;
#68849=ORIENTED_EDGE('',*,*,#49077,.F.) ;
#68850=ORIENTED_EDGE('',*,*,#49076,.F.) ;
#68851=ORIENTED_EDGE('',*,*,#49078,.F.) ;
#68852=ORIENTED_EDGE('',*,*,#49079,.T.) ;
#68853=ORIENTED_EDGE('',*,*,#49080,.F.) ;
#68854=ORIENTED_EDGE('',*,*,#49079,.F.) ;
#68855=ORIENTED_EDGE('',*,*,#49081,.F.) ;
#68856=ORIENTED_EDGE('',*,*,#49082,.T.) ;
#68857=ORIENTED_EDGE('',*,*,#49083,.F.) ;
#68858=ORIENTED_EDGE('',*,*,#49082,.F.) ;
#68859=ORIENTED_EDGE('',*,*,#49084,.F.) ;
#68860=ORIENTED_EDGE('',*,*,#49085,.T.) ;
#68861=ORIENTED_EDGE('',*,*,#49086,.F.) ;
#68862=ORIENTED_EDGE('',*,*,#49085,.F.) ;
#68863=ORIENTED_EDGE('',*,*,#49087,.F.) ;
#68864=ORIENTED_EDGE('',*,*,#49088,.T.) ;
#68865=ORIENTED_EDGE('',*,*,#49089,.F.) ;
#68866=ORIENTED_EDGE('',*,*,#49090,.T.) ;
#68867=ORIENTED_EDGE('',*,*,#49091,.F.) ;
#68868=ORIENTED_EDGE('',*,*,#49092,.T.) ;
#68869=ORIENTED_EDGE('',*,*,#49093,.T.) ;
#68870=ORIENTED_EDGE('',*,*,#49094,.T.) ;
#68871=ORIENTED_EDGE('',*,*,#49095,.F.) ;
#68872=ORIENTED_EDGE('',*,*,#49096,.T.) ;
#68873=ORIENTED_EDGE('',*,*,#49097,.F.) ;
#68874=ORIENTED_EDGE('',*,*,#49098,.T.) ;
#68875=ORIENTED_EDGE('',*,*,#49099,.F.) ;
#68876=ORIENTED_EDGE('',*,*,#49100,.T.) ;
#68877=ORIENTED_EDGE('',*,*,#49101,.T.) ;
#68878=ORIENTED_EDGE('',*,*,#49102,.T.) ;
#68879=ORIENTED_EDGE('',*,*,#49103,.F.) ;
#68880=ORIENTED_EDGE('',*,*,#49104,.T.) ;
#68881=ORIENTED_EDGE('',*,*,#49081,.T.) ;
#68882=ORIENTED_EDGE('',*,*,#49104,.F.) ;
#68883=ORIENTED_EDGE('',*,*,#49105,.F.) ;
#68884=ORIENTED_EDGE('',*,*,#49106,.T.) ;
#68885=ORIENTED_EDGE('',*,*,#49107,.F.) ;
#68886=ORIENTED_EDGE('',*,*,#49108,.T.) ;
#68887=ORIENTED_EDGE('',*,*,#49109,.F.) ;
#68888=ORIENTED_EDGE('',*,*,#49110,.T.) ;
#68889=ORIENTED_EDGE('',*,*,#49111,.T.) ;
#68890=ORIENTED_EDGE('',*,*,#49112,.T.) ;
#68891=ORIENTED_EDGE('',*,*,#49113,.F.) ;
#68892=ORIENTED_EDGE('',*,*,#49114,.T.) ;
#68893=ORIENTED_EDGE('',*,*,#49115,.F.) ;
#68894=ORIENTED_EDGE('',*,*,#49116,.T.) ;
#68895=ORIENTED_EDGE('',*,*,#49117,.F.) ;
#68896=ORIENTED_EDGE('',*,*,#49118,.T.) ;
#68897=ORIENTED_EDGE('',*,*,#49119,.T.) ;
#68898=ORIENTED_EDGE('',*,*,#49120,.T.) ;
#68899=ORIENTED_EDGE('',*,*,#49121,.F.) ;
#68900=ORIENTED_EDGE('',*,*,#49122,.T.) ;
#68901=ORIENTED_EDGE('',*,*,#49072,.T.) ;
#68902=ORIENTED_EDGE('',*,*,#49122,.F.) ;
#68903=ORIENTED_EDGE('',*,*,#49123,.F.) ;
#68904=ORIENTED_EDGE('',*,*,#49124,.T.) ;
#68905=ORIENTED_EDGE('',*,*,#49125,.F.) ;
#68906=ORIENTED_EDGE('',*,*,#49126,.T.) ;
#68907=ORIENTED_EDGE('',*,*,#49127,.F.) ;
#68908=ORIENTED_EDGE('',*,*,#49128,.T.) ;
#68909=ORIENTED_EDGE('',*,*,#49129,.T.) ;
#68910=ORIENTED_EDGE('',*,*,#49130,.T.) ;
#68911=ORIENTED_EDGE('',*,*,#49131,.F.) ;
#68912=ORIENTED_EDGE('',*,*,#49132,.T.) ;
#68913=ORIENTED_EDGE('',*,*,#49133,.F.) ;
#68914=ORIENTED_EDGE('',*,*,#49134,.T.) ;
#68915=ORIENTED_EDGE('',*,*,#49135,.F.) ;
#68916=ORIENTED_EDGE('',*,*,#49136,.T.) ;
#68917=ORIENTED_EDGE('',*,*,#49137,.T.) ;
#68918=ORIENTED_EDGE('',*,*,#49138,.T.) ;
#68919=ORIENTED_EDGE('',*,*,#49139,.F.) ;
#68920=ORIENTED_EDGE('',*,*,#49140,.T.) ;
#68921=ORIENTED_EDGE('',*,*,#49063,.T.) ;
#68922=ORIENTED_EDGE('',*,*,#49140,.F.) ;
#68923=ORIENTED_EDGE('',*,*,#49141,.F.) ;
#68924=ORIENTED_EDGE('',*,*,#49142,.T.) ;
#68925=ORIENTED_EDGE('',*,*,#49143,.F.) ;
#68926=ORIENTED_EDGE('',*,*,#49144,.T.) ;
#68927=ORIENTED_EDGE('',*,*,#49145,.F.) ;
#68928=ORIENTED_EDGE('',*,*,#49146,.T.) ;
#68929=ORIENTED_EDGE('',*,*,#49147,.T.) ;
#68930=ORIENTED_EDGE('',*,*,#49148,.T.) ;
#68931=ORIENTED_EDGE('',*,*,#49149,.F.) ;
#68932=ORIENTED_EDGE('',*,*,#49150,.T.) ;
#68933=ORIENTED_EDGE('',*,*,#49151,.F.) ;
#68934=ORIENTED_EDGE('',*,*,#49152,.T.) ;
#68935=ORIENTED_EDGE('',*,*,#49153,.F.) ;
#68936=ORIENTED_EDGE('',*,*,#49154,.T.) ;
#68937=ORIENTED_EDGE('',*,*,#49155,.T.) ;
#68938=ORIENTED_EDGE('',*,*,#49156,.T.) ;
#68939=ORIENTED_EDGE('',*,*,#49157,.F.) ;
#68940=ORIENTED_EDGE('',*,*,#49158,.T.) ;
#68941=ORIENTED_EDGE('',*,*,#49054,.T.) ;
#68942=ORIENTED_EDGE('',*,*,#49158,.F.) ;
#68943=ORIENTED_EDGE('',*,*,#49159,.F.) ;
#68944=ORIENTED_EDGE('',*,*,#49160,.T.) ;
#68945=ORIENTED_EDGE('',*,*,#49161,.F.) ;
#68946=ORIENTED_EDGE('',*,*,#49162,.T.) ;
#68947=ORIENTED_EDGE('',*,*,#49163,.F.) ;
#68948=ORIENTED_EDGE('',*,*,#49164,.T.) ;
#68949=ORIENTED_EDGE('',*,*,#49165,.T.) ;
#68950=ORIENTED_EDGE('',*,*,#49166,.T.) ;
#68951=ORIENTED_EDGE('',*,*,#49167,.F.) ;
#68952=ORIENTED_EDGE('',*,*,#49168,.T.) ;
#68953=ORIENTED_EDGE('',*,*,#49169,.F.) ;
#68954=ORIENTED_EDGE('',*,*,#49170,.T.) ;
#68955=ORIENTED_EDGE('',*,*,#49171,.F.) ;
#68956=ORIENTED_EDGE('',*,*,#49172,.T.) ;
#68957=ORIENTED_EDGE('',*,*,#49173,.T.) ;
#68958=ORIENTED_EDGE('',*,*,#49174,.T.) ;
#68959=ORIENTED_EDGE('',*,*,#49175,.F.) ;
#68960=ORIENTED_EDGE('',*,*,#49176,.T.) ;
#68961=ORIENTED_EDGE('',*,*,#49045,.T.) ;
#68962=ORIENTED_EDGE('',*,*,#49176,.F.) ;
#68963=ORIENTED_EDGE('',*,*,#49177,.F.) ;
#68964=ORIENTED_EDGE('',*,*,#49178,.T.) ;
#68965=ORIENTED_EDGE('',*,*,#49179,.F.) ;
#68966=ORIENTED_EDGE('',*,*,#49180,.T.) ;
#68967=ORIENTED_EDGE('',*,*,#49181,.F.) ;
#68968=ORIENTED_EDGE('',*,*,#49182,.T.) ;
#68969=ORIENTED_EDGE('',*,*,#49183,.T.) ;
#68970=ORIENTED_EDGE('',*,*,#49184,.T.) ;
#68971=ORIENTED_EDGE('',*,*,#49185,.F.) ;
#68972=ORIENTED_EDGE('',*,*,#49186,.T.) ;
#68973=ORIENTED_EDGE('',*,*,#49187,.F.) ;
#68974=ORIENTED_EDGE('',*,*,#49188,.T.) ;
#68975=ORIENTED_EDGE('',*,*,#49189,.F.) ;
#68976=ORIENTED_EDGE('',*,*,#49190,.T.) ;
#68977=ORIENTED_EDGE('',*,*,#49191,.T.) ;
#68978=ORIENTED_EDGE('',*,*,#49192,.T.) ;
#68979=ORIENTED_EDGE('',*,*,#49193,.F.) ;
#68980=ORIENTED_EDGE('',*,*,#49194,.T.) ;
#68981=ORIENTED_EDGE('',*,*,#49036,.T.) ;
#68982=ORIENTED_EDGE('',*,*,#49194,.F.) ;
#68983=ORIENTED_EDGE('',*,*,#49195,.F.) ;
#68984=ORIENTED_EDGE('',*,*,#49196,.T.) ;
#68985=ORIENTED_EDGE('',*,*,#49197,.F.) ;
#68986=ORIENTED_EDGE('',*,*,#49198,.T.) ;
#68987=ORIENTED_EDGE('',*,*,#49199,.F.) ;
#68988=ORIENTED_EDGE('',*,*,#49200,.T.) ;
#68989=ORIENTED_EDGE('',*,*,#49201,.T.) ;
#68990=ORIENTED_EDGE('',*,*,#49202,.T.) ;
#68991=ORIENTED_EDGE('',*,*,#49203,.F.) ;
#68992=ORIENTED_EDGE('',*,*,#49204,.T.) ;
#68993=ORIENTED_EDGE('',*,*,#49205,.F.) ;
#68994=ORIENTED_EDGE('',*,*,#49206,.T.) ;
#68995=ORIENTED_EDGE('',*,*,#49207,.F.) ;
#68996=ORIENTED_EDGE('',*,*,#49208,.T.) ;
#68997=ORIENTED_EDGE('',*,*,#49209,.T.) ;
#68998=ORIENTED_EDGE('',*,*,#49210,.T.) ;
#68999=ORIENTED_EDGE('',*,*,#49211,.F.) ;
#69000=ORIENTED_EDGE('',*,*,#49212,.T.) ;
#69001=ORIENTED_EDGE('',*,*,#49027,.T.) ;
#69002=ORIENTED_EDGE('',*,*,#49212,.F.) ;
#69003=ORIENTED_EDGE('',*,*,#49213,.F.) ;
#69004=ORIENTED_EDGE('',*,*,#49214,.T.) ;
#69005=ORIENTED_EDGE('',*,*,#49215,.F.) ;
#69006=ORIENTED_EDGE('',*,*,#49216,.T.) ;
#69007=ORIENTED_EDGE('',*,*,#49217,.F.) ;
#69008=ORIENTED_EDGE('',*,*,#49218,.T.) ;
#69009=ORIENTED_EDGE('',*,*,#49219,.T.) ;
#69010=ORIENTED_EDGE('',*,*,#49220,.T.) ;
#69011=ORIENTED_EDGE('',*,*,#49221,.F.) ;
#69012=ORIENTED_EDGE('',*,*,#49222,.T.) ;
#69013=ORIENTED_EDGE('',*,*,#49223,.F.) ;
#69014=ORIENTED_EDGE('',*,*,#49224,.T.) ;
#69015=ORIENTED_EDGE('',*,*,#49225,.F.) ;
#69016=ORIENTED_EDGE('',*,*,#49226,.T.) ;
#69017=ORIENTED_EDGE('',*,*,#49227,.T.) ;
#69018=ORIENTED_EDGE('',*,*,#49228,.T.) ;
#69019=ORIENTED_EDGE('',*,*,#49229,.F.) ;
#69020=ORIENTED_EDGE('',*,*,#49230,.T.) ;
#69021=ORIENTED_EDGE('',*,*,#49018,.T.) ;
#69022=ORIENTED_EDGE('',*,*,#49230,.F.) ;
#69023=ORIENTED_EDGE('',*,*,#49231,.F.) ;
#69024=ORIENTED_EDGE('',*,*,#49232,.T.) ;
#69025=ORIENTED_EDGE('',*,*,#49233,.F.) ;
#69026=ORIENTED_EDGE('',*,*,#49234,.T.) ;
#69027=ORIENTED_EDGE('',*,*,#49235,.F.) ;
#69028=ORIENTED_EDGE('',*,*,#49236,.T.) ;
#69029=ORIENTED_EDGE('',*,*,#49237,.T.) ;
#69030=ORIENTED_EDGE('',*,*,#49238,.T.) ;
#69031=ORIENTED_EDGE('',*,*,#49239,.F.) ;
#69032=ORIENTED_EDGE('',*,*,#49240,.T.) ;
#69033=ORIENTED_EDGE('',*,*,#49241,.F.) ;
#69034=ORIENTED_EDGE('',*,*,#49242,.T.) ;
#69035=ORIENTED_EDGE('',*,*,#49243,.F.) ;
#69036=ORIENTED_EDGE('',*,*,#49244,.T.) ;
#69037=ORIENTED_EDGE('',*,*,#49245,.T.) ;
#69038=ORIENTED_EDGE('',*,*,#49246,.T.) ;
#69039=ORIENTED_EDGE('',*,*,#49247,.F.) ;
#69040=ORIENTED_EDGE('',*,*,#49248,.T.) ;
#69041=ORIENTED_EDGE('',*,*,#49009,.T.) ;
#69042=ORIENTED_EDGE('',*,*,#49248,.F.) ;
#69043=ORIENTED_EDGE('',*,*,#49249,.F.) ;
#69044=ORIENTED_EDGE('',*,*,#49250,.T.) ;
#69045=ORIENTED_EDGE('',*,*,#49006,.T.) ;
#69046=ORIENTED_EDGE('',*,*,#49250,.F.) ;
#69047=ORIENTED_EDGE('',*,*,#49251,.F.) ;
#69048=ORIENTED_EDGE('',*,*,#49252,.T.) ;
#69049=ORIENTED_EDGE('',*,*,#49015,.T.) ;
#69050=ORIENTED_EDGE('',*,*,#49252,.F.) ;
#69051=ORIENTED_EDGE('',*,*,#49253,.F.) ;
#69052=ORIENTED_EDGE('',*,*,#49254,.T.) ;
#69053=ORIENTED_EDGE('',*,*,#49024,.T.) ;
#69054=ORIENTED_EDGE('',*,*,#49254,.F.) ;
#69055=ORIENTED_EDGE('',*,*,#49255,.F.) ;
#69056=ORIENTED_EDGE('',*,*,#49256,.T.) ;
#69057=ORIENTED_EDGE('',*,*,#49033,.T.) ;
#69058=ORIENTED_EDGE('',*,*,#49256,.F.) ;
#69059=ORIENTED_EDGE('',*,*,#49257,.F.) ;
#69060=ORIENTED_EDGE('',*,*,#49258,.T.) ;
#69061=ORIENTED_EDGE('',*,*,#49042,.T.) ;
#69062=ORIENTED_EDGE('',*,*,#49258,.F.) ;
#69063=ORIENTED_EDGE('',*,*,#49259,.F.) ;
#69064=ORIENTED_EDGE('',*,*,#49260,.T.) ;
#69065=ORIENTED_EDGE('',*,*,#49051,.T.) ;
#69066=ORIENTED_EDGE('',*,*,#49260,.F.) ;
#69067=ORIENTED_EDGE('',*,*,#49261,.F.) ;
#69068=ORIENTED_EDGE('',*,*,#49262,.T.) ;
#69069=ORIENTED_EDGE('',*,*,#49060,.T.) ;
#69070=ORIENTED_EDGE('',*,*,#49262,.F.) ;
#69071=ORIENTED_EDGE('',*,*,#49263,.F.) ;
#69072=ORIENTED_EDGE('',*,*,#49264,.T.) ;
#69073=ORIENTED_EDGE('',*,*,#49069,.T.) ;
#69074=ORIENTED_EDGE('',*,*,#49264,.F.) ;
#69075=ORIENTED_EDGE('',*,*,#49265,.F.) ;
#69076=ORIENTED_EDGE('',*,*,#49266,.T.) ;
#69077=ORIENTED_EDGE('',*,*,#49078,.T.) ;
#69078=ORIENTED_EDGE('',*,*,#49266,.F.) ;
#69079=ORIENTED_EDGE('',*,*,#49080,.T.) ;
#69080=ORIENTED_EDGE('',*,*,#49267,.T.) ;
#69081=ORIENTED_EDGE('',*,*,#49084,.T.) ;
#69082=ORIENTED_EDGE('',*,*,#49267,.F.) ;
#69083=ORIENTED_EDGE('',*,*,#49071,.T.) ;
#69084=ORIENTED_EDGE('',*,*,#49268,.T.) ;
#69085=ORIENTED_EDGE('',*,*,#49075,.T.) ;
#69086=ORIENTED_EDGE('',*,*,#49268,.F.) ;
#69087=ORIENTED_EDGE('',*,*,#49062,.T.) ;
#69088=ORIENTED_EDGE('',*,*,#49269,.T.) ;
#69089=ORIENTED_EDGE('',*,*,#49066,.T.) ;
#69090=ORIENTED_EDGE('',*,*,#49269,.F.) ;
#69091=ORIENTED_EDGE('',*,*,#49053,.T.) ;
#69092=ORIENTED_EDGE('',*,*,#49270,.T.) ;
#69093=ORIENTED_EDGE('',*,*,#49057,.T.) ;
#69094=ORIENTED_EDGE('',*,*,#49270,.F.) ;
#69095=ORIENTED_EDGE('',*,*,#49044,.T.) ;
#69096=ORIENTED_EDGE('',*,*,#49271,.T.) ;
#69097=ORIENTED_EDGE('',*,*,#49048,.T.) ;
#69098=ORIENTED_EDGE('',*,*,#49271,.F.) ;
#69099=ORIENTED_EDGE('',*,*,#49035,.T.) ;
#69100=ORIENTED_EDGE('',*,*,#49272,.T.) ;
#69101=ORIENTED_EDGE('',*,*,#49039,.T.) ;
#69102=ORIENTED_EDGE('',*,*,#49272,.F.) ;
#69103=ORIENTED_EDGE('',*,*,#49026,.T.) ;
#69104=ORIENTED_EDGE('',*,*,#49273,.T.) ;
#69105=ORIENTED_EDGE('',*,*,#49030,.T.) ;
#69106=ORIENTED_EDGE('',*,*,#49273,.F.) ;
#69107=ORIENTED_EDGE('',*,*,#49017,.T.) ;
#69108=ORIENTED_EDGE('',*,*,#49274,.T.) ;
#69109=ORIENTED_EDGE('',*,*,#49021,.T.) ;
#69110=ORIENTED_EDGE('',*,*,#49274,.F.) ;
#69111=ORIENTED_EDGE('',*,*,#49008,.T.) ;
#69112=ORIENTED_EDGE('',*,*,#49275,.T.) ;
#69113=ORIENTED_EDGE('',*,*,#49012,.T.) ;
#69114=ORIENTED_EDGE('',*,*,#49275,.F.) ;
#69115=ORIENTED_EDGE('',*,*,#49276,.F.) ;
#69116=ORIENTED_EDGE('',*,*,#49277,.T.) ;
#69117=ORIENTED_EDGE('',*,*,#49278,.F.) ;
#69118=ORIENTED_EDGE('',*,*,#49277,.F.) ;
#69119=ORIENTED_EDGE('',*,*,#49279,.F.) ;
#69120=ORIENTED_EDGE('',*,*,#49280,.T.) ;
#69121=ORIENTED_EDGE('',*,*,#49281,.F.) ;
#69122=ORIENTED_EDGE('',*,*,#49280,.F.) ;
#69123=ORIENTED_EDGE('',*,*,#49282,.F.) ;
#69124=ORIENTED_EDGE('',*,*,#49283,.T.) ;
#69125=ORIENTED_EDGE('',*,*,#49284,.F.) ;
#69126=ORIENTED_EDGE('',*,*,#49283,.F.) ;
#69127=ORIENTED_EDGE('',*,*,#49285,.T.) ;
#69128=ORIENTED_EDGE('',*,*,#49286,.T.) ;
#69129=ORIENTED_EDGE('',*,*,#48971,.T.) ;
#69130=ORIENTED_EDGE('',*,*,#49287,.F.) ;
#69131=ORIENTED_EDGE('',*,*,#49288,.T.) ;
#69132=ORIENTED_EDGE('',*,*,#49289,.T.) ;
#69133=ORIENTED_EDGE('',*,*,#48979,.T.) ;
#69134=ORIENTED_EDGE('',*,*,#49290,.F.) ;
#69135=ORIENTED_EDGE('',*,*,#49291,.T.) ;
#69136=ORIENTED_EDGE('',*,*,#49292,.T.) ;
#69137=ORIENTED_EDGE('',*,*,#48903,.T.) ;
#69138=ORIENTED_EDGE('',*,*,#49293,.F.) ;
#69139=ORIENTED_EDGE('',*,*,#49294,.T.) ;
#69140=ORIENTED_EDGE('',*,*,#49295,.T.) ;
#69141=ORIENTED_EDGE('',*,*,#48907,.T.) ;
#69142=ORIENTED_EDGE('',*,*,#49296,.F.) ;
#69143=ORIENTED_EDGE('',*,*,#49297,.F.) ;
#69144=ORIENTED_EDGE('',*,*,#49298,.T.) ;
#69145=ORIENTED_EDGE('',*,*,#49299,.F.) ;
#69146=ORIENTED_EDGE('',*,*,#49300,.T.) ;
#69147=ORIENTED_EDGE('',*,*,#49301,.F.) ;
#69148=ORIENTED_EDGE('',*,*,#49302,.T.) ;
#69149=ORIENTED_EDGE('',*,*,#49303,.T.) ;
#69150=ORIENTED_EDGE('',*,*,#49304,.T.) ;
#69151=ORIENTED_EDGE('',*,*,#49305,.F.) ;
#69152=ORIENTED_EDGE('',*,*,#49306,.T.) ;
#69153=ORIENTED_EDGE('',*,*,#49307,.F.) ;
#69154=ORIENTED_EDGE('',*,*,#49308,.T.) ;
#69155=ORIENTED_EDGE('',*,*,#49309,.F.) ;
#69156=ORIENTED_EDGE('',*,*,#49310,.T.) ;
#69157=ORIENTED_EDGE('',*,*,#49311,.T.) ;
#69158=ORIENTED_EDGE('',*,*,#49312,.T.) ;
#69159=ORIENTED_EDGE('',*,*,#49313,.F.) ;
#69160=ORIENTED_EDGE('',*,*,#49314,.T.) ;
#69161=ORIENTED_EDGE('',*,*,#49279,.T.) ;
#69162=ORIENTED_EDGE('',*,*,#49314,.F.) ;
#69163=ORIENTED_EDGE('',*,*,#49315,.F.) ;
#69164=ORIENTED_EDGE('',*,*,#49316,.T.) ;
#69165=ORIENTED_EDGE('',*,*,#49276,.T.) ;
#69166=ORIENTED_EDGE('',*,*,#49316,.F.) ;
#69167=ORIENTED_EDGE('',*,*,#49278,.T.) ;
#69168=ORIENTED_EDGE('',*,*,#49317,.T.) ;
#69169=ORIENTED_EDGE('',*,*,#49282,.T.) ;
#69170=ORIENTED_EDGE('',*,*,#49317,.F.) ;
#69171=ORIENTED_EDGE('',*,*,#49318,.T.) ;
#69172=ORIENTED_EDGE('',*,*,#49319,.T.) ;
#69173=ORIENTED_EDGE('',*,*,#49320,.T.) ;
#69174=ORIENTED_EDGE('',*,*,#49321,.T.) ;
#69175=ORIENTED_EDGE('',*,*,#48901,.T.) ;
#69176=ORIENTED_EDGE('',*,*,#49322,.T.) ;
#69177=ORIENTED_EDGE('',*,*,#48905,.T.) ;
#69178=ORIENTED_EDGE('',*,*,#49323,.T.) ;
#69179=ORIENTED_EDGE('',*,*,#48913,.T.) ;
#69180=ORIENTED_EDGE('',*,*,#49324,.T.) ;
#69181=ORIENTED_EDGE('',*,*,#48921,.T.) ;
#69182=ORIENTED_EDGE('',*,*,#49325,.T.) ;
#69183=ORIENTED_EDGE('',*,*,#48929,.T.) ;
#69184=ORIENTED_EDGE('',*,*,#49326,.T.) ;
#69185=ORIENTED_EDGE('',*,*,#48937,.T.) ;
#69186=ORIENTED_EDGE('',*,*,#49327,.T.) ;
#69187=ORIENTED_EDGE('',*,*,#48945,.T.) ;
#69188=ORIENTED_EDGE('',*,*,#49328,.T.) ;
#69189=ORIENTED_EDGE('',*,*,#48953,.T.) ;
#69190=ORIENTED_EDGE('',*,*,#49329,.T.) ;
#69191=ORIENTED_EDGE('',*,*,#48961,.T.) ;
#69192=ORIENTED_EDGE('',*,*,#49330,.T.) ;
#69193=ORIENTED_EDGE('',*,*,#48969,.T.) ;
#69194=ORIENTED_EDGE('',*,*,#49331,.T.) ;
#69195=ORIENTED_EDGE('',*,*,#48977,.T.) ;
#69196=ORIENTED_EDGE('',*,*,#49332,.T.) ;
#69197=ORIENTED_EDGE('',*,*,#49333,.T.) ;
#69198=ORIENTED_EDGE('',*,*,#49334,.T.) ;
#69199=ORIENTED_EDGE('',*,*,#49335,.F.) ;
#69200=ORIENTED_EDGE('',*,*,#49336,.T.) ;
#69201=ORIENTED_EDGE('',*,*,#49337,.F.) ;
#69202=ORIENTED_EDGE('',*,*,#49338,.T.) ;
#69203=ORIENTED_EDGE('',*,*,#49339,.F.) ;
#69204=ORIENTED_EDGE('',*,*,#49340,.T.) ;
#69205=ORIENTED_EDGE('',*,*,#49341,.F.) ;
#69206=ORIENTED_EDGE('',*,*,#49342,.T.) ;
#69207=ORIENTED_EDGE('',*,*,#49020,.T.) ;
#69208=ORIENTED_EDGE('',*,*,#49343,.F.) ;
#69209=ORIENTED_EDGE('',*,*,#49344,.T.) ;
#69210=ORIENTED_EDGE('',*,*,#49345,.F.) ;
#69211=ORIENTED_EDGE('',*,*,#49346,.T.) ;
#69212=ORIENTED_EDGE('',*,*,#49347,.F.) ;
#69213=ORIENTED_EDGE('',*,*,#49348,.T.) ;
#69214=ORIENTED_EDGE('',*,*,#49349,.F.) ;
#69215=ORIENTED_EDGE('',*,*,#49350,.T.) ;
#69216=ORIENTED_EDGE('',*,*,#49038,.T.) ;
#69217=ORIENTED_EDGE('',*,*,#49351,.F.) ;
#69218=ORIENTED_EDGE('',*,*,#49352,.T.) ;
#69219=ORIENTED_EDGE('',*,*,#49353,.F.) ;
#69220=ORIENTED_EDGE('',*,*,#49354,.T.) ;
#69221=ORIENTED_EDGE('',*,*,#49355,.F.) ;
#69222=ORIENTED_EDGE('',*,*,#49356,.T.) ;
#69223=ORIENTED_EDGE('',*,*,#49357,.F.) ;
#69224=ORIENTED_EDGE('',*,*,#49358,.T.) ;
#69225=ORIENTED_EDGE('',*,*,#49056,.T.) ;
#69226=ORIENTED_EDGE('',*,*,#49359,.F.) ;
#69227=ORIENTED_EDGE('',*,*,#49360,.T.) ;
#69228=ORIENTED_EDGE('',*,*,#49361,.F.) ;
#69229=ORIENTED_EDGE('',*,*,#49362,.T.) ;
#69230=ORIENTED_EDGE('',*,*,#49363,.F.) ;
#69231=ORIENTED_EDGE('',*,*,#49364,.T.) ;
#69232=ORIENTED_EDGE('',*,*,#49365,.F.) ;
#69233=ORIENTED_EDGE('',*,*,#49366,.T.) ;
#69234=ORIENTED_EDGE('',*,*,#49074,.T.) ;
#69235=ORIENTED_EDGE('',*,*,#49367,.F.) ;
#69236=ORIENTED_EDGE('',*,*,#49368,.T.) ;
#69237=ORIENTED_EDGE('',*,*,#49369,.F.) ;
#69238=ORIENTED_EDGE('',*,*,#49370,.T.) ;
#69239=ORIENTED_EDGE('',*,*,#49371,.F.) ;
#69240=ORIENTED_EDGE('',*,*,#49372,.T.) ;
#69241=ORIENTED_EDGE('',*,*,#49373,.F.) ;
#69242=ORIENTED_EDGE('',*,*,#49374,.T.) ;
#69243=ORIENTED_EDGE('',*,*,#49281,.T.) ;
#69244=ORIENTED_EDGE('',*,*,#49083,.T.) ;
#69245=ORIENTED_EDGE('',*,*,#49375,.F.) ;
#69246=ORIENTED_EDGE('',*,*,#49376,.T.) ;
#69247=ORIENTED_EDGE('',*,*,#49377,.F.) ;
#69248=ORIENTED_EDGE('',*,*,#49378,.T.) ;
#69249=ORIENTED_EDGE('',*,*,#49379,.F.) ;
#69250=ORIENTED_EDGE('',*,*,#49380,.T.) ;
#69251=ORIENTED_EDGE('',*,*,#49381,.F.) ;
#69252=ORIENTED_EDGE('',*,*,#49382,.T.) ;
#69253=ORIENTED_EDGE('',*,*,#49065,.T.) ;
#69254=ORIENTED_EDGE('',*,*,#49383,.F.) ;
#69255=ORIENTED_EDGE('',*,*,#49384,.T.) ;
#69256=ORIENTED_EDGE('',*,*,#49385,.F.) ;
#69257=ORIENTED_EDGE('',*,*,#49386,.T.) ;
#69258=ORIENTED_EDGE('',*,*,#49387,.F.) ;
#69259=ORIENTED_EDGE('',*,*,#49388,.T.) ;
#69260=ORIENTED_EDGE('',*,*,#49389,.F.) ;
#69261=ORIENTED_EDGE('',*,*,#49390,.T.) ;
#69262=ORIENTED_EDGE('',*,*,#49047,.T.) ;
#69263=ORIENTED_EDGE('',*,*,#49391,.F.) ;
#69264=ORIENTED_EDGE('',*,*,#49392,.T.) ;
#69265=ORIENTED_EDGE('',*,*,#49393,.F.) ;
#69266=ORIENTED_EDGE('',*,*,#49394,.T.) ;
#69267=ORIENTED_EDGE('',*,*,#49395,.F.) ;
#69268=ORIENTED_EDGE('',*,*,#49396,.T.) ;
#69269=ORIENTED_EDGE('',*,*,#49397,.F.) ;
#69270=ORIENTED_EDGE('',*,*,#49398,.T.) ;
#69271=ORIENTED_EDGE('',*,*,#49029,.T.) ;
#69272=ORIENTED_EDGE('',*,*,#49399,.F.) ;
#69273=ORIENTED_EDGE('',*,*,#49400,.T.) ;
#69274=ORIENTED_EDGE('',*,*,#49401,.F.) ;
#69275=ORIENTED_EDGE('',*,*,#49402,.T.) ;
#69276=ORIENTED_EDGE('',*,*,#49403,.F.) ;
#69277=ORIENTED_EDGE('',*,*,#49404,.T.) ;
#69278=ORIENTED_EDGE('',*,*,#49405,.F.) ;
#69279=ORIENTED_EDGE('',*,*,#49406,.T.) ;
#69280=ORIENTED_EDGE('',*,*,#49011,.T.) ;
#69281=ORIENTED_EDGE('',*,*,#49407,.F.) ;
#69282=ORIENTED_EDGE('',*,*,#49408,.T.) ;
#69283=ORIENTED_EDGE('',*,*,#49409,.F.) ;
#69284=ORIENTED_EDGE('',*,*,#49410,.T.) ;
#69285=ORIENTED_EDGE('',*,*,#49411,.F.) ;
#69286=ORIENTED_EDGE('',*,*,#49412,.T.) ;
#69287=ORIENTED_EDGE('',*,*,#49413,.F.) ;
#69288=ORIENTED_EDGE('',*,*,#49414,.T.) ;
#69289=ORIENTED_EDGE('',*,*,#49415,.T.) ;
#69290=ORIENTED_EDGE('',*,*,#49416,.T.) ;
#69291=ORIENTED_EDGE('',*,*,#49417,.T.) ;
#69292=ORIENTED_EDGE('',*,*,#49418,.T.) ;
#69293=ORIENTED_EDGE('',*,*,#49419,.T.) ;
#69294=ORIENTED_EDGE('',*,*,#49420,.T.) ;
#69295=ORIENTED_EDGE('',*,*,#49421,.T.) ;
#69296=ORIENTED_EDGE('',*,*,#49422,.T.) ;
#69297=ORIENTED_EDGE('',*,*,#49423,.T.) ;
#69298=ORIENTED_EDGE('',*,*,#49424,.T.) ;
#69299=ORIENTED_EDGE('',*,*,#49425,.T.) ;
#69300=ORIENTED_EDGE('',*,*,#49426,.T.) ;
#69301=ORIENTED_EDGE('',*,*,#49427,.T.) ;
#69302=ORIENTED_EDGE('',*,*,#49428,.T.) ;
#69303=ORIENTED_EDGE('',*,*,#49429,.T.) ;
#69304=ORIENTED_EDGE('',*,*,#49430,.T.) ;
#69305=ORIENTED_EDGE('',*,*,#49431,.T.) ;
#69306=ORIENTED_EDGE('',*,*,#49432,.T.) ;
#69307=ORIENTED_EDGE('',*,*,#49433,.T.) ;
#69308=ORIENTED_EDGE('',*,*,#49434,.T.) ;
#69309=ORIENTED_EDGE('',*,*,#49435,.T.) ;
#69310=ORIENTED_EDGE('',*,*,#49436,.T.) ;
#69311=ORIENTED_EDGE('',*,*,#49437,.T.) ;
#69312=ORIENTED_EDGE('',*,*,#49438,.T.) ;
#69313=ORIENTED_EDGE('',*,*,#49439,.T.) ;
#69314=ORIENTED_EDGE('',*,*,#49440,.T.) ;
#69315=ORIENTED_EDGE('',*,*,#49441,.T.) ;
#69316=ORIENTED_EDGE('',*,*,#49442,.T.) ;
#69317=ORIENTED_EDGE('',*,*,#49443,.T.) ;
#69318=ORIENTED_EDGE('',*,*,#49444,.T.) ;
#69319=ORIENTED_EDGE('',*,*,#49445,.T.) ;
#69320=ORIENTED_EDGE('',*,*,#49446,.T.) ;
#69321=ORIENTED_EDGE('',*,*,#49447,.T.) ;
#69322=ORIENTED_EDGE('',*,*,#49448,.T.) ;
#69323=ORIENTED_EDGE('',*,*,#49449,.T.) ;
#69324=ORIENTED_EDGE('',*,*,#49450,.T.) ;
#69325=ORIENTED_EDGE('',*,*,#49451,.T.) ;
#69326=ORIENTED_EDGE('',*,*,#49452,.T.) ;
#69327=ORIENTED_EDGE('',*,*,#49453,.T.) ;
#69328=ORIENTED_EDGE('',*,*,#49454,.T.) ;
#69329=ORIENTED_EDGE('',*,*,#49455,.T.) ;
#69330=ORIENTED_EDGE('',*,*,#49456,.T.) ;
#69331=ORIENTED_EDGE('',*,*,#49457,.T.) ;
#69332=ORIENTED_EDGE('',*,*,#49458,.T.) ;
#69333=ORIENTED_EDGE('',*,*,#49459,.T.) ;
#69334=ORIENTED_EDGE('',*,*,#49460,.T.) ;
#69335=ORIENTED_EDGE('',*,*,#49461,.T.) ;
#69336=ORIENTED_EDGE('',*,*,#49462,.T.) ;
#69337=ORIENTED_EDGE('',*,*,#49463,.T.) ;
#69338=ORIENTED_EDGE('',*,*,#49464,.T.) ;
#69339=ORIENTED_EDGE('',*,*,#49465,.T.) ;
#69340=ORIENTED_EDGE('',*,*,#49466,.T.) ;
#69341=ORIENTED_EDGE('',*,*,#49467,.T.) ;
#69342=ORIENTED_EDGE('',*,*,#49468,.T.) ;
#69343=ORIENTED_EDGE('',*,*,#49469,.T.) ;
#69344=ORIENTED_EDGE('',*,*,#49470,.T.) ;
#69345=ORIENTED_EDGE('',*,*,#49471,.T.) ;
#69346=ORIENTED_EDGE('',*,*,#49472,.T.) ;
#69347=ORIENTED_EDGE('',*,*,#49473,.T.) ;
#69348=ORIENTED_EDGE('',*,*,#49474,.T.) ;
#69349=ORIENTED_EDGE('',*,*,#49475,.T.) ;
#69350=ORIENTED_EDGE('',*,*,#49476,.T.) ;
#69351=ORIENTED_EDGE('',*,*,#49477,.T.) ;
#69352=ORIENTED_EDGE('',*,*,#49478,.T.) ;
#69353=ORIENTED_EDGE('',*,*,#49479,.T.) ;
#69354=ORIENTED_EDGE('',*,*,#49480,.T.) ;
#69355=ORIENTED_EDGE('',*,*,#49481,.T.) ;
#69356=ORIENTED_EDGE('',*,*,#49482,.T.) ;
#69357=ORIENTED_EDGE('',*,*,#49483,.T.) ;
#69358=ORIENTED_EDGE('',*,*,#49484,.T.) ;
#69359=ORIENTED_EDGE('',*,*,#49485,.T.) ;
#69360=ORIENTED_EDGE('',*,*,#49486,.T.) ;
#69361=ORIENTED_EDGE('',*,*,#49487,.T.) ;
#69362=ORIENTED_EDGE('',*,*,#49488,.T.) ;
#69363=ORIENTED_EDGE('',*,*,#49489,.T.) ;
#69364=ORIENTED_EDGE('',*,*,#49490,.T.) ;
#69365=ORIENTED_EDGE('',*,*,#49491,.T.) ;
#69366=ORIENTED_EDGE('',*,*,#49492,.T.) ;
#69367=ORIENTED_EDGE('',*,*,#49493,.T.) ;
#69368=ORIENTED_EDGE('',*,*,#49494,.T.) ;
#69369=ORIENTED_EDGE('',*,*,#49495,.T.) ;
#69370=ORIENTED_EDGE('',*,*,#49496,.T.) ;
#69371=ORIENTED_EDGE('',*,*,#49497,.T.) ;
#69372=ORIENTED_EDGE('',*,*,#49498,.T.) ;
#69373=ORIENTED_EDGE('',*,*,#49499,.T.) ;
#69374=ORIENTED_EDGE('',*,*,#49500,.T.) ;
#69375=ORIENTED_EDGE('',*,*,#49501,.T.) ;
#69376=ORIENTED_EDGE('',*,*,#49502,.T.) ;
#69377=ORIENTED_EDGE('',*,*,#49503,.T.) ;
#69378=ORIENTED_EDGE('',*,*,#49504,.T.) ;
#69379=ORIENTED_EDGE('',*,*,#49505,.T.) ;
#69380=ORIENTED_EDGE('',*,*,#49506,.T.) ;
#69381=ORIENTED_EDGE('',*,*,#49507,.T.) ;
#69382=ORIENTED_EDGE('',*,*,#49508,.T.) ;
#69383=ORIENTED_EDGE('',*,*,#49509,.T.) ;
#69384=ORIENTED_EDGE('',*,*,#49510,.T.) ;
#69385=ORIENTED_EDGE('',*,*,#49511,.T.) ;
#69386=ORIENTED_EDGE('',*,*,#49512,.T.) ;
#69387=ORIENTED_EDGE('',*,*,#49513,.T.) ;
#69388=ORIENTED_EDGE('',*,*,#49514,.T.) ;
#69389=ORIENTED_EDGE('',*,*,#49515,.T.) ;
#69390=ORIENTED_EDGE('',*,*,#49516,.T.) ;
#69391=ORIENTED_EDGE('',*,*,#49517,.T.) ;
#69392=ORIENTED_EDGE('',*,*,#49518,.T.) ;
#69393=ORIENTED_EDGE('',*,*,#49519,.T.) ;
#69394=ORIENTED_EDGE('',*,*,#49520,.T.) ;
#69395=ORIENTED_EDGE('',*,*,#49521,.T.) ;
#69396=ORIENTED_EDGE('',*,*,#49522,.T.) ;
#69397=ORIENTED_EDGE('',*,*,#49239,.T.) ;
#69398=ORIENTED_EDGE('',*,*,#49523,.T.) ;
#69399=ORIENTED_EDGE('',*,*,#49221,.T.) ;
#69400=ORIENTED_EDGE('',*,*,#49524,.T.) ;
#69401=ORIENTED_EDGE('',*,*,#49203,.T.) ;
#69402=ORIENTED_EDGE('',*,*,#49525,.T.) ;
#69403=ORIENTED_EDGE('',*,*,#49185,.T.) ;
#69404=ORIENTED_EDGE('',*,*,#49526,.T.) ;
#69405=ORIENTED_EDGE('',*,*,#49167,.T.) ;
#69406=ORIENTED_EDGE('',*,*,#49527,.T.) ;
#69407=ORIENTED_EDGE('',*,*,#49149,.T.) ;
#69408=ORIENTED_EDGE('',*,*,#49528,.T.) ;
#69409=ORIENTED_EDGE('',*,*,#49131,.T.) ;
#69410=ORIENTED_EDGE('',*,*,#49529,.T.) ;
#69411=ORIENTED_EDGE('',*,*,#49113,.T.) ;
#69412=ORIENTED_EDGE('',*,*,#49530,.T.) ;
#69413=ORIENTED_EDGE('',*,*,#49095,.T.) ;
#69414=ORIENTED_EDGE('',*,*,#49531,.T.) ;
#69415=ORIENTED_EDGE('',*,*,#49532,.T.) ;
#69416=ORIENTED_EDGE('',*,*,#49533,.T.) ;
#69417=ORIENTED_EDGE('',*,*,#49534,.T.) ;
#69418=ORIENTED_EDGE('',*,*,#49535,.T.) ;
#69419=ORIENTED_EDGE('',*,*,#49536,.T.) ;
#69420=ORIENTED_EDGE('',*,*,#49537,.T.) ;
#69421=ORIENTED_EDGE('',*,*,#49538,.T.) ;
#69422=ORIENTED_EDGE('',*,*,#49539,.T.) ;
#69423=ORIENTED_EDGE('',*,*,#49540,.T.) ;
#69424=ORIENTED_EDGE('',*,*,#49541,.T.) ;
#69425=ORIENTED_EDGE('',*,*,#49542,.T.) ;
#69426=ORIENTED_EDGE('',*,*,#49543,.T.) ;
#69427=ORIENTED_EDGE('',*,*,#49544,.T.) ;
#69428=ORIENTED_EDGE('',*,*,#49545,.T.) ;
#69429=ORIENTED_EDGE('',*,*,#49546,.T.) ;
#69430=ORIENTED_EDGE('',*,*,#49547,.T.) ;
#69431=ORIENTED_EDGE('',*,*,#49548,.T.) ;
#69432=ORIENTED_EDGE('',*,*,#49549,.T.) ;
#69433=ORIENTED_EDGE('',*,*,#49550,.T.) ;
#69434=ORIENTED_EDGE('',*,*,#49551,.T.) ;
#69435=ORIENTED_EDGE('',*,*,#49552,.T.) ;
#69436=ORIENTED_EDGE('',*,*,#49553,.T.) ;
#69437=ORIENTED_EDGE('',*,*,#49554,.T.) ;
#69438=ORIENTED_EDGE('',*,*,#49555,.T.) ;
#69439=ORIENTED_EDGE('',*,*,#49556,.T.) ;
#69440=ORIENTED_EDGE('',*,*,#49557,.T.) ;
#69441=ORIENTED_EDGE('',*,*,#49558,.T.) ;
#69442=ORIENTED_EDGE('',*,*,#49559,.T.) ;
#69443=ORIENTED_EDGE('',*,*,#49560,.T.) ;
#69444=ORIENTED_EDGE('',*,*,#49561,.T.) ;
#69445=ORIENTED_EDGE('',*,*,#49562,.T.) ;
#69446=ORIENTED_EDGE('',*,*,#49563,.T.) ;
#69447=ORIENTED_EDGE('',*,*,#49564,.T.) ;
#69448=ORIENTED_EDGE('',*,*,#49565,.T.) ;
#69449=ORIENTED_EDGE('',*,*,#49566,.T.) ;
#69450=ORIENTED_EDGE('',*,*,#49567,.T.) ;
#69451=ORIENTED_EDGE('',*,*,#49568,.T.) ;
#69452=ORIENTED_EDGE('',*,*,#49569,.T.) ;
#69453=ORIENTED_EDGE('',*,*,#49570,.T.) ;
#69454=ORIENTED_EDGE('',*,*,#49571,.T.) ;
#69455=ORIENTED_EDGE('',*,*,#49572,.T.) ;
#69456=ORIENTED_EDGE('',*,*,#49573,.T.) ;
#69457=ORIENTED_EDGE('',*,*,#49574,.T.) ;
#69458=ORIENTED_EDGE('',*,*,#49575,.T.) ;
#69459=ORIENTED_EDGE('',*,*,#49576,.T.) ;
#69460=ORIENTED_EDGE('',*,*,#49577,.T.) ;
#69461=ORIENTED_EDGE('',*,*,#49578,.T.) ;
#69462=ORIENTED_EDGE('',*,*,#49579,.T.) ;
#69463=ORIENTED_EDGE('',*,*,#49580,.T.) ;
#69464=ORIENTED_EDGE('',*,*,#49581,.T.) ;
#69465=ORIENTED_EDGE('',*,*,#49582,.T.) ;
#69466=ORIENTED_EDGE('',*,*,#49583,.T.) ;
#69467=ORIENTED_EDGE('',*,*,#49584,.T.) ;
#69468=ORIENTED_EDGE('',*,*,#49585,.T.) ;
#69469=ORIENTED_EDGE('',*,*,#49586,.T.) ;
#69470=ORIENTED_EDGE('',*,*,#49587,.T.) ;
#69471=ORIENTED_EDGE('',*,*,#49588,.T.) ;
#69472=ORIENTED_EDGE('',*,*,#49589,.T.) ;
#69473=ORIENTED_EDGE('',*,*,#49590,.T.) ;
#69474=ORIENTED_EDGE('',*,*,#49591,.T.) ;
#69475=ORIENTED_EDGE('',*,*,#49592,.T.) ;
#69476=ORIENTED_EDGE('',*,*,#49593,.T.) ;
#69477=ORIENTED_EDGE('',*,*,#49594,.T.) ;
#69478=ORIENTED_EDGE('',*,*,#49595,.T.) ;
#69479=ORIENTED_EDGE('',*,*,#49596,.F.) ;
#69480=ORIENTED_EDGE('',*,*,#49597,.T.) ;
#69481=ORIENTED_EDGE('',*,*,#49598,.T.) ;
#69482=ORIENTED_EDGE('',*,*,#49599,.T.) ;
#69483=ORIENTED_EDGE('',*,*,#49600,.T.) ;
#69484=ORIENTED_EDGE('',*,*,#49601,.T.) ;
#69485=ORIENTED_EDGE('',*,*,#49602,.F.) ;
#69486=ORIENTED_EDGE('',*,*,#49603,.T.) ;
#69487=ORIENTED_EDGE('',*,*,#49604,.F.) ;
#69488=ORIENTED_EDGE('',*,*,#49605,.T.) ;
#69489=ORIENTED_EDGE('',*,*,#49606,.T.) ;
#69490=ORIENTED_EDGE('',*,*,#49607,.T.) ;
#69491=ORIENTED_EDGE('',*,*,#49608,.T.) ;
#69492=ORIENTED_EDGE('',*,*,#49609,.T.) ;
#69493=ORIENTED_EDGE('',*,*,#49610,.F.) ;
#69494=ORIENTED_EDGE('',*,*,#49611,.T.) ;
#69495=ORIENTED_EDGE('',*,*,#49612,.F.) ;
#69496=ORIENTED_EDGE('',*,*,#49613,.T.) ;
#69497=ORIENTED_EDGE('',*,*,#49614,.T.) ;
#69498=ORIENTED_EDGE('',*,*,#49615,.T.) ;
#69499=ORIENTED_EDGE('',*,*,#49616,.T.) ;
#69500=ORIENTED_EDGE('',*,*,#49617,.T.) ;
#69501=ORIENTED_EDGE('',*,*,#49618,.F.) ;
#69502=ORIENTED_EDGE('',*,*,#49619,.T.) ;
#69503=ORIENTED_EDGE('',*,*,#49620,.F.) ;
#69504=ORIENTED_EDGE('',*,*,#49621,.T.) ;
#69505=ORIENTED_EDGE('',*,*,#49622,.T.) ;
#69506=ORIENTED_EDGE('',*,*,#49623,.T.) ;
#69507=ORIENTED_EDGE('',*,*,#49624,.T.) ;
#69508=ORIENTED_EDGE('',*,*,#49625,.T.) ;
#69509=ORIENTED_EDGE('',*,*,#49626,.F.) ;
#69510=ORIENTED_EDGE('',*,*,#49627,.T.) ;
#69511=ORIENTED_EDGE('',*,*,#49628,.F.) ;
#69512=ORIENTED_EDGE('',*,*,#49629,.T.) ;
#69513=ORIENTED_EDGE('',*,*,#49630,.T.) ;
#69514=ORIENTED_EDGE('',*,*,#49631,.T.) ;
#69515=ORIENTED_EDGE('',*,*,#49632,.T.) ;
#69516=ORIENTED_EDGE('',*,*,#49633,.T.) ;
#69517=ORIENTED_EDGE('',*,*,#49634,.F.) ;
#69518=ORIENTED_EDGE('',*,*,#49635,.T.) ;
#69519=ORIENTED_EDGE('',*,*,#49636,.F.) ;
#69520=ORIENTED_EDGE('',*,*,#49637,.T.) ;
#69521=ORIENTED_EDGE('',*,*,#49638,.T.) ;
#69522=ORIENTED_EDGE('',*,*,#49639,.T.) ;
#69523=ORIENTED_EDGE('',*,*,#49640,.T.) ;
#69524=ORIENTED_EDGE('',*,*,#49641,.T.) ;
#69525=ORIENTED_EDGE('',*,*,#49642,.F.) ;
#69526=ORIENTED_EDGE('',*,*,#49643,.T.) ;
#69527=ORIENTED_EDGE('',*,*,#49644,.F.) ;
#69528=ORIENTED_EDGE('',*,*,#49645,.T.) ;
#69529=ORIENTED_EDGE('',*,*,#49646,.T.) ;
#69530=ORIENTED_EDGE('',*,*,#49647,.T.) ;
#69531=ORIENTED_EDGE('',*,*,#49648,.T.) ;
#69532=ORIENTED_EDGE('',*,*,#49649,.T.) ;
#69533=ORIENTED_EDGE('',*,*,#49650,.F.) ;
#69534=ORIENTED_EDGE('',*,*,#49651,.T.) ;
#69535=ORIENTED_EDGE('',*,*,#49652,.F.) ;
#69536=ORIENTED_EDGE('',*,*,#49653,.T.) ;
#69537=ORIENTED_EDGE('',*,*,#49654,.T.) ;
#69538=ORIENTED_EDGE('',*,*,#49655,.T.) ;
#69539=ORIENTED_EDGE('',*,*,#49656,.T.) ;
#69540=ORIENTED_EDGE('',*,*,#49657,.T.) ;
#69541=ORIENTED_EDGE('',*,*,#49658,.F.) ;
#69542=ORIENTED_EDGE('',*,*,#49659,.T.) ;
#69543=ORIENTED_EDGE('',*,*,#49660,.F.) ;
#69544=ORIENTED_EDGE('',*,*,#49661,.T.) ;
#69545=ORIENTED_EDGE('',*,*,#49662,.T.) ;
#69546=ORIENTED_EDGE('',*,*,#49663,.T.) ;
#69547=ORIENTED_EDGE('',*,*,#49664,.T.) ;
#69548=ORIENTED_EDGE('',*,*,#49665,.T.) ;
#69549=ORIENTED_EDGE('',*,*,#49666,.F.) ;
#69550=ORIENTED_EDGE('',*,*,#49667,.T.) ;
#69551=ORIENTED_EDGE('',*,*,#49668,.T.) ;
#69552=ORIENTED_EDGE('',*,*,#49669,.T.) ;
#69553=ORIENTED_EDGE('',*,*,#49670,.T.) ;
#69554=ORIENTED_EDGE('',*,*,#49671,.T.) ;
#69555=ORIENTED_EDGE('',*,*,#49672,.T.) ;
#69556=ORIENTED_EDGE('',*,*,#49673,.T.) ;
#69557=ORIENTED_EDGE('',*,*,#49674,.T.) ;
#69558=ORIENTED_EDGE('',*,*,#49675,.T.) ;
#69559=ORIENTED_EDGE('',*,*,#49676,.F.) ;
#69560=ORIENTED_EDGE('',*,*,#49677,.T.) ;
#69561=ORIENTED_EDGE('',*,*,#49678,.F.) ;
#69562=ORIENTED_EDGE('',*,*,#49679,.T.) ;
#69563=ORIENTED_EDGE('',*,*,#49680,.T.) ;
#69564=ORIENTED_EDGE('',*,*,#49681,.T.) ;
#69565=ORIENTED_EDGE('',*,*,#49682,.F.) ;
#69566=ORIENTED_EDGE('',*,*,#49683,.T.) ;
#69567=ORIENTED_EDGE('',*,*,#49684,.F.) ;
#69568=ORIENTED_EDGE('',*,*,#49685,.T.) ;
#69569=ORIENTED_EDGE('',*,*,#49686,.T.) ;
#69570=ORIENTED_EDGE('',*,*,#49687,.T.) ;
#69571=ORIENTED_EDGE('',*,*,#49688,.F.) ;
#69572=ORIENTED_EDGE('',*,*,#49689,.T.) ;
#69573=ORIENTED_EDGE('',*,*,#49690,.F.) ;
#69574=ORIENTED_EDGE('',*,*,#49691,.T.) ;
#69575=ORIENTED_EDGE('',*,*,#49692,.T.) ;
#69576=ORIENTED_EDGE('',*,*,#49693,.T.) ;
#69577=ORIENTED_EDGE('',*,*,#49694,.F.) ;
#69578=ORIENTED_EDGE('',*,*,#49695,.T.) ;
#69579=ORIENTED_EDGE('',*,*,#49696,.F.) ;
#69580=ORIENTED_EDGE('',*,*,#49697,.T.) ;
#69581=ORIENTED_EDGE('',*,*,#49698,.T.) ;
#69582=ORIENTED_EDGE('',*,*,#49699,.T.) ;
#69583=ORIENTED_EDGE('',*,*,#49700,.F.) ;
#69584=ORIENTED_EDGE('',*,*,#49701,.T.) ;
#69585=ORIENTED_EDGE('',*,*,#49702,.F.) ;
#69586=ORIENTED_EDGE('',*,*,#49703,.T.) ;
#69587=ORIENTED_EDGE('',*,*,#49704,.T.) ;
#69588=ORIENTED_EDGE('',*,*,#49705,.T.) ;
#69589=ORIENTED_EDGE('',*,*,#49706,.F.) ;
#69590=ORIENTED_EDGE('',*,*,#49707,.T.) ;
#69591=ORIENTED_EDGE('',*,*,#49708,.F.) ;
#69592=ORIENTED_EDGE('',*,*,#49709,.T.) ;
#69593=ORIENTED_EDGE('',*,*,#49710,.T.) ;
#69594=ORIENTED_EDGE('',*,*,#49711,.T.) ;
#69595=ORIENTED_EDGE('',*,*,#49712,.F.) ;
#69596=ORIENTED_EDGE('',*,*,#49713,.T.) ;
#69597=ORIENTED_EDGE('',*,*,#49714,.F.) ;
#69598=ORIENTED_EDGE('',*,*,#49715,.T.) ;
#69599=ORIENTED_EDGE('',*,*,#49716,.T.) ;
#69600=ORIENTED_EDGE('',*,*,#49717,.T.) ;
#69601=ORIENTED_EDGE('',*,*,#49718,.F.) ;
#69602=ORIENTED_EDGE('',*,*,#49719,.T.) ;
#69603=ORIENTED_EDGE('',*,*,#49720,.F.) ;
#69604=ORIENTED_EDGE('',*,*,#49721,.T.) ;
#69605=ORIENTED_EDGE('',*,*,#49722,.T.) ;
#69606=ORIENTED_EDGE('',*,*,#49723,.T.) ;
#69607=ORIENTED_EDGE('',*,*,#49724,.F.) ;
#69608=ORIENTED_EDGE('',*,*,#49725,.T.) ;
#69609=ORIENTED_EDGE('',*,*,#49726,.F.) ;
#69610=ORIENTED_EDGE('',*,*,#49727,.T.) ;
#69611=ORIENTED_EDGE('',*,*,#49728,.T.) ;
#69612=ORIENTED_EDGE('',*,*,#49729,.T.) ;
#69613=ORIENTED_EDGE('',*,*,#49730,.F.) ;
#69614=ORIENTED_EDGE('',*,*,#49731,.T.) ;
#69615=ORIENTED_EDGE('',*,*,#49732,.F.) ;
#69616=ORIENTED_EDGE('',*,*,#49733,.T.) ;
#69617=ORIENTED_EDGE('',*,*,#49734,.T.) ;
#69618=ORIENTED_EDGE('',*,*,#49735,.T.) ;
#69619=ORIENTED_EDGE('',*,*,#49736,.F.) ;
#69620=ORIENTED_EDGE('',*,*,#49737,.T.) ;
#69621=ORIENTED_EDGE('',*,*,#49534,.F.) ;
#69622=ORIENTED_EDGE('',*,*,#49738,.T.) ;
#69623=ORIENTED_EDGE('',*,*,#49739,.F.) ;
#69624=ORIENTED_EDGE('',*,*,#49740,.F.) ;
#69625=ORIENTED_EDGE('',*,*,#49741,.F.) ;
#69626=ORIENTED_EDGE('',*,*,#49542,.F.) ;
#69627=ORIENTED_EDGE('',*,*,#49742,.F.) ;
#69628=ORIENTED_EDGE('',*,*,#49743,.F.) ;
#69629=ORIENTED_EDGE('',*,*,#49744,.T.) ;
#69630=ORIENTED_EDGE('',*,*,#49745,.T.) ;
#69631=ORIENTED_EDGE('',*,*,#49746,.T.) ;
#69632=ORIENTED_EDGE('',*,*,#49747,.T.) ;
#69633=ORIENTED_EDGE('',*,*,#49748,.F.) ;
#69634=ORIENTED_EDGE('',*,*,#49749,.T.) ;
#69635=ORIENTED_EDGE('',*,*,#49750,.F.) ;
#69636=ORIENTED_EDGE('',*,*,#49751,.T.) ;
#69637=ORIENTED_EDGE('',*,*,#49752,.F.) ;
#69638=ORIENTED_EDGE('',*,*,#49753,.T.) ;
#69639=ORIENTED_EDGE('',*,*,#49754,.F.) ;
#69640=ORIENTED_EDGE('',*,*,#49755,.T.) ;
#69641=ORIENTED_EDGE('',*,*,#49756,.T.) ;
#69642=ORIENTED_EDGE('',*,*,#49757,.T.) ;
#69643=ORIENTED_EDGE('',*,*,#49758,.T.) ;
#69644=ORIENTED_EDGE('',*,*,#49759,.T.) ;
#69645=ORIENTED_EDGE('',*,*,#49760,.T.) ;
#69646=ORIENTED_EDGE('',*,*,#49761,.T.) ;
#69647=ORIENTED_EDGE('',*,*,#49762,.T.) ;
#69648=ORIENTED_EDGE('',*,*,#49763,.T.) ;
#69649=ORIENTED_EDGE('',*,*,#49764,.T.) ;
#69650=ORIENTED_EDGE('',*,*,#49765,.T.) ;
#69651=ORIENTED_EDGE('',*,*,#49766,.T.) ;
#69652=ORIENTED_EDGE('',*,*,#49767,.T.) ;
#69653=ORIENTED_EDGE('',*,*,#49768,.T.) ;
#69654=ORIENTED_EDGE('',*,*,#49769,.T.) ;
#69655=ORIENTED_EDGE('',*,*,#49770,.T.) ;
#69656=ORIENTED_EDGE('',*,*,#49771,.T.) ;
#69657=ORIENTED_EDGE('',*,*,#49772,.T.) ;
#69658=ORIENTED_EDGE('',*,*,#49773,.T.) ;
#69659=ORIENTED_EDGE('',*,*,#49774,.T.) ;
#69660=ORIENTED_EDGE('',*,*,#49775,.T.) ;
#69661=ORIENTED_EDGE('',*,*,#49776,.T.) ;
#69662=ORIENTED_EDGE('',*,*,#49777,.T.) ;
#69663=ORIENTED_EDGE('',*,*,#49778,.T.) ;
#69664=ORIENTED_EDGE('',*,*,#49779,.T.) ;
#69665=ORIENTED_EDGE('',*,*,#49780,.T.) ;
#69666=ORIENTED_EDGE('',*,*,#49781,.T.) ;
#69667=ORIENTED_EDGE('',*,*,#49782,.T.) ;
#69668=ORIENTED_EDGE('',*,*,#49783,.T.) ;
#69669=ORIENTED_EDGE('',*,*,#49784,.T.) ;
#69670=ORIENTED_EDGE('',*,*,#49785,.T.) ;
#69671=ORIENTED_EDGE('',*,*,#49786,.T.) ;
#69672=ORIENTED_EDGE('',*,*,#49787,.T.) ;
#69673=ORIENTED_EDGE('',*,*,#49788,.F.) ;
#69674=ORIENTED_EDGE('',*,*,#49789,.T.) ;
#69675=ORIENTED_EDGE('',*,*,#49790,.F.) ;
#69676=ORIENTED_EDGE('',*,*,#49791,.T.) ;
#69677=ORIENTED_EDGE('',*,*,#49792,.F.) ;
#69678=ORIENTED_EDGE('',*,*,#49793,.T.) ;
#69679=ORIENTED_EDGE('',*,*,#49794,.F.) ;
#69680=ORIENTED_EDGE('',*,*,#49795,.T.) ;
#69681=ORIENTED_EDGE('',*,*,#49796,.T.) ;
#69682=ORIENTED_EDGE('',*,*,#49797,.T.) ;
#69683=ORIENTED_EDGE('',*,*,#49798,.T.) ;
#69684=ORIENTED_EDGE('',*,*,#49799,.T.) ;
#69685=ORIENTED_EDGE('',*,*,#49800,.T.) ;
#69686=ORIENTED_EDGE('',*,*,#49801,.T.) ;
#69687=ORIENTED_EDGE('',*,*,#49802,.T.) ;
#69688=ORIENTED_EDGE('',*,*,#49803,.T.) ;
#69689=ORIENTED_EDGE('',*,*,#49804,.T.) ;
#69690=ORIENTED_EDGE('',*,*,#49805,.T.) ;
#69691=ORIENTED_EDGE('',*,*,#49806,.T.) ;
#69692=ORIENTED_EDGE('',*,*,#49807,.T.) ;
#69693=ORIENTED_EDGE('',*,*,#49808,.T.) ;
#69694=ORIENTED_EDGE('',*,*,#49809,.T.) ;
#69695=ORIENTED_EDGE('',*,*,#49810,.T.) ;
#69696=ORIENTED_EDGE('',*,*,#49811,.T.) ;
#69697=ORIENTED_EDGE('',*,*,#49305,.T.) ;
#69698=ORIENTED_EDGE('',*,*,#49812,.T.) ;
#69699=ORIENTED_EDGE('',*,*,#49813,.T.) ;
#69700=ORIENTED_EDGE('',*,*,#49814,.T.) ;
#69701=ORIENTED_EDGE('',*,*,#49815,.T.) ;
#69702=ORIENTED_EDGE('',*,*,#49816,.T.) ;
#69703=ORIENTED_EDGE('',*,*,#49817,.F.) ;
#69704=ORIENTED_EDGE('',*,*,#49818,.T.) ;
#69705=ORIENTED_EDGE('',*,*,#49819,.F.) ;
#69706=ORIENTED_EDGE('',*,*,#49820,.T.) ;
#69707=ORIENTED_EDGE('',*,*,#49821,.T.) ;
#69708=ORIENTED_EDGE('',*,*,#49822,.T.) ;
#69709=ORIENTED_EDGE('',*,*,#49823,.T.) ;
#69710=ORIENTED_EDGE('',*,*,#49824,.T.) ;
#69711=ORIENTED_EDGE('',*,*,#49825,.T.) ;
#69712=ORIENTED_EDGE('',*,*,#48898,.T.) ;
#69713=ORIENTED_EDGE('',*,*,#49826,.T.) ;
#69714=ORIENTED_EDGE('',*,*,#49827,.T.) ;
#69715=ORIENTED_EDGE('',*,*,#49828,.T.) ;
#69716=ORIENTED_EDGE('',*,*,#49829,.T.) ;
#69717=ORIENTED_EDGE('',*,*,#49830,.T.) ;
#69718=ORIENTED_EDGE('',*,*,#49831,.T.) ;
#69719=ORIENTED_EDGE('',*,*,#49832,.T.) ;
#69720=ORIENTED_EDGE('',*,*,#49833,.T.) ;
#69721=ORIENTED_EDGE('',*,*,#49834,.T.) ;
#69722=ORIENTED_EDGE('',*,*,#49835,.T.) ;
#69723=ORIENTED_EDGE('',*,*,#49836,.T.) ;
#69724=ORIENTED_EDGE('',*,*,#49837,.T.) ;
#69725=ORIENTED_EDGE('',*,*,#49838,.T.) ;
#69726=ORIENTED_EDGE('',*,*,#49839,.T.) ;
#69727=ORIENTED_EDGE('',*,*,#49840,.T.) ;
#69728=ORIENTED_EDGE('',*,*,#49841,.T.) ;
#69729=ORIENTED_EDGE('',*,*,#49842,.T.) ;
#69730=ORIENTED_EDGE('',*,*,#49843,.T.) ;
#69731=ORIENTED_EDGE('',*,*,#49844,.T.) ;
#69732=ORIENTED_EDGE('',*,*,#49845,.T.) ;
#69733=ORIENTED_EDGE('',*,*,#49846,.T.) ;
#69734=ORIENTED_EDGE('',*,*,#49847,.T.) ;
#69735=ORIENTED_EDGE('',*,*,#49848,.T.) ;
#69736=ORIENTED_EDGE('',*,*,#49849,.T.) ;
#69737=ORIENTED_EDGE('',*,*,#49850,.T.) ;
#69738=ORIENTED_EDGE('',*,*,#49851,.T.) ;
#69739=ORIENTED_EDGE('',*,*,#49852,.T.) ;
#69740=ORIENTED_EDGE('',*,*,#49853,.T.) ;
#69741=ORIENTED_EDGE('',*,*,#49854,.T.) ;
#69742=ORIENTED_EDGE('',*,*,#49855,.T.) ;
#69743=ORIENTED_EDGE('',*,*,#49856,.T.) ;
#69744=ORIENTED_EDGE('',*,*,#49857,.T.) ;
#69745=ORIENTED_EDGE('',*,*,#49858,.T.) ;
#69746=ORIENTED_EDGE('',*,*,#49859,.T.) ;
#69747=ORIENTED_EDGE('',*,*,#49860,.T.) ;
#69748=ORIENTED_EDGE('',*,*,#49861,.T.) ;
#69749=ORIENTED_EDGE('',*,*,#49862,.T.) ;
#69750=ORIENTED_EDGE('',*,*,#49863,.T.) ;
#69751=ORIENTED_EDGE('',*,*,#49864,.T.) ;
#69752=ORIENTED_EDGE('',*,*,#49865,.T.) ;
#69753=ORIENTED_EDGE('',*,*,#49866,.T.) ;
#69754=ORIENTED_EDGE('',*,*,#49867,.T.) ;
#69755=ORIENTED_EDGE('',*,*,#49868,.F.) ;
#69756=ORIENTED_EDGE('',*,*,#49869,.T.) ;
#69757=ORIENTED_EDGE('',*,*,#49870,.F.) ;
#69758=ORIENTED_EDGE('',*,*,#49871,.T.) ;
#69759=ORIENTED_EDGE('',*,*,#49872,.F.) ;
#69760=ORIENTED_EDGE('',*,*,#49873,.T.) ;
#69761=ORIENTED_EDGE('',*,*,#49874,.F.) ;
#69762=ORIENTED_EDGE('',*,*,#49875,.T.) ;
#69763=ORIENTED_EDGE('',*,*,#49876,.F.) ;
#69764=ORIENTED_EDGE('',*,*,#49877,.T.) ;
#69765=ORIENTED_EDGE('',*,*,#49878,.F.) ;
#69766=ORIENTED_EDGE('',*,*,#49879,.T.) ;
#69767=ORIENTED_EDGE('',*,*,#49880,.F.) ;
#69768=ORIENTED_EDGE('',*,*,#49881,.T.) ;
#69769=ORIENTED_EDGE('',*,*,#49882,.F.) ;
#69770=ORIENTED_EDGE('',*,*,#49883,.T.) ;
#69771=ORIENTED_EDGE('',*,*,#49884,.T.) ;
#69772=ORIENTED_EDGE('',*,*,#49885,.T.) ;
#69773=ORIENTED_EDGE('',*,*,#49886,.T.) ;
#69774=ORIENTED_EDGE('',*,*,#49887,.F.) ;
#69775=ORIENTED_EDGE('',*,*,#49888,.T.) ;
#69776=ORIENTED_EDGE('',*,*,#49889,.T.) ;
#69777=ORIENTED_EDGE('',*,*,#49890,.T.) ;
#69778=ORIENTED_EDGE('',*,*,#49891,.T.) ;
#69779=ORIENTED_EDGE('',*,*,#49892,.T.) ;
#69780=ORIENTED_EDGE('',*,*,#49893,.T.) ;
#69781=ORIENTED_EDGE('',*,*,#49894,.T.) ;
#69782=ORIENTED_EDGE('',*,*,#49895,.T.) ;
#69783=ORIENTED_EDGE('',*,*,#49896,.F.) ;
#69784=ORIENTED_EDGE('',*,*,#49897,.T.) ;
#69785=ORIENTED_EDGE('',*,*,#49898,.T.) ;
#69786=ORIENTED_EDGE('',*,*,#49899,.T.) ;
#69787=ORIENTED_EDGE('',*,*,#49900,.T.) ;
#69788=ORIENTED_EDGE('',*,*,#49901,.T.) ;
#69789=ORIENTED_EDGE('',*,*,#49902,.T.) ;
#69790=ORIENTED_EDGE('',*,*,#49903,.T.) ;
#69791=ORIENTED_EDGE('',*,*,#49904,.F.) ;
#69792=ORIENTED_EDGE('',*,*,#49905,.T.) ;
#69793=ORIENTED_EDGE('',*,*,#49906,.T.) ;
#69794=ORIENTED_EDGE('',*,*,#49907,.T.) ;
#69795=ORIENTED_EDGE('',*,*,#49908,.T.) ;
#69796=ORIENTED_EDGE('',*,*,#49909,.T.) ;
#69797=ORIENTED_EDGE('',*,*,#49910,.T.) ;
#69798=ORIENTED_EDGE('',*,*,#49911,.T.) ;
#69799=ORIENTED_EDGE('',*,*,#49912,.T.) ;
#69800=ORIENTED_EDGE('',*,*,#49913,.F.) ;
#69801=ORIENTED_EDGE('',*,*,#49914,.T.) ;
#69802=ORIENTED_EDGE('',*,*,#49915,.T.) ;
#69803=ORIENTED_EDGE('',*,*,#49916,.T.) ;
#69804=ORIENTED_EDGE('',*,*,#49917,.T.) ;
#69805=ORIENTED_EDGE('',*,*,#49918,.T.) ;
#69806=ORIENTED_EDGE('',*,*,#49919,.T.) ;
#69807=ORIENTED_EDGE('',*,*,#49920,.T.) ;
#69808=ORIENTED_EDGE('',*,*,#49921,.T.) ;
#69809=ORIENTED_EDGE('',*,*,#49922,.F.) ;
#69810=ORIENTED_EDGE('',*,*,#49923,.T.) ;
#69811=ORIENTED_EDGE('',*,*,#49924,.T.) ;
#69812=ORIENTED_EDGE('',*,*,#49925,.T.) ;
#69813=ORIENTED_EDGE('',*,*,#49926,.T.) ;
#69814=ORIENTED_EDGE('',*,*,#49927,.T.) ;
#69815=ORIENTED_EDGE('',*,*,#49920,.F.) ;
#69816=ORIENTED_EDGE('',*,*,#49928,.T.) ;
#69817=ORIENTED_EDGE('',*,*,#49924,.F.) ;
#69818=ORIENTED_EDGE('',*,*,#49929,.T.) ;
#69819=ORIENTED_EDGE('',*,*,#49930,.T.) ;
#69820=ORIENTED_EDGE('',*,*,#49931,.T.) ;
#69821=ORIENTED_EDGE('',*,*,#49932,.T.) ;
#69822=ORIENTED_EDGE('',*,*,#49933,.T.) ;
#69823=ORIENTED_EDGE('',*,*,#49934,.T.) ;
#69824=ORIENTED_EDGE('',*,*,#49935,.T.) ;
#69825=ORIENTED_EDGE('',*,*,#49936,.T.) ;
#69826=ORIENTED_EDGE('',*,*,#49937,.T.) ;
#69827=ORIENTED_EDGE('',*,*,#49922,.T.) ;
#69828=ORIENTED_EDGE('',*,*,#49938,.T.) ;
#69829=ORIENTED_EDGE('',*,*,#49939,.T.) ;
#69830=ORIENTED_EDGE('',*,*,#49940,.T.) ;
#69831=ORIENTED_EDGE('',*,*,#49941,.T.) ;
#69832=ORIENTED_EDGE('',*,*,#49942,.T.) ;
#69833=ORIENTED_EDGE('',*,*,#49926,.F.) ;
#69834=ORIENTED_EDGE('',*,*,#49943,.T.) ;
#69835=ORIENTED_EDGE('',*,*,#49944,.T.) ;
#69836=ORIENTED_EDGE('',*,*,#49945,.T.) ;
#69837=ORIENTED_EDGE('',*,*,#49946,.T.) ;
#69838=ORIENTED_EDGE('',*,*,#49947,.T.) ;
#69839=ORIENTED_EDGE('',*,*,#49948,.T.) ;
#69840=ORIENTED_EDGE('',*,*,#49949,.T.) ;
#69841=ORIENTED_EDGE('',*,*,#49950,.T.) ;
#69842=ORIENTED_EDGE('',*,*,#49951,.T.) ;
#69843=ORIENTED_EDGE('',*,*,#49952,.T.) ;
#69844=ORIENTED_EDGE('',*,*,#49953,.T.) ;
#69845=ORIENTED_EDGE('',*,*,#49954,.T.) ;
#69846=ORIENTED_EDGE('',*,*,#49955,.T.) ;
#69847=ORIENTED_EDGE('',*,*,#49956,.T.) ;
#69848=ORIENTED_EDGE('',*,*,#49957,.T.) ;
#69849=ORIENTED_EDGE('',*,*,#49958,.T.) ;
#69850=ORIENTED_EDGE('',*,*,#49959,.T.) ;
#69851=ORIENTED_EDGE('',*,*,#49960,.T.) ;
#69852=ORIENTED_EDGE('',*,*,#49961,.T.) ;
#69853=ORIENTED_EDGE('',*,*,#49962,.T.) ;
#69854=ORIENTED_EDGE('',*,*,#49963,.T.) ;
#69855=ORIENTED_EDGE('',*,*,#49964,.T.) ;
#69856=ORIENTED_EDGE('',*,*,#49965,.T.) ;
#69857=ORIENTED_EDGE('',*,*,#49966,.F.) ;
#69858=ORIENTED_EDGE('',*,*,#49967,.T.) ;
#69859=ORIENTED_EDGE('',*,*,#49968,.F.) ;
#69860=ORIENTED_EDGE('',*,*,#49969,.T.) ;
#69861=ORIENTED_EDGE('',*,*,#49970,.F.) ;
#69862=ORIENTED_EDGE('',*,*,#49971,.T.) ;
#69863=ORIENTED_EDGE('',*,*,#49972,.F.) ;
#69864=ORIENTED_EDGE('',*,*,#49973,.T.) ;
#69865=ORIENTED_EDGE('',*,*,#49972,.T.) ;
#69866=ORIENTED_EDGE('',*,*,#49974,.T.) ;
#69867=ORIENTED_EDGE('',*,*,#49975,.T.) ;
#69868=ORIENTED_EDGE('',*,*,#49976,.T.) ;
#69869=ORIENTED_EDGE('',*,*,#49966,.T.) ;
#69870=ORIENTED_EDGE('',*,*,#49977,.T.) ;
#69871=ORIENTED_EDGE('',*,*,#49978,.T.) ;
#69872=ORIENTED_EDGE('',*,*,#49979,.T.) ;
#69873=ORIENTED_EDGE('',*,*,#49980,.T.) ;
#69874=ORIENTED_EDGE('',*,*,#49981,.T.) ;
#69875=ORIENTED_EDGE('',*,*,#49968,.T.) ;
#69876=ORIENTED_EDGE('',*,*,#49982,.T.) ;
#69877=ORIENTED_EDGE('',*,*,#49970,.T.) ;
#69878=ORIENTED_EDGE('',*,*,#49983,.T.) ;
#69879=ORIENTED_EDGE('',*,*,#49984,.T.) ;
#69880=ORIENTED_EDGE('',*,*,#49985,.T.) ;
#69881=ORIENTED_EDGE('',*,*,#49986,.T.) ;
#69882=ORIENTED_EDGE('',*,*,#49987,.T.) ;
#69883=ORIENTED_EDGE('',*,*,#49988,.T.) ;
#69884=ORIENTED_EDGE('',*,*,#49989,.T.) ;
#69885=ORIENTED_EDGE('',*,*,#49736,.T.) ;
#69886=ORIENTED_EDGE('',*,*,#49990,.T.) ;
#69887=ORIENTED_EDGE('',*,*,#49991,.T.) ;
#69888=ORIENTED_EDGE('',*,*,#49992,.F.) ;
#69889=ORIENTED_EDGE('',*,*,#49993,.T.) ;
#69890=ORIENTED_EDGE('',*,*,#48981,.T.) ;
#69891=ORIENTED_EDGE('',*,*,#48973,.T.) ;
#69892=ORIENTED_EDGE('',*,*,#48965,.T.) ;
#69893=ORIENTED_EDGE('',*,*,#48957,.T.) ;
#69894=ORIENTED_EDGE('',*,*,#48949,.T.) ;
#69895=ORIENTED_EDGE('',*,*,#48941,.T.) ;
#69896=ORIENTED_EDGE('',*,*,#48933,.T.) ;
#69897=ORIENTED_EDGE('',*,*,#48925,.T.) ;
#69898=ORIENTED_EDGE('',*,*,#48917,.T.) ;
#69899=ORIENTED_EDGE('',*,*,#48909,.T.) ;
#69900=ORIENTED_EDGE('',*,*,#49994,.T.) ;
#69901=ORIENTED_EDGE('',*,*,#49995,.F.) ;
#69902=ORIENTED_EDGE('',*,*,#49996,.T.) ;
#69903=ORIENTED_EDGE('',*,*,#49997,.T.) ;
#69904=ORIENTED_EDGE('',*,*,#49998,.T.) ;
#69905=ORIENTED_EDGE('',*,*,#49999,.T.) ;
#69906=ORIENTED_EDGE('',*,*,#50000,.T.) ;
#69907=ORIENTED_EDGE('',*,*,#50001,.T.) ;
#69908=ORIENTED_EDGE('',*,*,#50002,.T.) ;
#69909=ORIENTED_EDGE('',*,*,#50003,.T.) ;
#69910=ORIENTED_EDGE('',*,*,#50004,.T.) ;
#69911=ORIENTED_EDGE('',*,*,#50005,.T.) ;
#69912=ORIENTED_EDGE('',*,*,#50006,.T.) ;
#69913=ORIENTED_EDGE('',*,*,#50007,.T.) ;
#69914=ORIENTED_EDGE('',*,*,#50008,.F.) ;
#69915=ORIENTED_EDGE('',*,*,#50009,.T.) ;
#69916=ORIENTED_EDGE('',*,*,#50010,.T.) ;
#69917=ORIENTED_EDGE('',*,*,#50011,.T.) ;
#69918=ORIENTED_EDGE('',*,*,#50012,.T.) ;
#69919=ORIENTED_EDGE('',*,*,#50013,.T.) ;
#69920=ORIENTED_EDGE('',*,*,#50014,.T.) ;
#69921=ORIENTED_EDGE('',*,*,#50015,.T.) ;
#69922=ORIENTED_EDGE('',*,*,#50016,.T.) ;
#69923=ORIENTED_EDGE('',*,*,#50017,.T.) ;
#69924=ORIENTED_EDGE('',*,*,#50018,.T.) ;
#69925=ORIENTED_EDGE('',*,*,#50019,.T.) ;
#69926=ORIENTED_EDGE('',*,*,#50020,.T.) ;
#69927=ORIENTED_EDGE('',*,*,#50021,.T.) ;
#69928=ORIENTED_EDGE('',*,*,#50022,.F.) ;
#69929=ORIENTED_EDGE('',*,*,#50023,.T.) ;
#69930=ORIENTED_EDGE('',*,*,#50024,.T.) ;
#69931=ORIENTED_EDGE('',*,*,#50025,.T.) ;
#69932=ORIENTED_EDGE('',*,*,#50026,.T.) ;
#69933=ORIENTED_EDGE('',*,*,#49739,.T.) ;
#69934=ORIENTED_EDGE('',*,*,#50027,.T.) ;
#69935=ORIENTED_EDGE('',*,*,#50028,.T.) ;
#69936=ORIENTED_EDGE('',*,*,#50029,.T.) ;
#69937=ORIENTED_EDGE('',*,*,#50030,.T.) ;
#69938=ORIENTED_EDGE('',*,*,#50031,.T.) ;
#69939=ORIENTED_EDGE('',*,*,#50032,.T.) ;
#69940=ORIENTED_EDGE('',*,*,#50033,.T.) ;
#69941=ORIENTED_EDGE('',*,*,#50034,.T.) ;
#69942=ORIENTED_EDGE('',*,*,#50035,.T.) ;
#69943=ORIENTED_EDGE('',*,*,#50036,.T.) ;
#69944=ORIENTED_EDGE('',*,*,#50037,.T.) ;
#69945=ORIENTED_EDGE('',*,*,#50038,.T.) ;
#69946=ORIENTED_EDGE('',*,*,#50039,.T.) ;
#69947=ORIENTED_EDGE('',*,*,#50040,.T.) ;
#69948=ORIENTED_EDGE('',*,*,#50041,.T.) ;
#69949=ORIENTED_EDGE('',*,*,#50042,.T.) ;
#69950=ORIENTED_EDGE('',*,*,#50043,.T.) ;
#69951=ORIENTED_EDGE('',*,*,#50044,.T.) ;
#69952=ORIENTED_EDGE('',*,*,#50045,.T.) ;
#69953=ORIENTED_EDGE('',*,*,#50046,.T.) ;
#69954=ORIENTED_EDGE('',*,*,#49284,.T.) ;
#69955=ORIENTED_EDGE('',*,*,#49315,.T.) ;
#69956=ORIENTED_EDGE('',*,*,#50047,.T.) ;
#69957=ORIENTED_EDGE('',*,*,#50048,.T.) ;
#69958=ORIENTED_EDGE('',*,*,#50049,.T.) ;
#69959=ORIENTED_EDGE('',*,*,#50050,.T.) ;
#69960=ORIENTED_EDGE('',*,*,#50051,.T.) ;
#69961=ORIENTED_EDGE('',*,*,#50052,.T.) ;
#69962=ORIENTED_EDGE('',*,*,#50053,.T.) ;
#69963=ORIENTED_EDGE('',*,*,#50054,.T.) ;
#69964=ORIENTED_EDGE('',*,*,#50055,.T.) ;
#69965=ORIENTED_EDGE('',*,*,#50056,.T.) ;
#69966=ORIENTED_EDGE('',*,*,#50057,.T.) ;
#69967=ORIENTED_EDGE('',*,*,#50058,.T.) ;
#69968=ORIENTED_EDGE('',*,*,#50059,.T.) ;
#69969=ORIENTED_EDGE('',*,*,#50060,.T.) ;
#69970=ORIENTED_EDGE('',*,*,#50061,.T.) ;
#69971=ORIENTED_EDGE('',*,*,#50062,.T.) ;
#69972=ORIENTED_EDGE('',*,*,#50063,.T.) ;
#69973=ORIENTED_EDGE('',*,*,#50064,.T.) ;
#69974=ORIENTED_EDGE('',*,*,#50065,.T.) ;
#69975=ORIENTED_EDGE('',*,*,#50066,.T.) ;
#69976=ORIENTED_EDGE('',*,*,#50067,.F.) ;
#69977=ORIENTED_EDGE('',*,*,#50068,.T.) ;
#69978=ORIENTED_EDGE('',*,*,#50069,.F.) ;
#69979=ORIENTED_EDGE('',*,*,#50070,.T.) ;
#69980=ORIENTED_EDGE('',*,*,#50071,.F.) ;
#69981=ORIENTED_EDGE('',*,*,#50072,.T.) ;
#69982=ORIENTED_EDGE('',*,*,#50073,.F.) ;
#69983=ORIENTED_EDGE('',*,*,#50074,.T.) ;
#69984=ORIENTED_EDGE('',*,*,#50075,.T.) ;
#69985=ORIENTED_EDGE('',*,*,#50076,.T.) ;
#69986=ORIENTED_EDGE('',*,*,#50073,.T.) ;
#69987=ORIENTED_EDGE('',*,*,#50077,.T.) ;
#69988=ORIENTED_EDGE('',*,*,#50078,.T.) ;
#69989=ORIENTED_EDGE('',*,*,#50079,.T.) ;
#69990=ORIENTED_EDGE('',*,*,#50067,.T.) ;
#69991=ORIENTED_EDGE('',*,*,#50080,.T.) ;
#69992=ORIENTED_EDGE('',*,*,#50069,.T.) ;
#69993=ORIENTED_EDGE('',*,*,#50081,.T.) ;
#69994=ORIENTED_EDGE('',*,*,#50082,.T.) ;
#69995=ORIENTED_EDGE('',*,*,#50083,.T.) ;
#69996=ORIENTED_EDGE('',*,*,#50084,.T.) ;
#69997=ORIENTED_EDGE('',*,*,#50085,.T.) ;
#69998=ORIENTED_EDGE('',*,*,#50071,.T.) ;
#69999=ORIENTED_EDGE('',*,*,#50086,.T.) ;
#70000=ORIENTED_EDGE('',*,*,#50087,.T.) ;
#70001=ORIENTED_EDGE('',*,*,#50088,.T.) ;
#70002=ORIENTED_EDGE('',*,*,#50089,.T.) ;
#70003=ORIENTED_EDGE('',*,*,#50090,.T.) ;
#70004=ORIENTED_EDGE('',*,*,#49297,.T.) ;
#70005=ORIENTED_EDGE('',*,*,#49313,.T.) ;
#70006=ORIENTED_EDGE('',*,*,#50091,.T.) ;
#70007=ORIENTED_EDGE('',*,*,#49299,.T.) ;
#70008=ORIENTED_EDGE('',*,*,#50092,.T.) ;
#70009=ORIENTED_EDGE('',*,*,#49311,.F.) ;
#70010=ORIENTED_EDGE('',*,*,#50093,.T.) ;
#70011=ORIENTED_EDGE('',*,*,#49303,.F.) ;
#70012=ORIENTED_EDGE('',*,*,#50094,.T.) ;
#70013=ORIENTED_EDGE('',*,*,#49307,.T.) ;
#70014=ORIENTED_EDGE('',*,*,#50095,.T.) ;
#70015=ORIENTED_EDGE('',*,*,#49301,.T.) ;
#70016=ORIENTED_EDGE('',*,*,#50096,.T.) ;
#70017=ORIENTED_EDGE('',*,*,#49309,.T.) ;
#70018=ORIENTED_EDGE('',*,*,#50097,.T.) ;
#70019=ORIENTED_EDGE('',*,*,#49005,.T.) ;
#70020=ORIENTED_EDGE('',*,*,#50098,.T.) ;
#70021=ORIENTED_EDGE('',*,*,#49295,.F.) ;
#70022=ORIENTED_EDGE('',*,*,#48919,.T.) ;
#70023=ORIENTED_EDGE('',*,*,#49296,.T.) ;
#70024=ORIENTED_EDGE('',*,*,#50099,.T.) ;
#70025=ORIENTED_EDGE('',*,*,#49292,.F.) ;
#70026=ORIENTED_EDGE('',*,*,#48911,.T.) ;
#70027=ORIENTED_EDGE('',*,*,#49293,.T.) ;
#70028=ORIENTED_EDGE('',*,*,#50100,.T.) ;
#70029=ORIENTED_EDGE('',*,*,#50101,.T.) ;
#70030=ORIENTED_EDGE('',*,*,#50102,.T.) ;
#70031=ORIENTED_EDGE('',*,*,#50103,.T.) ;
#70032=ORIENTED_EDGE('',*,*,#50104,.T.) ;
#70033=ORIENTED_EDGE('',*,*,#49289,.F.) ;
#70034=ORIENTED_EDGE('',*,*,#50105,.T.) ;
#70035=ORIENTED_EDGE('',*,*,#49290,.T.) ;
#70036=ORIENTED_EDGE('',*,*,#50106,.T.) ;
#70037=ORIENTED_EDGE('',*,*,#49286,.F.) ;
#70038=ORIENTED_EDGE('',*,*,#48983,.T.) ;
#70039=ORIENTED_EDGE('',*,*,#49287,.T.) ;
#70040=ORIENTED_EDGE('',*,*,#50107,.T.) ;
#70041=ORIENTED_EDGE('',*,*,#48986,.F.) ;
#70042=ORIENTED_EDGE('',*,*,#48975,.T.) ;
#70043=ORIENTED_EDGE('',*,*,#50108,.T.) ;
#70044=ORIENTED_EDGE('',*,*,#50109,.T.) ;
#70045=ORIENTED_EDGE('',*,*,#50110,.F.) ;
#70046=ORIENTED_EDGE('',*,*,#50111,.T.) ;
#70047=ORIENTED_EDGE('',*,*,#50110,.T.) ;
#70048=ORIENTED_EDGE('',*,*,#50112,.T.) ;
#70049=ORIENTED_EDGE('',*,*,#50113,.F.) ;
#70050=ORIENTED_EDGE('',*,*,#50114,.T.) ;
#70051=ORIENTED_EDGE('',*,*,#50113,.T.) ;
#70052=ORIENTED_EDGE('',*,*,#50115,.T.) ;
#70053=ORIENTED_EDGE('',*,*,#50116,.F.) ;
#70054=ORIENTED_EDGE('',*,*,#50117,.T.) ;
#70055=ORIENTED_EDGE('',*,*,#50116,.T.) ;
#70056=ORIENTED_EDGE('',*,*,#50118,.T.) ;
#70057=ORIENTED_EDGE('',*,*,#50119,.F.) ;
#70058=ORIENTED_EDGE('',*,*,#50120,.T.) ;
#70059=ORIENTED_EDGE('',*,*,#50119,.T.) ;
#70060=ORIENTED_EDGE('',*,*,#50121,.T.) ;
#70061=ORIENTED_EDGE('',*,*,#50122,.F.) ;
#70062=ORIENTED_EDGE('',*,*,#50123,.T.) ;
#70063=ORIENTED_EDGE('',*,*,#50122,.T.) ;
#70064=ORIENTED_EDGE('',*,*,#50124,.T.) ;
#70065=ORIENTED_EDGE('',*,*,#50125,.F.) ;
#70066=ORIENTED_EDGE('',*,*,#50126,.T.) ;
#70067=ORIENTED_EDGE('',*,*,#50125,.T.) ;
#70068=ORIENTED_EDGE('',*,*,#50127,.T.) ;
#70069=ORIENTED_EDGE('',*,*,#50128,.F.) ;
#70070=ORIENTED_EDGE('',*,*,#50129,.T.) ;
#70071=ORIENTED_EDGE('',*,*,#50108,.F.) ;
#70072=ORIENTED_EDGE('',*,*,#50130,.T.) ;
#70073=ORIENTED_EDGE('',*,*,#50128,.T.) ;
#70074=ORIENTED_EDGE('',*,*,#50131,.T.) ;
#70075=ORIENTED_EDGE('',*,*,#50132,.T.) ;
#70076=ORIENTED_EDGE('',*,*,#50133,.T.) ;
#70077=ORIENTED_EDGE('',*,*,#50134,.T.) ;
#70078=ORIENTED_EDGE('',*,*,#50135,.T.) ;
#70079=ORIENTED_EDGE('',*,*,#49834,.F.) ;
#70080=ORIENTED_EDGE('',*,*,#50136,.T.) ;
#70081=ORIENTED_EDGE('',*,*,#49907,.F.) ;
#70082=ORIENTED_EDGE('',*,*,#50137,.F.) ;
#70083=ORIENTED_EDGE('',*,*,#50138,.F.) ;
#70084=ORIENTED_EDGE('',*,*,#50137,.T.) ;
#70085=ORIENTED_EDGE('',*,*,#50139,.F.) ;
#70086=ORIENTED_EDGE('',*,*,#49833,.F.) ;
#70087=ORIENTED_EDGE('',*,*,#50140,.T.) ;
#70088=ORIENTED_EDGE('',*,*,#49672,.F.) ;
#70089=ORIENTED_EDGE('',*,*,#50141,.T.) ;
#70090=ORIENTED_EDGE('',*,*,#50139,.T.) ;
#70091=ORIENTED_EDGE('',*,*,#49906,.F.) ;
#70092=ORIENTED_EDGE('',*,*,#50142,.F.) ;
#70093=ORIENTED_EDGE('',*,*,#49746,.F.) ;
#70094=ORIENTED_EDGE('',*,*,#50138,.T.) ;
#70095=ORIENTED_EDGE('',*,*,#49745,.F.) ;
#70096=ORIENTED_EDGE('',*,*,#50143,.F.) ;
#70097=ORIENTED_EDGE('',*,*,#49835,.F.) ;
#70098=ORIENTED_EDGE('',*,*,#49893,.F.) ;
#70099=ORIENTED_EDGE('',*,*,#50144,.T.) ;
#70100=ORIENTED_EDGE('',*,*,#49832,.F.) ;
#70101=ORIENTED_EDGE('',*,*,#50145,.F.) ;
#70102=ORIENTED_EDGE('',*,*,#49901,.F.) ;
#70103=ORIENTED_EDGE('',*,*,#50146,.T.) ;
#70104=ORIENTED_EDGE('',*,*,#49830,.F.) ;
#70105=ORIENTED_EDGE('',*,*,#50147,.F.) ;
#70106=ORIENTED_EDGE('',*,*,#50148,.F.) ;
#70107=ORIENTED_EDGE('',*,*,#50149,.T.) ;
#70108=ORIENTED_EDGE('',*,*,#50150,.T.) ;
#70109=ORIENTED_EDGE('',*,*,#49902,.F.) ;
#70110=ORIENTED_EDGE('',*,*,#50151,.F.) ;
#70111=ORIENTED_EDGE('',*,*,#50142,.T.) ;
#70112=ORIENTED_EDGE('',*,*,#50152,.F.) ;
#70113=ORIENTED_EDGE('',*,*,#50145,.T.) ;
#70114=ORIENTED_EDGE('',*,*,#50143,.T.) ;
#70115=ORIENTED_EDGE('',*,*,#50153,.F.) ;
#70116=ORIENTED_EDGE('',*,*,#49831,.F.) ;
#70117=ORIENTED_EDGE('',*,*,#50154,.T.) ;
#70118=ORIENTED_EDGE('',*,*,#49318,.F.) ;
#70119=ORIENTED_EDGE('',*,*,#50155,.T.) ;
#70120=ORIENTED_EDGE('',*,*,#50156,.F.) ;
#70121=ORIENTED_EDGE('',*,*,#50157,.T.) ;
#70122=ORIENTED_EDGE('',*,*,#50148,.T.) ;
#70123=ORIENTED_EDGE('',*,*,#50147,.T.) ;
#70124=ORIENTED_EDGE('',*,*,#49903,.F.) ;
#70125=ORIENTED_EDGE('',*,*,#50158,.T.) ;
#70126=ORIENTED_EDGE('',*,*,#50159,.T.) ;
#70127=ORIENTED_EDGE('',*,*,#50160,.T.) ;
#70128=ORIENTED_EDGE('',*,*,#49825,.F.) ;
#70129=ORIENTED_EDGE('',*,*,#50161,.F.) ;
#70130=ORIENTED_EDGE('',*,*,#50152,.T.) ;
#70131=ORIENTED_EDGE('',*,*,#49905,.F.) ;
#70132=ORIENTED_EDGE('',*,*,#50162,.F.) ;
#70133=ORIENTED_EDGE('',*,*,#49824,.F.) ;
#70134=ORIENTED_EDGE('',*,*,#50151,.T.) ;
#70135=ORIENTED_EDGE('',*,*,#49823,.F.) ;
#70136=ORIENTED_EDGE('',*,*,#50163,.F.) ;
#70137=ORIENTED_EDGE('',*,*,#49747,.F.) ;
#70138=ORIENTED_EDGE('',*,*,#50153,.T.) ;
#70139=ORIENTED_EDGE('',*,*,#49744,.F.) ;
#70140=ORIENTED_EDGE('',*,*,#50164,.F.) ;
#70141=ORIENTED_EDGE('',*,*,#49894,.F.) ;
#70142=ORIENTED_EDGE('',*,*,#49828,.F.) ;
#70143=ORIENTED_EDGE('',*,*,#50165,.T.) ;
#70144=ORIENTED_EDGE('',*,*,#49884,.F.) ;
#70145=ORIENTED_EDGE('',*,*,#50166,.F.) ;
#70146=ORIENTED_EDGE('',*,*,#50167,.F.) ;
#70147=ORIENTED_EDGE('',*,*,#48900,.T.) ;
#70148=ORIENTED_EDGE('',*,*,#50156,.T.) ;
#70149=ORIENTED_EDGE('',*,*,#49829,.F.) ;
#70150=ORIENTED_EDGE('',*,*,#49904,.T.) ;
#70151=ORIENTED_EDGE('',*,*,#50161,.T.) ;
#70152=ORIENTED_EDGE('',*,*,#50168,.F.) ;
#70153=ORIENTED_EDGE('',*,*,#50162,.T.) ;
#70154=ORIENTED_EDGE('',*,*,#50164,.T.) ;
#70155=ORIENTED_EDGE('',*,*,#50163,.T.) ;
#70156=ORIENTED_EDGE('',*,*,#50169,.F.) ;
#70157=ORIENTED_EDGE('',*,*,#50170,.F.) ;
#70158=ORIENTED_EDGE('',*,*,#50171,.T.) ;
#70159=ORIENTED_EDGE('',*,*,#50167,.T.) ;
#70160=ORIENTED_EDGE('',*,*,#50166,.T.) ;
#70161=ORIENTED_EDGE('',*,*,#50168,.T.) ;
#70162=ORIENTED_EDGE('',*,*,#49827,.F.) ;
#70163=ORIENTED_EDGE('',*,*,#50172,.F.) ;
#70164=ORIENTED_EDGE('',*,*,#49821,.F.) ;
#70165=ORIENTED_EDGE('',*,*,#50169,.T.) ;
#70166=ORIENTED_EDGE('',*,*,#49822,.F.) ;
#70167=ORIENTED_EDGE('',*,*,#50173,.F.) ;
#70168=ORIENTED_EDGE('',*,*,#49895,.F.) ;
#70169=ORIENTED_EDGE('',*,*,#49898,.F.) ;
#70170=ORIENTED_EDGE('',*,*,#50174,.T.) ;
#70171=ORIENTED_EDGE('',*,*,#50175,.T.) ;
#70172=ORIENTED_EDGE('',*,*,#50170,.T.) ;
#70173=ORIENTED_EDGE('',*,*,#50173,.T.) ;
#70174=ORIENTED_EDGE('',*,*,#50172,.T.) ;
#70175=ORIENTED_EDGE('',*,*,#50176,.F.) ;
#70176=ORIENTED_EDGE('',*,*,#49896,.T.) ;
#70177=ORIENTED_EDGE('',*,*,#49826,.F.) ;
#70178=ORIENTED_EDGE('',*,*,#50177,.T.) ;
#70179=ORIENTED_EDGE('',*,*,#50178,.T.) ;
#70180=ORIENTED_EDGE('',*,*,#50179,.T.) ;
#70181=ORIENTED_EDGE('',*,*,#49897,.F.) ;
#70182=ORIENTED_EDGE('',*,*,#50176,.T.) ;
#70183=ORIENTED_EDGE('',*,*,#50180,.F.) ;
#70184=ORIENTED_EDGE('',*,*,#50181,.F.) ;
#70185=ORIENTED_EDGE('',*,*,#50182,.F.) ;
#70186=ORIENTED_EDGE('',*,*,#50181,.T.) ;
#70187=ORIENTED_EDGE('',*,*,#50042,.F.) ;
#70188=ORIENTED_EDGE('',*,*,#50183,.F.) ;
#70189=ORIENTED_EDGE('',*,*,#50040,.F.) ;
#70190=ORIENTED_EDGE('',*,*,#50182,.T.) ;
#70191=ORIENTED_EDGE('',*,*,#50039,.F.) ;
#70192=ORIENTED_EDGE('',*,*,#50184,.F.) ;
#70193=ORIENTED_EDGE('',*,*,#50029,.F.) ;
#70194=ORIENTED_EDGE('',*,*,#50180,.T.) ;
#70195=ORIENTED_EDGE('',*,*,#50032,.F.) ;
#70196=ORIENTED_EDGE('',*,*,#50185,.F.) ;
#70197=ORIENTED_EDGE('',*,*,#50043,.F.) ;
#70198=ORIENTED_EDGE('',*,*,#50020,.F.) ;
#70199=ORIENTED_EDGE('',*,*,#50186,.T.) ;
#70200=ORIENTED_EDGE('',*,*,#50044,.F.) ;
#70201=ORIENTED_EDGE('',*,*,#50187,.F.) ;
#70202=ORIENTED_EDGE('',*,*,#50045,.F.) ;
#70203=ORIENTED_EDGE('',*,*,#50188,.T.) ;
#70204=ORIENTED_EDGE('',*,*,#49796,.F.) ;
#70205=ORIENTED_EDGE('',*,*,#50189,.T.) ;
#70206=ORIENTED_EDGE('',*,*,#50190,.F.) ;
#70207=ORIENTED_EDGE('',*,*,#50183,.T.) ;
#70208=ORIENTED_EDGE('',*,*,#50191,.F.) ;
#70209=ORIENTED_EDGE('',*,*,#50192,.F.) ;
#70210=ORIENTED_EDGE('',*,*,#50184,.T.) ;
#70211=ORIENTED_EDGE('',*,*,#50193,.F.) ;
#70212=ORIENTED_EDGE('',*,*,#49817,.T.) ;
#70213=ORIENTED_EDGE('',*,*,#50187,.T.) ;
#70214=ORIENTED_EDGE('',*,*,#50185,.T.) ;
#70215=ORIENTED_EDGE('',*,*,#50194,.F.) ;
#70216=ORIENTED_EDGE('',*,*,#50046,.F.) ;
#70217=ORIENTED_EDGE('',*,*,#50195,.T.) ;
#70218=ORIENTED_EDGE('',*,*,#50010,.F.) ;
#70219=ORIENTED_EDGE('',*,*,#50196,.F.) ;
#70220=ORIENTED_EDGE('',*,*,#50191,.T.) ;
#70221=ORIENTED_EDGE('',*,*,#50041,.F.) ;
#70222=ORIENTED_EDGE('',*,*,#50197,.F.) ;
#70223=ORIENTED_EDGE('',*,*,#50036,.F.) ;
#70224=ORIENTED_EDGE('',*,*,#50190,.T.) ;
#70225=ORIENTED_EDGE('',*,*,#50035,.F.) ;
#70226=ORIENTED_EDGE('',*,*,#50198,.F.) ;
#70227=ORIENTED_EDGE('',*,*,#50037,.F.) ;
#70228=ORIENTED_EDGE('',*,*,#50193,.T.) ;
#70229=ORIENTED_EDGE('',*,*,#50038,.F.) ;
#70230=ORIENTED_EDGE('',*,*,#50199,.F.) ;
#70231=ORIENTED_EDGE('',*,*,#49818,.F.) ;
#70232=ORIENTED_EDGE('',*,*,#50192,.T.) ;
#70233=ORIENTED_EDGE('',*,*,#49816,.F.) ;
#70234=ORIENTED_EDGE('',*,*,#50200,.F.) ;
#70235=ORIENTED_EDGE('',*,*,#50030,.F.) ;
#70236=ORIENTED_EDGE('',*,*,#50194,.T.) ;
#70237=ORIENTED_EDGE('',*,*,#50031,.F.) ;
#70238=ORIENTED_EDGE('',*,*,#50201,.F.) ;
#70239=ORIENTED_EDGE('',*,*,#50021,.F.) ;
#70240=ORIENTED_EDGE('',*,*,#50197,.T.) ;
#70241=ORIENTED_EDGE('',*,*,#50196,.T.) ;
#70242=ORIENTED_EDGE('',*,*,#50202,.F.) ;
#70243=ORIENTED_EDGE('',*,*,#50199,.T.) ;
#70244=ORIENTED_EDGE('',*,*,#50198,.T.) ;
#70245=ORIENTED_EDGE('',*,*,#50203,.F.) ;
#70246=ORIENTED_EDGE('',*,*,#49819,.T.) ;
#70247=ORIENTED_EDGE('',*,*,#50201,.T.) ;
#70248=ORIENTED_EDGE('',*,*,#50200,.T.) ;
#70249=ORIENTED_EDGE('',*,*,#50204,.F.) ;
#70250=ORIENTED_EDGE('',*,*,#50022,.T.) ;
#70251=ORIENTED_EDGE('',*,*,#50202,.T.) ;
#70252=ORIENTED_EDGE('',*,*,#50009,.F.) ;
#70253=ORIENTED_EDGE('',*,*,#50205,.F.) ;
#70254=ORIENTED_EDGE('',*,*,#50033,.F.) ;
#70255=ORIENTED_EDGE('',*,*,#50203,.T.) ;
#70256=ORIENTED_EDGE('',*,*,#50034,.F.) ;
#70257=ORIENTED_EDGE('',*,*,#50206,.F.) ;
#70258=ORIENTED_EDGE('',*,*,#49820,.F.) ;
#70259=ORIENTED_EDGE('',*,*,#50204,.T.) ;
#70260=ORIENTED_EDGE('',*,*,#49815,.F.) ;
#70261=ORIENTED_EDGE('',*,*,#50207,.F.) ;
#70262=ORIENTED_EDGE('',*,*,#50023,.F.) ;
#70263=ORIENTED_EDGE('',*,*,#50027,.F.) ;
#70264=ORIENTED_EDGE('',*,*,#50208,.T.) ;
#70265=ORIENTED_EDGE('',*,*,#50016,.F.) ;
#70266=ORIENTED_EDGE('',*,*,#50209,.F.) ;
#70267=ORIENTED_EDGE('',*,*,#50028,.F.) ;
#70268=ORIENTED_EDGE('',*,*,#50210,.F.) ;
#70269=ORIENTED_EDGE('',*,*,#49728,.F.) ;
#70270=ORIENTED_EDGE('',*,*,#50211,.F.) ;
#70271=ORIENTED_EDGE('',*,*,#50205,.T.) ;
#70272=ORIENTED_EDGE('',*,*,#50008,.T.) ;
#70273=ORIENTED_EDGE('',*,*,#50212,.F.) ;
#70274=ORIENTED_EDGE('',*,*,#50206,.T.) ;
#70275=ORIENTED_EDGE('',*,*,#50213,.F.) ;
#70276=ORIENTED_EDGE('',*,*,#50207,.T.) ;
#70277=ORIENTED_EDGE('',*,*,#50214,.F.) ;
#70278=ORIENTED_EDGE('',*,*,#50210,.T.) ;
#70279=ORIENTED_EDGE('',*,*,#50209,.T.) ;
#70280=ORIENTED_EDGE('',*,*,#50215,.F.) ;
#70281=ORIENTED_EDGE('',*,*,#50212,.T.) ;
#70282=ORIENTED_EDGE('',*,*,#50007,.F.) ;
#70283=ORIENTED_EDGE('',*,*,#50216,.F.) ;
#70284=ORIENTED_EDGE('',*,*,#49813,.F.) ;
#70285=ORIENTED_EDGE('',*,*,#50214,.T.) ;
#70286=ORIENTED_EDGE('',*,*,#49814,.F.) ;
#70287=ORIENTED_EDGE('',*,*,#50217,.F.) ;
#70288=ORIENTED_EDGE('',*,*,#50015,.F.) ;
#70289=ORIENTED_EDGE('',*,*,#50213,.T.) ;
#70290=ORIENTED_EDGE('',*,*,#50014,.F.) ;
#70291=ORIENTED_EDGE('',*,*,#50218,.F.) ;
#70292=ORIENTED_EDGE('',*,*,#50024,.F.) ;
#70293=ORIENTED_EDGE('',*,*,#50215,.T.) ;
#70294=ORIENTED_EDGE('',*,*,#50025,.F.) ;
#70295=ORIENTED_EDGE('',*,*,#50219,.F.) ;
#70296=ORIENTED_EDGE('',*,*,#49729,.F.) ;
#70297=ORIENTED_EDGE('',*,*,#50217,.T.) ;
#70298=ORIENTED_EDGE('',*,*,#50216,.T.) ;
#70299=ORIENTED_EDGE('',*,*,#50220,.F.) ;
#70300=ORIENTED_EDGE('',*,*,#50219,.T.) ;
#70301=ORIENTED_EDGE('',*,*,#50218,.T.) ;
#70302=ORIENTED_EDGE('',*,*,#50221,.F.) ;
#70303=ORIENTED_EDGE('',*,*,#49730,.T.) ;
#70304=ORIENTED_EDGE('',*,*,#50000,.F.) ;
#70305=ORIENTED_EDGE('',*,*,#50222,.T.) ;
#70306=ORIENTED_EDGE('',*,*,#49734,.F.) ;
#70307=ORIENTED_EDGE('',*,*,#50223,.F.) ;
#70308=ORIENTED_EDGE('',*,*,#50004,.F.) ;
#70309=ORIENTED_EDGE('',*,*,#50224,.T.) ;
#70310=ORIENTED_EDGE('',*,*,#50001,.F.) ;
#70311=ORIENTED_EDGE('',*,*,#50225,.F.) ;
#70312=ORIENTED_EDGE('',*,*,#50220,.T.) ;
#70313=ORIENTED_EDGE('',*,*,#50006,.F.) ;
#70314=ORIENTED_EDGE('',*,*,#50226,.F.) ;
#70315=ORIENTED_EDGE('',*,*,#50012,.F.) ;
#70316=ORIENTED_EDGE('',*,*,#50221,.T.) ;
#70317=ORIENTED_EDGE('',*,*,#50013,.F.) ;
#70318=ORIENTED_EDGE('',*,*,#50227,.F.) ;
#70319=ORIENTED_EDGE('',*,*,#49731,.F.) ;
#70320=ORIENTED_EDGE('',*,*,#50225,.T.) ;
#70321=ORIENTED_EDGE('',*,*,#50223,.T.) ;
#70322=ORIENTED_EDGE('',*,*,#50228,.F.) ;
#70323=ORIENTED_EDGE('',*,*,#50227,.T.) ;
#70324=ORIENTED_EDGE('',*,*,#50226,.T.) ;
#70325=ORIENTED_EDGE('',*,*,#50229,.F.) ;
#70326=ORIENTED_EDGE('',*,*,#49732,.T.) ;
#70327=ORIENTED_EDGE('',*,*,#50228,.T.) ;
#70328=ORIENTED_EDGE('',*,*,#49733,.F.) ;
#70329=ORIENTED_EDGE('',*,*,#50229,.T.) ;
#70330=ORIENTED_EDGE('',*,*,#50005,.F.) ;
#70331=ORIENTED_EDGE('',*,*,#50230,.F.) ;
#70332=ORIENTED_EDGE('',*,*,#49805,.F.) ;
#70333=ORIENTED_EDGE('',*,*,#50231,.F.) ;
#70334=ORIENTED_EDGE('',*,*,#50115,.F.) ;
#70335=ORIENTED_EDGE('',*,*,#50231,.T.) ;
#70336=ORIENTED_EDGE('',*,*,#49804,.F.) ;
#70337=ORIENTED_EDGE('',*,*,#50232,.F.) ;
#70338=ORIENTED_EDGE('',*,*,#50118,.F.) ;
#70339=ORIENTED_EDGE('',*,*,#50230,.T.) ;
#70340=ORIENTED_EDGE('',*,*,#50112,.F.) ;
#70341=ORIENTED_EDGE('',*,*,#50233,.F.) ;
#70342=ORIENTED_EDGE('',*,*,#49806,.F.) ;
#70343=ORIENTED_EDGE('',*,*,#50232,.T.) ;
#70344=ORIENTED_EDGE('',*,*,#49803,.F.) ;
#70345=ORIENTED_EDGE('',*,*,#50234,.F.) ;
#70346=ORIENTED_EDGE('',*,*,#50121,.F.) ;
#70347=ORIENTED_EDGE('',*,*,#50233,.T.) ;
#70348=ORIENTED_EDGE('',*,*,#50109,.F.) ;
#70349=ORIENTED_EDGE('',*,*,#50235,.F.) ;
#70350=ORIENTED_EDGE('',*,*,#49807,.F.) ;
#70351=ORIENTED_EDGE('',*,*,#50234,.T.) ;
#70352=ORIENTED_EDGE('',*,*,#49802,.F.) ;
#70353=ORIENTED_EDGE('',*,*,#50236,.F.) ;
#70354=ORIENTED_EDGE('',*,*,#50124,.F.) ;
#70355=ORIENTED_EDGE('',*,*,#50235,.T.) ;
#70356=ORIENTED_EDGE('',*,*,#50131,.F.) ;
#70357=ORIENTED_EDGE('',*,*,#50237,.F.) ;
#70358=ORIENTED_EDGE('',*,*,#49800,.F.) ;
#70359=ORIENTED_EDGE('',*,*,#50236,.T.) ;
#70360=ORIENTED_EDGE('',*,*,#49801,.F.) ;
#70361=ORIENTED_EDGE('',*,*,#50237,.T.) ;
#70362=ORIENTED_EDGE('',*,*,#50127,.F.) ;
#70363=ORIENTED_EDGE('',*,*,#50238,.F.) ;
#70364=ORIENTED_EDGE('',*,*,#49881,.F.) ;
#70365=ORIENTED_EDGE('',*,*,#50239,.F.) ;
#70366=ORIENTED_EDGE('',*,*,#49961,.F.) ;
#70367=ORIENTED_EDGE('',*,*,#50239,.T.) ;
#70368=ORIENTED_EDGE('',*,*,#49880,.T.) ;
#70369=ORIENTED_EDGE('',*,*,#50240,.F.) ;
#70370=ORIENTED_EDGE('',*,*,#50241,.F.) ;
#70371=ORIENTED_EDGE('',*,*,#49882,.T.) ;
#70372=ORIENTED_EDGE('',*,*,#50238,.T.) ;
#70373=ORIENTED_EDGE('',*,*,#50242,.F.) ;
#70374=ORIENTED_EDGE('',*,*,#50243,.F.) ;
#70375=ORIENTED_EDGE('',*,*,#50240,.T.) ;
#70376=ORIENTED_EDGE('',*,*,#49879,.F.) ;
#70377=ORIENTED_EDGE('',*,*,#50244,.F.) ;
#70378=ORIENTED_EDGE('',*,*,#49957,.F.) ;
#70379=ORIENTED_EDGE('',*,*,#50241,.T.) ;
#70380=ORIENTED_EDGE('',*,*,#49956,.F.) ;
#70381=ORIENTED_EDGE('',*,*,#50245,.F.) ;
#70382=ORIENTED_EDGE('',*,*,#49958,.F.) ;
#70383=ORIENTED_EDGE('',*,*,#50246,.F.) ;
#70384=ORIENTED_EDGE('',*,*,#49959,.F.) ;
#70385=ORIENTED_EDGE('',*,*,#50247,.F.) ;
#70386=ORIENTED_EDGE('',*,*,#49965,.F.) ;
#70387=ORIENTED_EDGE('',*,*,#50242,.T.) ;
#70388=ORIENTED_EDGE('',*,*,#49960,.F.) ;
#70389=ORIENTED_EDGE('',*,*,#50248,.F.) ;
#70390=ORIENTED_EDGE('',*,*,#49949,.F.) ;
#70391=ORIENTED_EDGE('',*,*,#50243,.T.) ;
#70392=ORIENTED_EDGE('',*,*,#49948,.F.) ;
#70393=ORIENTED_EDGE('',*,*,#50249,.F.) ;
#70394=ORIENTED_EDGE('',*,*,#49883,.F.) ;
#70395=ORIENTED_EDGE('',*,*,#50250,.F.) ;
#70396=ORIENTED_EDGE('',*,*,#49877,.F.) ;
#70397=ORIENTED_EDGE('',*,*,#50251,.F.) ;
#70398=ORIENTED_EDGE('',*,*,#49952,.F.) ;
#70399=ORIENTED_EDGE('',*,*,#49878,.T.) ;
#70400=ORIENTED_EDGE('',*,*,#50250,.T.) ;
#70401=ORIENTED_EDGE('',*,*,#50252,.F.) ;
#70402=ORIENTED_EDGE('',*,*,#50244,.T.) ;
#70403=ORIENTED_EDGE('',*,*,#50247,.T.) ;
#70404=ORIENTED_EDGE('',*,*,#50245,.T.) ;
#70405=ORIENTED_EDGE('',*,*,#50253,.F.) ;
#70406=ORIENTED_EDGE('',*,*,#50248,.T.) ;
#70407=ORIENTED_EDGE('',*,*,#50246,.T.) ;
#70408=ORIENTED_EDGE('',*,*,#50254,.F.) ;
#70409=ORIENTED_EDGE('',*,*,#49876,.T.) ;
#70410=ORIENTED_EDGE('',*,*,#50249,.T.) ;
#70411=ORIENTED_EDGE('',*,*,#50255,.F.) ;
#70412=ORIENTED_EDGE('',*,*,#50251,.T.) ;
#70413=ORIENTED_EDGE('',*,*,#50252,.T.) ;
#70414=ORIENTED_EDGE('',*,*,#49951,.F.) ;
#70415=ORIENTED_EDGE('',*,*,#50256,.F.) ;
#70416=ORIENTED_EDGE('',*,*,#49954,.F.) ;
#70417=ORIENTED_EDGE('',*,*,#50253,.T.) ;
#70418=ORIENTED_EDGE('',*,*,#49955,.F.) ;
#70419=ORIENTED_EDGE('',*,*,#50257,.F.) ;
#70420=ORIENTED_EDGE('',*,*,#49962,.F.) ;
#70421=ORIENTED_EDGE('',*,*,#50254,.T.) ;
#70422=ORIENTED_EDGE('',*,*,#49964,.F.) ;
#70423=ORIENTED_EDGE('',*,*,#50258,.F.) ;
#70424=ORIENTED_EDGE('',*,*,#49946,.F.) ;
#70425=ORIENTED_EDGE('',*,*,#50255,.T.) ;
#70426=ORIENTED_EDGE('',*,*,#49947,.F.) ;
#70427=ORIENTED_EDGE('',*,*,#50259,.F.) ;
#70428=ORIENTED_EDGE('',*,*,#49953,.F.) ;
#70429=ORIENTED_EDGE('',*,*,#50257,.T.) ;
#70430=ORIENTED_EDGE('',*,*,#50256,.T.) ;
#70431=ORIENTED_EDGE('',*,*,#50260,.F.) ;
#70432=ORIENTED_EDGE('',*,*,#50259,.T.) ;
#70433=ORIENTED_EDGE('',*,*,#50258,.T.) ;
#70434=ORIENTED_EDGE('',*,*,#50261,.F.) ;
#70435=ORIENTED_EDGE('',*,*,#50260,.T.) ;
#70436=ORIENTED_EDGE('',*,*,#49950,.F.) ;
#70437=ORIENTED_EDGE('',*,*,#50261,.T.) ;
#70438=ORIENTED_EDGE('',*,*,#49963,.F.) ;
#70439=ORIENTED_EDGE('',*,*,#49971,.F.) ;
#70440=ORIENTED_EDGE('',*,*,#49985,.F.) ;
#70441=ORIENTED_EDGE('',*,*,#50262,.F.) ;
#70442=ORIENTED_EDGE('',*,*,#49974,.F.) ;
#70443=ORIENTED_EDGE('',*,*,#50263,.F.) ;
#70444=ORIENTED_EDGE('',*,*,#49975,.F.) ;
#70445=ORIENTED_EDGE('',*,*,#50264,.F.) ;
#70446=ORIENTED_EDGE('',*,*,#49989,.F.) ;
#70447=ORIENTED_EDGE('',*,*,#49973,.F.) ;
#70448=ORIENTED_EDGE('',*,*,#49976,.F.) ;
#70449=ORIENTED_EDGE('',*,*,#50265,.F.) ;
#70450=ORIENTED_EDGE('',*,*,#49977,.F.) ;
#70451=ORIENTED_EDGE('',*,*,#50264,.T.) ;
#70452=ORIENTED_EDGE('',*,*,#50262,.T.) ;
#70453=ORIENTED_EDGE('',*,*,#50266,.F.) ;
#70454=ORIENTED_EDGE('',*,*,#50265,.T.) ;
#70455=ORIENTED_EDGE('',*,*,#50263,.T.) ;
#70456=ORIENTED_EDGE('',*,*,#50267,.F.) ;
#70457=ORIENTED_EDGE('',*,*,#49969,.F.) ;
#70458=ORIENTED_EDGE('',*,*,#49981,.F.) ;
#70459=ORIENTED_EDGE('',*,*,#50268,.F.) ;
#70460=ORIENTED_EDGE('',*,*,#49983,.F.) ;
#70461=ORIENTED_EDGE('',*,*,#50266,.T.) ;
#70462=ORIENTED_EDGE('',*,*,#49984,.F.) ;
#70463=ORIENTED_EDGE('',*,*,#50269,.F.) ;
#70464=ORIENTED_EDGE('',*,*,#49986,.F.) ;
#70465=ORIENTED_EDGE('',*,*,#50267,.T.) ;
#70466=ORIENTED_EDGE('',*,*,#49988,.F.) ;
#70467=ORIENTED_EDGE('',*,*,#50270,.F.) ;
#70468=ORIENTED_EDGE('',*,*,#49978,.F.) ;
#70469=ORIENTED_EDGE('',*,*,#49967,.F.) ;
#70470=ORIENTED_EDGE('',*,*,#49979,.F.) ;
#70471=ORIENTED_EDGE('',*,*,#50271,.F.) ;
#70472=ORIENTED_EDGE('',*,*,#49982,.F.) ;
#70473=ORIENTED_EDGE('',*,*,#50269,.T.) ;
#70474=ORIENTED_EDGE('',*,*,#50268,.T.) ;
#70475=ORIENTED_EDGE('',*,*,#50272,.F.) ;
#70476=ORIENTED_EDGE('',*,*,#50271,.T.) ;
#70477=ORIENTED_EDGE('',*,*,#50270,.T.) ;
#70478=ORIENTED_EDGE('',*,*,#50273,.F.) ;
#70479=ORIENTED_EDGE('',*,*,#50272,.T.) ;
#70480=ORIENTED_EDGE('',*,*,#49980,.F.) ;
#70481=ORIENTED_EDGE('',*,*,#50273,.T.) ;
#70482=ORIENTED_EDGE('',*,*,#49987,.F.) ;
#70483=ORIENTED_EDGE('',*,*,#50274,.F.) ;
#70484=ORIENTED_EDGE('',*,*,#49921,.F.) ;
#70485=ORIENTED_EDGE('',*,*,#49927,.F.) ;
#70486=ORIENTED_EDGE('',*,*,#49942,.F.) ;
#70487=ORIENTED_EDGE('',*,*,#50275,.F.) ;
#70488=ORIENTED_EDGE('',*,*,#50274,.T.) ;
#70489=ORIENTED_EDGE('',*,*,#50276,.F.) ;
#70490=ORIENTED_EDGE('',*,*,#50276,.T.) ;
#70491=ORIENTED_EDGE('',*,*,#49941,.F.) ;
#70492=ORIENTED_EDGE('',*,*,#50277,.F.) ;
#70493=ORIENTED_EDGE('',*,*,#49916,.F.) ;
#70494=ORIENTED_EDGE('',*,*,#50275,.T.) ;
#70495=ORIENTED_EDGE('',*,*,#49915,.F.) ;
#70496=ORIENTED_EDGE('',*,*,#50278,.F.) ;
#70497=ORIENTED_EDGE('',*,*,#49918,.F.) ;
#70498=ORIENTED_EDGE('',*,*,#49928,.F.) ;
#70499=ORIENTED_EDGE('',*,*,#49919,.F.) ;
#70500=ORIENTED_EDGE('',*,*,#50279,.F.) ;
#70501=ORIENTED_EDGE('',*,*,#49938,.F.) ;
#70502=ORIENTED_EDGE('',*,*,#50280,.F.) ;
#70503=ORIENTED_EDGE('',*,*,#50277,.T.) ;
#70504=ORIENTED_EDGE('',*,*,#50281,.F.) ;
#70505=ORIENTED_EDGE('',*,*,#49792,.T.) ;
#70506=ORIENTED_EDGE('',*,*,#50279,.T.) ;
#70507=ORIENTED_EDGE('',*,*,#50278,.T.) ;
#70508=ORIENTED_EDGE('',*,*,#50282,.F.) ;
#70509=ORIENTED_EDGE('',*,*,#49925,.F.) ;
#70510=ORIENTED_EDGE('',*,*,#49931,.F.) ;
#70511=ORIENTED_EDGE('',*,*,#50283,.F.) ;
#70512=ORIENTED_EDGE('',*,*,#49943,.F.) ;
#70513=ORIENTED_EDGE('',*,*,#50284,.F.) ;
#70514=ORIENTED_EDGE('',*,*,#49944,.F.) ;
#70515=ORIENTED_EDGE('',*,*,#50285,.F.) ;
#70516=ORIENTED_EDGE('',*,*,#49935,.F.) ;
#70517=ORIENTED_EDGE('',*,*,#50281,.T.) ;
#70518=ORIENTED_EDGE('',*,*,#49945,.F.) ;
#70519=ORIENTED_EDGE('',*,*,#50286,.F.) ;
#70520=ORIENTED_EDGE('',*,*,#49793,.F.) ;
#70521=ORIENTED_EDGE('',*,*,#50280,.T.) ;
#70522=ORIENTED_EDGE('',*,*,#49791,.F.) ;
#70523=ORIENTED_EDGE('',*,*,#50287,.F.) ;
#70524=ORIENTED_EDGE('',*,*,#49917,.F.) ;
#70525=ORIENTED_EDGE('',*,*,#50282,.T.) ;
#70526=ORIENTED_EDGE('',*,*,#49914,.F.) ;
#70527=ORIENTED_EDGE('',*,*,#50288,.F.) ;
#70528=ORIENTED_EDGE('',*,*,#49939,.F.) ;
#70529=ORIENTED_EDGE('',*,*,#50285,.T.) ;
#70530=ORIENTED_EDGE('',*,*,#50283,.T.) ;
#70531=ORIENTED_EDGE('',*,*,#50289,.F.) ;
#70532=ORIENTED_EDGE('',*,*,#50286,.T.) ;
#70533=ORIENTED_EDGE('',*,*,#50284,.T.) ;
#70534=ORIENTED_EDGE('',*,*,#50290,.F.) ;
#70535=ORIENTED_EDGE('',*,*,#49794,.T.) ;
#70536=ORIENTED_EDGE('',*,*,#50287,.T.) ;
#70537=ORIENTED_EDGE('',*,*,#49790,.T.) ;
#70538=ORIENTED_EDGE('',*,*,#50291,.F.) ;
#70539=ORIENTED_EDGE('',*,*,#50288,.T.) ;
#70540=ORIENTED_EDGE('',*,*,#49923,.F.) ;
#70541=ORIENTED_EDGE('',*,*,#49937,.F.) ;
#70542=ORIENTED_EDGE('',*,*,#50292,.F.) ;
#70543=ORIENTED_EDGE('',*,*,#49929,.F.) ;
#70544=ORIENTED_EDGE('',*,*,#50289,.T.) ;
#70545=ORIENTED_EDGE('',*,*,#49930,.F.) ;
#70546=ORIENTED_EDGE('',*,*,#50293,.F.) ;
#70547=ORIENTED_EDGE('',*,*,#49932,.F.) ;
#70548=ORIENTED_EDGE('',*,*,#50290,.T.) ;
#70549=ORIENTED_EDGE('',*,*,#49934,.F.) ;
#70550=ORIENTED_EDGE('',*,*,#50294,.F.) ;
#70551=ORIENTED_EDGE('',*,*,#49795,.F.) ;
#70552=ORIENTED_EDGE('',*,*,#50291,.T.) ;
#70553=ORIENTED_EDGE('',*,*,#49789,.F.) ;
#70554=ORIENTED_EDGE('',*,*,#50295,.F.) ;
#70555=ORIENTED_EDGE('',*,*,#49940,.F.) ;
#70556=ORIENTED_EDGE('',*,*,#50293,.T.) ;
#70557=ORIENTED_EDGE('',*,*,#50292,.T.) ;
#70558=ORIENTED_EDGE('',*,*,#50296,.F.) ;
#70559=ORIENTED_EDGE('',*,*,#49788,.T.) ;
#70560=ORIENTED_EDGE('',*,*,#50294,.T.) ;
#70561=ORIENTED_EDGE('',*,*,#50297,.F.) ;
#70562=ORIENTED_EDGE('',*,*,#50295,.T.) ;
#70563=ORIENTED_EDGE('',*,*,#50296,.T.) ;
#70564=ORIENTED_EDGE('',*,*,#49936,.F.) ;
#70565=ORIENTED_EDGE('',*,*,#50297,.T.) ;
#70566=ORIENTED_EDGE('',*,*,#49933,.F.) ;
#70567=ORIENTED_EDGE('',*,*,#50298,.F.) ;
#70568=ORIENTED_EDGE('',*,*,#49372,.F.) ;
#70569=ORIENTED_EDGE('',*,*,#50299,.F.) ;
#70570=ORIENTED_EDGE('',*,*,#50061,.F.) ;
#70571=ORIENTED_EDGE('',*,*,#50299,.T.) ;
#70572=ORIENTED_EDGE('',*,*,#49371,.T.) ;
#70573=ORIENTED_EDGE('',*,*,#50300,.F.) ;
#70574=ORIENTED_EDGE('',*,*,#50301,.F.) ;
#70575=ORIENTED_EDGE('',*,*,#49373,.T.) ;
#70576=ORIENTED_EDGE('',*,*,#50298,.T.) ;
#70577=ORIENTED_EDGE('',*,*,#50302,.F.) ;
#70578=ORIENTED_EDGE('',*,*,#50303,.F.) ;
#70579=ORIENTED_EDGE('',*,*,#50300,.T.) ;
#70580=ORIENTED_EDGE('',*,*,#49370,.F.) ;
#70581=ORIENTED_EDGE('',*,*,#50304,.F.) ;
#70582=ORIENTED_EDGE('',*,*,#50058,.F.) ;
#70583=ORIENTED_EDGE('',*,*,#50301,.T.) ;
#70584=ORIENTED_EDGE('',*,*,#50057,.F.) ;
#70585=ORIENTED_EDGE('',*,*,#50305,.F.) ;
#70586=ORIENTED_EDGE('',*,*,#50062,.F.) ;
#70587=ORIENTED_EDGE('',*,*,#50306,.F.) ;
#70588=ORIENTED_EDGE('',*,*,#50059,.F.) ;
#70589=ORIENTED_EDGE('',*,*,#50307,.F.) ;
#70590=ORIENTED_EDGE('',*,*,#50066,.F.) ;
#70591=ORIENTED_EDGE('',*,*,#50302,.T.) ;
#70592=ORIENTED_EDGE('',*,*,#50060,.F.) ;
#70593=ORIENTED_EDGE('',*,*,#50308,.F.) ;
#70594=ORIENTED_EDGE('',*,*,#50050,.F.) ;
#70595=ORIENTED_EDGE('',*,*,#50303,.T.) ;
#70596=ORIENTED_EDGE('',*,*,#50049,.F.) ;
#70597=ORIENTED_EDGE('',*,*,#50309,.F.) ;
#70598=ORIENTED_EDGE('',*,*,#49374,.F.) ;
#70599=ORIENTED_EDGE('',*,*,#50310,.F.) ;
#70600=ORIENTED_EDGE('',*,*,#49368,.F.) ;
#70601=ORIENTED_EDGE('',*,*,#50311,.F.) ;
#70602=ORIENTED_EDGE('',*,*,#50051,.F.) ;
#70603=ORIENTED_EDGE('',*,*,#49369,.T.) ;
#70604=ORIENTED_EDGE('',*,*,#50310,.T.) ;
#70605=ORIENTED_EDGE('',*,*,#50312,.F.) ;
#70606=ORIENTED_EDGE('',*,*,#50304,.T.) ;
#70607=ORIENTED_EDGE('',*,*,#50307,.T.) ;
#70608=ORIENTED_EDGE('',*,*,#50305,.T.) ;
#70609=ORIENTED_EDGE('',*,*,#50313,.F.) ;
#70610=ORIENTED_EDGE('',*,*,#50308,.T.) ;
#70611=ORIENTED_EDGE('',*,*,#50306,.T.) ;
#70612=ORIENTED_EDGE('',*,*,#50314,.F.) ;
#70613=ORIENTED_EDGE('',*,*,#49367,.T.) ;
#70614=ORIENTED_EDGE('',*,*,#50309,.T.) ;
#70615=ORIENTED_EDGE('',*,*,#50315,.F.) ;
#70616=ORIENTED_EDGE('',*,*,#50311,.T.) ;
#70617=ORIENTED_EDGE('',*,*,#50312,.T.) ;
#70618=ORIENTED_EDGE('',*,*,#50054,.F.) ;
#70619=ORIENTED_EDGE('',*,*,#50316,.F.) ;
#70620=ORIENTED_EDGE('',*,*,#50055,.F.) ;
#70621=ORIENTED_EDGE('',*,*,#50313,.T.) ;
#70622=ORIENTED_EDGE('',*,*,#50056,.F.) ;
#70623=ORIENTED_EDGE('',*,*,#50317,.F.) ;
#70624=ORIENTED_EDGE('',*,*,#50063,.F.) ;
#70625=ORIENTED_EDGE('',*,*,#50314,.T.) ;
#70626=ORIENTED_EDGE('',*,*,#50065,.F.) ;
#70627=ORIENTED_EDGE('',*,*,#50318,.F.) ;
#70628=ORIENTED_EDGE('',*,*,#50047,.F.) ;
#70629=ORIENTED_EDGE('',*,*,#50315,.T.) ;
#70630=ORIENTED_EDGE('',*,*,#50048,.F.) ;
#70631=ORIENTED_EDGE('',*,*,#50319,.F.) ;
#70632=ORIENTED_EDGE('',*,*,#50052,.F.) ;
#70633=ORIENTED_EDGE('',*,*,#50317,.T.) ;
#70634=ORIENTED_EDGE('',*,*,#50316,.T.) ;
#70635=ORIENTED_EDGE('',*,*,#50320,.F.) ;
#70636=ORIENTED_EDGE('',*,*,#50319,.T.) ;
#70637=ORIENTED_EDGE('',*,*,#50318,.T.) ;
#70638=ORIENTED_EDGE('',*,*,#50321,.F.) ;
#70639=ORIENTED_EDGE('',*,*,#50320,.T.) ;
#70640=ORIENTED_EDGE('',*,*,#50053,.F.) ;
#70641=ORIENTED_EDGE('',*,*,#50321,.T.) ;
#70642=ORIENTED_EDGE('',*,*,#50064,.F.) ;
#70643=ORIENTED_EDGE('',*,*,#50072,.F.) ;
#70644=ORIENTED_EDGE('',*,*,#50085,.F.) ;
#70645=ORIENTED_EDGE('',*,*,#50322,.F.) ;
#70646=ORIENTED_EDGE('',*,*,#50077,.F.) ;
#70647=ORIENTED_EDGE('',*,*,#50323,.F.) ;
#70648=ORIENTED_EDGE('',*,*,#50075,.F.) ;
#70649=ORIENTED_EDGE('',*,*,#50324,.F.) ;
#70650=ORIENTED_EDGE('',*,*,#50090,.F.) ;
#70651=ORIENTED_EDGE('',*,*,#50074,.F.) ;
#70652=ORIENTED_EDGE('',*,*,#50076,.F.) ;
#70653=ORIENTED_EDGE('',*,*,#50325,.F.) ;
#70654=ORIENTED_EDGE('',*,*,#50080,.F.) ;
#70655=ORIENTED_EDGE('',*,*,#50324,.T.) ;
#70656=ORIENTED_EDGE('',*,*,#50322,.T.) ;
#70657=ORIENTED_EDGE('',*,*,#50326,.F.) ;
#70658=ORIENTED_EDGE('',*,*,#50325,.T.) ;
#70659=ORIENTED_EDGE('',*,*,#50323,.T.) ;
#70660=ORIENTED_EDGE('',*,*,#50327,.F.) ;
#70661=ORIENTED_EDGE('',*,*,#50070,.F.) ;
#70662=ORIENTED_EDGE('',*,*,#50083,.F.) ;
#70663=ORIENTED_EDGE('',*,*,#50328,.F.) ;
#70664=ORIENTED_EDGE('',*,*,#50086,.F.) ;
#70665=ORIENTED_EDGE('',*,*,#50326,.T.) ;
#70666=ORIENTED_EDGE('',*,*,#50084,.F.) ;
#70667=ORIENTED_EDGE('',*,*,#50329,.F.) ;
#70668=ORIENTED_EDGE('',*,*,#50087,.F.) ;
#70669=ORIENTED_EDGE('',*,*,#50327,.T.) ;
#70670=ORIENTED_EDGE('',*,*,#50089,.F.) ;
#70671=ORIENTED_EDGE('',*,*,#50330,.F.) ;
#70672=ORIENTED_EDGE('',*,*,#50078,.F.) ;
#70673=ORIENTED_EDGE('',*,*,#50068,.F.) ;
#70674=ORIENTED_EDGE('',*,*,#50079,.F.) ;
#70675=ORIENTED_EDGE('',*,*,#50331,.F.) ;
#70676=ORIENTED_EDGE('',*,*,#50081,.F.) ;
#70677=ORIENTED_EDGE('',*,*,#50329,.T.) ;
#70678=ORIENTED_EDGE('',*,*,#50328,.T.) ;
#70679=ORIENTED_EDGE('',*,*,#50332,.F.) ;
#70680=ORIENTED_EDGE('',*,*,#50331,.T.) ;
#70681=ORIENTED_EDGE('',*,*,#50330,.T.) ;
#70682=ORIENTED_EDGE('',*,*,#50333,.F.) ;
#70683=ORIENTED_EDGE('',*,*,#50332,.T.) ;
#70684=ORIENTED_EDGE('',*,*,#50082,.F.) ;
#70685=ORIENTED_EDGE('',*,*,#50333,.T.) ;
#70686=ORIENTED_EDGE('',*,*,#50088,.F.) ;
#70687=ORIENTED_EDGE('',*,*,#50334,.F.) ;
#70688=ORIENTED_EDGE('',*,*,#50120,.F.) ;
#70689=ORIENTED_EDGE('',*,*,#50335,.F.) ;
#70690=ORIENTED_EDGE('',*,*,#50135,.F.) ;
#70691=ORIENTED_EDGE('',*,*,#50335,.T.) ;
#70692=ORIENTED_EDGE('',*,*,#50123,.F.) ;
#70693=ORIENTED_EDGE('',*,*,#50336,.F.) ;
#70694=ORIENTED_EDGE('',*,*,#50117,.F.) ;
#70695=ORIENTED_EDGE('',*,*,#50334,.T.) ;
#70696=ORIENTED_EDGE('',*,*,#50337,.F.) ;
#70697=ORIENTED_EDGE('',*,*,#50336,.T.) ;
#70698=ORIENTED_EDGE('',*,*,#50126,.F.) ;
#70699=ORIENTED_EDGE('',*,*,#50338,.F.) ;
#70700=ORIENTED_EDGE('',*,*,#50132,.F.) ;
#70701=ORIENTED_EDGE('',*,*,#50337,.T.) ;
#70702=ORIENTED_EDGE('',*,*,#50134,.F.) ;
#70703=ORIENTED_EDGE('',*,*,#50339,.F.) ;
#70704=ORIENTED_EDGE('',*,*,#50114,.F.) ;
#70705=ORIENTED_EDGE('',*,*,#50338,.T.) ;
#70706=ORIENTED_EDGE('',*,*,#50129,.F.) ;
#70707=ORIENTED_EDGE('',*,*,#50340,.F.) ;
#70708=ORIENTED_EDGE('',*,*,#50111,.F.) ;
#70709=ORIENTED_EDGE('',*,*,#50339,.T.) ;
#70710=ORIENTED_EDGE('',*,*,#50341,.F.) ;
#70711=ORIENTED_EDGE('',*,*,#50340,.T.) ;
#70712=ORIENTED_EDGE('',*,*,#50130,.F.) ;
#70713=ORIENTED_EDGE('',*,*,#50341,.T.) ;
#70714=ORIENTED_EDGE('',*,*,#50133,.F.) ;
#70715=ORIENTED_EDGE('',*,*,#49298,.F.) ;
#70716=ORIENTED_EDGE('',*,*,#50091,.F.) ;
#70717=ORIENTED_EDGE('',*,*,#49312,.F.) ;
#70718=ORIENTED_EDGE('',*,*,#50092,.F.) ;
#70719=ORIENTED_EDGE('',*,*,#49300,.F.) ;
#70720=ORIENTED_EDGE('',*,*,#50093,.F.) ;
#70721=ORIENTED_EDGE('',*,*,#49310,.F.) ;
#70722=ORIENTED_EDGE('',*,*,#50096,.F.) ;
#70723=ORIENTED_EDGE('',*,*,#49308,.F.) ;
#70724=ORIENTED_EDGE('',*,*,#50094,.F.) ;
#70725=ORIENTED_EDGE('',*,*,#49302,.F.) ;
#70726=ORIENTED_EDGE('',*,*,#50097,.F.) ;
#70727=ORIENTED_EDGE('',*,*,#49306,.F.) ;
#70728=ORIENTED_EDGE('',*,*,#49812,.F.) ;
#70729=ORIENTED_EDGE('',*,*,#49304,.F.) ;
#70730=ORIENTED_EDGE('',*,*,#50095,.F.) ;
#70731=ORIENTED_EDGE('',*,*,#49798,.F.) ;
#70732=ORIENTED_EDGE('',*,*,#50342,.T.) ;
#70733=ORIENTED_EDGE('',*,*,#49539,.F.) ;
#70734=ORIENTED_EDGE('',*,*,#50343,.T.) ;
#70735=ORIENTED_EDGE('',*,*,#49541,.F.) ;
#70736=ORIENTED_EDGE('',*,*,#50344,.T.) ;
#70737=ORIENTED_EDGE('',*,*,#49742,.T.) ;
#70738=ORIENTED_EDGE('',*,*,#49536,.F.) ;
#70739=ORIENTED_EDGE('',*,*,#50345,.T.) ;
#70740=ORIENTED_EDGE('',*,*,#49998,.F.) ;
#70741=ORIENTED_EDGE('',*,*,#50346,.F.) ;
#70742=ORIENTED_EDGE('',*,*,#50347,.F.) ;
#70743=ORIENTED_EDGE('',*,*,#50347,.T.) ;
#70744=ORIENTED_EDGE('',*,*,#50348,.T.) ;
#70745=ORIENTED_EDGE('',*,*,#49537,.F.) ;
#70746=ORIENTED_EDGE('',*,*,#50018,.F.) ;
#70747=ORIENTED_EDGE('',*,*,#50349,.T.) ;
#70748=ORIENTED_EDGE('',*,*,#50350,.F.) ;
#70749=ORIENTED_EDGE('',*,*,#50350,.T.) ;
#70750=ORIENTED_EDGE('',*,*,#50351,.T.) ;
#70751=ORIENTED_EDGE('',*,*,#49797,.F.) ;
#70752=ORIENTED_EDGE('',*,*,#50352,.F.) ;
#70753=ORIENTED_EDGE('',*,*,#50019,.F.) ;
#70754=ORIENTED_EDGE('',*,*,#50188,.F.) ;
#70755=ORIENTED_EDGE('',*,*,#50186,.F.) ;
#70756=ORIENTED_EDGE('',*,*,#50352,.T.) ;
#70757=ORIENTED_EDGE('',*,*,#50353,.F.) ;
#70758=ORIENTED_EDGE('',*,*,#50354,.T.) ;
#70759=ORIENTED_EDGE('',*,*,#50002,.F.) ;
#70760=ORIENTED_EDGE('',*,*,#50355,.T.) ;
#70761=ORIENTED_EDGE('',*,*,#50353,.T.) ;
#70762=ORIENTED_EDGE('',*,*,#50011,.F.) ;
#70763=ORIENTED_EDGE('',*,*,#50356,.F.) ;
#70764=ORIENTED_EDGE('',*,*,#49799,.F.) ;
#70765=ORIENTED_EDGE('',*,*,#50195,.F.) ;
#70766=ORIENTED_EDGE('',*,*,#50189,.F.) ;
#70767=ORIENTED_EDGE('',*,*,#50356,.T.) ;
#70768=ORIENTED_EDGE('',*,*,#50342,.F.) ;
#70769=ORIENTED_EDGE('',*,*,#50351,.F.) ;
#70770=ORIENTED_EDGE('',*,*,#50357,.F.) ;
#70771=ORIENTED_EDGE('',*,*,#49540,.F.) ;
#70772=ORIENTED_EDGE('',*,*,#50357,.T.) ;
#70773=ORIENTED_EDGE('',*,*,#50349,.F.) ;
#70774=ORIENTED_EDGE('',*,*,#50358,.F.) ;
#70775=ORIENTED_EDGE('',*,*,#50344,.F.) ;
#70776=ORIENTED_EDGE('',*,*,#50208,.F.) ;
#70777=ORIENTED_EDGE('',*,*,#49743,.T.) ;
#70778=ORIENTED_EDGE('',*,*,#50358,.T.) ;
#70779=ORIENTED_EDGE('',*,*,#50017,.F.) ;
#70780=ORIENTED_EDGE('',*,*,#50343,.F.) ;
#70781=ORIENTED_EDGE('',*,*,#49538,.F.) ;
#70782=ORIENTED_EDGE('',*,*,#50359,.F.) ;
#70783=ORIENTED_EDGE('',*,*,#50355,.F.) ;
#70784=ORIENTED_EDGE('',*,*,#50359,.T.) ;
#70785=ORIENTED_EDGE('',*,*,#50348,.F.) ;
#70786=ORIENTED_EDGE('',*,*,#50360,.F.) ;
#70787=ORIENTED_EDGE('',*,*,#50354,.F.) ;
#70788=ORIENTED_EDGE('',*,*,#50360,.T.) ;
#70789=ORIENTED_EDGE('',*,*,#50346,.T.) ;
#70790=ORIENTED_EDGE('',*,*,#50224,.F.) ;
#70791=ORIENTED_EDGE('',*,*,#50003,.F.) ;
#70792=ORIENTED_EDGE('',*,*,#50361,.T.) ;
#70793=ORIENTED_EDGE('',*,*,#50362,.T.) ;
#70794=ORIENTED_EDGE('',*,*,#50363,.T.) ;
#70795=ORIENTED_EDGE('',*,*,#50364,.T.) ;
#70796=ORIENTED_EDGE('',*,*,#50365,.T.) ;
#70797=ORIENTED_EDGE('',*,*,#50366,.T.) ;
#70798=ORIENTED_EDGE('',*,*,#50367,.T.) ;
#70799=ORIENTED_EDGE('',*,*,#50368,.T.) ;
#70800=ORIENTED_EDGE('',*,*,#50369,.F.) ;
#70801=ORIENTED_EDGE('',*,*,#50370,.T.) ;
#70802=ORIENTED_EDGE('',*,*,#50371,.T.) ;
#70803=ORIENTED_EDGE('',*,*,#50372,.T.) ;
#70804=ORIENTED_EDGE('',*,*,#50373,.T.) ;
#70805=ORIENTED_EDGE('',*,*,#50374,.T.) ;
#70806=ORIENTED_EDGE('',*,*,#50367,.F.) ;
#70807=ORIENTED_EDGE('',*,*,#50375,.T.) ;
#70808=ORIENTED_EDGE('',*,*,#50371,.F.) ;
#70809=ORIENTED_EDGE('',*,*,#50376,.T.) ;
#70810=ORIENTED_EDGE('',*,*,#50377,.T.) ;
#70811=ORIENTED_EDGE('',*,*,#50378,.T.) ;
#70812=ORIENTED_EDGE('',*,*,#50379,.T.) ;
#70813=ORIENTED_EDGE('',*,*,#50380,.T.) ;
#70814=ORIENTED_EDGE('',*,*,#50381,.T.) ;
#70815=ORIENTED_EDGE('',*,*,#50382,.T.) ;
#70816=ORIENTED_EDGE('',*,*,#50383,.T.) ;
#70817=ORIENTED_EDGE('',*,*,#50384,.T.) ;
#70818=ORIENTED_EDGE('',*,*,#50385,.T.) ;
#70819=ORIENTED_EDGE('',*,*,#50386,.T.) ;
#70820=ORIENTED_EDGE('',*,*,#50387,.T.) ;
#70821=ORIENTED_EDGE('',*,*,#50388,.T.) ;
#70822=ORIENTED_EDGE('',*,*,#50389,.T.) ;
#70823=ORIENTED_EDGE('',*,*,#50390,.T.) ;
#70824=ORIENTED_EDGE('',*,*,#50391,.F.) ;
#70825=ORIENTED_EDGE('',*,*,#50392,.T.) ;
#70826=ORIENTED_EDGE('',*,*,#50393,.T.) ;
#70827=ORIENTED_EDGE('',*,*,#50394,.T.) ;
#70828=ORIENTED_EDGE('',*,*,#50395,.T.) ;
#70829=ORIENTED_EDGE('',*,*,#50396,.T.) ;
#70830=ORIENTED_EDGE('',*,*,#50389,.F.) ;
#70831=ORIENTED_EDGE('',*,*,#50397,.T.) ;
#70832=ORIENTED_EDGE('',*,*,#50393,.F.) ;
#70833=ORIENTED_EDGE('',*,*,#50398,.T.) ;
#70834=ORIENTED_EDGE('',*,*,#50399,.T.) ;
#70835=ORIENTED_EDGE('',*,*,#50400,.T.) ;
#70836=ORIENTED_EDGE('',*,*,#50401,.T.) ;
#70837=ORIENTED_EDGE('',*,*,#50402,.T.) ;
#70838=ORIENTED_EDGE('',*,*,#50403,.T.) ;
#70839=ORIENTED_EDGE('',*,*,#50404,.T.) ;
#70840=ORIENTED_EDGE('',*,*,#50405,.T.) ;
#70841=ORIENTED_EDGE('',*,*,#50406,.T.) ;
#70842=ORIENTED_EDGE('',*,*,#50407,.T.) ;
#70843=ORIENTED_EDGE('',*,*,#50408,.T.) ;
#70844=ORIENTED_EDGE('',*,*,#50409,.T.) ;
#70845=ORIENTED_EDGE('',*,*,#50410,.T.) ;
#70846=ORIENTED_EDGE('',*,*,#50411,.T.) ;
#70847=ORIENTED_EDGE('',*,*,#50412,.T.) ;
#70848=ORIENTED_EDGE('',*,*,#50413,.F.) ;
#70849=ORIENTED_EDGE('',*,*,#50414,.T.) ;
#70850=ORIENTED_EDGE('',*,*,#50415,.T.) ;
#70851=ORIENTED_EDGE('',*,*,#50416,.T.) ;
#70852=ORIENTED_EDGE('',*,*,#50417,.T.) ;
#70853=ORIENTED_EDGE('',*,*,#50418,.T.) ;
#70854=ORIENTED_EDGE('',*,*,#50411,.F.) ;
#70855=ORIENTED_EDGE('',*,*,#50419,.T.) ;
#70856=ORIENTED_EDGE('',*,*,#50415,.F.) ;
#70857=ORIENTED_EDGE('',*,*,#50420,.T.) ;
#70858=ORIENTED_EDGE('',*,*,#50421,.T.) ;
#70859=ORIENTED_EDGE('',*,*,#50422,.T.) ;
#70860=ORIENTED_EDGE('',*,*,#50423,.T.) ;
#70861=ORIENTED_EDGE('',*,*,#50424,.T.) ;
#70862=ORIENTED_EDGE('',*,*,#50425,.T.) ;
#70863=ORIENTED_EDGE('',*,*,#50426,.T.) ;
#70864=ORIENTED_EDGE('',*,*,#50427,.T.) ;
#70865=ORIENTED_EDGE('',*,*,#50428,.T.) ;
#70866=ORIENTED_EDGE('',*,*,#50429,.T.) ;
#70867=ORIENTED_EDGE('',*,*,#50430,.T.) ;
#70868=ORIENTED_EDGE('',*,*,#50431,.T.) ;
#70869=ORIENTED_EDGE('',*,*,#50432,.T.) ;
#70870=ORIENTED_EDGE('',*,*,#50433,.T.) ;
#70871=ORIENTED_EDGE('',*,*,#50434,.T.) ;
#70872=ORIENTED_EDGE('',*,*,#50435,.F.) ;
#70873=ORIENTED_EDGE('',*,*,#50436,.T.) ;
#70874=ORIENTED_EDGE('',*,*,#50437,.T.) ;
#70875=ORIENTED_EDGE('',*,*,#50438,.T.) ;
#70876=ORIENTED_EDGE('',*,*,#50439,.T.) ;
#70877=ORIENTED_EDGE('',*,*,#50440,.T.) ;
#70878=ORIENTED_EDGE('',*,*,#50433,.F.) ;
#70879=ORIENTED_EDGE('',*,*,#50441,.T.) ;
#70880=ORIENTED_EDGE('',*,*,#50437,.F.) ;
#70881=ORIENTED_EDGE('',*,*,#50442,.T.) ;
#70882=ORIENTED_EDGE('',*,*,#50443,.T.) ;
#70883=ORIENTED_EDGE('',*,*,#50444,.T.) ;
#70884=ORIENTED_EDGE('',*,*,#50445,.T.) ;
#70885=ORIENTED_EDGE('',*,*,#50446,.T.) ;
#70886=ORIENTED_EDGE('',*,*,#50447,.T.) ;
#70887=ORIENTED_EDGE('',*,*,#50448,.T.) ;
#70888=ORIENTED_EDGE('',*,*,#50449,.T.) ;
#70889=ORIENTED_EDGE('',*,*,#50450,.T.) ;
#70890=ORIENTED_EDGE('',*,*,#50451,.T.) ;
#70891=ORIENTED_EDGE('',*,*,#50452,.T.) ;
#70892=ORIENTED_EDGE('',*,*,#50453,.T.) ;
#70893=ORIENTED_EDGE('',*,*,#50454,.T.) ;
#70894=ORIENTED_EDGE('',*,*,#50455,.T.) ;
#70895=ORIENTED_EDGE('',*,*,#50456,.T.) ;
#70896=ORIENTED_EDGE('',*,*,#50457,.F.) ;
#70897=ORIENTED_EDGE('',*,*,#50458,.T.) ;
#70898=ORIENTED_EDGE('',*,*,#50459,.T.) ;
#70899=ORIENTED_EDGE('',*,*,#50460,.T.) ;
#70900=ORIENTED_EDGE('',*,*,#50461,.T.) ;
#70901=ORIENTED_EDGE('',*,*,#50462,.T.) ;
#70902=ORIENTED_EDGE('',*,*,#50455,.F.) ;
#70903=ORIENTED_EDGE('',*,*,#50463,.T.) ;
#70904=ORIENTED_EDGE('',*,*,#50459,.F.) ;
#70905=ORIENTED_EDGE('',*,*,#50464,.T.) ;
#70906=ORIENTED_EDGE('',*,*,#50465,.T.) ;
#70907=ORIENTED_EDGE('',*,*,#50466,.T.) ;
#70908=ORIENTED_EDGE('',*,*,#50467,.T.) ;
#70909=ORIENTED_EDGE('',*,*,#50468,.T.) ;
#70910=ORIENTED_EDGE('',*,*,#50469,.T.) ;
#70911=ORIENTED_EDGE('',*,*,#50470,.T.) ;
#70912=ORIENTED_EDGE('',*,*,#50471,.T.) ;
#70913=ORIENTED_EDGE('',*,*,#50472,.T.) ;
#70914=ORIENTED_EDGE('',*,*,#50473,.T.) ;
#70915=ORIENTED_EDGE('',*,*,#50474,.T.) ;
#70916=ORIENTED_EDGE('',*,*,#50475,.T.) ;
#70917=ORIENTED_EDGE('',*,*,#50476,.T.) ;
#70918=ORIENTED_EDGE('',*,*,#50477,.T.) ;
#70919=ORIENTED_EDGE('',*,*,#50478,.T.) ;
#70920=ORIENTED_EDGE('',*,*,#50479,.F.) ;
#70921=ORIENTED_EDGE('',*,*,#50480,.T.) ;
#70922=ORIENTED_EDGE('',*,*,#50481,.T.) ;
#70923=ORIENTED_EDGE('',*,*,#50482,.T.) ;
#70924=ORIENTED_EDGE('',*,*,#50483,.T.) ;
#70925=ORIENTED_EDGE('',*,*,#50484,.T.) ;
#70926=ORIENTED_EDGE('',*,*,#50477,.F.) ;
#70927=ORIENTED_EDGE('',*,*,#50485,.T.) ;
#70928=ORIENTED_EDGE('',*,*,#50481,.F.) ;
#70929=ORIENTED_EDGE('',*,*,#50486,.T.) ;
#70930=ORIENTED_EDGE('',*,*,#50487,.T.) ;
#70931=ORIENTED_EDGE('',*,*,#50488,.T.) ;
#70932=ORIENTED_EDGE('',*,*,#50489,.T.) ;
#70933=ORIENTED_EDGE('',*,*,#50490,.T.) ;
#70934=ORIENTED_EDGE('',*,*,#50491,.T.) ;
#70935=ORIENTED_EDGE('',*,*,#50492,.T.) ;
#70936=ORIENTED_EDGE('',*,*,#50493,.T.) ;
#70937=ORIENTED_EDGE('',*,*,#50494,.T.) ;
#70938=ORIENTED_EDGE('',*,*,#50495,.T.) ;
#70939=ORIENTED_EDGE('',*,*,#50496,.T.) ;
#70940=ORIENTED_EDGE('',*,*,#50497,.T.) ;
#70941=ORIENTED_EDGE('',*,*,#50498,.T.) ;
#70942=ORIENTED_EDGE('',*,*,#50499,.T.) ;
#70943=ORIENTED_EDGE('',*,*,#50500,.T.) ;
#70944=ORIENTED_EDGE('',*,*,#50501,.F.) ;
#70945=ORIENTED_EDGE('',*,*,#50502,.T.) ;
#70946=ORIENTED_EDGE('',*,*,#50503,.T.) ;
#70947=ORIENTED_EDGE('',*,*,#50504,.T.) ;
#70948=ORIENTED_EDGE('',*,*,#50505,.T.) ;
#70949=ORIENTED_EDGE('',*,*,#50506,.T.) ;
#70950=ORIENTED_EDGE('',*,*,#50499,.F.) ;
#70951=ORIENTED_EDGE('',*,*,#50507,.T.) ;
#70952=ORIENTED_EDGE('',*,*,#50503,.F.) ;
#70953=ORIENTED_EDGE('',*,*,#50508,.T.) ;
#70954=ORIENTED_EDGE('',*,*,#50509,.T.) ;
#70955=ORIENTED_EDGE('',*,*,#50510,.T.) ;
#70956=ORIENTED_EDGE('',*,*,#50511,.T.) ;
#70957=ORIENTED_EDGE('',*,*,#50512,.T.) ;
#70958=ORIENTED_EDGE('',*,*,#50513,.T.) ;
#70959=ORIENTED_EDGE('',*,*,#50514,.T.) ;
#70960=ORIENTED_EDGE('',*,*,#50515,.T.) ;
#70961=ORIENTED_EDGE('',*,*,#50516,.T.) ;
#70962=ORIENTED_EDGE('',*,*,#50517,.T.) ;
#70963=ORIENTED_EDGE('',*,*,#50518,.T.) ;
#70964=ORIENTED_EDGE('',*,*,#50519,.T.) ;
#70965=ORIENTED_EDGE('',*,*,#50520,.T.) ;
#70966=ORIENTED_EDGE('',*,*,#50521,.T.) ;
#70967=ORIENTED_EDGE('',*,*,#50522,.T.) ;
#70968=ORIENTED_EDGE('',*,*,#50523,.F.) ;
#70969=ORIENTED_EDGE('',*,*,#50524,.T.) ;
#70970=ORIENTED_EDGE('',*,*,#50525,.T.) ;
#70971=ORIENTED_EDGE('',*,*,#50526,.T.) ;
#70972=ORIENTED_EDGE('',*,*,#50527,.T.) ;
#70973=ORIENTED_EDGE('',*,*,#50528,.T.) ;
#70974=ORIENTED_EDGE('',*,*,#50521,.F.) ;
#70975=ORIENTED_EDGE('',*,*,#50529,.T.) ;
#70976=ORIENTED_EDGE('',*,*,#50525,.F.) ;
#70977=ORIENTED_EDGE('',*,*,#50530,.T.) ;
#70978=ORIENTED_EDGE('',*,*,#50531,.T.) ;
#70979=ORIENTED_EDGE('',*,*,#50532,.T.) ;
#70980=ORIENTED_EDGE('',*,*,#50533,.T.) ;
#70981=ORIENTED_EDGE('',*,*,#50534,.T.) ;
#70982=ORIENTED_EDGE('',*,*,#50535,.T.) ;
#70983=ORIENTED_EDGE('',*,*,#50536,.T.) ;
#70984=ORIENTED_EDGE('',*,*,#50537,.T.) ;
#70985=ORIENTED_EDGE('',*,*,#50538,.T.) ;
#70986=ORIENTED_EDGE('',*,*,#50539,.T.) ;
#70987=ORIENTED_EDGE('',*,*,#50540,.T.) ;
#70988=ORIENTED_EDGE('',*,*,#50541,.T.) ;
#70989=ORIENTED_EDGE('',*,*,#50542,.T.) ;
#70990=ORIENTED_EDGE('',*,*,#50543,.T.) ;
#70991=ORIENTED_EDGE('',*,*,#50544,.T.) ;
#70992=ORIENTED_EDGE('',*,*,#50545,.F.) ;
#70993=ORIENTED_EDGE('',*,*,#50546,.T.) ;
#70994=ORIENTED_EDGE('',*,*,#50547,.T.) ;
#70995=ORIENTED_EDGE('',*,*,#50548,.T.) ;
#70996=ORIENTED_EDGE('',*,*,#50549,.T.) ;
#70997=ORIENTED_EDGE('',*,*,#50550,.T.) ;
#70998=ORIENTED_EDGE('',*,*,#50543,.F.) ;
#70999=ORIENTED_EDGE('',*,*,#50551,.T.) ;
#71000=ORIENTED_EDGE('',*,*,#50547,.F.) ;
#71001=ORIENTED_EDGE('',*,*,#50552,.T.) ;
#71002=ORIENTED_EDGE('',*,*,#50553,.T.) ;
#71003=ORIENTED_EDGE('',*,*,#50554,.T.) ;
#71004=ORIENTED_EDGE('',*,*,#50555,.T.) ;
#71005=ORIENTED_EDGE('',*,*,#50556,.T.) ;
#71006=ORIENTED_EDGE('',*,*,#50557,.T.) ;
#71007=ORIENTED_EDGE('',*,*,#50558,.T.) ;
#71008=ORIENTED_EDGE('',*,*,#50559,.T.) ;
#71009=ORIENTED_EDGE('',*,*,#50560,.T.) ;
#71010=ORIENTED_EDGE('',*,*,#50545,.T.) ;
#71011=ORIENTED_EDGE('',*,*,#50561,.T.) ;
#71012=ORIENTED_EDGE('',*,*,#50562,.T.) ;
#71013=ORIENTED_EDGE('',*,*,#50563,.T.) ;
#71014=ORIENTED_EDGE('',*,*,#50564,.T.) ;
#71015=ORIENTED_EDGE('',*,*,#50565,.T.) ;
#71016=ORIENTED_EDGE('',*,*,#50566,.T.) ;
#71017=ORIENTED_EDGE('',*,*,#50567,.T.) ;
#71018=ORIENTED_EDGE('',*,*,#50523,.T.) ;
#71019=ORIENTED_EDGE('',*,*,#50568,.T.) ;
#71020=ORIENTED_EDGE('',*,*,#50569,.T.) ;
#71021=ORIENTED_EDGE('',*,*,#50570,.T.) ;
#71022=ORIENTED_EDGE('',*,*,#50571,.T.) ;
#71023=ORIENTED_EDGE('',*,*,#50572,.T.) ;
#71024=ORIENTED_EDGE('',*,*,#50573,.T.) ;
#71025=ORIENTED_EDGE('',*,*,#50574,.T.) ;
#71026=ORIENTED_EDGE('',*,*,#50501,.T.) ;
#71027=ORIENTED_EDGE('',*,*,#50575,.T.) ;
#71028=ORIENTED_EDGE('',*,*,#50576,.T.) ;
#71029=ORIENTED_EDGE('',*,*,#50577,.T.) ;
#71030=ORIENTED_EDGE('',*,*,#50578,.T.) ;
#71031=ORIENTED_EDGE('',*,*,#50579,.T.) ;
#71032=ORIENTED_EDGE('',*,*,#50580,.T.) ;
#71033=ORIENTED_EDGE('',*,*,#50581,.T.) ;
#71034=ORIENTED_EDGE('',*,*,#50479,.T.) ;
#71035=ORIENTED_EDGE('',*,*,#50582,.T.) ;
#71036=ORIENTED_EDGE('',*,*,#50583,.T.) ;
#71037=ORIENTED_EDGE('',*,*,#50584,.T.) ;
#71038=ORIENTED_EDGE('',*,*,#50585,.T.) ;
#71039=ORIENTED_EDGE('',*,*,#50586,.T.) ;
#71040=ORIENTED_EDGE('',*,*,#50587,.T.) ;
#71041=ORIENTED_EDGE('',*,*,#50588,.T.) ;
#71042=ORIENTED_EDGE('',*,*,#50457,.T.) ;
#71043=ORIENTED_EDGE('',*,*,#50589,.T.) ;
#71044=ORIENTED_EDGE('',*,*,#50590,.T.) ;
#71045=ORIENTED_EDGE('',*,*,#50591,.T.) ;
#71046=ORIENTED_EDGE('',*,*,#50592,.T.) ;
#71047=ORIENTED_EDGE('',*,*,#50593,.T.) ;
#71048=ORIENTED_EDGE('',*,*,#50594,.T.) ;
#71049=ORIENTED_EDGE('',*,*,#50595,.T.) ;
#71050=ORIENTED_EDGE('',*,*,#50435,.T.) ;
#71051=ORIENTED_EDGE('',*,*,#50596,.T.) ;
#71052=ORIENTED_EDGE('',*,*,#50597,.T.) ;
#71053=ORIENTED_EDGE('',*,*,#50598,.T.) ;
#71054=ORIENTED_EDGE('',*,*,#50599,.T.) ;
#71055=ORIENTED_EDGE('',*,*,#50600,.T.) ;
#71056=ORIENTED_EDGE('',*,*,#50601,.T.) ;
#71057=ORIENTED_EDGE('',*,*,#50602,.T.) ;
#71058=ORIENTED_EDGE('',*,*,#50413,.T.) ;
#71059=ORIENTED_EDGE('',*,*,#50603,.T.) ;
#71060=ORIENTED_EDGE('',*,*,#50604,.T.) ;
#71061=ORIENTED_EDGE('',*,*,#50605,.T.) ;
#71062=ORIENTED_EDGE('',*,*,#50606,.T.) ;
#71063=ORIENTED_EDGE('',*,*,#50607,.T.) ;
#71064=ORIENTED_EDGE('',*,*,#50608,.T.) ;
#71065=ORIENTED_EDGE('',*,*,#50609,.T.) ;
#71066=ORIENTED_EDGE('',*,*,#50391,.T.) ;
#71067=ORIENTED_EDGE('',*,*,#50610,.T.) ;
#71068=ORIENTED_EDGE('',*,*,#50611,.T.) ;
#71069=ORIENTED_EDGE('',*,*,#50612,.T.) ;
#71070=ORIENTED_EDGE('',*,*,#50613,.T.) ;
#71071=ORIENTED_EDGE('',*,*,#50614,.T.) ;
#71072=ORIENTED_EDGE('',*,*,#50615,.T.) ;
#71073=ORIENTED_EDGE('',*,*,#50616,.T.) ;
#71074=ORIENTED_EDGE('',*,*,#50369,.T.) ;
#71075=ORIENTED_EDGE('',*,*,#50617,.T.) ;
#71076=ORIENTED_EDGE('',*,*,#50618,.T.) ;
#71077=ORIENTED_EDGE('',*,*,#50619,.T.) ;
#71078=ORIENTED_EDGE('',*,*,#50620,.T.) ;
#71079=ORIENTED_EDGE('',*,*,#50621,.T.) ;
#71080=ORIENTED_EDGE('',*,*,#50549,.F.) ;
#71081=ORIENTED_EDGE('',*,*,#50622,.T.) ;
#71082=ORIENTED_EDGE('',*,*,#50623,.T.) ;
#71083=ORIENTED_EDGE('',*,*,#50624,.T.) ;
#71084=ORIENTED_EDGE('',*,*,#50625,.T.) ;
#71085=ORIENTED_EDGE('',*,*,#50626,.T.) ;
#71086=ORIENTED_EDGE('',*,*,#50627,.T.) ;
#71087=ORIENTED_EDGE('',*,*,#50628,.T.) ;
#71088=ORIENTED_EDGE('',*,*,#50527,.F.) ;
#71089=ORIENTED_EDGE('',*,*,#50629,.T.) ;
#71090=ORIENTED_EDGE('',*,*,#50630,.T.) ;
#71091=ORIENTED_EDGE('',*,*,#50631,.T.) ;
#71092=ORIENTED_EDGE('',*,*,#50632,.T.) ;
#71093=ORIENTED_EDGE('',*,*,#50633,.T.) ;
#71094=ORIENTED_EDGE('',*,*,#50634,.T.) ;
#71095=ORIENTED_EDGE('',*,*,#50635,.T.) ;
#71096=ORIENTED_EDGE('',*,*,#50505,.F.) ;
#71097=ORIENTED_EDGE('',*,*,#50636,.T.) ;
#71098=ORIENTED_EDGE('',*,*,#50637,.T.) ;
#71099=ORIENTED_EDGE('',*,*,#50638,.T.) ;
#71100=ORIENTED_EDGE('',*,*,#50639,.T.) ;
#71101=ORIENTED_EDGE('',*,*,#50640,.T.) ;
#71102=ORIENTED_EDGE('',*,*,#50641,.T.) ;
#71103=ORIENTED_EDGE('',*,*,#50642,.T.) ;
#71104=ORIENTED_EDGE('',*,*,#50483,.F.) ;
#71105=ORIENTED_EDGE('',*,*,#50643,.T.) ;
#71106=ORIENTED_EDGE('',*,*,#50644,.T.) ;
#71107=ORIENTED_EDGE('',*,*,#50645,.T.) ;
#71108=ORIENTED_EDGE('',*,*,#50646,.T.) ;
#71109=ORIENTED_EDGE('',*,*,#50647,.T.) ;
#71110=ORIENTED_EDGE('',*,*,#50648,.T.) ;
#71111=ORIENTED_EDGE('',*,*,#50649,.T.) ;
#71112=ORIENTED_EDGE('',*,*,#50461,.F.) ;
#71113=ORIENTED_EDGE('',*,*,#50650,.T.) ;
#71114=ORIENTED_EDGE('',*,*,#50651,.T.) ;
#71115=ORIENTED_EDGE('',*,*,#50652,.T.) ;
#71116=ORIENTED_EDGE('',*,*,#50653,.T.) ;
#71117=ORIENTED_EDGE('',*,*,#50654,.T.) ;
#71118=ORIENTED_EDGE('',*,*,#50655,.T.) ;
#71119=ORIENTED_EDGE('',*,*,#50656,.T.) ;
#71120=ORIENTED_EDGE('',*,*,#50439,.F.) ;
#71121=ORIENTED_EDGE('',*,*,#50657,.T.) ;
#71122=ORIENTED_EDGE('',*,*,#50658,.T.) ;
#71123=ORIENTED_EDGE('',*,*,#50659,.T.) ;
#71124=ORIENTED_EDGE('',*,*,#50660,.T.) ;
#71125=ORIENTED_EDGE('',*,*,#50661,.T.) ;
#71126=ORIENTED_EDGE('',*,*,#50662,.T.) ;
#71127=ORIENTED_EDGE('',*,*,#50663,.T.) ;
#71128=ORIENTED_EDGE('',*,*,#50417,.F.) ;
#71129=ORIENTED_EDGE('',*,*,#50664,.T.) ;
#71130=ORIENTED_EDGE('',*,*,#50665,.T.) ;
#71131=ORIENTED_EDGE('',*,*,#50666,.T.) ;
#71132=ORIENTED_EDGE('',*,*,#50667,.T.) ;
#71133=ORIENTED_EDGE('',*,*,#50668,.T.) ;
#71134=ORIENTED_EDGE('',*,*,#50669,.T.) ;
#71135=ORIENTED_EDGE('',*,*,#50670,.T.) ;
#71136=ORIENTED_EDGE('',*,*,#50395,.F.) ;
#71137=ORIENTED_EDGE('',*,*,#50671,.T.) ;
#71138=ORIENTED_EDGE('',*,*,#50672,.T.) ;
#71139=ORIENTED_EDGE('',*,*,#50673,.T.) ;
#71140=ORIENTED_EDGE('',*,*,#50674,.T.) ;
#71141=ORIENTED_EDGE('',*,*,#50675,.T.) ;
#71142=ORIENTED_EDGE('',*,*,#50676,.T.) ;
#71143=ORIENTED_EDGE('',*,*,#50677,.T.) ;
#71144=ORIENTED_EDGE('',*,*,#50373,.F.) ;
#71145=ORIENTED_EDGE('',*,*,#50678,.T.) ;
#71146=ORIENTED_EDGE('',*,*,#50679,.T.) ;
#71147=ORIENTED_EDGE('',*,*,#50680,.T.) ;
#71148=ORIENTED_EDGE('',*,*,#50681,.T.) ;
#71149=ORIENTED_EDGE('',*,*,#50682,.T.) ;
#71150=ORIENTED_EDGE('',*,*,#50683,.T.) ;
#71151=ORIENTED_EDGE('',*,*,#50684,.T.) ;
#71152=ORIENTED_EDGE('',*,*,#50685,.T.) ;
#71153=ORIENTED_EDGE('',*,*,#50686,.T.) ;
#71154=ORIENTED_EDGE('',*,*,#50687,.T.) ;
#71155=ORIENTED_EDGE('',*,*,#50688,.T.) ;
#71156=ORIENTED_EDGE('',*,*,#50689,.T.) ;
#71157=ORIENTED_EDGE('',*,*,#50690,.T.) ;
#71158=ORIENTED_EDGE('',*,*,#50691,.T.) ;
#71159=ORIENTED_EDGE('',*,*,#50692,.T.) ;
#71160=ORIENTED_EDGE('',*,*,#50693,.T.) ;
#71161=ORIENTED_EDGE('',*,*,#50694,.T.) ;
#71162=ORIENTED_EDGE('',*,*,#50695,.T.) ;
#71163=ORIENTED_EDGE('',*,*,#50696,.T.) ;
#71164=ORIENTED_EDGE('',*,*,#50697,.T.) ;
#71165=ORIENTED_EDGE('',*,*,#50698,.T.) ;
#71166=ORIENTED_EDGE('',*,*,#50699,.T.) ;
#71167=ORIENTED_EDGE('',*,*,#50700,.T.) ;
#71168=ORIENTED_EDGE('',*,*,#50701,.T.) ;
#71169=ORIENTED_EDGE('',*,*,#50702,.T.) ;
#71170=ORIENTED_EDGE('',*,*,#50703,.T.) ;
#71171=ORIENTED_EDGE('',*,*,#50704,.T.) ;
#71172=ORIENTED_EDGE('',*,*,#50705,.T.) ;
#71173=ORIENTED_EDGE('',*,*,#50706,.T.) ;
#71174=ORIENTED_EDGE('',*,*,#50707,.T.) ;
#71175=ORIENTED_EDGE('',*,*,#50708,.T.) ;
#71176=ORIENTED_EDGE('',*,*,#50709,.T.) ;
#71177=ORIENTED_EDGE('',*,*,#50710,.T.) ;
#71178=ORIENTED_EDGE('',*,*,#50711,.T.) ;
#71179=ORIENTED_EDGE('',*,*,#50712,.T.) ;
#71180=ORIENTED_EDGE('',*,*,#50713,.T.) ;
#71181=ORIENTED_EDGE('',*,*,#50714,.T.) ;
#71182=ORIENTED_EDGE('',*,*,#50715,.T.) ;
#71183=ORIENTED_EDGE('',*,*,#50716,.T.) ;
#71184=ORIENTED_EDGE('',*,*,#50717,.T.) ;
#71185=ORIENTED_EDGE('',*,*,#50718,.T.) ;
#71186=ORIENTED_EDGE('',*,*,#50719,.T.) ;
#71187=ORIENTED_EDGE('',*,*,#50720,.T.) ;
#71188=ORIENTED_EDGE('',*,*,#50721,.T.) ;
#71189=ORIENTED_EDGE('',*,*,#50722,.T.) ;
#71190=ORIENTED_EDGE('',*,*,#50723,.T.) ;
#71191=ORIENTED_EDGE('',*,*,#50724,.T.) ;
#71192=ORIENTED_EDGE('',*,*,#50725,.T.) ;
#71193=ORIENTED_EDGE('',*,*,#50726,.T.) ;
#71194=ORIENTED_EDGE('',*,*,#50727,.T.) ;
#71195=ORIENTED_EDGE('',*,*,#50728,.T.) ;
#71196=ORIENTED_EDGE('',*,*,#50729,.T.) ;
#71197=ORIENTED_EDGE('',*,*,#50730,.T.) ;
#71198=ORIENTED_EDGE('',*,*,#50731,.T.) ;
#71199=ORIENTED_EDGE('',*,*,#50732,.T.) ;
#71200=ORIENTED_EDGE('',*,*,#50733,.T.) ;
#71201=ORIENTED_EDGE('',*,*,#50734,.T.) ;
#71202=ORIENTED_EDGE('',*,*,#50735,.T.) ;
#71203=ORIENTED_EDGE('',*,*,#50736,.T.) ;
#71204=ORIENTED_EDGE('',*,*,#50737,.T.) ;
#71205=ORIENTED_EDGE('',*,*,#50738,.T.) ;
#71206=ORIENTED_EDGE('',*,*,#50739,.T.) ;
#71207=ORIENTED_EDGE('',*,*,#50740,.T.) ;
#71208=ORIENTED_EDGE('',*,*,#50741,.T.) ;
#71209=ORIENTED_EDGE('',*,*,#50742,.T.) ;
#71210=ORIENTED_EDGE('',*,*,#50743,.T.) ;
#71211=ORIENTED_EDGE('',*,*,#50744,.T.) ;
#71212=ORIENTED_EDGE('',*,*,#50745,.T.) ;
#71213=ORIENTED_EDGE('',*,*,#50746,.T.) ;
#71214=ORIENTED_EDGE('',*,*,#50747,.T.) ;
#71215=ORIENTED_EDGE('',*,*,#50748,.T.) ;
#71216=ORIENTED_EDGE('',*,*,#50749,.T.) ;
#71217=ORIENTED_EDGE('',*,*,#50750,.T.) ;
#71218=ORIENTED_EDGE('',*,*,#50751,.T.) ;
#71219=ORIENTED_EDGE('',*,*,#50752,.T.) ;
#71220=ORIENTED_EDGE('',*,*,#50753,.T.) ;
#71221=ORIENTED_EDGE('',*,*,#50754,.T.) ;
#71222=ORIENTED_EDGE('',*,*,#50755,.T.) ;
#71223=ORIENTED_EDGE('',*,*,#50756,.T.) ;
#71224=ORIENTED_EDGE('',*,*,#50757,.T.) ;
#71225=ORIENTED_EDGE('',*,*,#50758,.T.) ;
#71226=ORIENTED_EDGE('',*,*,#50759,.T.) ;
#71227=ORIENTED_EDGE('',*,*,#50760,.T.) ;
#71228=ORIENTED_EDGE('',*,*,#50761,.T.) ;
#71229=ORIENTED_EDGE('',*,*,#50762,.T.) ;
#71230=ORIENTED_EDGE('',*,*,#50763,.T.) ;
#71231=ORIENTED_EDGE('',*,*,#50764,.T.) ;
#71232=ORIENTED_EDGE('',*,*,#50765,.T.) ;
#71233=ORIENTED_EDGE('',*,*,#50766,.T.) ;
#71234=ORIENTED_EDGE('',*,*,#50767,.T.) ;
#71235=ORIENTED_EDGE('',*,*,#50768,.T.) ;
#71236=ORIENTED_EDGE('',*,*,#50769,.T.) ;
#71237=ORIENTED_EDGE('',*,*,#50770,.T.) ;
#71238=ORIENTED_EDGE('',*,*,#50771,.T.) ;
#71239=ORIENTED_EDGE('',*,*,#50772,.T.) ;
#71240=ORIENTED_EDGE('',*,*,#50773,.T.) ;
#71241=ORIENTED_EDGE('',*,*,#50774,.T.) ;
#71242=ORIENTED_EDGE('',*,*,#50775,.T.) ;
#71243=ORIENTED_EDGE('',*,*,#50776,.T.) ;
#71244=ORIENTED_EDGE('',*,*,#50777,.T.) ;
#71245=ORIENTED_EDGE('',*,*,#50778,.T.) ;
#71246=ORIENTED_EDGE('',*,*,#50779,.T.) ;
#71247=ORIENTED_EDGE('',*,*,#50780,.T.) ;
#71248=ORIENTED_EDGE('',*,*,#50781,.T.) ;
#71249=ORIENTED_EDGE('',*,*,#50782,.T.) ;
#71250=ORIENTED_EDGE('',*,*,#50783,.T.) ;
#71251=ORIENTED_EDGE('',*,*,#50784,.T.) ;
#71252=ORIENTED_EDGE('',*,*,#50785,.T.) ;
#71253=ORIENTED_EDGE('',*,*,#50786,.T.) ;
#71254=ORIENTED_EDGE('',*,*,#50787,.T.) ;
#71255=ORIENTED_EDGE('',*,*,#50788,.T.) ;
#71256=ORIENTED_EDGE('',*,*,#50789,.T.) ;
#71257=ORIENTED_EDGE('',*,*,#50790,.T.) ;
#71258=ORIENTED_EDGE('',*,*,#50791,.T.) ;
#71259=ORIENTED_EDGE('',*,*,#50792,.T.) ;
#71260=ORIENTED_EDGE('',*,*,#50793,.T.) ;
#71261=ORIENTED_EDGE('',*,*,#50794,.T.) ;
#71262=ORIENTED_EDGE('',*,*,#50795,.T.) ;
#71263=ORIENTED_EDGE('',*,*,#50796,.T.) ;
#71264=ORIENTED_EDGE('',*,*,#50797,.T.) ;
#71265=ORIENTED_EDGE('',*,*,#50798,.T.) ;
#71266=ORIENTED_EDGE('',*,*,#50799,.T.) ;
#71267=ORIENTED_EDGE('',*,*,#50800,.T.) ;
#71268=ORIENTED_EDGE('',*,*,#50801,.T.) ;
#71269=ORIENTED_EDGE('',*,*,#50802,.T.) ;
#71270=ORIENTED_EDGE('',*,*,#50803,.T.) ;
#71271=ORIENTED_EDGE('',*,*,#50804,.T.) ;
#71272=ORIENTED_EDGE('',*,*,#50805,.T.) ;
#71273=ORIENTED_EDGE('',*,*,#50806,.T.) ;
#71274=ORIENTED_EDGE('',*,*,#50807,.T.) ;
#71275=ORIENTED_EDGE('',*,*,#50808,.T.) ;
#71276=ORIENTED_EDGE('',*,*,#50809,.T.) ;
#71277=ORIENTED_EDGE('',*,*,#50810,.T.) ;
#71278=ORIENTED_EDGE('',*,*,#50811,.T.) ;
#71279=ORIENTED_EDGE('',*,*,#50812,.T.) ;
#71280=ORIENTED_EDGE('',*,*,#50813,.T.) ;
#71281=ORIENTED_EDGE('',*,*,#50814,.T.) ;
#71282=ORIENTED_EDGE('',*,*,#50815,.T.) ;
#71283=ORIENTED_EDGE('',*,*,#50816,.T.) ;
#71284=ORIENTED_EDGE('',*,*,#50817,.T.) ;
#71285=ORIENTED_EDGE('',*,*,#50818,.T.) ;
#71286=ORIENTED_EDGE('',*,*,#50819,.T.) ;
#71287=ORIENTED_EDGE('',*,*,#50820,.T.) ;
#71288=ORIENTED_EDGE('',*,*,#50821,.T.) ;
#71289=ORIENTED_EDGE('',*,*,#50822,.T.) ;
#71290=ORIENTED_EDGE('',*,*,#50823,.T.) ;
#71291=ORIENTED_EDGE('',*,*,#50824,.T.) ;
#71292=ORIENTED_EDGE('',*,*,#50825,.T.) ;
#71293=ORIENTED_EDGE('',*,*,#50826,.T.) ;
#71294=ORIENTED_EDGE('',*,*,#50827,.T.) ;
#71295=ORIENTED_EDGE('',*,*,#50828,.T.) ;
#71296=ORIENTED_EDGE('',*,*,#50829,.F.) ;
#71297=ORIENTED_EDGE('',*,*,#50830,.T.) ;
#71298=ORIENTED_EDGE('',*,*,#50831,.F.) ;
#71299=ORIENTED_EDGE('',*,*,#50832,.T.) ;
#71300=ORIENTED_EDGE('',*,*,#50833,.F.) ;
#71301=ORIENTED_EDGE('',*,*,#50834,.T.) ;
#71302=ORIENTED_EDGE('',*,*,#50835,.F.) ;
#71303=ORIENTED_EDGE('',*,*,#50836,.T.) ;
#71304=ORIENTED_EDGE('',*,*,#50835,.T.) ;
#71305=ORIENTED_EDGE('',*,*,#50837,.T.) ;
#71306=ORIENTED_EDGE('',*,*,#50838,.T.) ;
#71307=ORIENTED_EDGE('',*,*,#50839,.T.) ;
#71308=ORIENTED_EDGE('',*,*,#50829,.T.) ;
#71309=ORIENTED_EDGE('',*,*,#50840,.T.) ;
#71310=ORIENTED_EDGE('',*,*,#50841,.T.) ;
#71311=ORIENTED_EDGE('',*,*,#50842,.T.) ;
#71312=ORIENTED_EDGE('',*,*,#50843,.T.) ;
#71313=ORIENTED_EDGE('',*,*,#50844,.T.) ;
#71314=ORIENTED_EDGE('',*,*,#50831,.T.) ;
#71315=ORIENTED_EDGE('',*,*,#50845,.T.) ;
#71316=ORIENTED_EDGE('',*,*,#50833,.T.) ;
#71317=ORIENTED_EDGE('',*,*,#50846,.T.) ;
#71318=ORIENTED_EDGE('',*,*,#50847,.T.) ;
#71319=ORIENTED_EDGE('',*,*,#50848,.T.) ;
#71320=ORIENTED_EDGE('',*,*,#50849,.T.) ;
#71321=ORIENTED_EDGE('',*,*,#50850,.T.) ;
#71322=ORIENTED_EDGE('',*,*,#50851,.T.) ;
#71323=ORIENTED_EDGE('',*,*,#50852,.T.) ;
#71324=ORIENTED_EDGE('',*,*,#50853,.F.) ;
#71325=ORIENTED_EDGE('',*,*,#50854,.T.) ;
#71326=ORIENTED_EDGE('',*,*,#50855,.F.) ;
#71327=ORIENTED_EDGE('',*,*,#50856,.T.) ;
#71328=ORIENTED_EDGE('',*,*,#50857,.F.) ;
#71329=ORIENTED_EDGE('',*,*,#50858,.T.) ;
#71330=ORIENTED_EDGE('',*,*,#50859,.F.) ;
#71331=ORIENTED_EDGE('',*,*,#50860,.T.) ;
#71332=ORIENTED_EDGE('',*,*,#50859,.T.) ;
#71333=ORIENTED_EDGE('',*,*,#50861,.T.) ;
#71334=ORIENTED_EDGE('',*,*,#50862,.T.) ;
#71335=ORIENTED_EDGE('',*,*,#50863,.T.) ;
#71336=ORIENTED_EDGE('',*,*,#50853,.T.) ;
#71337=ORIENTED_EDGE('',*,*,#50864,.T.) ;
#71338=ORIENTED_EDGE('',*,*,#50865,.T.) ;
#71339=ORIENTED_EDGE('',*,*,#50866,.T.) ;
#71340=ORIENTED_EDGE('',*,*,#50867,.T.) ;
#71341=ORIENTED_EDGE('',*,*,#50868,.T.) ;
#71342=ORIENTED_EDGE('',*,*,#50855,.T.) ;
#71343=ORIENTED_EDGE('',*,*,#50869,.T.) ;
#71344=ORIENTED_EDGE('',*,*,#50857,.T.) ;
#71345=ORIENTED_EDGE('',*,*,#50870,.T.) ;
#71346=ORIENTED_EDGE('',*,*,#50871,.T.) ;
#71347=ORIENTED_EDGE('',*,*,#50872,.T.) ;
#71348=ORIENTED_EDGE('',*,*,#50873,.T.) ;
#71349=ORIENTED_EDGE('',*,*,#50874,.T.) ;
#71350=ORIENTED_EDGE('',*,*,#50875,.T.) ;
#71351=ORIENTED_EDGE('',*,*,#50876,.T.) ;
#71352=ORIENTED_EDGE('',*,*,#50877,.F.) ;
#71353=ORIENTED_EDGE('',*,*,#50878,.T.) ;
#71354=ORIENTED_EDGE('',*,*,#50879,.F.) ;
#71355=ORIENTED_EDGE('',*,*,#50880,.T.) ;
#71356=ORIENTED_EDGE('',*,*,#50881,.F.) ;
#71357=ORIENTED_EDGE('',*,*,#50882,.T.) ;
#71358=ORIENTED_EDGE('',*,*,#50883,.F.) ;
#71359=ORIENTED_EDGE('',*,*,#50884,.T.) ;
#71360=ORIENTED_EDGE('',*,*,#50883,.T.) ;
#71361=ORIENTED_EDGE('',*,*,#50885,.T.) ;
#71362=ORIENTED_EDGE('',*,*,#50886,.T.) ;
#71363=ORIENTED_EDGE('',*,*,#50887,.T.) ;
#71364=ORIENTED_EDGE('',*,*,#50877,.T.) ;
#71365=ORIENTED_EDGE('',*,*,#50888,.T.) ;
#71366=ORIENTED_EDGE('',*,*,#50889,.T.) ;
#71367=ORIENTED_EDGE('',*,*,#50890,.T.) ;
#71368=ORIENTED_EDGE('',*,*,#50891,.T.) ;
#71369=ORIENTED_EDGE('',*,*,#50892,.T.) ;
#71370=ORIENTED_EDGE('',*,*,#50879,.T.) ;
#71371=ORIENTED_EDGE('',*,*,#50893,.T.) ;
#71372=ORIENTED_EDGE('',*,*,#50881,.T.) ;
#71373=ORIENTED_EDGE('',*,*,#50894,.T.) ;
#71374=ORIENTED_EDGE('',*,*,#50895,.T.) ;
#71375=ORIENTED_EDGE('',*,*,#50896,.T.) ;
#71376=ORIENTED_EDGE('',*,*,#50897,.T.) ;
#71377=ORIENTED_EDGE('',*,*,#50898,.T.) ;
#71378=ORIENTED_EDGE('',*,*,#50899,.T.) ;
#71379=ORIENTED_EDGE('',*,*,#50900,.T.) ;
#71380=ORIENTED_EDGE('',*,*,#50901,.F.) ;
#71381=ORIENTED_EDGE('',*,*,#50902,.T.) ;
#71382=ORIENTED_EDGE('',*,*,#50903,.F.) ;
#71383=ORIENTED_EDGE('',*,*,#50904,.T.) ;
#71384=ORIENTED_EDGE('',*,*,#50905,.F.) ;
#71385=ORIENTED_EDGE('',*,*,#50906,.T.) ;
#71386=ORIENTED_EDGE('',*,*,#50907,.F.) ;
#71387=ORIENTED_EDGE('',*,*,#50908,.T.) ;
#71388=ORIENTED_EDGE('',*,*,#50907,.T.) ;
#71389=ORIENTED_EDGE('',*,*,#50909,.T.) ;
#71390=ORIENTED_EDGE('',*,*,#50910,.T.) ;
#71391=ORIENTED_EDGE('',*,*,#50911,.T.) ;
#71392=ORIENTED_EDGE('',*,*,#50901,.T.) ;
#71393=ORIENTED_EDGE('',*,*,#50912,.T.) ;
#71394=ORIENTED_EDGE('',*,*,#50913,.T.) ;
#71395=ORIENTED_EDGE('',*,*,#50914,.T.) ;
#71396=ORIENTED_EDGE('',*,*,#50915,.T.) ;
#71397=ORIENTED_EDGE('',*,*,#50916,.T.) ;
#71398=ORIENTED_EDGE('',*,*,#50903,.T.) ;
#71399=ORIENTED_EDGE('',*,*,#50917,.T.) ;
#71400=ORIENTED_EDGE('',*,*,#50905,.T.) ;
#71401=ORIENTED_EDGE('',*,*,#50918,.T.) ;
#71402=ORIENTED_EDGE('',*,*,#50919,.T.) ;
#71403=ORIENTED_EDGE('',*,*,#50920,.T.) ;
#71404=ORIENTED_EDGE('',*,*,#50921,.T.) ;
#71405=ORIENTED_EDGE('',*,*,#50922,.T.) ;
#71406=ORIENTED_EDGE('',*,*,#50923,.T.) ;
#71407=ORIENTED_EDGE('',*,*,#50924,.T.) ;
#71408=ORIENTED_EDGE('',*,*,#50925,.F.) ;
#71409=ORIENTED_EDGE('',*,*,#50926,.T.) ;
#71410=ORIENTED_EDGE('',*,*,#50927,.F.) ;
#71411=ORIENTED_EDGE('',*,*,#50928,.T.) ;
#71412=ORIENTED_EDGE('',*,*,#50929,.F.) ;
#71413=ORIENTED_EDGE('',*,*,#50930,.T.) ;
#71414=ORIENTED_EDGE('',*,*,#50931,.F.) ;
#71415=ORIENTED_EDGE('',*,*,#50932,.T.) ;
#71416=ORIENTED_EDGE('',*,*,#50931,.T.) ;
#71417=ORIENTED_EDGE('',*,*,#50933,.T.) ;
#71418=ORIENTED_EDGE('',*,*,#50934,.T.) ;
#71419=ORIENTED_EDGE('',*,*,#50935,.T.) ;
#71420=ORIENTED_EDGE('',*,*,#50925,.T.) ;
#71421=ORIENTED_EDGE('',*,*,#50936,.T.) ;
#71422=ORIENTED_EDGE('',*,*,#50937,.T.) ;
#71423=ORIENTED_EDGE('',*,*,#50938,.T.) ;
#71424=ORIENTED_EDGE('',*,*,#50939,.T.) ;
#71425=ORIENTED_EDGE('',*,*,#50940,.T.) ;
#71426=ORIENTED_EDGE('',*,*,#50927,.T.) ;
#71427=ORIENTED_EDGE('',*,*,#50941,.T.) ;
#71428=ORIENTED_EDGE('',*,*,#50929,.T.) ;
#71429=ORIENTED_EDGE('',*,*,#50942,.T.) ;
#71430=ORIENTED_EDGE('',*,*,#50943,.T.) ;
#71431=ORIENTED_EDGE('',*,*,#50944,.T.) ;
#71432=ORIENTED_EDGE('',*,*,#50945,.T.) ;
#71433=ORIENTED_EDGE('',*,*,#50946,.T.) ;
#71434=ORIENTED_EDGE('',*,*,#50947,.T.) ;
#71435=ORIENTED_EDGE('',*,*,#50948,.T.) ;
#71436=ORIENTED_EDGE('',*,*,#50949,.F.) ;
#71437=ORIENTED_EDGE('',*,*,#50950,.T.) ;
#71438=ORIENTED_EDGE('',*,*,#50951,.F.) ;
#71439=ORIENTED_EDGE('',*,*,#50952,.T.) ;
#71440=ORIENTED_EDGE('',*,*,#50953,.F.) ;
#71441=ORIENTED_EDGE('',*,*,#50954,.T.) ;
#71442=ORIENTED_EDGE('',*,*,#50955,.F.) ;
#71443=ORIENTED_EDGE('',*,*,#50956,.T.) ;
#71444=ORIENTED_EDGE('',*,*,#50955,.T.) ;
#71445=ORIENTED_EDGE('',*,*,#50957,.T.) ;
#71446=ORIENTED_EDGE('',*,*,#50958,.T.) ;
#71447=ORIENTED_EDGE('',*,*,#50959,.T.) ;
#71448=ORIENTED_EDGE('',*,*,#50949,.T.) ;
#71449=ORIENTED_EDGE('',*,*,#50960,.T.) ;
#71450=ORIENTED_EDGE('',*,*,#50961,.T.) ;
#71451=ORIENTED_EDGE('',*,*,#50962,.T.) ;
#71452=ORIENTED_EDGE('',*,*,#50963,.T.) ;
#71453=ORIENTED_EDGE('',*,*,#50964,.T.) ;
#71454=ORIENTED_EDGE('',*,*,#50951,.T.) ;
#71455=ORIENTED_EDGE('',*,*,#50965,.T.) ;
#71456=ORIENTED_EDGE('',*,*,#50953,.T.) ;
#71457=ORIENTED_EDGE('',*,*,#50966,.T.) ;
#71458=ORIENTED_EDGE('',*,*,#50967,.T.) ;
#71459=ORIENTED_EDGE('',*,*,#50968,.T.) ;
#71460=ORIENTED_EDGE('',*,*,#50969,.T.) ;
#71461=ORIENTED_EDGE('',*,*,#50970,.T.) ;
#71462=ORIENTED_EDGE('',*,*,#50971,.T.) ;
#71463=ORIENTED_EDGE('',*,*,#50972,.T.) ;
#71464=ORIENTED_EDGE('',*,*,#50973,.F.) ;
#71465=ORIENTED_EDGE('',*,*,#50974,.T.) ;
#71466=ORIENTED_EDGE('',*,*,#50975,.F.) ;
#71467=ORIENTED_EDGE('',*,*,#50976,.T.) ;
#71468=ORIENTED_EDGE('',*,*,#50977,.F.) ;
#71469=ORIENTED_EDGE('',*,*,#50978,.T.) ;
#71470=ORIENTED_EDGE('',*,*,#50979,.F.) ;
#71471=ORIENTED_EDGE('',*,*,#50980,.T.) ;
#71472=ORIENTED_EDGE('',*,*,#50979,.T.) ;
#71473=ORIENTED_EDGE('',*,*,#50981,.T.) ;
#71474=ORIENTED_EDGE('',*,*,#50982,.T.) ;
#71475=ORIENTED_EDGE('',*,*,#50983,.T.) ;
#71476=ORIENTED_EDGE('',*,*,#50973,.T.) ;
#71477=ORIENTED_EDGE('',*,*,#50984,.T.) ;
#71478=ORIENTED_EDGE('',*,*,#50985,.T.) ;
#71479=ORIENTED_EDGE('',*,*,#50986,.T.) ;
#71480=ORIENTED_EDGE('',*,*,#50987,.T.) ;
#71481=ORIENTED_EDGE('',*,*,#50988,.T.) ;
#71482=ORIENTED_EDGE('',*,*,#50975,.T.) ;
#71483=ORIENTED_EDGE('',*,*,#50989,.T.) ;
#71484=ORIENTED_EDGE('',*,*,#50977,.T.) ;
#71485=ORIENTED_EDGE('',*,*,#50990,.T.) ;
#71486=ORIENTED_EDGE('',*,*,#50991,.T.) ;
#71487=ORIENTED_EDGE('',*,*,#50992,.T.) ;
#71488=ORIENTED_EDGE('',*,*,#50993,.T.) ;
#71489=ORIENTED_EDGE('',*,*,#50994,.T.) ;
#71490=ORIENTED_EDGE('',*,*,#50995,.T.) ;
#71491=ORIENTED_EDGE('',*,*,#50996,.T.) ;
#71492=ORIENTED_EDGE('',*,*,#50997,.F.) ;
#71493=ORIENTED_EDGE('',*,*,#50998,.T.) ;
#71494=ORIENTED_EDGE('',*,*,#50999,.F.) ;
#71495=ORIENTED_EDGE('',*,*,#51000,.T.) ;
#71496=ORIENTED_EDGE('',*,*,#51001,.F.) ;
#71497=ORIENTED_EDGE('',*,*,#51002,.T.) ;
#71498=ORIENTED_EDGE('',*,*,#51003,.F.) ;
#71499=ORIENTED_EDGE('',*,*,#51004,.T.) ;
#71500=ORIENTED_EDGE('',*,*,#51003,.T.) ;
#71501=ORIENTED_EDGE('',*,*,#51005,.T.) ;
#71502=ORIENTED_EDGE('',*,*,#51006,.T.) ;
#71503=ORIENTED_EDGE('',*,*,#51007,.T.) ;
#71504=ORIENTED_EDGE('',*,*,#50997,.T.) ;
#71505=ORIENTED_EDGE('',*,*,#51008,.T.) ;
#71506=ORIENTED_EDGE('',*,*,#51009,.T.) ;
#71507=ORIENTED_EDGE('',*,*,#51010,.T.) ;
#71508=ORIENTED_EDGE('',*,*,#51011,.T.) ;
#71509=ORIENTED_EDGE('',*,*,#51012,.T.) ;
#71510=ORIENTED_EDGE('',*,*,#50999,.T.) ;
#71511=ORIENTED_EDGE('',*,*,#51013,.T.) ;
#71512=ORIENTED_EDGE('',*,*,#51001,.T.) ;
#71513=ORIENTED_EDGE('',*,*,#51014,.T.) ;
#71514=ORIENTED_EDGE('',*,*,#51015,.T.) ;
#71515=ORIENTED_EDGE('',*,*,#51016,.T.) ;
#71516=ORIENTED_EDGE('',*,*,#51017,.T.) ;
#71517=ORIENTED_EDGE('',*,*,#51018,.T.) ;
#71518=ORIENTED_EDGE('',*,*,#51019,.T.) ;
#71519=ORIENTED_EDGE('',*,*,#51020,.T.) ;
#71520=ORIENTED_EDGE('',*,*,#51021,.F.) ;
#71521=ORIENTED_EDGE('',*,*,#51022,.T.) ;
#71522=ORIENTED_EDGE('',*,*,#51023,.F.) ;
#71523=ORIENTED_EDGE('',*,*,#51024,.T.) ;
#71524=ORIENTED_EDGE('',*,*,#51025,.F.) ;
#71525=ORIENTED_EDGE('',*,*,#51026,.T.) ;
#71526=ORIENTED_EDGE('',*,*,#51027,.F.) ;
#71527=ORIENTED_EDGE('',*,*,#51028,.T.) ;
#71528=ORIENTED_EDGE('',*,*,#51027,.T.) ;
#71529=ORIENTED_EDGE('',*,*,#51029,.T.) ;
#71530=ORIENTED_EDGE('',*,*,#51030,.T.) ;
#71531=ORIENTED_EDGE('',*,*,#51031,.T.) ;
#71532=ORIENTED_EDGE('',*,*,#51021,.T.) ;
#71533=ORIENTED_EDGE('',*,*,#51032,.T.) ;
#71534=ORIENTED_EDGE('',*,*,#51033,.T.) ;
#71535=ORIENTED_EDGE('',*,*,#51034,.T.) ;
#71536=ORIENTED_EDGE('',*,*,#51035,.T.) ;
#71537=ORIENTED_EDGE('',*,*,#51036,.T.) ;
#71538=ORIENTED_EDGE('',*,*,#51023,.T.) ;
#71539=ORIENTED_EDGE('',*,*,#51037,.T.) ;
#71540=ORIENTED_EDGE('',*,*,#51025,.T.) ;
#71541=ORIENTED_EDGE('',*,*,#51038,.T.) ;
#71542=ORIENTED_EDGE('',*,*,#51039,.T.) ;
#71543=ORIENTED_EDGE('',*,*,#51040,.T.) ;
#71544=ORIENTED_EDGE('',*,*,#51041,.T.) ;
#71545=ORIENTED_EDGE('',*,*,#51042,.T.) ;
#71546=ORIENTED_EDGE('',*,*,#51043,.T.) ;
#71547=ORIENTED_EDGE('',*,*,#51044,.T.) ;
#71548=ORIENTED_EDGE('',*,*,#51045,.T.) ;
#71549=ORIENTED_EDGE('',*,*,#51046,.T.) ;
#71550=ORIENTED_EDGE('',*,*,#51047,.T.) ;
#71551=ORIENTED_EDGE('',*,*,#51048,.T.) ;
#71552=ORIENTED_EDGE('',*,*,#51049,.T.) ;
#71553=ORIENTED_EDGE('',*,*,#51050,.T.) ;
#71554=ORIENTED_EDGE('',*,*,#51051,.T.) ;
#71555=ORIENTED_EDGE('',*,*,#51052,.T.) ;
#71556=ORIENTED_EDGE('',*,*,#51053,.T.) ;
#71557=ORIENTED_EDGE('',*,*,#51054,.T.) ;
#71558=ORIENTED_EDGE('',*,*,#51055,.T.) ;
#71559=ORIENTED_EDGE('',*,*,#51056,.T.) ;
#71560=ORIENTED_EDGE('',*,*,#51057,.T.) ;
#71561=ORIENTED_EDGE('',*,*,#51058,.T.) ;
#71562=ORIENTED_EDGE('',*,*,#51059,.T.) ;
#71563=ORIENTED_EDGE('',*,*,#51060,.T.) ;
#71564=ORIENTED_EDGE('',*,*,#51061,.T.) ;
#71565=ORIENTED_EDGE('',*,*,#51062,.T.) ;
#71566=ORIENTED_EDGE('',*,*,#51063,.T.) ;
#71567=ORIENTED_EDGE('',*,*,#51064,.T.) ;
#71568=ORIENTED_EDGE('',*,*,#51065,.T.) ;
#71569=ORIENTED_EDGE('',*,*,#51066,.T.) ;
#71570=ORIENTED_EDGE('',*,*,#51067,.T.) ;
#71571=ORIENTED_EDGE('',*,*,#51068,.T.) ;
#71572=ORIENTED_EDGE('',*,*,#51069,.T.) ;
#71573=ORIENTED_EDGE('',*,*,#51070,.T.) ;
#71574=ORIENTED_EDGE('',*,*,#51071,.T.) ;
#71575=ORIENTED_EDGE('',*,*,#51072,.T.) ;
#71576=ORIENTED_EDGE('',*,*,#51073,.T.) ;
#71577=ORIENTED_EDGE('',*,*,#51074,.T.) ;
#71578=ORIENTED_EDGE('',*,*,#51075,.T.) ;
#71579=ORIENTED_EDGE('',*,*,#51076,.T.) ;
#71580=ORIENTED_EDGE('',*,*,#51077,.T.) ;
#71581=ORIENTED_EDGE('',*,*,#51078,.T.) ;
#71582=ORIENTED_EDGE('',*,*,#51079,.T.) ;
#71583=ORIENTED_EDGE('',*,*,#51080,.T.) ;
#71584=ORIENTED_EDGE('',*,*,#51081,.T.) ;
#71585=ORIENTED_EDGE('',*,*,#51082,.T.) ;
#71586=ORIENTED_EDGE('',*,*,#51083,.F.) ;
#71587=ORIENTED_EDGE('',*,*,#51084,.T.) ;
#71588=ORIENTED_EDGE('',*,*,#51085,.T.) ;
#71589=ORIENTED_EDGE('',*,*,#51086,.T.) ;
#71590=ORIENTED_EDGE('',*,*,#51087,.T.) ;
#71591=ORIENTED_EDGE('',*,*,#51088,.T.) ;
#71592=ORIENTED_EDGE('',*,*,#51089,.T.) ;
#71593=ORIENTED_EDGE('',*,*,#51090,.T.) ;
#71594=ORIENTED_EDGE('',*,*,#51091,.T.) ;
#71595=ORIENTED_EDGE('',*,*,#51092,.T.) ;
#71596=ORIENTED_EDGE('',*,*,#51093,.T.) ;
#71597=ORIENTED_EDGE('',*,*,#51094,.T.) ;
#71598=ORIENTED_EDGE('',*,*,#51095,.T.) ;
#71599=ORIENTED_EDGE('',*,*,#51096,.T.) ;
#71600=ORIENTED_EDGE('',*,*,#51097,.F.) ;
#71601=ORIENTED_EDGE('',*,*,#51098,.T.) ;
#71602=ORIENTED_EDGE('',*,*,#51099,.T.) ;
#71603=ORIENTED_EDGE('',*,*,#51100,.T.) ;
#71604=ORIENTED_EDGE('',*,*,#51101,.T.) ;
#71605=ORIENTED_EDGE('',*,*,#51102,.T.) ;
#71606=ORIENTED_EDGE('',*,*,#51103,.T.) ;
#71607=ORIENTED_EDGE('',*,*,#51104,.T.) ;
#71608=ORIENTED_EDGE('',*,*,#51105,.T.) ;
#71609=ORIENTED_EDGE('',*,*,#51106,.T.) ;
#71610=ORIENTED_EDGE('',*,*,#51107,.T.) ;
#71611=ORIENTED_EDGE('',*,*,#51108,.T.) ;
#71612=ORIENTED_EDGE('',*,*,#51109,.T.) ;
#71613=ORIENTED_EDGE('',*,*,#51110,.T.) ;
#71614=ORIENTED_EDGE('',*,*,#51111,.F.) ;
#71615=ORIENTED_EDGE('',*,*,#51112,.T.) ;
#71616=ORIENTED_EDGE('',*,*,#51113,.T.) ;
#71617=ORIENTED_EDGE('',*,*,#51114,.T.) ;
#71618=ORIENTED_EDGE('',*,*,#51115,.T.) ;
#71619=ORIENTED_EDGE('',*,*,#51116,.T.) ;
#71620=ORIENTED_EDGE('',*,*,#51117,.T.) ;
#71621=ORIENTED_EDGE('',*,*,#51118,.T.) ;
#71622=ORIENTED_EDGE('',*,*,#51119,.T.) ;
#71623=ORIENTED_EDGE('',*,*,#51120,.T.) ;
#71624=ORIENTED_EDGE('',*,*,#51121,.T.) ;
#71625=ORIENTED_EDGE('',*,*,#51122,.T.) ;
#71626=ORIENTED_EDGE('',*,*,#51123,.T.) ;
#71627=ORIENTED_EDGE('',*,*,#51124,.T.) ;
#71628=ORIENTED_EDGE('',*,*,#51125,.F.) ;
#71629=ORIENTED_EDGE('',*,*,#51126,.T.) ;
#71630=ORIENTED_EDGE('',*,*,#51127,.T.) ;
#71631=ORIENTED_EDGE('',*,*,#51128,.T.) ;
#71632=ORIENTED_EDGE('',*,*,#51129,.T.) ;
#71633=ORIENTED_EDGE('',*,*,#51130,.T.) ;
#71634=ORIENTED_EDGE('',*,*,#51131,.T.) ;
#71635=ORIENTED_EDGE('',*,*,#51132,.T.) ;
#71636=ORIENTED_EDGE('',*,*,#51133,.T.) ;
#71637=ORIENTED_EDGE('',*,*,#51134,.T.) ;
#71638=ORIENTED_EDGE('',*,*,#51135,.T.) ;
#71639=ORIENTED_EDGE('',*,*,#51136,.T.) ;
#71640=ORIENTED_EDGE('',*,*,#51137,.T.) ;
#71641=ORIENTED_EDGE('',*,*,#51138,.T.) ;
#71642=ORIENTED_EDGE('',*,*,#51139,.F.) ;
#71643=ORIENTED_EDGE('',*,*,#51140,.T.) ;
#71644=ORIENTED_EDGE('',*,*,#51141,.T.) ;
#71645=ORIENTED_EDGE('',*,*,#51142,.T.) ;
#71646=ORIENTED_EDGE('',*,*,#51143,.T.) ;
#71647=ORIENTED_EDGE('',*,*,#51144,.T.) ;
#71648=ORIENTED_EDGE('',*,*,#51145,.T.) ;
#71649=ORIENTED_EDGE('',*,*,#51146,.T.) ;
#71650=ORIENTED_EDGE('',*,*,#51147,.T.) ;
#71651=ORIENTED_EDGE('',*,*,#51148,.T.) ;
#71652=ORIENTED_EDGE('',*,*,#51149,.T.) ;
#71653=ORIENTED_EDGE('',*,*,#51150,.T.) ;
#71654=ORIENTED_EDGE('',*,*,#51151,.T.) ;
#71655=ORIENTED_EDGE('',*,*,#51152,.T.) ;
#71656=ORIENTED_EDGE('',*,*,#51153,.F.) ;
#71657=ORIENTED_EDGE('',*,*,#51154,.T.) ;
#71658=ORIENTED_EDGE('',*,*,#51155,.T.) ;
#71659=ORIENTED_EDGE('',*,*,#51156,.T.) ;
#71660=ORIENTED_EDGE('',*,*,#51157,.T.) ;
#71661=ORIENTED_EDGE('',*,*,#51158,.T.) ;
#71662=ORIENTED_EDGE('',*,*,#51159,.T.) ;
#71663=ORIENTED_EDGE('',*,*,#51160,.T.) ;
#71664=ORIENTED_EDGE('',*,*,#51161,.T.) ;
#71665=ORIENTED_EDGE('',*,*,#51162,.T.) ;
#71666=ORIENTED_EDGE('',*,*,#51163,.T.) ;
#71667=ORIENTED_EDGE('',*,*,#51164,.T.) ;
#71668=ORIENTED_EDGE('',*,*,#51165,.T.) ;
#71669=ORIENTED_EDGE('',*,*,#51166,.T.) ;
#71670=ORIENTED_EDGE('',*,*,#51167,.F.) ;
#71671=ORIENTED_EDGE('',*,*,#51168,.T.) ;
#71672=ORIENTED_EDGE('',*,*,#51169,.T.) ;
#71673=ORIENTED_EDGE('',*,*,#51170,.T.) ;
#71674=ORIENTED_EDGE('',*,*,#51171,.T.) ;
#71675=ORIENTED_EDGE('',*,*,#51172,.T.) ;
#71676=ORIENTED_EDGE('',*,*,#51173,.T.) ;
#71677=ORIENTED_EDGE('',*,*,#51174,.T.) ;
#71678=ORIENTED_EDGE('',*,*,#51175,.T.) ;
#71679=ORIENTED_EDGE('',*,*,#51176,.T.) ;
#71680=ORIENTED_EDGE('',*,*,#51177,.T.) ;
#71681=ORIENTED_EDGE('',*,*,#51178,.T.) ;
#71682=ORIENTED_EDGE('',*,*,#51179,.T.) ;
#71683=ORIENTED_EDGE('',*,*,#51180,.T.) ;
#71684=ORIENTED_EDGE('',*,*,#51181,.F.) ;
#71685=ORIENTED_EDGE('',*,*,#51182,.T.) ;
#71686=ORIENTED_EDGE('',*,*,#51183,.T.) ;
#71687=ORIENTED_EDGE('',*,*,#51184,.T.) ;
#71688=ORIENTED_EDGE('',*,*,#51185,.T.) ;
#71689=ORIENTED_EDGE('',*,*,#51186,.T.) ;
#71690=ORIENTED_EDGE('',*,*,#51187,.T.) ;
#71691=ORIENTED_EDGE('',*,*,#51188,.T.) ;
#71692=ORIENTED_EDGE('',*,*,#51189,.T.) ;
#71693=ORIENTED_EDGE('',*,*,#51190,.T.) ;
#71694=ORIENTED_EDGE('',*,*,#51191,.T.) ;
#71695=ORIENTED_EDGE('',*,*,#51192,.T.) ;
#71696=ORIENTED_EDGE('',*,*,#51193,.T.) ;
#71697=ORIENTED_EDGE('',*,*,#51194,.T.) ;
#71698=ORIENTED_EDGE('',*,*,#51195,.F.) ;
#71699=ORIENTED_EDGE('',*,*,#51196,.T.) ;
#71700=ORIENTED_EDGE('',*,*,#51197,.T.) ;
#71701=ORIENTED_EDGE('',*,*,#51198,.T.) ;
#71702=ORIENTED_EDGE('',*,*,#51199,.T.) ;
#71703=ORIENTED_EDGE('',*,*,#51200,.T.) ;
#71704=ORIENTED_EDGE('',*,*,#51201,.T.) ;
#71705=ORIENTED_EDGE('',*,*,#51202,.T.) ;
#71706=ORIENTED_EDGE('',*,*,#51203,.T.) ;
#71707=ORIENTED_EDGE('',*,*,#51204,.T.) ;
#71708=ORIENTED_EDGE('',*,*,#51205,.T.) ;
#71709=ORIENTED_EDGE('',*,*,#51206,.T.) ;
#71710=ORIENTED_EDGE('',*,*,#51207,.T.) ;
#71711=ORIENTED_EDGE('',*,*,#51208,.T.) ;
#71712=ORIENTED_EDGE('',*,*,#51209,.F.) ;
#71713=ORIENTED_EDGE('',*,*,#51210,.T.) ;
#71714=ORIENTED_EDGE('',*,*,#51211,.T.) ;
#71715=ORIENTED_EDGE('',*,*,#51212,.T.) ;
#71716=ORIENTED_EDGE('',*,*,#51213,.T.) ;
#71717=ORIENTED_EDGE('',*,*,#51214,.T.) ;
#71718=ORIENTED_EDGE('',*,*,#51215,.T.) ;
#71719=ORIENTED_EDGE('',*,*,#51216,.T.) ;
#71720=ORIENTED_EDGE('',*,*,#51217,.T.) ;
#71721=ORIENTED_EDGE('',*,*,#51218,.T.) ;
#71722=ORIENTED_EDGE('',*,*,#51219,.T.) ;
#71723=ORIENTED_EDGE('',*,*,#51220,.T.) ;
#71724=ORIENTED_EDGE('',*,*,#51221,.T.) ;
#71725=ORIENTED_EDGE('',*,*,#51222,.T.) ;
#71726=ORIENTED_EDGE('',*,*,#51223,.F.) ;
#71727=ORIENTED_EDGE('',*,*,#51224,.T.) ;
#71728=ORIENTED_EDGE('',*,*,#51225,.T.) ;
#71729=ORIENTED_EDGE('',*,*,#51226,.T.) ;
#71730=ORIENTED_EDGE('',*,*,#51227,.T.) ;
#71731=ORIENTED_EDGE('',*,*,#51228,.T.) ;
#71732=ORIENTED_EDGE('',*,*,#51229,.T.) ;
#71733=ORIENTED_EDGE('',*,*,#51230,.T.) ;
#71734=ORIENTED_EDGE('',*,*,#51231,.T.) ;
#71735=ORIENTED_EDGE('',*,*,#51232,.T.) ;
#71736=ORIENTED_EDGE('',*,*,#51233,.T.) ;
#71737=ORIENTED_EDGE('',*,*,#51234,.T.) ;
#71738=ORIENTED_EDGE('',*,*,#51235,.T.) ;
#71739=ORIENTED_EDGE('',*,*,#51236,.T.) ;
#71740=ORIENTED_EDGE('',*,*,#51237,.F.) ;
#71741=ORIENTED_EDGE('',*,*,#51238,.T.) ;
#71742=ORIENTED_EDGE('',*,*,#51239,.T.) ;
#71743=ORIENTED_EDGE('',*,*,#51240,.T.) ;
#71744=ORIENTED_EDGE('',*,*,#51241,.T.) ;
#71745=ORIENTED_EDGE('',*,*,#51242,.T.) ;
#71746=ORIENTED_EDGE('',*,*,#51243,.T.) ;
#71747=ORIENTED_EDGE('',*,*,#51244,.T.) ;
#71748=ORIENTED_EDGE('',*,*,#51245,.T.) ;
#71749=ORIENTED_EDGE('',*,*,#51246,.T.) ;
#71750=ORIENTED_EDGE('',*,*,#51247,.T.) ;
#71751=ORIENTED_EDGE('',*,*,#51248,.T.) ;
#71752=ORIENTED_EDGE('',*,*,#51249,.T.) ;
#71753=ORIENTED_EDGE('',*,*,#51250,.T.) ;
#71754=ORIENTED_EDGE('',*,*,#51251,.F.) ;
#71755=ORIENTED_EDGE('',*,*,#51252,.T.) ;
#71756=ORIENTED_EDGE('',*,*,#51253,.T.) ;
#71757=ORIENTED_EDGE('',*,*,#51254,.T.) ;
#71758=ORIENTED_EDGE('',*,*,#51255,.T.) ;
#71759=ORIENTED_EDGE('',*,*,#51256,.T.) ;
#71760=ORIENTED_EDGE('',*,*,#51257,.T.) ;
#71761=ORIENTED_EDGE('',*,*,#51258,.T.) ;
#71762=ORIENTED_EDGE('',*,*,#51259,.T.) ;
#71763=ORIENTED_EDGE('',*,*,#51260,.T.) ;
#71764=ORIENTED_EDGE('',*,*,#51261,.T.) ;
#71765=ORIENTED_EDGE('',*,*,#51262,.T.) ;
#71766=ORIENTED_EDGE('',*,*,#51263,.T.) ;
#71767=ORIENTED_EDGE('',*,*,#51264,.T.) ;
#71768=ORIENTED_EDGE('',*,*,#51265,.F.) ;
#71769=ORIENTED_EDGE('',*,*,#51266,.T.) ;
#71770=ORIENTED_EDGE('',*,*,#51267,.T.) ;
#71771=ORIENTED_EDGE('',*,*,#51268,.T.) ;
#71772=ORIENTED_EDGE('',*,*,#51269,.T.) ;
#71773=ORIENTED_EDGE('',*,*,#51270,.T.) ;
#71774=ORIENTED_EDGE('',*,*,#51271,.T.) ;
#71775=ORIENTED_EDGE('',*,*,#51272,.T.) ;
#71776=ORIENTED_EDGE('',*,*,#51273,.T.) ;
#71777=ORIENTED_EDGE('',*,*,#51274,.T.) ;
#71778=ORIENTED_EDGE('',*,*,#51275,.T.) ;
#71779=ORIENTED_EDGE('',*,*,#51276,.T.) ;
#71780=ORIENTED_EDGE('',*,*,#51277,.T.) ;
#71781=ORIENTED_EDGE('',*,*,#51278,.T.) ;
#71782=ORIENTED_EDGE('',*,*,#51279,.F.) ;
#71783=ORIENTED_EDGE('',*,*,#51280,.T.) ;
#71784=ORIENTED_EDGE('',*,*,#51281,.T.) ;
#71785=ORIENTED_EDGE('',*,*,#51282,.T.) ;
#71786=ORIENTED_EDGE('',*,*,#51283,.T.) ;
#71787=ORIENTED_EDGE('',*,*,#51284,.T.) ;
#71788=ORIENTED_EDGE('',*,*,#51285,.T.) ;
#71789=ORIENTED_EDGE('',*,*,#51286,.T.) ;
#71790=ORIENTED_EDGE('',*,*,#51287,.T.) ;
#71791=ORIENTED_EDGE('',*,*,#51288,.T.) ;
#71792=ORIENTED_EDGE('',*,*,#51289,.T.) ;
#71793=ORIENTED_EDGE('',*,*,#51290,.T.) ;
#71794=ORIENTED_EDGE('',*,*,#51291,.T.) ;
#71795=ORIENTED_EDGE('',*,*,#51292,.T.) ;
#71796=ORIENTED_EDGE('',*,*,#51293,.F.) ;
#71797=ORIENTED_EDGE('',*,*,#51294,.T.) ;
#71798=ORIENTED_EDGE('',*,*,#51295,.T.) ;
#71799=ORIENTED_EDGE('',*,*,#51296,.T.) ;
#71800=ORIENTED_EDGE('',*,*,#51297,.T.) ;
#71801=ORIENTED_EDGE('',*,*,#51298,.T.) ;
#71802=ORIENTED_EDGE('',*,*,#51299,.T.) ;
#71803=ORIENTED_EDGE('',*,*,#51300,.T.) ;
#71804=ORIENTED_EDGE('',*,*,#51301,.T.) ;
#71805=ORIENTED_EDGE('',*,*,#51302,.T.) ;
#71806=ORIENTED_EDGE('',*,*,#51303,.T.) ;
#71807=ORIENTED_EDGE('',*,*,#51304,.T.) ;
#71808=ORIENTED_EDGE('',*,*,#51305,.T.) ;
#71809=ORIENTED_EDGE('',*,*,#51306,.T.) ;
#71810=ORIENTED_EDGE('',*,*,#51307,.F.) ;
#71811=ORIENTED_EDGE('',*,*,#51308,.T.) ;
#71812=ORIENTED_EDGE('',*,*,#51309,.T.) ;
#71813=ORIENTED_EDGE('',*,*,#51310,.T.) ;
#71814=ORIENTED_EDGE('',*,*,#51311,.T.) ;
#71815=ORIENTED_EDGE('',*,*,#51312,.T.) ;
#71816=ORIENTED_EDGE('',*,*,#51313,.T.) ;
#71817=ORIENTED_EDGE('',*,*,#51314,.T.) ;
#71818=ORIENTED_EDGE('',*,*,#51315,.T.) ;
#71819=ORIENTED_EDGE('',*,*,#51316,.T.) ;
#71820=ORIENTED_EDGE('',*,*,#51317,.T.) ;
#71821=ORIENTED_EDGE('',*,*,#51318,.T.) ;
#71822=ORIENTED_EDGE('',*,*,#51319,.T.) ;
#71823=ORIENTED_EDGE('',*,*,#51320,.T.) ;
#71824=ORIENTED_EDGE('',*,*,#51321,.F.) ;
#71825=ORIENTED_EDGE('',*,*,#51322,.T.) ;
#71826=ORIENTED_EDGE('',*,*,#51323,.T.) ;
#71827=ORIENTED_EDGE('',*,*,#51324,.T.) ;
#71828=ORIENTED_EDGE('',*,*,#51325,.T.) ;
#71829=ORIENTED_EDGE('',*,*,#51326,.T.) ;
#71830=ORIENTED_EDGE('',*,*,#51327,.T.) ;
#71831=ORIENTED_EDGE('',*,*,#51328,.T.) ;
#71832=ORIENTED_EDGE('',*,*,#51329,.T.) ;
#71833=ORIENTED_EDGE('',*,*,#51330,.T.) ;
#71834=ORIENTED_EDGE('',*,*,#51331,.T.) ;
#71835=ORIENTED_EDGE('',*,*,#51332,.T.) ;
#71836=ORIENTED_EDGE('',*,*,#51333,.T.) ;
#71837=ORIENTED_EDGE('',*,*,#51334,.T.) ;
#71838=ORIENTED_EDGE('',*,*,#51335,.T.) ;
#71839=ORIENTED_EDGE('',*,*,#51336,.T.) ;
#71840=ORIENTED_EDGE('',*,*,#51337,.T.) ;
#71841=ORIENTED_EDGE('',*,*,#51338,.T.) ;
#71842=ORIENTED_EDGE('',*,*,#51339,.T.) ;
#71843=ORIENTED_EDGE('',*,*,#51340,.T.) ;
#71844=ORIENTED_EDGE('',*,*,#51341,.T.) ;
#71845=ORIENTED_EDGE('',*,*,#51342,.T.) ;
#71846=ORIENTED_EDGE('',*,*,#51343,.T.) ;
#71847=ORIENTED_EDGE('',*,*,#51344,.T.) ;
#71848=ORIENTED_EDGE('',*,*,#51345,.T.) ;
#71849=ORIENTED_EDGE('',*,*,#51346,.T.) ;
#71850=ORIENTED_EDGE('',*,*,#49086,.T.) ;
#71851=ORIENTED_EDGE('',*,*,#51347,.T.) ;
#71852=ORIENTED_EDGE('',*,*,#51348,.T.) ;
#71853=ORIENTED_EDGE('',*,*,#51349,.T.) ;
#71854=ORIENTED_EDGE('',*,*,#51350,.T.) ;
#71855=ORIENTED_EDGE('',*,*,#51351,.T.) ;
#71856=ORIENTED_EDGE('',*,*,#51352,.T.) ;
#71857=ORIENTED_EDGE('',*,*,#51353,.T.) ;
#71858=ORIENTED_EDGE('',*,*,#51354,.T.) ;
#71859=ORIENTED_EDGE('',*,*,#51355,.T.) ;
#71860=ORIENTED_EDGE('',*,*,#51356,.T.) ;
#71861=ORIENTED_EDGE('',*,*,#51357,.T.) ;
#71862=ORIENTED_EDGE('',*,*,#51358,.T.) ;
#71863=ORIENTED_EDGE('',*,*,#51359,.T.) ;
#71864=ORIENTED_EDGE('',*,*,#51360,.T.) ;
#71865=ORIENTED_EDGE('',*,*,#51361,.T.) ;
#71866=ORIENTED_EDGE('',*,*,#51362,.T.) ;
#71867=ORIENTED_EDGE('',*,*,#51363,.T.) ;
#71868=ORIENTED_EDGE('',*,*,#51364,.T.) ;
#71869=ORIENTED_EDGE('',*,*,#49077,.T.) ;
#71870=ORIENTED_EDGE('',*,*,#51365,.T.) ;
#71871=ORIENTED_EDGE('',*,*,#51366,.T.) ;
#71872=ORIENTED_EDGE('',*,*,#51367,.T.) ;
#71873=ORIENTED_EDGE('',*,*,#51368,.T.) ;
#71874=ORIENTED_EDGE('',*,*,#51369,.T.) ;
#71875=ORIENTED_EDGE('',*,*,#51370,.T.) ;
#71876=ORIENTED_EDGE('',*,*,#51371,.T.) ;
#71877=ORIENTED_EDGE('',*,*,#51372,.T.) ;
#71878=ORIENTED_EDGE('',*,*,#51373,.T.) ;
#71879=ORIENTED_EDGE('',*,*,#51374,.T.) ;
#71880=ORIENTED_EDGE('',*,*,#51375,.T.) ;
#71881=ORIENTED_EDGE('',*,*,#51376,.T.) ;
#71882=ORIENTED_EDGE('',*,*,#51377,.T.) ;
#71883=ORIENTED_EDGE('',*,*,#51378,.T.) ;
#71884=ORIENTED_EDGE('',*,*,#51379,.T.) ;
#71885=ORIENTED_EDGE('',*,*,#51380,.T.) ;
#71886=ORIENTED_EDGE('',*,*,#51381,.T.) ;
#71887=ORIENTED_EDGE('',*,*,#51382,.T.) ;
#71888=ORIENTED_EDGE('',*,*,#49068,.T.) ;
#71889=ORIENTED_EDGE('',*,*,#51383,.T.) ;
#71890=ORIENTED_EDGE('',*,*,#51384,.T.) ;
#71891=ORIENTED_EDGE('',*,*,#51385,.T.) ;
#71892=ORIENTED_EDGE('',*,*,#51386,.T.) ;
#71893=ORIENTED_EDGE('',*,*,#51387,.T.) ;
#71894=ORIENTED_EDGE('',*,*,#51388,.T.) ;
#71895=ORIENTED_EDGE('',*,*,#51389,.T.) ;
#71896=ORIENTED_EDGE('',*,*,#51390,.T.) ;
#71897=ORIENTED_EDGE('',*,*,#51391,.T.) ;
#71898=ORIENTED_EDGE('',*,*,#51392,.T.) ;
#71899=ORIENTED_EDGE('',*,*,#51393,.T.) ;
#71900=ORIENTED_EDGE('',*,*,#51394,.T.) ;
#71901=ORIENTED_EDGE('',*,*,#51395,.T.) ;
#71902=ORIENTED_EDGE('',*,*,#51396,.T.) ;
#71903=ORIENTED_EDGE('',*,*,#51397,.T.) ;
#71904=ORIENTED_EDGE('',*,*,#51398,.T.) ;
#71905=ORIENTED_EDGE('',*,*,#51399,.T.) ;
#71906=ORIENTED_EDGE('',*,*,#51400,.T.) ;
#71907=ORIENTED_EDGE('',*,*,#49059,.T.) ;
#71908=ORIENTED_EDGE('',*,*,#51401,.T.) ;
#71909=ORIENTED_EDGE('',*,*,#51402,.T.) ;
#71910=ORIENTED_EDGE('',*,*,#51403,.T.) ;
#71911=ORIENTED_EDGE('',*,*,#51404,.T.) ;
#71912=ORIENTED_EDGE('',*,*,#51405,.T.) ;
#71913=ORIENTED_EDGE('',*,*,#51406,.T.) ;
#71914=ORIENTED_EDGE('',*,*,#51407,.T.) ;
#71915=ORIENTED_EDGE('',*,*,#51408,.T.) ;
#71916=ORIENTED_EDGE('',*,*,#51409,.T.) ;
#71917=ORIENTED_EDGE('',*,*,#51410,.T.) ;
#71918=ORIENTED_EDGE('',*,*,#51411,.T.) ;
#71919=ORIENTED_EDGE('',*,*,#51412,.T.) ;
#71920=ORIENTED_EDGE('',*,*,#51413,.T.) ;
#71921=ORIENTED_EDGE('',*,*,#51414,.T.) ;
#71922=ORIENTED_EDGE('',*,*,#51415,.T.) ;
#71923=ORIENTED_EDGE('',*,*,#51416,.T.) ;
#71924=ORIENTED_EDGE('',*,*,#51417,.T.) ;
#71925=ORIENTED_EDGE('',*,*,#51418,.T.) ;
#71926=ORIENTED_EDGE('',*,*,#49050,.T.) ;
#71927=ORIENTED_EDGE('',*,*,#51419,.T.) ;
#71928=ORIENTED_EDGE('',*,*,#51420,.T.) ;
#71929=ORIENTED_EDGE('',*,*,#51421,.T.) ;
#71930=ORIENTED_EDGE('',*,*,#51422,.T.) ;
#71931=ORIENTED_EDGE('',*,*,#51423,.T.) ;
#71932=ORIENTED_EDGE('',*,*,#51424,.T.) ;
#71933=ORIENTED_EDGE('',*,*,#51425,.T.) ;
#71934=ORIENTED_EDGE('',*,*,#51426,.T.) ;
#71935=ORIENTED_EDGE('',*,*,#51427,.T.) ;
#71936=ORIENTED_EDGE('',*,*,#51428,.T.) ;
#71937=ORIENTED_EDGE('',*,*,#51429,.T.) ;
#71938=ORIENTED_EDGE('',*,*,#51430,.T.) ;
#71939=ORIENTED_EDGE('',*,*,#51431,.T.) ;
#71940=ORIENTED_EDGE('',*,*,#51432,.T.) ;
#71941=ORIENTED_EDGE('',*,*,#51433,.T.) ;
#71942=ORIENTED_EDGE('',*,*,#51434,.T.) ;
#71943=ORIENTED_EDGE('',*,*,#51435,.T.) ;
#71944=ORIENTED_EDGE('',*,*,#51436,.T.) ;
#71945=ORIENTED_EDGE('',*,*,#49041,.T.) ;
#71946=ORIENTED_EDGE('',*,*,#51437,.T.) ;
#71947=ORIENTED_EDGE('',*,*,#51438,.T.) ;
#71948=ORIENTED_EDGE('',*,*,#51439,.T.) ;
#71949=ORIENTED_EDGE('',*,*,#51440,.T.) ;
#71950=ORIENTED_EDGE('',*,*,#51441,.T.) ;
#71951=ORIENTED_EDGE('',*,*,#51442,.T.) ;
#71952=ORIENTED_EDGE('',*,*,#51443,.T.) ;
#71953=ORIENTED_EDGE('',*,*,#51444,.T.) ;
#71954=ORIENTED_EDGE('',*,*,#51445,.T.) ;
#71955=ORIENTED_EDGE('',*,*,#51446,.T.) ;
#71956=ORIENTED_EDGE('',*,*,#51447,.T.) ;
#71957=ORIENTED_EDGE('',*,*,#51448,.T.) ;
#71958=ORIENTED_EDGE('',*,*,#51449,.T.) ;
#71959=ORIENTED_EDGE('',*,*,#51450,.T.) ;
#71960=ORIENTED_EDGE('',*,*,#51451,.T.) ;
#71961=ORIENTED_EDGE('',*,*,#51452,.T.) ;
#71962=ORIENTED_EDGE('',*,*,#51453,.T.) ;
#71963=ORIENTED_EDGE('',*,*,#51454,.T.) ;
#71964=ORIENTED_EDGE('',*,*,#49032,.T.) ;
#71965=ORIENTED_EDGE('',*,*,#51455,.T.) ;
#71966=ORIENTED_EDGE('',*,*,#51456,.T.) ;
#71967=ORIENTED_EDGE('',*,*,#51457,.T.) ;
#71968=ORIENTED_EDGE('',*,*,#51458,.T.) ;
#71969=ORIENTED_EDGE('',*,*,#51459,.T.) ;
#71970=ORIENTED_EDGE('',*,*,#51460,.T.) ;
#71971=ORIENTED_EDGE('',*,*,#51461,.T.) ;
#71972=ORIENTED_EDGE('',*,*,#51462,.T.) ;
#71973=ORIENTED_EDGE('',*,*,#51463,.T.) ;
#71974=ORIENTED_EDGE('',*,*,#51464,.T.) ;
#71975=ORIENTED_EDGE('',*,*,#51465,.T.) ;
#71976=ORIENTED_EDGE('',*,*,#51466,.T.) ;
#71977=ORIENTED_EDGE('',*,*,#51467,.T.) ;
#71978=ORIENTED_EDGE('',*,*,#51468,.T.) ;
#71979=ORIENTED_EDGE('',*,*,#51469,.T.) ;
#71980=ORIENTED_EDGE('',*,*,#51470,.T.) ;
#71981=ORIENTED_EDGE('',*,*,#51471,.T.) ;
#71982=ORIENTED_EDGE('',*,*,#51472,.T.) ;
#71983=ORIENTED_EDGE('',*,*,#49023,.T.) ;
#71984=ORIENTED_EDGE('',*,*,#51473,.T.) ;
#71985=ORIENTED_EDGE('',*,*,#51474,.T.) ;
#71986=ORIENTED_EDGE('',*,*,#51475,.T.) ;
#71987=ORIENTED_EDGE('',*,*,#51476,.T.) ;
#71988=ORIENTED_EDGE('',*,*,#51477,.T.) ;
#71989=ORIENTED_EDGE('',*,*,#51478,.T.) ;
#71990=ORIENTED_EDGE('',*,*,#51479,.T.) ;
#71991=ORIENTED_EDGE('',*,*,#51480,.T.) ;
#71992=ORIENTED_EDGE('',*,*,#51481,.T.) ;
#71993=ORIENTED_EDGE('',*,*,#51482,.T.) ;
#71994=ORIENTED_EDGE('',*,*,#51483,.T.) ;
#71995=ORIENTED_EDGE('',*,*,#51484,.T.) ;
#71996=ORIENTED_EDGE('',*,*,#51485,.T.) ;
#71997=ORIENTED_EDGE('',*,*,#51486,.T.) ;
#71998=ORIENTED_EDGE('',*,*,#51487,.T.) ;
#71999=ORIENTED_EDGE('',*,*,#51488,.T.) ;
#72000=ORIENTED_EDGE('',*,*,#51489,.T.) ;
#72001=ORIENTED_EDGE('',*,*,#51490,.T.) ;
#72002=ORIENTED_EDGE('',*,*,#49014,.T.) ;
#72003=ORIENTED_EDGE('',*,*,#49265,.T.) ;
#72004=ORIENTED_EDGE('',*,*,#49263,.T.) ;
#72005=ORIENTED_EDGE('',*,*,#49261,.T.) ;
#72006=ORIENTED_EDGE('',*,*,#49259,.T.) ;
#72007=ORIENTED_EDGE('',*,*,#49257,.T.) ;
#72008=ORIENTED_EDGE('',*,*,#49255,.T.) ;
#72009=ORIENTED_EDGE('',*,*,#49253,.T.) ;
#72010=ORIENTED_EDGE('',*,*,#49251,.T.) ;
#72011=ORIENTED_EDGE('',*,*,#49249,.T.) ;
#72012=ORIENTED_EDGE('',*,*,#51491,.T.) ;
#72013=ORIENTED_EDGE('',*,*,#51492,.T.) ;
#72014=ORIENTED_EDGE('',*,*,#51493,.T.) ;
#72015=ORIENTED_EDGE('',*,*,#51494,.T.) ;
#72016=ORIENTED_EDGE('',*,*,#51495,.T.) ;
#72017=ORIENTED_EDGE('',*,*,#51496,.T.) ;
#72018=ORIENTED_EDGE('',*,*,#51497,.T.) ;
#72019=ORIENTED_EDGE('',*,*,#51498,.T.) ;
#72020=ORIENTED_EDGE('',*,*,#51499,.T.) ;
#72021=ORIENTED_EDGE('',*,*,#51500,.T.) ;
#72022=ORIENTED_EDGE('',*,*,#51501,.T.) ;
#72023=ORIENTED_EDGE('',*,*,#51502,.T.) ;
#72024=ORIENTED_EDGE('',*,*,#51503,.T.) ;
#72025=ORIENTED_EDGE('',*,*,#51504,.T.) ;
#72026=ORIENTED_EDGE('',*,*,#51505,.T.) ;
#72027=ORIENTED_EDGE('',*,*,#51506,.T.) ;
#72028=ORIENTED_EDGE('',*,*,#51507,.T.) ;
#72029=ORIENTED_EDGE('',*,*,#51508,.T.) ;
#72030=ORIENTED_EDGE('',*,*,#51509,.T.) ;
#72031=ORIENTED_EDGE('',*,*,#51510,.T.) ;
#72032=ORIENTED_EDGE('',*,*,#51511,.T.) ;
#72033=ORIENTED_EDGE('',*,*,#51512,.T.) ;
#72034=ORIENTED_EDGE('',*,*,#51513,.T.) ;
#72035=ORIENTED_EDGE('',*,*,#51514,.T.) ;
#72036=ORIENTED_EDGE('',*,*,#51515,.T.) ;
#72037=ORIENTED_EDGE('',*,*,#51516,.T.) ;
#72038=ORIENTED_EDGE('',*,*,#51517,.T.) ;
#72039=ORIENTED_EDGE('',*,*,#51518,.T.) ;
#72040=ORIENTED_EDGE('',*,*,#51519,.T.) ;
#72041=ORIENTED_EDGE('',*,*,#51520,.T.) ;
#72042=ORIENTED_EDGE('',*,*,#51521,.T.) ;
#72043=ORIENTED_EDGE('',*,*,#51522,.T.) ;
#72044=ORIENTED_EDGE('',*,*,#51523,.T.) ;
#72045=ORIENTED_EDGE('',*,*,#51524,.T.) ;
#72046=ORIENTED_EDGE('',*,*,#51525,.T.) ;
#72047=ORIENTED_EDGE('',*,*,#51526,.T.) ;
#72048=ORIENTED_EDGE('',*,*,#51527,.T.) ;
#72049=ORIENTED_EDGE('',*,*,#51528,.T.) ;
#72050=ORIENTED_EDGE('',*,*,#51529,.T.) ;
#72051=ORIENTED_EDGE('',*,*,#51530,.T.) ;
#72052=ORIENTED_EDGE('',*,*,#51531,.T.) ;
#72053=ORIENTED_EDGE('',*,*,#51532,.T.) ;
#72054=ORIENTED_EDGE('',*,*,#51533,.T.) ;
#72055=ORIENTED_EDGE('',*,*,#51534,.T.) ;
#72056=ORIENTED_EDGE('',*,*,#51535,.T.) ;
#72057=ORIENTED_EDGE('',*,*,#51536,.T.) ;
#72058=ORIENTED_EDGE('',*,*,#51537,.T.) ;
#72059=ORIENTED_EDGE('',*,*,#51538,.T.) ;
#72060=ORIENTED_EDGE('',*,*,#51539,.T.) ;
#72061=ORIENTED_EDGE('',*,*,#51540,.T.) ;
#72062=ORIENTED_EDGE('',*,*,#51541,.T.) ;
#72063=ORIENTED_EDGE('',*,*,#51542,.T.) ;
#72064=ORIENTED_EDGE('',*,*,#51543,.T.) ;
#72065=ORIENTED_EDGE('',*,*,#51544,.T.) ;
#72066=ORIENTED_EDGE('',*,*,#51545,.T.) ;
#72067=ORIENTED_EDGE('',*,*,#51546,.T.) ;
#72068=ORIENTED_EDGE('',*,*,#51547,.T.) ;
#72069=ORIENTED_EDGE('',*,*,#51548,.T.) ;
#72070=ORIENTED_EDGE('',*,*,#51549,.T.) ;
#72071=ORIENTED_EDGE('',*,*,#51550,.T.) ;
#72072=ORIENTED_EDGE('',*,*,#51551,.T.) ;
#72073=ORIENTED_EDGE('',*,*,#51552,.T.) ;
#72074=ORIENTED_EDGE('',*,*,#51553,.T.) ;
#72075=ORIENTED_EDGE('',*,*,#51554,.T.) ;
#72076=ORIENTED_EDGE('',*,*,#51555,.T.) ;
#72077=ORIENTED_EDGE('',*,*,#51556,.T.) ;
#72078=ORIENTED_EDGE('',*,*,#51557,.T.) ;
#72079=ORIENTED_EDGE('',*,*,#51558,.T.) ;
#72080=ORIENTED_EDGE('',*,*,#51559,.T.) ;
#72081=ORIENTED_EDGE('',*,*,#51560,.T.) ;
#72082=ORIENTED_EDGE('',*,*,#51561,.T.) ;
#72083=ORIENTED_EDGE('',*,*,#51562,.T.) ;
#72084=ORIENTED_EDGE('',*,*,#51563,.T.) ;
#72085=ORIENTED_EDGE('',*,*,#51564,.T.) ;
#72086=ORIENTED_EDGE('',*,*,#51565,.T.) ;
#72087=ORIENTED_EDGE('',*,*,#51566,.T.) ;
#72088=ORIENTED_EDGE('',*,*,#51567,.T.) ;
#72089=ORIENTED_EDGE('',*,*,#51568,.T.) ;
#72090=ORIENTED_EDGE('',*,*,#51569,.T.) ;
#72091=ORIENTED_EDGE('',*,*,#51570,.T.) ;
#72092=ORIENTED_EDGE('',*,*,#51571,.T.) ;
#72093=ORIENTED_EDGE('',*,*,#51572,.T.) ;
#72094=ORIENTED_EDGE('',*,*,#51573,.T.) ;
#72095=ORIENTED_EDGE('',*,*,#51574,.T.) ;
#72096=ORIENTED_EDGE('',*,*,#51575,.T.) ;
#72097=ORIENTED_EDGE('',*,*,#51576,.T.) ;
#72098=ORIENTED_EDGE('',*,*,#51577,.T.) ;
#72099=ORIENTED_EDGE('',*,*,#51578,.T.) ;
#72100=ORIENTED_EDGE('',*,*,#51579,.T.) ;
#72101=ORIENTED_EDGE('',*,*,#51580,.T.) ;
#72102=ORIENTED_EDGE('',*,*,#51581,.T.) ;
#72103=ORIENTED_EDGE('',*,*,#51582,.T.) ;
#72104=ORIENTED_EDGE('',*,*,#51583,.T.) ;
#72105=ORIENTED_EDGE('',*,*,#51584,.T.) ;
#72106=ORIENTED_EDGE('',*,*,#51585,.T.) ;
#72107=ORIENTED_EDGE('',*,*,#51586,.T.) ;
#72108=ORIENTED_EDGE('',*,*,#51587,.T.) ;
#72109=ORIENTED_EDGE('',*,*,#51588,.T.) ;
#72110=ORIENTED_EDGE('',*,*,#51589,.T.) ;
#72111=ORIENTED_EDGE('',*,*,#51590,.T.) ;
#72112=ORIENTED_EDGE('',*,*,#51591,.T.) ;
#72113=ORIENTED_EDGE('',*,*,#51592,.T.) ;
#72114=ORIENTED_EDGE('',*,*,#51593,.T.) ;
#72115=ORIENTED_EDGE('',*,*,#51594,.T.) ;
#72116=ORIENTED_EDGE('',*,*,#51595,.T.) ;
#72117=ORIENTED_EDGE('',*,*,#51596,.T.) ;
#72118=ORIENTED_EDGE('',*,*,#51597,.T.) ;
#72119=ORIENTED_EDGE('',*,*,#51598,.T.) ;
#72120=ORIENTED_EDGE('',*,*,#51599,.T.) ;
#72121=ORIENTED_EDGE('',*,*,#51600,.T.) ;
#72122=ORIENTED_EDGE('',*,*,#51601,.T.) ;
#72123=ORIENTED_EDGE('',*,*,#51602,.T.) ;
#72124=ORIENTED_EDGE('',*,*,#51603,.T.) ;
#72125=ORIENTED_EDGE('',*,*,#51604,.T.) ;
#72126=ORIENTED_EDGE('',*,*,#51605,.T.) ;
#72127=ORIENTED_EDGE('',*,*,#51606,.T.) ;
#72128=ORIENTED_EDGE('',*,*,#51607,.T.) ;
#72129=ORIENTED_EDGE('',*,*,#51608,.T.) ;
#72130=ORIENTED_EDGE('',*,*,#51609,.T.) ;
#72131=ORIENTED_EDGE('',*,*,#51610,.T.) ;
#72132=ORIENTED_EDGE('',*,*,#51611,.T.) ;
#72133=ORIENTED_EDGE('',*,*,#51612,.T.) ;
#72134=ORIENTED_EDGE('',*,*,#51613,.T.) ;
#72135=ORIENTED_EDGE('',*,*,#51614,.T.) ;
#72136=ORIENTED_EDGE('',*,*,#51615,.T.) ;
#72137=ORIENTED_EDGE('',*,*,#51616,.T.) ;
#72138=ORIENTED_EDGE('',*,*,#51617,.T.) ;
#72139=ORIENTED_EDGE('',*,*,#51618,.T.) ;
#72140=ORIENTED_EDGE('',*,*,#51619,.T.) ;
#72141=ORIENTED_EDGE('',*,*,#51620,.T.) ;
#72142=ORIENTED_EDGE('',*,*,#51621,.T.) ;
#72143=ORIENTED_EDGE('',*,*,#51622,.T.) ;
#72144=ORIENTED_EDGE('',*,*,#51623,.T.) ;
#72145=ORIENTED_EDGE('',*,*,#51624,.T.) ;
#72146=ORIENTED_EDGE('',*,*,#51625,.T.) ;
#72147=ORIENTED_EDGE('',*,*,#51626,.T.) ;
#72148=ORIENTED_EDGE('',*,*,#51627,.T.) ;
#72149=ORIENTED_EDGE('',*,*,#51628,.T.) ;
#72150=ORIENTED_EDGE('',*,*,#51629,.T.) ;
#72151=ORIENTED_EDGE('',*,*,#51630,.T.) ;
#72152=ORIENTED_EDGE('',*,*,#51631,.T.) ;
#72153=ORIENTED_EDGE('',*,*,#51632,.T.) ;
#72154=ORIENTED_EDGE('',*,*,#51633,.T.) ;
#72155=ORIENTED_EDGE('',*,*,#51634,.T.) ;
#72156=ORIENTED_EDGE('',*,*,#51635,.T.) ;
#72157=ORIENTED_EDGE('',*,*,#51636,.T.) ;
#72158=ORIENTED_EDGE('',*,*,#51637,.T.) ;
#72159=ORIENTED_EDGE('',*,*,#51638,.T.) ;
#72160=ORIENTED_EDGE('',*,*,#51639,.F.) ;
#72161=ORIENTED_EDGE('',*,*,#51640,.T.) ;
#72162=ORIENTED_EDGE('',*,*,#51641,.F.) ;
#72163=ORIENTED_EDGE('',*,*,#51642,.T.) ;
#72164=ORIENTED_EDGE('',*,*,#51643,.F.) ;
#72165=ORIENTED_EDGE('',*,*,#51644,.T.) ;
#72166=ORIENTED_EDGE('',*,*,#51645,.F.) ;
#72167=ORIENTED_EDGE('',*,*,#51646,.T.) ;
#72168=ORIENTED_EDGE('',*,*,#51647,.T.) ;
#72169=ORIENTED_EDGE('',*,*,#51648,.T.) ;
#72170=ORIENTED_EDGE('',*,*,#51645,.T.) ;
#72171=ORIENTED_EDGE('',*,*,#51649,.T.) ;
#72172=ORIENTED_EDGE('',*,*,#51650,.T.) ;
#72173=ORIENTED_EDGE('',*,*,#51651,.T.) ;
#72174=ORIENTED_EDGE('',*,*,#51639,.T.) ;
#72175=ORIENTED_EDGE('',*,*,#51652,.T.) ;
#72176=ORIENTED_EDGE('',*,*,#51641,.T.) ;
#72177=ORIENTED_EDGE('',*,*,#51653,.T.) ;
#72178=ORIENTED_EDGE('',*,*,#51654,.T.) ;
#72179=ORIENTED_EDGE('',*,*,#51655,.T.) ;
#72180=ORIENTED_EDGE('',*,*,#51656,.T.) ;
#72181=ORIENTED_EDGE('',*,*,#51657,.T.) ;
#72182=ORIENTED_EDGE('',*,*,#51643,.T.) ;
#72183=ORIENTED_EDGE('',*,*,#51658,.T.) ;
#72184=ORIENTED_EDGE('',*,*,#51659,.T.) ;
#72185=ORIENTED_EDGE('',*,*,#51660,.T.) ;
#72186=ORIENTED_EDGE('',*,*,#51661,.T.) ;
#72187=ORIENTED_EDGE('',*,*,#51662,.T.) ;
#72188=ORIENTED_EDGE('',*,*,#51663,.F.) ;
#72189=ORIENTED_EDGE('',*,*,#51664,.T.) ;
#72190=ORIENTED_EDGE('',*,*,#51665,.F.) ;
#72191=ORIENTED_EDGE('',*,*,#51666,.T.) ;
#72192=ORIENTED_EDGE('',*,*,#51667,.F.) ;
#72193=ORIENTED_EDGE('',*,*,#51668,.T.) ;
#72194=ORIENTED_EDGE('',*,*,#51669,.F.) ;
#72195=ORIENTED_EDGE('',*,*,#51670,.T.) ;
#72196=ORIENTED_EDGE('',*,*,#51671,.T.) ;
#72197=ORIENTED_EDGE('',*,*,#51672,.T.) ;
#72198=ORIENTED_EDGE('',*,*,#51669,.T.) ;
#72199=ORIENTED_EDGE('',*,*,#51673,.T.) ;
#72200=ORIENTED_EDGE('',*,*,#51674,.T.) ;
#72201=ORIENTED_EDGE('',*,*,#51675,.T.) ;
#72202=ORIENTED_EDGE('',*,*,#51663,.T.) ;
#72203=ORIENTED_EDGE('',*,*,#51676,.T.) ;
#72204=ORIENTED_EDGE('',*,*,#51665,.T.) ;
#72205=ORIENTED_EDGE('',*,*,#51677,.T.) ;
#72206=ORIENTED_EDGE('',*,*,#51678,.T.) ;
#72207=ORIENTED_EDGE('',*,*,#51679,.T.) ;
#72208=ORIENTED_EDGE('',*,*,#51680,.T.) ;
#72209=ORIENTED_EDGE('',*,*,#51681,.T.) ;
#72210=ORIENTED_EDGE('',*,*,#51667,.T.) ;
#72211=ORIENTED_EDGE('',*,*,#51682,.T.) ;
#72212=ORIENTED_EDGE('',*,*,#51683,.T.) ;
#72213=ORIENTED_EDGE('',*,*,#51684,.T.) ;
#72214=ORIENTED_EDGE('',*,*,#51685,.T.) ;
#72215=ORIENTED_EDGE('',*,*,#51686,.T.) ;
#72216=ORIENTED_EDGE('',*,*,#51687,.F.) ;
#72217=ORIENTED_EDGE('',*,*,#51688,.T.) ;
#72218=ORIENTED_EDGE('',*,*,#51689,.F.) ;
#72219=ORIENTED_EDGE('',*,*,#51690,.T.) ;
#72220=ORIENTED_EDGE('',*,*,#51691,.F.) ;
#72221=ORIENTED_EDGE('',*,*,#51692,.T.) ;
#72222=ORIENTED_EDGE('',*,*,#51693,.F.) ;
#72223=ORIENTED_EDGE('',*,*,#51694,.T.) ;
#72224=ORIENTED_EDGE('',*,*,#51695,.T.) ;
#72225=ORIENTED_EDGE('',*,*,#51696,.T.) ;
#72226=ORIENTED_EDGE('',*,*,#51693,.T.) ;
#72227=ORIENTED_EDGE('',*,*,#51697,.T.) ;
#72228=ORIENTED_EDGE('',*,*,#51698,.T.) ;
#72229=ORIENTED_EDGE('',*,*,#51699,.T.) ;
#72230=ORIENTED_EDGE('',*,*,#51687,.T.) ;
#72231=ORIENTED_EDGE('',*,*,#51700,.T.) ;
#72232=ORIENTED_EDGE('',*,*,#51689,.T.) ;
#72233=ORIENTED_EDGE('',*,*,#51701,.T.) ;
#72234=ORIENTED_EDGE('',*,*,#51702,.T.) ;
#72235=ORIENTED_EDGE('',*,*,#51703,.T.) ;
#72236=ORIENTED_EDGE('',*,*,#51704,.T.) ;
#72237=ORIENTED_EDGE('',*,*,#51705,.T.) ;
#72238=ORIENTED_EDGE('',*,*,#51691,.T.) ;
#72239=ORIENTED_EDGE('',*,*,#51706,.T.) ;
#72240=ORIENTED_EDGE('',*,*,#51707,.T.) ;
#72241=ORIENTED_EDGE('',*,*,#51708,.T.) ;
#72242=ORIENTED_EDGE('',*,*,#51709,.T.) ;
#72243=ORIENTED_EDGE('',*,*,#51710,.T.) ;
#72244=ORIENTED_EDGE('',*,*,#51711,.F.) ;
#72245=ORIENTED_EDGE('',*,*,#51712,.T.) ;
#72246=ORIENTED_EDGE('',*,*,#51713,.F.) ;
#72247=ORIENTED_EDGE('',*,*,#51714,.T.) ;
#72248=ORIENTED_EDGE('',*,*,#51715,.F.) ;
#72249=ORIENTED_EDGE('',*,*,#51716,.T.) ;
#72250=ORIENTED_EDGE('',*,*,#51717,.F.) ;
#72251=ORIENTED_EDGE('',*,*,#51718,.T.) ;
#72252=ORIENTED_EDGE('',*,*,#51719,.T.) ;
#72253=ORIENTED_EDGE('',*,*,#51720,.T.) ;
#72254=ORIENTED_EDGE('',*,*,#51717,.T.) ;
#72255=ORIENTED_EDGE('',*,*,#51721,.T.) ;
#72256=ORIENTED_EDGE('',*,*,#51722,.T.) ;
#72257=ORIENTED_EDGE('',*,*,#51723,.T.) ;
#72258=ORIENTED_EDGE('',*,*,#51711,.T.) ;
#72259=ORIENTED_EDGE('',*,*,#51724,.T.) ;
#72260=ORIENTED_EDGE('',*,*,#51713,.T.) ;
#72261=ORIENTED_EDGE('',*,*,#51725,.T.) ;
#72262=ORIENTED_EDGE('',*,*,#51726,.T.) ;
#72263=ORIENTED_EDGE('',*,*,#51727,.T.) ;
#72264=ORIENTED_EDGE('',*,*,#51728,.T.) ;
#72265=ORIENTED_EDGE('',*,*,#51729,.T.) ;
#72266=ORIENTED_EDGE('',*,*,#51715,.T.) ;
#72267=ORIENTED_EDGE('',*,*,#51730,.T.) ;
#72268=ORIENTED_EDGE('',*,*,#51731,.T.) ;
#72269=ORIENTED_EDGE('',*,*,#51732,.T.) ;
#72270=ORIENTED_EDGE('',*,*,#51733,.T.) ;
#72271=ORIENTED_EDGE('',*,*,#51734,.T.) ;
#72272=ORIENTED_EDGE('',*,*,#51735,.F.) ;
#72273=ORIENTED_EDGE('',*,*,#51736,.T.) ;
#72274=ORIENTED_EDGE('',*,*,#51737,.F.) ;
#72275=ORIENTED_EDGE('',*,*,#51738,.T.) ;
#72276=ORIENTED_EDGE('',*,*,#51739,.F.) ;
#72277=ORIENTED_EDGE('',*,*,#51740,.T.) ;
#72278=ORIENTED_EDGE('',*,*,#51741,.F.) ;
#72279=ORIENTED_EDGE('',*,*,#51742,.T.) ;
#72280=ORIENTED_EDGE('',*,*,#51743,.T.) ;
#72281=ORIENTED_EDGE('',*,*,#51744,.T.) ;
#72282=ORIENTED_EDGE('',*,*,#51741,.T.) ;
#72283=ORIENTED_EDGE('',*,*,#51745,.T.) ;
#72284=ORIENTED_EDGE('',*,*,#51746,.T.) ;
#72285=ORIENTED_EDGE('',*,*,#51747,.T.) ;
#72286=ORIENTED_EDGE('',*,*,#51735,.T.) ;
#72287=ORIENTED_EDGE('',*,*,#51748,.T.) ;
#72288=ORIENTED_EDGE('',*,*,#51737,.T.) ;
#72289=ORIENTED_EDGE('',*,*,#51749,.T.) ;
#72290=ORIENTED_EDGE('',*,*,#51750,.T.) ;
#72291=ORIENTED_EDGE('',*,*,#51751,.T.) ;
#72292=ORIENTED_EDGE('',*,*,#51752,.T.) ;
#72293=ORIENTED_EDGE('',*,*,#51753,.T.) ;
#72294=ORIENTED_EDGE('',*,*,#51739,.T.) ;
#72295=ORIENTED_EDGE('',*,*,#51754,.T.) ;
#72296=ORIENTED_EDGE('',*,*,#51755,.T.) ;
#72297=ORIENTED_EDGE('',*,*,#51756,.T.) ;
#72298=ORIENTED_EDGE('',*,*,#51757,.T.) ;
#72299=ORIENTED_EDGE('',*,*,#51758,.T.) ;
#72300=ORIENTED_EDGE('',*,*,#51759,.F.) ;
#72301=ORIENTED_EDGE('',*,*,#51760,.T.) ;
#72302=ORIENTED_EDGE('',*,*,#51761,.F.) ;
#72303=ORIENTED_EDGE('',*,*,#51762,.T.) ;
#72304=ORIENTED_EDGE('',*,*,#51763,.F.) ;
#72305=ORIENTED_EDGE('',*,*,#51764,.T.) ;
#72306=ORIENTED_EDGE('',*,*,#51765,.F.) ;
#72307=ORIENTED_EDGE('',*,*,#51766,.T.) ;
#72308=ORIENTED_EDGE('',*,*,#51767,.T.) ;
#72309=ORIENTED_EDGE('',*,*,#51768,.T.) ;
#72310=ORIENTED_EDGE('',*,*,#51765,.T.) ;
#72311=ORIENTED_EDGE('',*,*,#51769,.T.) ;
#72312=ORIENTED_EDGE('',*,*,#51770,.T.) ;
#72313=ORIENTED_EDGE('',*,*,#51771,.T.) ;
#72314=ORIENTED_EDGE('',*,*,#51759,.T.) ;
#72315=ORIENTED_EDGE('',*,*,#51772,.T.) ;
#72316=ORIENTED_EDGE('',*,*,#51761,.T.) ;
#72317=ORIENTED_EDGE('',*,*,#51773,.T.) ;
#72318=ORIENTED_EDGE('',*,*,#51774,.T.) ;
#72319=ORIENTED_EDGE('',*,*,#51775,.T.) ;
#72320=ORIENTED_EDGE('',*,*,#51776,.T.) ;
#72321=ORIENTED_EDGE('',*,*,#51777,.T.) ;
#72322=ORIENTED_EDGE('',*,*,#51763,.T.) ;
#72323=ORIENTED_EDGE('',*,*,#51778,.T.) ;
#72324=ORIENTED_EDGE('',*,*,#51779,.T.) ;
#72325=ORIENTED_EDGE('',*,*,#51780,.T.) ;
#72326=ORIENTED_EDGE('',*,*,#51781,.T.) ;
#72327=ORIENTED_EDGE('',*,*,#51782,.T.) ;
#72328=ORIENTED_EDGE('',*,*,#51783,.F.) ;
#72329=ORIENTED_EDGE('',*,*,#51784,.T.) ;
#72330=ORIENTED_EDGE('',*,*,#51785,.F.) ;
#72331=ORIENTED_EDGE('',*,*,#51786,.T.) ;
#72332=ORIENTED_EDGE('',*,*,#51787,.F.) ;
#72333=ORIENTED_EDGE('',*,*,#51788,.T.) ;
#72334=ORIENTED_EDGE('',*,*,#51789,.F.) ;
#72335=ORIENTED_EDGE('',*,*,#51790,.T.) ;
#72336=ORIENTED_EDGE('',*,*,#51791,.T.) ;
#72337=ORIENTED_EDGE('',*,*,#51792,.T.) ;
#72338=ORIENTED_EDGE('',*,*,#51789,.T.) ;
#72339=ORIENTED_EDGE('',*,*,#51793,.T.) ;
#72340=ORIENTED_EDGE('',*,*,#51794,.T.) ;
#72341=ORIENTED_EDGE('',*,*,#51795,.T.) ;
#72342=ORIENTED_EDGE('',*,*,#51783,.T.) ;
#72343=ORIENTED_EDGE('',*,*,#51796,.T.) ;
#72344=ORIENTED_EDGE('',*,*,#51785,.T.) ;
#72345=ORIENTED_EDGE('',*,*,#51797,.T.) ;
#72346=ORIENTED_EDGE('',*,*,#51798,.T.) ;
#72347=ORIENTED_EDGE('',*,*,#51799,.T.) ;
#72348=ORIENTED_EDGE('',*,*,#51800,.T.) ;
#72349=ORIENTED_EDGE('',*,*,#51801,.T.) ;
#72350=ORIENTED_EDGE('',*,*,#51787,.T.) ;
#72351=ORIENTED_EDGE('',*,*,#51802,.T.) ;
#72352=ORIENTED_EDGE('',*,*,#51803,.T.) ;
#72353=ORIENTED_EDGE('',*,*,#51804,.T.) ;
#72354=ORIENTED_EDGE('',*,*,#51805,.T.) ;
#72355=ORIENTED_EDGE('',*,*,#51806,.T.) ;
#72356=ORIENTED_EDGE('',*,*,#51807,.F.) ;
#72357=ORIENTED_EDGE('',*,*,#51808,.T.) ;
#72358=ORIENTED_EDGE('',*,*,#51809,.F.) ;
#72359=ORIENTED_EDGE('',*,*,#51810,.T.) ;
#72360=ORIENTED_EDGE('',*,*,#51811,.F.) ;
#72361=ORIENTED_EDGE('',*,*,#51812,.T.) ;
#72362=ORIENTED_EDGE('',*,*,#51813,.F.) ;
#72363=ORIENTED_EDGE('',*,*,#51814,.T.) ;
#72364=ORIENTED_EDGE('',*,*,#51815,.T.) ;
#72365=ORIENTED_EDGE('',*,*,#51816,.T.) ;
#72366=ORIENTED_EDGE('',*,*,#51813,.T.) ;
#72367=ORIENTED_EDGE('',*,*,#51817,.T.) ;
#72368=ORIENTED_EDGE('',*,*,#51818,.T.) ;
#72369=ORIENTED_EDGE('',*,*,#51819,.T.) ;
#72370=ORIENTED_EDGE('',*,*,#51807,.T.) ;
#72371=ORIENTED_EDGE('',*,*,#51820,.T.) ;
#72372=ORIENTED_EDGE('',*,*,#51809,.T.) ;
#72373=ORIENTED_EDGE('',*,*,#51821,.T.) ;
#72374=ORIENTED_EDGE('',*,*,#51822,.T.) ;
#72375=ORIENTED_EDGE('',*,*,#51823,.T.) ;
#72376=ORIENTED_EDGE('',*,*,#51824,.T.) ;
#72377=ORIENTED_EDGE('',*,*,#51825,.T.) ;
#72378=ORIENTED_EDGE('',*,*,#51811,.T.) ;
#72379=ORIENTED_EDGE('',*,*,#51826,.T.) ;
#72380=ORIENTED_EDGE('',*,*,#51827,.T.) ;
#72381=ORIENTED_EDGE('',*,*,#51828,.T.) ;
#72382=ORIENTED_EDGE('',*,*,#51829,.T.) ;
#72383=ORIENTED_EDGE('',*,*,#51830,.T.) ;
#72384=ORIENTED_EDGE('',*,*,#51831,.F.) ;
#72385=ORIENTED_EDGE('',*,*,#51832,.T.) ;
#72386=ORIENTED_EDGE('',*,*,#51833,.F.) ;
#72387=ORIENTED_EDGE('',*,*,#51834,.T.) ;
#72388=ORIENTED_EDGE('',*,*,#51835,.F.) ;
#72389=ORIENTED_EDGE('',*,*,#51836,.T.) ;
#72390=ORIENTED_EDGE('',*,*,#51837,.F.) ;
#72391=ORIENTED_EDGE('',*,*,#51838,.T.) ;
#72392=ORIENTED_EDGE('',*,*,#51839,.T.) ;
#72393=ORIENTED_EDGE('',*,*,#51840,.T.) ;
#72394=ORIENTED_EDGE('',*,*,#51837,.T.) ;
#72395=ORIENTED_EDGE('',*,*,#51841,.T.) ;
#72396=ORIENTED_EDGE('',*,*,#51842,.T.) ;
#72397=ORIENTED_EDGE('',*,*,#51843,.T.) ;
#72398=ORIENTED_EDGE('',*,*,#51831,.T.) ;
#72399=ORIENTED_EDGE('',*,*,#51844,.T.) ;
#72400=ORIENTED_EDGE('',*,*,#51833,.T.) ;
#72401=ORIENTED_EDGE('',*,*,#51845,.T.) ;
#72402=ORIENTED_EDGE('',*,*,#51846,.T.) ;
#72403=ORIENTED_EDGE('',*,*,#51847,.T.) ;
#72404=ORIENTED_EDGE('',*,*,#51848,.T.) ;
#72405=ORIENTED_EDGE('',*,*,#51849,.T.) ;
#72406=ORIENTED_EDGE('',*,*,#51835,.T.) ;
#72407=ORIENTED_EDGE('',*,*,#51850,.T.) ;
#72408=ORIENTED_EDGE('',*,*,#51851,.T.) ;
#72409=ORIENTED_EDGE('',*,*,#51852,.T.) ;
#72410=ORIENTED_EDGE('',*,*,#51853,.T.) ;
#72411=ORIENTED_EDGE('',*,*,#51854,.T.) ;
#72412=ORIENTED_EDGE('',*,*,#51855,.T.) ;
#72413=ORIENTED_EDGE('',*,*,#51856,.T.) ;
#72414=ORIENTED_EDGE('',*,*,#51857,.T.) ;
#72415=ORIENTED_EDGE('',*,*,#51858,.T.) ;
#72416=ORIENTED_EDGE('',*,*,#51859,.T.) ;
#72417=ORIENTED_EDGE('',*,*,#51860,.T.) ;
#72418=ORIENTED_EDGE('',*,*,#51861,.T.) ;
#72419=ORIENTED_EDGE('',*,*,#51862,.T.) ;
#72420=ORIENTED_EDGE('',*,*,#51863,.T.) ;
#72421=ORIENTED_EDGE('',*,*,#51864,.T.) ;
#72422=ORIENTED_EDGE('',*,*,#51865,.T.) ;
#72423=ORIENTED_EDGE('',*,*,#51866,.T.) ;
#72424=ORIENTED_EDGE('',*,*,#51867,.T.) ;
#72425=ORIENTED_EDGE('',*,*,#51868,.T.) ;
#72426=ORIENTED_EDGE('',*,*,#51869,.T.) ;
#72427=ORIENTED_EDGE('',*,*,#51870,.T.) ;
#72428=ORIENTED_EDGE('',*,*,#51871,.T.) ;
#72429=ORIENTED_EDGE('',*,*,#51872,.T.) ;
#72430=ORIENTED_EDGE('',*,*,#51873,.T.) ;
#72431=ORIENTED_EDGE('',*,*,#51874,.T.) ;
#72432=ORIENTED_EDGE('',*,*,#51875,.T.) ;
#72433=ORIENTED_EDGE('',*,*,#51876,.T.) ;
#72434=ORIENTED_EDGE('',*,*,#51877,.T.) ;
#72435=ORIENTED_EDGE('',*,*,#51878,.T.) ;
#72436=ORIENTED_EDGE('',*,*,#51879,.T.) ;
#72437=ORIENTED_EDGE('',*,*,#51880,.T.) ;
#72438=ORIENTED_EDGE('',*,*,#51881,.T.) ;
#72439=ORIENTED_EDGE('',*,*,#51882,.T.) ;
#72440=ORIENTED_EDGE('',*,*,#51883,.T.) ;
#72441=ORIENTED_EDGE('',*,*,#51884,.T.) ;
#72442=ORIENTED_EDGE('',*,*,#51885,.T.) ;
#72443=ORIENTED_EDGE('',*,*,#51886,.T.) ;
#72444=ORIENTED_EDGE('',*,*,#49231,.T.) ;
#72445=ORIENTED_EDGE('',*,*,#49247,.T.) ;
#72446=ORIENTED_EDGE('',*,*,#51887,.T.) ;
#72447=ORIENTED_EDGE('',*,*,#49213,.T.) ;
#72448=ORIENTED_EDGE('',*,*,#49229,.T.) ;
#72449=ORIENTED_EDGE('',*,*,#51888,.T.) ;
#72450=ORIENTED_EDGE('',*,*,#49195,.T.) ;
#72451=ORIENTED_EDGE('',*,*,#49211,.T.) ;
#72452=ORIENTED_EDGE('',*,*,#51889,.T.) ;
#72453=ORIENTED_EDGE('',*,*,#49177,.T.) ;
#72454=ORIENTED_EDGE('',*,*,#49193,.T.) ;
#72455=ORIENTED_EDGE('',*,*,#51890,.T.) ;
#72456=ORIENTED_EDGE('',*,*,#49159,.T.) ;
#72457=ORIENTED_EDGE('',*,*,#49175,.T.) ;
#72458=ORIENTED_EDGE('',*,*,#51891,.T.) ;
#72459=ORIENTED_EDGE('',*,*,#49141,.T.) ;
#72460=ORIENTED_EDGE('',*,*,#49157,.T.) ;
#72461=ORIENTED_EDGE('',*,*,#51892,.T.) ;
#72462=ORIENTED_EDGE('',*,*,#49123,.T.) ;
#72463=ORIENTED_EDGE('',*,*,#49139,.T.) ;
#72464=ORIENTED_EDGE('',*,*,#51893,.T.) ;
#72465=ORIENTED_EDGE('',*,*,#49105,.T.) ;
#72466=ORIENTED_EDGE('',*,*,#49121,.T.) ;
#72467=ORIENTED_EDGE('',*,*,#51894,.T.) ;
#72468=ORIENTED_EDGE('',*,*,#49087,.T.) ;
#72469=ORIENTED_EDGE('',*,*,#49103,.T.) ;
#72470=ORIENTED_EDGE('',*,*,#51895,.T.) ;
#72471=ORIENTED_EDGE('',*,*,#49089,.T.) ;
#72472=ORIENTED_EDGE('',*,*,#51896,.T.) ;
#72473=ORIENTED_EDGE('',*,*,#49101,.F.) ;
#72474=ORIENTED_EDGE('',*,*,#51897,.T.) ;
#72475=ORIENTED_EDGE('',*,*,#49093,.F.) ;
#72476=ORIENTED_EDGE('',*,*,#51898,.T.) ;
#72477=ORIENTED_EDGE('',*,*,#49097,.T.) ;
#72478=ORIENTED_EDGE('',*,*,#51899,.T.) ;
#72479=ORIENTED_EDGE('',*,*,#49091,.T.) ;
#72480=ORIENTED_EDGE('',*,*,#51900,.T.) ;
#72481=ORIENTED_EDGE('',*,*,#49099,.T.) ;
#72482=ORIENTED_EDGE('',*,*,#51901,.T.) ;
#72483=ORIENTED_EDGE('',*,*,#49107,.T.) ;
#72484=ORIENTED_EDGE('',*,*,#51902,.T.) ;
#72485=ORIENTED_EDGE('',*,*,#49119,.F.) ;
#72486=ORIENTED_EDGE('',*,*,#51903,.T.) ;
#72487=ORIENTED_EDGE('',*,*,#49111,.F.) ;
#72488=ORIENTED_EDGE('',*,*,#51904,.T.) ;
#72489=ORIENTED_EDGE('',*,*,#49115,.T.) ;
#72490=ORIENTED_EDGE('',*,*,#51905,.T.) ;
#72491=ORIENTED_EDGE('',*,*,#49109,.T.) ;
#72492=ORIENTED_EDGE('',*,*,#51906,.T.) ;
#72493=ORIENTED_EDGE('',*,*,#49117,.T.) ;
#72494=ORIENTED_EDGE('',*,*,#51907,.T.) ;
#72495=ORIENTED_EDGE('',*,*,#49125,.T.) ;
#72496=ORIENTED_EDGE('',*,*,#51908,.T.) ;
#72497=ORIENTED_EDGE('',*,*,#49137,.F.) ;
#72498=ORIENTED_EDGE('',*,*,#51909,.T.) ;
#72499=ORIENTED_EDGE('',*,*,#49129,.F.) ;
#72500=ORIENTED_EDGE('',*,*,#51910,.T.) ;
#72501=ORIENTED_EDGE('',*,*,#49133,.T.) ;
#72502=ORIENTED_EDGE('',*,*,#51911,.T.) ;
#72503=ORIENTED_EDGE('',*,*,#49127,.T.) ;
#72504=ORIENTED_EDGE('',*,*,#51912,.T.) ;
#72505=ORIENTED_EDGE('',*,*,#49135,.T.) ;
#72506=ORIENTED_EDGE('',*,*,#51913,.T.) ;
#72507=ORIENTED_EDGE('',*,*,#49143,.T.) ;
#72508=ORIENTED_EDGE('',*,*,#51914,.T.) ;
#72509=ORIENTED_EDGE('',*,*,#49155,.F.) ;
#72510=ORIENTED_EDGE('',*,*,#51915,.T.) ;
#72511=ORIENTED_EDGE('',*,*,#49147,.F.) ;
#72512=ORIENTED_EDGE('',*,*,#51916,.T.) ;
#72513=ORIENTED_EDGE('',*,*,#49151,.T.) ;
#72514=ORIENTED_EDGE('',*,*,#51917,.T.) ;
#72515=ORIENTED_EDGE('',*,*,#49145,.T.) ;
#72516=ORIENTED_EDGE('',*,*,#51918,.T.) ;
#72517=ORIENTED_EDGE('',*,*,#49153,.T.) ;
#72518=ORIENTED_EDGE('',*,*,#51919,.T.) ;
#72519=ORIENTED_EDGE('',*,*,#49161,.T.) ;
#72520=ORIENTED_EDGE('',*,*,#51920,.T.) ;
#72521=ORIENTED_EDGE('',*,*,#49173,.F.) ;
#72522=ORIENTED_EDGE('',*,*,#51921,.T.) ;
#72523=ORIENTED_EDGE('',*,*,#49165,.F.) ;
#72524=ORIENTED_EDGE('',*,*,#51922,.T.) ;
#72525=ORIENTED_EDGE('',*,*,#49169,.T.) ;
#72526=ORIENTED_EDGE('',*,*,#51923,.T.) ;
#72527=ORIENTED_EDGE('',*,*,#49163,.T.) ;
#72528=ORIENTED_EDGE('',*,*,#51924,.T.) ;
#72529=ORIENTED_EDGE('',*,*,#49171,.T.) ;
#72530=ORIENTED_EDGE('',*,*,#51925,.T.) ;
#72531=ORIENTED_EDGE('',*,*,#49179,.T.) ;
#72532=ORIENTED_EDGE('',*,*,#51926,.T.) ;
#72533=ORIENTED_EDGE('',*,*,#49191,.F.) ;
#72534=ORIENTED_EDGE('',*,*,#51927,.T.) ;
#72535=ORIENTED_EDGE('',*,*,#49183,.F.) ;
#72536=ORIENTED_EDGE('',*,*,#51928,.T.) ;
#72537=ORIENTED_EDGE('',*,*,#49187,.T.) ;
#72538=ORIENTED_EDGE('',*,*,#51929,.T.) ;
#72539=ORIENTED_EDGE('',*,*,#49181,.T.) ;
#72540=ORIENTED_EDGE('',*,*,#51930,.T.) ;
#72541=ORIENTED_EDGE('',*,*,#49189,.T.) ;
#72542=ORIENTED_EDGE('',*,*,#51931,.T.) ;
#72543=ORIENTED_EDGE('',*,*,#49197,.T.) ;
#72544=ORIENTED_EDGE('',*,*,#51932,.T.) ;
#72545=ORIENTED_EDGE('',*,*,#49209,.F.) ;
#72546=ORIENTED_EDGE('',*,*,#51933,.T.) ;
#72547=ORIENTED_EDGE('',*,*,#49201,.F.) ;
#72548=ORIENTED_EDGE('',*,*,#51934,.T.) ;
#72549=ORIENTED_EDGE('',*,*,#49205,.T.) ;
#72550=ORIENTED_EDGE('',*,*,#51935,.T.) ;
#72551=ORIENTED_EDGE('',*,*,#49199,.T.) ;
#72552=ORIENTED_EDGE('',*,*,#51936,.T.) ;
#72553=ORIENTED_EDGE('',*,*,#49207,.T.) ;
#72554=ORIENTED_EDGE('',*,*,#51937,.T.) ;
#72555=ORIENTED_EDGE('',*,*,#49215,.T.) ;
#72556=ORIENTED_EDGE('',*,*,#51938,.T.) ;
#72557=ORIENTED_EDGE('',*,*,#49227,.F.) ;
#72558=ORIENTED_EDGE('',*,*,#51939,.T.) ;
#72559=ORIENTED_EDGE('',*,*,#49219,.F.) ;
#72560=ORIENTED_EDGE('',*,*,#51940,.T.) ;
#72561=ORIENTED_EDGE('',*,*,#49223,.T.) ;
#72562=ORIENTED_EDGE('',*,*,#51941,.T.) ;
#72563=ORIENTED_EDGE('',*,*,#49217,.T.) ;
#72564=ORIENTED_EDGE('',*,*,#51942,.T.) ;
#72565=ORIENTED_EDGE('',*,*,#49225,.T.) ;
#72566=ORIENTED_EDGE('',*,*,#51943,.T.) ;
#72567=ORIENTED_EDGE('',*,*,#49233,.T.) ;
#72568=ORIENTED_EDGE('',*,*,#51944,.T.) ;
#72569=ORIENTED_EDGE('',*,*,#49245,.F.) ;
#72570=ORIENTED_EDGE('',*,*,#51945,.T.) ;
#72571=ORIENTED_EDGE('',*,*,#49237,.F.) ;
#72572=ORIENTED_EDGE('',*,*,#51946,.T.) ;
#72573=ORIENTED_EDGE('',*,*,#49241,.T.) ;
#72574=ORIENTED_EDGE('',*,*,#51947,.T.) ;
#72575=ORIENTED_EDGE('',*,*,#49235,.T.) ;
#72576=ORIENTED_EDGE('',*,*,#51948,.T.) ;
#72577=ORIENTED_EDGE('',*,*,#49243,.T.) ;
#72578=ORIENTED_EDGE('',*,*,#51949,.T.) ;
#72579=ORIENTED_EDGE('',*,*,#51950,.T.) ;
#72580=ORIENTED_EDGE('',*,*,#51951,.T.) ;
#72581=ORIENTED_EDGE('',*,*,#51952,.F.) ;
#72582=ORIENTED_EDGE('',*,*,#51953,.T.) ;
#72583=ORIENTED_EDGE('',*,*,#51952,.T.) ;
#72584=ORIENTED_EDGE('',*,*,#51954,.T.) ;
#72585=ORIENTED_EDGE('',*,*,#51955,.F.) ;
#72586=ORIENTED_EDGE('',*,*,#51956,.T.) ;
#72587=ORIENTED_EDGE('',*,*,#51955,.T.) ;
#72588=ORIENTED_EDGE('',*,*,#51957,.T.) ;
#72589=ORIENTED_EDGE('',*,*,#51958,.F.) ;
#72590=ORIENTED_EDGE('',*,*,#51959,.T.) ;
#72591=ORIENTED_EDGE('',*,*,#51958,.T.) ;
#72592=ORIENTED_EDGE('',*,*,#51960,.T.) ;
#72593=ORIENTED_EDGE('',*,*,#51961,.F.) ;
#72594=ORIENTED_EDGE('',*,*,#51962,.T.) ;
#72595=ORIENTED_EDGE('',*,*,#51961,.T.) ;
#72596=ORIENTED_EDGE('',*,*,#51963,.T.) ;
#72597=ORIENTED_EDGE('',*,*,#51964,.F.) ;
#72598=ORIENTED_EDGE('',*,*,#51965,.T.) ;
#72599=ORIENTED_EDGE('',*,*,#51964,.T.) ;
#72600=ORIENTED_EDGE('',*,*,#51966,.T.) ;
#72601=ORIENTED_EDGE('',*,*,#51967,.F.) ;
#72602=ORIENTED_EDGE('',*,*,#51968,.T.) ;
#72603=ORIENTED_EDGE('',*,*,#51967,.T.) ;
#72604=ORIENTED_EDGE('',*,*,#51969,.T.) ;
#72605=ORIENTED_EDGE('',*,*,#51970,.F.) ;
#72606=ORIENTED_EDGE('',*,*,#51971,.T.) ;
#72607=ORIENTED_EDGE('',*,*,#51950,.F.) ;
#72608=ORIENTED_EDGE('',*,*,#51972,.T.) ;
#72609=ORIENTED_EDGE('',*,*,#51970,.T.) ;
#72610=ORIENTED_EDGE('',*,*,#51973,.T.) ;
#72611=ORIENTED_EDGE('',*,*,#51974,.T.) ;
#72612=ORIENTED_EDGE('',*,*,#51975,.T.) ;
#72613=ORIENTED_EDGE('',*,*,#51976,.T.) ;
#72614=ORIENTED_EDGE('',*,*,#51977,.T.) ;
#72615=ORIENTED_EDGE('',*,*,#51978,.T.) ;
#72616=ORIENTED_EDGE('',*,*,#51979,.T.) ;
#72617=ORIENTED_EDGE('',*,*,#51980,.F.) ;
#72618=ORIENTED_EDGE('',*,*,#51981,.T.) ;
#72619=ORIENTED_EDGE('',*,*,#51980,.T.) ;
#72620=ORIENTED_EDGE('',*,*,#51982,.T.) ;
#72621=ORIENTED_EDGE('',*,*,#51983,.F.) ;
#72622=ORIENTED_EDGE('',*,*,#51984,.T.) ;
#72623=ORIENTED_EDGE('',*,*,#51983,.T.) ;
#72624=ORIENTED_EDGE('',*,*,#51985,.T.) ;
#72625=ORIENTED_EDGE('',*,*,#51986,.F.) ;
#72626=ORIENTED_EDGE('',*,*,#51987,.T.) ;
#72627=ORIENTED_EDGE('',*,*,#51986,.T.) ;
#72628=ORIENTED_EDGE('',*,*,#51988,.T.) ;
#72629=ORIENTED_EDGE('',*,*,#51989,.F.) ;
#72630=ORIENTED_EDGE('',*,*,#51990,.T.) ;
#72631=ORIENTED_EDGE('',*,*,#51989,.T.) ;
#72632=ORIENTED_EDGE('',*,*,#51991,.T.) ;
#72633=ORIENTED_EDGE('',*,*,#51992,.F.) ;
#72634=ORIENTED_EDGE('',*,*,#51993,.T.) ;
#72635=ORIENTED_EDGE('',*,*,#51992,.T.) ;
#72636=ORIENTED_EDGE('',*,*,#51994,.T.) ;
#72637=ORIENTED_EDGE('',*,*,#51995,.F.) ;
#72638=ORIENTED_EDGE('',*,*,#51996,.T.) ;
#72639=ORIENTED_EDGE('',*,*,#51995,.T.) ;
#72640=ORIENTED_EDGE('',*,*,#51997,.T.) ;
#72641=ORIENTED_EDGE('',*,*,#51998,.F.) ;
#72642=ORIENTED_EDGE('',*,*,#51999,.T.) ;
#72643=ORIENTED_EDGE('',*,*,#51978,.F.) ;
#72644=ORIENTED_EDGE('',*,*,#52000,.T.) ;
#72645=ORIENTED_EDGE('',*,*,#51998,.T.) ;
#72646=ORIENTED_EDGE('',*,*,#52001,.T.) ;
#72647=ORIENTED_EDGE('',*,*,#52002,.T.) ;
#72648=ORIENTED_EDGE('',*,*,#52003,.T.) ;
#72649=ORIENTED_EDGE('',*,*,#52004,.T.) ;
#72650=ORIENTED_EDGE('',*,*,#52005,.T.) ;
#72651=ORIENTED_EDGE('',*,*,#52006,.T.) ;
#72652=ORIENTED_EDGE('',*,*,#52007,.T.) ;
#72653=ORIENTED_EDGE('',*,*,#52008,.F.) ;
#72654=ORIENTED_EDGE('',*,*,#52009,.T.) ;
#72655=ORIENTED_EDGE('',*,*,#52008,.T.) ;
#72656=ORIENTED_EDGE('',*,*,#52010,.T.) ;
#72657=ORIENTED_EDGE('',*,*,#52011,.F.) ;
#72658=ORIENTED_EDGE('',*,*,#52012,.T.) ;
#72659=ORIENTED_EDGE('',*,*,#52011,.T.) ;
#72660=ORIENTED_EDGE('',*,*,#52013,.T.) ;
#72661=ORIENTED_EDGE('',*,*,#52014,.F.) ;
#72662=ORIENTED_EDGE('',*,*,#52015,.T.) ;
#72663=ORIENTED_EDGE('',*,*,#52014,.T.) ;
#72664=ORIENTED_EDGE('',*,*,#52016,.T.) ;
#72665=ORIENTED_EDGE('',*,*,#52017,.F.) ;
#72666=ORIENTED_EDGE('',*,*,#52018,.T.) ;
#72667=ORIENTED_EDGE('',*,*,#52017,.T.) ;
#72668=ORIENTED_EDGE('',*,*,#52019,.T.) ;
#72669=ORIENTED_EDGE('',*,*,#52020,.F.) ;
#72670=ORIENTED_EDGE('',*,*,#52021,.T.) ;
#72671=ORIENTED_EDGE('',*,*,#52020,.T.) ;
#72672=ORIENTED_EDGE('',*,*,#52022,.T.) ;
#72673=ORIENTED_EDGE('',*,*,#52023,.F.) ;
#72674=ORIENTED_EDGE('',*,*,#52024,.T.) ;
#72675=ORIENTED_EDGE('',*,*,#52023,.T.) ;
#72676=ORIENTED_EDGE('',*,*,#52025,.T.) ;
#72677=ORIENTED_EDGE('',*,*,#52026,.F.) ;
#72678=ORIENTED_EDGE('',*,*,#52027,.T.) ;
#72679=ORIENTED_EDGE('',*,*,#52006,.F.) ;
#72680=ORIENTED_EDGE('',*,*,#52028,.T.) ;
#72681=ORIENTED_EDGE('',*,*,#52026,.T.) ;
#72682=ORIENTED_EDGE('',*,*,#52029,.T.) ;
#72683=ORIENTED_EDGE('',*,*,#52030,.T.) ;
#72684=ORIENTED_EDGE('',*,*,#52031,.T.) ;
#72685=ORIENTED_EDGE('',*,*,#52032,.T.) ;
#72686=ORIENTED_EDGE('',*,*,#52033,.T.) ;
#72687=ORIENTED_EDGE('',*,*,#52034,.T.) ;
#72688=ORIENTED_EDGE('',*,*,#52035,.T.) ;
#72689=ORIENTED_EDGE('',*,*,#52036,.F.) ;
#72690=ORIENTED_EDGE('',*,*,#52037,.T.) ;
#72691=ORIENTED_EDGE('',*,*,#52036,.T.) ;
#72692=ORIENTED_EDGE('',*,*,#52038,.T.) ;
#72693=ORIENTED_EDGE('',*,*,#52039,.F.) ;
#72694=ORIENTED_EDGE('',*,*,#52040,.T.) ;
#72695=ORIENTED_EDGE('',*,*,#52039,.T.) ;
#72696=ORIENTED_EDGE('',*,*,#52041,.T.) ;
#72697=ORIENTED_EDGE('',*,*,#52042,.F.) ;
#72698=ORIENTED_EDGE('',*,*,#52043,.T.) ;
#72699=ORIENTED_EDGE('',*,*,#52042,.T.) ;
#72700=ORIENTED_EDGE('',*,*,#52044,.T.) ;
#72701=ORIENTED_EDGE('',*,*,#52045,.F.) ;
#72702=ORIENTED_EDGE('',*,*,#52046,.T.) ;
#72703=ORIENTED_EDGE('',*,*,#52045,.T.) ;
#72704=ORIENTED_EDGE('',*,*,#52047,.T.) ;
#72705=ORIENTED_EDGE('',*,*,#52048,.F.) ;
#72706=ORIENTED_EDGE('',*,*,#52049,.T.) ;
#72707=ORIENTED_EDGE('',*,*,#52048,.T.) ;
#72708=ORIENTED_EDGE('',*,*,#52050,.T.) ;
#72709=ORIENTED_EDGE('',*,*,#52051,.F.) ;
#72710=ORIENTED_EDGE('',*,*,#52052,.T.) ;
#72711=ORIENTED_EDGE('',*,*,#52051,.T.) ;
#72712=ORIENTED_EDGE('',*,*,#52053,.T.) ;
#72713=ORIENTED_EDGE('',*,*,#52054,.F.) ;
#72714=ORIENTED_EDGE('',*,*,#52055,.T.) ;
#72715=ORIENTED_EDGE('',*,*,#52034,.F.) ;
#72716=ORIENTED_EDGE('',*,*,#52056,.T.) ;
#72717=ORIENTED_EDGE('',*,*,#52054,.T.) ;
#72718=ORIENTED_EDGE('',*,*,#52057,.T.) ;
#72719=ORIENTED_EDGE('',*,*,#52058,.T.) ;
#72720=ORIENTED_EDGE('',*,*,#52059,.T.) ;
#72721=ORIENTED_EDGE('',*,*,#52060,.T.) ;
#72722=ORIENTED_EDGE('',*,*,#52061,.T.) ;
#72723=ORIENTED_EDGE('',*,*,#52062,.T.) ;
#72724=ORIENTED_EDGE('',*,*,#52063,.T.) ;
#72725=ORIENTED_EDGE('',*,*,#52064,.F.) ;
#72726=ORIENTED_EDGE('',*,*,#52065,.T.) ;
#72727=ORIENTED_EDGE('',*,*,#52064,.T.) ;
#72728=ORIENTED_EDGE('',*,*,#52066,.T.) ;
#72729=ORIENTED_EDGE('',*,*,#52067,.F.) ;
#72730=ORIENTED_EDGE('',*,*,#52068,.T.) ;
#72731=ORIENTED_EDGE('',*,*,#52067,.T.) ;
#72732=ORIENTED_EDGE('',*,*,#52069,.T.) ;
#72733=ORIENTED_EDGE('',*,*,#52070,.F.) ;
#72734=ORIENTED_EDGE('',*,*,#52071,.T.) ;
#72735=ORIENTED_EDGE('',*,*,#52070,.T.) ;
#72736=ORIENTED_EDGE('',*,*,#52072,.T.) ;
#72737=ORIENTED_EDGE('',*,*,#52073,.F.) ;
#72738=ORIENTED_EDGE('',*,*,#52074,.T.) ;
#72739=ORIENTED_EDGE('',*,*,#52073,.T.) ;
#72740=ORIENTED_EDGE('',*,*,#52075,.T.) ;
#72741=ORIENTED_EDGE('',*,*,#52076,.F.) ;
#72742=ORIENTED_EDGE('',*,*,#52077,.T.) ;
#72743=ORIENTED_EDGE('',*,*,#52076,.T.) ;
#72744=ORIENTED_EDGE('',*,*,#52078,.T.) ;
#72745=ORIENTED_EDGE('',*,*,#52079,.F.) ;
#72746=ORIENTED_EDGE('',*,*,#52080,.T.) ;
#72747=ORIENTED_EDGE('',*,*,#52079,.T.) ;
#72748=ORIENTED_EDGE('',*,*,#52081,.T.) ;
#72749=ORIENTED_EDGE('',*,*,#52082,.F.) ;
#72750=ORIENTED_EDGE('',*,*,#52083,.T.) ;
#72751=ORIENTED_EDGE('',*,*,#52062,.F.) ;
#72752=ORIENTED_EDGE('',*,*,#52084,.T.) ;
#72753=ORIENTED_EDGE('',*,*,#52082,.T.) ;
#72754=ORIENTED_EDGE('',*,*,#52085,.T.) ;
#72755=ORIENTED_EDGE('',*,*,#52086,.T.) ;
#72756=ORIENTED_EDGE('',*,*,#52087,.T.) ;
#72757=ORIENTED_EDGE('',*,*,#52088,.T.) ;
#72758=ORIENTED_EDGE('',*,*,#52089,.T.) ;
#72759=ORIENTED_EDGE('',*,*,#52090,.T.) ;
#72760=ORIENTED_EDGE('',*,*,#52091,.T.) ;
#72761=ORIENTED_EDGE('',*,*,#52092,.F.) ;
#72762=ORIENTED_EDGE('',*,*,#52093,.T.) ;
#72763=ORIENTED_EDGE('',*,*,#52092,.T.) ;
#72764=ORIENTED_EDGE('',*,*,#52094,.T.) ;
#72765=ORIENTED_EDGE('',*,*,#52095,.F.) ;
#72766=ORIENTED_EDGE('',*,*,#52096,.T.) ;
#72767=ORIENTED_EDGE('',*,*,#52095,.T.) ;
#72768=ORIENTED_EDGE('',*,*,#52097,.T.) ;
#72769=ORIENTED_EDGE('',*,*,#52098,.F.) ;
#72770=ORIENTED_EDGE('',*,*,#52099,.T.) ;
#72771=ORIENTED_EDGE('',*,*,#52098,.T.) ;
#72772=ORIENTED_EDGE('',*,*,#52100,.T.) ;
#72773=ORIENTED_EDGE('',*,*,#52101,.F.) ;
#72774=ORIENTED_EDGE('',*,*,#52102,.T.) ;
#72775=ORIENTED_EDGE('',*,*,#52101,.T.) ;
#72776=ORIENTED_EDGE('',*,*,#52103,.T.) ;
#72777=ORIENTED_EDGE('',*,*,#52104,.F.) ;
#72778=ORIENTED_EDGE('',*,*,#52105,.T.) ;
#72779=ORIENTED_EDGE('',*,*,#52104,.T.) ;
#72780=ORIENTED_EDGE('',*,*,#52106,.T.) ;
#72781=ORIENTED_EDGE('',*,*,#52107,.F.) ;
#72782=ORIENTED_EDGE('',*,*,#52108,.T.) ;
#72783=ORIENTED_EDGE('',*,*,#52107,.T.) ;
#72784=ORIENTED_EDGE('',*,*,#52109,.T.) ;
#72785=ORIENTED_EDGE('',*,*,#52110,.F.) ;
#72786=ORIENTED_EDGE('',*,*,#52111,.T.) ;
#72787=ORIENTED_EDGE('',*,*,#52090,.F.) ;
#72788=ORIENTED_EDGE('',*,*,#52112,.T.) ;
#72789=ORIENTED_EDGE('',*,*,#52110,.T.) ;
#72790=ORIENTED_EDGE('',*,*,#52113,.T.) ;
#72791=ORIENTED_EDGE('',*,*,#52114,.T.) ;
#72792=ORIENTED_EDGE('',*,*,#52115,.T.) ;
#72793=ORIENTED_EDGE('',*,*,#52116,.T.) ;
#72794=ORIENTED_EDGE('',*,*,#52117,.T.) ;
#72795=ORIENTED_EDGE('',*,*,#52118,.T.) ;
#72796=ORIENTED_EDGE('',*,*,#52119,.T.) ;
#72797=ORIENTED_EDGE('',*,*,#52120,.F.) ;
#72798=ORIENTED_EDGE('',*,*,#52121,.T.) ;
#72799=ORIENTED_EDGE('',*,*,#52120,.T.) ;
#72800=ORIENTED_EDGE('',*,*,#52122,.T.) ;
#72801=ORIENTED_EDGE('',*,*,#52123,.F.) ;
#72802=ORIENTED_EDGE('',*,*,#52124,.T.) ;
#72803=ORIENTED_EDGE('',*,*,#52123,.T.) ;
#72804=ORIENTED_EDGE('',*,*,#52125,.T.) ;
#72805=ORIENTED_EDGE('',*,*,#52126,.F.) ;
#72806=ORIENTED_EDGE('',*,*,#52127,.T.) ;
#72807=ORIENTED_EDGE('',*,*,#52126,.T.) ;
#72808=ORIENTED_EDGE('',*,*,#52128,.T.) ;
#72809=ORIENTED_EDGE('',*,*,#52129,.F.) ;
#72810=ORIENTED_EDGE('',*,*,#52130,.T.) ;
#72811=ORIENTED_EDGE('',*,*,#52129,.T.) ;
#72812=ORIENTED_EDGE('',*,*,#52131,.T.) ;
#72813=ORIENTED_EDGE('',*,*,#52132,.F.) ;
#72814=ORIENTED_EDGE('',*,*,#52133,.T.) ;
#72815=ORIENTED_EDGE('',*,*,#52132,.T.) ;
#72816=ORIENTED_EDGE('',*,*,#52134,.T.) ;
#72817=ORIENTED_EDGE('',*,*,#52135,.F.) ;
#72818=ORIENTED_EDGE('',*,*,#52136,.T.) ;
#72819=ORIENTED_EDGE('',*,*,#52135,.T.) ;
#72820=ORIENTED_EDGE('',*,*,#52137,.T.) ;
#72821=ORIENTED_EDGE('',*,*,#52138,.F.) ;
#72822=ORIENTED_EDGE('',*,*,#52139,.T.) ;
#72823=ORIENTED_EDGE('',*,*,#52118,.F.) ;
#72824=ORIENTED_EDGE('',*,*,#52140,.T.) ;
#72825=ORIENTED_EDGE('',*,*,#52138,.T.) ;
#72826=ORIENTED_EDGE('',*,*,#52141,.T.) ;
#72827=ORIENTED_EDGE('',*,*,#52142,.T.) ;
#72828=ORIENTED_EDGE('',*,*,#52143,.T.) ;
#72829=ORIENTED_EDGE('',*,*,#52144,.T.) ;
#72830=ORIENTED_EDGE('',*,*,#52145,.T.) ;
#72831=ORIENTED_EDGE('',*,*,#52146,.T.) ;
#72832=ORIENTED_EDGE('',*,*,#52147,.T.) ;
#72833=ORIENTED_EDGE('',*,*,#52148,.F.) ;
#72834=ORIENTED_EDGE('',*,*,#52149,.T.) ;
#72835=ORIENTED_EDGE('',*,*,#52148,.T.) ;
#72836=ORIENTED_EDGE('',*,*,#52150,.T.) ;
#72837=ORIENTED_EDGE('',*,*,#52151,.F.) ;
#72838=ORIENTED_EDGE('',*,*,#52152,.T.) ;
#72839=ORIENTED_EDGE('',*,*,#52151,.T.) ;
#72840=ORIENTED_EDGE('',*,*,#52153,.T.) ;
#72841=ORIENTED_EDGE('',*,*,#52154,.F.) ;
#72842=ORIENTED_EDGE('',*,*,#52155,.T.) ;
#72843=ORIENTED_EDGE('',*,*,#52154,.T.) ;
#72844=ORIENTED_EDGE('',*,*,#52156,.T.) ;
#72845=ORIENTED_EDGE('',*,*,#52157,.F.) ;
#72846=ORIENTED_EDGE('',*,*,#52158,.T.) ;
#72847=ORIENTED_EDGE('',*,*,#52157,.T.) ;
#72848=ORIENTED_EDGE('',*,*,#52159,.T.) ;
#72849=ORIENTED_EDGE('',*,*,#52160,.F.) ;
#72850=ORIENTED_EDGE('',*,*,#52161,.T.) ;
#72851=ORIENTED_EDGE('',*,*,#52160,.T.) ;
#72852=ORIENTED_EDGE('',*,*,#52162,.T.) ;
#72853=ORIENTED_EDGE('',*,*,#52163,.F.) ;
#72854=ORIENTED_EDGE('',*,*,#52164,.T.) ;
#72855=ORIENTED_EDGE('',*,*,#52163,.T.) ;
#72856=ORIENTED_EDGE('',*,*,#52165,.T.) ;
#72857=ORIENTED_EDGE('',*,*,#52166,.F.) ;
#72858=ORIENTED_EDGE('',*,*,#52167,.T.) ;
#72859=ORIENTED_EDGE('',*,*,#52146,.F.) ;
#72860=ORIENTED_EDGE('',*,*,#52168,.T.) ;
#72861=ORIENTED_EDGE('',*,*,#52166,.T.) ;
#72862=ORIENTED_EDGE('',*,*,#52169,.T.) ;
#72863=ORIENTED_EDGE('',*,*,#52170,.T.) ;
#72864=ORIENTED_EDGE('',*,*,#52171,.T.) ;
#72865=ORIENTED_EDGE('',*,*,#52172,.T.) ;
#72866=ORIENTED_EDGE('',*,*,#52173,.T.) ;
#72867=ORIENTED_EDGE('',*,*,#52174,.T.) ;
#72868=ORIENTED_EDGE('',*,*,#52175,.T.) ;
#72869=ORIENTED_EDGE('',*,*,#52176,.F.) ;
#72870=ORIENTED_EDGE('',*,*,#52177,.T.) ;
#72871=ORIENTED_EDGE('',*,*,#52176,.T.) ;
#72872=ORIENTED_EDGE('',*,*,#52178,.T.) ;
#72873=ORIENTED_EDGE('',*,*,#52179,.F.) ;
#72874=ORIENTED_EDGE('',*,*,#52180,.T.) ;
#72875=ORIENTED_EDGE('',*,*,#52179,.T.) ;
#72876=ORIENTED_EDGE('',*,*,#52181,.T.) ;
#72877=ORIENTED_EDGE('',*,*,#52182,.F.) ;
#72878=ORIENTED_EDGE('',*,*,#52183,.T.) ;
#72879=ORIENTED_EDGE('',*,*,#52182,.T.) ;
#72880=ORIENTED_EDGE('',*,*,#52184,.T.) ;
#72881=ORIENTED_EDGE('',*,*,#52185,.F.) ;
#72882=ORIENTED_EDGE('',*,*,#52186,.T.) ;
#72883=ORIENTED_EDGE('',*,*,#52185,.T.) ;
#72884=ORIENTED_EDGE('',*,*,#52187,.T.) ;
#72885=ORIENTED_EDGE('',*,*,#52188,.F.) ;
#72886=ORIENTED_EDGE('',*,*,#52189,.T.) ;
#72887=ORIENTED_EDGE('',*,*,#52188,.T.) ;
#72888=ORIENTED_EDGE('',*,*,#52190,.T.) ;
#72889=ORIENTED_EDGE('',*,*,#52191,.F.) ;
#72890=ORIENTED_EDGE('',*,*,#52192,.T.) ;
#72891=ORIENTED_EDGE('',*,*,#52191,.T.) ;
#72892=ORIENTED_EDGE('',*,*,#52193,.T.) ;
#72893=ORIENTED_EDGE('',*,*,#52194,.F.) ;
#72894=ORIENTED_EDGE('',*,*,#52195,.T.) ;
#72895=ORIENTED_EDGE('',*,*,#52174,.F.) ;
#72896=ORIENTED_EDGE('',*,*,#52196,.T.) ;
#72897=ORIENTED_EDGE('',*,*,#52194,.T.) ;
#72898=ORIENTED_EDGE('',*,*,#52197,.T.) ;
#72899=ORIENTED_EDGE('',*,*,#52198,.T.) ;
#72900=ORIENTED_EDGE('',*,*,#52199,.T.) ;
#72901=ORIENTED_EDGE('',*,*,#52200,.T.) ;
#72902=ORIENTED_EDGE('',*,*,#52201,.T.) ;
#72903=ORIENTED_EDGE('',*,*,#52202,.F.) ;
#72904=ORIENTED_EDGE('',*,*,#52203,.F.) ;
#72905=ORIENTED_EDGE('',*,*,#52204,.F.) ;
#72906=ORIENTED_EDGE('',*,*,#52203,.T.) ;
#72907=ORIENTED_EDGE('',*,*,#51342,.F.) ;
#72908=ORIENTED_EDGE('',*,*,#52205,.F.) ;
#72909=ORIENTED_EDGE('',*,*,#51340,.F.) ;
#72910=ORIENTED_EDGE('',*,*,#52204,.T.) ;
#72911=ORIENTED_EDGE('',*,*,#51339,.F.) ;
#72912=ORIENTED_EDGE('',*,*,#52206,.F.) ;
#72913=ORIENTED_EDGE('',*,*,#51329,.F.) ;
#72914=ORIENTED_EDGE('',*,*,#52202,.T.) ;
#72915=ORIENTED_EDGE('',*,*,#51332,.F.) ;
#72916=ORIENTED_EDGE('',*,*,#52207,.F.) ;
#72917=ORIENTED_EDGE('',*,*,#51343,.F.) ;
#72918=ORIENTED_EDGE('',*,*,#51095,.F.) ;
#72919=ORIENTED_EDGE('',*,*,#52208,.T.) ;
#72920=ORIENTED_EDGE('',*,*,#51344,.F.) ;
#72921=ORIENTED_EDGE('',*,*,#52209,.F.) ;
#72922=ORIENTED_EDGE('',*,*,#51345,.F.) ;
#72923=ORIENTED_EDGE('',*,*,#52210,.T.) ;
#72924=ORIENTED_EDGE('',*,*,#49511,.F.) ;
#72925=ORIENTED_EDGE('',*,*,#52211,.T.) ;
#72926=ORIENTED_EDGE('',*,*,#52212,.F.) ;
#72927=ORIENTED_EDGE('',*,*,#52205,.T.) ;
#72928=ORIENTED_EDGE('',*,*,#52213,.F.) ;
#72929=ORIENTED_EDGE('',*,*,#52214,.F.) ;
#72930=ORIENTED_EDGE('',*,*,#52206,.T.) ;
#72931=ORIENTED_EDGE('',*,*,#52215,.F.) ;
#72932=ORIENTED_EDGE('',*,*,#49666,.T.) ;
#72933=ORIENTED_EDGE('',*,*,#52209,.T.) ;
#72934=ORIENTED_EDGE('',*,*,#52207,.T.) ;
#72935=ORIENTED_EDGE('',*,*,#52216,.F.) ;
#72936=ORIENTED_EDGE('',*,*,#51346,.F.) ;
#72937=ORIENTED_EDGE('',*,*,#52217,.T.) ;
#72938=ORIENTED_EDGE('',*,*,#51085,.F.) ;
#72939=ORIENTED_EDGE('',*,*,#52218,.F.) ;
#72940=ORIENTED_EDGE('',*,*,#52213,.T.) ;
#72941=ORIENTED_EDGE('',*,*,#51341,.F.) ;
#72942=ORIENTED_EDGE('',*,*,#52219,.F.) ;
#72943=ORIENTED_EDGE('',*,*,#51336,.F.) ;
#72944=ORIENTED_EDGE('',*,*,#52212,.T.) ;
#72945=ORIENTED_EDGE('',*,*,#51335,.F.) ;
#72946=ORIENTED_EDGE('',*,*,#52220,.F.) ;
#72947=ORIENTED_EDGE('',*,*,#51337,.F.) ;
#72948=ORIENTED_EDGE('',*,*,#52215,.T.) ;
#72949=ORIENTED_EDGE('',*,*,#51338,.F.) ;
#72950=ORIENTED_EDGE('',*,*,#52221,.F.) ;
#72951=ORIENTED_EDGE('',*,*,#49667,.F.) ;
#72952=ORIENTED_EDGE('',*,*,#52214,.T.) ;
#72953=ORIENTED_EDGE('',*,*,#49665,.F.) ;
#72954=ORIENTED_EDGE('',*,*,#52222,.F.) ;
#72955=ORIENTED_EDGE('',*,*,#51330,.F.) ;
#72956=ORIENTED_EDGE('',*,*,#52216,.T.) ;
#72957=ORIENTED_EDGE('',*,*,#51331,.F.) ;
#72958=ORIENTED_EDGE('',*,*,#52223,.F.) ;
#72959=ORIENTED_EDGE('',*,*,#51096,.F.) ;
#72960=ORIENTED_EDGE('',*,*,#52219,.T.) ;
#72961=ORIENTED_EDGE('',*,*,#52218,.T.) ;
#72962=ORIENTED_EDGE('',*,*,#52224,.F.) ;
#72963=ORIENTED_EDGE('',*,*,#52221,.T.) ;
#72964=ORIENTED_EDGE('',*,*,#52220,.T.) ;
#72965=ORIENTED_EDGE('',*,*,#52225,.F.) ;
#72966=ORIENTED_EDGE('',*,*,#49660,.T.) ;
#72967=ORIENTED_EDGE('',*,*,#52223,.T.) ;
#72968=ORIENTED_EDGE('',*,*,#52222,.T.) ;
#72969=ORIENTED_EDGE('',*,*,#52226,.F.) ;
#72970=ORIENTED_EDGE('',*,*,#51097,.T.) ;
#72971=ORIENTED_EDGE('',*,*,#52224,.T.) ;
#72972=ORIENTED_EDGE('',*,*,#51084,.F.) ;
#72973=ORIENTED_EDGE('',*,*,#52227,.F.) ;
#72974=ORIENTED_EDGE('',*,*,#51333,.F.) ;
#72975=ORIENTED_EDGE('',*,*,#52225,.T.) ;
#72976=ORIENTED_EDGE('',*,*,#51334,.F.) ;
#72977=ORIENTED_EDGE('',*,*,#52228,.F.) ;
#72978=ORIENTED_EDGE('',*,*,#49661,.F.) ;
#72979=ORIENTED_EDGE('',*,*,#52226,.T.) ;
#72980=ORIENTED_EDGE('',*,*,#49664,.F.) ;
#72981=ORIENTED_EDGE('',*,*,#52229,.F.) ;
#72982=ORIENTED_EDGE('',*,*,#51098,.F.) ;
#72983=ORIENTED_EDGE('',*,*,#51103,.F.) ;
#72984=ORIENTED_EDGE('',*,*,#52230,.T.) ;
#72985=ORIENTED_EDGE('',*,*,#51091,.F.) ;
#72986=ORIENTED_EDGE('',*,*,#52231,.F.) ;
#72987=ORIENTED_EDGE('',*,*,#49722,.F.) ;
#72988=ORIENTED_EDGE('',*,*,#52232,.T.) ;
#72989=ORIENTED_EDGE('',*,*,#51104,.F.) ;
#72990=ORIENTED_EDGE('',*,*,#52233,.F.) ;
#72991=ORIENTED_EDGE('',*,*,#52227,.T.) ;
#72992=ORIENTED_EDGE('',*,*,#51083,.T.) ;
#72993=ORIENTED_EDGE('',*,*,#52234,.F.) ;
#72994=ORIENTED_EDGE('',*,*,#52228,.T.) ;
#72995=ORIENTED_EDGE('',*,*,#52235,.F.) ;
#72996=ORIENTED_EDGE('',*,*,#52229,.T.) ;
#72997=ORIENTED_EDGE('',*,*,#52236,.F.) ;
#72998=ORIENTED_EDGE('',*,*,#52233,.T.) ;
#72999=ORIENTED_EDGE('',*,*,#52231,.T.) ;
#73000=ORIENTED_EDGE('',*,*,#52237,.F.) ;
#73001=ORIENTED_EDGE('',*,*,#52234,.T.) ;
#73002=ORIENTED_EDGE('',*,*,#51082,.F.) ;
#73003=ORIENTED_EDGE('',*,*,#52238,.F.) ;
#73004=ORIENTED_EDGE('',*,*,#49662,.F.) ;
#73005=ORIENTED_EDGE('',*,*,#52236,.T.) ;
#73006=ORIENTED_EDGE('',*,*,#49663,.F.) ;
#73007=ORIENTED_EDGE('',*,*,#52239,.F.) ;
#73008=ORIENTED_EDGE('',*,*,#51090,.F.) ;
#73009=ORIENTED_EDGE('',*,*,#52235,.T.) ;
#73010=ORIENTED_EDGE('',*,*,#51089,.F.) ;
#73011=ORIENTED_EDGE('',*,*,#52240,.F.) ;
#73012=ORIENTED_EDGE('',*,*,#51099,.F.) ;
#73013=ORIENTED_EDGE('',*,*,#52237,.T.) ;
#73014=ORIENTED_EDGE('',*,*,#51100,.F.) ;
#73015=ORIENTED_EDGE('',*,*,#52241,.F.) ;
#73016=ORIENTED_EDGE('',*,*,#49723,.F.) ;
#73017=ORIENTED_EDGE('',*,*,#52239,.T.) ;
#73018=ORIENTED_EDGE('',*,*,#52238,.T.) ;
#73019=ORIENTED_EDGE('',*,*,#52242,.F.) ;
#73020=ORIENTED_EDGE('',*,*,#52241,.T.) ;
#73021=ORIENTED_EDGE('',*,*,#52240,.T.) ;
#73022=ORIENTED_EDGE('',*,*,#52243,.F.) ;
#73023=ORIENTED_EDGE('',*,*,#49724,.T.) ;
#73024=ORIENTED_EDGE('',*,*,#51079,.F.) ;
#73025=ORIENTED_EDGE('',*,*,#52244,.T.) ;
#73026=ORIENTED_EDGE('',*,*,#50026,.F.) ;
#73027=ORIENTED_EDGE('',*,*,#52245,.F.) ;
#73028=ORIENTED_EDGE('',*,*,#52242,.T.) ;
#73029=ORIENTED_EDGE('',*,*,#51081,.F.) ;
#73030=ORIENTED_EDGE('',*,*,#52246,.F.) ;
#73031=ORIENTED_EDGE('',*,*,#51087,.F.) ;
#73032=ORIENTED_EDGE('',*,*,#52243,.T.) ;
#73033=ORIENTED_EDGE('',*,*,#51088,.F.) ;
#73034=ORIENTED_EDGE('',*,*,#52247,.F.) ;
#73035=ORIENTED_EDGE('',*,*,#49725,.F.) ;
#73036=ORIENTED_EDGE('',*,*,#52245,.T.) ;
#73037=ORIENTED_EDGE('',*,*,#50211,.T.) ;
#73038=ORIENTED_EDGE('',*,*,#52248,.F.) ;
#73039=ORIENTED_EDGE('',*,*,#52247,.T.) ;
#73040=ORIENTED_EDGE('',*,*,#52246,.T.) ;
#73041=ORIENTED_EDGE('',*,*,#52249,.F.) ;
#73042=ORIENTED_EDGE('',*,*,#49726,.T.) ;
#73043=ORIENTED_EDGE('',*,*,#52248,.T.) ;
#73044=ORIENTED_EDGE('',*,*,#49727,.F.) ;
#73045=ORIENTED_EDGE('',*,*,#52249,.T.) ;
#73046=ORIENTED_EDGE('',*,*,#51080,.F.) ;
#73047=ORIENTED_EDGE('',*,*,#52250,.F.) ;
#73048=ORIENTED_EDGE('',*,*,#49520,.F.) ;
#73049=ORIENTED_EDGE('',*,*,#52251,.F.) ;
#73050=ORIENTED_EDGE('',*,*,#51957,.F.) ;
#73051=ORIENTED_EDGE('',*,*,#52251,.T.) ;
#73052=ORIENTED_EDGE('',*,*,#49519,.F.) ;
#73053=ORIENTED_EDGE('',*,*,#52252,.F.) ;
#73054=ORIENTED_EDGE('',*,*,#51960,.F.) ;
#73055=ORIENTED_EDGE('',*,*,#52250,.T.) ;
#73056=ORIENTED_EDGE('',*,*,#51954,.F.) ;
#73057=ORIENTED_EDGE('',*,*,#52253,.F.) ;
#73058=ORIENTED_EDGE('',*,*,#49521,.F.) ;
#73059=ORIENTED_EDGE('',*,*,#52252,.T.) ;
#73060=ORIENTED_EDGE('',*,*,#49518,.F.) ;
#73061=ORIENTED_EDGE('',*,*,#52254,.F.) ;
#73062=ORIENTED_EDGE('',*,*,#51963,.F.) ;
#73063=ORIENTED_EDGE('',*,*,#52253,.T.) ;
#73064=ORIENTED_EDGE('',*,*,#51951,.F.) ;
#73065=ORIENTED_EDGE('',*,*,#52255,.F.) ;
#73066=ORIENTED_EDGE('',*,*,#49522,.F.) ;
#73067=ORIENTED_EDGE('',*,*,#52254,.T.) ;
#73068=ORIENTED_EDGE('',*,*,#49517,.F.) ;
#73069=ORIENTED_EDGE('',*,*,#52256,.F.) ;
#73070=ORIENTED_EDGE('',*,*,#51966,.F.) ;
#73071=ORIENTED_EDGE('',*,*,#52255,.T.) ;
#73072=ORIENTED_EDGE('',*,*,#51973,.F.) ;
#73073=ORIENTED_EDGE('',*,*,#52257,.F.) ;
#73074=ORIENTED_EDGE('',*,*,#49515,.F.) ;
#73075=ORIENTED_EDGE('',*,*,#52256,.T.) ;
#73076=ORIENTED_EDGE('',*,*,#49516,.F.) ;
#73077=ORIENTED_EDGE('',*,*,#52257,.T.) ;
#73078=ORIENTED_EDGE('',*,*,#51969,.F.) ;
#73079=ORIENTED_EDGE('',*,*,#50687,.F.) ;
#73080=ORIENTED_EDGE('',*,*,#52258,.T.) ;
#73081=ORIENTED_EDGE('',*,*,#52259,.T.) ;
#73082=ORIENTED_EDGE('',*,*,#49839,.F.) ;
#73083=ORIENTED_EDGE('',*,*,#52260,.T.) ;
#73084=ORIENTED_EDGE('',*,*,#52261,.T.) ;
#73085=ORIENTED_EDGE('',*,*,#49838,.F.) ;
#73086=ORIENTED_EDGE('',*,*,#52262,.T.) ;
#73087=ORIENTED_EDGE('',*,*,#52263,.T.) ;
#73088=ORIENTED_EDGE('',*,*,#50681,.F.) ;
#73089=ORIENTED_EDGE('',*,*,#52264,.T.) ;
#73090=ORIENTED_EDGE('',*,*,#52265,.T.) ;
#73091=ORIENTED_EDGE('',*,*,#49836,.F.) ;
#73092=ORIENTED_EDGE('',*,*,#52266,.T.) ;
#73093=ORIENTED_EDGE('',*,*,#52267,.T.) ;
#73094=ORIENTED_EDGE('',*,*,#50689,.F.) ;
#73095=ORIENTED_EDGE('',*,*,#52268,.T.) ;
#73096=ORIENTED_EDGE('',*,*,#52269,.T.) ;
#73097=ORIENTED_EDGE('',*,*,#49837,.F.) ;
#73098=ORIENTED_EDGE('',*,*,#52270,.T.) ;
#73099=ORIENTED_EDGE('',*,*,#52271,.T.) ;
#73100=ORIENTED_EDGE('',*,*,#50693,.F.) ;
#73101=ORIENTED_EDGE('',*,*,#52272,.T.) ;
#73102=ORIENTED_EDGE('',*,*,#52273,.T.) ;
#73103=ORIENTED_EDGE('',*,*,#50703,.F.) ;
#73104=ORIENTED_EDGE('',*,*,#52274,.T.) ;
#73105=ORIENTED_EDGE('',*,*,#52275,.T.) ;
#73106=ORIENTED_EDGE('',*,*,#49843,.F.) ;
#73107=ORIENTED_EDGE('',*,*,#52276,.T.) ;
#73108=ORIENTED_EDGE('',*,*,#52277,.T.) ;
#73109=ORIENTED_EDGE('',*,*,#49842,.F.) ;
#73110=ORIENTED_EDGE('',*,*,#52278,.T.) ;
#73111=ORIENTED_EDGE('',*,*,#52279,.T.) ;
#73112=ORIENTED_EDGE('',*,*,#50697,.F.) ;
#73113=ORIENTED_EDGE('',*,*,#52280,.T.) ;
#73114=ORIENTED_EDGE('',*,*,#52281,.T.) ;
#73115=ORIENTED_EDGE('',*,*,#49840,.F.) ;
#73116=ORIENTED_EDGE('',*,*,#52282,.T.) ;
#73117=ORIENTED_EDGE('',*,*,#52283,.T.) ;
#73118=ORIENTED_EDGE('',*,*,#50705,.F.) ;
#73119=ORIENTED_EDGE('',*,*,#52284,.T.) ;
#73120=ORIENTED_EDGE('',*,*,#52285,.T.) ;
#73121=ORIENTED_EDGE('',*,*,#49841,.F.) ;
#73122=ORIENTED_EDGE('',*,*,#52286,.T.) ;
#73123=ORIENTED_EDGE('',*,*,#52287,.T.) ;
#73124=ORIENTED_EDGE('',*,*,#50709,.F.) ;
#73125=ORIENTED_EDGE('',*,*,#52288,.T.) ;
#73126=ORIENTED_EDGE('',*,*,#52289,.T.) ;
#73127=ORIENTED_EDGE('',*,*,#50719,.F.) ;
#73128=ORIENTED_EDGE('',*,*,#52290,.T.) ;
#73129=ORIENTED_EDGE('',*,*,#52291,.T.) ;
#73130=ORIENTED_EDGE('',*,*,#49847,.F.) ;
#73131=ORIENTED_EDGE('',*,*,#52292,.T.) ;
#73132=ORIENTED_EDGE('',*,*,#52293,.T.) ;
#73133=ORIENTED_EDGE('',*,*,#49846,.F.) ;
#73134=ORIENTED_EDGE('',*,*,#52294,.T.) ;
#73135=ORIENTED_EDGE('',*,*,#52295,.T.) ;
#73136=ORIENTED_EDGE('',*,*,#50713,.F.) ;
#73137=ORIENTED_EDGE('',*,*,#52296,.T.) ;
#73138=ORIENTED_EDGE('',*,*,#52297,.T.) ;
#73139=ORIENTED_EDGE('',*,*,#49844,.F.) ;
#73140=ORIENTED_EDGE('',*,*,#52298,.T.) ;
#73141=ORIENTED_EDGE('',*,*,#52299,.T.) ;
#73142=ORIENTED_EDGE('',*,*,#50721,.F.) ;
#73143=ORIENTED_EDGE('',*,*,#52300,.T.) ;
#73144=ORIENTED_EDGE('',*,*,#52301,.T.) ;
#73145=ORIENTED_EDGE('',*,*,#49845,.F.) ;
#73146=ORIENTED_EDGE('',*,*,#52302,.T.) ;
#73147=ORIENTED_EDGE('',*,*,#52303,.T.) ;
#73148=ORIENTED_EDGE('',*,*,#50725,.F.) ;
#73149=ORIENTED_EDGE('',*,*,#52304,.T.) ;
#73150=ORIENTED_EDGE('',*,*,#52305,.T.) ;
#73151=ORIENTED_EDGE('',*,*,#50735,.F.) ;
#73152=ORIENTED_EDGE('',*,*,#52306,.T.) ;
#73153=ORIENTED_EDGE('',*,*,#52307,.T.) ;
#73154=ORIENTED_EDGE('',*,*,#49851,.F.) ;
#73155=ORIENTED_EDGE('',*,*,#52308,.T.) ;
#73156=ORIENTED_EDGE('',*,*,#52309,.T.) ;
#73157=ORIENTED_EDGE('',*,*,#49850,.F.) ;
#73158=ORIENTED_EDGE('',*,*,#52310,.T.) ;
#73159=ORIENTED_EDGE('',*,*,#52311,.T.) ;
#73160=ORIENTED_EDGE('',*,*,#50729,.F.) ;
#73161=ORIENTED_EDGE('',*,*,#52312,.T.) ;
#73162=ORIENTED_EDGE('',*,*,#52313,.T.) ;
#73163=ORIENTED_EDGE('',*,*,#49848,.F.) ;
#73164=ORIENTED_EDGE('',*,*,#52314,.T.) ;
#73165=ORIENTED_EDGE('',*,*,#52315,.T.) ;
#73166=ORIENTED_EDGE('',*,*,#50737,.F.) ;
#73167=ORIENTED_EDGE('',*,*,#52316,.T.) ;
#73168=ORIENTED_EDGE('',*,*,#52317,.T.) ;
#73169=ORIENTED_EDGE('',*,*,#49849,.F.) ;
#73170=ORIENTED_EDGE('',*,*,#52318,.T.) ;
#73171=ORIENTED_EDGE('',*,*,#52319,.T.) ;
#73172=ORIENTED_EDGE('',*,*,#50741,.F.) ;
#73173=ORIENTED_EDGE('',*,*,#52320,.T.) ;
#73174=ORIENTED_EDGE('',*,*,#52321,.T.) ;
#73175=ORIENTED_EDGE('',*,*,#50751,.F.) ;
#73176=ORIENTED_EDGE('',*,*,#52322,.T.) ;
#73177=ORIENTED_EDGE('',*,*,#52323,.T.) ;
#73178=ORIENTED_EDGE('',*,*,#49855,.F.) ;
#73179=ORIENTED_EDGE('',*,*,#52324,.T.) ;
#73180=ORIENTED_EDGE('',*,*,#52325,.T.) ;
#73181=ORIENTED_EDGE('',*,*,#49854,.F.) ;
#73182=ORIENTED_EDGE('',*,*,#52326,.T.) ;
#73183=ORIENTED_EDGE('',*,*,#52327,.T.) ;
#73184=ORIENTED_EDGE('',*,*,#50745,.F.) ;
#73185=ORIENTED_EDGE('',*,*,#52328,.T.) ;
#73186=ORIENTED_EDGE('',*,*,#52329,.T.) ;
#73187=ORIENTED_EDGE('',*,*,#49852,.F.) ;
#73188=ORIENTED_EDGE('',*,*,#52330,.T.) ;
#73189=ORIENTED_EDGE('',*,*,#52331,.T.) ;
#73190=ORIENTED_EDGE('',*,*,#50753,.F.) ;
#73191=ORIENTED_EDGE('',*,*,#52332,.T.) ;
#73192=ORIENTED_EDGE('',*,*,#52333,.T.) ;
#73193=ORIENTED_EDGE('',*,*,#49853,.F.) ;
#73194=ORIENTED_EDGE('',*,*,#52334,.T.) ;
#73195=ORIENTED_EDGE('',*,*,#52335,.T.) ;
#73196=ORIENTED_EDGE('',*,*,#50757,.F.) ;
#73197=ORIENTED_EDGE('',*,*,#52336,.T.) ;
#73198=ORIENTED_EDGE('',*,*,#52337,.T.) ;
#73199=ORIENTED_EDGE('',*,*,#50767,.F.) ;
#73200=ORIENTED_EDGE('',*,*,#52338,.T.) ;
#73201=ORIENTED_EDGE('',*,*,#52339,.T.) ;
#73202=ORIENTED_EDGE('',*,*,#49859,.F.) ;
#73203=ORIENTED_EDGE('',*,*,#52340,.T.) ;
#73204=ORIENTED_EDGE('',*,*,#52341,.T.) ;
#73205=ORIENTED_EDGE('',*,*,#49858,.F.) ;
#73206=ORIENTED_EDGE('',*,*,#52342,.T.) ;
#73207=ORIENTED_EDGE('',*,*,#52343,.T.) ;
#73208=ORIENTED_EDGE('',*,*,#50761,.F.) ;
#73209=ORIENTED_EDGE('',*,*,#52344,.T.) ;
#73210=ORIENTED_EDGE('',*,*,#52345,.T.) ;
#73211=ORIENTED_EDGE('',*,*,#49856,.F.) ;
#73212=ORIENTED_EDGE('',*,*,#52346,.T.) ;
#73213=ORIENTED_EDGE('',*,*,#52347,.T.) ;
#73214=ORIENTED_EDGE('',*,*,#50769,.F.) ;
#73215=ORIENTED_EDGE('',*,*,#52348,.T.) ;
#73216=ORIENTED_EDGE('',*,*,#52349,.T.) ;
#73217=ORIENTED_EDGE('',*,*,#49857,.F.) ;
#73218=ORIENTED_EDGE('',*,*,#52350,.T.) ;
#73219=ORIENTED_EDGE('',*,*,#52351,.T.) ;
#73220=ORIENTED_EDGE('',*,*,#50773,.F.) ;
#73221=ORIENTED_EDGE('',*,*,#52352,.T.) ;
#73222=ORIENTED_EDGE('',*,*,#52353,.T.) ;
#73223=ORIENTED_EDGE('',*,*,#50783,.F.) ;
#73224=ORIENTED_EDGE('',*,*,#52354,.T.) ;
#73225=ORIENTED_EDGE('',*,*,#52355,.T.) ;
#73226=ORIENTED_EDGE('',*,*,#49863,.F.) ;
#73227=ORIENTED_EDGE('',*,*,#52356,.T.) ;
#73228=ORIENTED_EDGE('',*,*,#52357,.T.) ;
#73229=ORIENTED_EDGE('',*,*,#49862,.F.) ;
#73230=ORIENTED_EDGE('',*,*,#52358,.T.) ;
#73231=ORIENTED_EDGE('',*,*,#52359,.T.) ;
#73232=ORIENTED_EDGE('',*,*,#50777,.F.) ;
#73233=ORIENTED_EDGE('',*,*,#52360,.T.) ;
#73234=ORIENTED_EDGE('',*,*,#52361,.T.) ;
#73235=ORIENTED_EDGE('',*,*,#49860,.F.) ;
#73236=ORIENTED_EDGE('',*,*,#52362,.T.) ;
#73237=ORIENTED_EDGE('',*,*,#52363,.T.) ;
#73238=ORIENTED_EDGE('',*,*,#50785,.F.) ;
#73239=ORIENTED_EDGE('',*,*,#52364,.T.) ;
#73240=ORIENTED_EDGE('',*,*,#52365,.T.) ;
#73241=ORIENTED_EDGE('',*,*,#49861,.F.) ;
#73242=ORIENTED_EDGE('',*,*,#52366,.T.) ;
#73243=ORIENTED_EDGE('',*,*,#52367,.T.) ;
#73244=ORIENTED_EDGE('',*,*,#50789,.F.) ;
#73245=ORIENTED_EDGE('',*,*,#52368,.T.) ;
#73246=ORIENTED_EDGE('',*,*,#52369,.T.) ;
#73247=ORIENTED_EDGE('',*,*,#50799,.F.) ;
#73248=ORIENTED_EDGE('',*,*,#52370,.T.) ;
#73249=ORIENTED_EDGE('',*,*,#52371,.T.) ;
#73250=ORIENTED_EDGE('',*,*,#49867,.F.) ;
#73251=ORIENTED_EDGE('',*,*,#52372,.T.) ;
#73252=ORIENTED_EDGE('',*,*,#52373,.T.) ;
#73253=ORIENTED_EDGE('',*,*,#49866,.F.) ;
#73254=ORIENTED_EDGE('',*,*,#52374,.T.) ;
#73255=ORIENTED_EDGE('',*,*,#52375,.T.) ;
#73256=ORIENTED_EDGE('',*,*,#50793,.F.) ;
#73257=ORIENTED_EDGE('',*,*,#52376,.T.) ;
#73258=ORIENTED_EDGE('',*,*,#52377,.T.) ;
#73259=ORIENTED_EDGE('',*,*,#49864,.F.) ;
#73260=ORIENTED_EDGE('',*,*,#52378,.T.) ;
#73261=ORIENTED_EDGE('',*,*,#52379,.T.) ;
#73262=ORIENTED_EDGE('',*,*,#50801,.F.) ;
#73263=ORIENTED_EDGE('',*,*,#52380,.T.) ;
#73264=ORIENTED_EDGE('',*,*,#52381,.T.) ;
#73265=ORIENTED_EDGE('',*,*,#49865,.F.) ;
#73266=ORIENTED_EDGE('',*,*,#52382,.T.) ;
#73267=ORIENTED_EDGE('',*,*,#52383,.T.) ;
#73268=ORIENTED_EDGE('',*,*,#50805,.F.) ;
#73269=ORIENTED_EDGE('',*,*,#52384,.T.) ;
#73270=ORIENTED_EDGE('',*,*,#52385,.T.) ;
#73271=ORIENTED_EDGE('',*,*,#52386,.F.) ;
#73272=ORIENTED_EDGE('',*,*,#49873,.F.) ;
#73273=ORIENTED_EDGE('',*,*,#52387,.F.) ;
#73274=ORIENTED_EDGE('',*,*,#50824,.F.) ;
#73275=ORIENTED_EDGE('',*,*,#52387,.T.) ;
#73276=ORIENTED_EDGE('',*,*,#49872,.T.) ;
#73277=ORIENTED_EDGE('',*,*,#52388,.F.) ;
#73278=ORIENTED_EDGE('',*,*,#52389,.F.) ;
#73279=ORIENTED_EDGE('',*,*,#49874,.T.) ;
#73280=ORIENTED_EDGE('',*,*,#52386,.T.) ;
#73281=ORIENTED_EDGE('',*,*,#52390,.F.) ;
#73282=ORIENTED_EDGE('',*,*,#52391,.F.) ;
#73283=ORIENTED_EDGE('',*,*,#52388,.T.) ;
#73284=ORIENTED_EDGE('',*,*,#49871,.F.) ;
#73285=ORIENTED_EDGE('',*,*,#52392,.F.) ;
#73286=ORIENTED_EDGE('',*,*,#50820,.F.) ;
#73287=ORIENTED_EDGE('',*,*,#52389,.T.) ;
#73288=ORIENTED_EDGE('',*,*,#50819,.F.) ;
#73289=ORIENTED_EDGE('',*,*,#52393,.F.) ;
#73290=ORIENTED_EDGE('',*,*,#50821,.F.) ;
#73291=ORIENTED_EDGE('',*,*,#52394,.F.) ;
#73292=ORIENTED_EDGE('',*,*,#50822,.F.) ;
#73293=ORIENTED_EDGE('',*,*,#52395,.F.) ;
#73294=ORIENTED_EDGE('',*,*,#50828,.F.) ;
#73295=ORIENTED_EDGE('',*,*,#52390,.T.) ;
#73296=ORIENTED_EDGE('',*,*,#50823,.F.) ;
#73297=ORIENTED_EDGE('',*,*,#52396,.F.) ;
#73298=ORIENTED_EDGE('',*,*,#50812,.F.) ;
#73299=ORIENTED_EDGE('',*,*,#52391,.T.) ;
#73300=ORIENTED_EDGE('',*,*,#50811,.F.) ;
#73301=ORIENTED_EDGE('',*,*,#52397,.F.) ;
#73302=ORIENTED_EDGE('',*,*,#49875,.F.) ;
#73303=ORIENTED_EDGE('',*,*,#52398,.F.) ;
#73304=ORIENTED_EDGE('',*,*,#49869,.F.) ;
#73305=ORIENTED_EDGE('',*,*,#52399,.F.) ;
#73306=ORIENTED_EDGE('',*,*,#50815,.F.) ;
#73307=ORIENTED_EDGE('',*,*,#49870,.T.) ;
#73308=ORIENTED_EDGE('',*,*,#52398,.T.) ;
#73309=ORIENTED_EDGE('',*,*,#52400,.F.) ;
#73310=ORIENTED_EDGE('',*,*,#52392,.T.) ;
#73311=ORIENTED_EDGE('',*,*,#52395,.T.) ;
#73312=ORIENTED_EDGE('',*,*,#52393,.T.) ;
#73313=ORIENTED_EDGE('',*,*,#52401,.F.) ;
#73314=ORIENTED_EDGE('',*,*,#52396,.T.) ;
#73315=ORIENTED_EDGE('',*,*,#52394,.T.) ;
#73316=ORIENTED_EDGE('',*,*,#52402,.F.) ;
#73317=ORIENTED_EDGE('',*,*,#49868,.T.) ;
#73318=ORIENTED_EDGE('',*,*,#52397,.T.) ;
#73319=ORIENTED_EDGE('',*,*,#52403,.F.) ;
#73320=ORIENTED_EDGE('',*,*,#52399,.T.) ;
#73321=ORIENTED_EDGE('',*,*,#52400,.T.) ;
#73322=ORIENTED_EDGE('',*,*,#50814,.F.) ;
#73323=ORIENTED_EDGE('',*,*,#52404,.F.) ;
#73324=ORIENTED_EDGE('',*,*,#50817,.F.) ;
#73325=ORIENTED_EDGE('',*,*,#52401,.T.) ;
#73326=ORIENTED_EDGE('',*,*,#50818,.F.) ;
#73327=ORIENTED_EDGE('',*,*,#52405,.F.) ;
#73328=ORIENTED_EDGE('',*,*,#50825,.F.) ;
#73329=ORIENTED_EDGE('',*,*,#52402,.T.) ;
#73330=ORIENTED_EDGE('',*,*,#50827,.F.) ;
#73331=ORIENTED_EDGE('',*,*,#52406,.F.) ;
#73332=ORIENTED_EDGE('',*,*,#50809,.F.) ;
#73333=ORIENTED_EDGE('',*,*,#52403,.T.) ;
#73334=ORIENTED_EDGE('',*,*,#50810,.F.) ;
#73335=ORIENTED_EDGE('',*,*,#52407,.F.) ;
#73336=ORIENTED_EDGE('',*,*,#50816,.F.) ;
#73337=ORIENTED_EDGE('',*,*,#52405,.T.) ;
#73338=ORIENTED_EDGE('',*,*,#52404,.T.) ;
#73339=ORIENTED_EDGE('',*,*,#52408,.F.) ;
#73340=ORIENTED_EDGE('',*,*,#52407,.T.) ;
#73341=ORIENTED_EDGE('',*,*,#52406,.T.) ;
#73342=ORIENTED_EDGE('',*,*,#52409,.F.) ;
#73343=ORIENTED_EDGE('',*,*,#52408,.T.) ;
#73344=ORIENTED_EDGE('',*,*,#50813,.F.) ;
#73345=ORIENTED_EDGE('',*,*,#52409,.T.) ;
#73346=ORIENTED_EDGE('',*,*,#50826,.F.) ;
#73347=ORIENTED_EDGE('',*,*,#50834,.F.) ;
#73348=ORIENTED_EDGE('',*,*,#50848,.F.) ;
#73349=ORIENTED_EDGE('',*,*,#52410,.F.) ;
#73350=ORIENTED_EDGE('',*,*,#50837,.F.) ;
#73351=ORIENTED_EDGE('',*,*,#52411,.F.) ;
#73352=ORIENTED_EDGE('',*,*,#50838,.F.) ;
#73353=ORIENTED_EDGE('',*,*,#52412,.F.) ;
#73354=ORIENTED_EDGE('',*,*,#51044,.F.) ;
#73355=ORIENTED_EDGE('',*,*,#50836,.F.) ;
#73356=ORIENTED_EDGE('',*,*,#50839,.F.) ;
#73357=ORIENTED_EDGE('',*,*,#52413,.F.) ;
#73358=ORIENTED_EDGE('',*,*,#50840,.F.) ;
#73359=ORIENTED_EDGE('',*,*,#52412,.T.) ;
#73360=ORIENTED_EDGE('',*,*,#52410,.T.) ;
#73361=ORIENTED_EDGE('',*,*,#52414,.F.) ;
#73362=ORIENTED_EDGE('',*,*,#52413,.T.) ;
#73363=ORIENTED_EDGE('',*,*,#52411,.T.) ;
#73364=ORIENTED_EDGE('',*,*,#52415,.F.) ;
#73365=ORIENTED_EDGE('',*,*,#50832,.F.) ;
#73366=ORIENTED_EDGE('',*,*,#50844,.F.) ;
#73367=ORIENTED_EDGE('',*,*,#52416,.F.) ;
#73368=ORIENTED_EDGE('',*,*,#50846,.F.) ;
#73369=ORIENTED_EDGE('',*,*,#52414,.T.) ;
#73370=ORIENTED_EDGE('',*,*,#50847,.F.) ;
#73371=ORIENTED_EDGE('',*,*,#52417,.F.) ;
#73372=ORIENTED_EDGE('',*,*,#51041,.F.) ;
#73373=ORIENTED_EDGE('',*,*,#52415,.T.) ;
#73374=ORIENTED_EDGE('',*,*,#51043,.F.) ;
#73375=ORIENTED_EDGE('',*,*,#52418,.F.) ;
#73376=ORIENTED_EDGE('',*,*,#50841,.F.) ;
#73377=ORIENTED_EDGE('',*,*,#50830,.F.) ;
#73378=ORIENTED_EDGE('',*,*,#50842,.F.) ;
#73379=ORIENTED_EDGE('',*,*,#52419,.F.) ;
#73380=ORIENTED_EDGE('',*,*,#50845,.F.) ;
#73381=ORIENTED_EDGE('',*,*,#52417,.T.) ;
#73382=ORIENTED_EDGE('',*,*,#52416,.T.) ;
#73383=ORIENTED_EDGE('',*,*,#52420,.F.) ;
#73384=ORIENTED_EDGE('',*,*,#52419,.T.) ;
#73385=ORIENTED_EDGE('',*,*,#52418,.T.) ;
#73386=ORIENTED_EDGE('',*,*,#52421,.F.) ;
#73387=ORIENTED_EDGE('',*,*,#52420,.T.) ;
#73388=ORIENTED_EDGE('',*,*,#50843,.F.) ;
#73389=ORIENTED_EDGE('',*,*,#52421,.T.) ;
#73390=ORIENTED_EDGE('',*,*,#51042,.F.) ;
#73391=ORIENTED_EDGE('',*,*,#52422,.F.) ;
#73392=ORIENTED_EDGE('',*,*,#50544,.F.) ;
#73393=ORIENTED_EDGE('',*,*,#50550,.F.) ;
#73394=ORIENTED_EDGE('',*,*,#50621,.F.) ;
#73395=ORIENTED_EDGE('',*,*,#52423,.F.) ;
#73396=ORIENTED_EDGE('',*,*,#52422,.T.) ;
#73397=ORIENTED_EDGE('',*,*,#52424,.F.) ;
#73398=ORIENTED_EDGE('',*,*,#52424,.T.) ;
#73399=ORIENTED_EDGE('',*,*,#50620,.F.) ;
#73400=ORIENTED_EDGE('',*,*,#52425,.F.) ;
#73401=ORIENTED_EDGE('',*,*,#50539,.F.) ;
#73402=ORIENTED_EDGE('',*,*,#52423,.T.) ;
#73403=ORIENTED_EDGE('',*,*,#50538,.F.) ;
#73404=ORIENTED_EDGE('',*,*,#52426,.F.) ;
#73405=ORIENTED_EDGE('',*,*,#50541,.F.) ;
#73406=ORIENTED_EDGE('',*,*,#50551,.F.) ;
#73407=ORIENTED_EDGE('',*,*,#50542,.F.) ;
#73408=ORIENTED_EDGE('',*,*,#52427,.F.) ;
#73409=ORIENTED_EDGE('',*,*,#50561,.F.) ;
#73410=ORIENTED_EDGE('',*,*,#52428,.F.) ;
#73411=ORIENTED_EDGE('',*,*,#52425,.T.) ;
#73412=ORIENTED_EDGE('',*,*,#52429,.F.) ;
#73413=ORIENTED_EDGE('',*,*,#49752,.T.) ;
#73414=ORIENTED_EDGE('',*,*,#52427,.T.) ;
#73415=ORIENTED_EDGE('',*,*,#52426,.T.) ;
#73416=ORIENTED_EDGE('',*,*,#52430,.F.) ;
#73417=ORIENTED_EDGE('',*,*,#50548,.F.) ;
#73418=ORIENTED_EDGE('',*,*,#50554,.F.) ;
#73419=ORIENTED_EDGE('',*,*,#52431,.F.) ;
#73420=ORIENTED_EDGE('',*,*,#50622,.F.) ;
#73421=ORIENTED_EDGE('',*,*,#52432,.F.) ;
#73422=ORIENTED_EDGE('',*,*,#50623,.F.) ;
#73423=ORIENTED_EDGE('',*,*,#52433,.F.) ;
#73424=ORIENTED_EDGE('',*,*,#50558,.F.) ;
#73425=ORIENTED_EDGE('',*,*,#52429,.T.) ;
#73426=ORIENTED_EDGE('',*,*,#50624,.F.) ;
#73427=ORIENTED_EDGE('',*,*,#52434,.F.) ;
#73428=ORIENTED_EDGE('',*,*,#49753,.F.) ;
#73429=ORIENTED_EDGE('',*,*,#52428,.T.) ;
#73430=ORIENTED_EDGE('',*,*,#49751,.F.) ;
#73431=ORIENTED_EDGE('',*,*,#52435,.F.) ;
#73432=ORIENTED_EDGE('',*,*,#50540,.F.) ;
#73433=ORIENTED_EDGE('',*,*,#52430,.T.) ;
#73434=ORIENTED_EDGE('',*,*,#50537,.F.) ;
#73435=ORIENTED_EDGE('',*,*,#52436,.F.) ;
#73436=ORIENTED_EDGE('',*,*,#50562,.F.) ;
#73437=ORIENTED_EDGE('',*,*,#52433,.T.) ;
#73438=ORIENTED_EDGE('',*,*,#52431,.T.) ;
#73439=ORIENTED_EDGE('',*,*,#52437,.F.) ;
#73440=ORIENTED_EDGE('',*,*,#52434,.T.) ;
#73441=ORIENTED_EDGE('',*,*,#52432,.T.) ;
#73442=ORIENTED_EDGE('',*,*,#52438,.F.) ;
#73443=ORIENTED_EDGE('',*,*,#49754,.T.) ;
#73444=ORIENTED_EDGE('',*,*,#52435,.T.) ;
#73445=ORIENTED_EDGE('',*,*,#49750,.T.) ;
#73446=ORIENTED_EDGE('',*,*,#52439,.F.) ;
#73447=ORIENTED_EDGE('',*,*,#52436,.T.) ;
#73448=ORIENTED_EDGE('',*,*,#50546,.F.) ;
#73449=ORIENTED_EDGE('',*,*,#50560,.F.) ;
#73450=ORIENTED_EDGE('',*,*,#52440,.F.) ;
#73451=ORIENTED_EDGE('',*,*,#50552,.F.) ;
#73452=ORIENTED_EDGE('',*,*,#52437,.T.) ;
#73453=ORIENTED_EDGE('',*,*,#50553,.F.) ;
#73454=ORIENTED_EDGE('',*,*,#52441,.F.) ;
#73455=ORIENTED_EDGE('',*,*,#50555,.F.) ;
#73456=ORIENTED_EDGE('',*,*,#52438,.T.) ;
#73457=ORIENTED_EDGE('',*,*,#50557,.F.) ;
#73458=ORIENTED_EDGE('',*,*,#52442,.F.) ;
#73459=ORIENTED_EDGE('',*,*,#49755,.F.) ;
#73460=ORIENTED_EDGE('',*,*,#52439,.T.) ;
#73461=ORIENTED_EDGE('',*,*,#49749,.F.) ;
#73462=ORIENTED_EDGE('',*,*,#52443,.F.) ;
#73463=ORIENTED_EDGE('',*,*,#50563,.F.) ;
#73464=ORIENTED_EDGE('',*,*,#52441,.T.) ;
#73465=ORIENTED_EDGE('',*,*,#52440,.T.) ;
#73466=ORIENTED_EDGE('',*,*,#52444,.F.) ;
#73467=ORIENTED_EDGE('',*,*,#49748,.T.) ;
#73468=ORIENTED_EDGE('',*,*,#52442,.T.) ;
#73469=ORIENTED_EDGE('',*,*,#52445,.F.) ;
#73470=ORIENTED_EDGE('',*,*,#52443,.T.) ;
#73471=ORIENTED_EDGE('',*,*,#52444,.T.) ;
#73472=ORIENTED_EDGE('',*,*,#50559,.F.) ;
#73473=ORIENTED_EDGE('',*,*,#52445,.T.) ;
#73474=ORIENTED_EDGE('',*,*,#50556,.F.) ;
#73475=ORIENTED_EDGE('',*,*,#49759,.F.) ;
#73476=ORIENTED_EDGE('',*,*,#52446,.T.) ;
#73477=ORIENTED_EDGE('',*,*,#52447,.T.) ;
#73478=ORIENTED_EDGE('',*,*,#50533,.F.) ;
#73479=ORIENTED_EDGE('',*,*,#52448,.T.) ;
#73480=ORIENTED_EDGE('',*,*,#52449,.T.) ;
#73481=ORIENTED_EDGE('',*,*,#52450,.T.) ;
#73482=ORIENTED_EDGE('',*,*,#49756,.F.) ;
#73483=ORIENTED_EDGE('',*,*,#52451,.T.) ;
#73484=ORIENTED_EDGE('',*,*,#52452,.T.) ;
#73485=ORIENTED_EDGE('',*,*,#50564,.F.) ;
#73486=ORIENTED_EDGE('',*,*,#52453,.T.) ;
#73487=ORIENTED_EDGE('',*,*,#52454,.T.) ;
#73488=ORIENTED_EDGE('',*,*,#50625,.F.) ;
#73489=ORIENTED_EDGE('',*,*,#52455,.T.) ;
#73490=ORIENTED_EDGE('',*,*,#49758,.F.) ;
#73491=ORIENTED_EDGE('',*,*,#52456,.T.) ;
#73492=ORIENTED_EDGE('',*,*,#49757,.F.) ;
#73493=ORIENTED_EDGE('',*,*,#52457,.T.) ;
#73494=ORIENTED_EDGE('',*,*,#52458,.T.) ;
#73495=ORIENTED_EDGE('',*,*,#52459,.T.) ;
#73496=ORIENTED_EDGE('',*,*,#50515,.F.) ;
#73497=ORIENTED_EDGE('',*,*,#52460,.T.) ;
#73498=ORIENTED_EDGE('',*,*,#52461,.T.) ;
#73499=ORIENTED_EDGE('',*,*,#49763,.F.) ;
#73500=ORIENTED_EDGE('',*,*,#52462,.T.) ;
#73501=ORIENTED_EDGE('',*,*,#52463,.T.) ;
#73502=ORIENTED_EDGE('',*,*,#50511,.F.) ;
#73503=ORIENTED_EDGE('',*,*,#52464,.T.) ;
#73504=ORIENTED_EDGE('',*,*,#52465,.T.) ;
#73505=ORIENTED_EDGE('',*,*,#52466,.T.) ;
#73506=ORIENTED_EDGE('',*,*,#49760,.F.) ;
#73507=ORIENTED_EDGE('',*,*,#52467,.T.) ;
#73508=ORIENTED_EDGE('',*,*,#52468,.T.) ;
#73509=ORIENTED_EDGE('',*,*,#50571,.F.) ;
#73510=ORIENTED_EDGE('',*,*,#52469,.T.) ;
#73511=ORIENTED_EDGE('',*,*,#52470,.T.) ;
#73512=ORIENTED_EDGE('',*,*,#50632,.F.) ;
#73513=ORIENTED_EDGE('',*,*,#52471,.T.) ;
#73514=ORIENTED_EDGE('',*,*,#49762,.F.) ;
#73515=ORIENTED_EDGE('',*,*,#52472,.T.) ;
#73516=ORIENTED_EDGE('',*,*,#49761,.F.) ;
#73517=ORIENTED_EDGE('',*,*,#52473,.T.) ;
#73518=ORIENTED_EDGE('',*,*,#52474,.T.) ;
#73519=ORIENTED_EDGE('',*,*,#52475,.T.) ;
#73520=ORIENTED_EDGE('',*,*,#50493,.F.) ;
#73521=ORIENTED_EDGE('',*,*,#52476,.T.) ;
#73522=ORIENTED_EDGE('',*,*,#52477,.T.) ;
#73523=ORIENTED_EDGE('',*,*,#49767,.F.) ;
#73524=ORIENTED_EDGE('',*,*,#52478,.T.) ;
#73525=ORIENTED_EDGE('',*,*,#52479,.T.) ;
#73526=ORIENTED_EDGE('',*,*,#50489,.F.) ;
#73527=ORIENTED_EDGE('',*,*,#52480,.T.) ;
#73528=ORIENTED_EDGE('',*,*,#52481,.T.) ;
#73529=ORIENTED_EDGE('',*,*,#52482,.T.) ;
#73530=ORIENTED_EDGE('',*,*,#49764,.F.) ;
#73531=ORIENTED_EDGE('',*,*,#52483,.T.) ;
#73532=ORIENTED_EDGE('',*,*,#52484,.T.) ;
#73533=ORIENTED_EDGE('',*,*,#50578,.F.) ;
#73534=ORIENTED_EDGE('',*,*,#52485,.T.) ;
#73535=ORIENTED_EDGE('',*,*,#52486,.T.) ;
#73536=ORIENTED_EDGE('',*,*,#50639,.F.) ;
#73537=ORIENTED_EDGE('',*,*,#52487,.T.) ;
#73538=ORIENTED_EDGE('',*,*,#49766,.F.) ;
#73539=ORIENTED_EDGE('',*,*,#52488,.T.) ;
#73540=ORIENTED_EDGE('',*,*,#49765,.F.) ;
#73541=ORIENTED_EDGE('',*,*,#52489,.T.) ;
#73542=ORIENTED_EDGE('',*,*,#52490,.T.) ;
#73543=ORIENTED_EDGE('',*,*,#52491,.T.) ;
#73544=ORIENTED_EDGE('',*,*,#50471,.F.) ;
#73545=ORIENTED_EDGE('',*,*,#52492,.T.) ;
#73546=ORIENTED_EDGE('',*,*,#52493,.T.) ;
#73547=ORIENTED_EDGE('',*,*,#49771,.F.) ;
#73548=ORIENTED_EDGE('',*,*,#52494,.T.) ;
#73549=ORIENTED_EDGE('',*,*,#52495,.T.) ;
#73550=ORIENTED_EDGE('',*,*,#50467,.F.) ;
#73551=ORIENTED_EDGE('',*,*,#52496,.T.) ;
#73552=ORIENTED_EDGE('',*,*,#52497,.T.) ;
#73553=ORIENTED_EDGE('',*,*,#52498,.T.) ;
#73554=ORIENTED_EDGE('',*,*,#49768,.F.) ;
#73555=ORIENTED_EDGE('',*,*,#52499,.T.) ;
#73556=ORIENTED_EDGE('',*,*,#52500,.T.) ;
#73557=ORIENTED_EDGE('',*,*,#50585,.F.) ;
#73558=ORIENTED_EDGE('',*,*,#52501,.T.) ;
#73559=ORIENTED_EDGE('',*,*,#52502,.T.) ;
#73560=ORIENTED_EDGE('',*,*,#50646,.F.) ;
#73561=ORIENTED_EDGE('',*,*,#52503,.T.) ;
#73562=ORIENTED_EDGE('',*,*,#49770,.F.) ;
#73563=ORIENTED_EDGE('',*,*,#52504,.T.) ;
#73564=ORIENTED_EDGE('',*,*,#49769,.F.) ;
#73565=ORIENTED_EDGE('',*,*,#52505,.T.) ;
#73566=ORIENTED_EDGE('',*,*,#52506,.T.) ;
#73567=ORIENTED_EDGE('',*,*,#52507,.T.) ;
#73568=ORIENTED_EDGE('',*,*,#50449,.F.) ;
#73569=ORIENTED_EDGE('',*,*,#52508,.T.) ;
#73570=ORIENTED_EDGE('',*,*,#52509,.T.) ;
#73571=ORIENTED_EDGE('',*,*,#49775,.F.) ;
#73572=ORIENTED_EDGE('',*,*,#52510,.T.) ;
#73573=ORIENTED_EDGE('',*,*,#52511,.T.) ;
#73574=ORIENTED_EDGE('',*,*,#50445,.F.) ;
#73575=ORIENTED_EDGE('',*,*,#52512,.T.) ;
#73576=ORIENTED_EDGE('',*,*,#52513,.T.) ;
#73577=ORIENTED_EDGE('',*,*,#52514,.T.) ;
#73578=ORIENTED_EDGE('',*,*,#49772,.F.) ;
#73579=ORIENTED_EDGE('',*,*,#52515,.T.) ;
#73580=ORIENTED_EDGE('',*,*,#52516,.T.) ;
#73581=ORIENTED_EDGE('',*,*,#50592,.F.) ;
#73582=ORIENTED_EDGE('',*,*,#52517,.T.) ;
#73583=ORIENTED_EDGE('',*,*,#52518,.T.) ;
#73584=ORIENTED_EDGE('',*,*,#50653,.F.) ;
#73585=ORIENTED_EDGE('',*,*,#52519,.T.) ;
#73586=ORIENTED_EDGE('',*,*,#49774,.F.) ;
#73587=ORIENTED_EDGE('',*,*,#52520,.T.) ;
#73588=ORIENTED_EDGE('',*,*,#49773,.F.) ;
#73589=ORIENTED_EDGE('',*,*,#52521,.T.) ;
#73590=ORIENTED_EDGE('',*,*,#52522,.T.) ;
#73591=ORIENTED_EDGE('',*,*,#52523,.T.) ;
#73592=ORIENTED_EDGE('',*,*,#50427,.F.) ;
#73593=ORIENTED_EDGE('',*,*,#52524,.T.) ;
#73594=ORIENTED_EDGE('',*,*,#52525,.T.) ;
#73595=ORIENTED_EDGE('',*,*,#49779,.F.) ;
#73596=ORIENTED_EDGE('',*,*,#52526,.T.) ;
#73597=ORIENTED_EDGE('',*,*,#52527,.T.) ;
#73598=ORIENTED_EDGE('',*,*,#50423,.F.) ;
#73599=ORIENTED_EDGE('',*,*,#52528,.T.) ;
#73600=ORIENTED_EDGE('',*,*,#52529,.T.) ;
#73601=ORIENTED_EDGE('',*,*,#52530,.T.) ;
#73602=ORIENTED_EDGE('',*,*,#49776,.F.) ;
#73603=ORIENTED_EDGE('',*,*,#52531,.T.) ;
#73604=ORIENTED_EDGE('',*,*,#52532,.T.) ;
#73605=ORIENTED_EDGE('',*,*,#50599,.F.) ;
#73606=ORIENTED_EDGE('',*,*,#52533,.T.) ;
#73607=ORIENTED_EDGE('',*,*,#52534,.T.) ;
#73608=ORIENTED_EDGE('',*,*,#50660,.F.) ;
#73609=ORIENTED_EDGE('',*,*,#52535,.T.) ;
#73610=ORIENTED_EDGE('',*,*,#49778,.F.) ;
#73611=ORIENTED_EDGE('',*,*,#52536,.T.) ;
#73612=ORIENTED_EDGE('',*,*,#49777,.F.) ;
#73613=ORIENTED_EDGE('',*,*,#52537,.T.) ;
#73614=ORIENTED_EDGE('',*,*,#52538,.T.) ;
#73615=ORIENTED_EDGE('',*,*,#52539,.T.) ;
#73616=ORIENTED_EDGE('',*,*,#50405,.F.) ;
#73617=ORIENTED_EDGE('',*,*,#52540,.T.) ;
#73618=ORIENTED_EDGE('',*,*,#52541,.T.) ;
#73619=ORIENTED_EDGE('',*,*,#49783,.F.) ;
#73620=ORIENTED_EDGE('',*,*,#52542,.T.) ;
#73621=ORIENTED_EDGE('',*,*,#52543,.T.) ;
#73622=ORIENTED_EDGE('',*,*,#50401,.F.) ;
#73623=ORIENTED_EDGE('',*,*,#52544,.T.) ;
#73624=ORIENTED_EDGE('',*,*,#52545,.T.) ;
#73625=ORIENTED_EDGE('',*,*,#52546,.T.) ;
#73626=ORIENTED_EDGE('',*,*,#49780,.F.) ;
#73627=ORIENTED_EDGE('',*,*,#52547,.T.) ;
#73628=ORIENTED_EDGE('',*,*,#52548,.T.) ;
#73629=ORIENTED_EDGE('',*,*,#50606,.F.) ;
#73630=ORIENTED_EDGE('',*,*,#52549,.T.) ;
#73631=ORIENTED_EDGE('',*,*,#52550,.T.) ;
#73632=ORIENTED_EDGE('',*,*,#50667,.F.) ;
#73633=ORIENTED_EDGE('',*,*,#52551,.T.) ;
#73634=ORIENTED_EDGE('',*,*,#49782,.F.) ;
#73635=ORIENTED_EDGE('',*,*,#52552,.T.) ;
#73636=ORIENTED_EDGE('',*,*,#49781,.F.) ;
#73637=ORIENTED_EDGE('',*,*,#52553,.T.) ;
#73638=ORIENTED_EDGE('',*,*,#52554,.T.) ;
#73639=ORIENTED_EDGE('',*,*,#52555,.T.) ;
#73640=ORIENTED_EDGE('',*,*,#50383,.F.) ;
#73641=ORIENTED_EDGE('',*,*,#52556,.T.) ;
#73642=ORIENTED_EDGE('',*,*,#52557,.T.) ;
#73643=ORIENTED_EDGE('',*,*,#49787,.F.) ;
#73644=ORIENTED_EDGE('',*,*,#52558,.T.) ;
#73645=ORIENTED_EDGE('',*,*,#52559,.T.) ;
#73646=ORIENTED_EDGE('',*,*,#50379,.F.) ;
#73647=ORIENTED_EDGE('',*,*,#52560,.T.) ;
#73648=ORIENTED_EDGE('',*,*,#52561,.T.) ;
#73649=ORIENTED_EDGE('',*,*,#52562,.T.) ;
#73650=ORIENTED_EDGE('',*,*,#49784,.F.) ;
#73651=ORIENTED_EDGE('',*,*,#52563,.T.) ;
#73652=ORIENTED_EDGE('',*,*,#52564,.T.) ;
#73653=ORIENTED_EDGE('',*,*,#50613,.F.) ;
#73654=ORIENTED_EDGE('',*,*,#52565,.T.) ;
#73655=ORIENTED_EDGE('',*,*,#52566,.T.) ;
#73656=ORIENTED_EDGE('',*,*,#50674,.F.) ;
#73657=ORIENTED_EDGE('',*,*,#52567,.T.) ;
#73658=ORIENTED_EDGE('',*,*,#49786,.F.) ;
#73659=ORIENTED_EDGE('',*,*,#52568,.T.) ;
#73660=ORIENTED_EDGE('',*,*,#49785,.F.) ;
#73661=ORIENTED_EDGE('',*,*,#52569,.T.) ;
#73662=ORIENTED_EDGE('',*,*,#52570,.T.) ;
#73663=ORIENTED_EDGE('',*,*,#52571,.T.) ;
#73664=ORIENTED_EDGE('',*,*,#50361,.F.) ;
#73665=ORIENTED_EDGE('',*,*,#52572,.T.) ;
#73666=ORIENTED_EDGE('',*,*,#52573,.T.) ;
#73667=ORIENTED_EDGE('',*,*,#52574,.F.) ;
#73668=ORIENTED_EDGE('',*,*,#49380,.F.) ;
#73669=ORIENTED_EDGE('',*,*,#52575,.F.) ;
#73670=ORIENTED_EDGE('',*,*,#51633,.F.) ;
#73671=ORIENTED_EDGE('',*,*,#52575,.T.) ;
#73672=ORIENTED_EDGE('',*,*,#49379,.T.) ;
#73673=ORIENTED_EDGE('',*,*,#52576,.F.) ;
#73674=ORIENTED_EDGE('',*,*,#52577,.F.) ;
#73675=ORIENTED_EDGE('',*,*,#49381,.T.) ;
#73676=ORIENTED_EDGE('',*,*,#52574,.T.) ;
#73677=ORIENTED_EDGE('',*,*,#52578,.F.) ;
#73678=ORIENTED_EDGE('',*,*,#52579,.F.) ;
#73679=ORIENTED_EDGE('',*,*,#52576,.T.) ;
#73680=ORIENTED_EDGE('',*,*,#49378,.F.) ;
#73681=ORIENTED_EDGE('',*,*,#52580,.F.) ;
#73682=ORIENTED_EDGE('',*,*,#51630,.F.) ;
#73683=ORIENTED_EDGE('',*,*,#52577,.T.) ;
#73684=ORIENTED_EDGE('',*,*,#51629,.F.) ;
#73685=ORIENTED_EDGE('',*,*,#52581,.F.) ;
#73686=ORIENTED_EDGE('',*,*,#51634,.F.) ;
#73687=ORIENTED_EDGE('',*,*,#52582,.F.) ;
#73688=ORIENTED_EDGE('',*,*,#51631,.F.) ;
#73689=ORIENTED_EDGE('',*,*,#52583,.F.) ;
#73690=ORIENTED_EDGE('',*,*,#51638,.F.) ;
#73691=ORIENTED_EDGE('',*,*,#52578,.T.) ;
#73692=ORIENTED_EDGE('',*,*,#51632,.F.) ;
#73693=ORIENTED_EDGE('',*,*,#52584,.F.) ;
#73694=ORIENTED_EDGE('',*,*,#51622,.F.) ;
#73695=ORIENTED_EDGE('',*,*,#52579,.T.) ;
#73696=ORIENTED_EDGE('',*,*,#51621,.F.) ;
#73697=ORIENTED_EDGE('',*,*,#52585,.F.) ;
#73698=ORIENTED_EDGE('',*,*,#49382,.F.) ;
#73699=ORIENTED_EDGE('',*,*,#52586,.F.) ;
#73700=ORIENTED_EDGE('',*,*,#49376,.F.) ;
#73701=ORIENTED_EDGE('',*,*,#52587,.F.) ;
#73702=ORIENTED_EDGE('',*,*,#51623,.F.) ;
#73703=ORIENTED_EDGE('',*,*,#49377,.T.) ;
#73704=ORIENTED_EDGE('',*,*,#52586,.T.) ;
#73705=ORIENTED_EDGE('',*,*,#52588,.F.) ;
#73706=ORIENTED_EDGE('',*,*,#52580,.T.) ;
#73707=ORIENTED_EDGE('',*,*,#52583,.T.) ;
#73708=ORIENTED_EDGE('',*,*,#52581,.T.) ;
#73709=ORIENTED_EDGE('',*,*,#52589,.F.) ;
#73710=ORIENTED_EDGE('',*,*,#52584,.T.) ;
#73711=ORIENTED_EDGE('',*,*,#52582,.T.) ;
#73712=ORIENTED_EDGE('',*,*,#52590,.F.) ;
#73713=ORIENTED_EDGE('',*,*,#49375,.T.) ;
#73714=ORIENTED_EDGE('',*,*,#52585,.T.) ;
#73715=ORIENTED_EDGE('',*,*,#52591,.F.) ;
#73716=ORIENTED_EDGE('',*,*,#52587,.T.) ;
#73717=ORIENTED_EDGE('',*,*,#52588,.T.) ;
#73718=ORIENTED_EDGE('',*,*,#51626,.F.) ;
#73719=ORIENTED_EDGE('',*,*,#52592,.F.) ;
#73720=ORIENTED_EDGE('',*,*,#51627,.F.) ;
#73721=ORIENTED_EDGE('',*,*,#52589,.T.) ;
#73722=ORIENTED_EDGE('',*,*,#51628,.F.) ;
#73723=ORIENTED_EDGE('',*,*,#52593,.F.) ;
#73724=ORIENTED_EDGE('',*,*,#51635,.F.) ;
#73725=ORIENTED_EDGE('',*,*,#52590,.T.) ;
#73726=ORIENTED_EDGE('',*,*,#51637,.F.) ;
#73727=ORIENTED_EDGE('',*,*,#52594,.F.) ;
#73728=ORIENTED_EDGE('',*,*,#51619,.F.) ;
#73729=ORIENTED_EDGE('',*,*,#52591,.T.) ;
#73730=ORIENTED_EDGE('',*,*,#51620,.F.) ;
#73731=ORIENTED_EDGE('',*,*,#52595,.F.) ;
#73732=ORIENTED_EDGE('',*,*,#51624,.F.) ;
#73733=ORIENTED_EDGE('',*,*,#52593,.T.) ;
#73734=ORIENTED_EDGE('',*,*,#52592,.T.) ;
#73735=ORIENTED_EDGE('',*,*,#52596,.F.) ;
#73736=ORIENTED_EDGE('',*,*,#52595,.T.) ;
#73737=ORIENTED_EDGE('',*,*,#52594,.T.) ;
#73738=ORIENTED_EDGE('',*,*,#52597,.F.) ;
#73739=ORIENTED_EDGE('',*,*,#52596,.T.) ;
#73740=ORIENTED_EDGE('',*,*,#51625,.F.) ;
#73741=ORIENTED_EDGE('',*,*,#52597,.T.) ;
#73742=ORIENTED_EDGE('',*,*,#51636,.F.) ;
#73743=ORIENTED_EDGE('',*,*,#51644,.F.) ;
#73744=ORIENTED_EDGE('',*,*,#51657,.F.) ;
#73745=ORIENTED_EDGE('',*,*,#52598,.F.) ;
#73746=ORIENTED_EDGE('',*,*,#51649,.F.) ;
#73747=ORIENTED_EDGE('',*,*,#52599,.F.) ;
#73748=ORIENTED_EDGE('',*,*,#51647,.F.) ;
#73749=ORIENTED_EDGE('',*,*,#52600,.F.) ;
#73750=ORIENTED_EDGE('',*,*,#51854,.F.) ;
#73751=ORIENTED_EDGE('',*,*,#51646,.F.) ;
#73752=ORIENTED_EDGE('',*,*,#51648,.F.) ;
#73753=ORIENTED_EDGE('',*,*,#52601,.F.) ;
#73754=ORIENTED_EDGE('',*,*,#51652,.F.) ;
#73755=ORIENTED_EDGE('',*,*,#52600,.T.) ;
#73756=ORIENTED_EDGE('',*,*,#52598,.T.) ;
#73757=ORIENTED_EDGE('',*,*,#52602,.F.) ;
#73758=ORIENTED_EDGE('',*,*,#52601,.T.) ;
#73759=ORIENTED_EDGE('',*,*,#52599,.T.) ;
#73760=ORIENTED_EDGE('',*,*,#52603,.F.) ;
#73761=ORIENTED_EDGE('',*,*,#51642,.F.) ;
#73762=ORIENTED_EDGE('',*,*,#51655,.F.) ;
#73763=ORIENTED_EDGE('',*,*,#52604,.F.) ;
#73764=ORIENTED_EDGE('',*,*,#51658,.F.) ;
#73765=ORIENTED_EDGE('',*,*,#52602,.T.) ;
#73766=ORIENTED_EDGE('',*,*,#51656,.F.) ;
#73767=ORIENTED_EDGE('',*,*,#52605,.F.) ;
#73768=ORIENTED_EDGE('',*,*,#51851,.F.) ;
#73769=ORIENTED_EDGE('',*,*,#52603,.T.) ;
#73770=ORIENTED_EDGE('',*,*,#51853,.F.) ;
#73771=ORIENTED_EDGE('',*,*,#52606,.F.) ;
#73772=ORIENTED_EDGE('',*,*,#51650,.F.) ;
#73773=ORIENTED_EDGE('',*,*,#51640,.F.) ;
#73774=ORIENTED_EDGE('',*,*,#51651,.F.) ;
#73775=ORIENTED_EDGE('',*,*,#52607,.F.) ;
#73776=ORIENTED_EDGE('',*,*,#51653,.F.) ;
#73777=ORIENTED_EDGE('',*,*,#52605,.T.) ;
#73778=ORIENTED_EDGE('',*,*,#52604,.T.) ;
#73779=ORIENTED_EDGE('',*,*,#52608,.F.) ;
#73780=ORIENTED_EDGE('',*,*,#52607,.T.) ;
#73781=ORIENTED_EDGE('',*,*,#52606,.T.) ;
#73782=ORIENTED_EDGE('',*,*,#52609,.F.) ;
#73783=ORIENTED_EDGE('',*,*,#52608,.T.) ;
#73784=ORIENTED_EDGE('',*,*,#51654,.F.) ;
#73785=ORIENTED_EDGE('',*,*,#52609,.T.) ;
#73786=ORIENTED_EDGE('',*,*,#51852,.F.) ;
#73787=ORIENTED_EDGE('',*,*,#52610,.F.) ;
#73788=ORIENTED_EDGE('',*,*,#51962,.F.) ;
#73789=ORIENTED_EDGE('',*,*,#52611,.F.) ;
#73790=ORIENTED_EDGE('',*,*,#51977,.F.) ;
#73791=ORIENTED_EDGE('',*,*,#52611,.T.) ;
#73792=ORIENTED_EDGE('',*,*,#51965,.F.) ;
#73793=ORIENTED_EDGE('',*,*,#52612,.F.) ;
#73794=ORIENTED_EDGE('',*,*,#51959,.F.) ;
#73795=ORIENTED_EDGE('',*,*,#52610,.T.) ;
#73796=ORIENTED_EDGE('',*,*,#52613,.F.) ;
#73797=ORIENTED_EDGE('',*,*,#52612,.T.) ;
#73798=ORIENTED_EDGE('',*,*,#51968,.F.) ;
#73799=ORIENTED_EDGE('',*,*,#52614,.F.) ;
#73800=ORIENTED_EDGE('',*,*,#51974,.F.) ;
#73801=ORIENTED_EDGE('',*,*,#52613,.T.) ;
#73802=ORIENTED_EDGE('',*,*,#51976,.F.) ;
#73803=ORIENTED_EDGE('',*,*,#52615,.F.) ;
#73804=ORIENTED_EDGE('',*,*,#51956,.F.) ;
#73805=ORIENTED_EDGE('',*,*,#52614,.T.) ;
#73806=ORIENTED_EDGE('',*,*,#51971,.F.) ;
#73807=ORIENTED_EDGE('',*,*,#52616,.F.) ;
#73808=ORIENTED_EDGE('',*,*,#51953,.F.) ;
#73809=ORIENTED_EDGE('',*,*,#52615,.T.) ;
#73810=ORIENTED_EDGE('',*,*,#52617,.F.) ;
#73811=ORIENTED_EDGE('',*,*,#52616,.T.) ;
#73812=ORIENTED_EDGE('',*,*,#51972,.F.) ;
#73813=ORIENTED_EDGE('',*,*,#52617,.T.) ;
#73814=ORIENTED_EDGE('',*,*,#51975,.F.) ;
#73815=ORIENTED_EDGE('',*,*,#49088,.F.) ;
#73816=ORIENTED_EDGE('',*,*,#51895,.F.) ;
#73817=ORIENTED_EDGE('',*,*,#49102,.F.) ;
#73818=ORIENTED_EDGE('',*,*,#51896,.F.) ;
#73819=ORIENTED_EDGE('',*,*,#49090,.F.) ;
#73820=ORIENTED_EDGE('',*,*,#51897,.F.) ;
#73821=ORIENTED_EDGE('',*,*,#49100,.F.) ;
#73822=ORIENTED_EDGE('',*,*,#51900,.F.) ;
#73823=ORIENTED_EDGE('',*,*,#49098,.F.) ;
#73824=ORIENTED_EDGE('',*,*,#51898,.F.) ;
#73825=ORIENTED_EDGE('',*,*,#49092,.F.) ;
#73826=ORIENTED_EDGE('',*,*,#51901,.F.) ;
#73827=ORIENTED_EDGE('',*,*,#49096,.F.) ;
#73828=ORIENTED_EDGE('',*,*,#49531,.F.) ;
#73829=ORIENTED_EDGE('',*,*,#49094,.F.) ;
#73830=ORIENTED_EDGE('',*,*,#51899,.F.) ;
#73831=ORIENTED_EDGE('',*,*,#52618,.F.) ;
#73832=ORIENTED_EDGE('',*,*,#52619,.F.) ;
#73833=ORIENTED_EDGE('',*,*,#52620,.F.) ;
#73834=ORIENTED_EDGE('',*,*,#52619,.T.) ;
#73835=ORIENTED_EDGE('',*,*,#51359,.F.) ;
#73836=ORIENTED_EDGE('',*,*,#52621,.F.) ;
#73837=ORIENTED_EDGE('',*,*,#51354,.F.) ;
#73838=ORIENTED_EDGE('',*,*,#52620,.T.) ;
#73839=ORIENTED_EDGE('',*,*,#51353,.F.) ;
#73840=ORIENTED_EDGE('',*,*,#52622,.F.) ;
#73841=ORIENTED_EDGE('',*,*,#51355,.F.) ;
#73842=ORIENTED_EDGE('',*,*,#52618,.T.) ;
#73843=ORIENTED_EDGE('',*,*,#51358,.F.) ;
#73844=ORIENTED_EDGE('',*,*,#52623,.F.) ;
#73845=ORIENTED_EDGE('',*,*,#51360,.F.) ;
#73846=ORIENTED_EDGE('',*,*,#51364,.F.) ;
#73847=ORIENTED_EDGE('',*,*,#52624,.T.) ;
#73848=ORIENTED_EDGE('',*,*,#51113,.F.) ;
#73849=ORIENTED_EDGE('',*,*,#52625,.F.) ;
#73850=ORIENTED_EDGE('',*,*,#52621,.T.) ;
#73851=ORIENTED_EDGE('',*,*,#52625,.T.) ;
#73852=ORIENTED_EDGE('',*,*,#52626,.F.) ;
#73853=ORIENTED_EDGE('',*,*,#52627,.F.) ;
#73854=ORIENTED_EDGE('',*,*,#52622,.T.) ;
#73855=ORIENTED_EDGE('',*,*,#52628,.F.) ;
#73856=ORIENTED_EDGE('',*,*,#49652,.T.) ;
#73857=ORIENTED_EDGE('',*,*,#52629,.F.) ;
#73858=ORIENTED_EDGE('',*,*,#52623,.T.) ;
#73859=ORIENTED_EDGE('',*,*,#52630,.F.) ;
#73860=ORIENTED_EDGE('',*,*,#51363,.F.) ;
#73861=ORIENTED_EDGE('',*,*,#52631,.T.) ;
#73862=ORIENTED_EDGE('',*,*,#49499,.F.) ;
#73863=ORIENTED_EDGE('',*,*,#52632,.T.) ;
#73864=ORIENTED_EDGE('',*,*,#52626,.T.) ;
#73865=ORIENTED_EDGE('',*,*,#51112,.F.) ;
#73866=ORIENTED_EDGE('',*,*,#52633,.F.) ;
#73867=ORIENTED_EDGE('',*,*,#51351,.F.) ;
#73868=ORIENTED_EDGE('',*,*,#52628,.T.) ;
#73869=ORIENTED_EDGE('',*,*,#51352,.F.) ;
#73870=ORIENTED_EDGE('',*,*,#52634,.F.) ;
#73871=ORIENTED_EDGE('',*,*,#49653,.F.) ;
#73872=ORIENTED_EDGE('',*,*,#52627,.T.) ;
#73873=ORIENTED_EDGE('',*,*,#49659,.F.) ;
#73874=ORIENTED_EDGE('',*,*,#52635,.F.) ;
#73875=ORIENTED_EDGE('',*,*,#51356,.F.) ;
#73876=ORIENTED_EDGE('',*,*,#52630,.T.) ;
#73877=ORIENTED_EDGE('',*,*,#51357,.F.) ;
#73878=ORIENTED_EDGE('',*,*,#52636,.F.) ;
#73879=ORIENTED_EDGE('',*,*,#51347,.F.) ;
#73880=ORIENTED_EDGE('',*,*,#52629,.T.) ;
#73881=ORIENTED_EDGE('',*,*,#51350,.F.) ;
#73882=ORIENTED_EDGE('',*,*,#52637,.F.) ;
#73883=ORIENTED_EDGE('',*,*,#51361,.F.) ;
#73884=ORIENTED_EDGE('',*,*,#51123,.F.) ;
#73885=ORIENTED_EDGE('',*,*,#52638,.T.) ;
#73886=ORIENTED_EDGE('',*,*,#51362,.F.) ;
#73887=ORIENTED_EDGE('',*,*,#52639,.F.) ;
#73888=ORIENTED_EDGE('',*,*,#52633,.T.) ;
#73889=ORIENTED_EDGE('',*,*,#51111,.T.) ;
#73890=ORIENTED_EDGE('',*,*,#52640,.F.) ;
#73891=ORIENTED_EDGE('',*,*,#52634,.T.) ;
#73892=ORIENTED_EDGE('',*,*,#52635,.T.) ;
#73893=ORIENTED_EDGE('',*,*,#49658,.T.) ;
#73894=ORIENTED_EDGE('',*,*,#52641,.F.) ;
#73895=ORIENTED_EDGE('',*,*,#52636,.T.) ;
#73896=ORIENTED_EDGE('',*,*,#52639,.T.) ;
#73897=ORIENTED_EDGE('',*,*,#52637,.T.) ;
#73898=ORIENTED_EDGE('',*,*,#52642,.F.) ;
#73899=ORIENTED_EDGE('',*,*,#51107,.F.) ;
#73900=ORIENTED_EDGE('',*,*,#52643,.T.) ;
#73901=ORIENTED_EDGE('',*,*,#51101,.F.) ;
#73902=ORIENTED_EDGE('',*,*,#52644,.F.) ;
#73903=ORIENTED_EDGE('',*,*,#52640,.T.) ;
#73904=ORIENTED_EDGE('',*,*,#51110,.F.) ;
#73905=ORIENTED_EDGE('',*,*,#52645,.F.) ;
#73906=ORIENTED_EDGE('',*,*,#49654,.F.) ;
#73907=ORIENTED_EDGE('',*,*,#52641,.T.) ;
#73908=ORIENTED_EDGE('',*,*,#49657,.F.) ;
#73909=ORIENTED_EDGE('',*,*,#52646,.F.) ;
#73910=ORIENTED_EDGE('',*,*,#51348,.F.) ;
#73911=ORIENTED_EDGE('',*,*,#52642,.T.) ;
#73912=ORIENTED_EDGE('',*,*,#51349,.F.) ;
#73913=ORIENTED_EDGE('',*,*,#52647,.F.) ;
#73914=ORIENTED_EDGE('',*,*,#51124,.F.) ;
#73915=ORIENTED_EDGE('',*,*,#52644,.T.) ;
#73916=ORIENTED_EDGE('',*,*,#52232,.F.) ;
#73917=ORIENTED_EDGE('',*,*,#52648,.F.) ;
#73918=ORIENTED_EDGE('',*,*,#52649,.F.) ;
#73919=ORIENTED_EDGE('',*,*,#52645,.T.) ;
#73920=ORIENTED_EDGE('',*,*,#52650,.F.) ;
#73921=ORIENTED_EDGE('',*,*,#52647,.T.) ;
#73922=ORIENTED_EDGE('',*,*,#52646,.T.) ;
#73923=ORIENTED_EDGE('',*,*,#52651,.F.) ;
#73924=ORIENTED_EDGE('',*,*,#51125,.T.) ;
#73925=ORIENTED_EDGE('',*,*,#52648,.T.) ;
#73926=ORIENTED_EDGE('',*,*,#49721,.F.) ;
#73927=ORIENTED_EDGE('',*,*,#52652,.F.) ;
#73928=ORIENTED_EDGE('',*,*,#51108,.F.) ;
#73929=ORIENTED_EDGE('',*,*,#52650,.T.) ;
#73930=ORIENTED_EDGE('',*,*,#51109,.F.) ;
#73931=ORIENTED_EDGE('',*,*,#52653,.F.) ;
#73932=ORIENTED_EDGE('',*,*,#51115,.F.) ;
#73933=ORIENTED_EDGE('',*,*,#52649,.T.) ;
#73934=ORIENTED_EDGE('',*,*,#51118,.F.) ;
#73935=ORIENTED_EDGE('',*,*,#52654,.F.) ;
#73936=ORIENTED_EDGE('',*,*,#49655,.F.) ;
#73937=ORIENTED_EDGE('',*,*,#52651,.T.) ;
#73938=ORIENTED_EDGE('',*,*,#49656,.F.) ;
#73939=ORIENTED_EDGE('',*,*,#52655,.F.) ;
#73940=ORIENTED_EDGE('',*,*,#51126,.F.) ;
#73941=ORIENTED_EDGE('',*,*,#52652,.T.) ;
#73942=ORIENTED_EDGE('',*,*,#49720,.T.) ;
#73943=ORIENTED_EDGE('',*,*,#52656,.F.) ;
#73944=ORIENTED_EDGE('',*,*,#52653,.T.) ;
#73945=ORIENTED_EDGE('',*,*,#52655,.T.) ;
#73946=ORIENTED_EDGE('',*,*,#52654,.T.) ;
#73947=ORIENTED_EDGE('',*,*,#52657,.F.) ;
#73948=ORIENTED_EDGE('',*,*,#52656,.T.) ;
#73949=ORIENTED_EDGE('',*,*,#49719,.F.) ;
#73950=ORIENTED_EDGE('',*,*,#52658,.F.) ;
#73951=ORIENTED_EDGE('',*,*,#51116,.F.) ;
#73952=ORIENTED_EDGE('',*,*,#52657,.T.) ;
#73953=ORIENTED_EDGE('',*,*,#51117,.F.) ;
#73954=ORIENTED_EDGE('',*,*,#52659,.F.) ;
#73955=ORIENTED_EDGE('',*,*,#51127,.F.) ;
#73956=ORIENTED_EDGE('',*,*,#51131,.F.) ;
#73957=ORIENTED_EDGE('',*,*,#52660,.T.) ;
#73958=ORIENTED_EDGE('',*,*,#51119,.F.) ;
#73959=ORIENTED_EDGE('',*,*,#52661,.F.) ;
#73960=ORIENTED_EDGE('',*,*,#49716,.F.) ;
#73961=ORIENTED_EDGE('',*,*,#52662,.T.) ;
#73962=ORIENTED_EDGE('',*,*,#51132,.F.) ;
#73963=ORIENTED_EDGE('',*,*,#52663,.F.) ;
#73964=ORIENTED_EDGE('',*,*,#52658,.T.) ;
#73965=ORIENTED_EDGE('',*,*,#49718,.T.) ;
#73966=ORIENTED_EDGE('',*,*,#52664,.F.) ;
#73967=ORIENTED_EDGE('',*,*,#52659,.T.) ;
#73968=ORIENTED_EDGE('',*,*,#52663,.T.) ;
#73969=ORIENTED_EDGE('',*,*,#52661,.T.) ;
#73970=ORIENTED_EDGE('',*,*,#52665,.F.) ;
#73971=ORIENTED_EDGE('',*,*,#52664,.T.) ;
#73972=ORIENTED_EDGE('',*,*,#49717,.F.) ;
#73973=ORIENTED_EDGE('',*,*,#52665,.T.) ;
#73974=ORIENTED_EDGE('',*,*,#51128,.F.) ;
#73975=ORIENTED_EDGE('',*,*,#52374,.F.) ;
#73976=ORIENTED_EDGE('',*,*,#52385,.F.) ;
#73977=ORIENTED_EDGE('',*,*,#52384,.F.) ;
#73978=ORIENTED_EDGE('',*,*,#52666,.F.) ;
#73979=ORIENTED_EDGE('',*,*,#52375,.F.) ;
#73980=ORIENTED_EDGE('',*,*,#52666,.T.) ;
#73981=ORIENTED_EDGE('',*,*,#50808,.F.) ;
#73982=ORIENTED_EDGE('',*,*,#52667,.F.) ;
#73983=ORIENTED_EDGE('',*,*,#50794,.F.) ;
#73984=ORIENTED_EDGE('',*,*,#52382,.F.) ;
#73985=ORIENTED_EDGE('',*,*,#52381,.F.) ;
#73986=ORIENTED_EDGE('',*,*,#52380,.F.) ;
#73987=ORIENTED_EDGE('',*,*,#52668,.F.) ;
#73988=ORIENTED_EDGE('',*,*,#52383,.F.) ;
#73989=ORIENTED_EDGE('',*,*,#52669,.F.) ;
#73990=ORIENTED_EDGE('',*,*,#52667,.T.) ;
#73991=ORIENTED_EDGE('',*,*,#52670,.F.) ;
#73992=ORIENTED_EDGE('',*,*,#52372,.F.) ;
#73993=ORIENTED_EDGE('',*,*,#52377,.F.) ;
#73994=ORIENTED_EDGE('',*,*,#52376,.F.) ;
#73995=ORIENTED_EDGE('',*,*,#52671,.F.) ;
#73996=ORIENTED_EDGE('',*,*,#52373,.F.) ;
#73997=ORIENTED_EDGE('',*,*,#52668,.T.) ;
#73998=ORIENTED_EDGE('',*,*,#50804,.F.) ;
#73999=ORIENTED_EDGE('',*,*,#52672,.F.) ;
#74000=ORIENTED_EDGE('',*,*,#50806,.F.) ;
#74001=ORIENTED_EDGE('',*,*,#52670,.T.) ;
#74002=ORIENTED_EDGE('',*,*,#50807,.F.) ;
#74003=ORIENTED_EDGE('',*,*,#52673,.F.) ;
#74004=ORIENTED_EDGE('',*,*,#50852,.F.) ;
#74005=ORIENTED_EDGE('',*,*,#52669,.T.) ;
#74006=ORIENTED_EDGE('',*,*,#50851,.F.) ;
#74007=ORIENTED_EDGE('',*,*,#52674,.F.) ;
#74008=ORIENTED_EDGE('',*,*,#50795,.F.) ;
#74009=ORIENTED_EDGE('',*,*,#52671,.T.) ;
#74010=ORIENTED_EDGE('',*,*,#50796,.F.) ;
#74011=ORIENTED_EDGE('',*,*,#52675,.F.) ;
#74012=ORIENTED_EDGE('',*,*,#50800,.F.) ;
#74013=ORIENTED_EDGE('',*,*,#52673,.T.) ;
#74014=ORIENTED_EDGE('',*,*,#52672,.T.) ;
#74015=ORIENTED_EDGE('',*,*,#52676,.F.) ;
#74016=ORIENTED_EDGE('',*,*,#52675,.T.) ;
#74017=ORIENTED_EDGE('',*,*,#52674,.T.) ;
#74018=ORIENTED_EDGE('',*,*,#52677,.F.) ;
#74019=ORIENTED_EDGE('',*,*,#52676,.T.) ;
#74020=ORIENTED_EDGE('',*,*,#50803,.F.) ;
#74021=ORIENTED_EDGE('',*,*,#52678,.F.) ;
#74022=ORIENTED_EDGE('',*,*,#50849,.F.) ;
#74023=ORIENTED_EDGE('',*,*,#52677,.T.) ;
#74024=ORIENTED_EDGE('',*,*,#50850,.F.) ;
#74025=ORIENTED_EDGE('',*,*,#52679,.F.) ;
#74026=ORIENTED_EDGE('',*,*,#50797,.F.) ;
#74027=ORIENTED_EDGE('',*,*,#52679,.T.) ;
#74028=ORIENTED_EDGE('',*,*,#52678,.T.) ;
#74029=ORIENTED_EDGE('',*,*,#52680,.F.) ;
#74030=ORIENTED_EDGE('',*,*,#52680,.T.) ;
#74031=ORIENTED_EDGE('',*,*,#50802,.F.) ;
#74032=ORIENTED_EDGE('',*,*,#52681,.F.) ;
#74033=ORIENTED_EDGE('',*,*,#50798,.F.) ;
#74034=ORIENTED_EDGE('',*,*,#52378,.F.) ;
#74035=ORIENTED_EDGE('',*,*,#52371,.F.) ;
#74036=ORIENTED_EDGE('',*,*,#52370,.F.) ;
#74037=ORIENTED_EDGE('',*,*,#52681,.T.) ;
#74038=ORIENTED_EDGE('',*,*,#52379,.F.) ;
#74039=ORIENTED_EDGE('',*,*,#52451,.F.) ;
#74040=ORIENTED_EDGE('',*,*,#52450,.F.) ;
#74041=ORIENTED_EDGE('',*,*,#52449,.F.) ;
#74042=ORIENTED_EDGE('',*,*,#52682,.F.) ;
#74043=ORIENTED_EDGE('',*,*,#52452,.F.) ;
#74044=ORIENTED_EDGE('',*,*,#52682,.T.) ;
#74045=ORIENTED_EDGE('',*,*,#52448,.F.) ;
#74046=ORIENTED_EDGE('',*,*,#52683,.F.) ;
#74047=ORIENTED_EDGE('',*,*,#50565,.F.) ;
#74048=ORIENTED_EDGE('',*,*,#52683,.T.) ;
#74049=ORIENTED_EDGE('',*,*,#50536,.F.) ;
#74050=ORIENTED_EDGE('',*,*,#52684,.F.) ;
#74051=ORIENTED_EDGE('',*,*,#50566,.F.) ;
#74052=ORIENTED_EDGE('',*,*,#50524,.F.) ;
#74053=ORIENTED_EDGE('',*,*,#50567,.F.) ;
#74054=ORIENTED_EDGE('',*,*,#52685,.F.) ;
#74055=ORIENTED_EDGE('',*,*,#50530,.F.) ;
#74056=ORIENTED_EDGE('',*,*,#52685,.T.) ;
#74057=ORIENTED_EDGE('',*,*,#52684,.T.) ;
#74058=ORIENTED_EDGE('',*,*,#52686,.F.) ;
#74059=ORIENTED_EDGE('',*,*,#52686,.T.) ;
#74060=ORIENTED_EDGE('',*,*,#50535,.F.) ;
#74061=ORIENTED_EDGE('',*,*,#52687,.F.) ;
#74062=ORIENTED_EDGE('',*,*,#50531,.F.) ;
#74063=ORIENTED_EDGE('',*,*,#50526,.F.) ;
#74064=ORIENTED_EDGE('',*,*,#50532,.F.) ;
#74065=ORIENTED_EDGE('',*,*,#52688,.F.) ;
#74066=ORIENTED_EDGE('',*,*,#50629,.F.) ;
#74067=ORIENTED_EDGE('',*,*,#52688,.T.) ;
#74068=ORIENTED_EDGE('',*,*,#52687,.T.) ;
#74069=ORIENTED_EDGE('',*,*,#52689,.F.) ;
#74070=ORIENTED_EDGE('',*,*,#52689,.T.) ;
#74071=ORIENTED_EDGE('',*,*,#50534,.F.) ;
#74072=ORIENTED_EDGE('',*,*,#52690,.F.) ;
#74073=ORIENTED_EDGE('',*,*,#50630,.F.) ;
#74074=ORIENTED_EDGE('',*,*,#52690,.T.) ;
#74075=ORIENTED_EDGE('',*,*,#52447,.F.) ;
#74076=ORIENTED_EDGE('',*,*,#52691,.F.) ;
#74077=ORIENTED_EDGE('',*,*,#50631,.F.) ;
#74078=ORIENTED_EDGE('',*,*,#52691,.T.) ;
#74079=ORIENTED_EDGE('',*,*,#52446,.F.) ;
#74080=ORIENTED_EDGE('',*,*,#52455,.F.) ;
#74081=ORIENTED_EDGE('',*,*,#52456,.F.) ;
#74082=ORIENTED_EDGE('',*,*,#52461,.F.) ;
#74083=ORIENTED_EDGE('',*,*,#52692,.F.) ;
#74084=ORIENTED_EDGE('',*,*,#52692,.T.) ;
#74085=ORIENTED_EDGE('',*,*,#52460,.F.) ;
#74086=ORIENTED_EDGE('',*,*,#52693,.F.) ;
#74087=ORIENTED_EDGE('',*,*,#50626,.F.) ;
#74088=ORIENTED_EDGE('',*,*,#52693,.T.) ;
#74089=ORIENTED_EDGE('',*,*,#50518,.F.) ;
#74090=ORIENTED_EDGE('',*,*,#52694,.F.) ;
#74091=ORIENTED_EDGE('',*,*,#50627,.F.) ;
#74092=ORIENTED_EDGE('',*,*,#50528,.F.) ;
#74093=ORIENTED_EDGE('',*,*,#50628,.F.) ;
#74094=ORIENTED_EDGE('',*,*,#52695,.F.) ;
#74095=ORIENTED_EDGE('',*,*,#50522,.F.) ;
#74096=ORIENTED_EDGE('',*,*,#52695,.T.) ;
#74097=ORIENTED_EDGE('',*,*,#52694,.T.) ;
#74098=ORIENTED_EDGE('',*,*,#52696,.F.) ;
#74099=ORIENTED_EDGE('',*,*,#52696,.T.) ;
#74100=ORIENTED_EDGE('',*,*,#50517,.F.) ;
#74101=ORIENTED_EDGE('',*,*,#52697,.F.) ;
#74102=ORIENTED_EDGE('',*,*,#50519,.F.) ;
#74103=ORIENTED_EDGE('',*,*,#50529,.F.) ;
#74104=ORIENTED_EDGE('',*,*,#50520,.F.) ;
#74105=ORIENTED_EDGE('',*,*,#52698,.F.) ;
#74106=ORIENTED_EDGE('',*,*,#50568,.F.) ;
#74107=ORIENTED_EDGE('',*,*,#52698,.T.) ;
#74108=ORIENTED_EDGE('',*,*,#52697,.T.) ;
#74109=ORIENTED_EDGE('',*,*,#52699,.F.) ;
#74110=ORIENTED_EDGE('',*,*,#52699,.T.) ;
#74111=ORIENTED_EDGE('',*,*,#50516,.F.) ;
#74112=ORIENTED_EDGE('',*,*,#52700,.F.) ;
#74113=ORIENTED_EDGE('',*,*,#50569,.F.) ;
#74114=ORIENTED_EDGE('',*,*,#52700,.T.) ;
#74115=ORIENTED_EDGE('',*,*,#52459,.F.) ;
#74116=ORIENTED_EDGE('',*,*,#52701,.F.) ;
#74117=ORIENTED_EDGE('',*,*,#50570,.F.) ;
#74118=ORIENTED_EDGE('',*,*,#52457,.F.) ;
#74119=ORIENTED_EDGE('',*,*,#52454,.F.) ;
#74120=ORIENTED_EDGE('',*,*,#52453,.F.) ;
#74121=ORIENTED_EDGE('',*,*,#52701,.T.) ;
#74122=ORIENTED_EDGE('',*,*,#52458,.F.) ;
#74123=ORIENTED_EDGE('',*,*,#52702,.F.) ;
#74124=ORIENTED_EDGE('',*,*,#49508,.F.) ;
#74125=ORIENTED_EDGE('',*,*,#52703,.F.) ;
#74126=ORIENTED_EDGE('',*,*,#51985,.F.) ;
#74127=ORIENTED_EDGE('',*,*,#52703,.T.) ;
#74128=ORIENTED_EDGE('',*,*,#49507,.F.) ;
#74129=ORIENTED_EDGE('',*,*,#52704,.F.) ;
#74130=ORIENTED_EDGE('',*,*,#51988,.F.) ;
#74131=ORIENTED_EDGE('',*,*,#52702,.T.) ;
#74132=ORIENTED_EDGE('',*,*,#51982,.F.) ;
#74133=ORIENTED_EDGE('',*,*,#52705,.F.) ;
#74134=ORIENTED_EDGE('',*,*,#49509,.F.) ;
#74135=ORIENTED_EDGE('',*,*,#52704,.T.) ;
#74136=ORIENTED_EDGE('',*,*,#49506,.F.) ;
#74137=ORIENTED_EDGE('',*,*,#52706,.F.) ;
#74138=ORIENTED_EDGE('',*,*,#51991,.F.) ;
#74139=ORIENTED_EDGE('',*,*,#52705,.T.) ;
#74140=ORIENTED_EDGE('',*,*,#51979,.F.) ;
#74141=ORIENTED_EDGE('',*,*,#52707,.F.) ;
#74142=ORIENTED_EDGE('',*,*,#49510,.F.) ;
#74143=ORIENTED_EDGE('',*,*,#52706,.T.) ;
#74144=ORIENTED_EDGE('',*,*,#49505,.F.) ;
#74145=ORIENTED_EDGE('',*,*,#52708,.F.) ;
#74146=ORIENTED_EDGE('',*,*,#51994,.F.) ;
#74147=ORIENTED_EDGE('',*,*,#52707,.T.) ;
#74148=ORIENTED_EDGE('',*,*,#52001,.F.) ;
#74149=ORIENTED_EDGE('',*,*,#52709,.F.) ;
#74150=ORIENTED_EDGE('',*,*,#49503,.F.) ;
#74151=ORIENTED_EDGE('',*,*,#52708,.T.) ;
#74152=ORIENTED_EDGE('',*,*,#49504,.F.) ;
#74153=ORIENTED_EDGE('',*,*,#52709,.T.) ;
#74154=ORIENTED_EDGE('',*,*,#51997,.F.) ;
#74155=ORIENTED_EDGE('',*,*,#50858,.F.) ;
#74156=ORIENTED_EDGE('',*,*,#50872,.F.) ;
#74157=ORIENTED_EDGE('',*,*,#52710,.F.) ;
#74158=ORIENTED_EDGE('',*,*,#50861,.F.) ;
#74159=ORIENTED_EDGE('',*,*,#52711,.F.) ;
#74160=ORIENTED_EDGE('',*,*,#50862,.F.) ;
#74161=ORIENTED_EDGE('',*,*,#52712,.F.) ;
#74162=ORIENTED_EDGE('',*,*,#51048,.F.) ;
#74163=ORIENTED_EDGE('',*,*,#50860,.F.) ;
#74164=ORIENTED_EDGE('',*,*,#50863,.F.) ;
#74165=ORIENTED_EDGE('',*,*,#52713,.F.) ;
#74166=ORIENTED_EDGE('',*,*,#50864,.F.) ;
#74167=ORIENTED_EDGE('',*,*,#52712,.T.) ;
#74168=ORIENTED_EDGE('',*,*,#52710,.T.) ;
#74169=ORIENTED_EDGE('',*,*,#52714,.F.) ;
#74170=ORIENTED_EDGE('',*,*,#52713,.T.) ;
#74171=ORIENTED_EDGE('',*,*,#52711,.T.) ;
#74172=ORIENTED_EDGE('',*,*,#52715,.F.) ;
#74173=ORIENTED_EDGE('',*,*,#50856,.F.) ;
#74174=ORIENTED_EDGE('',*,*,#50868,.F.) ;
#74175=ORIENTED_EDGE('',*,*,#52716,.F.) ;
#74176=ORIENTED_EDGE('',*,*,#50870,.F.) ;
#74177=ORIENTED_EDGE('',*,*,#52714,.T.) ;
#74178=ORIENTED_EDGE('',*,*,#50871,.F.) ;
#74179=ORIENTED_EDGE('',*,*,#52717,.F.) ;
#74180=ORIENTED_EDGE('',*,*,#51045,.F.) ;
#74181=ORIENTED_EDGE('',*,*,#52715,.T.) ;
#74182=ORIENTED_EDGE('',*,*,#51047,.F.) ;
#74183=ORIENTED_EDGE('',*,*,#52718,.F.) ;
#74184=ORIENTED_EDGE('',*,*,#50865,.F.) ;
#74185=ORIENTED_EDGE('',*,*,#50854,.F.) ;
#74186=ORIENTED_EDGE('',*,*,#50866,.F.) ;
#74187=ORIENTED_EDGE('',*,*,#52719,.F.) ;
#74188=ORIENTED_EDGE('',*,*,#50869,.F.) ;
#74189=ORIENTED_EDGE('',*,*,#52717,.T.) ;
#74190=ORIENTED_EDGE('',*,*,#52716,.T.) ;
#74191=ORIENTED_EDGE('',*,*,#52720,.F.) ;
#74192=ORIENTED_EDGE('',*,*,#52719,.T.) ;
#74193=ORIENTED_EDGE('',*,*,#52718,.T.) ;
#74194=ORIENTED_EDGE('',*,*,#52721,.F.) ;
#74195=ORIENTED_EDGE('',*,*,#52720,.T.) ;
#74196=ORIENTED_EDGE('',*,*,#50867,.F.) ;
#74197=ORIENTED_EDGE('',*,*,#52721,.T.) ;
#74198=ORIENTED_EDGE('',*,*,#51046,.F.) ;
#74199=ORIENTED_EDGE('',*,*,#52722,.F.) ;
#74200=ORIENTED_EDGE('',*,*,#49364,.F.) ;
#74201=ORIENTED_EDGE('',*,*,#52723,.F.) ;
#74202=ORIENTED_EDGE('',*,*,#51617,.F.) ;
#74203=ORIENTED_EDGE('',*,*,#52723,.T.) ;
#74204=ORIENTED_EDGE('',*,*,#49363,.T.) ;
#74205=ORIENTED_EDGE('',*,*,#52724,.F.) ;
#74206=ORIENTED_EDGE('',*,*,#52725,.F.) ;
#74207=ORIENTED_EDGE('',*,*,#49365,.T.) ;
#74208=ORIENTED_EDGE('',*,*,#52722,.T.) ;
#74209=ORIENTED_EDGE('',*,*,#52726,.F.) ;
#74210=ORIENTED_EDGE('',*,*,#52727,.F.) ;
#74211=ORIENTED_EDGE('',*,*,#52724,.T.) ;
#74212=ORIENTED_EDGE('',*,*,#49362,.F.) ;
#74213=ORIENTED_EDGE('',*,*,#52728,.F.) ;
#74214=ORIENTED_EDGE('',*,*,#51614,.F.) ;
#74215=ORIENTED_EDGE('',*,*,#52725,.T.) ;
#74216=ORIENTED_EDGE('',*,*,#51613,.F.) ;
#74217=ORIENTED_EDGE('',*,*,#52729,.F.) ;
#74218=ORIENTED_EDGE('',*,*,#51618,.F.) ;
#74219=ORIENTED_EDGE('',*,*,#52730,.F.) ;
#74220=ORIENTED_EDGE('',*,*,#51615,.F.) ;
#74221=ORIENTED_EDGE('',*,*,#52731,.F.) ;
#74222=ORIENTED_EDGE('',*,*,#51662,.F.) ;
#74223=ORIENTED_EDGE('',*,*,#52726,.T.) ;
#74224=ORIENTED_EDGE('',*,*,#51616,.F.) ;
#74225=ORIENTED_EDGE('',*,*,#52732,.F.) ;
#74226=ORIENTED_EDGE('',*,*,#51606,.F.) ;
#74227=ORIENTED_EDGE('',*,*,#52727,.T.) ;
#74228=ORIENTED_EDGE('',*,*,#51605,.F.) ;
#74229=ORIENTED_EDGE('',*,*,#52733,.F.) ;
#74230=ORIENTED_EDGE('',*,*,#49366,.F.) ;
#74231=ORIENTED_EDGE('',*,*,#52734,.F.) ;
#74232=ORIENTED_EDGE('',*,*,#49360,.F.) ;
#74233=ORIENTED_EDGE('',*,*,#52735,.F.) ;
#74234=ORIENTED_EDGE('',*,*,#51607,.F.) ;
#74235=ORIENTED_EDGE('',*,*,#49361,.T.) ;
#74236=ORIENTED_EDGE('',*,*,#52734,.T.) ;
#74237=ORIENTED_EDGE('',*,*,#52736,.F.) ;
#74238=ORIENTED_EDGE('',*,*,#52728,.T.) ;
#74239=ORIENTED_EDGE('',*,*,#52731,.T.) ;
#74240=ORIENTED_EDGE('',*,*,#52729,.T.) ;
#74241=ORIENTED_EDGE('',*,*,#52737,.F.) ;
#74242=ORIENTED_EDGE('',*,*,#52732,.T.) ;
#74243=ORIENTED_EDGE('',*,*,#52730,.T.) ;
#74244=ORIENTED_EDGE('',*,*,#52738,.F.) ;
#74245=ORIENTED_EDGE('',*,*,#49359,.T.) ;
#74246=ORIENTED_EDGE('',*,*,#52733,.T.) ;
#74247=ORIENTED_EDGE('',*,*,#52739,.F.) ;
#74248=ORIENTED_EDGE('',*,*,#52735,.T.) ;
#74249=ORIENTED_EDGE('',*,*,#52736,.T.) ;
#74250=ORIENTED_EDGE('',*,*,#51610,.F.) ;
#74251=ORIENTED_EDGE('',*,*,#52740,.F.) ;
#74252=ORIENTED_EDGE('',*,*,#51611,.F.) ;
#74253=ORIENTED_EDGE('',*,*,#52737,.T.) ;
#74254=ORIENTED_EDGE('',*,*,#51612,.F.) ;
#74255=ORIENTED_EDGE('',*,*,#52741,.F.) ;
#74256=ORIENTED_EDGE('',*,*,#51659,.F.) ;
#74257=ORIENTED_EDGE('',*,*,#52738,.T.) ;
#74258=ORIENTED_EDGE('',*,*,#51661,.F.) ;
#74259=ORIENTED_EDGE('',*,*,#52742,.F.) ;
#74260=ORIENTED_EDGE('',*,*,#51603,.F.) ;
#74261=ORIENTED_EDGE('',*,*,#52739,.T.) ;
#74262=ORIENTED_EDGE('',*,*,#51604,.F.) ;
#74263=ORIENTED_EDGE('',*,*,#52743,.F.) ;
#74264=ORIENTED_EDGE('',*,*,#51608,.F.) ;
#74265=ORIENTED_EDGE('',*,*,#52741,.T.) ;
#74266=ORIENTED_EDGE('',*,*,#52740,.T.) ;
#74267=ORIENTED_EDGE('',*,*,#52744,.F.) ;
#74268=ORIENTED_EDGE('',*,*,#52743,.T.) ;
#74269=ORIENTED_EDGE('',*,*,#52742,.T.) ;
#74270=ORIENTED_EDGE('',*,*,#52745,.F.) ;
#74271=ORIENTED_EDGE('',*,*,#52744,.T.) ;
#74272=ORIENTED_EDGE('',*,*,#51609,.F.) ;
#74273=ORIENTED_EDGE('',*,*,#52745,.T.) ;
#74274=ORIENTED_EDGE('',*,*,#51660,.F.) ;
#74275=ORIENTED_EDGE('',*,*,#51668,.F.) ;
#74276=ORIENTED_EDGE('',*,*,#51681,.F.) ;
#74277=ORIENTED_EDGE('',*,*,#52746,.F.) ;
#74278=ORIENTED_EDGE('',*,*,#51673,.F.) ;
#74279=ORIENTED_EDGE('',*,*,#52747,.F.) ;
#74280=ORIENTED_EDGE('',*,*,#51671,.F.) ;
#74281=ORIENTED_EDGE('',*,*,#52748,.F.) ;
#74282=ORIENTED_EDGE('',*,*,#51858,.F.) ;
#74283=ORIENTED_EDGE('',*,*,#51670,.F.) ;
#74284=ORIENTED_EDGE('',*,*,#51672,.F.) ;
#74285=ORIENTED_EDGE('',*,*,#52749,.F.) ;
#74286=ORIENTED_EDGE('',*,*,#51676,.F.) ;
#74287=ORIENTED_EDGE('',*,*,#52748,.T.) ;
#74288=ORIENTED_EDGE('',*,*,#52746,.T.) ;
#74289=ORIENTED_EDGE('',*,*,#52750,.F.) ;
#74290=ORIENTED_EDGE('',*,*,#52749,.T.) ;
#74291=ORIENTED_EDGE('',*,*,#52747,.T.) ;
#74292=ORIENTED_EDGE('',*,*,#52751,.F.) ;
#74293=ORIENTED_EDGE('',*,*,#51666,.F.) ;
#74294=ORIENTED_EDGE('',*,*,#51679,.F.) ;
#74295=ORIENTED_EDGE('',*,*,#52752,.F.) ;
#74296=ORIENTED_EDGE('',*,*,#51682,.F.) ;
#74297=ORIENTED_EDGE('',*,*,#52750,.T.) ;
#74298=ORIENTED_EDGE('',*,*,#51680,.F.) ;
#74299=ORIENTED_EDGE('',*,*,#52753,.F.) ;
#74300=ORIENTED_EDGE('',*,*,#51855,.F.) ;
#74301=ORIENTED_EDGE('',*,*,#52751,.T.) ;
#74302=ORIENTED_EDGE('',*,*,#51857,.F.) ;
#74303=ORIENTED_EDGE('',*,*,#52754,.F.) ;
#74304=ORIENTED_EDGE('',*,*,#51674,.F.) ;
#74305=ORIENTED_EDGE('',*,*,#51664,.F.) ;
#74306=ORIENTED_EDGE('',*,*,#51675,.F.) ;
#74307=ORIENTED_EDGE('',*,*,#52755,.F.) ;
#74308=ORIENTED_EDGE('',*,*,#51677,.F.) ;
#74309=ORIENTED_EDGE('',*,*,#52753,.T.) ;
#74310=ORIENTED_EDGE('',*,*,#52752,.T.) ;
#74311=ORIENTED_EDGE('',*,*,#52756,.F.) ;
#74312=ORIENTED_EDGE('',*,*,#52755,.T.) ;
#74313=ORIENTED_EDGE('',*,*,#52754,.T.) ;
#74314=ORIENTED_EDGE('',*,*,#52757,.F.) ;
#74315=ORIENTED_EDGE('',*,*,#52756,.T.) ;
#74316=ORIENTED_EDGE('',*,*,#51678,.F.) ;
#74317=ORIENTED_EDGE('',*,*,#52757,.T.) ;
#74318=ORIENTED_EDGE('',*,*,#51856,.F.) ;
#74319=ORIENTED_EDGE('',*,*,#52758,.F.) ;
#74320=ORIENTED_EDGE('',*,*,#51990,.F.) ;
#74321=ORIENTED_EDGE('',*,*,#52759,.F.) ;
#74322=ORIENTED_EDGE('',*,*,#52005,.F.) ;
#74323=ORIENTED_EDGE('',*,*,#52759,.T.) ;
#74324=ORIENTED_EDGE('',*,*,#51993,.F.) ;
#74325=ORIENTED_EDGE('',*,*,#52760,.F.) ;
#74326=ORIENTED_EDGE('',*,*,#51987,.F.) ;
#74327=ORIENTED_EDGE('',*,*,#52758,.T.) ;
#74328=ORIENTED_EDGE('',*,*,#52761,.F.) ;
#74329=ORIENTED_EDGE('',*,*,#52760,.T.) ;
#74330=ORIENTED_EDGE('',*,*,#51996,.F.) ;
#74331=ORIENTED_EDGE('',*,*,#52762,.F.) ;
#74332=ORIENTED_EDGE('',*,*,#52002,.F.) ;
#74333=ORIENTED_EDGE('',*,*,#52761,.T.) ;
#74334=ORIENTED_EDGE('',*,*,#52004,.F.) ;
#74335=ORIENTED_EDGE('',*,*,#52763,.F.) ;
#74336=ORIENTED_EDGE('',*,*,#51984,.F.) ;
#74337=ORIENTED_EDGE('',*,*,#52762,.T.) ;
#74338=ORIENTED_EDGE('',*,*,#51999,.F.) ;
#74339=ORIENTED_EDGE('',*,*,#52764,.F.) ;
#74340=ORIENTED_EDGE('',*,*,#51981,.F.) ;
#74341=ORIENTED_EDGE('',*,*,#52763,.T.) ;
#74342=ORIENTED_EDGE('',*,*,#52765,.F.) ;
#74343=ORIENTED_EDGE('',*,*,#52764,.T.) ;
#74344=ORIENTED_EDGE('',*,*,#52000,.F.) ;
#74345=ORIENTED_EDGE('',*,*,#52765,.T.) ;
#74346=ORIENTED_EDGE('',*,*,#52003,.F.) ;
#74347=ORIENTED_EDGE('',*,*,#49106,.F.) ;
#74348=ORIENTED_EDGE('',*,*,#51894,.F.) ;
#74349=ORIENTED_EDGE('',*,*,#49120,.F.) ;
#74350=ORIENTED_EDGE('',*,*,#51902,.F.) ;
#74351=ORIENTED_EDGE('',*,*,#49108,.F.) ;
#74352=ORIENTED_EDGE('',*,*,#51903,.F.) ;
#74353=ORIENTED_EDGE('',*,*,#49118,.F.) ;
#74354=ORIENTED_EDGE('',*,*,#51906,.F.) ;
#74355=ORIENTED_EDGE('',*,*,#49116,.F.) ;
#74356=ORIENTED_EDGE('',*,*,#51904,.F.) ;
#74357=ORIENTED_EDGE('',*,*,#49110,.F.) ;
#74358=ORIENTED_EDGE('',*,*,#51907,.F.) ;
#74359=ORIENTED_EDGE('',*,*,#49114,.F.) ;
#74360=ORIENTED_EDGE('',*,*,#49530,.F.) ;
#74361=ORIENTED_EDGE('',*,*,#49112,.F.) ;
#74362=ORIENTED_EDGE('',*,*,#51905,.F.) ;
#74363=ORIENTED_EDGE('',*,*,#52766,.F.) ;
#74364=ORIENTED_EDGE('',*,*,#52767,.F.) ;
#74365=ORIENTED_EDGE('',*,*,#52768,.F.) ;
#74366=ORIENTED_EDGE('',*,*,#52767,.T.) ;
#74367=ORIENTED_EDGE('',*,*,#51377,.F.) ;
#74368=ORIENTED_EDGE('',*,*,#52769,.F.) ;
#74369=ORIENTED_EDGE('',*,*,#51372,.F.) ;
#74370=ORIENTED_EDGE('',*,*,#52768,.T.) ;
#74371=ORIENTED_EDGE('',*,*,#51371,.F.) ;
#74372=ORIENTED_EDGE('',*,*,#52770,.F.) ;
#74373=ORIENTED_EDGE('',*,*,#51373,.F.) ;
#74374=ORIENTED_EDGE('',*,*,#52766,.T.) ;
#74375=ORIENTED_EDGE('',*,*,#51376,.F.) ;
#74376=ORIENTED_EDGE('',*,*,#52771,.F.) ;
#74377=ORIENTED_EDGE('',*,*,#51378,.F.) ;
#74378=ORIENTED_EDGE('',*,*,#51382,.F.) ;
#74379=ORIENTED_EDGE('',*,*,#52772,.T.) ;
#74380=ORIENTED_EDGE('',*,*,#51141,.F.) ;
#74381=ORIENTED_EDGE('',*,*,#52773,.F.) ;
#74382=ORIENTED_EDGE('',*,*,#52769,.T.) ;
#74383=ORIENTED_EDGE('',*,*,#52773,.T.) ;
#74384=ORIENTED_EDGE('',*,*,#52774,.F.) ;
#74385=ORIENTED_EDGE('',*,*,#52775,.F.) ;
#74386=ORIENTED_EDGE('',*,*,#52770,.T.) ;
#74387=ORIENTED_EDGE('',*,*,#52776,.F.) ;
#74388=ORIENTED_EDGE('',*,*,#49644,.T.) ;
#74389=ORIENTED_EDGE('',*,*,#52777,.F.) ;
#74390=ORIENTED_EDGE('',*,*,#52771,.T.) ;
#74391=ORIENTED_EDGE('',*,*,#52778,.F.) ;
#74392=ORIENTED_EDGE('',*,*,#51381,.F.) ;
#74393=ORIENTED_EDGE('',*,*,#52779,.T.) ;
#74394=ORIENTED_EDGE('',*,*,#49487,.F.) ;
#74395=ORIENTED_EDGE('',*,*,#52780,.T.) ;
#74396=ORIENTED_EDGE('',*,*,#52774,.T.) ;
#74397=ORIENTED_EDGE('',*,*,#51140,.F.) ;
#74398=ORIENTED_EDGE('',*,*,#52781,.F.) ;
#74399=ORIENTED_EDGE('',*,*,#51369,.F.) ;
#74400=ORIENTED_EDGE('',*,*,#52776,.T.) ;
#74401=ORIENTED_EDGE('',*,*,#51370,.F.) ;
#74402=ORIENTED_EDGE('',*,*,#52782,.F.) ;
#74403=ORIENTED_EDGE('',*,*,#49645,.F.) ;
#74404=ORIENTED_EDGE('',*,*,#52775,.T.) ;
#74405=ORIENTED_EDGE('',*,*,#49651,.F.) ;
#74406=ORIENTED_EDGE('',*,*,#52783,.F.) ;
#74407=ORIENTED_EDGE('',*,*,#51374,.F.) ;
#74408=ORIENTED_EDGE('',*,*,#52778,.T.) ;
#74409=ORIENTED_EDGE('',*,*,#51375,.F.) ;
#74410=ORIENTED_EDGE('',*,*,#52784,.F.) ;
#74411=ORIENTED_EDGE('',*,*,#51365,.F.) ;
#74412=ORIENTED_EDGE('',*,*,#52777,.T.) ;
#74413=ORIENTED_EDGE('',*,*,#51368,.F.) ;
#74414=ORIENTED_EDGE('',*,*,#52785,.F.) ;
#74415=ORIENTED_EDGE('',*,*,#51379,.F.) ;
#74416=ORIENTED_EDGE('',*,*,#51151,.F.) ;
#74417=ORIENTED_EDGE('',*,*,#52786,.T.) ;
#74418=ORIENTED_EDGE('',*,*,#51380,.F.) ;
#74419=ORIENTED_EDGE('',*,*,#52787,.F.) ;
#74420=ORIENTED_EDGE('',*,*,#52781,.T.) ;
#74421=ORIENTED_EDGE('',*,*,#51139,.T.) ;
#74422=ORIENTED_EDGE('',*,*,#52788,.F.) ;
#74423=ORIENTED_EDGE('',*,*,#52782,.T.) ;
#74424=ORIENTED_EDGE('',*,*,#52783,.T.) ;
#74425=ORIENTED_EDGE('',*,*,#49650,.T.) ;
#74426=ORIENTED_EDGE('',*,*,#52789,.F.) ;
#74427=ORIENTED_EDGE('',*,*,#52784,.T.) ;
#74428=ORIENTED_EDGE('',*,*,#52787,.T.) ;
#74429=ORIENTED_EDGE('',*,*,#52785,.T.) ;
#74430=ORIENTED_EDGE('',*,*,#52790,.F.) ;
#74431=ORIENTED_EDGE('',*,*,#51135,.F.) ;
#74432=ORIENTED_EDGE('',*,*,#52791,.T.) ;
#74433=ORIENTED_EDGE('',*,*,#51129,.F.) ;
#74434=ORIENTED_EDGE('',*,*,#52792,.F.) ;
#74435=ORIENTED_EDGE('',*,*,#52788,.T.) ;
#74436=ORIENTED_EDGE('',*,*,#51138,.F.) ;
#74437=ORIENTED_EDGE('',*,*,#52793,.F.) ;
#74438=ORIENTED_EDGE('',*,*,#49646,.F.) ;
#74439=ORIENTED_EDGE('',*,*,#52789,.T.) ;
#74440=ORIENTED_EDGE('',*,*,#49649,.F.) ;
#74441=ORIENTED_EDGE('',*,*,#52794,.F.) ;
#74442=ORIENTED_EDGE('',*,*,#51366,.F.) ;
#74443=ORIENTED_EDGE('',*,*,#52790,.T.) ;
#74444=ORIENTED_EDGE('',*,*,#51367,.F.) ;
#74445=ORIENTED_EDGE('',*,*,#52795,.F.) ;
#74446=ORIENTED_EDGE('',*,*,#51152,.F.) ;
#74447=ORIENTED_EDGE('',*,*,#52792,.T.) ;
#74448=ORIENTED_EDGE('',*,*,#52662,.F.) ;
#74449=ORIENTED_EDGE('',*,*,#52796,.F.) ;
#74450=ORIENTED_EDGE('',*,*,#52797,.F.) ;
#74451=ORIENTED_EDGE('',*,*,#52793,.T.) ;
#74452=ORIENTED_EDGE('',*,*,#52798,.F.) ;
#74453=ORIENTED_EDGE('',*,*,#52795,.T.) ;
#74454=ORIENTED_EDGE('',*,*,#52794,.T.) ;
#74455=ORIENTED_EDGE('',*,*,#52799,.F.) ;
#74456=ORIENTED_EDGE('',*,*,#51153,.T.) ;
#74457=ORIENTED_EDGE('',*,*,#52796,.T.) ;
#74458=ORIENTED_EDGE('',*,*,#49715,.F.) ;
#74459=ORIENTED_EDGE('',*,*,#52800,.F.) ;
#74460=ORIENTED_EDGE('',*,*,#51136,.F.) ;
#74461=ORIENTED_EDGE('',*,*,#52798,.T.) ;
#74462=ORIENTED_EDGE('',*,*,#51137,.F.) ;
#74463=ORIENTED_EDGE('',*,*,#52801,.F.) ;
#74464=ORIENTED_EDGE('',*,*,#51143,.F.) ;
#74465=ORIENTED_EDGE('',*,*,#52797,.T.) ;
#74466=ORIENTED_EDGE('',*,*,#51146,.F.) ;
#74467=ORIENTED_EDGE('',*,*,#52802,.F.) ;
#74468=ORIENTED_EDGE('',*,*,#49647,.F.) ;
#74469=ORIENTED_EDGE('',*,*,#52799,.T.) ;
#74470=ORIENTED_EDGE('',*,*,#49648,.F.) ;
#74471=ORIENTED_EDGE('',*,*,#52803,.F.) ;
#74472=ORIENTED_EDGE('',*,*,#51154,.F.) ;
#74473=ORIENTED_EDGE('',*,*,#52800,.T.) ;
#74474=ORIENTED_EDGE('',*,*,#49714,.T.) ;
#74475=ORIENTED_EDGE('',*,*,#52804,.F.) ;
#74476=ORIENTED_EDGE('',*,*,#52801,.T.) ;
#74477=ORIENTED_EDGE('',*,*,#52803,.T.) ;
#74478=ORIENTED_EDGE('',*,*,#52802,.T.) ;
#74479=ORIENTED_EDGE('',*,*,#52805,.F.) ;
#74480=ORIENTED_EDGE('',*,*,#52804,.T.) ;
#74481=ORIENTED_EDGE('',*,*,#49713,.F.) ;
#74482=ORIENTED_EDGE('',*,*,#52806,.F.) ;
#74483=ORIENTED_EDGE('',*,*,#51144,.F.) ;
#74484=ORIENTED_EDGE('',*,*,#52805,.T.) ;
#74485=ORIENTED_EDGE('',*,*,#51145,.F.) ;
#74486=ORIENTED_EDGE('',*,*,#52807,.F.) ;
#74487=ORIENTED_EDGE('',*,*,#51155,.F.) ;
#74488=ORIENTED_EDGE('',*,*,#51159,.F.) ;
#74489=ORIENTED_EDGE('',*,*,#52808,.T.) ;
#74490=ORIENTED_EDGE('',*,*,#51147,.F.) ;
#74491=ORIENTED_EDGE('',*,*,#52809,.F.) ;
#74492=ORIENTED_EDGE('',*,*,#49710,.F.) ;
#74493=ORIENTED_EDGE('',*,*,#52810,.T.) ;
#74494=ORIENTED_EDGE('',*,*,#51160,.F.) ;
#74495=ORIENTED_EDGE('',*,*,#52811,.F.) ;
#74496=ORIENTED_EDGE('',*,*,#52806,.T.) ;
#74497=ORIENTED_EDGE('',*,*,#49712,.T.) ;
#74498=ORIENTED_EDGE('',*,*,#52812,.F.) ;
#74499=ORIENTED_EDGE('',*,*,#52807,.T.) ;
#74500=ORIENTED_EDGE('',*,*,#52811,.T.) ;
#74501=ORIENTED_EDGE('',*,*,#52809,.T.) ;
#74502=ORIENTED_EDGE('',*,*,#52813,.F.) ;
#74503=ORIENTED_EDGE('',*,*,#52812,.T.) ;
#74504=ORIENTED_EDGE('',*,*,#49711,.F.) ;
#74505=ORIENTED_EDGE('',*,*,#52813,.T.) ;
#74506=ORIENTED_EDGE('',*,*,#51156,.F.) ;
#74507=ORIENTED_EDGE('',*,*,#52358,.F.) ;
#74508=ORIENTED_EDGE('',*,*,#52369,.F.) ;
#74509=ORIENTED_EDGE('',*,*,#52368,.F.) ;
#74510=ORIENTED_EDGE('',*,*,#52814,.F.) ;
#74511=ORIENTED_EDGE('',*,*,#52359,.F.) ;
#74512=ORIENTED_EDGE('',*,*,#52814,.T.) ;
#74513=ORIENTED_EDGE('',*,*,#50792,.F.) ;
#74514=ORIENTED_EDGE('',*,*,#52815,.F.) ;
#74515=ORIENTED_EDGE('',*,*,#50778,.F.) ;
#74516=ORIENTED_EDGE('',*,*,#52366,.F.) ;
#74517=ORIENTED_EDGE('',*,*,#52365,.F.) ;
#74518=ORIENTED_EDGE('',*,*,#52364,.F.) ;
#74519=ORIENTED_EDGE('',*,*,#52816,.F.) ;
#74520=ORIENTED_EDGE('',*,*,#52367,.F.) ;
#74521=ORIENTED_EDGE('',*,*,#52817,.F.) ;
#74522=ORIENTED_EDGE('',*,*,#52815,.T.) ;
#74523=ORIENTED_EDGE('',*,*,#52818,.F.) ;
#74524=ORIENTED_EDGE('',*,*,#52356,.F.) ;
#74525=ORIENTED_EDGE('',*,*,#52361,.F.) ;
#74526=ORIENTED_EDGE('',*,*,#52360,.F.) ;
#74527=ORIENTED_EDGE('',*,*,#52819,.F.) ;
#74528=ORIENTED_EDGE('',*,*,#52357,.F.) ;
#74529=ORIENTED_EDGE('',*,*,#52816,.T.) ;
#74530=ORIENTED_EDGE('',*,*,#50788,.F.) ;
#74531=ORIENTED_EDGE('',*,*,#52820,.F.) ;
#74532=ORIENTED_EDGE('',*,*,#50790,.F.) ;
#74533=ORIENTED_EDGE('',*,*,#52818,.T.) ;
#74534=ORIENTED_EDGE('',*,*,#50791,.F.) ;
#74535=ORIENTED_EDGE('',*,*,#52821,.F.) ;
#74536=ORIENTED_EDGE('',*,*,#50876,.F.) ;
#74537=ORIENTED_EDGE('',*,*,#52817,.T.) ;
#74538=ORIENTED_EDGE('',*,*,#50875,.F.) ;
#74539=ORIENTED_EDGE('',*,*,#52822,.F.) ;
#74540=ORIENTED_EDGE('',*,*,#50779,.F.) ;
#74541=ORIENTED_EDGE('',*,*,#52819,.T.) ;
#74542=ORIENTED_EDGE('',*,*,#50780,.F.) ;
#74543=ORIENTED_EDGE('',*,*,#52823,.F.) ;
#74544=ORIENTED_EDGE('',*,*,#50784,.F.) ;
#74545=ORIENTED_EDGE('',*,*,#52821,.T.) ;
#74546=ORIENTED_EDGE('',*,*,#52820,.T.) ;
#74547=ORIENTED_EDGE('',*,*,#52824,.F.) ;
#74548=ORIENTED_EDGE('',*,*,#52823,.T.) ;
#74549=ORIENTED_EDGE('',*,*,#52822,.T.) ;
#74550=ORIENTED_EDGE('',*,*,#52825,.F.) ;
#74551=ORIENTED_EDGE('',*,*,#52824,.T.) ;
#74552=ORIENTED_EDGE('',*,*,#50787,.F.) ;
#74553=ORIENTED_EDGE('',*,*,#52826,.F.) ;
#74554=ORIENTED_EDGE('',*,*,#50873,.F.) ;
#74555=ORIENTED_EDGE('',*,*,#52825,.T.) ;
#74556=ORIENTED_EDGE('',*,*,#50874,.F.) ;
#74557=ORIENTED_EDGE('',*,*,#52827,.F.) ;
#74558=ORIENTED_EDGE('',*,*,#50781,.F.) ;
#74559=ORIENTED_EDGE('',*,*,#52827,.T.) ;
#74560=ORIENTED_EDGE('',*,*,#52826,.T.) ;
#74561=ORIENTED_EDGE('',*,*,#52828,.F.) ;
#74562=ORIENTED_EDGE('',*,*,#52828,.T.) ;
#74563=ORIENTED_EDGE('',*,*,#50786,.F.) ;
#74564=ORIENTED_EDGE('',*,*,#52829,.F.) ;
#74565=ORIENTED_EDGE('',*,*,#50782,.F.) ;
#74566=ORIENTED_EDGE('',*,*,#52362,.F.) ;
#74567=ORIENTED_EDGE('',*,*,#52355,.F.) ;
#74568=ORIENTED_EDGE('',*,*,#52354,.F.) ;
#74569=ORIENTED_EDGE('',*,*,#52829,.T.) ;
#74570=ORIENTED_EDGE('',*,*,#52363,.F.) ;
#74571=ORIENTED_EDGE('',*,*,#52467,.F.) ;
#74572=ORIENTED_EDGE('',*,*,#52466,.F.) ;
#74573=ORIENTED_EDGE('',*,*,#52465,.F.) ;
#74574=ORIENTED_EDGE('',*,*,#52830,.F.) ;
#74575=ORIENTED_EDGE('',*,*,#52468,.F.) ;
#74576=ORIENTED_EDGE('',*,*,#52830,.T.) ;
#74577=ORIENTED_EDGE('',*,*,#52464,.F.) ;
#74578=ORIENTED_EDGE('',*,*,#52831,.F.) ;
#74579=ORIENTED_EDGE('',*,*,#50572,.F.) ;
#74580=ORIENTED_EDGE('',*,*,#52831,.T.) ;
#74581=ORIENTED_EDGE('',*,*,#50514,.F.) ;
#74582=ORIENTED_EDGE('',*,*,#52832,.F.) ;
#74583=ORIENTED_EDGE('',*,*,#50573,.F.) ;
#74584=ORIENTED_EDGE('',*,*,#50502,.F.) ;
#74585=ORIENTED_EDGE('',*,*,#50574,.F.) ;
#74586=ORIENTED_EDGE('',*,*,#52833,.F.) ;
#74587=ORIENTED_EDGE('',*,*,#50508,.F.) ;
#74588=ORIENTED_EDGE('',*,*,#52833,.T.) ;
#74589=ORIENTED_EDGE('',*,*,#52832,.T.) ;
#74590=ORIENTED_EDGE('',*,*,#52834,.F.) ;
#74591=ORIENTED_EDGE('',*,*,#52834,.T.) ;
#74592=ORIENTED_EDGE('',*,*,#50513,.F.) ;
#74593=ORIENTED_EDGE('',*,*,#52835,.F.) ;
#74594=ORIENTED_EDGE('',*,*,#50509,.F.) ;
#74595=ORIENTED_EDGE('',*,*,#50504,.F.) ;
#74596=ORIENTED_EDGE('',*,*,#50510,.F.) ;
#74597=ORIENTED_EDGE('',*,*,#52836,.F.) ;
#74598=ORIENTED_EDGE('',*,*,#50636,.F.) ;
#74599=ORIENTED_EDGE('',*,*,#52836,.T.) ;
#74600=ORIENTED_EDGE('',*,*,#52835,.T.) ;
#74601=ORIENTED_EDGE('',*,*,#52837,.F.) ;
#74602=ORIENTED_EDGE('',*,*,#52837,.T.) ;
#74603=ORIENTED_EDGE('',*,*,#50512,.F.) ;
#74604=ORIENTED_EDGE('',*,*,#52838,.F.) ;
#74605=ORIENTED_EDGE('',*,*,#50637,.F.) ;
#74606=ORIENTED_EDGE('',*,*,#52838,.T.) ;
#74607=ORIENTED_EDGE('',*,*,#52463,.F.) ;
#74608=ORIENTED_EDGE('',*,*,#52839,.F.) ;
#74609=ORIENTED_EDGE('',*,*,#50638,.F.) ;
#74610=ORIENTED_EDGE('',*,*,#52839,.T.) ;
#74611=ORIENTED_EDGE('',*,*,#52462,.F.) ;
#74612=ORIENTED_EDGE('',*,*,#52471,.F.) ;
#74613=ORIENTED_EDGE('',*,*,#52472,.F.) ;
#74614=ORIENTED_EDGE('',*,*,#52477,.F.) ;
#74615=ORIENTED_EDGE('',*,*,#52840,.F.) ;
#74616=ORIENTED_EDGE('',*,*,#52840,.T.) ;
#74617=ORIENTED_EDGE('',*,*,#52476,.F.) ;
#74618=ORIENTED_EDGE('',*,*,#52841,.F.) ;
#74619=ORIENTED_EDGE('',*,*,#50633,.F.) ;
#74620=ORIENTED_EDGE('',*,*,#52841,.T.) ;
#74621=ORIENTED_EDGE('',*,*,#50496,.F.) ;
#74622=ORIENTED_EDGE('',*,*,#52842,.F.) ;
#74623=ORIENTED_EDGE('',*,*,#50634,.F.) ;
#74624=ORIENTED_EDGE('',*,*,#50506,.F.) ;
#74625=ORIENTED_EDGE('',*,*,#50635,.F.) ;
#74626=ORIENTED_EDGE('',*,*,#52843,.F.) ;
#74627=ORIENTED_EDGE('',*,*,#50500,.F.) ;
#74628=ORIENTED_EDGE('',*,*,#52843,.T.) ;
#74629=ORIENTED_EDGE('',*,*,#52842,.T.) ;
#74630=ORIENTED_EDGE('',*,*,#52844,.F.) ;
#74631=ORIENTED_EDGE('',*,*,#52844,.T.) ;
#74632=ORIENTED_EDGE('',*,*,#50495,.F.) ;
#74633=ORIENTED_EDGE('',*,*,#52845,.F.) ;
#74634=ORIENTED_EDGE('',*,*,#50497,.F.) ;
#74635=ORIENTED_EDGE('',*,*,#50507,.F.) ;
#74636=ORIENTED_EDGE('',*,*,#50498,.F.) ;
#74637=ORIENTED_EDGE('',*,*,#52846,.F.) ;
#74638=ORIENTED_EDGE('',*,*,#50575,.F.) ;
#74639=ORIENTED_EDGE('',*,*,#52846,.T.) ;
#74640=ORIENTED_EDGE('',*,*,#52845,.T.) ;
#74641=ORIENTED_EDGE('',*,*,#52847,.F.) ;
#74642=ORIENTED_EDGE('',*,*,#52847,.T.) ;
#74643=ORIENTED_EDGE('',*,*,#50494,.F.) ;
#74644=ORIENTED_EDGE('',*,*,#52848,.F.) ;
#74645=ORIENTED_EDGE('',*,*,#50576,.F.) ;
#74646=ORIENTED_EDGE('',*,*,#52848,.T.) ;
#74647=ORIENTED_EDGE('',*,*,#52475,.F.) ;
#74648=ORIENTED_EDGE('',*,*,#52849,.F.) ;
#74649=ORIENTED_EDGE('',*,*,#50577,.F.) ;
#74650=ORIENTED_EDGE('',*,*,#52473,.F.) ;
#74651=ORIENTED_EDGE('',*,*,#52470,.F.) ;
#74652=ORIENTED_EDGE('',*,*,#52469,.F.) ;
#74653=ORIENTED_EDGE('',*,*,#52849,.T.) ;
#74654=ORIENTED_EDGE('',*,*,#52474,.F.) ;
#74655=ORIENTED_EDGE('',*,*,#52850,.F.) ;
#74656=ORIENTED_EDGE('',*,*,#49496,.F.) ;
#74657=ORIENTED_EDGE('',*,*,#52851,.F.) ;
#74658=ORIENTED_EDGE('',*,*,#52013,.F.) ;
#74659=ORIENTED_EDGE('',*,*,#52851,.T.) ;
#74660=ORIENTED_EDGE('',*,*,#49495,.F.) ;
#74661=ORIENTED_EDGE('',*,*,#52852,.F.) ;
#74662=ORIENTED_EDGE('',*,*,#52016,.F.) ;
#74663=ORIENTED_EDGE('',*,*,#52850,.T.) ;
#74664=ORIENTED_EDGE('',*,*,#52010,.F.) ;
#74665=ORIENTED_EDGE('',*,*,#52853,.F.) ;
#74666=ORIENTED_EDGE('',*,*,#49497,.F.) ;
#74667=ORIENTED_EDGE('',*,*,#52852,.T.) ;
#74668=ORIENTED_EDGE('',*,*,#49494,.F.) ;
#74669=ORIENTED_EDGE('',*,*,#52854,.F.) ;
#74670=ORIENTED_EDGE('',*,*,#52019,.F.) ;
#74671=ORIENTED_EDGE('',*,*,#52853,.T.) ;
#74672=ORIENTED_EDGE('',*,*,#52007,.F.) ;
#74673=ORIENTED_EDGE('',*,*,#52855,.F.) ;
#74674=ORIENTED_EDGE('',*,*,#49498,.F.) ;
#74675=ORIENTED_EDGE('',*,*,#52854,.T.) ;
#74676=ORIENTED_EDGE('',*,*,#49493,.F.) ;
#74677=ORIENTED_EDGE('',*,*,#52856,.F.) ;
#74678=ORIENTED_EDGE('',*,*,#52022,.F.) ;
#74679=ORIENTED_EDGE('',*,*,#52855,.T.) ;
#74680=ORIENTED_EDGE('',*,*,#52029,.F.) ;
#74681=ORIENTED_EDGE('',*,*,#52857,.F.) ;
#74682=ORIENTED_EDGE('',*,*,#49491,.F.) ;
#74683=ORIENTED_EDGE('',*,*,#52856,.T.) ;
#74684=ORIENTED_EDGE('',*,*,#49492,.F.) ;
#74685=ORIENTED_EDGE('',*,*,#52857,.T.) ;
#74686=ORIENTED_EDGE('',*,*,#52025,.F.) ;
#74687=ORIENTED_EDGE('',*,*,#50882,.F.) ;
#74688=ORIENTED_EDGE('',*,*,#50896,.F.) ;
#74689=ORIENTED_EDGE('',*,*,#52858,.F.) ;
#74690=ORIENTED_EDGE('',*,*,#50885,.F.) ;
#74691=ORIENTED_EDGE('',*,*,#52859,.F.) ;
#74692=ORIENTED_EDGE('',*,*,#50886,.F.) ;
#74693=ORIENTED_EDGE('',*,*,#52860,.F.) ;
#74694=ORIENTED_EDGE('',*,*,#51052,.F.) ;
#74695=ORIENTED_EDGE('',*,*,#50884,.F.) ;
#74696=ORIENTED_EDGE('',*,*,#50887,.F.) ;
#74697=ORIENTED_EDGE('',*,*,#52861,.F.) ;
#74698=ORIENTED_EDGE('',*,*,#50888,.F.) ;
#74699=ORIENTED_EDGE('',*,*,#52860,.T.) ;
#74700=ORIENTED_EDGE('',*,*,#52858,.T.) ;
#74701=ORIENTED_EDGE('',*,*,#52862,.F.) ;
#74702=ORIENTED_EDGE('',*,*,#52861,.T.) ;
#74703=ORIENTED_EDGE('',*,*,#52859,.T.) ;
#74704=ORIENTED_EDGE('',*,*,#52863,.F.) ;
#74705=ORIENTED_EDGE('',*,*,#50880,.F.) ;
#74706=ORIENTED_EDGE('',*,*,#50892,.F.) ;
#74707=ORIENTED_EDGE('',*,*,#52864,.F.) ;
#74708=ORIENTED_EDGE('',*,*,#50894,.F.) ;
#74709=ORIENTED_EDGE('',*,*,#52862,.T.) ;
#74710=ORIENTED_EDGE('',*,*,#50895,.F.) ;
#74711=ORIENTED_EDGE('',*,*,#52865,.F.) ;
#74712=ORIENTED_EDGE('',*,*,#51049,.F.) ;
#74713=ORIENTED_EDGE('',*,*,#52863,.T.) ;
#74714=ORIENTED_EDGE('',*,*,#51051,.F.) ;
#74715=ORIENTED_EDGE('',*,*,#52866,.F.) ;
#74716=ORIENTED_EDGE('',*,*,#50889,.F.) ;
#74717=ORIENTED_EDGE('',*,*,#50878,.F.) ;
#74718=ORIENTED_EDGE('',*,*,#50890,.F.) ;
#74719=ORIENTED_EDGE('',*,*,#52867,.F.) ;
#74720=ORIENTED_EDGE('',*,*,#50893,.F.) ;
#74721=ORIENTED_EDGE('',*,*,#52865,.T.) ;
#74722=ORIENTED_EDGE('',*,*,#52864,.T.) ;
#74723=ORIENTED_EDGE('',*,*,#52868,.F.) ;
#74724=ORIENTED_EDGE('',*,*,#52867,.T.) ;
#74725=ORIENTED_EDGE('',*,*,#52866,.T.) ;
#74726=ORIENTED_EDGE('',*,*,#52869,.F.) ;
#74727=ORIENTED_EDGE('',*,*,#52868,.T.) ;
#74728=ORIENTED_EDGE('',*,*,#50891,.F.) ;
#74729=ORIENTED_EDGE('',*,*,#52869,.T.) ;
#74730=ORIENTED_EDGE('',*,*,#51050,.F.) ;
#74731=ORIENTED_EDGE('',*,*,#52870,.F.) ;
#74732=ORIENTED_EDGE('',*,*,#49388,.F.) ;
#74733=ORIENTED_EDGE('',*,*,#52871,.F.) ;
#74734=ORIENTED_EDGE('',*,*,#51601,.F.) ;
#74735=ORIENTED_EDGE('',*,*,#52871,.T.) ;
#74736=ORIENTED_EDGE('',*,*,#49387,.T.) ;
#74737=ORIENTED_EDGE('',*,*,#52872,.F.) ;
#74738=ORIENTED_EDGE('',*,*,#52873,.F.) ;
#74739=ORIENTED_EDGE('',*,*,#49389,.T.) ;
#74740=ORIENTED_EDGE('',*,*,#52870,.T.) ;
#74741=ORIENTED_EDGE('',*,*,#52874,.F.) ;
#74742=ORIENTED_EDGE('',*,*,#52875,.F.) ;
#74743=ORIENTED_EDGE('',*,*,#52872,.T.) ;
#74744=ORIENTED_EDGE('',*,*,#49386,.F.) ;
#74745=ORIENTED_EDGE('',*,*,#52876,.F.) ;
#74746=ORIENTED_EDGE('',*,*,#51598,.F.) ;
#74747=ORIENTED_EDGE('',*,*,#52873,.T.) ;
#74748=ORIENTED_EDGE('',*,*,#51597,.F.) ;
#74749=ORIENTED_EDGE('',*,*,#52877,.F.) ;
#74750=ORIENTED_EDGE('',*,*,#51602,.F.) ;
#74751=ORIENTED_EDGE('',*,*,#52878,.F.) ;
#74752=ORIENTED_EDGE('',*,*,#51599,.F.) ;
#74753=ORIENTED_EDGE('',*,*,#52879,.F.) ;
#74754=ORIENTED_EDGE('',*,*,#51686,.F.) ;
#74755=ORIENTED_EDGE('',*,*,#52874,.T.) ;
#74756=ORIENTED_EDGE('',*,*,#51600,.F.) ;
#74757=ORIENTED_EDGE('',*,*,#52880,.F.) ;
#74758=ORIENTED_EDGE('',*,*,#51590,.F.) ;
#74759=ORIENTED_EDGE('',*,*,#52875,.T.) ;
#74760=ORIENTED_EDGE('',*,*,#51589,.F.) ;
#74761=ORIENTED_EDGE('',*,*,#52881,.F.) ;
#74762=ORIENTED_EDGE('',*,*,#49390,.F.) ;
#74763=ORIENTED_EDGE('',*,*,#52882,.F.) ;
#74764=ORIENTED_EDGE('',*,*,#49384,.F.) ;
#74765=ORIENTED_EDGE('',*,*,#52883,.F.) ;
#74766=ORIENTED_EDGE('',*,*,#51591,.F.) ;
#74767=ORIENTED_EDGE('',*,*,#49385,.T.) ;
#74768=ORIENTED_EDGE('',*,*,#52882,.T.) ;
#74769=ORIENTED_EDGE('',*,*,#52884,.F.) ;
#74770=ORIENTED_EDGE('',*,*,#52876,.T.) ;
#74771=ORIENTED_EDGE('',*,*,#52879,.T.) ;
#74772=ORIENTED_EDGE('',*,*,#52877,.T.) ;
#74773=ORIENTED_EDGE('',*,*,#52885,.F.) ;
#74774=ORIENTED_EDGE('',*,*,#52880,.T.) ;
#74775=ORIENTED_EDGE('',*,*,#52878,.T.) ;
#74776=ORIENTED_EDGE('',*,*,#52886,.F.) ;
#74777=ORIENTED_EDGE('',*,*,#49383,.T.) ;
#74778=ORIENTED_EDGE('',*,*,#52881,.T.) ;
#74779=ORIENTED_EDGE('',*,*,#52887,.F.) ;
#74780=ORIENTED_EDGE('',*,*,#52883,.T.) ;
#74781=ORIENTED_EDGE('',*,*,#52884,.T.) ;
#74782=ORIENTED_EDGE('',*,*,#51594,.F.) ;
#74783=ORIENTED_EDGE('',*,*,#52888,.F.) ;
#74784=ORIENTED_EDGE('',*,*,#51595,.F.) ;
#74785=ORIENTED_EDGE('',*,*,#52885,.T.) ;
#74786=ORIENTED_EDGE('',*,*,#51596,.F.) ;
#74787=ORIENTED_EDGE('',*,*,#52889,.F.) ;
#74788=ORIENTED_EDGE('',*,*,#51683,.F.) ;
#74789=ORIENTED_EDGE('',*,*,#52886,.T.) ;
#74790=ORIENTED_EDGE('',*,*,#51685,.F.) ;
#74791=ORIENTED_EDGE('',*,*,#52890,.F.) ;
#74792=ORIENTED_EDGE('',*,*,#51587,.F.) ;
#74793=ORIENTED_EDGE('',*,*,#52887,.T.) ;
#74794=ORIENTED_EDGE('',*,*,#51588,.F.) ;
#74795=ORIENTED_EDGE('',*,*,#52891,.F.) ;
#74796=ORIENTED_EDGE('',*,*,#51592,.F.) ;
#74797=ORIENTED_EDGE('',*,*,#52889,.T.) ;
#74798=ORIENTED_EDGE('',*,*,#52888,.T.) ;
#74799=ORIENTED_EDGE('',*,*,#52892,.F.) ;
#74800=ORIENTED_EDGE('',*,*,#52891,.T.) ;
#74801=ORIENTED_EDGE('',*,*,#52890,.T.) ;
#74802=ORIENTED_EDGE('',*,*,#52893,.F.) ;
#74803=ORIENTED_EDGE('',*,*,#52892,.T.) ;
#74804=ORIENTED_EDGE('',*,*,#51593,.F.) ;
#74805=ORIENTED_EDGE('',*,*,#52893,.T.) ;
#74806=ORIENTED_EDGE('',*,*,#51684,.F.) ;
#74807=ORIENTED_EDGE('',*,*,#51692,.F.) ;
#74808=ORIENTED_EDGE('',*,*,#51705,.F.) ;
#74809=ORIENTED_EDGE('',*,*,#52894,.F.) ;
#74810=ORIENTED_EDGE('',*,*,#51697,.F.) ;
#74811=ORIENTED_EDGE('',*,*,#52895,.F.) ;
#74812=ORIENTED_EDGE('',*,*,#51695,.F.) ;
#74813=ORIENTED_EDGE('',*,*,#52896,.F.) ;
#74814=ORIENTED_EDGE('',*,*,#51862,.F.) ;
#74815=ORIENTED_EDGE('',*,*,#51694,.F.) ;
#74816=ORIENTED_EDGE('',*,*,#51696,.F.) ;
#74817=ORIENTED_EDGE('',*,*,#52897,.F.) ;
#74818=ORIENTED_EDGE('',*,*,#51700,.F.) ;
#74819=ORIENTED_EDGE('',*,*,#52896,.T.) ;
#74820=ORIENTED_EDGE('',*,*,#52894,.T.) ;
#74821=ORIENTED_EDGE('',*,*,#52898,.F.) ;
#74822=ORIENTED_EDGE('',*,*,#52897,.T.) ;
#74823=ORIENTED_EDGE('',*,*,#52895,.T.) ;
#74824=ORIENTED_EDGE('',*,*,#52899,.F.) ;
#74825=ORIENTED_EDGE('',*,*,#51690,.F.) ;
#74826=ORIENTED_EDGE('',*,*,#51703,.F.) ;
#74827=ORIENTED_EDGE('',*,*,#52900,.F.) ;
#74828=ORIENTED_EDGE('',*,*,#51706,.F.) ;
#74829=ORIENTED_EDGE('',*,*,#52898,.T.) ;
#74830=ORIENTED_EDGE('',*,*,#51704,.F.) ;
#74831=ORIENTED_EDGE('',*,*,#52901,.F.) ;
#74832=ORIENTED_EDGE('',*,*,#51859,.F.) ;
#74833=ORIENTED_EDGE('',*,*,#52899,.T.) ;
#74834=ORIENTED_EDGE('',*,*,#51861,.F.) ;
#74835=ORIENTED_EDGE('',*,*,#52902,.F.) ;
#74836=ORIENTED_EDGE('',*,*,#51698,.F.) ;
#74837=ORIENTED_EDGE('',*,*,#51688,.F.) ;
#74838=ORIENTED_EDGE('',*,*,#51699,.F.) ;
#74839=ORIENTED_EDGE('',*,*,#52903,.F.) ;
#74840=ORIENTED_EDGE('',*,*,#51701,.F.) ;
#74841=ORIENTED_EDGE('',*,*,#52901,.T.) ;
#74842=ORIENTED_EDGE('',*,*,#52900,.T.) ;
#74843=ORIENTED_EDGE('',*,*,#52904,.F.) ;
#74844=ORIENTED_EDGE('',*,*,#52903,.T.) ;
#74845=ORIENTED_EDGE('',*,*,#52902,.T.) ;
#74846=ORIENTED_EDGE('',*,*,#52905,.F.) ;
#74847=ORIENTED_EDGE('',*,*,#52904,.T.) ;
#74848=ORIENTED_EDGE('',*,*,#51702,.F.) ;
#74849=ORIENTED_EDGE('',*,*,#52905,.T.) ;
#74850=ORIENTED_EDGE('',*,*,#51860,.F.) ;
#74851=ORIENTED_EDGE('',*,*,#52906,.F.) ;
#74852=ORIENTED_EDGE('',*,*,#52018,.F.) ;
#74853=ORIENTED_EDGE('',*,*,#52907,.F.) ;
#74854=ORIENTED_EDGE('',*,*,#52033,.F.) ;
#74855=ORIENTED_EDGE('',*,*,#52907,.T.) ;
#74856=ORIENTED_EDGE('',*,*,#52021,.F.) ;
#74857=ORIENTED_EDGE('',*,*,#52908,.F.) ;
#74858=ORIENTED_EDGE('',*,*,#52015,.F.) ;
#74859=ORIENTED_EDGE('',*,*,#52906,.T.) ;
#74860=ORIENTED_EDGE('',*,*,#52909,.F.) ;
#74861=ORIENTED_EDGE('',*,*,#52908,.T.) ;
#74862=ORIENTED_EDGE('',*,*,#52024,.F.) ;
#74863=ORIENTED_EDGE('',*,*,#52910,.F.) ;
#74864=ORIENTED_EDGE('',*,*,#52030,.F.) ;
#74865=ORIENTED_EDGE('',*,*,#52909,.T.) ;
#74866=ORIENTED_EDGE('',*,*,#52032,.F.) ;
#74867=ORIENTED_EDGE('',*,*,#52911,.F.) ;
#74868=ORIENTED_EDGE('',*,*,#52012,.F.) ;
#74869=ORIENTED_EDGE('',*,*,#52910,.T.) ;
#74870=ORIENTED_EDGE('',*,*,#52027,.F.) ;
#74871=ORIENTED_EDGE('',*,*,#52912,.F.) ;
#74872=ORIENTED_EDGE('',*,*,#52009,.F.) ;
#74873=ORIENTED_EDGE('',*,*,#52911,.T.) ;
#74874=ORIENTED_EDGE('',*,*,#52913,.F.) ;
#74875=ORIENTED_EDGE('',*,*,#52912,.T.) ;
#74876=ORIENTED_EDGE('',*,*,#52028,.F.) ;
#74877=ORIENTED_EDGE('',*,*,#52913,.T.) ;
#74878=ORIENTED_EDGE('',*,*,#52031,.F.) ;
#74879=ORIENTED_EDGE('',*,*,#49124,.F.) ;
#74880=ORIENTED_EDGE('',*,*,#51893,.F.) ;
#74881=ORIENTED_EDGE('',*,*,#49138,.F.) ;
#74882=ORIENTED_EDGE('',*,*,#51908,.F.) ;
#74883=ORIENTED_EDGE('',*,*,#49126,.F.) ;
#74884=ORIENTED_EDGE('',*,*,#51909,.F.) ;
#74885=ORIENTED_EDGE('',*,*,#49136,.F.) ;
#74886=ORIENTED_EDGE('',*,*,#51912,.F.) ;
#74887=ORIENTED_EDGE('',*,*,#49134,.F.) ;
#74888=ORIENTED_EDGE('',*,*,#51910,.F.) ;
#74889=ORIENTED_EDGE('',*,*,#49128,.F.) ;
#74890=ORIENTED_EDGE('',*,*,#51913,.F.) ;
#74891=ORIENTED_EDGE('',*,*,#49132,.F.) ;
#74892=ORIENTED_EDGE('',*,*,#49529,.F.) ;
#74893=ORIENTED_EDGE('',*,*,#49130,.F.) ;
#74894=ORIENTED_EDGE('',*,*,#51911,.F.) ;
#74895=ORIENTED_EDGE('',*,*,#52914,.F.) ;
#74896=ORIENTED_EDGE('',*,*,#52915,.F.) ;
#74897=ORIENTED_EDGE('',*,*,#52916,.F.) ;
#74898=ORIENTED_EDGE('',*,*,#52915,.T.) ;
#74899=ORIENTED_EDGE('',*,*,#51395,.F.) ;
#74900=ORIENTED_EDGE('',*,*,#52917,.F.) ;
#74901=ORIENTED_EDGE('',*,*,#51390,.F.) ;
#74902=ORIENTED_EDGE('',*,*,#52916,.T.) ;
#74903=ORIENTED_EDGE('',*,*,#51389,.F.) ;
#74904=ORIENTED_EDGE('',*,*,#52918,.F.) ;
#74905=ORIENTED_EDGE('',*,*,#51391,.F.) ;
#74906=ORIENTED_EDGE('',*,*,#52914,.T.) ;
#74907=ORIENTED_EDGE('',*,*,#51394,.F.) ;
#74908=ORIENTED_EDGE('',*,*,#52919,.F.) ;
#74909=ORIENTED_EDGE('',*,*,#51396,.F.) ;
#74910=ORIENTED_EDGE('',*,*,#51400,.F.) ;
#74911=ORIENTED_EDGE('',*,*,#52920,.T.) ;
#74912=ORIENTED_EDGE('',*,*,#51169,.F.) ;
#74913=ORIENTED_EDGE('',*,*,#52921,.F.) ;
#74914=ORIENTED_EDGE('',*,*,#52917,.T.) ;
#74915=ORIENTED_EDGE('',*,*,#52921,.T.) ;
#74916=ORIENTED_EDGE('',*,*,#52922,.F.) ;
#74917=ORIENTED_EDGE('',*,*,#52923,.F.) ;
#74918=ORIENTED_EDGE('',*,*,#52918,.T.) ;
#74919=ORIENTED_EDGE('',*,*,#52924,.F.) ;
#74920=ORIENTED_EDGE('',*,*,#49636,.T.) ;
#74921=ORIENTED_EDGE('',*,*,#52925,.F.) ;
#74922=ORIENTED_EDGE('',*,*,#52919,.T.) ;
#74923=ORIENTED_EDGE('',*,*,#52926,.F.) ;
#74924=ORIENTED_EDGE('',*,*,#51399,.F.) ;
#74925=ORIENTED_EDGE('',*,*,#52927,.T.) ;
#74926=ORIENTED_EDGE('',*,*,#49475,.F.) ;
#74927=ORIENTED_EDGE('',*,*,#52928,.T.) ;
#74928=ORIENTED_EDGE('',*,*,#52922,.T.) ;
#74929=ORIENTED_EDGE('',*,*,#51168,.F.) ;
#74930=ORIENTED_EDGE('',*,*,#52929,.F.) ;
#74931=ORIENTED_EDGE('',*,*,#51387,.F.) ;
#74932=ORIENTED_EDGE('',*,*,#52924,.T.) ;
#74933=ORIENTED_EDGE('',*,*,#51388,.F.) ;
#74934=ORIENTED_EDGE('',*,*,#52930,.F.) ;
#74935=ORIENTED_EDGE('',*,*,#49637,.F.) ;
#74936=ORIENTED_EDGE('',*,*,#52923,.T.) ;
#74937=ORIENTED_EDGE('',*,*,#49643,.F.) ;
#74938=ORIENTED_EDGE('',*,*,#52931,.F.) ;
#74939=ORIENTED_EDGE('',*,*,#51392,.F.) ;
#74940=ORIENTED_EDGE('',*,*,#52926,.T.) ;
#74941=ORIENTED_EDGE('',*,*,#51393,.F.) ;
#74942=ORIENTED_EDGE('',*,*,#52932,.F.) ;
#74943=ORIENTED_EDGE('',*,*,#51383,.F.) ;
#74944=ORIENTED_EDGE('',*,*,#52925,.T.) ;
#74945=ORIENTED_EDGE('',*,*,#51386,.F.) ;
#74946=ORIENTED_EDGE('',*,*,#52933,.F.) ;
#74947=ORIENTED_EDGE('',*,*,#51397,.F.) ;
#74948=ORIENTED_EDGE('',*,*,#51179,.F.) ;
#74949=ORIENTED_EDGE('',*,*,#52934,.T.) ;
#74950=ORIENTED_EDGE('',*,*,#51398,.F.) ;
#74951=ORIENTED_EDGE('',*,*,#52935,.F.) ;
#74952=ORIENTED_EDGE('',*,*,#52929,.T.) ;
#74953=ORIENTED_EDGE('',*,*,#51167,.T.) ;
#74954=ORIENTED_EDGE('',*,*,#52936,.F.) ;
#74955=ORIENTED_EDGE('',*,*,#52930,.T.) ;
#74956=ORIENTED_EDGE('',*,*,#52931,.T.) ;
#74957=ORIENTED_EDGE('',*,*,#49642,.T.) ;
#74958=ORIENTED_EDGE('',*,*,#52937,.F.) ;
#74959=ORIENTED_EDGE('',*,*,#52932,.T.) ;
#74960=ORIENTED_EDGE('',*,*,#52935,.T.) ;
#74961=ORIENTED_EDGE('',*,*,#52933,.T.) ;
#74962=ORIENTED_EDGE('',*,*,#52938,.F.) ;
#74963=ORIENTED_EDGE('',*,*,#51163,.F.) ;
#74964=ORIENTED_EDGE('',*,*,#52939,.T.) ;
#74965=ORIENTED_EDGE('',*,*,#51157,.F.) ;
#74966=ORIENTED_EDGE('',*,*,#52940,.F.) ;
#74967=ORIENTED_EDGE('',*,*,#52936,.T.) ;
#74968=ORIENTED_EDGE('',*,*,#51166,.F.) ;
#74969=ORIENTED_EDGE('',*,*,#52941,.F.) ;
#74970=ORIENTED_EDGE('',*,*,#49638,.F.) ;
#74971=ORIENTED_EDGE('',*,*,#52937,.T.) ;
#74972=ORIENTED_EDGE('',*,*,#49641,.F.) ;
#74973=ORIENTED_EDGE('',*,*,#52942,.F.) ;
#74974=ORIENTED_EDGE('',*,*,#51384,.F.) ;
#74975=ORIENTED_EDGE('',*,*,#52938,.T.) ;
#74976=ORIENTED_EDGE('',*,*,#51385,.F.) ;
#74977=ORIENTED_EDGE('',*,*,#52943,.F.) ;
#74978=ORIENTED_EDGE('',*,*,#51180,.F.) ;
#74979=ORIENTED_EDGE('',*,*,#52940,.T.) ;
#74980=ORIENTED_EDGE('',*,*,#52810,.F.) ;
#74981=ORIENTED_EDGE('',*,*,#52944,.F.) ;
#74982=ORIENTED_EDGE('',*,*,#52945,.F.) ;
#74983=ORIENTED_EDGE('',*,*,#52941,.T.) ;
#74984=ORIENTED_EDGE('',*,*,#52946,.F.) ;
#74985=ORIENTED_EDGE('',*,*,#52943,.T.) ;
#74986=ORIENTED_EDGE('',*,*,#52942,.T.) ;
#74987=ORIENTED_EDGE('',*,*,#52947,.F.) ;
#74988=ORIENTED_EDGE('',*,*,#51181,.T.) ;
#74989=ORIENTED_EDGE('',*,*,#52944,.T.) ;
#74990=ORIENTED_EDGE('',*,*,#49709,.F.) ;
#74991=ORIENTED_EDGE('',*,*,#52948,.F.) ;
#74992=ORIENTED_EDGE('',*,*,#51164,.F.) ;
#74993=ORIENTED_EDGE('',*,*,#52946,.T.) ;
#74994=ORIENTED_EDGE('',*,*,#51165,.F.) ;
#74995=ORIENTED_EDGE('',*,*,#52949,.F.) ;
#74996=ORIENTED_EDGE('',*,*,#51171,.F.) ;
#74997=ORIENTED_EDGE('',*,*,#52945,.T.) ;
#74998=ORIENTED_EDGE('',*,*,#51174,.F.) ;
#74999=ORIENTED_EDGE('',*,*,#52950,.F.) ;
#75000=ORIENTED_EDGE('',*,*,#49639,.F.) ;
#75001=ORIENTED_EDGE('',*,*,#52947,.T.) ;
#75002=ORIENTED_EDGE('',*,*,#49640,.F.) ;
#75003=ORIENTED_EDGE('',*,*,#52951,.F.) ;
#75004=ORIENTED_EDGE('',*,*,#51182,.F.) ;
#75005=ORIENTED_EDGE('',*,*,#52948,.T.) ;
#75006=ORIENTED_EDGE('',*,*,#49708,.T.) ;
#75007=ORIENTED_EDGE('',*,*,#52952,.F.) ;
#75008=ORIENTED_EDGE('',*,*,#52949,.T.) ;
#75009=ORIENTED_EDGE('',*,*,#52951,.T.) ;
#75010=ORIENTED_EDGE('',*,*,#52950,.T.) ;
#75011=ORIENTED_EDGE('',*,*,#52953,.F.) ;
#75012=ORIENTED_EDGE('',*,*,#52952,.T.) ;
#75013=ORIENTED_EDGE('',*,*,#49707,.F.) ;
#75014=ORIENTED_EDGE('',*,*,#52954,.F.) ;
#75015=ORIENTED_EDGE('',*,*,#51172,.F.) ;
#75016=ORIENTED_EDGE('',*,*,#52953,.T.) ;
#75017=ORIENTED_EDGE('',*,*,#51173,.F.) ;
#75018=ORIENTED_EDGE('',*,*,#52955,.F.) ;
#75019=ORIENTED_EDGE('',*,*,#51183,.F.) ;
#75020=ORIENTED_EDGE('',*,*,#51187,.F.) ;
#75021=ORIENTED_EDGE('',*,*,#52956,.T.) ;
#75022=ORIENTED_EDGE('',*,*,#51175,.F.) ;
#75023=ORIENTED_EDGE('',*,*,#52957,.F.) ;
#75024=ORIENTED_EDGE('',*,*,#49704,.F.) ;
#75025=ORIENTED_EDGE('',*,*,#52958,.T.) ;
#75026=ORIENTED_EDGE('',*,*,#51188,.F.) ;
#75027=ORIENTED_EDGE('',*,*,#52959,.F.) ;
#75028=ORIENTED_EDGE('',*,*,#52954,.T.) ;
#75029=ORIENTED_EDGE('',*,*,#49706,.T.) ;
#75030=ORIENTED_EDGE('',*,*,#52960,.F.) ;
#75031=ORIENTED_EDGE('',*,*,#52955,.T.) ;
#75032=ORIENTED_EDGE('',*,*,#52959,.T.) ;
#75033=ORIENTED_EDGE('',*,*,#52957,.T.) ;
#75034=ORIENTED_EDGE('',*,*,#52961,.F.) ;
#75035=ORIENTED_EDGE('',*,*,#52960,.T.) ;
#75036=ORIENTED_EDGE('',*,*,#49705,.F.) ;
#75037=ORIENTED_EDGE('',*,*,#52961,.T.) ;
#75038=ORIENTED_EDGE('',*,*,#51184,.F.) ;
#75039=ORIENTED_EDGE('',*,*,#52342,.F.) ;
#75040=ORIENTED_EDGE('',*,*,#52353,.F.) ;
#75041=ORIENTED_EDGE('',*,*,#52352,.F.) ;
#75042=ORIENTED_EDGE('',*,*,#52962,.F.) ;
#75043=ORIENTED_EDGE('',*,*,#52343,.F.) ;
#75044=ORIENTED_EDGE('',*,*,#52962,.T.) ;
#75045=ORIENTED_EDGE('',*,*,#50776,.F.) ;
#75046=ORIENTED_EDGE('',*,*,#52963,.F.) ;
#75047=ORIENTED_EDGE('',*,*,#50762,.F.) ;
#75048=ORIENTED_EDGE('',*,*,#52350,.F.) ;
#75049=ORIENTED_EDGE('',*,*,#52349,.F.) ;
#75050=ORIENTED_EDGE('',*,*,#52348,.F.) ;
#75051=ORIENTED_EDGE('',*,*,#52964,.F.) ;
#75052=ORIENTED_EDGE('',*,*,#52351,.F.) ;
#75053=ORIENTED_EDGE('',*,*,#52965,.F.) ;
#75054=ORIENTED_EDGE('',*,*,#52963,.T.) ;
#75055=ORIENTED_EDGE('',*,*,#52966,.F.) ;
#75056=ORIENTED_EDGE('',*,*,#52340,.F.) ;
#75057=ORIENTED_EDGE('',*,*,#52345,.F.) ;
#75058=ORIENTED_EDGE('',*,*,#52344,.F.) ;
#75059=ORIENTED_EDGE('',*,*,#52967,.F.) ;
#75060=ORIENTED_EDGE('',*,*,#52341,.F.) ;
#75061=ORIENTED_EDGE('',*,*,#52964,.T.) ;
#75062=ORIENTED_EDGE('',*,*,#50772,.F.) ;
#75063=ORIENTED_EDGE('',*,*,#52968,.F.) ;
#75064=ORIENTED_EDGE('',*,*,#50774,.F.) ;
#75065=ORIENTED_EDGE('',*,*,#52966,.T.) ;
#75066=ORIENTED_EDGE('',*,*,#50775,.F.) ;
#75067=ORIENTED_EDGE('',*,*,#52969,.F.) ;
#75068=ORIENTED_EDGE('',*,*,#50900,.F.) ;
#75069=ORIENTED_EDGE('',*,*,#52965,.T.) ;
#75070=ORIENTED_EDGE('',*,*,#50899,.F.) ;
#75071=ORIENTED_EDGE('',*,*,#52970,.F.) ;
#75072=ORIENTED_EDGE('',*,*,#50763,.F.) ;
#75073=ORIENTED_EDGE('',*,*,#52967,.T.) ;
#75074=ORIENTED_EDGE('',*,*,#50764,.F.) ;
#75075=ORIENTED_EDGE('',*,*,#52971,.F.) ;
#75076=ORIENTED_EDGE('',*,*,#50768,.F.) ;
#75077=ORIENTED_EDGE('',*,*,#52969,.T.) ;
#75078=ORIENTED_EDGE('',*,*,#52968,.T.) ;
#75079=ORIENTED_EDGE('',*,*,#52972,.F.) ;
#75080=ORIENTED_EDGE('',*,*,#52971,.T.) ;
#75081=ORIENTED_EDGE('',*,*,#52970,.T.) ;
#75082=ORIENTED_EDGE('',*,*,#52973,.F.) ;
#75083=ORIENTED_EDGE('',*,*,#52972,.T.) ;
#75084=ORIENTED_EDGE('',*,*,#50771,.F.) ;
#75085=ORIENTED_EDGE('',*,*,#52974,.F.) ;
#75086=ORIENTED_EDGE('',*,*,#50897,.F.) ;
#75087=ORIENTED_EDGE('',*,*,#52973,.T.) ;
#75088=ORIENTED_EDGE('',*,*,#50898,.F.) ;
#75089=ORIENTED_EDGE('',*,*,#52975,.F.) ;
#75090=ORIENTED_EDGE('',*,*,#50765,.F.) ;
#75091=ORIENTED_EDGE('',*,*,#52975,.T.) ;
#75092=ORIENTED_EDGE('',*,*,#52974,.T.) ;
#75093=ORIENTED_EDGE('',*,*,#52976,.F.) ;
#75094=ORIENTED_EDGE('',*,*,#52976,.T.) ;
#75095=ORIENTED_EDGE('',*,*,#50770,.F.) ;
#75096=ORIENTED_EDGE('',*,*,#52977,.F.) ;
#75097=ORIENTED_EDGE('',*,*,#50766,.F.) ;
#75098=ORIENTED_EDGE('',*,*,#52346,.F.) ;
#75099=ORIENTED_EDGE('',*,*,#52339,.F.) ;
#75100=ORIENTED_EDGE('',*,*,#52338,.F.) ;
#75101=ORIENTED_EDGE('',*,*,#52977,.T.) ;
#75102=ORIENTED_EDGE('',*,*,#52347,.F.) ;
#75103=ORIENTED_EDGE('',*,*,#52483,.F.) ;
#75104=ORIENTED_EDGE('',*,*,#52482,.F.) ;
#75105=ORIENTED_EDGE('',*,*,#52481,.F.) ;
#75106=ORIENTED_EDGE('',*,*,#52978,.F.) ;
#75107=ORIENTED_EDGE('',*,*,#52484,.F.) ;
#75108=ORIENTED_EDGE('',*,*,#52978,.T.) ;
#75109=ORIENTED_EDGE('',*,*,#52480,.F.) ;
#75110=ORIENTED_EDGE('',*,*,#52979,.F.) ;
#75111=ORIENTED_EDGE('',*,*,#50579,.F.) ;
#75112=ORIENTED_EDGE('',*,*,#52979,.T.) ;
#75113=ORIENTED_EDGE('',*,*,#50492,.F.) ;
#75114=ORIENTED_EDGE('',*,*,#52980,.F.) ;
#75115=ORIENTED_EDGE('',*,*,#50580,.F.) ;
#75116=ORIENTED_EDGE('',*,*,#50480,.F.) ;
#75117=ORIENTED_EDGE('',*,*,#50581,.F.) ;
#75118=ORIENTED_EDGE('',*,*,#52981,.F.) ;
#75119=ORIENTED_EDGE('',*,*,#50486,.F.) ;
#75120=ORIENTED_EDGE('',*,*,#52981,.T.) ;
#75121=ORIENTED_EDGE('',*,*,#52980,.T.) ;
#75122=ORIENTED_EDGE('',*,*,#52982,.F.) ;
#75123=ORIENTED_EDGE('',*,*,#52982,.T.) ;
#75124=ORIENTED_EDGE('',*,*,#50491,.F.) ;
#75125=ORIENTED_EDGE('',*,*,#52983,.F.) ;
#75126=ORIENTED_EDGE('',*,*,#50487,.F.) ;
#75127=ORIENTED_EDGE('',*,*,#50482,.F.) ;
#75128=ORIENTED_EDGE('',*,*,#50488,.F.) ;
#75129=ORIENTED_EDGE('',*,*,#52984,.F.) ;
#75130=ORIENTED_EDGE('',*,*,#50643,.F.) ;
#75131=ORIENTED_EDGE('',*,*,#52984,.T.) ;
#75132=ORIENTED_EDGE('',*,*,#52983,.T.) ;
#75133=ORIENTED_EDGE('',*,*,#52985,.F.) ;
#75134=ORIENTED_EDGE('',*,*,#52985,.T.) ;
#75135=ORIENTED_EDGE('',*,*,#50490,.F.) ;
#75136=ORIENTED_EDGE('',*,*,#52986,.F.) ;
#75137=ORIENTED_EDGE('',*,*,#50644,.F.) ;
#75138=ORIENTED_EDGE('',*,*,#52986,.T.) ;
#75139=ORIENTED_EDGE('',*,*,#52479,.F.) ;
#75140=ORIENTED_EDGE('',*,*,#52987,.F.) ;
#75141=ORIENTED_EDGE('',*,*,#50645,.F.) ;
#75142=ORIENTED_EDGE('',*,*,#52987,.T.) ;
#75143=ORIENTED_EDGE('',*,*,#52478,.F.) ;
#75144=ORIENTED_EDGE('',*,*,#52487,.F.) ;
#75145=ORIENTED_EDGE('',*,*,#52488,.F.) ;
#75146=ORIENTED_EDGE('',*,*,#52493,.F.) ;
#75147=ORIENTED_EDGE('',*,*,#52988,.F.) ;
#75148=ORIENTED_EDGE('',*,*,#52988,.T.) ;
#75149=ORIENTED_EDGE('',*,*,#52492,.F.) ;
#75150=ORIENTED_EDGE('',*,*,#52989,.F.) ;
#75151=ORIENTED_EDGE('',*,*,#50640,.F.) ;
#75152=ORIENTED_EDGE('',*,*,#52989,.T.) ;
#75153=ORIENTED_EDGE('',*,*,#50474,.F.) ;
#75154=ORIENTED_EDGE('',*,*,#52990,.F.) ;
#75155=ORIENTED_EDGE('',*,*,#50641,.F.) ;
#75156=ORIENTED_EDGE('',*,*,#50484,.F.) ;
#75157=ORIENTED_EDGE('',*,*,#50642,.F.) ;
#75158=ORIENTED_EDGE('',*,*,#52991,.F.) ;
#75159=ORIENTED_EDGE('',*,*,#50478,.F.) ;
#75160=ORIENTED_EDGE('',*,*,#52991,.T.) ;
#75161=ORIENTED_EDGE('',*,*,#52990,.T.) ;
#75162=ORIENTED_EDGE('',*,*,#52992,.F.) ;
#75163=ORIENTED_EDGE('',*,*,#52992,.T.) ;
#75164=ORIENTED_EDGE('',*,*,#50473,.F.) ;
#75165=ORIENTED_EDGE('',*,*,#52993,.F.) ;
#75166=ORIENTED_EDGE('',*,*,#50475,.F.) ;
#75167=ORIENTED_EDGE('',*,*,#50485,.F.) ;
#75168=ORIENTED_EDGE('',*,*,#50476,.F.) ;
#75169=ORIENTED_EDGE('',*,*,#52994,.F.) ;
#75170=ORIENTED_EDGE('',*,*,#50582,.F.) ;
#75171=ORIENTED_EDGE('',*,*,#52994,.T.) ;
#75172=ORIENTED_EDGE('',*,*,#52993,.T.) ;
#75173=ORIENTED_EDGE('',*,*,#52995,.F.) ;
#75174=ORIENTED_EDGE('',*,*,#52995,.T.) ;
#75175=ORIENTED_EDGE('',*,*,#50472,.F.) ;
#75176=ORIENTED_EDGE('',*,*,#52996,.F.) ;
#75177=ORIENTED_EDGE('',*,*,#50583,.F.) ;
#75178=ORIENTED_EDGE('',*,*,#52996,.T.) ;
#75179=ORIENTED_EDGE('',*,*,#52491,.F.) ;
#75180=ORIENTED_EDGE('',*,*,#52997,.F.) ;
#75181=ORIENTED_EDGE('',*,*,#50584,.F.) ;
#75182=ORIENTED_EDGE('',*,*,#52489,.F.) ;
#75183=ORIENTED_EDGE('',*,*,#52486,.F.) ;
#75184=ORIENTED_EDGE('',*,*,#52485,.F.) ;
#75185=ORIENTED_EDGE('',*,*,#52997,.T.) ;
#75186=ORIENTED_EDGE('',*,*,#52490,.F.) ;
#75187=ORIENTED_EDGE('',*,*,#52998,.F.) ;
#75188=ORIENTED_EDGE('',*,*,#49484,.F.) ;
#75189=ORIENTED_EDGE('',*,*,#52999,.F.) ;
#75190=ORIENTED_EDGE('',*,*,#52041,.F.) ;
#75191=ORIENTED_EDGE('',*,*,#52999,.T.) ;
#75192=ORIENTED_EDGE('',*,*,#49483,.F.) ;
#75193=ORIENTED_EDGE('',*,*,#53000,.F.) ;
#75194=ORIENTED_EDGE('',*,*,#52044,.F.) ;
#75195=ORIENTED_EDGE('',*,*,#52998,.T.) ;
#75196=ORIENTED_EDGE('',*,*,#52038,.F.) ;
#75197=ORIENTED_EDGE('',*,*,#53001,.F.) ;
#75198=ORIENTED_EDGE('',*,*,#49485,.F.) ;
#75199=ORIENTED_EDGE('',*,*,#53000,.T.) ;
#75200=ORIENTED_EDGE('',*,*,#49482,.F.) ;
#75201=ORIENTED_EDGE('',*,*,#53002,.F.) ;
#75202=ORIENTED_EDGE('',*,*,#52047,.F.) ;
#75203=ORIENTED_EDGE('',*,*,#53001,.T.) ;
#75204=ORIENTED_EDGE('',*,*,#52035,.F.) ;
#75205=ORIENTED_EDGE('',*,*,#53003,.F.) ;
#75206=ORIENTED_EDGE('',*,*,#49486,.F.) ;
#75207=ORIENTED_EDGE('',*,*,#53002,.T.) ;
#75208=ORIENTED_EDGE('',*,*,#49481,.F.) ;
#75209=ORIENTED_EDGE('',*,*,#53004,.F.) ;
#75210=ORIENTED_EDGE('',*,*,#52050,.F.) ;
#75211=ORIENTED_EDGE('',*,*,#53003,.T.) ;
#75212=ORIENTED_EDGE('',*,*,#52057,.F.) ;
#75213=ORIENTED_EDGE('',*,*,#53005,.F.) ;
#75214=ORIENTED_EDGE('',*,*,#49479,.F.) ;
#75215=ORIENTED_EDGE('',*,*,#53004,.T.) ;
#75216=ORIENTED_EDGE('',*,*,#49480,.F.) ;
#75217=ORIENTED_EDGE('',*,*,#53005,.T.) ;
#75218=ORIENTED_EDGE('',*,*,#52053,.F.) ;
#75219=ORIENTED_EDGE('',*,*,#50906,.F.) ;
#75220=ORIENTED_EDGE('',*,*,#50920,.F.) ;
#75221=ORIENTED_EDGE('',*,*,#53006,.F.) ;
#75222=ORIENTED_EDGE('',*,*,#50909,.F.) ;
#75223=ORIENTED_EDGE('',*,*,#53007,.F.) ;
#75224=ORIENTED_EDGE('',*,*,#50910,.F.) ;
#75225=ORIENTED_EDGE('',*,*,#53008,.F.) ;
#75226=ORIENTED_EDGE('',*,*,#51056,.F.) ;
#75227=ORIENTED_EDGE('',*,*,#50908,.F.) ;
#75228=ORIENTED_EDGE('',*,*,#50911,.F.) ;
#75229=ORIENTED_EDGE('',*,*,#53009,.F.) ;
#75230=ORIENTED_EDGE('',*,*,#50912,.F.) ;
#75231=ORIENTED_EDGE('',*,*,#53008,.T.) ;
#75232=ORIENTED_EDGE('',*,*,#53006,.T.) ;
#75233=ORIENTED_EDGE('',*,*,#53010,.F.) ;
#75234=ORIENTED_EDGE('',*,*,#53009,.T.) ;
#75235=ORIENTED_EDGE('',*,*,#53007,.T.) ;
#75236=ORIENTED_EDGE('',*,*,#53011,.F.) ;
#75237=ORIENTED_EDGE('',*,*,#50904,.F.) ;
#75238=ORIENTED_EDGE('',*,*,#50916,.F.) ;
#75239=ORIENTED_EDGE('',*,*,#53012,.F.) ;
#75240=ORIENTED_EDGE('',*,*,#50918,.F.) ;
#75241=ORIENTED_EDGE('',*,*,#53010,.T.) ;
#75242=ORIENTED_EDGE('',*,*,#50919,.F.) ;
#75243=ORIENTED_EDGE('',*,*,#53013,.F.) ;
#75244=ORIENTED_EDGE('',*,*,#51053,.F.) ;
#75245=ORIENTED_EDGE('',*,*,#53011,.T.) ;
#75246=ORIENTED_EDGE('',*,*,#51055,.F.) ;
#75247=ORIENTED_EDGE('',*,*,#53014,.F.) ;
#75248=ORIENTED_EDGE('',*,*,#50913,.F.) ;
#75249=ORIENTED_EDGE('',*,*,#50902,.F.) ;
#75250=ORIENTED_EDGE('',*,*,#50914,.F.) ;
#75251=ORIENTED_EDGE('',*,*,#53015,.F.) ;
#75252=ORIENTED_EDGE('',*,*,#50917,.F.) ;
#75253=ORIENTED_EDGE('',*,*,#53013,.T.) ;
#75254=ORIENTED_EDGE('',*,*,#53012,.T.) ;
#75255=ORIENTED_EDGE('',*,*,#53016,.F.) ;
#75256=ORIENTED_EDGE('',*,*,#53015,.T.) ;
#75257=ORIENTED_EDGE('',*,*,#53014,.T.) ;
#75258=ORIENTED_EDGE('',*,*,#53017,.F.) ;
#75259=ORIENTED_EDGE('',*,*,#53016,.T.) ;
#75260=ORIENTED_EDGE('',*,*,#50915,.F.) ;
#75261=ORIENTED_EDGE('',*,*,#53017,.T.) ;
#75262=ORIENTED_EDGE('',*,*,#51054,.F.) ;
#75263=ORIENTED_EDGE('',*,*,#53018,.F.) ;
#75264=ORIENTED_EDGE('',*,*,#49356,.F.) ;
#75265=ORIENTED_EDGE('',*,*,#53019,.F.) ;
#75266=ORIENTED_EDGE('',*,*,#51585,.F.) ;
#75267=ORIENTED_EDGE('',*,*,#53019,.T.) ;
#75268=ORIENTED_EDGE('',*,*,#49355,.T.) ;
#75269=ORIENTED_EDGE('',*,*,#53020,.F.) ;
#75270=ORIENTED_EDGE('',*,*,#53021,.F.) ;
#75271=ORIENTED_EDGE('',*,*,#49357,.T.) ;
#75272=ORIENTED_EDGE('',*,*,#53018,.T.) ;
#75273=ORIENTED_EDGE('',*,*,#53022,.F.) ;
#75274=ORIENTED_EDGE('',*,*,#53023,.F.) ;
#75275=ORIENTED_EDGE('',*,*,#53020,.T.) ;
#75276=ORIENTED_EDGE('',*,*,#49354,.F.) ;
#75277=ORIENTED_EDGE('',*,*,#53024,.F.) ;
#75278=ORIENTED_EDGE('',*,*,#51582,.F.) ;
#75279=ORIENTED_EDGE('',*,*,#53021,.T.) ;
#75280=ORIENTED_EDGE('',*,*,#51581,.F.) ;
#75281=ORIENTED_EDGE('',*,*,#53025,.F.) ;
#75282=ORIENTED_EDGE('',*,*,#51586,.F.) ;
#75283=ORIENTED_EDGE('',*,*,#53026,.F.) ;
#75284=ORIENTED_EDGE('',*,*,#51583,.F.) ;
#75285=ORIENTED_EDGE('',*,*,#53027,.F.) ;
#75286=ORIENTED_EDGE('',*,*,#51710,.F.) ;
#75287=ORIENTED_EDGE('',*,*,#53022,.T.) ;
#75288=ORIENTED_EDGE('',*,*,#51584,.F.) ;
#75289=ORIENTED_EDGE('',*,*,#53028,.F.) ;
#75290=ORIENTED_EDGE('',*,*,#51574,.F.) ;
#75291=ORIENTED_EDGE('',*,*,#53023,.T.) ;
#75292=ORIENTED_EDGE('',*,*,#51573,.F.) ;
#75293=ORIENTED_EDGE('',*,*,#53029,.F.) ;
#75294=ORIENTED_EDGE('',*,*,#49358,.F.) ;
#75295=ORIENTED_EDGE('',*,*,#53030,.F.) ;
#75296=ORIENTED_EDGE('',*,*,#49352,.F.) ;
#75297=ORIENTED_EDGE('',*,*,#53031,.F.) ;
#75298=ORIENTED_EDGE('',*,*,#51575,.F.) ;
#75299=ORIENTED_EDGE('',*,*,#49353,.T.) ;
#75300=ORIENTED_EDGE('',*,*,#53030,.T.) ;
#75301=ORIENTED_EDGE('',*,*,#53032,.F.) ;
#75302=ORIENTED_EDGE('',*,*,#53024,.T.) ;
#75303=ORIENTED_EDGE('',*,*,#53027,.T.) ;
#75304=ORIENTED_EDGE('',*,*,#53025,.T.) ;
#75305=ORIENTED_EDGE('',*,*,#53033,.F.) ;
#75306=ORIENTED_EDGE('',*,*,#53028,.T.) ;
#75307=ORIENTED_EDGE('',*,*,#53026,.T.) ;
#75308=ORIENTED_EDGE('',*,*,#53034,.F.) ;
#75309=ORIENTED_EDGE('',*,*,#49351,.T.) ;
#75310=ORIENTED_EDGE('',*,*,#53029,.T.) ;
#75311=ORIENTED_EDGE('',*,*,#53035,.F.) ;
#75312=ORIENTED_EDGE('',*,*,#53031,.T.) ;
#75313=ORIENTED_EDGE('',*,*,#53032,.T.) ;
#75314=ORIENTED_EDGE('',*,*,#51578,.F.) ;
#75315=ORIENTED_EDGE('',*,*,#53036,.F.) ;
#75316=ORIENTED_EDGE('',*,*,#51579,.F.) ;
#75317=ORIENTED_EDGE('',*,*,#53033,.T.) ;
#75318=ORIENTED_EDGE('',*,*,#51580,.F.) ;
#75319=ORIENTED_EDGE('',*,*,#53037,.F.) ;
#75320=ORIENTED_EDGE('',*,*,#51707,.F.) ;
#75321=ORIENTED_EDGE('',*,*,#53034,.T.) ;
#75322=ORIENTED_EDGE('',*,*,#51709,.F.) ;
#75323=ORIENTED_EDGE('',*,*,#53038,.F.) ;
#75324=ORIENTED_EDGE('',*,*,#51571,.F.) ;
#75325=ORIENTED_EDGE('',*,*,#53035,.T.) ;
#75326=ORIENTED_EDGE('',*,*,#51572,.F.) ;
#75327=ORIENTED_EDGE('',*,*,#53039,.F.) ;
#75328=ORIENTED_EDGE('',*,*,#51576,.F.) ;
#75329=ORIENTED_EDGE('',*,*,#53037,.T.) ;
#75330=ORIENTED_EDGE('',*,*,#53036,.T.) ;
#75331=ORIENTED_EDGE('',*,*,#53040,.F.) ;
#75332=ORIENTED_EDGE('',*,*,#53039,.T.) ;
#75333=ORIENTED_EDGE('',*,*,#53038,.T.) ;
#75334=ORIENTED_EDGE('',*,*,#53041,.F.) ;
#75335=ORIENTED_EDGE('',*,*,#53040,.T.) ;
#75336=ORIENTED_EDGE('',*,*,#51577,.F.) ;
#75337=ORIENTED_EDGE('',*,*,#53041,.T.) ;
#75338=ORIENTED_EDGE('',*,*,#51708,.F.) ;
#75339=ORIENTED_EDGE('',*,*,#51716,.F.) ;
#75340=ORIENTED_EDGE('',*,*,#51729,.F.) ;
#75341=ORIENTED_EDGE('',*,*,#53042,.F.) ;
#75342=ORIENTED_EDGE('',*,*,#51721,.F.) ;
#75343=ORIENTED_EDGE('',*,*,#53043,.F.) ;
#75344=ORIENTED_EDGE('',*,*,#51719,.F.) ;
#75345=ORIENTED_EDGE('',*,*,#53044,.F.) ;
#75346=ORIENTED_EDGE('',*,*,#51866,.F.) ;
#75347=ORIENTED_EDGE('',*,*,#51718,.F.) ;
#75348=ORIENTED_EDGE('',*,*,#51720,.F.) ;
#75349=ORIENTED_EDGE('',*,*,#53045,.F.) ;
#75350=ORIENTED_EDGE('',*,*,#51724,.F.) ;
#75351=ORIENTED_EDGE('',*,*,#53044,.T.) ;
#75352=ORIENTED_EDGE('',*,*,#53042,.T.) ;
#75353=ORIENTED_EDGE('',*,*,#53046,.F.) ;
#75354=ORIENTED_EDGE('',*,*,#53045,.T.) ;
#75355=ORIENTED_EDGE('',*,*,#53043,.T.) ;
#75356=ORIENTED_EDGE('',*,*,#53047,.F.) ;
#75357=ORIENTED_EDGE('',*,*,#51714,.F.) ;
#75358=ORIENTED_EDGE('',*,*,#51727,.F.) ;
#75359=ORIENTED_EDGE('',*,*,#53048,.F.) ;
#75360=ORIENTED_EDGE('',*,*,#51730,.F.) ;
#75361=ORIENTED_EDGE('',*,*,#53046,.T.) ;
#75362=ORIENTED_EDGE('',*,*,#51728,.F.) ;
#75363=ORIENTED_EDGE('',*,*,#53049,.F.) ;
#75364=ORIENTED_EDGE('',*,*,#51863,.F.) ;
#75365=ORIENTED_EDGE('',*,*,#53047,.T.) ;
#75366=ORIENTED_EDGE('',*,*,#51865,.F.) ;
#75367=ORIENTED_EDGE('',*,*,#53050,.F.) ;
#75368=ORIENTED_EDGE('',*,*,#51722,.F.) ;
#75369=ORIENTED_EDGE('',*,*,#51712,.F.) ;
#75370=ORIENTED_EDGE('',*,*,#51723,.F.) ;
#75371=ORIENTED_EDGE('',*,*,#53051,.F.) ;
#75372=ORIENTED_EDGE('',*,*,#51725,.F.) ;
#75373=ORIENTED_EDGE('',*,*,#53049,.T.) ;
#75374=ORIENTED_EDGE('',*,*,#53048,.T.) ;
#75375=ORIENTED_EDGE('',*,*,#53052,.F.) ;
#75376=ORIENTED_EDGE('',*,*,#53051,.T.) ;
#75377=ORIENTED_EDGE('',*,*,#53050,.T.) ;
#75378=ORIENTED_EDGE('',*,*,#53053,.F.) ;
#75379=ORIENTED_EDGE('',*,*,#53052,.T.) ;
#75380=ORIENTED_EDGE('',*,*,#51726,.F.) ;
#75381=ORIENTED_EDGE('',*,*,#53053,.T.) ;
#75382=ORIENTED_EDGE('',*,*,#51864,.F.) ;
#75383=ORIENTED_EDGE('',*,*,#53054,.F.) ;
#75384=ORIENTED_EDGE('',*,*,#52046,.F.) ;
#75385=ORIENTED_EDGE('',*,*,#53055,.F.) ;
#75386=ORIENTED_EDGE('',*,*,#52061,.F.) ;
#75387=ORIENTED_EDGE('',*,*,#53055,.T.) ;
#75388=ORIENTED_EDGE('',*,*,#52049,.F.) ;
#75389=ORIENTED_EDGE('',*,*,#53056,.F.) ;
#75390=ORIENTED_EDGE('',*,*,#52043,.F.) ;
#75391=ORIENTED_EDGE('',*,*,#53054,.T.) ;
#75392=ORIENTED_EDGE('',*,*,#53057,.F.) ;
#75393=ORIENTED_EDGE('',*,*,#53056,.T.) ;
#75394=ORIENTED_EDGE('',*,*,#52052,.F.) ;
#75395=ORIENTED_EDGE('',*,*,#53058,.F.) ;
#75396=ORIENTED_EDGE('',*,*,#52058,.F.) ;
#75397=ORIENTED_EDGE('',*,*,#53057,.T.) ;
#75398=ORIENTED_EDGE('',*,*,#52060,.F.) ;
#75399=ORIENTED_EDGE('',*,*,#53059,.F.) ;
#75400=ORIENTED_EDGE('',*,*,#52040,.F.) ;
#75401=ORIENTED_EDGE('',*,*,#53058,.T.) ;
#75402=ORIENTED_EDGE('',*,*,#52055,.F.) ;
#75403=ORIENTED_EDGE('',*,*,#53060,.F.) ;
#75404=ORIENTED_EDGE('',*,*,#52037,.F.) ;
#75405=ORIENTED_EDGE('',*,*,#53059,.T.) ;
#75406=ORIENTED_EDGE('',*,*,#53061,.F.) ;
#75407=ORIENTED_EDGE('',*,*,#53060,.T.) ;
#75408=ORIENTED_EDGE('',*,*,#52056,.F.) ;
#75409=ORIENTED_EDGE('',*,*,#53061,.T.) ;
#75410=ORIENTED_EDGE('',*,*,#52059,.F.) ;
#75411=ORIENTED_EDGE('',*,*,#49142,.F.) ;
#75412=ORIENTED_EDGE('',*,*,#51892,.F.) ;
#75413=ORIENTED_EDGE('',*,*,#49156,.F.) ;
#75414=ORIENTED_EDGE('',*,*,#51914,.F.) ;
#75415=ORIENTED_EDGE('',*,*,#49144,.F.) ;
#75416=ORIENTED_EDGE('',*,*,#51915,.F.) ;
#75417=ORIENTED_EDGE('',*,*,#49154,.F.) ;
#75418=ORIENTED_EDGE('',*,*,#51918,.F.) ;
#75419=ORIENTED_EDGE('',*,*,#49152,.F.) ;
#75420=ORIENTED_EDGE('',*,*,#51916,.F.) ;
#75421=ORIENTED_EDGE('',*,*,#49146,.F.) ;
#75422=ORIENTED_EDGE('',*,*,#51919,.F.) ;
#75423=ORIENTED_EDGE('',*,*,#49150,.F.) ;
#75424=ORIENTED_EDGE('',*,*,#49528,.F.) ;
#75425=ORIENTED_EDGE('',*,*,#49148,.F.) ;
#75426=ORIENTED_EDGE('',*,*,#51917,.F.) ;
#75427=ORIENTED_EDGE('',*,*,#53062,.F.) ;
#75428=ORIENTED_EDGE('',*,*,#53063,.F.) ;
#75429=ORIENTED_EDGE('',*,*,#53064,.F.) ;
#75430=ORIENTED_EDGE('',*,*,#53063,.T.) ;
#75431=ORIENTED_EDGE('',*,*,#51413,.F.) ;
#75432=ORIENTED_EDGE('',*,*,#53065,.F.) ;
#75433=ORIENTED_EDGE('',*,*,#51408,.F.) ;
#75434=ORIENTED_EDGE('',*,*,#53064,.T.) ;
#75435=ORIENTED_EDGE('',*,*,#51407,.F.) ;
#75436=ORIENTED_EDGE('',*,*,#53066,.F.) ;
#75437=ORIENTED_EDGE('',*,*,#51409,.F.) ;
#75438=ORIENTED_EDGE('',*,*,#53062,.T.) ;
#75439=ORIENTED_EDGE('',*,*,#51412,.F.) ;
#75440=ORIENTED_EDGE('',*,*,#53067,.F.) ;
#75441=ORIENTED_EDGE('',*,*,#51414,.F.) ;
#75442=ORIENTED_EDGE('',*,*,#51418,.F.) ;
#75443=ORIENTED_EDGE('',*,*,#53068,.T.) ;
#75444=ORIENTED_EDGE('',*,*,#51197,.F.) ;
#75445=ORIENTED_EDGE('',*,*,#53069,.F.) ;
#75446=ORIENTED_EDGE('',*,*,#53065,.T.) ;
#75447=ORIENTED_EDGE('',*,*,#53069,.T.) ;
#75448=ORIENTED_EDGE('',*,*,#53070,.F.) ;
#75449=ORIENTED_EDGE('',*,*,#53071,.F.) ;
#75450=ORIENTED_EDGE('',*,*,#53066,.T.) ;
#75451=ORIENTED_EDGE('',*,*,#53072,.F.) ;
#75452=ORIENTED_EDGE('',*,*,#49628,.T.) ;
#75453=ORIENTED_EDGE('',*,*,#53073,.F.) ;
#75454=ORIENTED_EDGE('',*,*,#53067,.T.) ;
#75455=ORIENTED_EDGE('',*,*,#53074,.F.) ;
#75456=ORIENTED_EDGE('',*,*,#51417,.F.) ;
#75457=ORIENTED_EDGE('',*,*,#53075,.T.) ;
#75458=ORIENTED_EDGE('',*,*,#49463,.F.) ;
#75459=ORIENTED_EDGE('',*,*,#53076,.T.) ;
#75460=ORIENTED_EDGE('',*,*,#53070,.T.) ;
#75461=ORIENTED_EDGE('',*,*,#51196,.F.) ;
#75462=ORIENTED_EDGE('',*,*,#53077,.F.) ;
#75463=ORIENTED_EDGE('',*,*,#51405,.F.) ;
#75464=ORIENTED_EDGE('',*,*,#53072,.T.) ;
#75465=ORIENTED_EDGE('',*,*,#51406,.F.) ;
#75466=ORIENTED_EDGE('',*,*,#53078,.F.) ;
#75467=ORIENTED_EDGE('',*,*,#49629,.F.) ;
#75468=ORIENTED_EDGE('',*,*,#53071,.T.) ;
#75469=ORIENTED_EDGE('',*,*,#49635,.F.) ;
#75470=ORIENTED_EDGE('',*,*,#53079,.F.) ;
#75471=ORIENTED_EDGE('',*,*,#51410,.F.) ;
#75472=ORIENTED_EDGE('',*,*,#53074,.T.) ;
#75473=ORIENTED_EDGE('',*,*,#51411,.F.) ;
#75474=ORIENTED_EDGE('',*,*,#53080,.F.) ;
#75475=ORIENTED_EDGE('',*,*,#51401,.F.) ;
#75476=ORIENTED_EDGE('',*,*,#53073,.T.) ;
#75477=ORIENTED_EDGE('',*,*,#51404,.F.) ;
#75478=ORIENTED_EDGE('',*,*,#53081,.F.) ;
#75479=ORIENTED_EDGE('',*,*,#51415,.F.) ;
#75480=ORIENTED_EDGE('',*,*,#51207,.F.) ;
#75481=ORIENTED_EDGE('',*,*,#53082,.T.) ;
#75482=ORIENTED_EDGE('',*,*,#51416,.F.) ;
#75483=ORIENTED_EDGE('',*,*,#53083,.F.) ;
#75484=ORIENTED_EDGE('',*,*,#53077,.T.) ;
#75485=ORIENTED_EDGE('',*,*,#51195,.T.) ;
#75486=ORIENTED_EDGE('',*,*,#53084,.F.) ;
#75487=ORIENTED_EDGE('',*,*,#53078,.T.) ;
#75488=ORIENTED_EDGE('',*,*,#53079,.T.) ;
#75489=ORIENTED_EDGE('',*,*,#49634,.T.) ;
#75490=ORIENTED_EDGE('',*,*,#53085,.F.) ;
#75491=ORIENTED_EDGE('',*,*,#53080,.T.) ;
#75492=ORIENTED_EDGE('',*,*,#53083,.T.) ;
#75493=ORIENTED_EDGE('',*,*,#53081,.T.) ;
#75494=ORIENTED_EDGE('',*,*,#53086,.F.) ;
#75495=ORIENTED_EDGE('',*,*,#51191,.F.) ;
#75496=ORIENTED_EDGE('',*,*,#53087,.T.) ;
#75497=ORIENTED_EDGE('',*,*,#51185,.F.) ;
#75498=ORIENTED_EDGE('',*,*,#53088,.F.) ;
#75499=ORIENTED_EDGE('',*,*,#53084,.T.) ;
#75500=ORIENTED_EDGE('',*,*,#51194,.F.) ;
#75501=ORIENTED_EDGE('',*,*,#53089,.F.) ;
#75502=ORIENTED_EDGE('',*,*,#49630,.F.) ;
#75503=ORIENTED_EDGE('',*,*,#53085,.T.) ;
#75504=ORIENTED_EDGE('',*,*,#49633,.F.) ;
#75505=ORIENTED_EDGE('',*,*,#53090,.F.) ;
#75506=ORIENTED_EDGE('',*,*,#51402,.F.) ;
#75507=ORIENTED_EDGE('',*,*,#53086,.T.) ;
#75508=ORIENTED_EDGE('',*,*,#51403,.F.) ;
#75509=ORIENTED_EDGE('',*,*,#53091,.F.) ;
#75510=ORIENTED_EDGE('',*,*,#51208,.F.) ;
#75511=ORIENTED_EDGE('',*,*,#53088,.T.) ;
#75512=ORIENTED_EDGE('',*,*,#52958,.F.) ;
#75513=ORIENTED_EDGE('',*,*,#53092,.F.) ;
#75514=ORIENTED_EDGE('',*,*,#53093,.F.) ;
#75515=ORIENTED_EDGE('',*,*,#53089,.T.) ;
#75516=ORIENTED_EDGE('',*,*,#53094,.F.) ;
#75517=ORIENTED_EDGE('',*,*,#53091,.T.) ;
#75518=ORIENTED_EDGE('',*,*,#53090,.T.) ;
#75519=ORIENTED_EDGE('',*,*,#53095,.F.) ;
#75520=ORIENTED_EDGE('',*,*,#51209,.T.) ;
#75521=ORIENTED_EDGE('',*,*,#53092,.T.) ;
#75522=ORIENTED_EDGE('',*,*,#49703,.F.) ;
#75523=ORIENTED_EDGE('',*,*,#53096,.F.) ;
#75524=ORIENTED_EDGE('',*,*,#51192,.F.) ;
#75525=ORIENTED_EDGE('',*,*,#53094,.T.) ;
#75526=ORIENTED_EDGE('',*,*,#51193,.F.) ;
#75527=ORIENTED_EDGE('',*,*,#53097,.F.) ;
#75528=ORIENTED_EDGE('',*,*,#51199,.F.) ;
#75529=ORIENTED_EDGE('',*,*,#53093,.T.) ;
#75530=ORIENTED_EDGE('',*,*,#51202,.F.) ;
#75531=ORIENTED_EDGE('',*,*,#53098,.F.) ;
#75532=ORIENTED_EDGE('',*,*,#49631,.F.) ;
#75533=ORIENTED_EDGE('',*,*,#53095,.T.) ;
#75534=ORIENTED_EDGE('',*,*,#49632,.F.) ;
#75535=ORIENTED_EDGE('',*,*,#53099,.F.) ;
#75536=ORIENTED_EDGE('',*,*,#51210,.F.) ;
#75537=ORIENTED_EDGE('',*,*,#53096,.T.) ;
#75538=ORIENTED_EDGE('',*,*,#49702,.T.) ;
#75539=ORIENTED_EDGE('',*,*,#53100,.F.) ;
#75540=ORIENTED_EDGE('',*,*,#53097,.T.) ;
#75541=ORIENTED_EDGE('',*,*,#53099,.T.) ;
#75542=ORIENTED_EDGE('',*,*,#53098,.T.) ;
#75543=ORIENTED_EDGE('',*,*,#53101,.F.) ;
#75544=ORIENTED_EDGE('',*,*,#53100,.T.) ;
#75545=ORIENTED_EDGE('',*,*,#49701,.F.) ;
#75546=ORIENTED_EDGE('',*,*,#53102,.F.) ;
#75547=ORIENTED_EDGE('',*,*,#51200,.F.) ;
#75548=ORIENTED_EDGE('',*,*,#53101,.T.) ;
#75549=ORIENTED_EDGE('',*,*,#51201,.F.) ;
#75550=ORIENTED_EDGE('',*,*,#53103,.F.) ;
#75551=ORIENTED_EDGE('',*,*,#51211,.F.) ;
#75552=ORIENTED_EDGE('',*,*,#51215,.F.) ;
#75553=ORIENTED_EDGE('',*,*,#53104,.T.) ;
#75554=ORIENTED_EDGE('',*,*,#51203,.F.) ;
#75555=ORIENTED_EDGE('',*,*,#53105,.F.) ;
#75556=ORIENTED_EDGE('',*,*,#49698,.F.) ;
#75557=ORIENTED_EDGE('',*,*,#53106,.T.) ;
#75558=ORIENTED_EDGE('',*,*,#51216,.F.) ;
#75559=ORIENTED_EDGE('',*,*,#53107,.F.) ;
#75560=ORIENTED_EDGE('',*,*,#53102,.T.) ;
#75561=ORIENTED_EDGE('',*,*,#49700,.T.) ;
#75562=ORIENTED_EDGE('',*,*,#53108,.F.) ;
#75563=ORIENTED_EDGE('',*,*,#53103,.T.) ;
#75564=ORIENTED_EDGE('',*,*,#53107,.T.) ;
#75565=ORIENTED_EDGE('',*,*,#53105,.T.) ;
#75566=ORIENTED_EDGE('',*,*,#53109,.F.) ;
#75567=ORIENTED_EDGE('',*,*,#53108,.T.) ;
#75568=ORIENTED_EDGE('',*,*,#49699,.F.) ;
#75569=ORIENTED_EDGE('',*,*,#53109,.T.) ;
#75570=ORIENTED_EDGE('',*,*,#51212,.F.) ;
#75571=ORIENTED_EDGE('',*,*,#52326,.F.) ;
#75572=ORIENTED_EDGE('',*,*,#52337,.F.) ;
#75573=ORIENTED_EDGE('',*,*,#52336,.F.) ;
#75574=ORIENTED_EDGE('',*,*,#53110,.F.) ;
#75575=ORIENTED_EDGE('',*,*,#52327,.F.) ;
#75576=ORIENTED_EDGE('',*,*,#53110,.T.) ;
#75577=ORIENTED_EDGE('',*,*,#50760,.F.) ;
#75578=ORIENTED_EDGE('',*,*,#53111,.F.) ;
#75579=ORIENTED_EDGE('',*,*,#50746,.F.) ;
#75580=ORIENTED_EDGE('',*,*,#52334,.F.) ;
#75581=ORIENTED_EDGE('',*,*,#52333,.F.) ;
#75582=ORIENTED_EDGE('',*,*,#52332,.F.) ;
#75583=ORIENTED_EDGE('',*,*,#53112,.F.) ;
#75584=ORIENTED_EDGE('',*,*,#52335,.F.) ;
#75585=ORIENTED_EDGE('',*,*,#53113,.F.) ;
#75586=ORIENTED_EDGE('',*,*,#53111,.T.) ;
#75587=ORIENTED_EDGE('',*,*,#53114,.F.) ;
#75588=ORIENTED_EDGE('',*,*,#52324,.F.) ;
#75589=ORIENTED_EDGE('',*,*,#52329,.F.) ;
#75590=ORIENTED_EDGE('',*,*,#52328,.F.) ;
#75591=ORIENTED_EDGE('',*,*,#53115,.F.) ;
#75592=ORIENTED_EDGE('',*,*,#52325,.F.) ;
#75593=ORIENTED_EDGE('',*,*,#53112,.T.) ;
#75594=ORIENTED_EDGE('',*,*,#50756,.F.) ;
#75595=ORIENTED_EDGE('',*,*,#53116,.F.) ;
#75596=ORIENTED_EDGE('',*,*,#50758,.F.) ;
#75597=ORIENTED_EDGE('',*,*,#53114,.T.) ;
#75598=ORIENTED_EDGE('',*,*,#50759,.F.) ;
#75599=ORIENTED_EDGE('',*,*,#53117,.F.) ;
#75600=ORIENTED_EDGE('',*,*,#50924,.F.) ;
#75601=ORIENTED_EDGE('',*,*,#53113,.T.) ;
#75602=ORIENTED_EDGE('',*,*,#50923,.F.) ;
#75603=ORIENTED_EDGE('',*,*,#53118,.F.) ;
#75604=ORIENTED_EDGE('',*,*,#50747,.F.) ;
#75605=ORIENTED_EDGE('',*,*,#53115,.T.) ;
#75606=ORIENTED_EDGE('',*,*,#50748,.F.) ;
#75607=ORIENTED_EDGE('',*,*,#53119,.F.) ;
#75608=ORIENTED_EDGE('',*,*,#50752,.F.) ;
#75609=ORIENTED_EDGE('',*,*,#53117,.T.) ;
#75610=ORIENTED_EDGE('',*,*,#53116,.T.) ;
#75611=ORIENTED_EDGE('',*,*,#53120,.F.) ;
#75612=ORIENTED_EDGE('',*,*,#53119,.T.) ;
#75613=ORIENTED_EDGE('',*,*,#53118,.T.) ;
#75614=ORIENTED_EDGE('',*,*,#53121,.F.) ;
#75615=ORIENTED_EDGE('',*,*,#53120,.T.) ;
#75616=ORIENTED_EDGE('',*,*,#50755,.F.) ;
#75617=ORIENTED_EDGE('',*,*,#53122,.F.) ;
#75618=ORIENTED_EDGE('',*,*,#50921,.F.) ;
#75619=ORIENTED_EDGE('',*,*,#53121,.T.) ;
#75620=ORIENTED_EDGE('',*,*,#50922,.F.) ;
#75621=ORIENTED_EDGE('',*,*,#53123,.F.) ;
#75622=ORIENTED_EDGE('',*,*,#50749,.F.) ;
#75623=ORIENTED_EDGE('',*,*,#53123,.T.) ;
#75624=ORIENTED_EDGE('',*,*,#53122,.T.) ;
#75625=ORIENTED_EDGE('',*,*,#53124,.F.) ;
#75626=ORIENTED_EDGE('',*,*,#53124,.T.) ;
#75627=ORIENTED_EDGE('',*,*,#50754,.F.) ;
#75628=ORIENTED_EDGE('',*,*,#53125,.F.) ;
#75629=ORIENTED_EDGE('',*,*,#50750,.F.) ;
#75630=ORIENTED_EDGE('',*,*,#52330,.F.) ;
#75631=ORIENTED_EDGE('',*,*,#52323,.F.) ;
#75632=ORIENTED_EDGE('',*,*,#52322,.F.) ;
#75633=ORIENTED_EDGE('',*,*,#53125,.T.) ;
#75634=ORIENTED_EDGE('',*,*,#52331,.F.) ;
#75635=ORIENTED_EDGE('',*,*,#52499,.F.) ;
#75636=ORIENTED_EDGE('',*,*,#52498,.F.) ;
#75637=ORIENTED_EDGE('',*,*,#52497,.F.) ;
#75638=ORIENTED_EDGE('',*,*,#53126,.F.) ;
#75639=ORIENTED_EDGE('',*,*,#52500,.F.) ;
#75640=ORIENTED_EDGE('',*,*,#53126,.T.) ;
#75641=ORIENTED_EDGE('',*,*,#52496,.F.) ;
#75642=ORIENTED_EDGE('',*,*,#53127,.F.) ;
#75643=ORIENTED_EDGE('',*,*,#50586,.F.) ;
#75644=ORIENTED_EDGE('',*,*,#53127,.T.) ;
#75645=ORIENTED_EDGE('',*,*,#50470,.F.) ;
#75646=ORIENTED_EDGE('',*,*,#53128,.F.) ;
#75647=ORIENTED_EDGE('',*,*,#50587,.F.) ;
#75648=ORIENTED_EDGE('',*,*,#50458,.F.) ;
#75649=ORIENTED_EDGE('',*,*,#50588,.F.) ;
#75650=ORIENTED_EDGE('',*,*,#53129,.F.) ;
#75651=ORIENTED_EDGE('',*,*,#50464,.F.) ;
#75652=ORIENTED_EDGE('',*,*,#53129,.T.) ;
#75653=ORIENTED_EDGE('',*,*,#53128,.T.) ;
#75654=ORIENTED_EDGE('',*,*,#53130,.F.) ;
#75655=ORIENTED_EDGE('',*,*,#53130,.T.) ;
#75656=ORIENTED_EDGE('',*,*,#50469,.F.) ;
#75657=ORIENTED_EDGE('',*,*,#53131,.F.) ;
#75658=ORIENTED_EDGE('',*,*,#50465,.F.) ;
#75659=ORIENTED_EDGE('',*,*,#50460,.F.) ;
#75660=ORIENTED_EDGE('',*,*,#50466,.F.) ;
#75661=ORIENTED_EDGE('',*,*,#53132,.F.) ;
#75662=ORIENTED_EDGE('',*,*,#50650,.F.) ;
#75663=ORIENTED_EDGE('',*,*,#53132,.T.) ;
#75664=ORIENTED_EDGE('',*,*,#53131,.T.) ;
#75665=ORIENTED_EDGE('',*,*,#53133,.F.) ;
#75666=ORIENTED_EDGE('',*,*,#53133,.T.) ;
#75667=ORIENTED_EDGE('',*,*,#50468,.F.) ;
#75668=ORIENTED_EDGE('',*,*,#53134,.F.) ;
#75669=ORIENTED_EDGE('',*,*,#50651,.F.) ;
#75670=ORIENTED_EDGE('',*,*,#53134,.T.) ;
#75671=ORIENTED_EDGE('',*,*,#52495,.F.) ;
#75672=ORIENTED_EDGE('',*,*,#53135,.F.) ;
#75673=ORIENTED_EDGE('',*,*,#50652,.F.) ;
#75674=ORIENTED_EDGE('',*,*,#53135,.T.) ;
#75675=ORIENTED_EDGE('',*,*,#52494,.F.) ;
#75676=ORIENTED_EDGE('',*,*,#52503,.F.) ;
#75677=ORIENTED_EDGE('',*,*,#52504,.F.) ;
#75678=ORIENTED_EDGE('',*,*,#52509,.F.) ;
#75679=ORIENTED_EDGE('',*,*,#53136,.F.) ;
#75680=ORIENTED_EDGE('',*,*,#53136,.T.) ;
#75681=ORIENTED_EDGE('',*,*,#52508,.F.) ;
#75682=ORIENTED_EDGE('',*,*,#53137,.F.) ;
#75683=ORIENTED_EDGE('',*,*,#50647,.F.) ;
#75684=ORIENTED_EDGE('',*,*,#53137,.T.) ;
#75685=ORIENTED_EDGE('',*,*,#50452,.F.) ;
#75686=ORIENTED_EDGE('',*,*,#53138,.F.) ;
#75687=ORIENTED_EDGE('',*,*,#50648,.F.) ;
#75688=ORIENTED_EDGE('',*,*,#50462,.F.) ;
#75689=ORIENTED_EDGE('',*,*,#50649,.F.) ;
#75690=ORIENTED_EDGE('',*,*,#53139,.F.) ;
#75691=ORIENTED_EDGE('',*,*,#50456,.F.) ;
#75692=ORIENTED_EDGE('',*,*,#53139,.T.) ;
#75693=ORIENTED_EDGE('',*,*,#53138,.T.) ;
#75694=ORIENTED_EDGE('',*,*,#53140,.F.) ;
#75695=ORIENTED_EDGE('',*,*,#53140,.T.) ;
#75696=ORIENTED_EDGE('',*,*,#50451,.F.) ;
#75697=ORIENTED_EDGE('',*,*,#53141,.F.) ;
#75698=ORIENTED_EDGE('',*,*,#50453,.F.) ;
#75699=ORIENTED_EDGE('',*,*,#50463,.F.) ;
#75700=ORIENTED_EDGE('',*,*,#50454,.F.) ;
#75701=ORIENTED_EDGE('',*,*,#53142,.F.) ;
#75702=ORIENTED_EDGE('',*,*,#50589,.F.) ;
#75703=ORIENTED_EDGE('',*,*,#53142,.T.) ;
#75704=ORIENTED_EDGE('',*,*,#53141,.T.) ;
#75705=ORIENTED_EDGE('',*,*,#53143,.F.) ;
#75706=ORIENTED_EDGE('',*,*,#53143,.T.) ;
#75707=ORIENTED_EDGE('',*,*,#50450,.F.) ;
#75708=ORIENTED_EDGE('',*,*,#53144,.F.) ;
#75709=ORIENTED_EDGE('',*,*,#50590,.F.) ;
#75710=ORIENTED_EDGE('',*,*,#53144,.T.) ;
#75711=ORIENTED_EDGE('',*,*,#52507,.F.) ;
#75712=ORIENTED_EDGE('',*,*,#53145,.F.) ;
#75713=ORIENTED_EDGE('',*,*,#50591,.F.) ;
#75714=ORIENTED_EDGE('',*,*,#52505,.F.) ;
#75715=ORIENTED_EDGE('',*,*,#52502,.F.) ;
#75716=ORIENTED_EDGE('',*,*,#52501,.F.) ;
#75717=ORIENTED_EDGE('',*,*,#53145,.T.) ;
#75718=ORIENTED_EDGE('',*,*,#52506,.F.) ;
#75719=ORIENTED_EDGE('',*,*,#53146,.F.) ;
#75720=ORIENTED_EDGE('',*,*,#49472,.F.) ;
#75721=ORIENTED_EDGE('',*,*,#53147,.F.) ;
#75722=ORIENTED_EDGE('',*,*,#52069,.F.) ;
#75723=ORIENTED_EDGE('',*,*,#53147,.T.) ;
#75724=ORIENTED_EDGE('',*,*,#49471,.F.) ;
#75725=ORIENTED_EDGE('',*,*,#53148,.F.) ;
#75726=ORIENTED_EDGE('',*,*,#52072,.F.) ;
#75727=ORIENTED_EDGE('',*,*,#53146,.T.) ;
#75728=ORIENTED_EDGE('',*,*,#52066,.F.) ;
#75729=ORIENTED_EDGE('',*,*,#53149,.F.) ;
#75730=ORIENTED_EDGE('',*,*,#49473,.F.) ;
#75731=ORIENTED_EDGE('',*,*,#53148,.T.) ;
#75732=ORIENTED_EDGE('',*,*,#49470,.F.) ;
#75733=ORIENTED_EDGE('',*,*,#53150,.F.) ;
#75734=ORIENTED_EDGE('',*,*,#52075,.F.) ;
#75735=ORIENTED_EDGE('',*,*,#53149,.T.) ;
#75736=ORIENTED_EDGE('',*,*,#52063,.F.) ;
#75737=ORIENTED_EDGE('',*,*,#53151,.F.) ;
#75738=ORIENTED_EDGE('',*,*,#49474,.F.) ;
#75739=ORIENTED_EDGE('',*,*,#53150,.T.) ;
#75740=ORIENTED_EDGE('',*,*,#49469,.F.) ;
#75741=ORIENTED_EDGE('',*,*,#53152,.F.) ;
#75742=ORIENTED_EDGE('',*,*,#52078,.F.) ;
#75743=ORIENTED_EDGE('',*,*,#53151,.T.) ;
#75744=ORIENTED_EDGE('',*,*,#52085,.F.) ;
#75745=ORIENTED_EDGE('',*,*,#53153,.F.) ;
#75746=ORIENTED_EDGE('',*,*,#49467,.F.) ;
#75747=ORIENTED_EDGE('',*,*,#53152,.T.) ;
#75748=ORIENTED_EDGE('',*,*,#49468,.F.) ;
#75749=ORIENTED_EDGE('',*,*,#53153,.T.) ;
#75750=ORIENTED_EDGE('',*,*,#52081,.F.) ;
#75751=ORIENTED_EDGE('',*,*,#50930,.F.) ;
#75752=ORIENTED_EDGE('',*,*,#50944,.F.) ;
#75753=ORIENTED_EDGE('',*,*,#53154,.F.) ;
#75754=ORIENTED_EDGE('',*,*,#50933,.F.) ;
#75755=ORIENTED_EDGE('',*,*,#53155,.F.) ;
#75756=ORIENTED_EDGE('',*,*,#50934,.F.) ;
#75757=ORIENTED_EDGE('',*,*,#53156,.F.) ;
#75758=ORIENTED_EDGE('',*,*,#51060,.F.) ;
#75759=ORIENTED_EDGE('',*,*,#50932,.F.) ;
#75760=ORIENTED_EDGE('',*,*,#50935,.F.) ;
#75761=ORIENTED_EDGE('',*,*,#53157,.F.) ;
#75762=ORIENTED_EDGE('',*,*,#50936,.F.) ;
#75763=ORIENTED_EDGE('',*,*,#53156,.T.) ;
#75764=ORIENTED_EDGE('',*,*,#53154,.T.) ;
#75765=ORIENTED_EDGE('',*,*,#53158,.F.) ;
#75766=ORIENTED_EDGE('',*,*,#53157,.T.) ;
#75767=ORIENTED_EDGE('',*,*,#53155,.T.) ;
#75768=ORIENTED_EDGE('',*,*,#53159,.F.) ;
#75769=ORIENTED_EDGE('',*,*,#50928,.F.) ;
#75770=ORIENTED_EDGE('',*,*,#50940,.F.) ;
#75771=ORIENTED_EDGE('',*,*,#53160,.F.) ;
#75772=ORIENTED_EDGE('',*,*,#50942,.F.) ;
#75773=ORIENTED_EDGE('',*,*,#53158,.T.) ;
#75774=ORIENTED_EDGE('',*,*,#50943,.F.) ;
#75775=ORIENTED_EDGE('',*,*,#53161,.F.) ;
#75776=ORIENTED_EDGE('',*,*,#51057,.F.) ;
#75777=ORIENTED_EDGE('',*,*,#53159,.T.) ;
#75778=ORIENTED_EDGE('',*,*,#51059,.F.) ;
#75779=ORIENTED_EDGE('',*,*,#53162,.F.) ;
#75780=ORIENTED_EDGE('',*,*,#50937,.F.) ;
#75781=ORIENTED_EDGE('',*,*,#50926,.F.) ;
#75782=ORIENTED_EDGE('',*,*,#50938,.F.) ;
#75783=ORIENTED_EDGE('',*,*,#53163,.F.) ;
#75784=ORIENTED_EDGE('',*,*,#50941,.F.) ;
#75785=ORIENTED_EDGE('',*,*,#53161,.T.) ;
#75786=ORIENTED_EDGE('',*,*,#53160,.T.) ;
#75787=ORIENTED_EDGE('',*,*,#53164,.F.) ;
#75788=ORIENTED_EDGE('',*,*,#53163,.T.) ;
#75789=ORIENTED_EDGE('',*,*,#53162,.T.) ;
#75790=ORIENTED_EDGE('',*,*,#53165,.F.) ;
#75791=ORIENTED_EDGE('',*,*,#53164,.T.) ;
#75792=ORIENTED_EDGE('',*,*,#50939,.F.) ;
#75793=ORIENTED_EDGE('',*,*,#53165,.T.) ;
#75794=ORIENTED_EDGE('',*,*,#51058,.F.) ;
#75795=ORIENTED_EDGE('',*,*,#53166,.F.) ;
#75796=ORIENTED_EDGE('',*,*,#49396,.F.) ;
#75797=ORIENTED_EDGE('',*,*,#53167,.F.) ;
#75798=ORIENTED_EDGE('',*,*,#51569,.F.) ;
#75799=ORIENTED_EDGE('',*,*,#53167,.T.) ;
#75800=ORIENTED_EDGE('',*,*,#49395,.T.) ;
#75801=ORIENTED_EDGE('',*,*,#53168,.F.) ;
#75802=ORIENTED_EDGE('',*,*,#53169,.F.) ;
#75803=ORIENTED_EDGE('',*,*,#49397,.T.) ;
#75804=ORIENTED_EDGE('',*,*,#53166,.T.) ;
#75805=ORIENTED_EDGE('',*,*,#53170,.F.) ;
#75806=ORIENTED_EDGE('',*,*,#53171,.F.) ;
#75807=ORIENTED_EDGE('',*,*,#53168,.T.) ;
#75808=ORIENTED_EDGE('',*,*,#49394,.F.) ;
#75809=ORIENTED_EDGE('',*,*,#53172,.F.) ;
#75810=ORIENTED_EDGE('',*,*,#51566,.F.) ;
#75811=ORIENTED_EDGE('',*,*,#53169,.T.) ;
#75812=ORIENTED_EDGE('',*,*,#51565,.F.) ;
#75813=ORIENTED_EDGE('',*,*,#53173,.F.) ;
#75814=ORIENTED_EDGE('',*,*,#51570,.F.) ;
#75815=ORIENTED_EDGE('',*,*,#53174,.F.) ;
#75816=ORIENTED_EDGE('',*,*,#51567,.F.) ;
#75817=ORIENTED_EDGE('',*,*,#53175,.F.) ;
#75818=ORIENTED_EDGE('',*,*,#51734,.F.) ;
#75819=ORIENTED_EDGE('',*,*,#53170,.T.) ;
#75820=ORIENTED_EDGE('',*,*,#51568,.F.) ;
#75821=ORIENTED_EDGE('',*,*,#53176,.F.) ;
#75822=ORIENTED_EDGE('',*,*,#51558,.F.) ;
#75823=ORIENTED_EDGE('',*,*,#53171,.T.) ;
#75824=ORIENTED_EDGE('',*,*,#51557,.F.) ;
#75825=ORIENTED_EDGE('',*,*,#53177,.F.) ;
#75826=ORIENTED_EDGE('',*,*,#49398,.F.) ;
#75827=ORIENTED_EDGE('',*,*,#53178,.F.) ;
#75828=ORIENTED_EDGE('',*,*,#49392,.F.) ;
#75829=ORIENTED_EDGE('',*,*,#53179,.F.) ;
#75830=ORIENTED_EDGE('',*,*,#51559,.F.) ;
#75831=ORIENTED_EDGE('',*,*,#49393,.T.) ;
#75832=ORIENTED_EDGE('',*,*,#53178,.T.) ;
#75833=ORIENTED_EDGE('',*,*,#53180,.F.) ;
#75834=ORIENTED_EDGE('',*,*,#53172,.T.) ;
#75835=ORIENTED_EDGE('',*,*,#53175,.T.) ;
#75836=ORIENTED_EDGE('',*,*,#53173,.T.) ;
#75837=ORIENTED_EDGE('',*,*,#53181,.F.) ;
#75838=ORIENTED_EDGE('',*,*,#53176,.T.) ;
#75839=ORIENTED_EDGE('',*,*,#53174,.T.) ;
#75840=ORIENTED_EDGE('',*,*,#53182,.F.) ;
#75841=ORIENTED_EDGE('',*,*,#49391,.T.) ;
#75842=ORIENTED_EDGE('',*,*,#53177,.T.) ;
#75843=ORIENTED_EDGE('',*,*,#53183,.F.) ;
#75844=ORIENTED_EDGE('',*,*,#53179,.T.) ;
#75845=ORIENTED_EDGE('',*,*,#53180,.T.) ;
#75846=ORIENTED_EDGE('',*,*,#51562,.F.) ;
#75847=ORIENTED_EDGE('',*,*,#53184,.F.) ;
#75848=ORIENTED_EDGE('',*,*,#51563,.F.) ;
#75849=ORIENTED_EDGE('',*,*,#53181,.T.) ;
#75850=ORIENTED_EDGE('',*,*,#51564,.F.) ;
#75851=ORIENTED_EDGE('',*,*,#53185,.F.) ;
#75852=ORIENTED_EDGE('',*,*,#51731,.F.) ;
#75853=ORIENTED_EDGE('',*,*,#53182,.T.) ;
#75854=ORIENTED_EDGE('',*,*,#51733,.F.) ;
#75855=ORIENTED_EDGE('',*,*,#53186,.F.) ;
#75856=ORIENTED_EDGE('',*,*,#51555,.F.) ;
#75857=ORIENTED_EDGE('',*,*,#53183,.T.) ;
#75858=ORIENTED_EDGE('',*,*,#51556,.F.) ;
#75859=ORIENTED_EDGE('',*,*,#53187,.F.) ;
#75860=ORIENTED_EDGE('',*,*,#51560,.F.) ;
#75861=ORIENTED_EDGE('',*,*,#53185,.T.) ;
#75862=ORIENTED_EDGE('',*,*,#53184,.T.) ;
#75863=ORIENTED_EDGE('',*,*,#53188,.F.) ;
#75864=ORIENTED_EDGE('',*,*,#53187,.T.) ;
#75865=ORIENTED_EDGE('',*,*,#53186,.T.) ;
#75866=ORIENTED_EDGE('',*,*,#53189,.F.) ;
#75867=ORIENTED_EDGE('',*,*,#53188,.T.) ;
#75868=ORIENTED_EDGE('',*,*,#51561,.F.) ;
#75869=ORIENTED_EDGE('',*,*,#53189,.T.) ;
#75870=ORIENTED_EDGE('',*,*,#51732,.F.) ;
#75871=ORIENTED_EDGE('',*,*,#51740,.F.) ;
#75872=ORIENTED_EDGE('',*,*,#51753,.F.) ;
#75873=ORIENTED_EDGE('',*,*,#53190,.F.) ;
#75874=ORIENTED_EDGE('',*,*,#51745,.F.) ;
#75875=ORIENTED_EDGE('',*,*,#53191,.F.) ;
#75876=ORIENTED_EDGE('',*,*,#51743,.F.) ;
#75877=ORIENTED_EDGE('',*,*,#53192,.F.) ;
#75878=ORIENTED_EDGE('',*,*,#51870,.F.) ;
#75879=ORIENTED_EDGE('',*,*,#51742,.F.) ;
#75880=ORIENTED_EDGE('',*,*,#51744,.F.) ;
#75881=ORIENTED_EDGE('',*,*,#53193,.F.) ;
#75882=ORIENTED_EDGE('',*,*,#51748,.F.) ;
#75883=ORIENTED_EDGE('',*,*,#53192,.T.) ;
#75884=ORIENTED_EDGE('',*,*,#53190,.T.) ;
#75885=ORIENTED_EDGE('',*,*,#53194,.F.) ;
#75886=ORIENTED_EDGE('',*,*,#53193,.T.) ;
#75887=ORIENTED_EDGE('',*,*,#53191,.T.) ;
#75888=ORIENTED_EDGE('',*,*,#53195,.F.) ;
#75889=ORIENTED_EDGE('',*,*,#51738,.F.) ;
#75890=ORIENTED_EDGE('',*,*,#51751,.F.) ;
#75891=ORIENTED_EDGE('',*,*,#53196,.F.) ;
#75892=ORIENTED_EDGE('',*,*,#51754,.F.) ;
#75893=ORIENTED_EDGE('',*,*,#53194,.T.) ;
#75894=ORIENTED_EDGE('',*,*,#51752,.F.) ;
#75895=ORIENTED_EDGE('',*,*,#53197,.F.) ;
#75896=ORIENTED_EDGE('',*,*,#51867,.F.) ;
#75897=ORIENTED_EDGE('',*,*,#53195,.T.) ;
#75898=ORIENTED_EDGE('',*,*,#51869,.F.) ;
#75899=ORIENTED_EDGE('',*,*,#53198,.F.) ;
#75900=ORIENTED_EDGE('',*,*,#51746,.F.) ;
#75901=ORIENTED_EDGE('',*,*,#51736,.F.) ;
#75902=ORIENTED_EDGE('',*,*,#51747,.F.) ;
#75903=ORIENTED_EDGE('',*,*,#53199,.F.) ;
#75904=ORIENTED_EDGE('',*,*,#51749,.F.) ;
#75905=ORIENTED_EDGE('',*,*,#53197,.T.) ;
#75906=ORIENTED_EDGE('',*,*,#53196,.T.) ;
#75907=ORIENTED_EDGE('',*,*,#53200,.F.) ;
#75908=ORIENTED_EDGE('',*,*,#53199,.T.) ;
#75909=ORIENTED_EDGE('',*,*,#53198,.T.) ;
#75910=ORIENTED_EDGE('',*,*,#53201,.F.) ;
#75911=ORIENTED_EDGE('',*,*,#53200,.T.) ;
#75912=ORIENTED_EDGE('',*,*,#51750,.F.) ;
#75913=ORIENTED_EDGE('',*,*,#53201,.T.) ;
#75914=ORIENTED_EDGE('',*,*,#51868,.F.) ;
#75915=ORIENTED_EDGE('',*,*,#53202,.F.) ;
#75916=ORIENTED_EDGE('',*,*,#52074,.F.) ;
#75917=ORIENTED_EDGE('',*,*,#53203,.F.) ;
#75918=ORIENTED_EDGE('',*,*,#52089,.F.) ;
#75919=ORIENTED_EDGE('',*,*,#53203,.T.) ;
#75920=ORIENTED_EDGE('',*,*,#52077,.F.) ;
#75921=ORIENTED_EDGE('',*,*,#53204,.F.) ;
#75922=ORIENTED_EDGE('',*,*,#52071,.F.) ;
#75923=ORIENTED_EDGE('',*,*,#53202,.T.) ;
#75924=ORIENTED_EDGE('',*,*,#53205,.F.) ;
#75925=ORIENTED_EDGE('',*,*,#53204,.T.) ;
#75926=ORIENTED_EDGE('',*,*,#52080,.F.) ;
#75927=ORIENTED_EDGE('',*,*,#53206,.F.) ;
#75928=ORIENTED_EDGE('',*,*,#52086,.F.) ;
#75929=ORIENTED_EDGE('',*,*,#53205,.T.) ;
#75930=ORIENTED_EDGE('',*,*,#52088,.F.) ;
#75931=ORIENTED_EDGE('',*,*,#53207,.F.) ;
#75932=ORIENTED_EDGE('',*,*,#52068,.F.) ;
#75933=ORIENTED_EDGE('',*,*,#53206,.T.) ;
#75934=ORIENTED_EDGE('',*,*,#52083,.F.) ;
#75935=ORIENTED_EDGE('',*,*,#53208,.F.) ;
#75936=ORIENTED_EDGE('',*,*,#52065,.F.) ;
#75937=ORIENTED_EDGE('',*,*,#53207,.T.) ;
#75938=ORIENTED_EDGE('',*,*,#53209,.F.) ;
#75939=ORIENTED_EDGE('',*,*,#53208,.T.) ;
#75940=ORIENTED_EDGE('',*,*,#52084,.F.) ;
#75941=ORIENTED_EDGE('',*,*,#53209,.T.) ;
#75942=ORIENTED_EDGE('',*,*,#52087,.F.) ;
#75943=ORIENTED_EDGE('',*,*,#49160,.F.) ;
#75944=ORIENTED_EDGE('',*,*,#51891,.F.) ;
#75945=ORIENTED_EDGE('',*,*,#49174,.F.) ;
#75946=ORIENTED_EDGE('',*,*,#51920,.F.) ;
#75947=ORIENTED_EDGE('',*,*,#49162,.F.) ;
#75948=ORIENTED_EDGE('',*,*,#51921,.F.) ;
#75949=ORIENTED_EDGE('',*,*,#49172,.F.) ;
#75950=ORIENTED_EDGE('',*,*,#51924,.F.) ;
#75951=ORIENTED_EDGE('',*,*,#49170,.F.) ;
#75952=ORIENTED_EDGE('',*,*,#51922,.F.) ;
#75953=ORIENTED_EDGE('',*,*,#49164,.F.) ;
#75954=ORIENTED_EDGE('',*,*,#51925,.F.) ;
#75955=ORIENTED_EDGE('',*,*,#49168,.F.) ;
#75956=ORIENTED_EDGE('',*,*,#49527,.F.) ;
#75957=ORIENTED_EDGE('',*,*,#49166,.F.) ;
#75958=ORIENTED_EDGE('',*,*,#51923,.F.) ;
#75959=ORIENTED_EDGE('',*,*,#53210,.F.) ;
#75960=ORIENTED_EDGE('',*,*,#53211,.F.) ;
#75961=ORIENTED_EDGE('',*,*,#53212,.F.) ;
#75962=ORIENTED_EDGE('',*,*,#53211,.T.) ;
#75963=ORIENTED_EDGE('',*,*,#51431,.F.) ;
#75964=ORIENTED_EDGE('',*,*,#53213,.F.) ;
#75965=ORIENTED_EDGE('',*,*,#51426,.F.) ;
#75966=ORIENTED_EDGE('',*,*,#53212,.T.) ;
#75967=ORIENTED_EDGE('',*,*,#51425,.F.) ;
#75968=ORIENTED_EDGE('',*,*,#53214,.F.) ;
#75969=ORIENTED_EDGE('',*,*,#51427,.F.) ;
#75970=ORIENTED_EDGE('',*,*,#53210,.T.) ;
#75971=ORIENTED_EDGE('',*,*,#51430,.F.) ;
#75972=ORIENTED_EDGE('',*,*,#53215,.F.) ;
#75973=ORIENTED_EDGE('',*,*,#51432,.F.) ;
#75974=ORIENTED_EDGE('',*,*,#51436,.F.) ;
#75975=ORIENTED_EDGE('',*,*,#53216,.T.) ;
#75976=ORIENTED_EDGE('',*,*,#51225,.F.) ;
#75977=ORIENTED_EDGE('',*,*,#53217,.F.) ;
#75978=ORIENTED_EDGE('',*,*,#53213,.T.) ;
#75979=ORIENTED_EDGE('',*,*,#53217,.T.) ;
#75980=ORIENTED_EDGE('',*,*,#53218,.F.) ;
#75981=ORIENTED_EDGE('',*,*,#53219,.F.) ;
#75982=ORIENTED_EDGE('',*,*,#53214,.T.) ;
#75983=ORIENTED_EDGE('',*,*,#53220,.F.) ;
#75984=ORIENTED_EDGE('',*,*,#49620,.T.) ;
#75985=ORIENTED_EDGE('',*,*,#53221,.F.) ;
#75986=ORIENTED_EDGE('',*,*,#53215,.T.) ;
#75987=ORIENTED_EDGE('',*,*,#53222,.F.) ;
#75988=ORIENTED_EDGE('',*,*,#51435,.F.) ;
#75989=ORIENTED_EDGE('',*,*,#53223,.T.) ;
#75990=ORIENTED_EDGE('',*,*,#49451,.F.) ;
#75991=ORIENTED_EDGE('',*,*,#53224,.T.) ;
#75992=ORIENTED_EDGE('',*,*,#53218,.T.) ;
#75993=ORIENTED_EDGE('',*,*,#51224,.F.) ;
#75994=ORIENTED_EDGE('',*,*,#53225,.F.) ;
#75995=ORIENTED_EDGE('',*,*,#51423,.F.) ;
#75996=ORIENTED_EDGE('',*,*,#53220,.T.) ;
#75997=ORIENTED_EDGE('',*,*,#51424,.F.) ;
#75998=ORIENTED_EDGE('',*,*,#53226,.F.) ;
#75999=ORIENTED_EDGE('',*,*,#49621,.F.) ;
#76000=ORIENTED_EDGE('',*,*,#53219,.T.) ;
#76001=ORIENTED_EDGE('',*,*,#49627,.F.) ;
#76002=ORIENTED_EDGE('',*,*,#53227,.F.) ;
#76003=ORIENTED_EDGE('',*,*,#51428,.F.) ;
#76004=ORIENTED_EDGE('',*,*,#53222,.T.) ;
#76005=ORIENTED_EDGE('',*,*,#51429,.F.) ;
#76006=ORIENTED_EDGE('',*,*,#53228,.F.) ;
#76007=ORIENTED_EDGE('',*,*,#51419,.F.) ;
#76008=ORIENTED_EDGE('',*,*,#53221,.T.) ;
#76009=ORIENTED_EDGE('',*,*,#51422,.F.) ;
#76010=ORIENTED_EDGE('',*,*,#53229,.F.) ;
#76011=ORIENTED_EDGE('',*,*,#51433,.F.) ;
#76012=ORIENTED_EDGE('',*,*,#51235,.F.) ;
#76013=ORIENTED_EDGE('',*,*,#53230,.T.) ;
#76014=ORIENTED_EDGE('',*,*,#51434,.F.) ;
#76015=ORIENTED_EDGE('',*,*,#53231,.F.) ;
#76016=ORIENTED_EDGE('',*,*,#53225,.T.) ;
#76017=ORIENTED_EDGE('',*,*,#51223,.T.) ;
#76018=ORIENTED_EDGE('',*,*,#53232,.F.) ;
#76019=ORIENTED_EDGE('',*,*,#53226,.T.) ;
#76020=ORIENTED_EDGE('',*,*,#53227,.T.) ;
#76021=ORIENTED_EDGE('',*,*,#49626,.T.) ;
#76022=ORIENTED_EDGE('',*,*,#53233,.F.) ;
#76023=ORIENTED_EDGE('',*,*,#53228,.T.) ;
#76024=ORIENTED_EDGE('',*,*,#53231,.T.) ;
#76025=ORIENTED_EDGE('',*,*,#53229,.T.) ;
#76026=ORIENTED_EDGE('',*,*,#53234,.F.) ;
#76027=ORIENTED_EDGE('',*,*,#51219,.F.) ;
#76028=ORIENTED_EDGE('',*,*,#53235,.T.) ;
#76029=ORIENTED_EDGE('',*,*,#51213,.F.) ;
#76030=ORIENTED_EDGE('',*,*,#53236,.F.) ;
#76031=ORIENTED_EDGE('',*,*,#53232,.T.) ;
#76032=ORIENTED_EDGE('',*,*,#51222,.F.) ;
#76033=ORIENTED_EDGE('',*,*,#53237,.F.) ;
#76034=ORIENTED_EDGE('',*,*,#49622,.F.) ;
#76035=ORIENTED_EDGE('',*,*,#53233,.T.) ;
#76036=ORIENTED_EDGE('',*,*,#49625,.F.) ;
#76037=ORIENTED_EDGE('',*,*,#53238,.F.) ;
#76038=ORIENTED_EDGE('',*,*,#51420,.F.) ;
#76039=ORIENTED_EDGE('',*,*,#53234,.T.) ;
#76040=ORIENTED_EDGE('',*,*,#51421,.F.) ;
#76041=ORIENTED_EDGE('',*,*,#53239,.F.) ;
#76042=ORIENTED_EDGE('',*,*,#51236,.F.) ;
#76043=ORIENTED_EDGE('',*,*,#53236,.T.) ;
#76044=ORIENTED_EDGE('',*,*,#53106,.F.) ;
#76045=ORIENTED_EDGE('',*,*,#53240,.F.) ;
#76046=ORIENTED_EDGE('',*,*,#53241,.F.) ;
#76047=ORIENTED_EDGE('',*,*,#53237,.T.) ;
#76048=ORIENTED_EDGE('',*,*,#53242,.F.) ;
#76049=ORIENTED_EDGE('',*,*,#53239,.T.) ;
#76050=ORIENTED_EDGE('',*,*,#53238,.T.) ;
#76051=ORIENTED_EDGE('',*,*,#53243,.F.) ;
#76052=ORIENTED_EDGE('',*,*,#51237,.T.) ;
#76053=ORIENTED_EDGE('',*,*,#53240,.T.) ;
#76054=ORIENTED_EDGE('',*,*,#49697,.F.) ;
#76055=ORIENTED_EDGE('',*,*,#53244,.F.) ;
#76056=ORIENTED_EDGE('',*,*,#51220,.F.) ;
#76057=ORIENTED_EDGE('',*,*,#53242,.T.) ;
#76058=ORIENTED_EDGE('',*,*,#51221,.F.) ;
#76059=ORIENTED_EDGE('',*,*,#53245,.F.) ;
#76060=ORIENTED_EDGE('',*,*,#51227,.F.) ;
#76061=ORIENTED_EDGE('',*,*,#53241,.T.) ;
#76062=ORIENTED_EDGE('',*,*,#51230,.F.) ;
#76063=ORIENTED_EDGE('',*,*,#53246,.F.) ;
#76064=ORIENTED_EDGE('',*,*,#49623,.F.) ;
#76065=ORIENTED_EDGE('',*,*,#53243,.T.) ;
#76066=ORIENTED_EDGE('',*,*,#49624,.F.) ;
#76067=ORIENTED_EDGE('',*,*,#53247,.F.) ;
#76068=ORIENTED_EDGE('',*,*,#51238,.F.) ;
#76069=ORIENTED_EDGE('',*,*,#53244,.T.) ;
#76070=ORIENTED_EDGE('',*,*,#49696,.T.) ;
#76071=ORIENTED_EDGE('',*,*,#53248,.F.) ;
#76072=ORIENTED_EDGE('',*,*,#53245,.T.) ;
#76073=ORIENTED_EDGE('',*,*,#53247,.T.) ;
#76074=ORIENTED_EDGE('',*,*,#53246,.T.) ;
#76075=ORIENTED_EDGE('',*,*,#53249,.F.) ;
#76076=ORIENTED_EDGE('',*,*,#53248,.T.) ;
#76077=ORIENTED_EDGE('',*,*,#49695,.F.) ;
#76078=ORIENTED_EDGE('',*,*,#53250,.F.) ;
#76079=ORIENTED_EDGE('',*,*,#51228,.F.) ;
#76080=ORIENTED_EDGE('',*,*,#53249,.T.) ;
#76081=ORIENTED_EDGE('',*,*,#51229,.F.) ;
#76082=ORIENTED_EDGE('',*,*,#53251,.F.) ;
#76083=ORIENTED_EDGE('',*,*,#51239,.F.) ;
#76084=ORIENTED_EDGE('',*,*,#51243,.F.) ;
#76085=ORIENTED_EDGE('',*,*,#53252,.T.) ;
#76086=ORIENTED_EDGE('',*,*,#51231,.F.) ;
#76087=ORIENTED_EDGE('',*,*,#53253,.F.) ;
#76088=ORIENTED_EDGE('',*,*,#49692,.F.) ;
#76089=ORIENTED_EDGE('',*,*,#53254,.T.) ;
#76090=ORIENTED_EDGE('',*,*,#51244,.F.) ;
#76091=ORIENTED_EDGE('',*,*,#53255,.F.) ;
#76092=ORIENTED_EDGE('',*,*,#53250,.T.) ;
#76093=ORIENTED_EDGE('',*,*,#49694,.T.) ;
#76094=ORIENTED_EDGE('',*,*,#53256,.F.) ;
#76095=ORIENTED_EDGE('',*,*,#53251,.T.) ;
#76096=ORIENTED_EDGE('',*,*,#53255,.T.) ;
#76097=ORIENTED_EDGE('',*,*,#53253,.T.) ;
#76098=ORIENTED_EDGE('',*,*,#53257,.F.) ;
#76099=ORIENTED_EDGE('',*,*,#53256,.T.) ;
#76100=ORIENTED_EDGE('',*,*,#49693,.F.) ;
#76101=ORIENTED_EDGE('',*,*,#53257,.T.) ;
#76102=ORIENTED_EDGE('',*,*,#51240,.F.) ;
#76103=ORIENTED_EDGE('',*,*,#52310,.F.) ;
#76104=ORIENTED_EDGE('',*,*,#52321,.F.) ;
#76105=ORIENTED_EDGE('',*,*,#52320,.F.) ;
#76106=ORIENTED_EDGE('',*,*,#53258,.F.) ;
#76107=ORIENTED_EDGE('',*,*,#52311,.F.) ;
#76108=ORIENTED_EDGE('',*,*,#53258,.T.) ;
#76109=ORIENTED_EDGE('',*,*,#50744,.F.) ;
#76110=ORIENTED_EDGE('',*,*,#53259,.F.) ;
#76111=ORIENTED_EDGE('',*,*,#50730,.F.) ;
#76112=ORIENTED_EDGE('',*,*,#52318,.F.) ;
#76113=ORIENTED_EDGE('',*,*,#52317,.F.) ;
#76114=ORIENTED_EDGE('',*,*,#52316,.F.) ;
#76115=ORIENTED_EDGE('',*,*,#53260,.F.) ;
#76116=ORIENTED_EDGE('',*,*,#52319,.F.) ;
#76117=ORIENTED_EDGE('',*,*,#53261,.F.) ;
#76118=ORIENTED_EDGE('',*,*,#53259,.T.) ;
#76119=ORIENTED_EDGE('',*,*,#53262,.F.) ;
#76120=ORIENTED_EDGE('',*,*,#52308,.F.) ;
#76121=ORIENTED_EDGE('',*,*,#52313,.F.) ;
#76122=ORIENTED_EDGE('',*,*,#52312,.F.) ;
#76123=ORIENTED_EDGE('',*,*,#53263,.F.) ;
#76124=ORIENTED_EDGE('',*,*,#52309,.F.) ;
#76125=ORIENTED_EDGE('',*,*,#53260,.T.) ;
#76126=ORIENTED_EDGE('',*,*,#50740,.F.) ;
#76127=ORIENTED_EDGE('',*,*,#53264,.F.) ;
#76128=ORIENTED_EDGE('',*,*,#50742,.F.) ;
#76129=ORIENTED_EDGE('',*,*,#53262,.T.) ;
#76130=ORIENTED_EDGE('',*,*,#50743,.F.) ;
#76131=ORIENTED_EDGE('',*,*,#53265,.F.) ;
#76132=ORIENTED_EDGE('',*,*,#50948,.F.) ;
#76133=ORIENTED_EDGE('',*,*,#53261,.T.) ;
#76134=ORIENTED_EDGE('',*,*,#50947,.F.) ;
#76135=ORIENTED_EDGE('',*,*,#53266,.F.) ;
#76136=ORIENTED_EDGE('',*,*,#50731,.F.) ;
#76137=ORIENTED_EDGE('',*,*,#53263,.T.) ;
#76138=ORIENTED_EDGE('',*,*,#50732,.F.) ;
#76139=ORIENTED_EDGE('',*,*,#53267,.F.) ;
#76140=ORIENTED_EDGE('',*,*,#50736,.F.) ;
#76141=ORIENTED_EDGE('',*,*,#53265,.T.) ;
#76142=ORIENTED_EDGE('',*,*,#53264,.T.) ;
#76143=ORIENTED_EDGE('',*,*,#53268,.F.) ;
#76144=ORIENTED_EDGE('',*,*,#53267,.T.) ;
#76145=ORIENTED_EDGE('',*,*,#53266,.T.) ;
#76146=ORIENTED_EDGE('',*,*,#53269,.F.) ;
#76147=ORIENTED_EDGE('',*,*,#53268,.T.) ;
#76148=ORIENTED_EDGE('',*,*,#50739,.F.) ;
#76149=ORIENTED_EDGE('',*,*,#53270,.F.) ;
#76150=ORIENTED_EDGE('',*,*,#50945,.F.) ;
#76151=ORIENTED_EDGE('',*,*,#53269,.T.) ;
#76152=ORIENTED_EDGE('',*,*,#50946,.F.) ;
#76153=ORIENTED_EDGE('',*,*,#53271,.F.) ;
#76154=ORIENTED_EDGE('',*,*,#50733,.F.) ;
#76155=ORIENTED_EDGE('',*,*,#53271,.T.) ;
#76156=ORIENTED_EDGE('',*,*,#53270,.T.) ;
#76157=ORIENTED_EDGE('',*,*,#53272,.F.) ;
#76158=ORIENTED_EDGE('',*,*,#53272,.T.) ;
#76159=ORIENTED_EDGE('',*,*,#50738,.F.) ;
#76160=ORIENTED_EDGE('',*,*,#53273,.F.) ;
#76161=ORIENTED_EDGE('',*,*,#50734,.F.) ;
#76162=ORIENTED_EDGE('',*,*,#52314,.F.) ;
#76163=ORIENTED_EDGE('',*,*,#52307,.F.) ;
#76164=ORIENTED_EDGE('',*,*,#52306,.F.) ;
#76165=ORIENTED_EDGE('',*,*,#53273,.T.) ;
#76166=ORIENTED_EDGE('',*,*,#52315,.F.) ;
#76167=ORIENTED_EDGE('',*,*,#52515,.F.) ;
#76168=ORIENTED_EDGE('',*,*,#52514,.F.) ;
#76169=ORIENTED_EDGE('',*,*,#52513,.F.) ;
#76170=ORIENTED_EDGE('',*,*,#53274,.F.) ;
#76171=ORIENTED_EDGE('',*,*,#52516,.F.) ;
#76172=ORIENTED_EDGE('',*,*,#53274,.T.) ;
#76173=ORIENTED_EDGE('',*,*,#52512,.F.) ;
#76174=ORIENTED_EDGE('',*,*,#53275,.F.) ;
#76175=ORIENTED_EDGE('',*,*,#50593,.F.) ;
#76176=ORIENTED_EDGE('',*,*,#53275,.T.) ;
#76177=ORIENTED_EDGE('',*,*,#50448,.F.) ;
#76178=ORIENTED_EDGE('',*,*,#53276,.F.) ;
#76179=ORIENTED_EDGE('',*,*,#50594,.F.) ;
#76180=ORIENTED_EDGE('',*,*,#50436,.F.) ;
#76181=ORIENTED_EDGE('',*,*,#50595,.F.) ;
#76182=ORIENTED_EDGE('',*,*,#53277,.F.) ;
#76183=ORIENTED_EDGE('',*,*,#50442,.F.) ;
#76184=ORIENTED_EDGE('',*,*,#53277,.T.) ;
#76185=ORIENTED_EDGE('',*,*,#53276,.T.) ;
#76186=ORIENTED_EDGE('',*,*,#53278,.F.) ;
#76187=ORIENTED_EDGE('',*,*,#53278,.T.) ;
#76188=ORIENTED_EDGE('',*,*,#50447,.F.) ;
#76189=ORIENTED_EDGE('',*,*,#53279,.F.) ;
#76190=ORIENTED_EDGE('',*,*,#50443,.F.) ;
#76191=ORIENTED_EDGE('',*,*,#50438,.F.) ;
#76192=ORIENTED_EDGE('',*,*,#50444,.F.) ;
#76193=ORIENTED_EDGE('',*,*,#53280,.F.) ;
#76194=ORIENTED_EDGE('',*,*,#50657,.F.) ;
#76195=ORIENTED_EDGE('',*,*,#53280,.T.) ;
#76196=ORIENTED_EDGE('',*,*,#53279,.T.) ;
#76197=ORIENTED_EDGE('',*,*,#53281,.F.) ;
#76198=ORIENTED_EDGE('',*,*,#53281,.T.) ;
#76199=ORIENTED_EDGE('',*,*,#50446,.F.) ;
#76200=ORIENTED_EDGE('',*,*,#53282,.F.) ;
#76201=ORIENTED_EDGE('',*,*,#50658,.F.) ;
#76202=ORIENTED_EDGE('',*,*,#53282,.T.) ;
#76203=ORIENTED_EDGE('',*,*,#52511,.F.) ;
#76204=ORIENTED_EDGE('',*,*,#53283,.F.) ;
#76205=ORIENTED_EDGE('',*,*,#50659,.F.) ;
#76206=ORIENTED_EDGE('',*,*,#53283,.T.) ;
#76207=ORIENTED_EDGE('',*,*,#52510,.F.) ;
#76208=ORIENTED_EDGE('',*,*,#52519,.F.) ;
#76209=ORIENTED_EDGE('',*,*,#52520,.F.) ;
#76210=ORIENTED_EDGE('',*,*,#52525,.F.) ;
#76211=ORIENTED_EDGE('',*,*,#53284,.F.) ;
#76212=ORIENTED_EDGE('',*,*,#53284,.T.) ;
#76213=ORIENTED_EDGE('',*,*,#52524,.F.) ;
#76214=ORIENTED_EDGE('',*,*,#53285,.F.) ;
#76215=ORIENTED_EDGE('',*,*,#50654,.F.) ;
#76216=ORIENTED_EDGE('',*,*,#53285,.T.) ;
#76217=ORIENTED_EDGE('',*,*,#50430,.F.) ;
#76218=ORIENTED_EDGE('',*,*,#53286,.F.) ;
#76219=ORIENTED_EDGE('',*,*,#50655,.F.) ;
#76220=ORIENTED_EDGE('',*,*,#50440,.F.) ;
#76221=ORIENTED_EDGE('',*,*,#50656,.F.) ;
#76222=ORIENTED_EDGE('',*,*,#53287,.F.) ;
#76223=ORIENTED_EDGE('',*,*,#50434,.F.) ;
#76224=ORIENTED_EDGE('',*,*,#53287,.T.) ;
#76225=ORIENTED_EDGE('',*,*,#53286,.T.) ;
#76226=ORIENTED_EDGE('',*,*,#53288,.F.) ;
#76227=ORIENTED_EDGE('',*,*,#53288,.T.) ;
#76228=ORIENTED_EDGE('',*,*,#50429,.F.) ;
#76229=ORIENTED_EDGE('',*,*,#53289,.F.) ;
#76230=ORIENTED_EDGE('',*,*,#50431,.F.) ;
#76231=ORIENTED_EDGE('',*,*,#50441,.F.) ;
#76232=ORIENTED_EDGE('',*,*,#50432,.F.) ;
#76233=ORIENTED_EDGE('',*,*,#53290,.F.) ;
#76234=ORIENTED_EDGE('',*,*,#50596,.F.) ;
#76235=ORIENTED_EDGE('',*,*,#53290,.T.) ;
#76236=ORIENTED_EDGE('',*,*,#53289,.T.) ;
#76237=ORIENTED_EDGE('',*,*,#53291,.F.) ;
#76238=ORIENTED_EDGE('',*,*,#53291,.T.) ;
#76239=ORIENTED_EDGE('',*,*,#50428,.F.) ;
#76240=ORIENTED_EDGE('',*,*,#53292,.F.) ;
#76241=ORIENTED_EDGE('',*,*,#50597,.F.) ;
#76242=ORIENTED_EDGE('',*,*,#53292,.T.) ;
#76243=ORIENTED_EDGE('',*,*,#52523,.F.) ;
#76244=ORIENTED_EDGE('',*,*,#53293,.F.) ;
#76245=ORIENTED_EDGE('',*,*,#50598,.F.) ;
#76246=ORIENTED_EDGE('',*,*,#52521,.F.) ;
#76247=ORIENTED_EDGE('',*,*,#52518,.F.) ;
#76248=ORIENTED_EDGE('',*,*,#52517,.F.) ;
#76249=ORIENTED_EDGE('',*,*,#53293,.T.) ;
#76250=ORIENTED_EDGE('',*,*,#52522,.F.) ;
#76251=ORIENTED_EDGE('',*,*,#53294,.F.) ;
#76252=ORIENTED_EDGE('',*,*,#49460,.F.) ;
#76253=ORIENTED_EDGE('',*,*,#53295,.F.) ;
#76254=ORIENTED_EDGE('',*,*,#52097,.F.) ;
#76255=ORIENTED_EDGE('',*,*,#53295,.T.) ;
#76256=ORIENTED_EDGE('',*,*,#49459,.F.) ;
#76257=ORIENTED_EDGE('',*,*,#53296,.F.) ;
#76258=ORIENTED_EDGE('',*,*,#52100,.F.) ;
#76259=ORIENTED_EDGE('',*,*,#53294,.T.) ;
#76260=ORIENTED_EDGE('',*,*,#52094,.F.) ;
#76261=ORIENTED_EDGE('',*,*,#53297,.F.) ;
#76262=ORIENTED_EDGE('',*,*,#49461,.F.) ;
#76263=ORIENTED_EDGE('',*,*,#53296,.T.) ;
#76264=ORIENTED_EDGE('',*,*,#49458,.F.) ;
#76265=ORIENTED_EDGE('',*,*,#53298,.F.) ;
#76266=ORIENTED_EDGE('',*,*,#52103,.F.) ;
#76267=ORIENTED_EDGE('',*,*,#53297,.T.) ;
#76268=ORIENTED_EDGE('',*,*,#52091,.F.) ;
#76269=ORIENTED_EDGE('',*,*,#53299,.F.) ;
#76270=ORIENTED_EDGE('',*,*,#49462,.F.) ;
#76271=ORIENTED_EDGE('',*,*,#53298,.T.) ;
#76272=ORIENTED_EDGE('',*,*,#49457,.F.) ;
#76273=ORIENTED_EDGE('',*,*,#53300,.F.) ;
#76274=ORIENTED_EDGE('',*,*,#52106,.F.) ;
#76275=ORIENTED_EDGE('',*,*,#53299,.T.) ;
#76276=ORIENTED_EDGE('',*,*,#52113,.F.) ;
#76277=ORIENTED_EDGE('',*,*,#53301,.F.) ;
#76278=ORIENTED_EDGE('',*,*,#49455,.F.) ;
#76279=ORIENTED_EDGE('',*,*,#53300,.T.) ;
#76280=ORIENTED_EDGE('',*,*,#49456,.F.) ;
#76281=ORIENTED_EDGE('',*,*,#53301,.T.) ;
#76282=ORIENTED_EDGE('',*,*,#52109,.F.) ;
#76283=ORIENTED_EDGE('',*,*,#50954,.F.) ;
#76284=ORIENTED_EDGE('',*,*,#50968,.F.) ;
#76285=ORIENTED_EDGE('',*,*,#53302,.F.) ;
#76286=ORIENTED_EDGE('',*,*,#50957,.F.) ;
#76287=ORIENTED_EDGE('',*,*,#53303,.F.) ;
#76288=ORIENTED_EDGE('',*,*,#50958,.F.) ;
#76289=ORIENTED_EDGE('',*,*,#53304,.F.) ;
#76290=ORIENTED_EDGE('',*,*,#51064,.F.) ;
#76291=ORIENTED_EDGE('',*,*,#50956,.F.) ;
#76292=ORIENTED_EDGE('',*,*,#50959,.F.) ;
#76293=ORIENTED_EDGE('',*,*,#53305,.F.) ;
#76294=ORIENTED_EDGE('',*,*,#50960,.F.) ;
#76295=ORIENTED_EDGE('',*,*,#53304,.T.) ;
#76296=ORIENTED_EDGE('',*,*,#53302,.T.) ;
#76297=ORIENTED_EDGE('',*,*,#53306,.F.) ;
#76298=ORIENTED_EDGE('',*,*,#53305,.T.) ;
#76299=ORIENTED_EDGE('',*,*,#53303,.T.) ;
#76300=ORIENTED_EDGE('',*,*,#53307,.F.) ;
#76301=ORIENTED_EDGE('',*,*,#50952,.F.) ;
#76302=ORIENTED_EDGE('',*,*,#50964,.F.) ;
#76303=ORIENTED_EDGE('',*,*,#53308,.F.) ;
#76304=ORIENTED_EDGE('',*,*,#50966,.F.) ;
#76305=ORIENTED_EDGE('',*,*,#53306,.T.) ;
#76306=ORIENTED_EDGE('',*,*,#50967,.F.) ;
#76307=ORIENTED_EDGE('',*,*,#53309,.F.) ;
#76308=ORIENTED_EDGE('',*,*,#51061,.F.) ;
#76309=ORIENTED_EDGE('',*,*,#53307,.T.) ;
#76310=ORIENTED_EDGE('',*,*,#51063,.F.) ;
#76311=ORIENTED_EDGE('',*,*,#53310,.F.) ;
#76312=ORIENTED_EDGE('',*,*,#50961,.F.) ;
#76313=ORIENTED_EDGE('',*,*,#50950,.F.) ;
#76314=ORIENTED_EDGE('',*,*,#50962,.F.) ;
#76315=ORIENTED_EDGE('',*,*,#53311,.F.) ;
#76316=ORIENTED_EDGE('',*,*,#50965,.F.) ;
#76317=ORIENTED_EDGE('',*,*,#53309,.T.) ;
#76318=ORIENTED_EDGE('',*,*,#53308,.T.) ;
#76319=ORIENTED_EDGE('',*,*,#53312,.F.) ;
#76320=ORIENTED_EDGE('',*,*,#53311,.T.) ;
#76321=ORIENTED_EDGE('',*,*,#53310,.T.) ;
#76322=ORIENTED_EDGE('',*,*,#53313,.F.) ;
#76323=ORIENTED_EDGE('',*,*,#53312,.T.) ;
#76324=ORIENTED_EDGE('',*,*,#50963,.F.) ;
#76325=ORIENTED_EDGE('',*,*,#53313,.T.) ;
#76326=ORIENTED_EDGE('',*,*,#51062,.F.) ;
#76327=ORIENTED_EDGE('',*,*,#53314,.F.) ;
#76328=ORIENTED_EDGE('',*,*,#49348,.F.) ;
#76329=ORIENTED_EDGE('',*,*,#53315,.F.) ;
#76330=ORIENTED_EDGE('',*,*,#51553,.F.) ;
#76331=ORIENTED_EDGE('',*,*,#53315,.T.) ;
#76332=ORIENTED_EDGE('',*,*,#49347,.T.) ;
#76333=ORIENTED_EDGE('',*,*,#53316,.F.) ;
#76334=ORIENTED_EDGE('',*,*,#53317,.F.) ;
#76335=ORIENTED_EDGE('',*,*,#49349,.T.) ;
#76336=ORIENTED_EDGE('',*,*,#53314,.T.) ;
#76337=ORIENTED_EDGE('',*,*,#53318,.F.) ;
#76338=ORIENTED_EDGE('',*,*,#53319,.F.) ;
#76339=ORIENTED_EDGE('',*,*,#53316,.T.) ;
#76340=ORIENTED_EDGE('',*,*,#49346,.F.) ;
#76341=ORIENTED_EDGE('',*,*,#53320,.F.) ;
#76342=ORIENTED_EDGE('',*,*,#51550,.F.) ;
#76343=ORIENTED_EDGE('',*,*,#53317,.T.) ;
#76344=ORIENTED_EDGE('',*,*,#51549,.F.) ;
#76345=ORIENTED_EDGE('',*,*,#53321,.F.) ;
#76346=ORIENTED_EDGE('',*,*,#51554,.F.) ;
#76347=ORIENTED_EDGE('',*,*,#53322,.F.) ;
#76348=ORIENTED_EDGE('',*,*,#51551,.F.) ;
#76349=ORIENTED_EDGE('',*,*,#53323,.F.) ;
#76350=ORIENTED_EDGE('',*,*,#51758,.F.) ;
#76351=ORIENTED_EDGE('',*,*,#53318,.T.) ;
#76352=ORIENTED_EDGE('',*,*,#51552,.F.) ;
#76353=ORIENTED_EDGE('',*,*,#53324,.F.) ;
#76354=ORIENTED_EDGE('',*,*,#51542,.F.) ;
#76355=ORIENTED_EDGE('',*,*,#53319,.T.) ;
#76356=ORIENTED_EDGE('',*,*,#51541,.F.) ;
#76357=ORIENTED_EDGE('',*,*,#53325,.F.) ;
#76358=ORIENTED_EDGE('',*,*,#49350,.F.) ;
#76359=ORIENTED_EDGE('',*,*,#53326,.F.) ;
#76360=ORIENTED_EDGE('',*,*,#49344,.F.) ;
#76361=ORIENTED_EDGE('',*,*,#53327,.F.) ;
#76362=ORIENTED_EDGE('',*,*,#51543,.F.) ;
#76363=ORIENTED_EDGE('',*,*,#49345,.T.) ;
#76364=ORIENTED_EDGE('',*,*,#53326,.T.) ;
#76365=ORIENTED_EDGE('',*,*,#53328,.F.) ;
#76366=ORIENTED_EDGE('',*,*,#53320,.T.) ;
#76367=ORIENTED_EDGE('',*,*,#53323,.T.) ;
#76368=ORIENTED_EDGE('',*,*,#53321,.T.) ;
#76369=ORIENTED_EDGE('',*,*,#53329,.F.) ;
#76370=ORIENTED_EDGE('',*,*,#53324,.T.) ;
#76371=ORIENTED_EDGE('',*,*,#53322,.T.) ;
#76372=ORIENTED_EDGE('',*,*,#53330,.F.) ;
#76373=ORIENTED_EDGE('',*,*,#49343,.T.) ;
#76374=ORIENTED_EDGE('',*,*,#53325,.T.) ;
#76375=ORIENTED_EDGE('',*,*,#53331,.F.) ;
#76376=ORIENTED_EDGE('',*,*,#53327,.T.) ;
#76377=ORIENTED_EDGE('',*,*,#53328,.T.) ;
#76378=ORIENTED_EDGE('',*,*,#51546,.F.) ;
#76379=ORIENTED_EDGE('',*,*,#53332,.F.) ;
#76380=ORIENTED_EDGE('',*,*,#51547,.F.) ;
#76381=ORIENTED_EDGE('',*,*,#53329,.T.) ;
#76382=ORIENTED_EDGE('',*,*,#51548,.F.) ;
#76383=ORIENTED_EDGE('',*,*,#53333,.F.) ;
#76384=ORIENTED_EDGE('',*,*,#51755,.F.) ;
#76385=ORIENTED_EDGE('',*,*,#53330,.T.) ;
#76386=ORIENTED_EDGE('',*,*,#51757,.F.) ;
#76387=ORIENTED_EDGE('',*,*,#53334,.F.) ;
#76388=ORIENTED_EDGE('',*,*,#51539,.F.) ;
#76389=ORIENTED_EDGE('',*,*,#53331,.T.) ;
#76390=ORIENTED_EDGE('',*,*,#51540,.F.) ;
#76391=ORIENTED_EDGE('',*,*,#53335,.F.) ;
#76392=ORIENTED_EDGE('',*,*,#51544,.F.) ;
#76393=ORIENTED_EDGE('',*,*,#53333,.T.) ;
#76394=ORIENTED_EDGE('',*,*,#53332,.T.) ;
#76395=ORIENTED_EDGE('',*,*,#53336,.F.) ;
#76396=ORIENTED_EDGE('',*,*,#53335,.T.) ;
#76397=ORIENTED_EDGE('',*,*,#53334,.T.) ;
#76398=ORIENTED_EDGE('',*,*,#53337,.F.) ;
#76399=ORIENTED_EDGE('',*,*,#53336,.T.) ;
#76400=ORIENTED_EDGE('',*,*,#51545,.F.) ;
#76401=ORIENTED_EDGE('',*,*,#53337,.T.) ;
#76402=ORIENTED_EDGE('',*,*,#51756,.F.) ;
#76403=ORIENTED_EDGE('',*,*,#51764,.F.) ;
#76404=ORIENTED_EDGE('',*,*,#51777,.F.) ;
#76405=ORIENTED_EDGE('',*,*,#53338,.F.) ;
#76406=ORIENTED_EDGE('',*,*,#51769,.F.) ;
#76407=ORIENTED_EDGE('',*,*,#53339,.F.) ;
#76408=ORIENTED_EDGE('',*,*,#51767,.F.) ;
#76409=ORIENTED_EDGE('',*,*,#53340,.F.) ;
#76410=ORIENTED_EDGE('',*,*,#51874,.F.) ;
#76411=ORIENTED_EDGE('',*,*,#51766,.F.) ;
#76412=ORIENTED_EDGE('',*,*,#51768,.F.) ;
#76413=ORIENTED_EDGE('',*,*,#53341,.F.) ;
#76414=ORIENTED_EDGE('',*,*,#51772,.F.) ;
#76415=ORIENTED_EDGE('',*,*,#53340,.T.) ;
#76416=ORIENTED_EDGE('',*,*,#53338,.T.) ;
#76417=ORIENTED_EDGE('',*,*,#53342,.F.) ;
#76418=ORIENTED_EDGE('',*,*,#53341,.T.) ;
#76419=ORIENTED_EDGE('',*,*,#53339,.T.) ;
#76420=ORIENTED_EDGE('',*,*,#53343,.F.) ;
#76421=ORIENTED_EDGE('',*,*,#51762,.F.) ;
#76422=ORIENTED_EDGE('',*,*,#51775,.F.) ;
#76423=ORIENTED_EDGE('',*,*,#53344,.F.) ;
#76424=ORIENTED_EDGE('',*,*,#51778,.F.) ;
#76425=ORIENTED_EDGE('',*,*,#53342,.T.) ;
#76426=ORIENTED_EDGE('',*,*,#51776,.F.) ;
#76427=ORIENTED_EDGE('',*,*,#53345,.F.) ;
#76428=ORIENTED_EDGE('',*,*,#51871,.F.) ;
#76429=ORIENTED_EDGE('',*,*,#53343,.T.) ;
#76430=ORIENTED_EDGE('',*,*,#51873,.F.) ;
#76431=ORIENTED_EDGE('',*,*,#53346,.F.) ;
#76432=ORIENTED_EDGE('',*,*,#51770,.F.) ;
#76433=ORIENTED_EDGE('',*,*,#51760,.F.) ;
#76434=ORIENTED_EDGE('',*,*,#51771,.F.) ;
#76435=ORIENTED_EDGE('',*,*,#53347,.F.) ;
#76436=ORIENTED_EDGE('',*,*,#51773,.F.) ;
#76437=ORIENTED_EDGE('',*,*,#53345,.T.) ;
#76438=ORIENTED_EDGE('',*,*,#53344,.T.) ;
#76439=ORIENTED_EDGE('',*,*,#53348,.F.) ;
#76440=ORIENTED_EDGE('',*,*,#53347,.T.) ;
#76441=ORIENTED_EDGE('',*,*,#53346,.T.) ;
#76442=ORIENTED_EDGE('',*,*,#53349,.F.) ;
#76443=ORIENTED_EDGE('',*,*,#53348,.T.) ;
#76444=ORIENTED_EDGE('',*,*,#51774,.F.) ;
#76445=ORIENTED_EDGE('',*,*,#53349,.T.) ;
#76446=ORIENTED_EDGE('',*,*,#51872,.F.) ;
#76447=ORIENTED_EDGE('',*,*,#53350,.F.) ;
#76448=ORIENTED_EDGE('',*,*,#52102,.F.) ;
#76449=ORIENTED_EDGE('',*,*,#53351,.F.) ;
#76450=ORIENTED_EDGE('',*,*,#52117,.F.) ;
#76451=ORIENTED_EDGE('',*,*,#53351,.T.) ;
#76452=ORIENTED_EDGE('',*,*,#52105,.F.) ;
#76453=ORIENTED_EDGE('',*,*,#53352,.F.) ;
#76454=ORIENTED_EDGE('',*,*,#52099,.F.) ;
#76455=ORIENTED_EDGE('',*,*,#53350,.T.) ;
#76456=ORIENTED_EDGE('',*,*,#53353,.F.) ;
#76457=ORIENTED_EDGE('',*,*,#53352,.T.) ;
#76458=ORIENTED_EDGE('',*,*,#52108,.F.) ;
#76459=ORIENTED_EDGE('',*,*,#53354,.F.) ;
#76460=ORIENTED_EDGE('',*,*,#52114,.F.) ;
#76461=ORIENTED_EDGE('',*,*,#53353,.T.) ;
#76462=ORIENTED_EDGE('',*,*,#52116,.F.) ;
#76463=ORIENTED_EDGE('',*,*,#53355,.F.) ;
#76464=ORIENTED_EDGE('',*,*,#52096,.F.) ;
#76465=ORIENTED_EDGE('',*,*,#53354,.T.) ;
#76466=ORIENTED_EDGE('',*,*,#52111,.F.) ;
#76467=ORIENTED_EDGE('',*,*,#53356,.F.) ;
#76468=ORIENTED_EDGE('',*,*,#52093,.F.) ;
#76469=ORIENTED_EDGE('',*,*,#53355,.T.) ;
#76470=ORIENTED_EDGE('',*,*,#53357,.F.) ;
#76471=ORIENTED_EDGE('',*,*,#53356,.T.) ;
#76472=ORIENTED_EDGE('',*,*,#52112,.F.) ;
#76473=ORIENTED_EDGE('',*,*,#53357,.T.) ;
#76474=ORIENTED_EDGE('',*,*,#52115,.F.) ;
#76475=ORIENTED_EDGE('',*,*,#49178,.F.) ;
#76476=ORIENTED_EDGE('',*,*,#51890,.F.) ;
#76477=ORIENTED_EDGE('',*,*,#49192,.F.) ;
#76478=ORIENTED_EDGE('',*,*,#51926,.F.) ;
#76479=ORIENTED_EDGE('',*,*,#49180,.F.) ;
#76480=ORIENTED_EDGE('',*,*,#51927,.F.) ;
#76481=ORIENTED_EDGE('',*,*,#49190,.F.) ;
#76482=ORIENTED_EDGE('',*,*,#51930,.F.) ;
#76483=ORIENTED_EDGE('',*,*,#49188,.F.) ;
#76484=ORIENTED_EDGE('',*,*,#51928,.F.) ;
#76485=ORIENTED_EDGE('',*,*,#49182,.F.) ;
#76486=ORIENTED_EDGE('',*,*,#51931,.F.) ;
#76487=ORIENTED_EDGE('',*,*,#49186,.F.) ;
#76488=ORIENTED_EDGE('',*,*,#49526,.F.) ;
#76489=ORIENTED_EDGE('',*,*,#49184,.F.) ;
#76490=ORIENTED_EDGE('',*,*,#51929,.F.) ;
#76491=ORIENTED_EDGE('',*,*,#53358,.F.) ;
#76492=ORIENTED_EDGE('',*,*,#53359,.F.) ;
#76493=ORIENTED_EDGE('',*,*,#53360,.F.) ;
#76494=ORIENTED_EDGE('',*,*,#53359,.T.) ;
#76495=ORIENTED_EDGE('',*,*,#51449,.F.) ;
#76496=ORIENTED_EDGE('',*,*,#53361,.F.) ;
#76497=ORIENTED_EDGE('',*,*,#51444,.F.) ;
#76498=ORIENTED_EDGE('',*,*,#53360,.T.) ;
#76499=ORIENTED_EDGE('',*,*,#51443,.F.) ;
#76500=ORIENTED_EDGE('',*,*,#53362,.F.) ;
#76501=ORIENTED_EDGE('',*,*,#51445,.F.) ;
#76502=ORIENTED_EDGE('',*,*,#53358,.T.) ;
#76503=ORIENTED_EDGE('',*,*,#51448,.F.) ;
#76504=ORIENTED_EDGE('',*,*,#53363,.F.) ;
#76505=ORIENTED_EDGE('',*,*,#51450,.F.) ;
#76506=ORIENTED_EDGE('',*,*,#51454,.F.) ;
#76507=ORIENTED_EDGE('',*,*,#53364,.T.) ;
#76508=ORIENTED_EDGE('',*,*,#51253,.F.) ;
#76509=ORIENTED_EDGE('',*,*,#53365,.F.) ;
#76510=ORIENTED_EDGE('',*,*,#53361,.T.) ;
#76511=ORIENTED_EDGE('',*,*,#53365,.T.) ;
#76512=ORIENTED_EDGE('',*,*,#53366,.F.) ;
#76513=ORIENTED_EDGE('',*,*,#53367,.F.) ;
#76514=ORIENTED_EDGE('',*,*,#53362,.T.) ;
#76515=ORIENTED_EDGE('',*,*,#53368,.F.) ;
#76516=ORIENTED_EDGE('',*,*,#49612,.T.) ;
#76517=ORIENTED_EDGE('',*,*,#53369,.F.) ;
#76518=ORIENTED_EDGE('',*,*,#53363,.T.) ;
#76519=ORIENTED_EDGE('',*,*,#53370,.F.) ;
#76520=ORIENTED_EDGE('',*,*,#51453,.F.) ;
#76521=ORIENTED_EDGE('',*,*,#53371,.T.) ;
#76522=ORIENTED_EDGE('',*,*,#49439,.F.) ;
#76523=ORIENTED_EDGE('',*,*,#53372,.T.) ;
#76524=ORIENTED_EDGE('',*,*,#53366,.T.) ;
#76525=ORIENTED_EDGE('',*,*,#51252,.F.) ;
#76526=ORIENTED_EDGE('',*,*,#53373,.F.) ;
#76527=ORIENTED_EDGE('',*,*,#51441,.F.) ;
#76528=ORIENTED_EDGE('',*,*,#53368,.T.) ;
#76529=ORIENTED_EDGE('',*,*,#51442,.F.) ;
#76530=ORIENTED_EDGE('',*,*,#53374,.F.) ;
#76531=ORIENTED_EDGE('',*,*,#49613,.F.) ;
#76532=ORIENTED_EDGE('',*,*,#53367,.T.) ;
#76533=ORIENTED_EDGE('',*,*,#49619,.F.) ;
#76534=ORIENTED_EDGE('',*,*,#53375,.F.) ;
#76535=ORIENTED_EDGE('',*,*,#51446,.F.) ;
#76536=ORIENTED_EDGE('',*,*,#53370,.T.) ;
#76537=ORIENTED_EDGE('',*,*,#51447,.F.) ;
#76538=ORIENTED_EDGE('',*,*,#53376,.F.) ;
#76539=ORIENTED_EDGE('',*,*,#51437,.F.) ;
#76540=ORIENTED_EDGE('',*,*,#53369,.T.) ;
#76541=ORIENTED_EDGE('',*,*,#51440,.F.) ;
#76542=ORIENTED_EDGE('',*,*,#53377,.F.) ;
#76543=ORIENTED_EDGE('',*,*,#51451,.F.) ;
#76544=ORIENTED_EDGE('',*,*,#51263,.F.) ;
#76545=ORIENTED_EDGE('',*,*,#53378,.T.) ;
#76546=ORIENTED_EDGE('',*,*,#51452,.F.) ;
#76547=ORIENTED_EDGE('',*,*,#53379,.F.) ;
#76548=ORIENTED_EDGE('',*,*,#53373,.T.) ;
#76549=ORIENTED_EDGE('',*,*,#51251,.T.) ;
#76550=ORIENTED_EDGE('',*,*,#53380,.F.) ;
#76551=ORIENTED_EDGE('',*,*,#53374,.T.) ;
#76552=ORIENTED_EDGE('',*,*,#53375,.T.) ;
#76553=ORIENTED_EDGE('',*,*,#49618,.T.) ;
#76554=ORIENTED_EDGE('',*,*,#53381,.F.) ;
#76555=ORIENTED_EDGE('',*,*,#53376,.T.) ;
#76556=ORIENTED_EDGE('',*,*,#53379,.T.) ;
#76557=ORIENTED_EDGE('',*,*,#53377,.T.) ;
#76558=ORIENTED_EDGE('',*,*,#53382,.F.) ;
#76559=ORIENTED_EDGE('',*,*,#51247,.F.) ;
#76560=ORIENTED_EDGE('',*,*,#53383,.T.) ;
#76561=ORIENTED_EDGE('',*,*,#51241,.F.) ;
#76562=ORIENTED_EDGE('',*,*,#53384,.F.) ;
#76563=ORIENTED_EDGE('',*,*,#53380,.T.) ;
#76564=ORIENTED_EDGE('',*,*,#51250,.F.) ;
#76565=ORIENTED_EDGE('',*,*,#53385,.F.) ;
#76566=ORIENTED_EDGE('',*,*,#49614,.F.) ;
#76567=ORIENTED_EDGE('',*,*,#53381,.T.) ;
#76568=ORIENTED_EDGE('',*,*,#49617,.F.) ;
#76569=ORIENTED_EDGE('',*,*,#53386,.F.) ;
#76570=ORIENTED_EDGE('',*,*,#51438,.F.) ;
#76571=ORIENTED_EDGE('',*,*,#53382,.T.) ;
#76572=ORIENTED_EDGE('',*,*,#51439,.F.) ;
#76573=ORIENTED_EDGE('',*,*,#53387,.F.) ;
#76574=ORIENTED_EDGE('',*,*,#51264,.F.) ;
#76575=ORIENTED_EDGE('',*,*,#53384,.T.) ;
#76576=ORIENTED_EDGE('',*,*,#53254,.F.) ;
#76577=ORIENTED_EDGE('',*,*,#53388,.F.) ;
#76578=ORIENTED_EDGE('',*,*,#53389,.F.) ;
#76579=ORIENTED_EDGE('',*,*,#53385,.T.) ;
#76580=ORIENTED_EDGE('',*,*,#53390,.F.) ;
#76581=ORIENTED_EDGE('',*,*,#53387,.T.) ;
#76582=ORIENTED_EDGE('',*,*,#53386,.T.) ;
#76583=ORIENTED_EDGE('',*,*,#53391,.F.) ;
#76584=ORIENTED_EDGE('',*,*,#51265,.T.) ;
#76585=ORIENTED_EDGE('',*,*,#53388,.T.) ;
#76586=ORIENTED_EDGE('',*,*,#49691,.F.) ;
#76587=ORIENTED_EDGE('',*,*,#53392,.F.) ;
#76588=ORIENTED_EDGE('',*,*,#51248,.F.) ;
#76589=ORIENTED_EDGE('',*,*,#53390,.T.) ;
#76590=ORIENTED_EDGE('',*,*,#51249,.F.) ;
#76591=ORIENTED_EDGE('',*,*,#53393,.F.) ;
#76592=ORIENTED_EDGE('',*,*,#51255,.F.) ;
#76593=ORIENTED_EDGE('',*,*,#53389,.T.) ;
#76594=ORIENTED_EDGE('',*,*,#51258,.F.) ;
#76595=ORIENTED_EDGE('',*,*,#53394,.F.) ;
#76596=ORIENTED_EDGE('',*,*,#49615,.F.) ;
#76597=ORIENTED_EDGE('',*,*,#53391,.T.) ;
#76598=ORIENTED_EDGE('',*,*,#49616,.F.) ;
#76599=ORIENTED_EDGE('',*,*,#53395,.F.) ;
#76600=ORIENTED_EDGE('',*,*,#51266,.F.) ;
#76601=ORIENTED_EDGE('',*,*,#53392,.T.) ;
#76602=ORIENTED_EDGE('',*,*,#49690,.T.) ;
#76603=ORIENTED_EDGE('',*,*,#53396,.F.) ;
#76604=ORIENTED_EDGE('',*,*,#53393,.T.) ;
#76605=ORIENTED_EDGE('',*,*,#53395,.T.) ;
#76606=ORIENTED_EDGE('',*,*,#53394,.T.) ;
#76607=ORIENTED_EDGE('',*,*,#53397,.F.) ;
#76608=ORIENTED_EDGE('',*,*,#53396,.T.) ;
#76609=ORIENTED_EDGE('',*,*,#49689,.F.) ;
#76610=ORIENTED_EDGE('',*,*,#53398,.F.) ;
#76611=ORIENTED_EDGE('',*,*,#51256,.F.) ;
#76612=ORIENTED_EDGE('',*,*,#53397,.T.) ;
#76613=ORIENTED_EDGE('',*,*,#51257,.F.) ;
#76614=ORIENTED_EDGE('',*,*,#53399,.F.) ;
#76615=ORIENTED_EDGE('',*,*,#51267,.F.) ;
#76616=ORIENTED_EDGE('',*,*,#51271,.F.) ;
#76617=ORIENTED_EDGE('',*,*,#53400,.T.) ;
#76618=ORIENTED_EDGE('',*,*,#51259,.F.) ;
#76619=ORIENTED_EDGE('',*,*,#53401,.F.) ;
#76620=ORIENTED_EDGE('',*,*,#49686,.F.) ;
#76621=ORIENTED_EDGE('',*,*,#53402,.T.) ;
#76622=ORIENTED_EDGE('',*,*,#51272,.F.) ;
#76623=ORIENTED_EDGE('',*,*,#53403,.F.) ;
#76624=ORIENTED_EDGE('',*,*,#53398,.T.) ;
#76625=ORIENTED_EDGE('',*,*,#49688,.T.) ;
#76626=ORIENTED_EDGE('',*,*,#53404,.F.) ;
#76627=ORIENTED_EDGE('',*,*,#53399,.T.) ;
#76628=ORIENTED_EDGE('',*,*,#53403,.T.) ;
#76629=ORIENTED_EDGE('',*,*,#53401,.T.) ;
#76630=ORIENTED_EDGE('',*,*,#53405,.F.) ;
#76631=ORIENTED_EDGE('',*,*,#53404,.T.) ;
#76632=ORIENTED_EDGE('',*,*,#49687,.F.) ;
#76633=ORIENTED_EDGE('',*,*,#53405,.T.) ;
#76634=ORIENTED_EDGE('',*,*,#51268,.F.) ;
#76635=ORIENTED_EDGE('',*,*,#52294,.F.) ;
#76636=ORIENTED_EDGE('',*,*,#52305,.F.) ;
#76637=ORIENTED_EDGE('',*,*,#52304,.F.) ;
#76638=ORIENTED_EDGE('',*,*,#53406,.F.) ;
#76639=ORIENTED_EDGE('',*,*,#52295,.F.) ;
#76640=ORIENTED_EDGE('',*,*,#53406,.T.) ;
#76641=ORIENTED_EDGE('',*,*,#50728,.F.) ;
#76642=ORIENTED_EDGE('',*,*,#53407,.F.) ;
#76643=ORIENTED_EDGE('',*,*,#50714,.F.) ;
#76644=ORIENTED_EDGE('',*,*,#52302,.F.) ;
#76645=ORIENTED_EDGE('',*,*,#52301,.F.) ;
#76646=ORIENTED_EDGE('',*,*,#52300,.F.) ;
#76647=ORIENTED_EDGE('',*,*,#53408,.F.) ;
#76648=ORIENTED_EDGE('',*,*,#52303,.F.) ;
#76649=ORIENTED_EDGE('',*,*,#53409,.F.) ;
#76650=ORIENTED_EDGE('',*,*,#53407,.T.) ;
#76651=ORIENTED_EDGE('',*,*,#53410,.F.) ;
#76652=ORIENTED_EDGE('',*,*,#52292,.F.) ;
#76653=ORIENTED_EDGE('',*,*,#52297,.F.) ;
#76654=ORIENTED_EDGE('',*,*,#52296,.F.) ;
#76655=ORIENTED_EDGE('',*,*,#53411,.F.) ;
#76656=ORIENTED_EDGE('',*,*,#52293,.F.) ;
#76657=ORIENTED_EDGE('',*,*,#53408,.T.) ;
#76658=ORIENTED_EDGE('',*,*,#50724,.F.) ;
#76659=ORIENTED_EDGE('',*,*,#53412,.F.) ;
#76660=ORIENTED_EDGE('',*,*,#50726,.F.) ;
#76661=ORIENTED_EDGE('',*,*,#53410,.T.) ;
#76662=ORIENTED_EDGE('',*,*,#50727,.F.) ;
#76663=ORIENTED_EDGE('',*,*,#53413,.F.) ;
#76664=ORIENTED_EDGE('',*,*,#50972,.F.) ;
#76665=ORIENTED_EDGE('',*,*,#53409,.T.) ;
#76666=ORIENTED_EDGE('',*,*,#50971,.F.) ;
#76667=ORIENTED_EDGE('',*,*,#53414,.F.) ;
#76668=ORIENTED_EDGE('',*,*,#50715,.F.) ;
#76669=ORIENTED_EDGE('',*,*,#53411,.T.) ;
#76670=ORIENTED_EDGE('',*,*,#50716,.F.) ;
#76671=ORIENTED_EDGE('',*,*,#53415,.F.) ;
#76672=ORIENTED_EDGE('',*,*,#50720,.F.) ;
#76673=ORIENTED_EDGE('',*,*,#53413,.T.) ;
#76674=ORIENTED_EDGE('',*,*,#53412,.T.) ;
#76675=ORIENTED_EDGE('',*,*,#53416,.F.) ;
#76676=ORIENTED_EDGE('',*,*,#53415,.T.) ;
#76677=ORIENTED_EDGE('',*,*,#53414,.T.) ;
#76678=ORIENTED_EDGE('',*,*,#53417,.F.) ;
#76679=ORIENTED_EDGE('',*,*,#53416,.T.) ;
#76680=ORIENTED_EDGE('',*,*,#50723,.F.) ;
#76681=ORIENTED_EDGE('',*,*,#53418,.F.) ;
#76682=ORIENTED_EDGE('',*,*,#50969,.F.) ;
#76683=ORIENTED_EDGE('',*,*,#53417,.T.) ;
#76684=ORIENTED_EDGE('',*,*,#50970,.F.) ;
#76685=ORIENTED_EDGE('',*,*,#53419,.F.) ;
#76686=ORIENTED_EDGE('',*,*,#50717,.F.) ;
#76687=ORIENTED_EDGE('',*,*,#53419,.T.) ;
#76688=ORIENTED_EDGE('',*,*,#53418,.T.) ;
#76689=ORIENTED_EDGE('',*,*,#53420,.F.) ;
#76690=ORIENTED_EDGE('',*,*,#53420,.T.) ;
#76691=ORIENTED_EDGE('',*,*,#50722,.F.) ;
#76692=ORIENTED_EDGE('',*,*,#53421,.F.) ;
#76693=ORIENTED_EDGE('',*,*,#50718,.F.) ;
#76694=ORIENTED_EDGE('',*,*,#52298,.F.) ;
#76695=ORIENTED_EDGE('',*,*,#52291,.F.) ;
#76696=ORIENTED_EDGE('',*,*,#52290,.F.) ;
#76697=ORIENTED_EDGE('',*,*,#53421,.T.) ;
#76698=ORIENTED_EDGE('',*,*,#52299,.F.) ;
#76699=ORIENTED_EDGE('',*,*,#52531,.F.) ;
#76700=ORIENTED_EDGE('',*,*,#52530,.F.) ;
#76701=ORIENTED_EDGE('',*,*,#52529,.F.) ;
#76702=ORIENTED_EDGE('',*,*,#53422,.F.) ;
#76703=ORIENTED_EDGE('',*,*,#52532,.F.) ;
#76704=ORIENTED_EDGE('',*,*,#53422,.T.) ;
#76705=ORIENTED_EDGE('',*,*,#52528,.F.) ;
#76706=ORIENTED_EDGE('',*,*,#53423,.F.) ;
#76707=ORIENTED_EDGE('',*,*,#50600,.F.) ;
#76708=ORIENTED_EDGE('',*,*,#53423,.T.) ;
#76709=ORIENTED_EDGE('',*,*,#50426,.F.) ;
#76710=ORIENTED_EDGE('',*,*,#53424,.F.) ;
#76711=ORIENTED_EDGE('',*,*,#50601,.F.) ;
#76712=ORIENTED_EDGE('',*,*,#50414,.F.) ;
#76713=ORIENTED_EDGE('',*,*,#50602,.F.) ;
#76714=ORIENTED_EDGE('',*,*,#53425,.F.) ;
#76715=ORIENTED_EDGE('',*,*,#50420,.F.) ;
#76716=ORIENTED_EDGE('',*,*,#53425,.T.) ;
#76717=ORIENTED_EDGE('',*,*,#53424,.T.) ;
#76718=ORIENTED_EDGE('',*,*,#53426,.F.) ;
#76719=ORIENTED_EDGE('',*,*,#53426,.T.) ;
#76720=ORIENTED_EDGE('',*,*,#50425,.F.) ;
#76721=ORIENTED_EDGE('',*,*,#53427,.F.) ;
#76722=ORIENTED_EDGE('',*,*,#50421,.F.) ;
#76723=ORIENTED_EDGE('',*,*,#50416,.F.) ;
#76724=ORIENTED_EDGE('',*,*,#50422,.F.) ;
#76725=ORIENTED_EDGE('',*,*,#53428,.F.) ;
#76726=ORIENTED_EDGE('',*,*,#50664,.F.) ;
#76727=ORIENTED_EDGE('',*,*,#53428,.T.) ;
#76728=ORIENTED_EDGE('',*,*,#53427,.T.) ;
#76729=ORIENTED_EDGE('',*,*,#53429,.F.) ;
#76730=ORIENTED_EDGE('',*,*,#53429,.T.) ;
#76731=ORIENTED_EDGE('',*,*,#50424,.F.) ;
#76732=ORIENTED_EDGE('',*,*,#53430,.F.) ;
#76733=ORIENTED_EDGE('',*,*,#50665,.F.) ;
#76734=ORIENTED_EDGE('',*,*,#53430,.T.) ;
#76735=ORIENTED_EDGE('',*,*,#52527,.F.) ;
#76736=ORIENTED_EDGE('',*,*,#53431,.F.) ;
#76737=ORIENTED_EDGE('',*,*,#50666,.F.) ;
#76738=ORIENTED_EDGE('',*,*,#53431,.T.) ;
#76739=ORIENTED_EDGE('',*,*,#52526,.F.) ;
#76740=ORIENTED_EDGE('',*,*,#52535,.F.) ;
#76741=ORIENTED_EDGE('',*,*,#52536,.F.) ;
#76742=ORIENTED_EDGE('',*,*,#52541,.F.) ;
#76743=ORIENTED_EDGE('',*,*,#53432,.F.) ;
#76744=ORIENTED_EDGE('',*,*,#53432,.T.) ;
#76745=ORIENTED_EDGE('',*,*,#52540,.F.) ;
#76746=ORIENTED_EDGE('',*,*,#53433,.F.) ;
#76747=ORIENTED_EDGE('',*,*,#50661,.F.) ;
#76748=ORIENTED_EDGE('',*,*,#53433,.T.) ;
#76749=ORIENTED_EDGE('',*,*,#50408,.F.) ;
#76750=ORIENTED_EDGE('',*,*,#53434,.F.) ;
#76751=ORIENTED_EDGE('',*,*,#50662,.F.) ;
#76752=ORIENTED_EDGE('',*,*,#50418,.F.) ;
#76753=ORIENTED_EDGE('',*,*,#50663,.F.) ;
#76754=ORIENTED_EDGE('',*,*,#53435,.F.) ;
#76755=ORIENTED_EDGE('',*,*,#50412,.F.) ;
#76756=ORIENTED_EDGE('',*,*,#53435,.T.) ;
#76757=ORIENTED_EDGE('',*,*,#53434,.T.) ;
#76758=ORIENTED_EDGE('',*,*,#53436,.F.) ;
#76759=ORIENTED_EDGE('',*,*,#53436,.T.) ;
#76760=ORIENTED_EDGE('',*,*,#50407,.F.) ;
#76761=ORIENTED_EDGE('',*,*,#53437,.F.) ;
#76762=ORIENTED_EDGE('',*,*,#50409,.F.) ;
#76763=ORIENTED_EDGE('',*,*,#50419,.F.) ;
#76764=ORIENTED_EDGE('',*,*,#50410,.F.) ;
#76765=ORIENTED_EDGE('',*,*,#53438,.F.) ;
#76766=ORIENTED_EDGE('',*,*,#50603,.F.) ;
#76767=ORIENTED_EDGE('',*,*,#53438,.T.) ;
#76768=ORIENTED_EDGE('',*,*,#53437,.T.) ;
#76769=ORIENTED_EDGE('',*,*,#53439,.F.) ;
#76770=ORIENTED_EDGE('',*,*,#53439,.T.) ;
#76771=ORIENTED_EDGE('',*,*,#50406,.F.) ;
#76772=ORIENTED_EDGE('',*,*,#53440,.F.) ;
#76773=ORIENTED_EDGE('',*,*,#50604,.F.) ;
#76774=ORIENTED_EDGE('',*,*,#53440,.T.) ;
#76775=ORIENTED_EDGE('',*,*,#52539,.F.) ;
#76776=ORIENTED_EDGE('',*,*,#53441,.F.) ;
#76777=ORIENTED_EDGE('',*,*,#50605,.F.) ;
#76778=ORIENTED_EDGE('',*,*,#52537,.F.) ;
#76779=ORIENTED_EDGE('',*,*,#52534,.F.) ;
#76780=ORIENTED_EDGE('',*,*,#52533,.F.) ;
#76781=ORIENTED_EDGE('',*,*,#53441,.T.) ;
#76782=ORIENTED_EDGE('',*,*,#52538,.F.) ;
#76783=ORIENTED_EDGE('',*,*,#53442,.F.) ;
#76784=ORIENTED_EDGE('',*,*,#49448,.F.) ;
#76785=ORIENTED_EDGE('',*,*,#53443,.F.) ;
#76786=ORIENTED_EDGE('',*,*,#52125,.F.) ;
#76787=ORIENTED_EDGE('',*,*,#53443,.T.) ;
#76788=ORIENTED_EDGE('',*,*,#49447,.F.) ;
#76789=ORIENTED_EDGE('',*,*,#53444,.F.) ;
#76790=ORIENTED_EDGE('',*,*,#52128,.F.) ;
#76791=ORIENTED_EDGE('',*,*,#53442,.T.) ;
#76792=ORIENTED_EDGE('',*,*,#52122,.F.) ;
#76793=ORIENTED_EDGE('',*,*,#53445,.F.) ;
#76794=ORIENTED_EDGE('',*,*,#49449,.F.) ;
#76795=ORIENTED_EDGE('',*,*,#53444,.T.) ;
#76796=ORIENTED_EDGE('',*,*,#49446,.F.) ;
#76797=ORIENTED_EDGE('',*,*,#53446,.F.) ;
#76798=ORIENTED_EDGE('',*,*,#52131,.F.) ;
#76799=ORIENTED_EDGE('',*,*,#53445,.T.) ;
#76800=ORIENTED_EDGE('',*,*,#52119,.F.) ;
#76801=ORIENTED_EDGE('',*,*,#53447,.F.) ;
#76802=ORIENTED_EDGE('',*,*,#49450,.F.) ;
#76803=ORIENTED_EDGE('',*,*,#53446,.T.) ;
#76804=ORIENTED_EDGE('',*,*,#49445,.F.) ;
#76805=ORIENTED_EDGE('',*,*,#53448,.F.) ;
#76806=ORIENTED_EDGE('',*,*,#52134,.F.) ;
#76807=ORIENTED_EDGE('',*,*,#53447,.T.) ;
#76808=ORIENTED_EDGE('',*,*,#52141,.F.) ;
#76809=ORIENTED_EDGE('',*,*,#53449,.F.) ;
#76810=ORIENTED_EDGE('',*,*,#49443,.F.) ;
#76811=ORIENTED_EDGE('',*,*,#53448,.T.) ;
#76812=ORIENTED_EDGE('',*,*,#49444,.F.) ;
#76813=ORIENTED_EDGE('',*,*,#53449,.T.) ;
#76814=ORIENTED_EDGE('',*,*,#52137,.F.) ;
#76815=ORIENTED_EDGE('',*,*,#50978,.F.) ;
#76816=ORIENTED_EDGE('',*,*,#50992,.F.) ;
#76817=ORIENTED_EDGE('',*,*,#53450,.F.) ;
#76818=ORIENTED_EDGE('',*,*,#50981,.F.) ;
#76819=ORIENTED_EDGE('',*,*,#53451,.F.) ;
#76820=ORIENTED_EDGE('',*,*,#50982,.F.) ;
#76821=ORIENTED_EDGE('',*,*,#53452,.F.) ;
#76822=ORIENTED_EDGE('',*,*,#51068,.F.) ;
#76823=ORIENTED_EDGE('',*,*,#50980,.F.) ;
#76824=ORIENTED_EDGE('',*,*,#50983,.F.) ;
#76825=ORIENTED_EDGE('',*,*,#53453,.F.) ;
#76826=ORIENTED_EDGE('',*,*,#50984,.F.) ;
#76827=ORIENTED_EDGE('',*,*,#53452,.T.) ;
#76828=ORIENTED_EDGE('',*,*,#53450,.T.) ;
#76829=ORIENTED_EDGE('',*,*,#53454,.F.) ;
#76830=ORIENTED_EDGE('',*,*,#53453,.T.) ;
#76831=ORIENTED_EDGE('',*,*,#53451,.T.) ;
#76832=ORIENTED_EDGE('',*,*,#53455,.F.) ;
#76833=ORIENTED_EDGE('',*,*,#50976,.F.) ;
#76834=ORIENTED_EDGE('',*,*,#50988,.F.) ;
#76835=ORIENTED_EDGE('',*,*,#53456,.F.) ;
#76836=ORIENTED_EDGE('',*,*,#50990,.F.) ;
#76837=ORIENTED_EDGE('',*,*,#53454,.T.) ;
#76838=ORIENTED_EDGE('',*,*,#50991,.F.) ;
#76839=ORIENTED_EDGE('',*,*,#53457,.F.) ;
#76840=ORIENTED_EDGE('',*,*,#51065,.F.) ;
#76841=ORIENTED_EDGE('',*,*,#53455,.T.) ;
#76842=ORIENTED_EDGE('',*,*,#51067,.F.) ;
#76843=ORIENTED_EDGE('',*,*,#53458,.F.) ;
#76844=ORIENTED_EDGE('',*,*,#50985,.F.) ;
#76845=ORIENTED_EDGE('',*,*,#50974,.F.) ;
#76846=ORIENTED_EDGE('',*,*,#50986,.F.) ;
#76847=ORIENTED_EDGE('',*,*,#53459,.F.) ;
#76848=ORIENTED_EDGE('',*,*,#50989,.F.) ;
#76849=ORIENTED_EDGE('',*,*,#53457,.T.) ;
#76850=ORIENTED_EDGE('',*,*,#53456,.T.) ;
#76851=ORIENTED_EDGE('',*,*,#53460,.F.) ;
#76852=ORIENTED_EDGE('',*,*,#53459,.T.) ;
#76853=ORIENTED_EDGE('',*,*,#53458,.T.) ;
#76854=ORIENTED_EDGE('',*,*,#53461,.F.) ;
#76855=ORIENTED_EDGE('',*,*,#53460,.T.) ;
#76856=ORIENTED_EDGE('',*,*,#50987,.F.) ;
#76857=ORIENTED_EDGE('',*,*,#53461,.T.) ;
#76858=ORIENTED_EDGE('',*,*,#51066,.F.) ;
#76859=ORIENTED_EDGE('',*,*,#53462,.F.) ;
#76860=ORIENTED_EDGE('',*,*,#49404,.F.) ;
#76861=ORIENTED_EDGE('',*,*,#53463,.F.) ;
#76862=ORIENTED_EDGE('',*,*,#51537,.F.) ;
#76863=ORIENTED_EDGE('',*,*,#53463,.T.) ;
#76864=ORIENTED_EDGE('',*,*,#49403,.T.) ;
#76865=ORIENTED_EDGE('',*,*,#53464,.F.) ;
#76866=ORIENTED_EDGE('',*,*,#53465,.F.) ;
#76867=ORIENTED_EDGE('',*,*,#49405,.T.) ;
#76868=ORIENTED_EDGE('',*,*,#53462,.T.) ;
#76869=ORIENTED_EDGE('',*,*,#53466,.F.) ;
#76870=ORIENTED_EDGE('',*,*,#53467,.F.) ;
#76871=ORIENTED_EDGE('',*,*,#53464,.T.) ;
#76872=ORIENTED_EDGE('',*,*,#49402,.F.) ;
#76873=ORIENTED_EDGE('',*,*,#53468,.F.) ;
#76874=ORIENTED_EDGE('',*,*,#51534,.F.) ;
#76875=ORIENTED_EDGE('',*,*,#53465,.T.) ;
#76876=ORIENTED_EDGE('',*,*,#51533,.F.) ;
#76877=ORIENTED_EDGE('',*,*,#53469,.F.) ;
#76878=ORIENTED_EDGE('',*,*,#51538,.F.) ;
#76879=ORIENTED_EDGE('',*,*,#53470,.F.) ;
#76880=ORIENTED_EDGE('',*,*,#51535,.F.) ;
#76881=ORIENTED_EDGE('',*,*,#53471,.F.) ;
#76882=ORIENTED_EDGE('',*,*,#51782,.F.) ;
#76883=ORIENTED_EDGE('',*,*,#53466,.T.) ;
#76884=ORIENTED_EDGE('',*,*,#51536,.F.) ;
#76885=ORIENTED_EDGE('',*,*,#53472,.F.) ;
#76886=ORIENTED_EDGE('',*,*,#51526,.F.) ;
#76887=ORIENTED_EDGE('',*,*,#53467,.T.) ;
#76888=ORIENTED_EDGE('',*,*,#51525,.F.) ;
#76889=ORIENTED_EDGE('',*,*,#53473,.F.) ;
#76890=ORIENTED_EDGE('',*,*,#49406,.F.) ;
#76891=ORIENTED_EDGE('',*,*,#53474,.F.) ;
#76892=ORIENTED_EDGE('',*,*,#49400,.F.) ;
#76893=ORIENTED_EDGE('',*,*,#53475,.F.) ;
#76894=ORIENTED_EDGE('',*,*,#51527,.F.) ;
#76895=ORIENTED_EDGE('',*,*,#49401,.T.) ;
#76896=ORIENTED_EDGE('',*,*,#53474,.T.) ;
#76897=ORIENTED_EDGE('',*,*,#53476,.F.) ;
#76898=ORIENTED_EDGE('',*,*,#53468,.T.) ;
#76899=ORIENTED_EDGE('',*,*,#53471,.T.) ;
#76900=ORIENTED_EDGE('',*,*,#53469,.T.) ;
#76901=ORIENTED_EDGE('',*,*,#53477,.F.) ;
#76902=ORIENTED_EDGE('',*,*,#53472,.T.) ;
#76903=ORIENTED_EDGE('',*,*,#53470,.T.) ;
#76904=ORIENTED_EDGE('',*,*,#53478,.F.) ;
#76905=ORIENTED_EDGE('',*,*,#49399,.T.) ;
#76906=ORIENTED_EDGE('',*,*,#53473,.T.) ;
#76907=ORIENTED_EDGE('',*,*,#53479,.F.) ;
#76908=ORIENTED_EDGE('',*,*,#53475,.T.) ;
#76909=ORIENTED_EDGE('',*,*,#53476,.T.) ;
#76910=ORIENTED_EDGE('',*,*,#51530,.F.) ;
#76911=ORIENTED_EDGE('',*,*,#53480,.F.) ;
#76912=ORIENTED_EDGE('',*,*,#51531,.F.) ;
#76913=ORIENTED_EDGE('',*,*,#53477,.T.) ;
#76914=ORIENTED_EDGE('',*,*,#51532,.F.) ;
#76915=ORIENTED_EDGE('',*,*,#53481,.F.) ;
#76916=ORIENTED_EDGE('',*,*,#51779,.F.) ;
#76917=ORIENTED_EDGE('',*,*,#53478,.T.) ;
#76918=ORIENTED_EDGE('',*,*,#51781,.F.) ;
#76919=ORIENTED_EDGE('',*,*,#53482,.F.) ;
#76920=ORIENTED_EDGE('',*,*,#51523,.F.) ;
#76921=ORIENTED_EDGE('',*,*,#53479,.T.) ;
#76922=ORIENTED_EDGE('',*,*,#51524,.F.) ;
#76923=ORIENTED_EDGE('',*,*,#53483,.F.) ;
#76924=ORIENTED_EDGE('',*,*,#51528,.F.) ;
#76925=ORIENTED_EDGE('',*,*,#53481,.T.) ;
#76926=ORIENTED_EDGE('',*,*,#53480,.T.) ;
#76927=ORIENTED_EDGE('',*,*,#53484,.F.) ;
#76928=ORIENTED_EDGE('',*,*,#53483,.T.) ;
#76929=ORIENTED_EDGE('',*,*,#53482,.T.) ;
#76930=ORIENTED_EDGE('',*,*,#53485,.F.) ;
#76931=ORIENTED_EDGE('',*,*,#53484,.T.) ;
#76932=ORIENTED_EDGE('',*,*,#51529,.F.) ;
#76933=ORIENTED_EDGE('',*,*,#53485,.T.) ;
#76934=ORIENTED_EDGE('',*,*,#51780,.F.) ;
#76935=ORIENTED_EDGE('',*,*,#51788,.F.) ;
#76936=ORIENTED_EDGE('',*,*,#51801,.F.) ;
#76937=ORIENTED_EDGE('',*,*,#53486,.F.) ;
#76938=ORIENTED_EDGE('',*,*,#51793,.F.) ;
#76939=ORIENTED_EDGE('',*,*,#53487,.F.) ;
#76940=ORIENTED_EDGE('',*,*,#51791,.F.) ;
#76941=ORIENTED_EDGE('',*,*,#53488,.F.) ;
#76942=ORIENTED_EDGE('',*,*,#51878,.F.) ;
#76943=ORIENTED_EDGE('',*,*,#51790,.F.) ;
#76944=ORIENTED_EDGE('',*,*,#51792,.F.) ;
#76945=ORIENTED_EDGE('',*,*,#53489,.F.) ;
#76946=ORIENTED_EDGE('',*,*,#51796,.F.) ;
#76947=ORIENTED_EDGE('',*,*,#53488,.T.) ;
#76948=ORIENTED_EDGE('',*,*,#53486,.T.) ;
#76949=ORIENTED_EDGE('',*,*,#53490,.F.) ;
#76950=ORIENTED_EDGE('',*,*,#53489,.T.) ;
#76951=ORIENTED_EDGE('',*,*,#53487,.T.) ;
#76952=ORIENTED_EDGE('',*,*,#53491,.F.) ;
#76953=ORIENTED_EDGE('',*,*,#51786,.F.) ;
#76954=ORIENTED_EDGE('',*,*,#51799,.F.) ;
#76955=ORIENTED_EDGE('',*,*,#53492,.F.) ;
#76956=ORIENTED_EDGE('',*,*,#51802,.F.) ;
#76957=ORIENTED_EDGE('',*,*,#53490,.T.) ;
#76958=ORIENTED_EDGE('',*,*,#51800,.F.) ;
#76959=ORIENTED_EDGE('',*,*,#53493,.F.) ;
#76960=ORIENTED_EDGE('',*,*,#51875,.F.) ;
#76961=ORIENTED_EDGE('',*,*,#53491,.T.) ;
#76962=ORIENTED_EDGE('',*,*,#51877,.F.) ;
#76963=ORIENTED_EDGE('',*,*,#53494,.F.) ;
#76964=ORIENTED_EDGE('',*,*,#51794,.F.) ;
#76965=ORIENTED_EDGE('',*,*,#51784,.F.) ;
#76966=ORIENTED_EDGE('',*,*,#51795,.F.) ;
#76967=ORIENTED_EDGE('',*,*,#53495,.F.) ;
#76968=ORIENTED_EDGE('',*,*,#51797,.F.) ;
#76969=ORIENTED_EDGE('',*,*,#53493,.T.) ;
#76970=ORIENTED_EDGE('',*,*,#53492,.T.) ;
#76971=ORIENTED_EDGE('',*,*,#53496,.F.) ;
#76972=ORIENTED_EDGE('',*,*,#53495,.T.) ;
#76973=ORIENTED_EDGE('',*,*,#53494,.T.) ;
#76974=ORIENTED_EDGE('',*,*,#53497,.F.) ;
#76975=ORIENTED_EDGE('',*,*,#53496,.T.) ;
#76976=ORIENTED_EDGE('',*,*,#51798,.F.) ;
#76977=ORIENTED_EDGE('',*,*,#53497,.T.) ;
#76978=ORIENTED_EDGE('',*,*,#51876,.F.) ;
#76979=ORIENTED_EDGE('',*,*,#53498,.F.) ;
#76980=ORIENTED_EDGE('',*,*,#52130,.F.) ;
#76981=ORIENTED_EDGE('',*,*,#53499,.F.) ;
#76982=ORIENTED_EDGE('',*,*,#52145,.F.) ;
#76983=ORIENTED_EDGE('',*,*,#53499,.T.) ;
#76984=ORIENTED_EDGE('',*,*,#52133,.F.) ;
#76985=ORIENTED_EDGE('',*,*,#53500,.F.) ;
#76986=ORIENTED_EDGE('',*,*,#52127,.F.) ;
#76987=ORIENTED_EDGE('',*,*,#53498,.T.) ;
#76988=ORIENTED_EDGE('',*,*,#53501,.F.) ;
#76989=ORIENTED_EDGE('',*,*,#53500,.T.) ;
#76990=ORIENTED_EDGE('',*,*,#52136,.F.) ;
#76991=ORIENTED_EDGE('',*,*,#53502,.F.) ;
#76992=ORIENTED_EDGE('',*,*,#52142,.F.) ;
#76993=ORIENTED_EDGE('',*,*,#53501,.T.) ;
#76994=ORIENTED_EDGE('',*,*,#52144,.F.) ;
#76995=ORIENTED_EDGE('',*,*,#53503,.F.) ;
#76996=ORIENTED_EDGE('',*,*,#52124,.F.) ;
#76997=ORIENTED_EDGE('',*,*,#53502,.T.) ;
#76998=ORIENTED_EDGE('',*,*,#52139,.F.) ;
#76999=ORIENTED_EDGE('',*,*,#53504,.F.) ;
#77000=ORIENTED_EDGE('',*,*,#52121,.F.) ;
#77001=ORIENTED_EDGE('',*,*,#53503,.T.) ;
#77002=ORIENTED_EDGE('',*,*,#53505,.F.) ;
#77003=ORIENTED_EDGE('',*,*,#53504,.T.) ;
#77004=ORIENTED_EDGE('',*,*,#52140,.F.) ;
#77005=ORIENTED_EDGE('',*,*,#53505,.T.) ;
#77006=ORIENTED_EDGE('',*,*,#52143,.F.) ;
#77007=ORIENTED_EDGE('',*,*,#49196,.F.) ;
#77008=ORIENTED_EDGE('',*,*,#51889,.F.) ;
#77009=ORIENTED_EDGE('',*,*,#49210,.F.) ;
#77010=ORIENTED_EDGE('',*,*,#51932,.F.) ;
#77011=ORIENTED_EDGE('',*,*,#49198,.F.) ;
#77012=ORIENTED_EDGE('',*,*,#51933,.F.) ;
#77013=ORIENTED_EDGE('',*,*,#49208,.F.) ;
#77014=ORIENTED_EDGE('',*,*,#51936,.F.) ;
#77015=ORIENTED_EDGE('',*,*,#49206,.F.) ;
#77016=ORIENTED_EDGE('',*,*,#51934,.F.) ;
#77017=ORIENTED_EDGE('',*,*,#49200,.F.) ;
#77018=ORIENTED_EDGE('',*,*,#51937,.F.) ;
#77019=ORIENTED_EDGE('',*,*,#49204,.F.) ;
#77020=ORIENTED_EDGE('',*,*,#49525,.F.) ;
#77021=ORIENTED_EDGE('',*,*,#49202,.F.) ;
#77022=ORIENTED_EDGE('',*,*,#51935,.F.) ;
#77023=ORIENTED_EDGE('',*,*,#53506,.F.) ;
#77024=ORIENTED_EDGE('',*,*,#53507,.F.) ;
#77025=ORIENTED_EDGE('',*,*,#53508,.F.) ;
#77026=ORIENTED_EDGE('',*,*,#53507,.T.) ;
#77027=ORIENTED_EDGE('',*,*,#51467,.F.) ;
#77028=ORIENTED_EDGE('',*,*,#53509,.F.) ;
#77029=ORIENTED_EDGE('',*,*,#51462,.F.) ;
#77030=ORIENTED_EDGE('',*,*,#53508,.T.) ;
#77031=ORIENTED_EDGE('',*,*,#51461,.F.) ;
#77032=ORIENTED_EDGE('',*,*,#53510,.F.) ;
#77033=ORIENTED_EDGE('',*,*,#51463,.F.) ;
#77034=ORIENTED_EDGE('',*,*,#53506,.T.) ;
#77035=ORIENTED_EDGE('',*,*,#51466,.F.) ;
#77036=ORIENTED_EDGE('',*,*,#53511,.F.) ;
#77037=ORIENTED_EDGE('',*,*,#51468,.F.) ;
#77038=ORIENTED_EDGE('',*,*,#51472,.F.) ;
#77039=ORIENTED_EDGE('',*,*,#53512,.T.) ;
#77040=ORIENTED_EDGE('',*,*,#51281,.F.) ;
#77041=ORIENTED_EDGE('',*,*,#53513,.F.) ;
#77042=ORIENTED_EDGE('',*,*,#53509,.T.) ;
#77043=ORIENTED_EDGE('',*,*,#53513,.T.) ;
#77044=ORIENTED_EDGE('',*,*,#53514,.F.) ;
#77045=ORIENTED_EDGE('',*,*,#53515,.F.) ;
#77046=ORIENTED_EDGE('',*,*,#53510,.T.) ;
#77047=ORIENTED_EDGE('',*,*,#53516,.F.) ;
#77048=ORIENTED_EDGE('',*,*,#49604,.T.) ;
#77049=ORIENTED_EDGE('',*,*,#53517,.F.) ;
#77050=ORIENTED_EDGE('',*,*,#53511,.T.) ;
#77051=ORIENTED_EDGE('',*,*,#53518,.F.) ;
#77052=ORIENTED_EDGE('',*,*,#51471,.F.) ;
#77053=ORIENTED_EDGE('',*,*,#53519,.T.) ;
#77054=ORIENTED_EDGE('',*,*,#49427,.F.) ;
#77055=ORIENTED_EDGE('',*,*,#53520,.T.) ;
#77056=ORIENTED_EDGE('',*,*,#53514,.T.) ;
#77057=ORIENTED_EDGE('',*,*,#51280,.F.) ;
#77058=ORIENTED_EDGE('',*,*,#53521,.F.) ;
#77059=ORIENTED_EDGE('',*,*,#51459,.F.) ;
#77060=ORIENTED_EDGE('',*,*,#53516,.T.) ;
#77061=ORIENTED_EDGE('',*,*,#51460,.F.) ;
#77062=ORIENTED_EDGE('',*,*,#53522,.F.) ;
#77063=ORIENTED_EDGE('',*,*,#49605,.F.) ;
#77064=ORIENTED_EDGE('',*,*,#53515,.T.) ;
#77065=ORIENTED_EDGE('',*,*,#49611,.F.) ;
#77066=ORIENTED_EDGE('',*,*,#53523,.F.) ;
#77067=ORIENTED_EDGE('',*,*,#51464,.F.) ;
#77068=ORIENTED_EDGE('',*,*,#53518,.T.) ;
#77069=ORIENTED_EDGE('',*,*,#51465,.F.) ;
#77070=ORIENTED_EDGE('',*,*,#53524,.F.) ;
#77071=ORIENTED_EDGE('',*,*,#51455,.F.) ;
#77072=ORIENTED_EDGE('',*,*,#53517,.T.) ;
#77073=ORIENTED_EDGE('',*,*,#51458,.F.) ;
#77074=ORIENTED_EDGE('',*,*,#53525,.F.) ;
#77075=ORIENTED_EDGE('',*,*,#51469,.F.) ;
#77076=ORIENTED_EDGE('',*,*,#51291,.F.) ;
#77077=ORIENTED_EDGE('',*,*,#53526,.T.) ;
#77078=ORIENTED_EDGE('',*,*,#51470,.F.) ;
#77079=ORIENTED_EDGE('',*,*,#53527,.F.) ;
#77080=ORIENTED_EDGE('',*,*,#53521,.T.) ;
#77081=ORIENTED_EDGE('',*,*,#51279,.T.) ;
#77082=ORIENTED_EDGE('',*,*,#53528,.F.) ;
#77083=ORIENTED_EDGE('',*,*,#53522,.T.) ;
#77084=ORIENTED_EDGE('',*,*,#53523,.T.) ;
#77085=ORIENTED_EDGE('',*,*,#49610,.T.) ;
#77086=ORIENTED_EDGE('',*,*,#53529,.F.) ;
#77087=ORIENTED_EDGE('',*,*,#53524,.T.) ;
#77088=ORIENTED_EDGE('',*,*,#53527,.T.) ;
#77089=ORIENTED_EDGE('',*,*,#53525,.T.) ;
#77090=ORIENTED_EDGE('',*,*,#53530,.F.) ;
#77091=ORIENTED_EDGE('',*,*,#51275,.F.) ;
#77092=ORIENTED_EDGE('',*,*,#53531,.T.) ;
#77093=ORIENTED_EDGE('',*,*,#51269,.F.) ;
#77094=ORIENTED_EDGE('',*,*,#53532,.F.) ;
#77095=ORIENTED_EDGE('',*,*,#53528,.T.) ;
#77096=ORIENTED_EDGE('',*,*,#51278,.F.) ;
#77097=ORIENTED_EDGE('',*,*,#53533,.F.) ;
#77098=ORIENTED_EDGE('',*,*,#49606,.F.) ;
#77099=ORIENTED_EDGE('',*,*,#53529,.T.) ;
#77100=ORIENTED_EDGE('',*,*,#49609,.F.) ;
#77101=ORIENTED_EDGE('',*,*,#53534,.F.) ;
#77102=ORIENTED_EDGE('',*,*,#51456,.F.) ;
#77103=ORIENTED_EDGE('',*,*,#53530,.T.) ;
#77104=ORIENTED_EDGE('',*,*,#51457,.F.) ;
#77105=ORIENTED_EDGE('',*,*,#53535,.F.) ;
#77106=ORIENTED_EDGE('',*,*,#51292,.F.) ;
#77107=ORIENTED_EDGE('',*,*,#53532,.T.) ;
#77108=ORIENTED_EDGE('',*,*,#53402,.F.) ;
#77109=ORIENTED_EDGE('',*,*,#53536,.F.) ;
#77110=ORIENTED_EDGE('',*,*,#53537,.F.) ;
#77111=ORIENTED_EDGE('',*,*,#53533,.T.) ;
#77112=ORIENTED_EDGE('',*,*,#53538,.F.) ;
#77113=ORIENTED_EDGE('',*,*,#53535,.T.) ;
#77114=ORIENTED_EDGE('',*,*,#53534,.T.) ;
#77115=ORIENTED_EDGE('',*,*,#53539,.F.) ;
#77116=ORIENTED_EDGE('',*,*,#51293,.T.) ;
#77117=ORIENTED_EDGE('',*,*,#53536,.T.) ;
#77118=ORIENTED_EDGE('',*,*,#49685,.F.) ;
#77119=ORIENTED_EDGE('',*,*,#53540,.F.) ;
#77120=ORIENTED_EDGE('',*,*,#51276,.F.) ;
#77121=ORIENTED_EDGE('',*,*,#53538,.T.) ;
#77122=ORIENTED_EDGE('',*,*,#51277,.F.) ;
#77123=ORIENTED_EDGE('',*,*,#53541,.F.) ;
#77124=ORIENTED_EDGE('',*,*,#51283,.F.) ;
#77125=ORIENTED_EDGE('',*,*,#53537,.T.) ;
#77126=ORIENTED_EDGE('',*,*,#51286,.F.) ;
#77127=ORIENTED_EDGE('',*,*,#53542,.F.) ;
#77128=ORIENTED_EDGE('',*,*,#49607,.F.) ;
#77129=ORIENTED_EDGE('',*,*,#53539,.T.) ;
#77130=ORIENTED_EDGE('',*,*,#49608,.F.) ;
#77131=ORIENTED_EDGE('',*,*,#53543,.F.) ;
#77132=ORIENTED_EDGE('',*,*,#51294,.F.) ;
#77133=ORIENTED_EDGE('',*,*,#53540,.T.) ;
#77134=ORIENTED_EDGE('',*,*,#49684,.T.) ;
#77135=ORIENTED_EDGE('',*,*,#53544,.F.) ;
#77136=ORIENTED_EDGE('',*,*,#53541,.T.) ;
#77137=ORIENTED_EDGE('',*,*,#53543,.T.) ;
#77138=ORIENTED_EDGE('',*,*,#53542,.T.) ;
#77139=ORIENTED_EDGE('',*,*,#53545,.F.) ;
#77140=ORIENTED_EDGE('',*,*,#53544,.T.) ;
#77141=ORIENTED_EDGE('',*,*,#49683,.F.) ;
#77142=ORIENTED_EDGE('',*,*,#53546,.F.) ;
#77143=ORIENTED_EDGE('',*,*,#51284,.F.) ;
#77144=ORIENTED_EDGE('',*,*,#53545,.T.) ;
#77145=ORIENTED_EDGE('',*,*,#51285,.F.) ;
#77146=ORIENTED_EDGE('',*,*,#53547,.F.) ;
#77147=ORIENTED_EDGE('',*,*,#51295,.F.) ;
#77148=ORIENTED_EDGE('',*,*,#51299,.F.) ;
#77149=ORIENTED_EDGE('',*,*,#53548,.T.) ;
#77150=ORIENTED_EDGE('',*,*,#51287,.F.) ;
#77151=ORIENTED_EDGE('',*,*,#53549,.F.) ;
#77152=ORIENTED_EDGE('',*,*,#49680,.F.) ;
#77153=ORIENTED_EDGE('',*,*,#53550,.T.) ;
#77154=ORIENTED_EDGE('',*,*,#51300,.F.) ;
#77155=ORIENTED_EDGE('',*,*,#53551,.F.) ;
#77156=ORIENTED_EDGE('',*,*,#53546,.T.) ;
#77157=ORIENTED_EDGE('',*,*,#49682,.T.) ;
#77158=ORIENTED_EDGE('',*,*,#53552,.F.) ;
#77159=ORIENTED_EDGE('',*,*,#53547,.T.) ;
#77160=ORIENTED_EDGE('',*,*,#53551,.T.) ;
#77161=ORIENTED_EDGE('',*,*,#53549,.T.) ;
#77162=ORIENTED_EDGE('',*,*,#53553,.F.) ;
#77163=ORIENTED_EDGE('',*,*,#53552,.T.) ;
#77164=ORIENTED_EDGE('',*,*,#49681,.F.) ;
#77165=ORIENTED_EDGE('',*,*,#53553,.T.) ;
#77166=ORIENTED_EDGE('',*,*,#51296,.F.) ;
#77167=ORIENTED_EDGE('',*,*,#52278,.F.) ;
#77168=ORIENTED_EDGE('',*,*,#52289,.F.) ;
#77169=ORIENTED_EDGE('',*,*,#52288,.F.) ;
#77170=ORIENTED_EDGE('',*,*,#53554,.F.) ;
#77171=ORIENTED_EDGE('',*,*,#52279,.F.) ;
#77172=ORIENTED_EDGE('',*,*,#53554,.T.) ;
#77173=ORIENTED_EDGE('',*,*,#50712,.F.) ;
#77174=ORIENTED_EDGE('',*,*,#53555,.F.) ;
#77175=ORIENTED_EDGE('',*,*,#50698,.F.) ;
#77176=ORIENTED_EDGE('',*,*,#52286,.F.) ;
#77177=ORIENTED_EDGE('',*,*,#52285,.F.) ;
#77178=ORIENTED_EDGE('',*,*,#52284,.F.) ;
#77179=ORIENTED_EDGE('',*,*,#53556,.F.) ;
#77180=ORIENTED_EDGE('',*,*,#52287,.F.) ;
#77181=ORIENTED_EDGE('',*,*,#53557,.F.) ;
#77182=ORIENTED_EDGE('',*,*,#53555,.T.) ;
#77183=ORIENTED_EDGE('',*,*,#53558,.F.) ;
#77184=ORIENTED_EDGE('',*,*,#52276,.F.) ;
#77185=ORIENTED_EDGE('',*,*,#52281,.F.) ;
#77186=ORIENTED_EDGE('',*,*,#52280,.F.) ;
#77187=ORIENTED_EDGE('',*,*,#53559,.F.) ;
#77188=ORIENTED_EDGE('',*,*,#52277,.F.) ;
#77189=ORIENTED_EDGE('',*,*,#53556,.T.) ;
#77190=ORIENTED_EDGE('',*,*,#50708,.F.) ;
#77191=ORIENTED_EDGE('',*,*,#53560,.F.) ;
#77192=ORIENTED_EDGE('',*,*,#50710,.F.) ;
#77193=ORIENTED_EDGE('',*,*,#53558,.T.) ;
#77194=ORIENTED_EDGE('',*,*,#50711,.F.) ;
#77195=ORIENTED_EDGE('',*,*,#53561,.F.) ;
#77196=ORIENTED_EDGE('',*,*,#50996,.F.) ;
#77197=ORIENTED_EDGE('',*,*,#53557,.T.) ;
#77198=ORIENTED_EDGE('',*,*,#50995,.F.) ;
#77199=ORIENTED_EDGE('',*,*,#53562,.F.) ;
#77200=ORIENTED_EDGE('',*,*,#50699,.F.) ;
#77201=ORIENTED_EDGE('',*,*,#53559,.T.) ;
#77202=ORIENTED_EDGE('',*,*,#50700,.F.) ;
#77203=ORIENTED_EDGE('',*,*,#53563,.F.) ;
#77204=ORIENTED_EDGE('',*,*,#50704,.F.) ;
#77205=ORIENTED_EDGE('',*,*,#53561,.T.) ;
#77206=ORIENTED_EDGE('',*,*,#53560,.T.) ;
#77207=ORIENTED_EDGE('',*,*,#53564,.F.) ;
#77208=ORIENTED_EDGE('',*,*,#53563,.T.) ;
#77209=ORIENTED_EDGE('',*,*,#53562,.T.) ;
#77210=ORIENTED_EDGE('',*,*,#53565,.F.) ;
#77211=ORIENTED_EDGE('',*,*,#53564,.T.) ;
#77212=ORIENTED_EDGE('',*,*,#50707,.F.) ;
#77213=ORIENTED_EDGE('',*,*,#53566,.F.) ;
#77214=ORIENTED_EDGE('',*,*,#50993,.F.) ;
#77215=ORIENTED_EDGE('',*,*,#53565,.T.) ;
#77216=ORIENTED_EDGE('',*,*,#50994,.F.) ;
#77217=ORIENTED_EDGE('',*,*,#53567,.F.) ;
#77218=ORIENTED_EDGE('',*,*,#50701,.F.) ;
#77219=ORIENTED_EDGE('',*,*,#53567,.T.) ;
#77220=ORIENTED_EDGE('',*,*,#53566,.T.) ;
#77221=ORIENTED_EDGE('',*,*,#53568,.F.) ;
#77222=ORIENTED_EDGE('',*,*,#53568,.T.) ;
#77223=ORIENTED_EDGE('',*,*,#50706,.F.) ;
#77224=ORIENTED_EDGE('',*,*,#53569,.F.) ;
#77225=ORIENTED_EDGE('',*,*,#50702,.F.) ;
#77226=ORIENTED_EDGE('',*,*,#52282,.F.) ;
#77227=ORIENTED_EDGE('',*,*,#52275,.F.) ;
#77228=ORIENTED_EDGE('',*,*,#52274,.F.) ;
#77229=ORIENTED_EDGE('',*,*,#53569,.T.) ;
#77230=ORIENTED_EDGE('',*,*,#52283,.F.) ;
#77231=ORIENTED_EDGE('',*,*,#52547,.F.) ;
#77232=ORIENTED_EDGE('',*,*,#52546,.F.) ;
#77233=ORIENTED_EDGE('',*,*,#52545,.F.) ;
#77234=ORIENTED_EDGE('',*,*,#53570,.F.) ;
#77235=ORIENTED_EDGE('',*,*,#52548,.F.) ;
#77236=ORIENTED_EDGE('',*,*,#53570,.T.) ;
#77237=ORIENTED_EDGE('',*,*,#52544,.F.) ;
#77238=ORIENTED_EDGE('',*,*,#53571,.F.) ;
#77239=ORIENTED_EDGE('',*,*,#50607,.F.) ;
#77240=ORIENTED_EDGE('',*,*,#53571,.T.) ;
#77241=ORIENTED_EDGE('',*,*,#50404,.F.) ;
#77242=ORIENTED_EDGE('',*,*,#53572,.F.) ;
#77243=ORIENTED_EDGE('',*,*,#50608,.F.) ;
#77244=ORIENTED_EDGE('',*,*,#50392,.F.) ;
#77245=ORIENTED_EDGE('',*,*,#50609,.F.) ;
#77246=ORIENTED_EDGE('',*,*,#53573,.F.) ;
#77247=ORIENTED_EDGE('',*,*,#50398,.F.) ;
#77248=ORIENTED_EDGE('',*,*,#53573,.T.) ;
#77249=ORIENTED_EDGE('',*,*,#53572,.T.) ;
#77250=ORIENTED_EDGE('',*,*,#53574,.F.) ;
#77251=ORIENTED_EDGE('',*,*,#53574,.T.) ;
#77252=ORIENTED_EDGE('',*,*,#50403,.F.) ;
#77253=ORIENTED_EDGE('',*,*,#53575,.F.) ;
#77254=ORIENTED_EDGE('',*,*,#50399,.F.) ;
#77255=ORIENTED_EDGE('',*,*,#50394,.F.) ;
#77256=ORIENTED_EDGE('',*,*,#50400,.F.) ;
#77257=ORIENTED_EDGE('',*,*,#53576,.F.) ;
#77258=ORIENTED_EDGE('',*,*,#50671,.F.) ;
#77259=ORIENTED_EDGE('',*,*,#53576,.T.) ;
#77260=ORIENTED_EDGE('',*,*,#53575,.T.) ;
#77261=ORIENTED_EDGE('',*,*,#53577,.F.) ;
#77262=ORIENTED_EDGE('',*,*,#53577,.T.) ;
#77263=ORIENTED_EDGE('',*,*,#50402,.F.) ;
#77264=ORIENTED_EDGE('',*,*,#53578,.F.) ;
#77265=ORIENTED_EDGE('',*,*,#50672,.F.) ;
#77266=ORIENTED_EDGE('',*,*,#53578,.T.) ;
#77267=ORIENTED_EDGE('',*,*,#52543,.F.) ;
#77268=ORIENTED_EDGE('',*,*,#53579,.F.) ;
#77269=ORIENTED_EDGE('',*,*,#50673,.F.) ;
#77270=ORIENTED_EDGE('',*,*,#53579,.T.) ;
#77271=ORIENTED_EDGE('',*,*,#52542,.F.) ;
#77272=ORIENTED_EDGE('',*,*,#52551,.F.) ;
#77273=ORIENTED_EDGE('',*,*,#52552,.F.) ;
#77274=ORIENTED_EDGE('',*,*,#52557,.F.) ;
#77275=ORIENTED_EDGE('',*,*,#53580,.F.) ;
#77276=ORIENTED_EDGE('',*,*,#53580,.T.) ;
#77277=ORIENTED_EDGE('',*,*,#52556,.F.) ;
#77278=ORIENTED_EDGE('',*,*,#53581,.F.) ;
#77279=ORIENTED_EDGE('',*,*,#50668,.F.) ;
#77280=ORIENTED_EDGE('',*,*,#53581,.T.) ;
#77281=ORIENTED_EDGE('',*,*,#50386,.F.) ;
#77282=ORIENTED_EDGE('',*,*,#53582,.F.) ;
#77283=ORIENTED_EDGE('',*,*,#50669,.F.) ;
#77284=ORIENTED_EDGE('',*,*,#50396,.F.) ;
#77285=ORIENTED_EDGE('',*,*,#50670,.F.) ;
#77286=ORIENTED_EDGE('',*,*,#53583,.F.) ;
#77287=ORIENTED_EDGE('',*,*,#50390,.F.) ;
#77288=ORIENTED_EDGE('',*,*,#53583,.T.) ;
#77289=ORIENTED_EDGE('',*,*,#53582,.T.) ;
#77290=ORIENTED_EDGE('',*,*,#53584,.F.) ;
#77291=ORIENTED_EDGE('',*,*,#53584,.T.) ;
#77292=ORIENTED_EDGE('',*,*,#50385,.F.) ;
#77293=ORIENTED_EDGE('',*,*,#53585,.F.) ;
#77294=ORIENTED_EDGE('',*,*,#50387,.F.) ;
#77295=ORIENTED_EDGE('',*,*,#50397,.F.) ;
#77296=ORIENTED_EDGE('',*,*,#50388,.F.) ;
#77297=ORIENTED_EDGE('',*,*,#53586,.F.) ;
#77298=ORIENTED_EDGE('',*,*,#50610,.F.) ;
#77299=ORIENTED_EDGE('',*,*,#53586,.T.) ;
#77300=ORIENTED_EDGE('',*,*,#53585,.T.) ;
#77301=ORIENTED_EDGE('',*,*,#53587,.F.) ;
#77302=ORIENTED_EDGE('',*,*,#53587,.T.) ;
#77303=ORIENTED_EDGE('',*,*,#50384,.F.) ;
#77304=ORIENTED_EDGE('',*,*,#53588,.F.) ;
#77305=ORIENTED_EDGE('',*,*,#50611,.F.) ;
#77306=ORIENTED_EDGE('',*,*,#53588,.T.) ;
#77307=ORIENTED_EDGE('',*,*,#52555,.F.) ;
#77308=ORIENTED_EDGE('',*,*,#53589,.F.) ;
#77309=ORIENTED_EDGE('',*,*,#50612,.F.) ;
#77310=ORIENTED_EDGE('',*,*,#52553,.F.) ;
#77311=ORIENTED_EDGE('',*,*,#52550,.F.) ;
#77312=ORIENTED_EDGE('',*,*,#52549,.F.) ;
#77313=ORIENTED_EDGE('',*,*,#53589,.T.) ;
#77314=ORIENTED_EDGE('',*,*,#52554,.F.) ;
#77315=ORIENTED_EDGE('',*,*,#53590,.F.) ;
#77316=ORIENTED_EDGE('',*,*,#49436,.F.) ;
#77317=ORIENTED_EDGE('',*,*,#53591,.F.) ;
#77318=ORIENTED_EDGE('',*,*,#52153,.F.) ;
#77319=ORIENTED_EDGE('',*,*,#53591,.T.) ;
#77320=ORIENTED_EDGE('',*,*,#49435,.F.) ;
#77321=ORIENTED_EDGE('',*,*,#53592,.F.) ;
#77322=ORIENTED_EDGE('',*,*,#52156,.F.) ;
#77323=ORIENTED_EDGE('',*,*,#53590,.T.) ;
#77324=ORIENTED_EDGE('',*,*,#52150,.F.) ;
#77325=ORIENTED_EDGE('',*,*,#53593,.F.) ;
#77326=ORIENTED_EDGE('',*,*,#49437,.F.) ;
#77327=ORIENTED_EDGE('',*,*,#53592,.T.) ;
#77328=ORIENTED_EDGE('',*,*,#49434,.F.) ;
#77329=ORIENTED_EDGE('',*,*,#53594,.F.) ;
#77330=ORIENTED_EDGE('',*,*,#52159,.F.) ;
#77331=ORIENTED_EDGE('',*,*,#53593,.T.) ;
#77332=ORIENTED_EDGE('',*,*,#52147,.F.) ;
#77333=ORIENTED_EDGE('',*,*,#53595,.F.) ;
#77334=ORIENTED_EDGE('',*,*,#49438,.F.) ;
#77335=ORIENTED_EDGE('',*,*,#53594,.T.) ;
#77336=ORIENTED_EDGE('',*,*,#49433,.F.) ;
#77337=ORIENTED_EDGE('',*,*,#53596,.F.) ;
#77338=ORIENTED_EDGE('',*,*,#52162,.F.) ;
#77339=ORIENTED_EDGE('',*,*,#53595,.T.) ;
#77340=ORIENTED_EDGE('',*,*,#52169,.F.) ;
#77341=ORIENTED_EDGE('',*,*,#53597,.F.) ;
#77342=ORIENTED_EDGE('',*,*,#49431,.F.) ;
#77343=ORIENTED_EDGE('',*,*,#53596,.T.) ;
#77344=ORIENTED_EDGE('',*,*,#49432,.F.) ;
#77345=ORIENTED_EDGE('',*,*,#53597,.T.) ;
#77346=ORIENTED_EDGE('',*,*,#52165,.F.) ;
#77347=ORIENTED_EDGE('',*,*,#51002,.F.) ;
#77348=ORIENTED_EDGE('',*,*,#51016,.F.) ;
#77349=ORIENTED_EDGE('',*,*,#53598,.F.) ;
#77350=ORIENTED_EDGE('',*,*,#51005,.F.) ;
#77351=ORIENTED_EDGE('',*,*,#53599,.F.) ;
#77352=ORIENTED_EDGE('',*,*,#51006,.F.) ;
#77353=ORIENTED_EDGE('',*,*,#53600,.F.) ;
#77354=ORIENTED_EDGE('',*,*,#51072,.F.) ;
#77355=ORIENTED_EDGE('',*,*,#51004,.F.) ;
#77356=ORIENTED_EDGE('',*,*,#51007,.F.) ;
#77357=ORIENTED_EDGE('',*,*,#53601,.F.) ;
#77358=ORIENTED_EDGE('',*,*,#51008,.F.) ;
#77359=ORIENTED_EDGE('',*,*,#53600,.T.) ;
#77360=ORIENTED_EDGE('',*,*,#53598,.T.) ;
#77361=ORIENTED_EDGE('',*,*,#53602,.F.) ;
#77362=ORIENTED_EDGE('',*,*,#53601,.T.) ;
#77363=ORIENTED_EDGE('',*,*,#53599,.T.) ;
#77364=ORIENTED_EDGE('',*,*,#53603,.F.) ;
#77365=ORIENTED_EDGE('',*,*,#51000,.F.) ;
#77366=ORIENTED_EDGE('',*,*,#51012,.F.) ;
#77367=ORIENTED_EDGE('',*,*,#53604,.F.) ;
#77368=ORIENTED_EDGE('',*,*,#51014,.F.) ;
#77369=ORIENTED_EDGE('',*,*,#53602,.T.) ;
#77370=ORIENTED_EDGE('',*,*,#51015,.F.) ;
#77371=ORIENTED_EDGE('',*,*,#53605,.F.) ;
#77372=ORIENTED_EDGE('',*,*,#51069,.F.) ;
#77373=ORIENTED_EDGE('',*,*,#53603,.T.) ;
#77374=ORIENTED_EDGE('',*,*,#51071,.F.) ;
#77375=ORIENTED_EDGE('',*,*,#53606,.F.) ;
#77376=ORIENTED_EDGE('',*,*,#51009,.F.) ;
#77377=ORIENTED_EDGE('',*,*,#50998,.F.) ;
#77378=ORIENTED_EDGE('',*,*,#51010,.F.) ;
#77379=ORIENTED_EDGE('',*,*,#53607,.F.) ;
#77380=ORIENTED_EDGE('',*,*,#51013,.F.) ;
#77381=ORIENTED_EDGE('',*,*,#53605,.T.) ;
#77382=ORIENTED_EDGE('',*,*,#53604,.T.) ;
#77383=ORIENTED_EDGE('',*,*,#53608,.F.) ;
#77384=ORIENTED_EDGE('',*,*,#53607,.T.) ;
#77385=ORIENTED_EDGE('',*,*,#53606,.T.) ;
#77386=ORIENTED_EDGE('',*,*,#53609,.F.) ;
#77387=ORIENTED_EDGE('',*,*,#53608,.T.) ;
#77388=ORIENTED_EDGE('',*,*,#51011,.F.) ;
#77389=ORIENTED_EDGE('',*,*,#53609,.T.) ;
#77390=ORIENTED_EDGE('',*,*,#51070,.F.) ;
#77391=ORIENTED_EDGE('',*,*,#53610,.F.) ;
#77392=ORIENTED_EDGE('',*,*,#49340,.F.) ;
#77393=ORIENTED_EDGE('',*,*,#53611,.F.) ;
#77394=ORIENTED_EDGE('',*,*,#51521,.F.) ;
#77395=ORIENTED_EDGE('',*,*,#53611,.T.) ;
#77396=ORIENTED_EDGE('',*,*,#49339,.T.) ;
#77397=ORIENTED_EDGE('',*,*,#53612,.F.) ;
#77398=ORIENTED_EDGE('',*,*,#53613,.F.) ;
#77399=ORIENTED_EDGE('',*,*,#49341,.T.) ;
#77400=ORIENTED_EDGE('',*,*,#53610,.T.) ;
#77401=ORIENTED_EDGE('',*,*,#53614,.F.) ;
#77402=ORIENTED_EDGE('',*,*,#53615,.F.) ;
#77403=ORIENTED_EDGE('',*,*,#53612,.T.) ;
#77404=ORIENTED_EDGE('',*,*,#49338,.F.) ;
#77405=ORIENTED_EDGE('',*,*,#53616,.F.) ;
#77406=ORIENTED_EDGE('',*,*,#51518,.F.) ;
#77407=ORIENTED_EDGE('',*,*,#53613,.T.) ;
#77408=ORIENTED_EDGE('',*,*,#51517,.F.) ;
#77409=ORIENTED_EDGE('',*,*,#53617,.F.) ;
#77410=ORIENTED_EDGE('',*,*,#51522,.F.) ;
#77411=ORIENTED_EDGE('',*,*,#53618,.F.) ;
#77412=ORIENTED_EDGE('',*,*,#51519,.F.) ;
#77413=ORIENTED_EDGE('',*,*,#53619,.F.) ;
#77414=ORIENTED_EDGE('',*,*,#51806,.F.) ;
#77415=ORIENTED_EDGE('',*,*,#53614,.T.) ;
#77416=ORIENTED_EDGE('',*,*,#51520,.F.) ;
#77417=ORIENTED_EDGE('',*,*,#53620,.F.) ;
#77418=ORIENTED_EDGE('',*,*,#51510,.F.) ;
#77419=ORIENTED_EDGE('',*,*,#53615,.T.) ;
#77420=ORIENTED_EDGE('',*,*,#51509,.F.) ;
#77421=ORIENTED_EDGE('',*,*,#53621,.F.) ;
#77422=ORIENTED_EDGE('',*,*,#49342,.F.) ;
#77423=ORIENTED_EDGE('',*,*,#53622,.F.) ;
#77424=ORIENTED_EDGE('',*,*,#49336,.F.) ;
#77425=ORIENTED_EDGE('',*,*,#53623,.F.) ;
#77426=ORIENTED_EDGE('',*,*,#51511,.F.) ;
#77427=ORIENTED_EDGE('',*,*,#49337,.T.) ;
#77428=ORIENTED_EDGE('',*,*,#53622,.T.) ;
#77429=ORIENTED_EDGE('',*,*,#53624,.F.) ;
#77430=ORIENTED_EDGE('',*,*,#53616,.T.) ;
#77431=ORIENTED_EDGE('',*,*,#53619,.T.) ;
#77432=ORIENTED_EDGE('',*,*,#53617,.T.) ;
#77433=ORIENTED_EDGE('',*,*,#53625,.F.) ;
#77434=ORIENTED_EDGE('',*,*,#53620,.T.) ;
#77435=ORIENTED_EDGE('',*,*,#53618,.T.) ;
#77436=ORIENTED_EDGE('',*,*,#53626,.F.) ;
#77437=ORIENTED_EDGE('',*,*,#49335,.T.) ;
#77438=ORIENTED_EDGE('',*,*,#53621,.T.) ;
#77439=ORIENTED_EDGE('',*,*,#53627,.F.) ;
#77440=ORIENTED_EDGE('',*,*,#53623,.T.) ;
#77441=ORIENTED_EDGE('',*,*,#53624,.T.) ;
#77442=ORIENTED_EDGE('',*,*,#51514,.F.) ;
#77443=ORIENTED_EDGE('',*,*,#53628,.F.) ;
#77444=ORIENTED_EDGE('',*,*,#51515,.F.) ;
#77445=ORIENTED_EDGE('',*,*,#53625,.T.) ;
#77446=ORIENTED_EDGE('',*,*,#51516,.F.) ;
#77447=ORIENTED_EDGE('',*,*,#53629,.F.) ;
#77448=ORIENTED_EDGE('',*,*,#51803,.F.) ;
#77449=ORIENTED_EDGE('',*,*,#53626,.T.) ;
#77450=ORIENTED_EDGE('',*,*,#51805,.F.) ;
#77451=ORIENTED_EDGE('',*,*,#53630,.F.) ;
#77452=ORIENTED_EDGE('',*,*,#51507,.F.) ;
#77453=ORIENTED_EDGE('',*,*,#53627,.T.) ;
#77454=ORIENTED_EDGE('',*,*,#51508,.F.) ;
#77455=ORIENTED_EDGE('',*,*,#53631,.F.) ;
#77456=ORIENTED_EDGE('',*,*,#51512,.F.) ;
#77457=ORIENTED_EDGE('',*,*,#53629,.T.) ;
#77458=ORIENTED_EDGE('',*,*,#53628,.T.) ;
#77459=ORIENTED_EDGE('',*,*,#53632,.F.) ;
#77460=ORIENTED_EDGE('',*,*,#53631,.T.) ;
#77461=ORIENTED_EDGE('',*,*,#53630,.T.) ;
#77462=ORIENTED_EDGE('',*,*,#53633,.F.) ;
#77463=ORIENTED_EDGE('',*,*,#53632,.T.) ;
#77464=ORIENTED_EDGE('',*,*,#51513,.F.) ;
#77465=ORIENTED_EDGE('',*,*,#53633,.T.) ;
#77466=ORIENTED_EDGE('',*,*,#51804,.F.) ;
#77467=ORIENTED_EDGE('',*,*,#51812,.F.) ;
#77468=ORIENTED_EDGE('',*,*,#51825,.F.) ;
#77469=ORIENTED_EDGE('',*,*,#53634,.F.) ;
#77470=ORIENTED_EDGE('',*,*,#51817,.F.) ;
#77471=ORIENTED_EDGE('',*,*,#53635,.F.) ;
#77472=ORIENTED_EDGE('',*,*,#51815,.F.) ;
#77473=ORIENTED_EDGE('',*,*,#53636,.F.) ;
#77474=ORIENTED_EDGE('',*,*,#51882,.F.) ;
#77475=ORIENTED_EDGE('',*,*,#51814,.F.) ;
#77476=ORIENTED_EDGE('',*,*,#51816,.F.) ;
#77477=ORIENTED_EDGE('',*,*,#53637,.F.) ;
#77478=ORIENTED_EDGE('',*,*,#51820,.F.) ;
#77479=ORIENTED_EDGE('',*,*,#53636,.T.) ;
#77480=ORIENTED_EDGE('',*,*,#53634,.T.) ;
#77481=ORIENTED_EDGE('',*,*,#53638,.F.) ;
#77482=ORIENTED_EDGE('',*,*,#53637,.T.) ;
#77483=ORIENTED_EDGE('',*,*,#53635,.T.) ;
#77484=ORIENTED_EDGE('',*,*,#53639,.F.) ;
#77485=ORIENTED_EDGE('',*,*,#51810,.F.) ;
#77486=ORIENTED_EDGE('',*,*,#51823,.F.) ;
#77487=ORIENTED_EDGE('',*,*,#53640,.F.) ;
#77488=ORIENTED_EDGE('',*,*,#51826,.F.) ;
#77489=ORIENTED_EDGE('',*,*,#53638,.T.) ;
#77490=ORIENTED_EDGE('',*,*,#51824,.F.) ;
#77491=ORIENTED_EDGE('',*,*,#53641,.F.) ;
#77492=ORIENTED_EDGE('',*,*,#51879,.F.) ;
#77493=ORIENTED_EDGE('',*,*,#53639,.T.) ;
#77494=ORIENTED_EDGE('',*,*,#51881,.F.) ;
#77495=ORIENTED_EDGE('',*,*,#53642,.F.) ;
#77496=ORIENTED_EDGE('',*,*,#51818,.F.) ;
#77497=ORIENTED_EDGE('',*,*,#51808,.F.) ;
#77498=ORIENTED_EDGE('',*,*,#51819,.F.) ;
#77499=ORIENTED_EDGE('',*,*,#53643,.F.) ;
#77500=ORIENTED_EDGE('',*,*,#51821,.F.) ;
#77501=ORIENTED_EDGE('',*,*,#53641,.T.) ;
#77502=ORIENTED_EDGE('',*,*,#53640,.T.) ;
#77503=ORIENTED_EDGE('',*,*,#53644,.F.) ;
#77504=ORIENTED_EDGE('',*,*,#53643,.T.) ;
#77505=ORIENTED_EDGE('',*,*,#53642,.T.) ;
#77506=ORIENTED_EDGE('',*,*,#53645,.F.) ;
#77507=ORIENTED_EDGE('',*,*,#53644,.T.) ;
#77508=ORIENTED_EDGE('',*,*,#51822,.F.) ;
#77509=ORIENTED_EDGE('',*,*,#53645,.T.) ;
#77510=ORIENTED_EDGE('',*,*,#51880,.F.) ;
#77511=ORIENTED_EDGE('',*,*,#53646,.F.) ;
#77512=ORIENTED_EDGE('',*,*,#52158,.F.) ;
#77513=ORIENTED_EDGE('',*,*,#53647,.F.) ;
#77514=ORIENTED_EDGE('',*,*,#52173,.F.) ;
#77515=ORIENTED_EDGE('',*,*,#53647,.T.) ;
#77516=ORIENTED_EDGE('',*,*,#52161,.F.) ;
#77517=ORIENTED_EDGE('',*,*,#53648,.F.) ;
#77518=ORIENTED_EDGE('',*,*,#52155,.F.) ;
#77519=ORIENTED_EDGE('',*,*,#53646,.T.) ;
#77520=ORIENTED_EDGE('',*,*,#53649,.F.) ;
#77521=ORIENTED_EDGE('',*,*,#53648,.T.) ;
#77522=ORIENTED_EDGE('',*,*,#52164,.F.) ;
#77523=ORIENTED_EDGE('',*,*,#53650,.F.) ;
#77524=ORIENTED_EDGE('',*,*,#52170,.F.) ;
#77525=ORIENTED_EDGE('',*,*,#53649,.T.) ;
#77526=ORIENTED_EDGE('',*,*,#52172,.F.) ;
#77527=ORIENTED_EDGE('',*,*,#53651,.F.) ;
#77528=ORIENTED_EDGE('',*,*,#52152,.F.) ;
#77529=ORIENTED_EDGE('',*,*,#53650,.T.) ;
#77530=ORIENTED_EDGE('',*,*,#52167,.F.) ;
#77531=ORIENTED_EDGE('',*,*,#53652,.F.) ;
#77532=ORIENTED_EDGE('',*,*,#52149,.F.) ;
#77533=ORIENTED_EDGE('',*,*,#53651,.T.) ;
#77534=ORIENTED_EDGE('',*,*,#53653,.F.) ;
#77535=ORIENTED_EDGE('',*,*,#53652,.T.) ;
#77536=ORIENTED_EDGE('',*,*,#52168,.F.) ;
#77537=ORIENTED_EDGE('',*,*,#53653,.T.) ;
#77538=ORIENTED_EDGE('',*,*,#52171,.F.) ;
#77539=ORIENTED_EDGE('',*,*,#49214,.F.) ;
#77540=ORIENTED_EDGE('',*,*,#51888,.F.) ;
#77541=ORIENTED_EDGE('',*,*,#49228,.F.) ;
#77542=ORIENTED_EDGE('',*,*,#51938,.F.) ;
#77543=ORIENTED_EDGE('',*,*,#49216,.F.) ;
#77544=ORIENTED_EDGE('',*,*,#51939,.F.) ;
#77545=ORIENTED_EDGE('',*,*,#49226,.F.) ;
#77546=ORIENTED_EDGE('',*,*,#51942,.F.) ;
#77547=ORIENTED_EDGE('',*,*,#49224,.F.) ;
#77548=ORIENTED_EDGE('',*,*,#51940,.F.) ;
#77549=ORIENTED_EDGE('',*,*,#49218,.F.) ;
#77550=ORIENTED_EDGE('',*,*,#51943,.F.) ;
#77551=ORIENTED_EDGE('',*,*,#49222,.F.) ;
#77552=ORIENTED_EDGE('',*,*,#49524,.F.) ;
#77553=ORIENTED_EDGE('',*,*,#49220,.F.) ;
#77554=ORIENTED_EDGE('',*,*,#51941,.F.) ;
#77555=ORIENTED_EDGE('',*,*,#53654,.F.) ;
#77556=ORIENTED_EDGE('',*,*,#53655,.F.) ;
#77557=ORIENTED_EDGE('',*,*,#53656,.F.) ;
#77558=ORIENTED_EDGE('',*,*,#53655,.T.) ;
#77559=ORIENTED_EDGE('',*,*,#51485,.F.) ;
#77560=ORIENTED_EDGE('',*,*,#53657,.F.) ;
#77561=ORIENTED_EDGE('',*,*,#51480,.F.) ;
#77562=ORIENTED_EDGE('',*,*,#53656,.T.) ;
#77563=ORIENTED_EDGE('',*,*,#51479,.F.) ;
#77564=ORIENTED_EDGE('',*,*,#53658,.F.) ;
#77565=ORIENTED_EDGE('',*,*,#51481,.F.) ;
#77566=ORIENTED_EDGE('',*,*,#53654,.T.) ;
#77567=ORIENTED_EDGE('',*,*,#51484,.F.) ;
#77568=ORIENTED_EDGE('',*,*,#53659,.F.) ;
#77569=ORIENTED_EDGE('',*,*,#51486,.F.) ;
#77570=ORIENTED_EDGE('',*,*,#51490,.F.) ;
#77571=ORIENTED_EDGE('',*,*,#53660,.T.) ;
#77572=ORIENTED_EDGE('',*,*,#51309,.F.) ;
#77573=ORIENTED_EDGE('',*,*,#53661,.F.) ;
#77574=ORIENTED_EDGE('',*,*,#53657,.T.) ;
#77575=ORIENTED_EDGE('',*,*,#53661,.T.) ;
#77576=ORIENTED_EDGE('',*,*,#53662,.F.) ;
#77577=ORIENTED_EDGE('',*,*,#53663,.F.) ;
#77578=ORIENTED_EDGE('',*,*,#53658,.T.) ;
#77579=ORIENTED_EDGE('',*,*,#53664,.F.) ;
#77580=ORIENTED_EDGE('',*,*,#49596,.T.) ;
#77581=ORIENTED_EDGE('',*,*,#53665,.F.) ;
#77582=ORIENTED_EDGE('',*,*,#53659,.T.) ;
#77583=ORIENTED_EDGE('',*,*,#53666,.F.) ;
#77584=ORIENTED_EDGE('',*,*,#51489,.F.) ;
#77585=ORIENTED_EDGE('',*,*,#53667,.T.) ;
#77586=ORIENTED_EDGE('',*,*,#49415,.F.) ;
#77587=ORIENTED_EDGE('',*,*,#53668,.T.) ;
#77588=ORIENTED_EDGE('',*,*,#53662,.T.) ;
#77589=ORIENTED_EDGE('',*,*,#51308,.F.) ;
#77590=ORIENTED_EDGE('',*,*,#53669,.F.) ;
#77591=ORIENTED_EDGE('',*,*,#51477,.F.) ;
#77592=ORIENTED_EDGE('',*,*,#53664,.T.) ;
#77593=ORIENTED_EDGE('',*,*,#51478,.F.) ;
#77594=ORIENTED_EDGE('',*,*,#53670,.F.) ;
#77595=ORIENTED_EDGE('',*,*,#49597,.F.) ;
#77596=ORIENTED_EDGE('',*,*,#53663,.T.) ;
#77597=ORIENTED_EDGE('',*,*,#49603,.F.) ;
#77598=ORIENTED_EDGE('',*,*,#53671,.F.) ;
#77599=ORIENTED_EDGE('',*,*,#51482,.F.) ;
#77600=ORIENTED_EDGE('',*,*,#53666,.T.) ;
#77601=ORIENTED_EDGE('',*,*,#51483,.F.) ;
#77602=ORIENTED_EDGE('',*,*,#53672,.F.) ;
#77603=ORIENTED_EDGE('',*,*,#51473,.F.) ;
#77604=ORIENTED_EDGE('',*,*,#53665,.T.) ;
#77605=ORIENTED_EDGE('',*,*,#51476,.F.) ;
#77606=ORIENTED_EDGE('',*,*,#53673,.F.) ;
#77607=ORIENTED_EDGE('',*,*,#51487,.F.) ;
#77608=ORIENTED_EDGE('',*,*,#51319,.F.) ;
#77609=ORIENTED_EDGE('',*,*,#53674,.T.) ;
#77610=ORIENTED_EDGE('',*,*,#51488,.F.) ;
#77611=ORIENTED_EDGE('',*,*,#53675,.F.) ;
#77612=ORIENTED_EDGE('',*,*,#53669,.T.) ;
#77613=ORIENTED_EDGE('',*,*,#51307,.T.) ;
#77614=ORIENTED_EDGE('',*,*,#53676,.F.) ;
#77615=ORIENTED_EDGE('',*,*,#53670,.T.) ;
#77616=ORIENTED_EDGE('',*,*,#53671,.T.) ;
#77617=ORIENTED_EDGE('',*,*,#49602,.T.) ;
#77618=ORIENTED_EDGE('',*,*,#53677,.F.) ;
#77619=ORIENTED_EDGE('',*,*,#53672,.T.) ;
#77620=ORIENTED_EDGE('',*,*,#53675,.T.) ;
#77621=ORIENTED_EDGE('',*,*,#53673,.T.) ;
#77622=ORIENTED_EDGE('',*,*,#53678,.F.) ;
#77623=ORIENTED_EDGE('',*,*,#51303,.F.) ;
#77624=ORIENTED_EDGE('',*,*,#53679,.T.) ;
#77625=ORIENTED_EDGE('',*,*,#51297,.F.) ;
#77626=ORIENTED_EDGE('',*,*,#53680,.F.) ;
#77627=ORIENTED_EDGE('',*,*,#53676,.T.) ;
#77628=ORIENTED_EDGE('',*,*,#51306,.F.) ;
#77629=ORIENTED_EDGE('',*,*,#53681,.F.) ;
#77630=ORIENTED_EDGE('',*,*,#49598,.F.) ;
#77631=ORIENTED_EDGE('',*,*,#53677,.T.) ;
#77632=ORIENTED_EDGE('',*,*,#49601,.F.) ;
#77633=ORIENTED_EDGE('',*,*,#53682,.F.) ;
#77634=ORIENTED_EDGE('',*,*,#51474,.F.) ;
#77635=ORIENTED_EDGE('',*,*,#53678,.T.) ;
#77636=ORIENTED_EDGE('',*,*,#51475,.F.) ;
#77637=ORIENTED_EDGE('',*,*,#53683,.F.) ;
#77638=ORIENTED_EDGE('',*,*,#51320,.F.) ;
#77639=ORIENTED_EDGE('',*,*,#53680,.T.) ;
#77640=ORIENTED_EDGE('',*,*,#53550,.F.) ;
#77641=ORIENTED_EDGE('',*,*,#53684,.F.) ;
#77642=ORIENTED_EDGE('',*,*,#53685,.F.) ;
#77643=ORIENTED_EDGE('',*,*,#53681,.T.) ;
#77644=ORIENTED_EDGE('',*,*,#53686,.F.) ;
#77645=ORIENTED_EDGE('',*,*,#53683,.T.) ;
#77646=ORIENTED_EDGE('',*,*,#53682,.T.) ;
#77647=ORIENTED_EDGE('',*,*,#53687,.F.) ;
#77648=ORIENTED_EDGE('',*,*,#51321,.T.) ;
#77649=ORIENTED_EDGE('',*,*,#53684,.T.) ;
#77650=ORIENTED_EDGE('',*,*,#49679,.F.) ;
#77651=ORIENTED_EDGE('',*,*,#53688,.F.) ;
#77652=ORIENTED_EDGE('',*,*,#51304,.F.) ;
#77653=ORIENTED_EDGE('',*,*,#53686,.T.) ;
#77654=ORIENTED_EDGE('',*,*,#51305,.F.) ;
#77655=ORIENTED_EDGE('',*,*,#53689,.F.) ;
#77656=ORIENTED_EDGE('',*,*,#51311,.F.) ;
#77657=ORIENTED_EDGE('',*,*,#53685,.T.) ;
#77658=ORIENTED_EDGE('',*,*,#51314,.F.) ;
#77659=ORIENTED_EDGE('',*,*,#53690,.F.) ;
#77660=ORIENTED_EDGE('',*,*,#49599,.F.) ;
#77661=ORIENTED_EDGE('',*,*,#53687,.T.) ;
#77662=ORIENTED_EDGE('',*,*,#49600,.F.) ;
#77663=ORIENTED_EDGE('',*,*,#53691,.F.) ;
#77664=ORIENTED_EDGE('',*,*,#51322,.F.) ;
#77665=ORIENTED_EDGE('',*,*,#53688,.T.) ;
#77666=ORIENTED_EDGE('',*,*,#49678,.T.) ;
#77667=ORIENTED_EDGE('',*,*,#53692,.F.) ;
#77668=ORIENTED_EDGE('',*,*,#53689,.T.) ;
#77669=ORIENTED_EDGE('',*,*,#53691,.T.) ;
#77670=ORIENTED_EDGE('',*,*,#53690,.T.) ;
#77671=ORIENTED_EDGE('',*,*,#53693,.F.) ;
#77672=ORIENTED_EDGE('',*,*,#53692,.T.) ;
#77673=ORIENTED_EDGE('',*,*,#49677,.F.) ;
#77674=ORIENTED_EDGE('',*,*,#53694,.F.) ;
#77675=ORIENTED_EDGE('',*,*,#51312,.F.) ;
#77676=ORIENTED_EDGE('',*,*,#53693,.T.) ;
#77677=ORIENTED_EDGE('',*,*,#51313,.F.) ;
#77678=ORIENTED_EDGE('',*,*,#53695,.F.) ;
#77679=ORIENTED_EDGE('',*,*,#51323,.F.) ;
#77680=ORIENTED_EDGE('',*,*,#51328,.F.) ;
#77681=ORIENTED_EDGE('',*,*,#53696,.T.) ;
#77682=ORIENTED_EDGE('',*,*,#51315,.F.) ;
#77683=ORIENTED_EDGE('',*,*,#53697,.F.) ;
#77684=ORIENTED_EDGE('',*,*,#49674,.F.) ;
#77685=ORIENTED_EDGE('',*,*,#53698,.T.) ;
#77686=ORIENTED_EDGE('',*,*,#51325,.F.) ;
#77687=ORIENTED_EDGE('',*,*,#53699,.F.) ;
#77688=ORIENTED_EDGE('',*,*,#53694,.T.) ;
#77689=ORIENTED_EDGE('',*,*,#49676,.T.) ;
#77690=ORIENTED_EDGE('',*,*,#53700,.F.) ;
#77691=ORIENTED_EDGE('',*,*,#53695,.T.) ;
#77692=ORIENTED_EDGE('',*,*,#53699,.T.) ;
#77693=ORIENTED_EDGE('',*,*,#53697,.T.) ;
#77694=ORIENTED_EDGE('',*,*,#53701,.F.) ;
#77695=ORIENTED_EDGE('',*,*,#53700,.T.) ;
#77696=ORIENTED_EDGE('',*,*,#49675,.F.) ;
#77697=ORIENTED_EDGE('',*,*,#53701,.T.) ;
#77698=ORIENTED_EDGE('',*,*,#51324,.F.) ;
#77699=ORIENTED_EDGE('',*,*,#52262,.F.) ;
#77700=ORIENTED_EDGE('',*,*,#52273,.F.) ;
#77701=ORIENTED_EDGE('',*,*,#52272,.F.) ;
#77702=ORIENTED_EDGE('',*,*,#53702,.F.) ;
#77703=ORIENTED_EDGE('',*,*,#52263,.F.) ;
#77704=ORIENTED_EDGE('',*,*,#53702,.T.) ;
#77705=ORIENTED_EDGE('',*,*,#50696,.F.) ;
#77706=ORIENTED_EDGE('',*,*,#53703,.F.) ;
#77707=ORIENTED_EDGE('',*,*,#50682,.F.) ;
#77708=ORIENTED_EDGE('',*,*,#52270,.F.) ;
#77709=ORIENTED_EDGE('',*,*,#52269,.F.) ;
#77710=ORIENTED_EDGE('',*,*,#52268,.F.) ;
#77711=ORIENTED_EDGE('',*,*,#53704,.F.) ;
#77712=ORIENTED_EDGE('',*,*,#52271,.F.) ;
#77713=ORIENTED_EDGE('',*,*,#53705,.F.) ;
#77714=ORIENTED_EDGE('',*,*,#53703,.T.) ;
#77715=ORIENTED_EDGE('',*,*,#53706,.F.) ;
#77716=ORIENTED_EDGE('',*,*,#52260,.F.) ;
#77717=ORIENTED_EDGE('',*,*,#52265,.F.) ;
#77718=ORIENTED_EDGE('',*,*,#52264,.F.) ;
#77719=ORIENTED_EDGE('',*,*,#53707,.F.) ;
#77720=ORIENTED_EDGE('',*,*,#52261,.F.) ;
#77721=ORIENTED_EDGE('',*,*,#53704,.T.) ;
#77722=ORIENTED_EDGE('',*,*,#50692,.F.) ;
#77723=ORIENTED_EDGE('',*,*,#53708,.F.) ;
#77724=ORIENTED_EDGE('',*,*,#50694,.F.) ;
#77725=ORIENTED_EDGE('',*,*,#53706,.T.) ;
#77726=ORIENTED_EDGE('',*,*,#50695,.F.) ;
#77727=ORIENTED_EDGE('',*,*,#53709,.F.) ;
#77728=ORIENTED_EDGE('',*,*,#51020,.F.) ;
#77729=ORIENTED_EDGE('',*,*,#53705,.T.) ;
#77730=ORIENTED_EDGE('',*,*,#51019,.F.) ;
#77731=ORIENTED_EDGE('',*,*,#53710,.F.) ;
#77732=ORIENTED_EDGE('',*,*,#50683,.F.) ;
#77733=ORIENTED_EDGE('',*,*,#53707,.T.) ;
#77734=ORIENTED_EDGE('',*,*,#50684,.F.) ;
#77735=ORIENTED_EDGE('',*,*,#53711,.F.) ;
#77736=ORIENTED_EDGE('',*,*,#50688,.F.) ;
#77737=ORIENTED_EDGE('',*,*,#53709,.T.) ;
#77738=ORIENTED_EDGE('',*,*,#53708,.T.) ;
#77739=ORIENTED_EDGE('',*,*,#53712,.F.) ;
#77740=ORIENTED_EDGE('',*,*,#53711,.T.) ;
#77741=ORIENTED_EDGE('',*,*,#53710,.T.) ;
#77742=ORIENTED_EDGE('',*,*,#53713,.F.) ;
#77743=ORIENTED_EDGE('',*,*,#53712,.T.) ;
#77744=ORIENTED_EDGE('',*,*,#50691,.F.) ;
#77745=ORIENTED_EDGE('',*,*,#53714,.F.) ;
#77746=ORIENTED_EDGE('',*,*,#51017,.F.) ;
#77747=ORIENTED_EDGE('',*,*,#53713,.T.) ;
#77748=ORIENTED_EDGE('',*,*,#51018,.F.) ;
#77749=ORIENTED_EDGE('',*,*,#53715,.F.) ;
#77750=ORIENTED_EDGE('',*,*,#50685,.F.) ;
#77751=ORIENTED_EDGE('',*,*,#53715,.T.) ;
#77752=ORIENTED_EDGE('',*,*,#53714,.T.) ;
#77753=ORIENTED_EDGE('',*,*,#53716,.F.) ;
#77754=ORIENTED_EDGE('',*,*,#53716,.T.) ;
#77755=ORIENTED_EDGE('',*,*,#50690,.F.) ;
#77756=ORIENTED_EDGE('',*,*,#53717,.F.) ;
#77757=ORIENTED_EDGE('',*,*,#50686,.F.) ;
#77758=ORIENTED_EDGE('',*,*,#52266,.F.) ;
#77759=ORIENTED_EDGE('',*,*,#52259,.F.) ;
#77760=ORIENTED_EDGE('',*,*,#52258,.F.) ;
#77761=ORIENTED_EDGE('',*,*,#53717,.T.) ;
#77762=ORIENTED_EDGE('',*,*,#52267,.F.) ;
#77763=ORIENTED_EDGE('',*,*,#52563,.F.) ;
#77764=ORIENTED_EDGE('',*,*,#52562,.F.) ;
#77765=ORIENTED_EDGE('',*,*,#52561,.F.) ;
#77766=ORIENTED_EDGE('',*,*,#53718,.F.) ;
#77767=ORIENTED_EDGE('',*,*,#52564,.F.) ;
#77768=ORIENTED_EDGE('',*,*,#53718,.T.) ;
#77769=ORIENTED_EDGE('',*,*,#52560,.F.) ;
#77770=ORIENTED_EDGE('',*,*,#53719,.F.) ;
#77771=ORIENTED_EDGE('',*,*,#50614,.F.) ;
#77772=ORIENTED_EDGE('',*,*,#53719,.T.) ;
#77773=ORIENTED_EDGE('',*,*,#50382,.F.) ;
#77774=ORIENTED_EDGE('',*,*,#53720,.F.) ;
#77775=ORIENTED_EDGE('',*,*,#50615,.F.) ;
#77776=ORIENTED_EDGE('',*,*,#50370,.F.) ;
#77777=ORIENTED_EDGE('',*,*,#50616,.F.) ;
#77778=ORIENTED_EDGE('',*,*,#53721,.F.) ;
#77779=ORIENTED_EDGE('',*,*,#50376,.F.) ;
#77780=ORIENTED_EDGE('',*,*,#53721,.T.) ;
#77781=ORIENTED_EDGE('',*,*,#53720,.T.) ;
#77782=ORIENTED_EDGE('',*,*,#53722,.F.) ;
#77783=ORIENTED_EDGE('',*,*,#53722,.T.) ;
#77784=ORIENTED_EDGE('',*,*,#50381,.F.) ;
#77785=ORIENTED_EDGE('',*,*,#53723,.F.) ;
#77786=ORIENTED_EDGE('',*,*,#50377,.F.) ;
#77787=ORIENTED_EDGE('',*,*,#50372,.F.) ;
#77788=ORIENTED_EDGE('',*,*,#50378,.F.) ;
#77789=ORIENTED_EDGE('',*,*,#53724,.F.) ;
#77790=ORIENTED_EDGE('',*,*,#50678,.F.) ;
#77791=ORIENTED_EDGE('',*,*,#53724,.T.) ;
#77792=ORIENTED_EDGE('',*,*,#53723,.T.) ;
#77793=ORIENTED_EDGE('',*,*,#53725,.F.) ;
#77794=ORIENTED_EDGE('',*,*,#53725,.T.) ;
#77795=ORIENTED_EDGE('',*,*,#50380,.F.) ;
#77796=ORIENTED_EDGE('',*,*,#53726,.F.) ;
#77797=ORIENTED_EDGE('',*,*,#50679,.F.) ;
#77798=ORIENTED_EDGE('',*,*,#53726,.T.) ;
#77799=ORIENTED_EDGE('',*,*,#52559,.F.) ;
#77800=ORIENTED_EDGE('',*,*,#53727,.F.) ;
#77801=ORIENTED_EDGE('',*,*,#50680,.F.) ;
#77802=ORIENTED_EDGE('',*,*,#53727,.T.) ;
#77803=ORIENTED_EDGE('',*,*,#52558,.F.) ;
#77804=ORIENTED_EDGE('',*,*,#52567,.F.) ;
#77805=ORIENTED_EDGE('',*,*,#52568,.F.) ;
#77806=ORIENTED_EDGE('',*,*,#52573,.F.) ;
#77807=ORIENTED_EDGE('',*,*,#53728,.F.) ;
#77808=ORIENTED_EDGE('',*,*,#53728,.T.) ;
#77809=ORIENTED_EDGE('',*,*,#52572,.F.) ;
#77810=ORIENTED_EDGE('',*,*,#53729,.F.) ;
#77811=ORIENTED_EDGE('',*,*,#50675,.F.) ;
#77812=ORIENTED_EDGE('',*,*,#53729,.T.) ;
#77813=ORIENTED_EDGE('',*,*,#50364,.F.) ;
#77814=ORIENTED_EDGE('',*,*,#53730,.F.) ;
#77815=ORIENTED_EDGE('',*,*,#50676,.F.) ;
#77816=ORIENTED_EDGE('',*,*,#50374,.F.) ;
#77817=ORIENTED_EDGE('',*,*,#50677,.F.) ;
#77818=ORIENTED_EDGE('',*,*,#53731,.F.) ;
#77819=ORIENTED_EDGE('',*,*,#50368,.F.) ;
#77820=ORIENTED_EDGE('',*,*,#53731,.T.) ;
#77821=ORIENTED_EDGE('',*,*,#53730,.T.) ;
#77822=ORIENTED_EDGE('',*,*,#53732,.F.) ;
#77823=ORIENTED_EDGE('',*,*,#53732,.T.) ;
#77824=ORIENTED_EDGE('',*,*,#50363,.F.) ;
#77825=ORIENTED_EDGE('',*,*,#53733,.F.) ;
#77826=ORIENTED_EDGE('',*,*,#50365,.F.) ;
#77827=ORIENTED_EDGE('',*,*,#50375,.F.) ;
#77828=ORIENTED_EDGE('',*,*,#50366,.F.) ;
#77829=ORIENTED_EDGE('',*,*,#53734,.F.) ;
#77830=ORIENTED_EDGE('',*,*,#50617,.F.) ;
#77831=ORIENTED_EDGE('',*,*,#53734,.T.) ;
#77832=ORIENTED_EDGE('',*,*,#53733,.T.) ;
#77833=ORIENTED_EDGE('',*,*,#53735,.F.) ;
#77834=ORIENTED_EDGE('',*,*,#53735,.T.) ;
#77835=ORIENTED_EDGE('',*,*,#50362,.F.) ;
#77836=ORIENTED_EDGE('',*,*,#53736,.F.) ;
#77837=ORIENTED_EDGE('',*,*,#50618,.F.) ;
#77838=ORIENTED_EDGE('',*,*,#53736,.T.) ;
#77839=ORIENTED_EDGE('',*,*,#52571,.F.) ;
#77840=ORIENTED_EDGE('',*,*,#53737,.F.) ;
#77841=ORIENTED_EDGE('',*,*,#50619,.F.) ;
#77842=ORIENTED_EDGE('',*,*,#52569,.F.) ;
#77843=ORIENTED_EDGE('',*,*,#52566,.F.) ;
#77844=ORIENTED_EDGE('',*,*,#52565,.F.) ;
#77845=ORIENTED_EDGE('',*,*,#53737,.T.) ;
#77846=ORIENTED_EDGE('',*,*,#52570,.F.) ;
#77847=ORIENTED_EDGE('',*,*,#53738,.F.) ;
#77848=ORIENTED_EDGE('',*,*,#49424,.F.) ;
#77849=ORIENTED_EDGE('',*,*,#53739,.F.) ;
#77850=ORIENTED_EDGE('',*,*,#52181,.F.) ;
#77851=ORIENTED_EDGE('',*,*,#53739,.T.) ;
#77852=ORIENTED_EDGE('',*,*,#49423,.F.) ;
#77853=ORIENTED_EDGE('',*,*,#53740,.F.) ;
#77854=ORIENTED_EDGE('',*,*,#52184,.F.) ;
#77855=ORIENTED_EDGE('',*,*,#53738,.T.) ;
#77856=ORIENTED_EDGE('',*,*,#52178,.F.) ;
#77857=ORIENTED_EDGE('',*,*,#53741,.F.) ;
#77858=ORIENTED_EDGE('',*,*,#49425,.F.) ;
#77859=ORIENTED_EDGE('',*,*,#53740,.T.) ;
#77860=ORIENTED_EDGE('',*,*,#49422,.F.) ;
#77861=ORIENTED_EDGE('',*,*,#53742,.F.) ;
#77862=ORIENTED_EDGE('',*,*,#52187,.F.) ;
#77863=ORIENTED_EDGE('',*,*,#53741,.T.) ;
#77864=ORIENTED_EDGE('',*,*,#52175,.F.) ;
#77865=ORIENTED_EDGE('',*,*,#53743,.F.) ;
#77866=ORIENTED_EDGE('',*,*,#49426,.F.) ;
#77867=ORIENTED_EDGE('',*,*,#53742,.T.) ;
#77868=ORIENTED_EDGE('',*,*,#49421,.F.) ;
#77869=ORIENTED_EDGE('',*,*,#53744,.F.) ;
#77870=ORIENTED_EDGE('',*,*,#52190,.F.) ;
#77871=ORIENTED_EDGE('',*,*,#53743,.T.) ;
#77872=ORIENTED_EDGE('',*,*,#52197,.F.) ;
#77873=ORIENTED_EDGE('',*,*,#53745,.F.) ;
#77874=ORIENTED_EDGE('',*,*,#49419,.F.) ;
#77875=ORIENTED_EDGE('',*,*,#53744,.T.) ;
#77876=ORIENTED_EDGE('',*,*,#49420,.F.) ;
#77877=ORIENTED_EDGE('',*,*,#53745,.T.) ;
#77878=ORIENTED_EDGE('',*,*,#52193,.F.) ;
#77879=ORIENTED_EDGE('',*,*,#51026,.F.) ;
#77880=ORIENTED_EDGE('',*,*,#51040,.F.) ;
#77881=ORIENTED_EDGE('',*,*,#53746,.F.) ;
#77882=ORIENTED_EDGE('',*,*,#51029,.F.) ;
#77883=ORIENTED_EDGE('',*,*,#53747,.F.) ;
#77884=ORIENTED_EDGE('',*,*,#51030,.F.) ;
#77885=ORIENTED_EDGE('',*,*,#53748,.F.) ;
#77886=ORIENTED_EDGE('',*,*,#51076,.F.) ;
#77887=ORIENTED_EDGE('',*,*,#51028,.F.) ;
#77888=ORIENTED_EDGE('',*,*,#51031,.F.) ;
#77889=ORIENTED_EDGE('',*,*,#53749,.F.) ;
#77890=ORIENTED_EDGE('',*,*,#51032,.F.) ;
#77891=ORIENTED_EDGE('',*,*,#53748,.T.) ;
#77892=ORIENTED_EDGE('',*,*,#53746,.T.) ;
#77893=ORIENTED_EDGE('',*,*,#53750,.F.) ;
#77894=ORIENTED_EDGE('',*,*,#53749,.T.) ;
#77895=ORIENTED_EDGE('',*,*,#53747,.T.) ;
#77896=ORIENTED_EDGE('',*,*,#53751,.F.) ;
#77897=ORIENTED_EDGE('',*,*,#51024,.F.) ;
#77898=ORIENTED_EDGE('',*,*,#51036,.F.) ;
#77899=ORIENTED_EDGE('',*,*,#53752,.F.) ;
#77900=ORIENTED_EDGE('',*,*,#51038,.F.) ;
#77901=ORIENTED_EDGE('',*,*,#53750,.T.) ;
#77902=ORIENTED_EDGE('',*,*,#51039,.F.) ;
#77903=ORIENTED_EDGE('',*,*,#53753,.F.) ;
#77904=ORIENTED_EDGE('',*,*,#51073,.F.) ;
#77905=ORIENTED_EDGE('',*,*,#53751,.T.) ;
#77906=ORIENTED_EDGE('',*,*,#51075,.F.) ;
#77907=ORIENTED_EDGE('',*,*,#53754,.F.) ;
#77908=ORIENTED_EDGE('',*,*,#51033,.F.) ;
#77909=ORIENTED_EDGE('',*,*,#51022,.F.) ;
#77910=ORIENTED_EDGE('',*,*,#51034,.F.) ;
#77911=ORIENTED_EDGE('',*,*,#53755,.F.) ;
#77912=ORIENTED_EDGE('',*,*,#51037,.F.) ;
#77913=ORIENTED_EDGE('',*,*,#53753,.T.) ;
#77914=ORIENTED_EDGE('',*,*,#53752,.T.) ;
#77915=ORIENTED_EDGE('',*,*,#53756,.F.) ;
#77916=ORIENTED_EDGE('',*,*,#53755,.T.) ;
#77917=ORIENTED_EDGE('',*,*,#53754,.T.) ;
#77918=ORIENTED_EDGE('',*,*,#53757,.F.) ;
#77919=ORIENTED_EDGE('',*,*,#53756,.T.) ;
#77920=ORIENTED_EDGE('',*,*,#51035,.F.) ;
#77921=ORIENTED_EDGE('',*,*,#53757,.T.) ;
#77922=ORIENTED_EDGE('',*,*,#51074,.F.) ;
#77923=ORIENTED_EDGE('',*,*,#53758,.F.) ;
#77924=ORIENTED_EDGE('',*,*,#49412,.F.) ;
#77925=ORIENTED_EDGE('',*,*,#53759,.F.) ;
#77926=ORIENTED_EDGE('',*,*,#51505,.F.) ;
#77927=ORIENTED_EDGE('',*,*,#53759,.T.) ;
#77928=ORIENTED_EDGE('',*,*,#49411,.T.) ;
#77929=ORIENTED_EDGE('',*,*,#53760,.F.) ;
#77930=ORIENTED_EDGE('',*,*,#53761,.F.) ;
#77931=ORIENTED_EDGE('',*,*,#49413,.T.) ;
#77932=ORIENTED_EDGE('',*,*,#53758,.T.) ;
#77933=ORIENTED_EDGE('',*,*,#53762,.F.) ;
#77934=ORIENTED_EDGE('',*,*,#53763,.F.) ;
#77935=ORIENTED_EDGE('',*,*,#53760,.T.) ;
#77936=ORIENTED_EDGE('',*,*,#49410,.F.) ;
#77937=ORIENTED_EDGE('',*,*,#53764,.F.) ;
#77938=ORIENTED_EDGE('',*,*,#51502,.F.) ;
#77939=ORIENTED_EDGE('',*,*,#53761,.T.) ;
#77940=ORIENTED_EDGE('',*,*,#51501,.F.) ;
#77941=ORIENTED_EDGE('',*,*,#53765,.F.) ;
#77942=ORIENTED_EDGE('',*,*,#51506,.F.) ;
#77943=ORIENTED_EDGE('',*,*,#53766,.F.) ;
#77944=ORIENTED_EDGE('',*,*,#51503,.F.) ;
#77945=ORIENTED_EDGE('',*,*,#53767,.F.) ;
#77946=ORIENTED_EDGE('',*,*,#51830,.F.) ;
#77947=ORIENTED_EDGE('',*,*,#53762,.T.) ;
#77948=ORIENTED_EDGE('',*,*,#51504,.F.) ;
#77949=ORIENTED_EDGE('',*,*,#53768,.F.) ;
#77950=ORIENTED_EDGE('',*,*,#51494,.F.) ;
#77951=ORIENTED_EDGE('',*,*,#53763,.T.) ;
#77952=ORIENTED_EDGE('',*,*,#51493,.F.) ;
#77953=ORIENTED_EDGE('',*,*,#53769,.F.) ;
#77954=ORIENTED_EDGE('',*,*,#49414,.F.) ;
#77955=ORIENTED_EDGE('',*,*,#53770,.F.) ;
#77956=ORIENTED_EDGE('',*,*,#49408,.F.) ;
#77957=ORIENTED_EDGE('',*,*,#53771,.F.) ;
#77958=ORIENTED_EDGE('',*,*,#51495,.F.) ;
#77959=ORIENTED_EDGE('',*,*,#49409,.T.) ;
#77960=ORIENTED_EDGE('',*,*,#53770,.T.) ;
#77961=ORIENTED_EDGE('',*,*,#53772,.F.) ;
#77962=ORIENTED_EDGE('',*,*,#53764,.T.) ;
#77963=ORIENTED_EDGE('',*,*,#53767,.T.) ;
#77964=ORIENTED_EDGE('',*,*,#53765,.T.) ;
#77965=ORIENTED_EDGE('',*,*,#53773,.F.) ;
#77966=ORIENTED_EDGE('',*,*,#53768,.T.) ;
#77967=ORIENTED_EDGE('',*,*,#53766,.T.) ;
#77968=ORIENTED_EDGE('',*,*,#53774,.F.) ;
#77969=ORIENTED_EDGE('',*,*,#49407,.T.) ;
#77970=ORIENTED_EDGE('',*,*,#53769,.T.) ;
#77971=ORIENTED_EDGE('',*,*,#53775,.F.) ;
#77972=ORIENTED_EDGE('',*,*,#53771,.T.) ;
#77973=ORIENTED_EDGE('',*,*,#53772,.T.) ;
#77974=ORIENTED_EDGE('',*,*,#51498,.F.) ;
#77975=ORIENTED_EDGE('',*,*,#53776,.F.) ;
#77976=ORIENTED_EDGE('',*,*,#51499,.F.) ;
#77977=ORIENTED_EDGE('',*,*,#53773,.T.) ;
#77978=ORIENTED_EDGE('',*,*,#51500,.F.) ;
#77979=ORIENTED_EDGE('',*,*,#53777,.F.) ;
#77980=ORIENTED_EDGE('',*,*,#51827,.F.) ;
#77981=ORIENTED_EDGE('',*,*,#53774,.T.) ;
#77982=ORIENTED_EDGE('',*,*,#51829,.F.) ;
#77983=ORIENTED_EDGE('',*,*,#53778,.F.) ;
#77984=ORIENTED_EDGE('',*,*,#51491,.F.) ;
#77985=ORIENTED_EDGE('',*,*,#53775,.T.) ;
#77986=ORIENTED_EDGE('',*,*,#51492,.F.) ;
#77987=ORIENTED_EDGE('',*,*,#53779,.F.) ;
#77988=ORIENTED_EDGE('',*,*,#51496,.F.) ;
#77989=ORIENTED_EDGE('',*,*,#53777,.T.) ;
#77990=ORIENTED_EDGE('',*,*,#53776,.T.) ;
#77991=ORIENTED_EDGE('',*,*,#53780,.F.) ;
#77992=ORIENTED_EDGE('',*,*,#53779,.T.) ;
#77993=ORIENTED_EDGE('',*,*,#53778,.T.) ;
#77994=ORIENTED_EDGE('',*,*,#53781,.F.) ;
#77995=ORIENTED_EDGE('',*,*,#53780,.T.) ;
#77996=ORIENTED_EDGE('',*,*,#51497,.F.) ;
#77997=ORIENTED_EDGE('',*,*,#53781,.T.) ;
#77998=ORIENTED_EDGE('',*,*,#51828,.F.) ;
#77999=ORIENTED_EDGE('',*,*,#51836,.F.) ;
#78000=ORIENTED_EDGE('',*,*,#51849,.F.) ;
#78001=ORIENTED_EDGE('',*,*,#53782,.F.) ;
#78002=ORIENTED_EDGE('',*,*,#51841,.F.) ;
#78003=ORIENTED_EDGE('',*,*,#53783,.F.) ;
#78004=ORIENTED_EDGE('',*,*,#51839,.F.) ;
#78005=ORIENTED_EDGE('',*,*,#53784,.F.) ;
#78006=ORIENTED_EDGE('',*,*,#51886,.F.) ;
#78007=ORIENTED_EDGE('',*,*,#51838,.F.) ;
#78008=ORIENTED_EDGE('',*,*,#51840,.F.) ;
#78009=ORIENTED_EDGE('',*,*,#53785,.F.) ;
#78010=ORIENTED_EDGE('',*,*,#51844,.F.) ;
#78011=ORIENTED_EDGE('',*,*,#53784,.T.) ;
#78012=ORIENTED_EDGE('',*,*,#53782,.T.) ;
#78013=ORIENTED_EDGE('',*,*,#53786,.F.) ;
#78014=ORIENTED_EDGE('',*,*,#53785,.T.) ;
#78015=ORIENTED_EDGE('',*,*,#53783,.T.) ;
#78016=ORIENTED_EDGE('',*,*,#53787,.F.) ;
#78017=ORIENTED_EDGE('',*,*,#51834,.F.) ;
#78018=ORIENTED_EDGE('',*,*,#51847,.F.) ;
#78019=ORIENTED_EDGE('',*,*,#53788,.F.) ;
#78020=ORIENTED_EDGE('',*,*,#51850,.F.) ;
#78021=ORIENTED_EDGE('',*,*,#53786,.T.) ;
#78022=ORIENTED_EDGE('',*,*,#51848,.F.) ;
#78023=ORIENTED_EDGE('',*,*,#53789,.F.) ;
#78024=ORIENTED_EDGE('',*,*,#51883,.F.) ;
#78025=ORIENTED_EDGE('',*,*,#53787,.T.) ;
#78026=ORIENTED_EDGE('',*,*,#51885,.F.) ;
#78027=ORIENTED_EDGE('',*,*,#53790,.F.) ;
#78028=ORIENTED_EDGE('',*,*,#51842,.F.) ;
#78029=ORIENTED_EDGE('',*,*,#51832,.F.) ;
#78030=ORIENTED_EDGE('',*,*,#51843,.F.) ;
#78031=ORIENTED_EDGE('',*,*,#53791,.F.) ;
#78032=ORIENTED_EDGE('',*,*,#51845,.F.) ;
#78033=ORIENTED_EDGE('',*,*,#53789,.T.) ;
#78034=ORIENTED_EDGE('',*,*,#53788,.T.) ;
#78035=ORIENTED_EDGE('',*,*,#53792,.F.) ;
#78036=ORIENTED_EDGE('',*,*,#53791,.T.) ;
#78037=ORIENTED_EDGE('',*,*,#53790,.T.) ;
#78038=ORIENTED_EDGE('',*,*,#53793,.F.) ;
#78039=ORIENTED_EDGE('',*,*,#53792,.T.) ;
#78040=ORIENTED_EDGE('',*,*,#51846,.F.) ;
#78041=ORIENTED_EDGE('',*,*,#53793,.T.) ;
#78042=ORIENTED_EDGE('',*,*,#51884,.F.) ;
#78043=ORIENTED_EDGE('',*,*,#53794,.F.) ;
#78044=ORIENTED_EDGE('',*,*,#52186,.F.) ;
#78045=ORIENTED_EDGE('',*,*,#53795,.F.) ;
#78046=ORIENTED_EDGE('',*,*,#52201,.F.) ;
#78047=ORIENTED_EDGE('',*,*,#53795,.T.) ;
#78048=ORIENTED_EDGE('',*,*,#52189,.F.) ;
#78049=ORIENTED_EDGE('',*,*,#53796,.F.) ;
#78050=ORIENTED_EDGE('',*,*,#52183,.F.) ;
#78051=ORIENTED_EDGE('',*,*,#53794,.T.) ;
#78052=ORIENTED_EDGE('',*,*,#53797,.F.) ;
#78053=ORIENTED_EDGE('',*,*,#53796,.T.) ;
#78054=ORIENTED_EDGE('',*,*,#52192,.F.) ;
#78055=ORIENTED_EDGE('',*,*,#53798,.F.) ;
#78056=ORIENTED_EDGE('',*,*,#52198,.F.) ;
#78057=ORIENTED_EDGE('',*,*,#53797,.T.) ;
#78058=ORIENTED_EDGE('',*,*,#52200,.F.) ;
#78059=ORIENTED_EDGE('',*,*,#53799,.F.) ;
#78060=ORIENTED_EDGE('',*,*,#52180,.F.) ;
#78061=ORIENTED_EDGE('',*,*,#53798,.T.) ;
#78062=ORIENTED_EDGE('',*,*,#52195,.F.) ;
#78063=ORIENTED_EDGE('',*,*,#53800,.F.) ;
#78064=ORIENTED_EDGE('',*,*,#52177,.F.) ;
#78065=ORIENTED_EDGE('',*,*,#53799,.T.) ;
#78066=ORIENTED_EDGE('',*,*,#53801,.F.) ;
#78067=ORIENTED_EDGE('',*,*,#53800,.T.) ;
#78068=ORIENTED_EDGE('',*,*,#52196,.F.) ;
#78069=ORIENTED_EDGE('',*,*,#53801,.T.) ;
#78070=ORIENTED_EDGE('',*,*,#52199,.F.) ;
#78071=ORIENTED_EDGE('',*,*,#49232,.F.) ;
#78072=ORIENTED_EDGE('',*,*,#51887,.F.) ;
#78073=ORIENTED_EDGE('',*,*,#49246,.F.) ;
#78074=ORIENTED_EDGE('',*,*,#51944,.F.) ;
#78075=ORIENTED_EDGE('',*,*,#49234,.F.) ;
#78076=ORIENTED_EDGE('',*,*,#51945,.F.) ;
#78077=ORIENTED_EDGE('',*,*,#49244,.F.) ;
#78078=ORIENTED_EDGE('',*,*,#51948,.F.) ;
#78079=ORIENTED_EDGE('',*,*,#49242,.F.) ;
#78080=ORIENTED_EDGE('',*,*,#51946,.F.) ;
#78081=ORIENTED_EDGE('',*,*,#49236,.F.) ;
#78082=ORIENTED_EDGE('',*,*,#51949,.F.) ;
#78083=ORIENTED_EDGE('',*,*,#49240,.F.) ;
#78084=ORIENTED_EDGE('',*,*,#49523,.F.) ;
#78085=ORIENTED_EDGE('',*,*,#49238,.F.) ;
#78086=ORIENTED_EDGE('',*,*,#51947,.F.) ;
#78087=ORIENTED_EDGE('',*,*,#49513,.F.) ;
#78088=ORIENTED_EDGE('',*,*,#53802,.T.) ;
#78089=ORIENTED_EDGE('',*,*,#49545,.F.) ;
#78090=ORIENTED_EDGE('',*,*,#53803,.T.) ;
#78091=ORIENTED_EDGE('',*,*,#49501,.F.) ;
#78092=ORIENTED_EDGE('',*,*,#53804,.T.) ;
#78093=ORIENTED_EDGE('',*,*,#49551,.F.) ;
#78094=ORIENTED_EDGE('',*,*,#53805,.T.) ;
#78095=ORIENTED_EDGE('',*,*,#49489,.F.) ;
#78096=ORIENTED_EDGE('',*,*,#53806,.T.) ;
#78097=ORIENTED_EDGE('',*,*,#49557,.F.) ;
#78098=ORIENTED_EDGE('',*,*,#53807,.T.) ;
#78099=ORIENTED_EDGE('',*,*,#49477,.F.) ;
#78100=ORIENTED_EDGE('',*,*,#53808,.T.) ;
#78101=ORIENTED_EDGE('',*,*,#49563,.F.) ;
#78102=ORIENTED_EDGE('',*,*,#53809,.T.) ;
#78103=ORIENTED_EDGE('',*,*,#49465,.F.) ;
#78104=ORIENTED_EDGE('',*,*,#53810,.T.) ;
#78105=ORIENTED_EDGE('',*,*,#49569,.F.) ;
#78106=ORIENTED_EDGE('',*,*,#53811,.T.) ;
#78107=ORIENTED_EDGE('',*,*,#49453,.F.) ;
#78108=ORIENTED_EDGE('',*,*,#53812,.T.) ;
#78109=ORIENTED_EDGE('',*,*,#49575,.F.) ;
#78110=ORIENTED_EDGE('',*,*,#53813,.T.) ;
#78111=ORIENTED_EDGE('',*,*,#49441,.F.) ;
#78112=ORIENTED_EDGE('',*,*,#53814,.T.) ;
#78113=ORIENTED_EDGE('',*,*,#49581,.F.) ;
#78114=ORIENTED_EDGE('',*,*,#53815,.T.) ;
#78115=ORIENTED_EDGE('',*,*,#49429,.F.) ;
#78116=ORIENTED_EDGE('',*,*,#53816,.T.) ;
#78117=ORIENTED_EDGE('',*,*,#49587,.F.) ;
#78118=ORIENTED_EDGE('',*,*,#53817,.T.) ;
#78119=ORIENTED_EDGE('',*,*,#49417,.F.) ;
#78120=ORIENTED_EDGE('',*,*,#53818,.T.) ;
#78121=ORIENTED_EDGE('',*,*,#49593,.F.) ;
#78122=ORIENTED_EDGE('',*,*,#53819,.T.) ;
#78123=ORIENTED_EDGE('',*,*,#53820,.F.) ;
#78124=ORIENTED_EDGE('',*,*,#53821,.T.) ;
#78125=ORIENTED_EDGE('',*,*,#49549,.F.) ;
#78126=ORIENTED_EDGE('',*,*,#53822,.T.) ;
#78127=ORIENTED_EDGE('',*,*,#53820,.T.) ;
#78128=ORIENTED_EDGE('',*,*,#49548,.F.) ;
#78129=ORIENTED_EDGE('',*,*,#53823,.F.) ;
#78130=ORIENTED_EDGE('',*,*,#53824,.F.) ;
#78131=ORIENTED_EDGE('',*,*,#51102,.F.) ;
#78132=ORIENTED_EDGE('',*,*,#49547,.F.) ;
#78133=ORIENTED_EDGE('',*,*,#53825,.T.) ;
#78134=ORIENTED_EDGE('',*,*,#53823,.T.) ;
#78135=ORIENTED_EDGE('',*,*,#49741,.T.) ;
#78136=ORIENTED_EDGE('',*,*,#53826,.T.) ;
#78137=ORIENTED_EDGE('',*,*,#49543,.F.) ;
#78138=ORIENTED_EDGE('',*,*,#53827,.F.) ;
#78139=ORIENTED_EDGE('',*,*,#53828,.T.) ;
#78140=ORIENTED_EDGE('',*,*,#49555,.F.) ;
#78141=ORIENTED_EDGE('',*,*,#53829,.T.) ;
#78142=ORIENTED_EDGE('',*,*,#53827,.T.) ;
#78143=ORIENTED_EDGE('',*,*,#49554,.F.) ;
#78144=ORIENTED_EDGE('',*,*,#53830,.F.) ;
#78145=ORIENTED_EDGE('',*,*,#53831,.F.) ;
#78146=ORIENTED_EDGE('',*,*,#51130,.F.) ;
#78147=ORIENTED_EDGE('',*,*,#49553,.F.) ;
#78148=ORIENTED_EDGE('',*,*,#53832,.T.) ;
#78149=ORIENTED_EDGE('',*,*,#53830,.T.) ;
#78150=ORIENTED_EDGE('',*,*,#53833,.F.) ;
#78151=ORIENTED_EDGE('',*,*,#53834,.T.) ;
#78152=ORIENTED_EDGE('',*,*,#49561,.F.) ;
#78153=ORIENTED_EDGE('',*,*,#53835,.T.) ;
#78154=ORIENTED_EDGE('',*,*,#53833,.T.) ;
#78155=ORIENTED_EDGE('',*,*,#49560,.F.) ;
#78156=ORIENTED_EDGE('',*,*,#53836,.F.) ;
#78157=ORIENTED_EDGE('',*,*,#53837,.F.) ;
#78158=ORIENTED_EDGE('',*,*,#51158,.F.) ;
#78159=ORIENTED_EDGE('',*,*,#49559,.F.) ;
#78160=ORIENTED_EDGE('',*,*,#53838,.T.) ;
#78161=ORIENTED_EDGE('',*,*,#53836,.T.) ;
#78162=ORIENTED_EDGE('',*,*,#53839,.F.) ;
#78163=ORIENTED_EDGE('',*,*,#53840,.T.) ;
#78164=ORIENTED_EDGE('',*,*,#49567,.F.) ;
#78165=ORIENTED_EDGE('',*,*,#53841,.T.) ;
#78166=ORIENTED_EDGE('',*,*,#53839,.T.) ;
#78167=ORIENTED_EDGE('',*,*,#49566,.F.) ;
#78168=ORIENTED_EDGE('',*,*,#53842,.F.) ;
#78169=ORIENTED_EDGE('',*,*,#53843,.F.) ;
#78170=ORIENTED_EDGE('',*,*,#51186,.F.) ;
#78171=ORIENTED_EDGE('',*,*,#49565,.F.) ;
#78172=ORIENTED_EDGE('',*,*,#53844,.T.) ;
#78173=ORIENTED_EDGE('',*,*,#53842,.T.) ;
#78174=ORIENTED_EDGE('',*,*,#53845,.F.) ;
#78175=ORIENTED_EDGE('',*,*,#53846,.T.) ;
#78176=ORIENTED_EDGE('',*,*,#49573,.F.) ;
#78177=ORIENTED_EDGE('',*,*,#53847,.T.) ;
#78178=ORIENTED_EDGE('',*,*,#53845,.T.) ;
#78179=ORIENTED_EDGE('',*,*,#49572,.F.) ;
#78180=ORIENTED_EDGE('',*,*,#53848,.F.) ;
#78181=ORIENTED_EDGE('',*,*,#53849,.F.) ;
#78182=ORIENTED_EDGE('',*,*,#51214,.F.) ;
#78183=ORIENTED_EDGE('',*,*,#49571,.F.) ;
#78184=ORIENTED_EDGE('',*,*,#53850,.T.) ;
#78185=ORIENTED_EDGE('',*,*,#53848,.T.) ;
#78186=ORIENTED_EDGE('',*,*,#53851,.F.) ;
#78187=ORIENTED_EDGE('',*,*,#53852,.T.) ;
#78188=ORIENTED_EDGE('',*,*,#49579,.F.) ;
#78189=ORIENTED_EDGE('',*,*,#53853,.T.) ;
#78190=ORIENTED_EDGE('',*,*,#53851,.T.) ;
#78191=ORIENTED_EDGE('',*,*,#49578,.F.) ;
#78192=ORIENTED_EDGE('',*,*,#53854,.F.) ;
#78193=ORIENTED_EDGE('',*,*,#53855,.F.) ;
#78194=ORIENTED_EDGE('',*,*,#51242,.F.) ;
#78195=ORIENTED_EDGE('',*,*,#49577,.F.) ;
#78196=ORIENTED_EDGE('',*,*,#53856,.T.) ;
#78197=ORIENTED_EDGE('',*,*,#53854,.T.) ;
#78198=ORIENTED_EDGE('',*,*,#53857,.F.) ;
#78199=ORIENTED_EDGE('',*,*,#53858,.T.) ;
#78200=ORIENTED_EDGE('',*,*,#49585,.F.) ;
#78201=ORIENTED_EDGE('',*,*,#53859,.T.) ;
#78202=ORIENTED_EDGE('',*,*,#53857,.T.) ;
#78203=ORIENTED_EDGE('',*,*,#49584,.F.) ;
#78204=ORIENTED_EDGE('',*,*,#53860,.F.) ;
#78205=ORIENTED_EDGE('',*,*,#53861,.F.) ;
#78206=ORIENTED_EDGE('',*,*,#51270,.F.) ;
#78207=ORIENTED_EDGE('',*,*,#49583,.F.) ;
#78208=ORIENTED_EDGE('',*,*,#53862,.T.) ;
#78209=ORIENTED_EDGE('',*,*,#53860,.T.) ;
#78210=ORIENTED_EDGE('',*,*,#53863,.F.) ;
#78211=ORIENTED_EDGE('',*,*,#53864,.T.) ;
#78212=ORIENTED_EDGE('',*,*,#49591,.F.) ;
#78213=ORIENTED_EDGE('',*,*,#53865,.T.) ;
#78214=ORIENTED_EDGE('',*,*,#53863,.T.) ;
#78215=ORIENTED_EDGE('',*,*,#49590,.F.) ;
#78216=ORIENTED_EDGE('',*,*,#53866,.F.) ;
#78217=ORIENTED_EDGE('',*,*,#53867,.F.) ;
#78218=ORIENTED_EDGE('',*,*,#51298,.F.) ;
#78219=ORIENTED_EDGE('',*,*,#49589,.F.) ;
#78220=ORIENTED_EDGE('',*,*,#53868,.T.) ;
#78221=ORIENTED_EDGE('',*,*,#53866,.T.) ;
#78222=ORIENTED_EDGE('',*,*,#51327,.F.) ;
#78223=ORIENTED_EDGE('',*,*,#53869,.T.) ;
#78224=ORIENTED_EDGE('',*,*,#49532,.F.) ;
#78225=ORIENTED_EDGE('',*,*,#53870,.F.) ;
#78226=ORIENTED_EDGE('',*,*,#53871,.F.) ;
#78227=ORIENTED_EDGE('',*,*,#49595,.F.) ;
#78228=ORIENTED_EDGE('',*,*,#53872,.T.) ;
#78229=ORIENTED_EDGE('',*,*,#53870,.T.) ;
#78230=ORIENTED_EDGE('',*,*,#51093,.F.) ;
#78231=ORIENTED_EDGE('',*,*,#53873,.T.) ;
#78232=ORIENTED_EDGE('',*,*,#53874,.F.) ;
#78233=ORIENTED_EDGE('',*,*,#53874,.T.) ;
#78234=ORIENTED_EDGE('',*,*,#53875,.T.) ;
#78235=ORIENTED_EDGE('',*,*,#49512,.F.) ;
#78236=ORIENTED_EDGE('',*,*,#53876,.F.) ;
#78237=ORIENTED_EDGE('',*,*,#51094,.F.) ;
#78238=ORIENTED_EDGE('',*,*,#52210,.F.) ;
#78239=ORIENTED_EDGE('',*,*,#52208,.F.) ;
#78240=ORIENTED_EDGE('',*,*,#53876,.T.) ;
#78241=ORIENTED_EDGE('',*,*,#53877,.F.) ;
#78242=ORIENTED_EDGE('',*,*,#53878,.T.) ;
#78243=ORIENTED_EDGE('',*,*,#51077,.F.) ;
#78244=ORIENTED_EDGE('',*,*,#53879,.T.) ;
#78245=ORIENTED_EDGE('',*,*,#53877,.T.) ;
#78246=ORIENTED_EDGE('',*,*,#51086,.F.) ;
#78247=ORIENTED_EDGE('',*,*,#53880,.F.) ;
#78248=ORIENTED_EDGE('',*,*,#49514,.F.) ;
#78249=ORIENTED_EDGE('',*,*,#52217,.F.) ;
#78250=ORIENTED_EDGE('',*,*,#52211,.F.) ;
#78251=ORIENTED_EDGE('',*,*,#53880,.T.) ;
#78252=ORIENTED_EDGE('',*,*,#51121,.F.) ;
#78253=ORIENTED_EDGE('',*,*,#53881,.T.) ;
#78254=ORIENTED_EDGE('',*,*,#53882,.F.) ;
#78255=ORIENTED_EDGE('',*,*,#53882,.T.) ;
#78256=ORIENTED_EDGE('',*,*,#53883,.T.) ;
#78257=ORIENTED_EDGE('',*,*,#49500,.F.) ;
#78258=ORIENTED_EDGE('',*,*,#53884,.F.) ;
#78259=ORIENTED_EDGE('',*,*,#51122,.F.) ;
#78260=ORIENTED_EDGE('',*,*,#53884,.T.) ;
#78261=ORIENTED_EDGE('',*,*,#52631,.F.) ;
#78262=ORIENTED_EDGE('',*,*,#52638,.F.) ;
#78263=ORIENTED_EDGE('',*,*,#53885,.F.) ;
#78264=ORIENTED_EDGE('',*,*,#53886,.T.) ;
#78265=ORIENTED_EDGE('',*,*,#51105,.F.) ;
#78266=ORIENTED_EDGE('',*,*,#53887,.T.) ;
#78267=ORIENTED_EDGE('',*,*,#53885,.T.) ;
#78268=ORIENTED_EDGE('',*,*,#51114,.F.) ;
#78269=ORIENTED_EDGE('',*,*,#53888,.F.) ;
#78270=ORIENTED_EDGE('',*,*,#49502,.F.) ;
#78271=ORIENTED_EDGE('',*,*,#53888,.T.) ;
#78272=ORIENTED_EDGE('',*,*,#52624,.F.) ;
#78273=ORIENTED_EDGE('',*,*,#52632,.F.) ;
#78274=ORIENTED_EDGE('',*,*,#51149,.F.) ;
#78275=ORIENTED_EDGE('',*,*,#53889,.T.) ;
#78276=ORIENTED_EDGE('',*,*,#53890,.F.) ;
#78277=ORIENTED_EDGE('',*,*,#53890,.T.) ;
#78278=ORIENTED_EDGE('',*,*,#53891,.T.) ;
#78279=ORIENTED_EDGE('',*,*,#49488,.F.) ;
#78280=ORIENTED_EDGE('',*,*,#53892,.F.) ;
#78281=ORIENTED_EDGE('',*,*,#51150,.F.) ;
#78282=ORIENTED_EDGE('',*,*,#53892,.T.) ;
#78283=ORIENTED_EDGE('',*,*,#52779,.F.) ;
#78284=ORIENTED_EDGE('',*,*,#52786,.F.) ;
#78285=ORIENTED_EDGE('',*,*,#53893,.F.) ;
#78286=ORIENTED_EDGE('',*,*,#53894,.T.) ;
#78287=ORIENTED_EDGE('',*,*,#51133,.F.) ;
#78288=ORIENTED_EDGE('',*,*,#53895,.T.) ;
#78289=ORIENTED_EDGE('',*,*,#53893,.T.) ;
#78290=ORIENTED_EDGE('',*,*,#51142,.F.) ;
#78291=ORIENTED_EDGE('',*,*,#53896,.F.) ;
#78292=ORIENTED_EDGE('',*,*,#49490,.F.) ;
#78293=ORIENTED_EDGE('',*,*,#53896,.T.) ;
#78294=ORIENTED_EDGE('',*,*,#52772,.F.) ;
#78295=ORIENTED_EDGE('',*,*,#52780,.F.) ;
#78296=ORIENTED_EDGE('',*,*,#51177,.F.) ;
#78297=ORIENTED_EDGE('',*,*,#53897,.T.) ;
#78298=ORIENTED_EDGE('',*,*,#53898,.F.) ;
#78299=ORIENTED_EDGE('',*,*,#53898,.T.) ;
#78300=ORIENTED_EDGE('',*,*,#53899,.T.) ;
#78301=ORIENTED_EDGE('',*,*,#49476,.F.) ;
#78302=ORIENTED_EDGE('',*,*,#53900,.F.) ;
#78303=ORIENTED_EDGE('',*,*,#51178,.F.) ;
#78304=ORIENTED_EDGE('',*,*,#53900,.T.) ;
#78305=ORIENTED_EDGE('',*,*,#52927,.F.) ;
#78306=ORIENTED_EDGE('',*,*,#52934,.F.) ;
#78307=ORIENTED_EDGE('',*,*,#53901,.F.) ;
#78308=ORIENTED_EDGE('',*,*,#53902,.T.) ;
#78309=ORIENTED_EDGE('',*,*,#51161,.F.) ;
#78310=ORIENTED_EDGE('',*,*,#53903,.T.) ;
#78311=ORIENTED_EDGE('',*,*,#53901,.T.) ;
#78312=ORIENTED_EDGE('',*,*,#51170,.F.) ;
#78313=ORIENTED_EDGE('',*,*,#53904,.F.) ;
#78314=ORIENTED_EDGE('',*,*,#49478,.F.) ;
#78315=ORIENTED_EDGE('',*,*,#53904,.T.) ;
#78316=ORIENTED_EDGE('',*,*,#52920,.F.) ;
#78317=ORIENTED_EDGE('',*,*,#52928,.F.) ;
#78318=ORIENTED_EDGE('',*,*,#51205,.F.) ;
#78319=ORIENTED_EDGE('',*,*,#53905,.T.) ;
#78320=ORIENTED_EDGE('',*,*,#53906,.F.) ;
#78321=ORIENTED_EDGE('',*,*,#53906,.T.) ;
#78322=ORIENTED_EDGE('',*,*,#53907,.T.) ;
#78323=ORIENTED_EDGE('',*,*,#49464,.F.) ;
#78324=ORIENTED_EDGE('',*,*,#53908,.F.) ;
#78325=ORIENTED_EDGE('',*,*,#51206,.F.) ;
#78326=ORIENTED_EDGE('',*,*,#53908,.T.) ;
#78327=ORIENTED_EDGE('',*,*,#53075,.F.) ;
#78328=ORIENTED_EDGE('',*,*,#53082,.F.) ;
#78329=ORIENTED_EDGE('',*,*,#53909,.F.) ;
#78330=ORIENTED_EDGE('',*,*,#53910,.T.) ;
#78331=ORIENTED_EDGE('',*,*,#51189,.F.) ;
#78332=ORIENTED_EDGE('',*,*,#53911,.T.) ;
#78333=ORIENTED_EDGE('',*,*,#53909,.T.) ;
#78334=ORIENTED_EDGE('',*,*,#51198,.F.) ;
#78335=ORIENTED_EDGE('',*,*,#53912,.F.) ;
#78336=ORIENTED_EDGE('',*,*,#49466,.F.) ;
#78337=ORIENTED_EDGE('',*,*,#53912,.T.) ;
#78338=ORIENTED_EDGE('',*,*,#53068,.F.) ;
#78339=ORIENTED_EDGE('',*,*,#53076,.F.) ;
#78340=ORIENTED_EDGE('',*,*,#51233,.F.) ;
#78341=ORIENTED_EDGE('',*,*,#53913,.T.) ;
#78342=ORIENTED_EDGE('',*,*,#53914,.F.) ;
#78343=ORIENTED_EDGE('',*,*,#53914,.T.) ;
#78344=ORIENTED_EDGE('',*,*,#53915,.T.) ;
#78345=ORIENTED_EDGE('',*,*,#49452,.F.) ;
#78346=ORIENTED_EDGE('',*,*,#53916,.F.) ;
#78347=ORIENTED_EDGE('',*,*,#51234,.F.) ;
#78348=ORIENTED_EDGE('',*,*,#53916,.T.) ;
#78349=ORIENTED_EDGE('',*,*,#53223,.F.) ;
#78350=ORIENTED_EDGE('',*,*,#53230,.F.) ;
#78351=ORIENTED_EDGE('',*,*,#53917,.F.) ;
#78352=ORIENTED_EDGE('',*,*,#53918,.T.) ;
#78353=ORIENTED_EDGE('',*,*,#51217,.F.) ;
#78354=ORIENTED_EDGE('',*,*,#53919,.T.) ;
#78355=ORIENTED_EDGE('',*,*,#53917,.T.) ;
#78356=ORIENTED_EDGE('',*,*,#51226,.F.) ;
#78357=ORIENTED_EDGE('',*,*,#53920,.F.) ;
#78358=ORIENTED_EDGE('',*,*,#49454,.F.) ;
#78359=ORIENTED_EDGE('',*,*,#53920,.T.) ;
#78360=ORIENTED_EDGE('',*,*,#53216,.F.) ;
#78361=ORIENTED_EDGE('',*,*,#53224,.F.) ;
#78362=ORIENTED_EDGE('',*,*,#51261,.F.) ;
#78363=ORIENTED_EDGE('',*,*,#53921,.T.) ;
#78364=ORIENTED_EDGE('',*,*,#53922,.F.) ;
#78365=ORIENTED_EDGE('',*,*,#53922,.T.) ;
#78366=ORIENTED_EDGE('',*,*,#53923,.T.) ;
#78367=ORIENTED_EDGE('',*,*,#49440,.F.) ;
#78368=ORIENTED_EDGE('',*,*,#53924,.F.) ;
#78369=ORIENTED_EDGE('',*,*,#51262,.F.) ;
#78370=ORIENTED_EDGE('',*,*,#53924,.T.) ;
#78371=ORIENTED_EDGE('',*,*,#53371,.F.) ;
#78372=ORIENTED_EDGE('',*,*,#53378,.F.) ;
#78373=ORIENTED_EDGE('',*,*,#53925,.F.) ;
#78374=ORIENTED_EDGE('',*,*,#53926,.T.) ;
#78375=ORIENTED_EDGE('',*,*,#51245,.F.) ;
#78376=ORIENTED_EDGE('',*,*,#53927,.T.) ;
#78377=ORIENTED_EDGE('',*,*,#53925,.T.) ;
#78378=ORIENTED_EDGE('',*,*,#51254,.F.) ;
#78379=ORIENTED_EDGE('',*,*,#53928,.F.) ;
#78380=ORIENTED_EDGE('',*,*,#49442,.F.) ;
#78381=ORIENTED_EDGE('',*,*,#53928,.T.) ;
#78382=ORIENTED_EDGE('',*,*,#53364,.F.) ;
#78383=ORIENTED_EDGE('',*,*,#53372,.F.) ;
#78384=ORIENTED_EDGE('',*,*,#51289,.F.) ;
#78385=ORIENTED_EDGE('',*,*,#53929,.T.) ;
#78386=ORIENTED_EDGE('',*,*,#53930,.F.) ;
#78387=ORIENTED_EDGE('',*,*,#53930,.T.) ;
#78388=ORIENTED_EDGE('',*,*,#53931,.T.) ;
#78389=ORIENTED_EDGE('',*,*,#49428,.F.) ;
#78390=ORIENTED_EDGE('',*,*,#53932,.F.) ;
#78391=ORIENTED_EDGE('',*,*,#51290,.F.) ;
#78392=ORIENTED_EDGE('',*,*,#53932,.T.) ;
#78393=ORIENTED_EDGE('',*,*,#53519,.F.) ;
#78394=ORIENTED_EDGE('',*,*,#53526,.F.) ;
#78395=ORIENTED_EDGE('',*,*,#53933,.F.) ;
#78396=ORIENTED_EDGE('',*,*,#53934,.T.) ;
#78397=ORIENTED_EDGE('',*,*,#51273,.F.) ;
#78398=ORIENTED_EDGE('',*,*,#53935,.T.) ;
#78399=ORIENTED_EDGE('',*,*,#53933,.T.) ;
#78400=ORIENTED_EDGE('',*,*,#51282,.F.) ;
#78401=ORIENTED_EDGE('',*,*,#53936,.F.) ;
#78402=ORIENTED_EDGE('',*,*,#49430,.F.) ;
#78403=ORIENTED_EDGE('',*,*,#53936,.T.) ;
#78404=ORIENTED_EDGE('',*,*,#53512,.F.) ;
#78405=ORIENTED_EDGE('',*,*,#53520,.F.) ;
#78406=ORIENTED_EDGE('',*,*,#51317,.F.) ;
#78407=ORIENTED_EDGE('',*,*,#53937,.T.) ;
#78408=ORIENTED_EDGE('',*,*,#53938,.F.) ;
#78409=ORIENTED_EDGE('',*,*,#53938,.T.) ;
#78410=ORIENTED_EDGE('',*,*,#53939,.T.) ;
#78411=ORIENTED_EDGE('',*,*,#49416,.F.) ;
#78412=ORIENTED_EDGE('',*,*,#53940,.F.) ;
#78413=ORIENTED_EDGE('',*,*,#51318,.F.) ;
#78414=ORIENTED_EDGE('',*,*,#53940,.T.) ;
#78415=ORIENTED_EDGE('',*,*,#53667,.F.) ;
#78416=ORIENTED_EDGE('',*,*,#53674,.F.) ;
#78417=ORIENTED_EDGE('',*,*,#53941,.F.) ;
#78418=ORIENTED_EDGE('',*,*,#53942,.T.) ;
#78419=ORIENTED_EDGE('',*,*,#51301,.F.) ;
#78420=ORIENTED_EDGE('',*,*,#53943,.T.) ;
#78421=ORIENTED_EDGE('',*,*,#53941,.T.) ;
#78422=ORIENTED_EDGE('',*,*,#51310,.F.) ;
#78423=ORIENTED_EDGE('',*,*,#53944,.F.) ;
#78424=ORIENTED_EDGE('',*,*,#49418,.F.) ;
#78425=ORIENTED_EDGE('',*,*,#53944,.T.) ;
#78426=ORIENTED_EDGE('',*,*,#53660,.F.) ;
#78427=ORIENTED_EDGE('',*,*,#53668,.F.) ;
#78428=ORIENTED_EDGE('',*,*,#53802,.F.) ;
#78429=ORIENTED_EDGE('',*,*,#53875,.F.) ;
#78430=ORIENTED_EDGE('',*,*,#53945,.F.) ;
#78431=ORIENTED_EDGE('',*,*,#49546,.F.) ;
#78432=ORIENTED_EDGE('',*,*,#53945,.T.) ;
#78433=ORIENTED_EDGE('',*,*,#53873,.F.) ;
#78434=ORIENTED_EDGE('',*,*,#53946,.F.) ;
#78435=ORIENTED_EDGE('',*,*,#53825,.F.) ;
#78436=ORIENTED_EDGE('',*,*,#52230,.F.) ;
#78437=ORIENTED_EDGE('',*,*,#53824,.T.) ;
#78438=ORIENTED_EDGE('',*,*,#53946,.T.) ;
#78439=ORIENTED_EDGE('',*,*,#51092,.F.) ;
#78440=ORIENTED_EDGE('',*,*,#53803,.F.) ;
#78441=ORIENTED_EDGE('',*,*,#49544,.F.) ;
#78442=ORIENTED_EDGE('',*,*,#53947,.F.) ;
#78443=ORIENTED_EDGE('',*,*,#53879,.F.) ;
#78444=ORIENTED_EDGE('',*,*,#53947,.T.) ;
#78445=ORIENTED_EDGE('',*,*,#53826,.F.) ;
#78446=ORIENTED_EDGE('',*,*,#53948,.F.) ;
#78447=ORIENTED_EDGE('',*,*,#53878,.F.) ;
#78448=ORIENTED_EDGE('',*,*,#53948,.T.) ;
#78449=ORIENTED_EDGE('',*,*,#49740,.T.) ;
#78450=ORIENTED_EDGE('',*,*,#52244,.F.) ;
#78451=ORIENTED_EDGE('',*,*,#51078,.F.) ;
#78452=ORIENTED_EDGE('',*,*,#53804,.F.) ;
#78453=ORIENTED_EDGE('',*,*,#53883,.F.) ;
#78454=ORIENTED_EDGE('',*,*,#53949,.F.) ;
#78455=ORIENTED_EDGE('',*,*,#49552,.F.) ;
#78456=ORIENTED_EDGE('',*,*,#53949,.T.) ;
#78457=ORIENTED_EDGE('',*,*,#53881,.F.) ;
#78458=ORIENTED_EDGE('',*,*,#53950,.F.) ;
#78459=ORIENTED_EDGE('',*,*,#53832,.F.) ;
#78460=ORIENTED_EDGE('',*,*,#52660,.F.) ;
#78461=ORIENTED_EDGE('',*,*,#53831,.T.) ;
#78462=ORIENTED_EDGE('',*,*,#53950,.T.) ;
#78463=ORIENTED_EDGE('',*,*,#51120,.F.) ;
#78464=ORIENTED_EDGE('',*,*,#53805,.F.) ;
#78465=ORIENTED_EDGE('',*,*,#49550,.F.) ;
#78466=ORIENTED_EDGE('',*,*,#53951,.F.) ;
#78467=ORIENTED_EDGE('',*,*,#53887,.F.) ;
#78468=ORIENTED_EDGE('',*,*,#53951,.T.) ;
#78469=ORIENTED_EDGE('',*,*,#53821,.F.) ;
#78470=ORIENTED_EDGE('',*,*,#53952,.F.) ;
#78471=ORIENTED_EDGE('',*,*,#53886,.F.) ;
#78472=ORIENTED_EDGE('',*,*,#53952,.T.) ;
#78473=ORIENTED_EDGE('',*,*,#53822,.F.) ;
#78474=ORIENTED_EDGE('',*,*,#52643,.F.) ;
#78475=ORIENTED_EDGE('',*,*,#51106,.F.) ;
#78476=ORIENTED_EDGE('',*,*,#53806,.F.) ;
#78477=ORIENTED_EDGE('',*,*,#53891,.F.) ;
#78478=ORIENTED_EDGE('',*,*,#53953,.F.) ;
#78479=ORIENTED_EDGE('',*,*,#49558,.F.) ;
#78480=ORIENTED_EDGE('',*,*,#53953,.T.) ;
#78481=ORIENTED_EDGE('',*,*,#53889,.F.) ;
#78482=ORIENTED_EDGE('',*,*,#53954,.F.) ;
#78483=ORIENTED_EDGE('',*,*,#53838,.F.) ;
#78484=ORIENTED_EDGE('',*,*,#52808,.F.) ;
#78485=ORIENTED_EDGE('',*,*,#53837,.T.) ;
#78486=ORIENTED_EDGE('',*,*,#53954,.T.) ;
#78487=ORIENTED_EDGE('',*,*,#51148,.F.) ;
#78488=ORIENTED_EDGE('',*,*,#53807,.F.) ;
#78489=ORIENTED_EDGE('',*,*,#49556,.F.) ;
#78490=ORIENTED_EDGE('',*,*,#53955,.F.) ;
#78491=ORIENTED_EDGE('',*,*,#53895,.F.) ;
#78492=ORIENTED_EDGE('',*,*,#53955,.T.) ;
#78493=ORIENTED_EDGE('',*,*,#53828,.F.) ;
#78494=ORIENTED_EDGE('',*,*,#53956,.F.) ;
#78495=ORIENTED_EDGE('',*,*,#53894,.F.) ;
#78496=ORIENTED_EDGE('',*,*,#53956,.T.) ;
#78497=ORIENTED_EDGE('',*,*,#53829,.F.) ;
#78498=ORIENTED_EDGE('',*,*,#52791,.F.) ;
#78499=ORIENTED_EDGE('',*,*,#51134,.F.) ;
#78500=ORIENTED_EDGE('',*,*,#53808,.F.) ;
#78501=ORIENTED_EDGE('',*,*,#53899,.F.) ;
#78502=ORIENTED_EDGE('',*,*,#53957,.F.) ;
#78503=ORIENTED_EDGE('',*,*,#49564,.F.) ;
#78504=ORIENTED_EDGE('',*,*,#53957,.T.) ;
#78505=ORIENTED_EDGE('',*,*,#53897,.F.) ;
#78506=ORIENTED_EDGE('',*,*,#53958,.F.) ;
#78507=ORIENTED_EDGE('',*,*,#53844,.F.) ;
#78508=ORIENTED_EDGE('',*,*,#52956,.F.) ;
#78509=ORIENTED_EDGE('',*,*,#53843,.T.) ;
#78510=ORIENTED_EDGE('',*,*,#53958,.T.) ;
#78511=ORIENTED_EDGE('',*,*,#51176,.F.) ;
#78512=ORIENTED_EDGE('',*,*,#53809,.F.) ;
#78513=ORIENTED_EDGE('',*,*,#49562,.F.) ;
#78514=ORIENTED_EDGE('',*,*,#53959,.F.) ;
#78515=ORIENTED_EDGE('',*,*,#53903,.F.) ;
#78516=ORIENTED_EDGE('',*,*,#53959,.T.) ;
#78517=ORIENTED_EDGE('',*,*,#53834,.F.) ;
#78518=ORIENTED_EDGE('',*,*,#53960,.F.) ;
#78519=ORIENTED_EDGE('',*,*,#53902,.F.) ;
#78520=ORIENTED_EDGE('',*,*,#53960,.T.) ;
#78521=ORIENTED_EDGE('',*,*,#53835,.F.) ;
#78522=ORIENTED_EDGE('',*,*,#52939,.F.) ;
#78523=ORIENTED_EDGE('',*,*,#51162,.F.) ;
#78524=ORIENTED_EDGE('',*,*,#53810,.F.) ;
#78525=ORIENTED_EDGE('',*,*,#53907,.F.) ;
#78526=ORIENTED_EDGE('',*,*,#53961,.F.) ;
#78527=ORIENTED_EDGE('',*,*,#49570,.F.) ;
#78528=ORIENTED_EDGE('',*,*,#53961,.T.) ;
#78529=ORIENTED_EDGE('',*,*,#53905,.F.) ;
#78530=ORIENTED_EDGE('',*,*,#53962,.F.) ;
#78531=ORIENTED_EDGE('',*,*,#53850,.F.) ;
#78532=ORIENTED_EDGE('',*,*,#53104,.F.) ;
#78533=ORIENTED_EDGE('',*,*,#53849,.T.) ;
#78534=ORIENTED_EDGE('',*,*,#53962,.T.) ;
#78535=ORIENTED_EDGE('',*,*,#51204,.F.) ;
#78536=ORIENTED_EDGE('',*,*,#53811,.F.) ;
#78537=ORIENTED_EDGE('',*,*,#49568,.F.) ;
#78538=ORIENTED_EDGE('',*,*,#53963,.F.) ;
#78539=ORIENTED_EDGE('',*,*,#53911,.F.) ;
#78540=ORIENTED_EDGE('',*,*,#53963,.T.) ;
#78541=ORIENTED_EDGE('',*,*,#53840,.F.) ;
#78542=ORIENTED_EDGE('',*,*,#53964,.F.) ;
#78543=ORIENTED_EDGE('',*,*,#53910,.F.) ;
#78544=ORIENTED_EDGE('',*,*,#53964,.T.) ;
#78545=ORIENTED_EDGE('',*,*,#53841,.F.) ;
#78546=ORIENTED_EDGE('',*,*,#53087,.F.) ;
#78547=ORIENTED_EDGE('',*,*,#51190,.F.) ;
#78548=ORIENTED_EDGE('',*,*,#53812,.F.) ;
#78549=ORIENTED_EDGE('',*,*,#53915,.F.) ;
#78550=ORIENTED_EDGE('',*,*,#53965,.F.) ;
#78551=ORIENTED_EDGE('',*,*,#49576,.F.) ;
#78552=ORIENTED_EDGE('',*,*,#53965,.T.) ;
#78553=ORIENTED_EDGE('',*,*,#53913,.F.) ;
#78554=ORIENTED_EDGE('',*,*,#53966,.F.) ;
#78555=ORIENTED_EDGE('',*,*,#53856,.F.) ;
#78556=ORIENTED_EDGE('',*,*,#53252,.F.) ;
#78557=ORIENTED_EDGE('',*,*,#53855,.T.) ;
#78558=ORIENTED_EDGE('',*,*,#53966,.T.) ;
#78559=ORIENTED_EDGE('',*,*,#51232,.F.) ;
#78560=ORIENTED_EDGE('',*,*,#53813,.F.) ;
#78561=ORIENTED_EDGE('',*,*,#49574,.F.) ;
#78562=ORIENTED_EDGE('',*,*,#53967,.F.) ;
#78563=ORIENTED_EDGE('',*,*,#53919,.F.) ;
#78564=ORIENTED_EDGE('',*,*,#53967,.T.) ;
#78565=ORIENTED_EDGE('',*,*,#53846,.F.) ;
#78566=ORIENTED_EDGE('',*,*,#53968,.F.) ;
#78567=ORIENTED_EDGE('',*,*,#53918,.F.) ;
#78568=ORIENTED_EDGE('',*,*,#53968,.T.) ;
#78569=ORIENTED_EDGE('',*,*,#53847,.F.) ;
#78570=ORIENTED_EDGE('',*,*,#53235,.F.) ;
#78571=ORIENTED_EDGE('',*,*,#51218,.F.) ;
#78572=ORIENTED_EDGE('',*,*,#53814,.F.) ;
#78573=ORIENTED_EDGE('',*,*,#53923,.F.) ;
#78574=ORIENTED_EDGE('',*,*,#53969,.F.) ;
#78575=ORIENTED_EDGE('',*,*,#49582,.F.) ;
#78576=ORIENTED_EDGE('',*,*,#53969,.T.) ;
#78577=ORIENTED_EDGE('',*,*,#53921,.F.) ;
#78578=ORIENTED_EDGE('',*,*,#53970,.F.) ;
#78579=ORIENTED_EDGE('',*,*,#53862,.F.) ;
#78580=ORIENTED_EDGE('',*,*,#53400,.F.) ;
#78581=ORIENTED_EDGE('',*,*,#53861,.T.) ;
#78582=ORIENTED_EDGE('',*,*,#53970,.T.) ;
#78583=ORIENTED_EDGE('',*,*,#51260,.F.) ;
#78584=ORIENTED_EDGE('',*,*,#53815,.F.) ;
#78585=ORIENTED_EDGE('',*,*,#49580,.F.) ;
#78586=ORIENTED_EDGE('',*,*,#53971,.F.) ;
#78587=ORIENTED_EDGE('',*,*,#53927,.F.) ;
#78588=ORIENTED_EDGE('',*,*,#53971,.T.) ;
#78589=ORIENTED_EDGE('',*,*,#53852,.F.) ;
#78590=ORIENTED_EDGE('',*,*,#53972,.F.) ;
#78591=ORIENTED_EDGE('',*,*,#53926,.F.) ;
#78592=ORIENTED_EDGE('',*,*,#53972,.T.) ;
#78593=ORIENTED_EDGE('',*,*,#53853,.F.) ;
#78594=ORIENTED_EDGE('',*,*,#53383,.F.) ;
#78595=ORIENTED_EDGE('',*,*,#51246,.F.) ;
#78596=ORIENTED_EDGE('',*,*,#53816,.F.) ;
#78597=ORIENTED_EDGE('',*,*,#53931,.F.) ;
#78598=ORIENTED_EDGE('',*,*,#53973,.F.) ;
#78599=ORIENTED_EDGE('',*,*,#49588,.F.) ;
#78600=ORIENTED_EDGE('',*,*,#53973,.T.) ;
#78601=ORIENTED_EDGE('',*,*,#53929,.F.) ;
#78602=ORIENTED_EDGE('',*,*,#53974,.F.) ;
#78603=ORIENTED_EDGE('',*,*,#53868,.F.) ;
#78604=ORIENTED_EDGE('',*,*,#53548,.F.) ;
#78605=ORIENTED_EDGE('',*,*,#53867,.T.) ;
#78606=ORIENTED_EDGE('',*,*,#53974,.T.) ;
#78607=ORIENTED_EDGE('',*,*,#51288,.F.) ;
#78608=ORIENTED_EDGE('',*,*,#53817,.F.) ;
#78609=ORIENTED_EDGE('',*,*,#49586,.F.) ;
#78610=ORIENTED_EDGE('',*,*,#53975,.F.) ;
#78611=ORIENTED_EDGE('',*,*,#53935,.F.) ;
#78612=ORIENTED_EDGE('',*,*,#53975,.T.) ;
#78613=ORIENTED_EDGE('',*,*,#53858,.F.) ;
#78614=ORIENTED_EDGE('',*,*,#53976,.F.) ;
#78615=ORIENTED_EDGE('',*,*,#53934,.F.) ;
#78616=ORIENTED_EDGE('',*,*,#53976,.T.) ;
#78617=ORIENTED_EDGE('',*,*,#53859,.F.) ;
#78618=ORIENTED_EDGE('',*,*,#53531,.F.) ;
#78619=ORIENTED_EDGE('',*,*,#51274,.F.) ;
#78620=ORIENTED_EDGE('',*,*,#53818,.F.) ;
#78621=ORIENTED_EDGE('',*,*,#53939,.F.) ;
#78622=ORIENTED_EDGE('',*,*,#53977,.F.) ;
#78623=ORIENTED_EDGE('',*,*,#49594,.F.) ;
#78624=ORIENTED_EDGE('',*,*,#53977,.T.) ;
#78625=ORIENTED_EDGE('',*,*,#53937,.F.) ;
#78626=ORIENTED_EDGE('',*,*,#53978,.F.) ;
#78627=ORIENTED_EDGE('',*,*,#53872,.F.) ;
#78628=ORIENTED_EDGE('',*,*,#53696,.F.) ;
#78629=ORIENTED_EDGE('',*,*,#53871,.T.) ;
#78630=ORIENTED_EDGE('',*,*,#53978,.T.) ;
#78631=ORIENTED_EDGE('',*,*,#51316,.F.) ;
#78632=ORIENTED_EDGE('',*,*,#53819,.F.) ;
#78633=ORIENTED_EDGE('',*,*,#49592,.F.) ;
#78634=ORIENTED_EDGE('',*,*,#53979,.F.) ;
#78635=ORIENTED_EDGE('',*,*,#53943,.F.) ;
#78636=ORIENTED_EDGE('',*,*,#53979,.T.) ;
#78637=ORIENTED_EDGE('',*,*,#53864,.F.) ;
#78638=ORIENTED_EDGE('',*,*,#53980,.F.) ;
#78639=ORIENTED_EDGE('',*,*,#53942,.F.) ;
#78640=ORIENTED_EDGE('',*,*,#53980,.T.) ;
#78641=ORIENTED_EDGE('',*,*,#53865,.F.) ;
#78642=ORIENTED_EDGE('',*,*,#53679,.F.) ;
#78643=ORIENTED_EDGE('',*,*,#51302,.F.) ;
#78644=ORIENTED_EDGE('',*,*,#49002,.T.) ;
#78645=ORIENTED_EDGE('',*,*,#53981,.T.) ;
#78646=ORIENTED_EDGE('',*,*,#49004,.F.) ;
#78647=ORIENTED_EDGE('',*,*,#48927,.T.) ;
#78648=ORIENTED_EDGE('',*,*,#48999,.T.) ;
#78649=ORIENTED_EDGE('',*,*,#53982,.T.) ;
#78650=ORIENTED_EDGE('',*,*,#49001,.F.) ;
#78651=ORIENTED_EDGE('',*,*,#48935,.T.) ;
#78652=ORIENTED_EDGE('',*,*,#48996,.T.) ;
#78653=ORIENTED_EDGE('',*,*,#53983,.T.) ;
#78654=ORIENTED_EDGE('',*,*,#48998,.F.) ;
#78655=ORIENTED_EDGE('',*,*,#48943,.T.) ;
#78656=ORIENTED_EDGE('',*,*,#48993,.T.) ;
#78657=ORIENTED_EDGE('',*,*,#53984,.T.) ;
#78658=ORIENTED_EDGE('',*,*,#48995,.F.) ;
#78659=ORIENTED_EDGE('',*,*,#48951,.T.) ;
#78660=ORIENTED_EDGE('',*,*,#48990,.T.) ;
#78661=ORIENTED_EDGE('',*,*,#53985,.T.) ;
#78662=ORIENTED_EDGE('',*,*,#48992,.F.) ;
#78663=ORIENTED_EDGE('',*,*,#48959,.T.) ;
#78664=ORIENTED_EDGE('',*,*,#48987,.T.) ;
#78665=ORIENTED_EDGE('',*,*,#53986,.T.) ;
#78666=ORIENTED_EDGE('',*,*,#48989,.F.) ;
#78667=ORIENTED_EDGE('',*,*,#48967,.T.) ;
#78668=ORIENTED_EDGE('',*,*,#50140,.F.) ;
#78669=ORIENTED_EDGE('',*,*,#50144,.F.) ;
#78670=ORIENTED_EDGE('',*,*,#53987,.F.) ;
#78671=ORIENTED_EDGE('',*,*,#53987,.T.) ;
#78672=ORIENTED_EDGE('',*,*,#49892,.F.) ;
#78673=ORIENTED_EDGE('',*,*,#53988,.F.) ;
#78674=ORIENTED_EDGE('',*,*,#49673,.F.) ;
#78675=ORIENTED_EDGE('',*,*,#53988,.T.) ;
#78676=ORIENTED_EDGE('',*,*,#49891,.F.) ;
#78677=ORIENTED_EDGE('',*,*,#53989,.F.) ;
#78678=ORIENTED_EDGE('',*,*,#53698,.F.) ;
#78679=ORIENTED_EDGE('',*,*,#53990,.F.) ;
#78680=ORIENTED_EDGE('',*,*,#51326,.F.) ;
#78681=ORIENTED_EDGE('',*,*,#53989,.T.) ;
#78682=ORIENTED_EDGE('',*,*,#49890,.F.) ;
#78683=ORIENTED_EDGE('',*,*,#53869,.F.) ;
#78684=ORIENTED_EDGE('',*,*,#53990,.T.) ;
#78685=ORIENTED_EDGE('',*,*,#53991,.F.) ;
#78686=ORIENTED_EDGE('',*,*,#53992,.F.) ;
#78687=ORIENTED_EDGE('',*,*,#49533,.F.) ;
#78688=ORIENTED_EDGE('',*,*,#53991,.T.) ;
#78689=ORIENTED_EDGE('',*,*,#49889,.F.) ;
#78690=ORIENTED_EDGE('',*,*,#49738,.F.) ;
#78691=ORIENTED_EDGE('',*,*,#53992,.T.) ;
#78692=ORIENTED_EDGE('',*,*,#53993,.F.) ;
#78693=ORIENTED_EDGE('',*,*,#53993,.T.) ;
#78694=ORIENTED_EDGE('',*,*,#49888,.F.) ;
#78695=ORIENTED_EDGE('',*,*,#53994,.F.) ;
#78696=ORIENTED_EDGE('',*,*,#49990,.F.) ;
#78697=ORIENTED_EDGE('',*,*,#50165,.F.) ;
#78698=ORIENTED_EDGE('',*,*,#50155,.F.) ;
#78699=ORIENTED_EDGE('',*,*,#53995,.F.) ;
#78700=ORIENTED_EDGE('',*,*,#53994,.T.) ;
#78701=ORIENTED_EDGE('',*,*,#49887,.T.) ;
#78702=ORIENTED_EDGE('',*,*,#53996,.F.) ;
#78703=ORIENTED_EDGE('',*,*,#53997,.F.) ;
#78704=ORIENTED_EDGE('',*,*,#53995,.T.) ;
#78705=ORIENTED_EDGE('',*,*,#49334,.F.) ;
#78706=ORIENTED_EDGE('',*,*,#53998,.F.) ;
#78707=ORIENTED_EDGE('',*,*,#49885,.F.) ;
#78708=ORIENTED_EDGE('',*,*,#53996,.T.) ;
#78709=ORIENTED_EDGE('',*,*,#49886,.F.) ;
#78710=ORIENTED_EDGE('',*,*,#53999,.F.) ;
#78711=ORIENTED_EDGE('',*,*,#49668,.F.) ;
#78712=ORIENTED_EDGE('',*,*,#53997,.T.) ;
#78713=ORIENTED_EDGE('',*,*,#49671,.F.) ;
#78714=ORIENTED_EDGE('',*,*,#54000,.F.) ;
#78715=ORIENTED_EDGE('',*,*,#49991,.F.) ;
#78716=ORIENTED_EDGE('',*,*,#53999,.T.) ;
#78717=ORIENTED_EDGE('',*,*,#53998,.T.) ;
#78718=ORIENTED_EDGE('',*,*,#54001,.F.) ;
#78719=ORIENTED_EDGE('',*,*,#49992,.T.) ;
#78720=ORIENTED_EDGE('',*,*,#54000,.T.) ;
#78721=ORIENTED_EDGE('',*,*,#54002,.F.) ;
#78722=ORIENTED_EDGE('',*,*,#54003,.F.) ;
#78723=ORIENTED_EDGE('',*,*,#54001,.T.) ;
#78724=ORIENTED_EDGE('',*,*,#49333,.F.) ;
#78725=ORIENTED_EDGE('',*,*,#54004,.F.) ;
#78726=ORIENTED_EDGE('',*,*,#49669,.F.) ;
#78727=ORIENTED_EDGE('',*,*,#54002,.T.) ;
#78728=ORIENTED_EDGE('',*,*,#49670,.F.) ;
#78729=ORIENTED_EDGE('',*,*,#54005,.F.) ;
#78730=ORIENTED_EDGE('',*,*,#50103,.F.) ;
#78731=ORIENTED_EDGE('',*,*,#54003,.T.) ;
#78732=ORIENTED_EDGE('',*,*,#50105,.F.) ;
#78733=ORIENTED_EDGE('',*,*,#54006,.F.) ;
#78734=ORIENTED_EDGE('',*,*,#49993,.F.) ;
#78735=ORIENTED_EDGE('',*,*,#54005,.T.) ;
#78736=ORIENTED_EDGE('',*,*,#54004,.T.) ;
#78737=ORIENTED_EDGE('',*,*,#54007,.F.) ;
#78738=ORIENTED_EDGE('',*,*,#54006,.T.) ;
#78739=ORIENTED_EDGE('',*,*,#49288,.F.) ;
#78740=ORIENTED_EDGE('',*,*,#48982,.F.) ;
#78741=ORIENTED_EDGE('',*,*,#54007,.T.) ;
#78742=ORIENTED_EDGE('',*,*,#49332,.F.) ;
#78743=ORIENTED_EDGE('',*,*,#48980,.F.) ;
#78744=ORIENTED_EDGE('',*,*,#50104,.F.) ;
#78745=ORIENTED_EDGE('',*,*,#48984,.T.) ;
#78746=ORIENTED_EDGE('',*,*,#49285,.F.) ;
#78747=ORIENTED_EDGE('',*,*,#48974,.F.) ;
#78748=ORIENTED_EDGE('',*,*,#48978,.T.) ;
#78749=ORIENTED_EDGE('',*,*,#49331,.F.) ;
#78750=ORIENTED_EDGE('',*,*,#48972,.F.) ;
#78751=ORIENTED_EDGE('',*,*,#50106,.F.) ;
#78752=ORIENTED_EDGE('',*,*,#48976,.T.) ;
#78753=ORIENTED_EDGE('',*,*,#48985,.F.) ;
#78754=ORIENTED_EDGE('',*,*,#48966,.F.) ;
#78755=ORIENTED_EDGE('',*,*,#48970,.T.) ;
#78756=ORIENTED_EDGE('',*,*,#49330,.F.) ;
#78757=ORIENTED_EDGE('',*,*,#48964,.F.) ;
#78758=ORIENTED_EDGE('',*,*,#50107,.F.) ;
#78759=ORIENTED_EDGE('',*,*,#48968,.T.) ;
#78760=ORIENTED_EDGE('',*,*,#48988,.F.) ;
#78761=ORIENTED_EDGE('',*,*,#48958,.F.) ;
#78762=ORIENTED_EDGE('',*,*,#48962,.T.) ;
#78763=ORIENTED_EDGE('',*,*,#49329,.F.) ;
#78764=ORIENTED_EDGE('',*,*,#48956,.F.) ;
#78765=ORIENTED_EDGE('',*,*,#53986,.F.) ;
#78766=ORIENTED_EDGE('',*,*,#48960,.T.) ;
#78767=ORIENTED_EDGE('',*,*,#48991,.F.) ;
#78768=ORIENTED_EDGE('',*,*,#48950,.F.) ;
#78769=ORIENTED_EDGE('',*,*,#48954,.T.) ;
#78770=ORIENTED_EDGE('',*,*,#49328,.F.) ;
#78771=ORIENTED_EDGE('',*,*,#48948,.F.) ;
#78772=ORIENTED_EDGE('',*,*,#53985,.F.) ;
#78773=ORIENTED_EDGE('',*,*,#48952,.T.) ;
#78774=ORIENTED_EDGE('',*,*,#48994,.F.) ;
#78775=ORIENTED_EDGE('',*,*,#48942,.F.) ;
#78776=ORIENTED_EDGE('',*,*,#48946,.T.) ;
#78777=ORIENTED_EDGE('',*,*,#49327,.F.) ;
#78778=ORIENTED_EDGE('',*,*,#48940,.F.) ;
#78779=ORIENTED_EDGE('',*,*,#53984,.F.) ;
#78780=ORIENTED_EDGE('',*,*,#48944,.T.) ;
#78781=ORIENTED_EDGE('',*,*,#48997,.F.) ;
#78782=ORIENTED_EDGE('',*,*,#48934,.F.) ;
#78783=ORIENTED_EDGE('',*,*,#48938,.T.) ;
#78784=ORIENTED_EDGE('',*,*,#49326,.F.) ;
#78785=ORIENTED_EDGE('',*,*,#48932,.F.) ;
#78786=ORIENTED_EDGE('',*,*,#53983,.F.) ;
#78787=ORIENTED_EDGE('',*,*,#48936,.T.) ;
#78788=ORIENTED_EDGE('',*,*,#49000,.F.) ;
#78789=ORIENTED_EDGE('',*,*,#48926,.F.) ;
#78790=ORIENTED_EDGE('',*,*,#48930,.T.) ;
#78791=ORIENTED_EDGE('',*,*,#49325,.F.) ;
#78792=ORIENTED_EDGE('',*,*,#48924,.F.) ;
#78793=ORIENTED_EDGE('',*,*,#53982,.F.) ;
#78794=ORIENTED_EDGE('',*,*,#48928,.T.) ;
#78795=ORIENTED_EDGE('',*,*,#49003,.F.) ;
#78796=ORIENTED_EDGE('',*,*,#48918,.F.) ;
#78797=ORIENTED_EDGE('',*,*,#50136,.F.) ;
#78798=ORIENTED_EDGE('',*,*,#50141,.F.) ;
#78799=ORIENTED_EDGE('',*,*,#54008,.F.) ;
#78800=ORIENTED_EDGE('',*,*,#48922,.T.) ;
#78801=ORIENTED_EDGE('',*,*,#49324,.F.) ;
#78802=ORIENTED_EDGE('',*,*,#48916,.F.) ;
#78803=ORIENTED_EDGE('',*,*,#53981,.F.) ;
#78804=ORIENTED_EDGE('',*,*,#54008,.T.) ;
#78805=ORIENTED_EDGE('',*,*,#49735,.F.) ;
#78806=ORIENTED_EDGE('',*,*,#54009,.F.) ;
#78807=ORIENTED_EDGE('',*,*,#49908,.F.) ;
#78808=ORIENTED_EDGE('',*,*,#48920,.T.) ;
#78809=ORIENTED_EDGE('',*,*,#49294,.F.) ;
#78810=ORIENTED_EDGE('',*,*,#48910,.F.) ;
#78811=ORIENTED_EDGE('',*,*,#54009,.T.) ;
#78812=ORIENTED_EDGE('',*,*,#50222,.F.) ;
#78813=ORIENTED_EDGE('',*,*,#54010,.F.) ;
#78814=ORIENTED_EDGE('',*,*,#49909,.F.) ;
#78815=ORIENTED_EDGE('',*,*,#48914,.T.) ;
#78816=ORIENTED_EDGE('',*,*,#49323,.F.) ;
#78817=ORIENTED_EDGE('',*,*,#48908,.F.) ;
#78818=ORIENTED_EDGE('',*,*,#50098,.F.) ;
#78819=ORIENTED_EDGE('',*,*,#54010,.T.) ;
#78820=ORIENTED_EDGE('',*,*,#49999,.F.) ;
#78821=ORIENTED_EDGE('',*,*,#54011,.F.) ;
#78822=ORIENTED_EDGE('',*,*,#49910,.F.) ;
#78823=ORIENTED_EDGE('',*,*,#48912,.T.) ;
#78824=ORIENTED_EDGE('',*,*,#49291,.F.) ;
#78825=ORIENTED_EDGE('',*,*,#54012,.F.) ;
#78826=ORIENTED_EDGE('',*,*,#54011,.T.) ;
#78827=ORIENTED_EDGE('',*,*,#50345,.F.) ;
#78828=ORIENTED_EDGE('',*,*,#54013,.F.) ;
#78829=ORIENTED_EDGE('',*,*,#48906,.T.) ;
#78830=ORIENTED_EDGE('',*,*,#49322,.F.) ;
#78831=ORIENTED_EDGE('',*,*,#48904,.F.) ;
#78832=ORIENTED_EDGE('',*,*,#50099,.F.) ;
#78833=ORIENTED_EDGE('',*,*,#54012,.T.) ;
#78834=ORIENTED_EDGE('',*,*,#50102,.F.) ;
#78835=ORIENTED_EDGE('',*,*,#54014,.F.) ;
#78836=ORIENTED_EDGE('',*,*,#49994,.F.) ;
#78837=ORIENTED_EDGE('',*,*,#54013,.T.) ;
#78838=ORIENTED_EDGE('',*,*,#49535,.F.) ;
#78839=ORIENTED_EDGE('',*,*,#54015,.F.) ;
#78840=ORIENTED_EDGE('',*,*,#49911,.F.) ;
#78841=ORIENTED_EDGE('',*,*,#49995,.T.) ;
#78842=ORIENTED_EDGE('',*,*,#54014,.T.) ;
#78843=ORIENTED_EDGE('',*,*,#54016,.F.) ;
#78844=ORIENTED_EDGE('',*,*,#54017,.F.) ;
#78845=ORIENTED_EDGE('',*,*,#54015,.T.) ;
#78846=ORIENTED_EDGE('',*,*,#49737,.F.) ;
#78847=ORIENTED_EDGE('',*,*,#54018,.F.) ;
#78848=ORIENTED_EDGE('',*,*,#48902,.T.) ;
#78849=ORIENTED_EDGE('',*,*,#49321,.F.) ;
#78850=ORIENTED_EDGE('',*,*,#54019,.F.) ;
#78851=ORIENTED_EDGE('',*,*,#50100,.F.) ;
#78852=ORIENTED_EDGE('',*,*,#54016,.T.) ;
#78853=ORIENTED_EDGE('',*,*,#50101,.F.) ;
#78854=ORIENTED_EDGE('',*,*,#54020,.F.) ;
#78855=ORIENTED_EDGE('',*,*,#49808,.F.) ;
#78856=ORIENTED_EDGE('',*,*,#54017,.T.) ;
#78857=ORIENTED_EDGE('',*,*,#49811,.F.) ;
#78858=ORIENTED_EDGE('',*,*,#54021,.F.) ;
#78859=ORIENTED_EDGE('',*,*,#49996,.F.) ;
#78860=ORIENTED_EDGE('',*,*,#54018,.T.) ;
#78861=ORIENTED_EDGE('',*,*,#49997,.F.) ;
#78862=ORIENTED_EDGE('',*,*,#54022,.F.) ;
#78863=ORIENTED_EDGE('',*,*,#49912,.F.) ;
#78864=ORIENTED_EDGE('',*,*,#54020,.T.) ;
#78865=ORIENTED_EDGE('',*,*,#54019,.T.) ;
#78866=ORIENTED_EDGE('',*,*,#54023,.F.) ;
#78867=ORIENTED_EDGE('',*,*,#54022,.T.) ;
#78868=ORIENTED_EDGE('',*,*,#54021,.T.) ;
#78869=ORIENTED_EDGE('',*,*,#54024,.F.) ;
#78870=ORIENTED_EDGE('',*,*,#49913,.T.) ;
#78871=ORIENTED_EDGE('',*,*,#54023,.T.) ;
#78872=ORIENTED_EDGE('',*,*,#49320,.F.) ;
#78873=ORIENTED_EDGE('',*,*,#54025,.F.) ;
#78874=ORIENTED_EDGE('',*,*,#49809,.F.) ;
#78875=ORIENTED_EDGE('',*,*,#54024,.T.) ;
#78876=ORIENTED_EDGE('',*,*,#49810,.F.) ;
#78877=ORIENTED_EDGE('',*,*,#54026,.F.) ;
#78878=ORIENTED_EDGE('',*,*,#49899,.F.) ;
#78879=ORIENTED_EDGE('',*,*,#54026,.T.) ;
#78880=ORIENTED_EDGE('',*,*,#54025,.T.) ;
#78881=ORIENTED_EDGE('',*,*,#54027,.F.) ;
#78882=ORIENTED_EDGE('',*,*,#54027,.T.) ;
#78883=ORIENTED_EDGE('',*,*,#49319,.F.) ;
#78884=ORIENTED_EDGE('',*,*,#54028,.F.) ;
#78885=ORIENTED_EDGE('',*,*,#49900,.F.) ;
#78886=ORIENTED_EDGE('',*,*,#50154,.F.) ;
#78887=ORIENTED_EDGE('',*,*,#50146,.F.) ;
#78888=ORIENTED_EDGE('',*,*,#54028,.T.) ;
#78889=ORIENTED_EDGE('',*,*,#50158,.F.) ;
#78890=ORIENTED_EDGE('',*,*,#50150,.F.) ;
#78891=ORIENTED_EDGE('',*,*,#50149,.F.) ;
#78892=ORIENTED_EDGE('',*,*,#54029,.F.) ;
#78893=ORIENTED_EDGE('',*,*,#50159,.F.) ;
#78894=ORIENTED_EDGE('',*,*,#54029,.T.) ;
#78895=ORIENTED_EDGE('',*,*,#50157,.F.) ;
#78896=ORIENTED_EDGE('',*,*,#48899,.F.) ;
#78897=ORIENTED_EDGE('',*,*,#50160,.F.) ;
#78898=ORIENTED_EDGE('',*,*,#50174,.F.) ;
#78899=ORIENTED_EDGE('',*,*,#50179,.F.) ;
#78900=ORIENTED_EDGE('',*,*,#50178,.F.) ;
#78901=ORIENTED_EDGE('',*,*,#54030,.F.) ;
#78902=ORIENTED_EDGE('',*,*,#50175,.F.) ;
#78903=ORIENTED_EDGE('',*,*,#48897,.T.) ;
#78904=ORIENTED_EDGE('',*,*,#50171,.F.) ;
#78905=ORIENTED_EDGE('',*,*,#54030,.T.) ;
#78906=ORIENTED_EDGE('',*,*,#50177,.F.) ;
#79344=TOROIDAL_SURFACE('',#98155,0.1645125,0.1) ;
#79345=TOROIDAL_SURFACE('',#98160,0.1645125,0.1) ;
#79346=TOROIDAL_SURFACE('',#98165,2.35,0.1) ;
#79347=TOROIDAL_SURFACE('',#98168,0.1645125,0.1) ;
#79348=TOROIDAL_SURFACE('',#98173,2.35,0.1) ;
#79349=TOROIDAL_SURFACE('',#98176,0.1645125,0.1) ;
#79350=TOROIDAL_SURFACE('',#98181,2.35,0.1) ;
#79351=TOROIDAL_SURFACE('',#98184,0.1645125,0.1) ;
#79352=TOROIDAL_SURFACE('',#98189,2.35,0.1) ;
#79353=TOROIDAL_SURFACE('',#98192,0.1645125,0.1) ;
#79354=TOROIDAL_SURFACE('',#98197,2.35,0.1) ;
#79355=TOROIDAL_SURFACE('',#98200,0.1645125,0.1) ;
#79356=TOROIDAL_SURFACE('',#98205,2.35,0.1) ;
#79357=TOROIDAL_SURFACE('',#98208,0.1645125,0.1) ;
#79358=TOROIDAL_SURFACE('',#98213,2.35,0.1) ;
#79359=TOROIDAL_SURFACE('',#98216,0.1645125,0.1) ;
#79360=TOROIDAL_SURFACE('',#98221,2.35,0.1) ;
#79361=TOROIDAL_SURFACE('',#98224,0.164512500000005,0.1) ;
#79362=TOROIDAL_SURFACE('',#98229,2.35,0.1) ;
#79363=TOROIDAL_SURFACE('',#98232,0.164512500000006,0.1) ;
#79364=TOROIDAL_SURFACE('',#98237,2.35,0.1) ;
#79365=TOROIDAL_SURFACE('',#98254,0.899999999999998,0.1) ;
#79366=TOROIDAL_SURFACE('',#98258,1.6,0.1) ;
#79367=TOROIDAL_SURFACE('',#98262,1.1,0.1) ;
#79368=TOROIDAL_SURFACE('',#98266,0.900000000000001,0.1) ;
#79369=TOROIDAL_SURFACE('',#98270,1.6,0.1) ;
#79370=TOROIDAL_SURFACE('',#98274,1.1,0.1) ;
#79371=TOROIDAL_SURFACE('',#98278,0.900000000000001,0.1) ;
#79372=TOROIDAL_SURFACE('',#98282,1.6,0.1) ;
#79373=TOROIDAL_SURFACE('',#98286,1.1,0.1) ;
#79374=TOROIDAL_SURFACE('',#98290,0.900000000000001,0.1) ;
#79375=TOROIDAL_SURFACE('',#98294,1.6,0.1) ;
#79376=TOROIDAL_SURFACE('',#98298,1.1,0.1) ;
#79377=TOROIDAL_SURFACE('',#98302,0.900000000000001,0.1) ;
#79378=TOROIDAL_SURFACE('',#98306,1.6,0.1) ;
#79379=TOROIDAL_SURFACE('',#98310,1.1,0.1) ;
#79380=TOROIDAL_SURFACE('',#98314,0.900000000000001,0.1) ;
#79381=TOROIDAL_SURFACE('',#98318,1.6,0.1) ;
#79382=TOROIDAL_SURFACE('',#98322,1.1,0.1) ;
#79383=TOROIDAL_SURFACE('',#98326,0.900000000000001,0.1) ;
#79384=TOROIDAL_SURFACE('',#98330,1.6,0.1) ;
#79385=TOROIDAL_SURFACE('',#98334,1.1,0.1) ;
#79386=TOROIDAL_SURFACE('',#98338,0.9,0.1) ;
#79387=TOROIDAL_SURFACE('',#98342,1.6,0.1) ;
#79388=TOROIDAL_SURFACE('',#98346,1.1,0.1) ;
#79389=TOROIDAL_SURFACE('',#98350,0.900000000000001,0.1) ;
#79390=TOROIDAL_SURFACE('',#98354,1.6,0.1) ;
#79391=TOROIDAL_SURFACE('',#98358,1.1,0.1) ;
#79392=TOROIDAL_SURFACE('',#98443,0.9,0.1) ;
#79393=TOROIDAL_SURFACE('',#98447,1.6,0.1) ;
#79394=TOROIDAL_SURFACE('',#98451,1.1,0.1) ;
#79395=TOROIDAL_SURFACE('',#98858,0.2,0.1) ;
#79396=TOROIDAL_SURFACE('',#98872,0.2,0.1) ;
#79397=TOROIDAL_SURFACE('',#98882,1.75625,0.1) ;
#79398=TOROIDAL_SURFACE('',#98897,0.2,0.1) ;
#79399=TOROIDAL_SURFACE('',#98909,1.55625,0.1) ;
#79400=TOROIDAL_SURFACE('',#98917,0.2,0.1) ;
#79401=TOROIDAL_SURFACE('',#98919,0.2,0.1) ;
#79402=TOROIDAL_SURFACE('',#98933,0.2,0.1) ;
#79403=TOROIDAL_SURFACE('',#98950,0.2,0.1) ;
#79404=TOROIDAL_SURFACE('',#98964,0.2,0.1) ;
#79405=TOROIDAL_SURFACE('',#98967,0.2,0.1) ;
#79406=TOROIDAL_SURFACE('',#98974,0.2,0.1) ;
#79407=TOROIDAL_SURFACE('',#98976,0.2,0.1) ;
#79408=TOROIDAL_SURFACE('',#98982,0.2,0.1) ;
#79409=TOROIDAL_SURFACE('',#98986,0.2,0.1) ;
#79410=TOROIDAL_SURFACE('',#98989,0.2,0.1) ;
#79411=TOROIDAL_SURFACE('',#99006,0.2,0.1) ;
#79412=TOROIDAL_SURFACE('',#99012,0.2,0.1) ;
#79413=TOROIDAL_SURFACE('',#99094,0.2,0.1) ;
#79414=TOROIDAL_SURFACE('',#99097,0.2,0.1) ;
#79415=TOROIDAL_SURFACE('',#99114,0.2,0.1) ;
#79416=TOROIDAL_SURFACE('',#99120,0.2,0.1) ;
#79417=TOROIDAL_SURFACE('',#99182,0.2,0.1) ;
#79418=TOROIDAL_SURFACE('',#99187,0.2,0.1) ;
#79419=TOROIDAL_SURFACE('',#99188,0.2,0.1) ;
#79420=TOROIDAL_SURFACE('',#99194,0.2,0.1) ;
#79421=TOROIDAL_SURFACE('',#99200,0.2,0.1) ;
#79422=TOROIDAL_SURFACE('',#99203,0.2,0.1) ;
#79423=TOROIDAL_SURFACE('',#99204,0.2,0.1) ;
#79424=TOROIDAL_SURFACE('',#99207,0.2,0.1) ;
#79425=TOROIDAL_SURFACE('',#99946,1.75625,0.1) ;
#79426=TOROIDAL_SURFACE('',#99961,0.2,0.1) ;
#79427=TOROIDAL_SURFACE('',#99973,1.55625,0.1) ;
#79428=TOROIDAL_SURFACE('',#99981,0.2,0.1) ;
#79429=TOROIDAL_SURFACE('',#99983,0.2,0.1) ;
#79430=TOROIDAL_SURFACE('',#99997,0.2,0.1) ;
#79431=TOROIDAL_SURFACE('',#100014,0.2,0.1) ;
#79432=TOROIDAL_SURFACE('',#100025,0.2,0.1) ;
#79433=TOROIDAL_SURFACE('',#100028,0.2,0.1) ;
#79434=TOROIDAL_SURFACE('',#100035,0.2,0.1) ;
#79435=TOROIDAL_SURFACE('',#100037,0.2,0.1) ;
#79436=TOROIDAL_SURFACE('',#100043,0.2,0.1) ;
#79437=TOROIDAL_SURFACE('',#100143,0.2,0.1) ;
#79438=TOROIDAL_SURFACE('',#100146,0.2,0.1) ;
#79439=TOROIDAL_SURFACE('',#100163,0.2,0.1) ;
#79440=TOROIDAL_SURFACE('',#100169,0.2,0.1) ;
#79441=TOROIDAL_SURFACE('',#100411,0.2,0.1) ;
#79442=TOROIDAL_SURFACE('',#100414,0.2,0.1) ;
#79443=TOROIDAL_SURFACE('',#100431,0.2,0.1) ;
#79444=TOROIDAL_SURFACE('',#100437,0.2,0.1) ;
#79445=TOROIDAL_SURFACE('',#100504,1.75625,0.1) ;
#79446=TOROIDAL_SURFACE('',#100511,0.2,0.1) ;
#79447=TOROIDAL_SURFACE('',#100524,1.55625,0.1) ;
#79448=TOROIDAL_SURFACE('',#100533,0.2,0.1) ;
#79449=TOROIDAL_SURFACE('',#100535,0.2,0.1) ;
#79450=TOROIDAL_SURFACE('',#100553,0.2,0.1) ;
#79451=TOROIDAL_SURFACE('',#100563,0.2,0.1) ;
#79452=TOROIDAL_SURFACE('',#100577,0.2,0.1) ;
#79453=TOROIDAL_SURFACE('',#100644,0.2,0.1) ;
#79454=TOROIDAL_SURFACE('',#100651,0.2,0.1) ;
#79455=TOROIDAL_SURFACE('',#100653,0.2,0.1) ;
#79456=TOROIDAL_SURFACE('',#100659,0.2,0.1) ;
#79457=TOROIDAL_SURFACE('',#100687,0.2,0.1) ;
#79458=TOROIDAL_SURFACE('',#100690,0.2,0.1) ;
#79459=TOROIDAL_SURFACE('',#100707,0.2,0.1) ;
#79460=TOROIDAL_SURFACE('',#100713,0.2,0.1) ;
#79461=TOROIDAL_SURFACE('',#100780,1.75625,0.1) ;
#79462=TOROIDAL_SURFACE('',#100787,0.2,0.1) ;
#79463=TOROIDAL_SURFACE('',#100800,1.55625,0.1) ;
#79464=TOROIDAL_SURFACE('',#100809,0.2,0.1) ;
#79465=TOROIDAL_SURFACE('',#100811,0.2,0.1) ;
#79466=TOROIDAL_SURFACE('',#100829,0.2,0.1) ;
#79467=TOROIDAL_SURFACE('',#100839,0.2,0.1) ;
#79468=TOROIDAL_SURFACE('',#100853,0.2,0.1) ;
#79469=TOROIDAL_SURFACE('',#100920,0.2,0.1) ;
#79470=TOROIDAL_SURFACE('',#100927,0.2,0.1) ;
#79471=TOROIDAL_SURFACE('',#100929,0.2,0.1) ;
#79472=TOROIDAL_SURFACE('',#100935,0.2,0.1) ;
#79473=TOROIDAL_SURFACE('',#100963,0.2,0.1) ;
#79474=TOROIDAL_SURFACE('',#100966,0.2,0.1) ;
#79475=TOROIDAL_SURFACE('',#100983,0.2,0.1) ;
#79476=TOROIDAL_SURFACE('',#100989,0.2,0.1) ;
#79477=TOROIDAL_SURFACE('',#101056,1.75625,0.1) ;
#79478=TOROIDAL_SURFACE('',#101063,0.2,0.1) ;
#79479=TOROIDAL_SURFACE('',#101076,1.55625,0.1) ;
#79480=TOROIDAL_SURFACE('',#101085,0.2,0.1) ;
#79481=TOROIDAL_SURFACE('',#101087,0.2,0.1) ;
#79482=TOROIDAL_SURFACE('',#101105,0.2,0.1) ;
#79483=TOROIDAL_SURFACE('',#101115,0.2,0.1) ;
#79484=TOROIDAL_SURFACE('',#101129,0.2,0.1) ;
#79485=TOROIDAL_SURFACE('',#101196,0.2,0.1) ;
#79486=TOROIDAL_SURFACE('',#101203,0.2,0.1) ;
#79487=TOROIDAL_SURFACE('',#101205,0.2,0.1) ;
#79488=TOROIDAL_SURFACE('',#101211,0.2,0.1) ;
#79489=TOROIDAL_SURFACE('',#101239,0.2,0.1) ;
#79490=TOROIDAL_SURFACE('',#101242,0.2,0.1) ;
#79491=TOROIDAL_SURFACE('',#101259,0.2,0.1) ;
#79492=TOROIDAL_SURFACE('',#101265,0.2,0.1) ;
#79493=TOROIDAL_SURFACE('',#101332,1.75625,0.1) ;
#79494=TOROIDAL_SURFACE('',#101339,0.2,0.1) ;
#79495=TOROIDAL_SURFACE('',#101352,1.55625,0.1) ;
#79496=TOROIDAL_SURFACE('',#101361,0.2,0.1) ;
#79497=TOROIDAL_SURFACE('',#101363,0.2,0.1) ;
#79498=TOROIDAL_SURFACE('',#101381,0.2,0.1) ;
#79499=TOROIDAL_SURFACE('',#101391,0.2,0.1) ;
#79500=TOROIDAL_SURFACE('',#101405,0.2,0.1) ;
#79501=TOROIDAL_SURFACE('',#101472,0.2,0.1) ;
#79502=TOROIDAL_SURFACE('',#101479,0.2,0.1) ;
#79503=TOROIDAL_SURFACE('',#101481,0.2,0.1) ;
#79504=TOROIDAL_SURFACE('',#101487,0.2,0.1) ;
#79505=TOROIDAL_SURFACE('',#101515,0.2,0.1) ;
#79506=TOROIDAL_SURFACE('',#101518,0.2,0.1) ;
#79507=TOROIDAL_SURFACE('',#101535,0.2,0.1) ;
#79508=TOROIDAL_SURFACE('',#101541,0.2,0.1) ;
#79509=TOROIDAL_SURFACE('',#101608,1.75625,0.1) ;
#79510=TOROIDAL_SURFACE('',#101615,0.2,0.1) ;
#79511=TOROIDAL_SURFACE('',#101628,1.55625,0.1) ;
#79512=TOROIDAL_SURFACE('',#101637,0.2,0.1) ;
#79513=TOROIDAL_SURFACE('',#101639,0.2,0.1) ;
#79514=TOROIDAL_SURFACE('',#101657,0.2,0.1) ;
#79515=TOROIDAL_SURFACE('',#101667,0.2,0.1) ;
#79516=TOROIDAL_SURFACE('',#101681,0.2,0.1) ;
#79517=TOROIDAL_SURFACE('',#101748,0.2,0.1) ;
#79518=TOROIDAL_SURFACE('',#101755,0.2,0.1) ;
#79519=TOROIDAL_SURFACE('',#101757,0.2,0.1) ;
#79520=TOROIDAL_SURFACE('',#101763,0.2,0.1) ;
#79521=TOROIDAL_SURFACE('',#101791,0.2,0.1) ;
#79522=TOROIDAL_SURFACE('',#101794,0.2,0.1) ;
#79523=TOROIDAL_SURFACE('',#101811,0.2,0.1) ;
#79524=TOROIDAL_SURFACE('',#101817,0.2,0.1) ;
#79525=TOROIDAL_SURFACE('',#101884,1.75625,0.1) ;
#79526=TOROIDAL_SURFACE('',#101891,0.2,0.1) ;
#79527=TOROIDAL_SURFACE('',#101904,1.55625,0.1) ;
#79528=TOROIDAL_SURFACE('',#101913,0.2,0.1) ;
#79529=TOROIDAL_SURFACE('',#101915,0.2,0.1) ;
#79530=TOROIDAL_SURFACE('',#101933,0.2,0.1) ;
#79531=TOROIDAL_SURFACE('',#101943,0.2,0.1) ;
#79532=TOROIDAL_SURFACE('',#101957,0.2,0.1) ;
#79533=TOROIDAL_SURFACE('',#102024,0.2,0.1) ;
#79534=TOROIDAL_SURFACE('',#102031,0.2,0.1) ;
#79535=TOROIDAL_SURFACE('',#102033,0.2,0.1) ;
#79536=TOROIDAL_SURFACE('',#102039,0.2,0.1) ;
#79537=TOROIDAL_SURFACE('',#102067,0.2,0.1) ;
#79538=TOROIDAL_SURFACE('',#102070,0.2,0.1) ;
#79539=TOROIDAL_SURFACE('',#102087,0.2,0.1) ;
#79540=TOROIDAL_SURFACE('',#102093,0.2,0.1) ;
#79541=TOROIDAL_SURFACE('',#102160,1.75625,0.1) ;
#79542=TOROIDAL_SURFACE('',#102167,0.2,0.1) ;
#79543=TOROIDAL_SURFACE('',#102180,1.55625,0.1) ;
#79544=TOROIDAL_SURFACE('',#102189,0.2,0.1) ;
#79545=TOROIDAL_SURFACE('',#102191,0.2,0.1) ;
#79546=TOROIDAL_SURFACE('',#102209,0.2,0.1) ;
#79547=TOROIDAL_SURFACE('',#102219,0.2,0.1) ;
#79548=TOROIDAL_SURFACE('',#102233,0.2,0.1) ;
#79549=TOROIDAL_SURFACE('',#102300,0.2,0.1) ;
#79550=TOROIDAL_SURFACE('',#102307,0.2,0.1) ;
#79551=TOROIDAL_SURFACE('',#102309,0.2,0.1) ;
#79552=TOROIDAL_SURFACE('',#102315,0.2,0.1) ;
#79553=TOROIDAL_SURFACE('',#102343,0.2,0.1) ;
#79554=TOROIDAL_SURFACE('',#102346,0.2,0.1) ;
#79555=TOROIDAL_SURFACE('',#102363,0.2,0.1) ;
#79556=TOROIDAL_SURFACE('',#102369,0.2,0.1) ;
#79557=TOROIDAL_SURFACE('',#102436,1.75625,0.1) ;
#79558=TOROIDAL_SURFACE('',#102443,0.2,0.1) ;
#79559=TOROIDAL_SURFACE('',#102456,1.55625,0.1) ;
#79560=TOROIDAL_SURFACE('',#102465,0.2,0.1) ;
#79561=TOROIDAL_SURFACE('',#102467,0.2,0.1) ;
#79562=TOROIDAL_SURFACE('',#102485,0.2,0.1) ;
#79563=TOROIDAL_SURFACE('',#102495,0.2,0.1) ;
#79564=TOROIDAL_SURFACE('',#102509,0.2,0.1) ;
#79565=TOROIDAL_SURFACE('',#102576,0.2,0.1) ;
#79566=TOROIDAL_SURFACE('',#102583,0.2,0.1) ;
#79567=TOROIDAL_SURFACE('',#102585,0.2,0.1) ;
#79568=TOROIDAL_SURFACE('',#102591,0.2,0.1) ;
#79569=TOROIDAL_SURFACE('',#102619,0.2,0.1) ;
#79570=TOROIDAL_SURFACE('',#102622,0.2,0.1) ;
#79571=TOROIDAL_SURFACE('',#102639,0.2,0.1) ;
#79572=TOROIDAL_SURFACE('',#102645,0.2,0.1) ;
#79573=TOROIDAL_SURFACE('',#102731,0.2,0.1) ;
#79574=TOROIDAL_SURFACE('',#102737,0.2,0.1) ;
#79575=TOROIDAL_SURFACE('',#102738,0.2,0.1) ;
#79576=TOROIDAL_SURFACE('',#102739,0.2,0.1) ;
#79577=TOROIDAL_SURFACE('',#102745,0.2,0.1) ;
#79578=TOROIDAL_SURFACE('',#102746,0.2,0.1) ;
#79579=TOROIDAL_SURFACE('',#102752,0.2,0.1) ;
#79580=TOROIDAL_SURFACE('',#102753,0.2,0.1) ;
#79581=TOROIDAL_SURFACE('',#102759,0.2,0.1) ;
#79582=TOROIDAL_SURFACE('',#102760,0.2,0.1) ;
#79583=TOROIDAL_SURFACE('',#102766,0.2,0.1) ;
#79584=TOROIDAL_SURFACE('',#102767,0.2,0.1) ;
#79585=TOROIDAL_SURFACE('',#102773,0.2,0.1) ;
#79586=TOROIDAL_SURFACE('',#102774,0.2,0.1) ;
#79587=TOROIDAL_SURFACE('',#102780,0.2,0.1) ;
#79588=TOROIDAL_SURFACE('',#102781,0.2,0.1) ;
#79589=TOROIDAL_SURFACE('',#102787,0.2,0.1) ;
#79590=TOROIDAL_SURFACE('',#102792,0.2,0.1) ;
#79591=TOROIDAL_SURFACE('',#102793,0.2,0.1) ;
#79592=TOROIDAL_SURFACE('',#102799,0.2,0.1) ;
#79593=TOROIDAL_SURFACE('',#102805,0.2,0.1) ;
#79594=TOROIDAL_SURFACE('',#102811,0.2,0.1) ;
#79595=TOROIDAL_SURFACE('',#102817,0.2,0.1) ;
#79596=TOROIDAL_SURFACE('',#102823,0.2,0.1) ;
#79597=TOROIDAL_SURFACE('',#102829,0.2,0.1) ;
#79598=TOROIDAL_SURFACE('',#102835,0.2,0.1) ;
#79599=TOROIDAL_SURFACE('',#102841,0.2,0.1) ;
#79600=TOROIDAL_SURFACE('',#102847,0.2,0.1) ;
#79601=TOROIDAL_SURFACE('',#102853,0.2,0.1) ;
#79602=TOROIDAL_SURFACE('',#102859,0.2,0.1) ;
#79603=TOROIDAL_SURFACE('',#102865,0.2,0.1) ;
#79604=TOROIDAL_SURFACE('',#102871,0.2,0.1) ;
#79605=TOROIDAL_SURFACE('',#102877,0.2,0.1) ;
#79606=TOROIDAL_SURFACE('',#102883,0.2,0.1) ;
#79607=TOROIDAL_SURFACE('',#102889,0.2,0.1) ;
#79608=TOROIDAL_SURFACE('',#102895,0.2,0.1) ;
#79609=TOROIDAL_SURFACE('',#102901,0.2,0.1) ;
#79610=TOROIDAL_SURFACE('',#102904,0.2,0.1) ;
#79611=TOROIDAL_SURFACE('',#102905,0.2,0.1) ;
#79612=TOROIDAL_SURFACE('',#102908,0.2,0.1) ;
#79613=TOROIDAL_SURFACE('',#102909,0.2,0.1) ;
#79614=TOROIDAL_SURFACE('',#102912,0.2,0.1) ;
#79615=TOROIDAL_SURFACE('',#102913,0.2,0.1) ;
#79616=TOROIDAL_SURFACE('',#102916,0.2,0.1) ;
#79617=TOROIDAL_SURFACE('',#102917,0.2,0.1) ;
#79618=TOROIDAL_SURFACE('',#102920,0.2,0.1) ;
#79619=TOROIDAL_SURFACE('',#102921,0.2,0.1) ;
#79620=TOROIDAL_SURFACE('',#102924,0.2,0.1) ;
#79621=TOROIDAL_SURFACE('',#102925,0.2,0.1) ;
#79622=TOROIDAL_SURFACE('',#102928,0.2,0.1) ;
#79623=TOROIDAL_SURFACE('',#102929,0.2,0.1) ;
#79624=TOROIDAL_SURFACE('',#102932,0.2,0.1) ;
#79625=TOROIDAL_SURFACE('',#102933,0.2,0.1) ;
#79626=TOROIDAL_SURFACE('',#102936,0.2,0.1) ;
#79627=TOROIDAL_SURFACE('',#102937,0.2,0.1) ;
#79628=TOROIDAL_SURFACE('',#102940,0.2,0.1) ;
#79629=TOROIDAL_SURFACE('',#102941,0.2,0.1) ;
#79630=TOROIDAL_SURFACE('',#102944,0.2,0.1) ;
#79631=TOROIDAL_SURFACE('',#102945,0.2,0.1) ;
#79632=TOROIDAL_SURFACE('',#102948,0.2,0.1) ;
#79633=TOROIDAL_SURFACE('',#102949,0.2,0.1) ;
#79634=TOROIDAL_SURFACE('',#102952,0.2,0.1) ;
#79635=TOROIDAL_SURFACE('',#102953,0.2,0.1) ;
#79636=TOROIDAL_SURFACE('',#102956,0.2,0.1) ;
#79637=TOROIDAL_SURFACE('',#102957,0.2,0.1) ;
#79638=TOROIDAL_SURFACE('',#102960,0.2,0.1) ;
#79639=TOROIDAL_SURFACE('',#102961,0.2,0.1) ;
#79640=TOROIDAL_SURFACE('',#102964,0.2,0.1) ;
#79641=TOROIDAL_SURFACE('',#102965,0.2,0.1) ;
#79642=TOROIDAL_SURFACE('',#102968,0.2,0.1) ;
#79643=TOROIDAL_SURFACE('',#102969,0.2,0.1) ;
#79644=TOROIDAL_SURFACE('',#102972,0.2,0.1) ;
#79645=TOROIDAL_SURFACE('',#102989,0.2,0.1) ;
#79646=TOROIDAL_SURFACE('',#103003,0.2,0.1) ;
#79647=TOROIDAL_SURFACE('',#103014,0.2,0.1) ;
#79648=TOROIDAL_SURFACE('',#103025,2.15,0.1) ;
#79649=TOROIDAL_SURFACE('',#103026,2.15,0.1) ;
#79650=TOROIDAL_SURFACE('',#103027,2.15,0.1) ;
#79651=TOROIDAL_SURFACE('',#103028,2.15,0.1) ;
#79652=TOROIDAL_SURFACE('',#103029,2.15,0.1) ;
#79653=TOROIDAL_SURFACE('',#103030,2.15,0.1) ;
#79654=TOROIDAL_SURFACE('',#103031,2.15,0.1) ;
#79655=TOROIDAL_SURFACE('',#103034,2.15,0.1) ;
#79656=TOROIDAL_SURFACE('',#103037,0.2,0.1) ;
#79657=TOROIDAL_SURFACE('',#103039,2.15,0.1) ;
#79658=TOROIDAL_SURFACE('',#103044,2.15,0.1) ;
#79659=TOROIDAL_SURFACE('',#103049,0.2,0.1) ;
#79660=TOROIDAL_SURFACE('',#103064,0.2,0.1) ;
#83011=STYLED_ITEM('',(#170169),#88718) ;
#83012=STYLED_ITEM('',(#170169),#88719) ;
#83013=STYLED_ITEM('',(#170169),#88720) ;
#83014=STYLED_ITEM('',(#170169),#88721) ;
#83015=STYLED_ITEM('',(#170169),#88722) ;
#83016=STYLED_ITEM('',(#170169),#88723) ;
#83017=STYLED_ITEM('',(#170169),#88724) ;
#83018=STYLED_ITEM('',(#170169),#88725) ;
#83019=STYLED_ITEM('',(#170169),#88726) ;
#83020=STYLED_ITEM('',(#170169),#88727) ;
#83021=STYLED_ITEM('',(#170169),#88728) ;
#83022=STYLED_ITEM('',(#170169),#88729) ;
#83023=STYLED_ITEM('',(#170169),#88730) ;
#83024=STYLED_ITEM('',(#170169),#88731) ;
#83025=STYLED_ITEM('',(#170169),#88732) ;
#83026=STYLED_ITEM('',(#170169),#88733) ;
#83027=STYLED_ITEM('',(#170169),#88734) ;
#83028=STYLED_ITEM('',(#170169),#88735) ;
#83029=STYLED_ITEM('',(#170169),#88736) ;
#83030=STYLED_ITEM('',(#170169),#88737) ;
#83031=STYLED_ITEM('',(#170169),#88738) ;
#83032=STYLED_ITEM('',(#170169),#88739) ;
#83033=STYLED_ITEM('',(#170169),#88740) ;
#83034=STYLED_ITEM('',(#170169),#88741) ;
#83035=STYLED_ITEM('',(#170169),#88742) ;
#83036=STYLED_ITEM('',(#170169),#88743) ;
#83037=STYLED_ITEM('',(#170169),#88744) ;
#83038=STYLED_ITEM('',(#170169),#88745) ;
#83039=STYLED_ITEM('',(#170169),#88746) ;
#83040=STYLED_ITEM('',(#170169),#88747) ;
#83041=STYLED_ITEM('',(#170169),#88748) ;
#83042=STYLED_ITEM('',(#170169),#88749) ;
#83043=STYLED_ITEM('',(#170169),#88750) ;
#83044=STYLED_ITEM('',(#170169),#88751) ;
#83045=STYLED_ITEM('',(#170169),#88752) ;
#83046=STYLED_ITEM('',(#170169),#88753) ;
#83047=STYLED_ITEM('',(#170169),#88754) ;
#83048=STYLED_ITEM('',(#170169),#88755) ;
#83049=STYLED_ITEM('',(#170169),#88756) ;
#83050=STYLED_ITEM('',(#170169),#88757) ;
#83051=STYLED_ITEM('',(#170169),#88758) ;
#83052=STYLED_ITEM('',(#170169),#88759) ;
#83053=STYLED_ITEM('',(#170169),#88760) ;
#83054=STYLED_ITEM('',(#170169),#88761) ;
#83055=STYLED_ITEM('',(#170169),#88762) ;
#83056=STYLED_ITEM('',(#170169),#88763) ;
#83057=STYLED_ITEM('',(#170169),#88764) ;
#83058=STYLED_ITEM('',(#170169),#88765) ;
#83059=STYLED_ITEM('',(#170169),#88766) ;
#83060=STYLED_ITEM('',(#170169),#88767) ;
#83061=STYLED_ITEM('',(#170169),#88768) ;
#83062=STYLED_ITEM('',(#170169),#88769) ;
#83063=STYLED_ITEM('',(#170169),#88770) ;
#83064=STYLED_ITEM('',(#170169),#88771) ;
#83065=STYLED_ITEM('',(#170169),#88772) ;
#83066=STYLED_ITEM('',(#170169),#88773) ;
#83067=STYLED_ITEM('',(#170169),#88774) ;
#83068=STYLED_ITEM('',(#170169),#88775) ;
#83069=STYLED_ITEM('',(#170169),#88776) ;
#83070=STYLED_ITEM('',(#170169),#88777) ;
#83071=STYLED_ITEM('',(#170169),#88778) ;
#83072=STYLED_ITEM('',(#170169),#88779) ;
#83073=STYLED_ITEM('',(#170169),#88780) ;
#83074=STYLED_ITEM('',(#170169),#88781) ;
#83075=STYLED_ITEM('',(#170169),#88782) ;
#83076=STYLED_ITEM('',(#170169),#88783) ;
#83077=STYLED_ITEM('',(#170169),#88784) ;
#83078=STYLED_ITEM('',(#170169),#88785) ;
#83079=STYLED_ITEM('',(#170169),#88786) ;
#83080=STYLED_ITEM('',(#170169),#88787) ;
#83081=STYLED_ITEM('',(#170169),#88788) ;
#83082=STYLED_ITEM('',(#170169),#88789) ;
#83083=STYLED_ITEM('',(#170169),#88790) ;
#83084=STYLED_ITEM('',(#170169),#88791) ;
#83085=STYLED_ITEM('',(#170169),#88792) ;
#83086=STYLED_ITEM('',(#170169),#88793) ;
#83087=STYLED_ITEM('',(#170169),#88794) ;
#83088=STYLED_ITEM('',(#170169),#88795) ;
#83089=STYLED_ITEM('',(#170169),#88796) ;
#83090=STYLED_ITEM('',(#170169),#88797) ;
#83091=STYLED_ITEM('',(#170169),#88798) ;
#83092=STYLED_ITEM('',(#170169),#88799) ;
#83093=STYLED_ITEM('',(#170169),#88800) ;
#83094=STYLED_ITEM('',(#170169),#88801) ;
#83095=STYLED_ITEM('',(#170169),#88802) ;
#83096=STYLED_ITEM('',(#170169),#88803) ;
#83097=STYLED_ITEM('',(#170169),#88804) ;
#83098=STYLED_ITEM('',(#170169),#88805) ;
#83099=STYLED_ITEM('',(#170169),#88806) ;
#83100=STYLED_ITEM('',(#170169),#88807) ;
#83101=STYLED_ITEM('',(#170169),#88808) ;
#83102=STYLED_ITEM('',(#170169),#88809) ;
#83103=STYLED_ITEM('',(#170169),#88810) ;
#83104=STYLED_ITEM('',(#170169),#88811) ;
#83105=STYLED_ITEM('',(#170169),#88812) ;
#83106=STYLED_ITEM('',(#170169),#88813) ;
#83107=STYLED_ITEM('',(#170169),#88814) ;
#83108=STYLED_ITEM('',(#170169),#88815) ;
#83109=STYLED_ITEM('',(#170169),#88816) ;
#83110=STYLED_ITEM('',(#170169),#88817) ;
#83111=STYLED_ITEM('',(#170169),#88818) ;
#83112=STYLED_ITEM('',(#170169),#88819) ;
#83113=STYLED_ITEM('',(#170169),#88820) ;
#83114=STYLED_ITEM('',(#170172),#88821) ;
#83115=STYLED_ITEM('',(#170172),#88822) ;
#83116=STYLED_ITEM('',(#170172),#88823) ;
#83117=STYLED_ITEM('',(#170172),#88824) ;
#83118=STYLED_ITEM('',(#170172),#88825) ;
#83119=STYLED_ITEM('',(#170172),#88826) ;
#83120=STYLED_ITEM('',(#170172),#88827) ;
#83121=STYLED_ITEM('',(#170172),#88828) ;
#83122=STYLED_ITEM('',(#170172),#88829) ;
#83123=STYLED_ITEM('',(#170169),#88830) ;
#83124=STYLED_ITEM('',(#170169),#88831) ;
#83125=STYLED_ITEM('',(#170169),#88832) ;
#83126=STYLED_ITEM('',(#170169),#88833) ;
#83127=STYLED_ITEM('',(#170169),#88834) ;
#83128=STYLED_ITEM('',(#170169),#88835) ;
#83129=STYLED_ITEM('',(#170169),#88836) ;
#83130=STYLED_ITEM('',(#170169),#88837) ;
#83131=STYLED_ITEM('',(#170169),#88838) ;
#83132=STYLED_ITEM('',(#170169),#88839) ;
#83133=STYLED_ITEM('',(#170169),#88840) ;
#83134=STYLED_ITEM('',(#170169),#88841) ;
#83135=STYLED_ITEM('',(#170169),#88842) ;
#83136=STYLED_ITEM('',(#170169),#88843) ;
#83137=STYLED_ITEM('',(#170169),#88844) ;
#83138=STYLED_ITEM('',(#170169),#88845) ;
#83139=STYLED_ITEM('',(#170169),#88846) ;
#83140=STYLED_ITEM('',(#170172),#88847) ;
#83141=STYLED_ITEM('',(#170169),#88848) ;
#83142=STYLED_ITEM('',(#170169),#88849) ;
#83143=STYLED_ITEM('',(#170169),#88850) ;
#83144=STYLED_ITEM('',(#170169),#88851) ;
#83145=STYLED_ITEM('',(#170169),#88852) ;
#83146=STYLED_ITEM('',(#170169),#88853) ;
#83147=STYLED_ITEM('',(#170169),#88854) ;
#83148=STYLED_ITEM('',(#170169),#88855) ;
#83149=STYLED_ITEM('',(#170169),#88856) ;
#83150=STYLED_ITEM('',(#170171),#88857) ;
#83151=STYLED_ITEM('',(#170169),#88858) ;
#83152=STYLED_ITEM('',(#170169),#88859) ;
#83153=STYLED_ITEM('',(#170169),#88860) ;
#83154=STYLED_ITEM('',(#170169),#88861) ;
#83155=STYLED_ITEM('',(#170169),#88862) ;
#83156=STYLED_ITEM('',(#170169),#88863) ;
#83157=STYLED_ITEM('',(#170169),#88864) ;
#83158=STYLED_ITEM('',(#170169),#88865) ;
#83159=STYLED_ITEM('',(#170169),#88866) ;
#83160=STYLED_ITEM('',(#170169),#88867) ;
#83161=STYLED_ITEM('',(#170169),#88868) ;
#83162=STYLED_ITEM('',(#170169),#88869) ;
#83163=STYLED_ITEM('',(#170169),#88870) ;
#83164=STYLED_ITEM('',(#170169),#88871) ;
#83165=STYLED_ITEM('',(#170169),#88872) ;
#83166=STYLED_ITEM('',(#170169),#88873) ;
#83167=STYLED_ITEM('',(#170169),#88874) ;
#83168=STYLED_ITEM('',(#170169),#88875) ;
#83169=STYLED_ITEM('',(#170169),#88876) ;
#83170=STYLED_ITEM('',(#170169),#88877) ;
#83171=STYLED_ITEM('',(#170169),#88878) ;
#83172=STYLED_ITEM('',(#170169),#88879) ;
#83173=STYLED_ITEM('',(#170169),#88880) ;
#83174=STYLED_ITEM('',(#170169),#88881) ;
#83175=STYLED_ITEM('',(#170171),#88882) ;
#83176=STYLED_ITEM('',(#170169),#88883) ;
#83177=STYLED_ITEM('',(#170169),#88884) ;
#83178=STYLED_ITEM('',(#170169),#88885) ;
#83179=STYLED_ITEM('',(#170169),#88886) ;
#83180=STYLED_ITEM('',(#170169),#88887) ;
#83181=STYLED_ITEM('',(#170169),#88888) ;
#83182=STYLED_ITEM('',(#170169),#88889) ;
#83183=STYLED_ITEM('',(#170169),#88890) ;
#83184=STYLED_ITEM('',(#170169),#88891) ;
#83185=STYLED_ITEM('',(#170169),#88892) ;
#83186=STYLED_ITEM('',(#170172),#88893) ;
#83187=STYLED_ITEM('',(#170172),#88894) ;
#83188=STYLED_ITEM('',(#170172),#88895) ;
#83189=STYLED_ITEM('',(#170172),#88896) ;
#83190=STYLED_ITEM('',(#170169),#88897) ;
#83191=STYLED_ITEM('',(#170169),#88898) ;
#83192=STYLED_ITEM('',(#170169),#88899) ;
#83193=STYLED_ITEM('',(#170169),#88900) ;
#83194=STYLED_ITEM('',(#170169),#88901) ;
#83195=STYLED_ITEM('',(#170169),#88902) ;
#83196=STYLED_ITEM('',(#170169),#88903) ;
#83197=STYLED_ITEM('',(#170169),#88904) ;
#83198=STYLED_ITEM('',(#170169),#88905) ;
#83199=STYLED_ITEM('',(#170169),#88906) ;
#83200=STYLED_ITEM('',(#170169),#88907) ;
#83201=STYLED_ITEM('',(#170169),#88908) ;
#83202=STYLED_ITEM('',(#170169),#88909) ;
#83203=STYLED_ITEM('',(#170169),#88910) ;
#83204=STYLED_ITEM('',(#170169),#88911) ;
#83205=STYLED_ITEM('',(#170169),#88912) ;
#83206=STYLED_ITEM('',(#170169),#88913) ;
#83207=STYLED_ITEM('',(#170169),#88914) ;
#83208=STYLED_ITEM('',(#170169),#88915) ;
#83209=STYLED_ITEM('',(#170169),#88916) ;
#83210=STYLED_ITEM('',(#170169),#88918) ;
#83211=STYLED_ITEM('',(#170169),#88919) ;
#83212=STYLED_ITEM('',(#170169),#88920) ;
#83213=STYLED_ITEM('',(#170169),#88922) ;
#83214=STYLED_ITEM('',(#170169),#88923) ;
#83215=STYLED_ITEM('',(#170169),#88924) ;
#83216=STYLED_ITEM('',(#170169),#88925) ;
#83217=STYLED_ITEM('',(#170169),#88926) ;
#83218=STYLED_ITEM('',(#170169),#88929) ;
#83219=STYLED_ITEM('',(#170169),#88930) ;
#83220=STYLED_ITEM('',(#170169),#88933) ;
#83221=STYLED_ITEM('',(#170169),#88938) ;
#83222=STYLED_ITEM('',(#170169),#88939) ;
#83223=STYLED_ITEM('',(#170169),#88940) ;
#83224=STYLED_ITEM('',(#170169),#88941) ;
#83225=STYLED_ITEM('',(#170169),#88942) ;
#83226=STYLED_ITEM('',(#170169),#88943) ;
#83227=STYLED_ITEM('',(#170169),#88944) ;
#83228=STYLED_ITEM('',(#170169),#88945) ;
#83229=STYLED_ITEM('',(#170169),#88946) ;
#83230=STYLED_ITEM('',(#170169),#88947) ;
#83231=STYLED_ITEM('',(#170169),#88948) ;
#83232=STYLED_ITEM('',(#170169),#88949) ;
#83233=STYLED_ITEM('',(#170169),#88950) ;
#83234=STYLED_ITEM('',(#170169),#88951) ;
#83235=STYLED_ITEM('',(#170169),#88952) ;
#83236=STYLED_ITEM('',(#170169),#88953) ;
#83237=STYLED_ITEM('',(#170169),#88954) ;
#83238=STYLED_ITEM('',(#170169),#88955) ;
#83239=STYLED_ITEM('',(#170169),#88956) ;
#83240=STYLED_ITEM('',(#170169),#88957) ;
#83241=STYLED_ITEM('',(#170169),#88958) ;
#83242=STYLED_ITEM('',(#170169),#88959) ;
#83243=STYLED_ITEM('',(#170169),#88960) ;
#83244=STYLED_ITEM('',(#170169),#88961) ;
#83245=STYLED_ITEM('',(#170169),#88962) ;
#83246=STYLED_ITEM('',(#170169),#88963) ;
#83247=STYLED_ITEM('',(#170169),#88964) ;
#83248=STYLED_ITEM('',(#170169),#88965) ;
#83249=STYLED_ITEM('',(#170169),#88966) ;
#83250=STYLED_ITEM('',(#170169),#88967) ;
#83251=STYLED_ITEM('',(#170169),#88968) ;
#83252=STYLED_ITEM('',(#170169),#88969) ;
#83253=STYLED_ITEM('',(#170169),#88970) ;
#83254=STYLED_ITEM('',(#170169),#88971) ;
#83255=STYLED_ITEM('',(#170169),#88972) ;
#83256=STYLED_ITEM('',(#170169),#88973) ;
#83257=STYLED_ITEM('',(#170169),#88974) ;
#83258=STYLED_ITEM('',(#170169),#88975) ;
#83259=STYLED_ITEM('',(#170169),#88976) ;
#83260=STYLED_ITEM('',(#170169),#88977) ;
#83261=STYLED_ITEM('',(#170169),#88978) ;
#83262=STYLED_ITEM('',(#170169),#88979) ;
#83263=STYLED_ITEM('',(#170169),#88980) ;
#83264=STYLED_ITEM('',(#170169),#88981) ;
#83265=STYLED_ITEM('',(#170169),#88982) ;
#83266=STYLED_ITEM('',(#170169),#88983) ;
#83267=STYLED_ITEM('',(#170169),#88984) ;
#83268=STYLED_ITEM('',(#170169),#88985) ;
#83269=STYLED_ITEM('',(#170169),#88986) ;
#83270=STYLED_ITEM('',(#170169),#88987) ;
#83271=STYLED_ITEM('',(#170169),#88988) ;
#83272=STYLED_ITEM('',(#170169),#88989) ;
#83273=STYLED_ITEM('',(#170169),#88990) ;
#83274=STYLED_ITEM('',(#170169),#88991) ;
#83275=STYLED_ITEM('',(#170169),#88992) ;
#83276=STYLED_ITEM('',(#170169),#88993) ;
#83277=STYLED_ITEM('',(#170169),#88994) ;
#83278=STYLED_ITEM('',(#170169),#88995) ;
#83279=STYLED_ITEM('',(#170169),#88996) ;
#83280=STYLED_ITEM('',(#170169),#88997) ;
#83281=STYLED_ITEM('',(#170169),#88998) ;
#83282=STYLED_ITEM('',(#170169),#88999) ;
#83283=STYLED_ITEM('',(#170169),#89000) ;
#83284=STYLED_ITEM('',(#170169),#89001) ;
#83285=STYLED_ITEM('',(#170169),#89002) ;
#83286=STYLED_ITEM('',(#170169),#89003) ;
#83287=STYLED_ITEM('',(#170169),#89004) ;
#83288=STYLED_ITEM('',(#170169),#89005) ;
#83289=STYLED_ITEM('',(#170169),#89006) ;
#83290=STYLED_ITEM('',(#170169),#89007) ;
#83291=STYLED_ITEM('',(#170169),#89008) ;
#83292=STYLED_ITEM('',(#170169),#89009) ;
#83293=STYLED_ITEM('',(#170169),#89010) ;
#83294=STYLED_ITEM('',(#170169),#89011) ;
#83295=STYLED_ITEM('',(#170169),#89012) ;
#83296=STYLED_ITEM('',(#170169),#89013) ;
#83297=STYLED_ITEM('',(#170169),#89014) ;
#83298=STYLED_ITEM('',(#170169),#89015) ;
#83299=STYLED_ITEM('',(#170169),#89016) ;
#83300=STYLED_ITEM('',(#170169),#89017) ;
#83301=STYLED_ITEM('',(#170169),#89018) ;
#83302=STYLED_ITEM('',(#170169),#89019) ;
#83303=STYLED_ITEM('',(#170169),#89020) ;
#83304=STYLED_ITEM('',(#170169),#89021) ;
#83305=STYLED_ITEM('',(#170169),#89022) ;
#83306=STYLED_ITEM('',(#170169),#89023) ;
#83307=STYLED_ITEM('',(#170169),#89024) ;
#83308=STYLED_ITEM('',(#170169),#89025) ;
#83309=STYLED_ITEM('',(#170169),#89026) ;
#83310=STYLED_ITEM('',(#170169),#89027) ;
#83311=STYLED_ITEM('',(#170169),#89028) ;
#83312=STYLED_ITEM('',(#170169),#89029) ;
#83313=STYLED_ITEM('',(#170169),#89030) ;
#83314=STYLED_ITEM('',(#170169),#89031) ;
#83315=STYLED_ITEM('',(#170169),#89032) ;
#83316=STYLED_ITEM('',(#170169),#89033) ;
#83317=STYLED_ITEM('',(#170169),#89034) ;
#83318=STYLED_ITEM('',(#170169),#89035) ;
#83319=STYLED_ITEM('',(#170169),#89036) ;
#83320=STYLED_ITEM('',(#170169),#89037) ;
#83321=STYLED_ITEM('',(#170169),#89038) ;
#83322=STYLED_ITEM('',(#170169),#89039) ;
#83323=STYLED_ITEM('',(#170169),#89040) ;
#83324=STYLED_ITEM('',(#170169),#89041) ;
#83325=STYLED_ITEM('',(#170169),#89042) ;
#83326=STYLED_ITEM('',(#170169),#89043) ;
#83327=STYLED_ITEM('',(#170169),#89044) ;
#83328=STYLED_ITEM('',(#170169),#89045) ;
#83329=STYLED_ITEM('',(#170169),#89046) ;
#83330=STYLED_ITEM('',(#170169),#89047) ;
#83331=STYLED_ITEM('',(#170169),#89048) ;
#83332=STYLED_ITEM('',(#170169),#89049) ;
#83333=STYLED_ITEM('',(#170169),#89050) ;
#83334=STYLED_ITEM('',(#170169),#89051) ;
#83335=STYLED_ITEM('',(#170169),#89052) ;
#83336=STYLED_ITEM('',(#170169),#89053) ;
#83337=STYLED_ITEM('',(#170169),#89054) ;
#83338=STYLED_ITEM('',(#170169),#89055) ;
#83339=STYLED_ITEM('',(#170169),#89056) ;
#83340=STYLED_ITEM('',(#170169),#89057) ;
#83341=STYLED_ITEM('',(#170169),#89058) ;
#83342=STYLED_ITEM('',(#170169),#89059) ;
#83343=STYLED_ITEM('',(#170169),#89060) ;
#83344=STYLED_ITEM('',(#170169),#89061) ;
#83345=STYLED_ITEM('',(#170169),#89062) ;
#83346=STYLED_ITEM('',(#170169),#89063) ;
#83347=STYLED_ITEM('',(#170169),#89064) ;
#83348=STYLED_ITEM('',(#170169),#89065) ;
#83349=STYLED_ITEM('',(#170169),#89066) ;
#83350=STYLED_ITEM('',(#170169),#89067) ;
#83351=STYLED_ITEM('',(#170169),#89068) ;
#83352=STYLED_ITEM('',(#170169),#89069) ;
#83353=STYLED_ITEM('',(#170169),#89070) ;
#83354=STYLED_ITEM('',(#170169),#89071) ;
#83355=STYLED_ITEM('',(#170169),#89072) ;
#83356=STYLED_ITEM('',(#170169),#89073) ;
#83357=STYLED_ITEM('',(#170169),#89074) ;
#83358=STYLED_ITEM('',(#170169),#89075) ;
#83359=STYLED_ITEM('',(#170169),#89076) ;
#83360=STYLED_ITEM('',(#170169),#89077) ;
#83361=STYLED_ITEM('',(#170169),#89078) ;
#83362=STYLED_ITEM('',(#170172),#89079) ;
#83363=STYLED_ITEM('',(#170172),#89080) ;
#83364=STYLED_ITEM('',(#170172),#89081) ;
#83365=STYLED_ITEM('',(#170172),#89082) ;
#83366=STYLED_ITEM('',(#170169),#89083) ;
#83367=STYLED_ITEM('',(#170169),#89084) ;
#83368=STYLED_ITEM('',(#170169),#89085) ;
#83369=STYLED_ITEM('',(#170169),#89086) ;
#83370=STYLED_ITEM('',(#170169),#89087) ;
#83371=STYLED_ITEM('',(#170169),#89088) ;
#83372=STYLED_ITEM('',(#170169),#89089) ;
#83373=STYLED_ITEM('',(#170169),#89090) ;
#83374=STYLED_ITEM('',(#170169),#89091) ;
#83375=STYLED_ITEM('',(#170169),#89092) ;
#83376=STYLED_ITEM('',(#170169),#89093) ;
#83377=STYLED_ITEM('',(#170169),#89094) ;
#83378=STYLED_ITEM('',(#170169),#89095) ;
#83379=STYLED_ITEM('',(#170169),#89096) ;
#83380=STYLED_ITEM('',(#170169),#89097) ;
#83381=STYLED_ITEM('',(#170169),#89098) ;
#83382=STYLED_ITEM('',(#170169),#89099) ;
#83383=STYLED_ITEM('',(#170169),#89100) ;
#83384=STYLED_ITEM('',(#170171),#89101) ;
#83385=STYLED_ITEM('',(#170169),#89102) ;
#83386=STYLED_ITEM('',(#170169),#89103) ;
#83387=STYLED_ITEM('',(#170169),#89104) ;
#83388=STYLED_ITEM('',(#170169),#89105) ;
#83389=STYLED_ITEM('',(#170171),#89106) ;
#83390=STYLED_ITEM('',(#170169),#89107) ;
#83391=STYLED_ITEM('',(#170169),#89108) ;
#83392=STYLED_ITEM('',(#170169),#89109) ;
#83393=STYLED_ITEM('',(#170169),#89110) ;
#83394=STYLED_ITEM('',(#170171),#89111) ;
#83395=STYLED_ITEM('',(#170169),#89112) ;
#83396=STYLED_ITEM('',(#170169),#89113) ;
#83397=STYLED_ITEM('',(#170169),#89114) ;
#83398=STYLED_ITEM('',(#170169),#89115) ;
#83399=STYLED_ITEM('',(#170171),#89116) ;
#83400=STYLED_ITEM('',(#170169),#89117) ;
#83401=STYLED_ITEM('',(#170169),#89118) ;
#83402=STYLED_ITEM('',(#170169),#89119) ;
#83403=STYLED_ITEM('',(#170169),#89120) ;
#83404=STYLED_ITEM('',(#170171),#89121) ;
#83405=STYLED_ITEM('',(#170169),#89122) ;
#83406=STYLED_ITEM('',(#170169),#89123) ;
#83407=STYLED_ITEM('',(#170169),#89124) ;
#83408=STYLED_ITEM('',(#170169),#89125) ;
#83409=STYLED_ITEM('',(#170171),#89126) ;
#83410=STYLED_ITEM('',(#170169),#89127) ;
#83411=STYLED_ITEM('',(#170169),#89128) ;
#83412=STYLED_ITEM('',(#170169),#89129) ;
#83413=STYLED_ITEM('',(#170169),#89130) ;
#83414=STYLED_ITEM('',(#170171),#89131) ;
#83415=STYLED_ITEM('',(#170169),#89132) ;
#83416=STYLED_ITEM('',(#170169),#89133) ;
#83417=STYLED_ITEM('',(#170169),#89134) ;
#83418=STYLED_ITEM('',(#170169),#89135) ;
#83419=STYLED_ITEM('',(#170171),#89136) ;
#83420=STYLED_ITEM('',(#170169),#89137) ;
#83421=STYLED_ITEM('',(#170169),#89138) ;
#83422=STYLED_ITEM('',(#170169),#89139) ;
#83423=STYLED_ITEM('',(#170169),#89140) ;
#83424=STYLED_ITEM('',(#170171),#89141) ;
#83425=STYLED_ITEM('',(#170169),#89142) ;
#83426=STYLED_ITEM('',(#170169),#89143) ;
#83427=STYLED_ITEM('',(#170169),#89144) ;
#83428=STYLED_ITEM('',(#170169),#89145) ;
#83429=STYLED_ITEM('',(#170169),#89146) ;
#83430=STYLED_ITEM('',(#170169),#89147) ;
#83431=STYLED_ITEM('',(#170169),#89148) ;
#83432=STYLED_ITEM('',(#170169),#89149) ;
#83433=STYLED_ITEM('',(#170169),#89150) ;
#83434=STYLED_ITEM('',(#170169),#89151) ;
#83435=STYLED_ITEM('',(#170169),#89152) ;
#83436=STYLED_ITEM('',(#170169),#89153) ;
#83437=STYLED_ITEM('',(#170169),#89154) ;
#83438=STYLED_ITEM('',(#170169),#89155) ;
#83439=STYLED_ITEM('',(#170169),#89156) ;
#83440=STYLED_ITEM('',(#170169),#89157) ;
#83441=STYLED_ITEM('',(#170169),#89158) ;
#83442=STYLED_ITEM('',(#170169),#89159) ;
#83443=STYLED_ITEM('',(#170169),#89160) ;
#83444=STYLED_ITEM('',(#170169),#89161) ;
#83445=STYLED_ITEM('',(#170169),#89162) ;
#83446=STYLED_ITEM('',(#170169),#89163) ;
#83447=STYLED_ITEM('',(#170169),#89164) ;
#83448=STYLED_ITEM('',(#170169),#89165) ;
#83449=STYLED_ITEM('',(#170169),#89166) ;
#83450=STYLED_ITEM('',(#170169),#89167) ;
#83451=STYLED_ITEM('',(#170169),#89168) ;
#83452=STYLED_ITEM('',(#170169),#89169) ;
#83453=STYLED_ITEM('',(#170169),#89170) ;
#83454=STYLED_ITEM('',(#170169),#89171) ;
#83455=STYLED_ITEM('',(#170169),#89172) ;
#83456=STYLED_ITEM('',(#170169),#89173) ;
#83457=STYLED_ITEM('',(#170169),#89174) ;
#83458=STYLED_ITEM('',(#170169),#89175) ;
#83459=STYLED_ITEM('',(#170169),#89176) ;
#83460=STYLED_ITEM('',(#170169),#89177) ;
#83461=STYLED_ITEM('',(#170169),#89178) ;
#83462=STYLED_ITEM('',(#170169),#89179) ;
#83463=STYLED_ITEM('',(#170169),#89180) ;
#83464=STYLED_ITEM('',(#170169),#89181) ;
#83465=STYLED_ITEM('',(#170169),#89182) ;
#83466=STYLED_ITEM('',(#170169),#89183) ;
#83467=STYLED_ITEM('',(#170169),#89184) ;
#83468=STYLED_ITEM('',(#170169),#89185) ;
#83469=STYLED_ITEM('',(#170169),#89186) ;
#83470=STYLED_ITEM('',(#170169),#89187) ;
#83471=STYLED_ITEM('',(#170169),#89188) ;
#83472=STYLED_ITEM('',(#170169),#89189) ;
#83473=STYLED_ITEM('',(#170169),#89190) ;
#83474=STYLED_ITEM('',(#170169),#89191) ;
#83475=STYLED_ITEM('',(#170169),#89192) ;
#83476=STYLED_ITEM('',(#170169),#89193) ;
#83477=STYLED_ITEM('',(#170169),#89194) ;
#83478=STYLED_ITEM('',(#170169),#89195) ;
#83479=STYLED_ITEM('',(#170169),#89196) ;
#83480=STYLED_ITEM('',(#170169),#89197) ;
#83481=STYLED_ITEM('',(#170169),#89198) ;
#83482=STYLED_ITEM('',(#170169),#89199) ;
#83483=STYLED_ITEM('',(#170169),#89200) ;
#83484=STYLED_ITEM('',(#170169),#89201) ;
#83485=STYLED_ITEM('',(#170169),#89202) ;
#83486=STYLED_ITEM('',(#170169),#89203) ;
#83487=STYLED_ITEM('',(#170169),#89204) ;
#83488=STYLED_ITEM('',(#170169),#89205) ;
#83489=STYLED_ITEM('',(#170169),#89206) ;
#83490=STYLED_ITEM('',(#170169),#89207) ;
#83491=STYLED_ITEM('',(#170169),#89208) ;
#83492=STYLED_ITEM('',(#170169),#89209) ;
#83493=STYLED_ITEM('',(#170169),#89210) ;
#83494=STYLED_ITEM('',(#170169),#89211) ;
#83495=STYLED_ITEM('',(#170169),#89212) ;
#83496=STYLED_ITEM('',(#170169),#89213) ;
#83497=STYLED_ITEM('',(#170169),#89214) ;
#83498=STYLED_ITEM('',(#170169),#89215) ;
#83499=STYLED_ITEM('',(#170169),#89216) ;
#83500=STYLED_ITEM('',(#170169),#89217) ;
#83501=STYLED_ITEM('',(#170169),#89218) ;
#83502=STYLED_ITEM('',(#170169),#89219) ;
#83503=STYLED_ITEM('',(#170169),#89220) ;
#83504=STYLED_ITEM('',(#170169),#89221) ;
#83505=STYLED_ITEM('',(#170169),#89222) ;
#83506=STYLED_ITEM('',(#170169),#89223) ;
#83507=STYLED_ITEM('',(#170169),#89224) ;
#83508=STYLED_ITEM('',(#170169),#89225) ;
#83509=STYLED_ITEM('',(#170169),#89226) ;
#83510=STYLED_ITEM('',(#170169),#89227) ;
#83511=STYLED_ITEM('',(#170169),#89228) ;
#83512=STYLED_ITEM('',(#170169),#89229) ;
#83513=STYLED_ITEM('',(#170169),#89230) ;
#83514=STYLED_ITEM('',(#170169),#89231) ;
#83515=STYLED_ITEM('',(#170169),#89232) ;
#83516=STYLED_ITEM('',(#170169),#89233) ;
#83517=STYLED_ITEM('',(#170169),#89234) ;
#83518=STYLED_ITEM('',(#170169),#89235) ;
#83519=STYLED_ITEM('',(#170169),#89236) ;
#83520=STYLED_ITEM('',(#170169),#89237) ;
#83521=STYLED_ITEM('',(#170169),#89238) ;
#83522=STYLED_ITEM('',(#170169),#89239) ;
#83523=STYLED_ITEM('',(#170169),#89240) ;
#83524=STYLED_ITEM('',(#170169),#89241) ;
#83525=STYLED_ITEM('',(#170169),#89242) ;
#83526=STYLED_ITEM('',(#170169),#89243) ;
#83527=STYLED_ITEM('',(#170169),#89244) ;
#83528=STYLED_ITEM('',(#170169),#89245) ;
#83529=STYLED_ITEM('',(#170169),#89246) ;
#83530=STYLED_ITEM('',(#170169),#89247) ;
#83531=STYLED_ITEM('',(#170169),#89248) ;
#83532=STYLED_ITEM('',(#170169),#89249) ;
#83533=STYLED_ITEM('',(#170169),#89250) ;
#83534=STYLED_ITEM('',(#170169),#89251) ;
#83535=STYLED_ITEM('',(#170169),#89252) ;
#83536=STYLED_ITEM('',(#170169),#89253) ;
#83537=STYLED_ITEM('',(#170169),#89254) ;
#83538=STYLED_ITEM('',(#170169),#89255) ;
#83539=STYLED_ITEM('',(#170169),#89256) ;
#83540=STYLED_ITEM('',(#170169),#89257) ;
#83541=STYLED_ITEM('',(#170169),#89258) ;
#83542=STYLED_ITEM('',(#170169),#89259) ;
#83543=STYLED_ITEM('',(#170169),#89260) ;
#83544=STYLED_ITEM('',(#170169),#89261) ;
#83545=STYLED_ITEM('',(#170169),#89262) ;
#83546=STYLED_ITEM('',(#170169),#89263) ;
#83547=STYLED_ITEM('',(#170169),#89264) ;
#83548=STYLED_ITEM('',(#170169),#89265) ;
#83549=STYLED_ITEM('',(#170169),#89266) ;
#83550=STYLED_ITEM('',(#170169),#89267) ;
#83551=STYLED_ITEM('',(#170169),#89268) ;
#83552=STYLED_ITEM('',(#170169),#89269) ;
#83553=STYLED_ITEM('',(#170169),#89270) ;
#83554=STYLED_ITEM('',(#170169),#89271) ;
#83555=STYLED_ITEM('',(#170169),#89272) ;
#83556=STYLED_ITEM('',(#170169),#89273) ;
#83557=STYLED_ITEM('',(#170169),#89274) ;
#83558=STYLED_ITEM('',(#170169),#89275) ;
#83559=STYLED_ITEM('',(#170169),#89276) ;
#83560=STYLED_ITEM('',(#170169),#89277) ;
#83561=STYLED_ITEM('',(#170169),#89278) ;
#83562=STYLED_ITEM('',(#170169),#89279) ;
#83563=STYLED_ITEM('',(#170169),#89280) ;
#83564=STYLED_ITEM('',(#170169),#89281) ;
#83565=STYLED_ITEM('',(#170169),#89282) ;
#83566=STYLED_ITEM('',(#170169),#89283) ;
#83567=STYLED_ITEM('',(#170169),#89284) ;
#83568=STYLED_ITEM('',(#170169),#89285) ;
#83569=STYLED_ITEM('',(#170169),#89286) ;
#83570=STYLED_ITEM('',(#170169),#89287) ;
#83571=STYLED_ITEM('',(#170169),#89288) ;
#83572=STYLED_ITEM('',(#170169),#89289) ;
#83573=STYLED_ITEM('',(#170169),#89290) ;
#83574=STYLED_ITEM('',(#170169),#89291) ;
#83575=STYLED_ITEM('',(#170169),#89292) ;
#83576=STYLED_ITEM('',(#170169),#89293) ;
#83577=STYLED_ITEM('',(#170169),#89294) ;
#83578=STYLED_ITEM('',(#170169),#89295) ;
#83579=STYLED_ITEM('',(#170169),#89296) ;
#83580=STYLED_ITEM('',(#170169),#89297) ;
#83581=STYLED_ITEM('',(#170169),#89298) ;
#83582=STYLED_ITEM('',(#170169),#89299) ;
#83583=STYLED_ITEM('',(#170169),#89300) ;
#83584=STYLED_ITEM('',(#170169),#89301) ;
#83585=STYLED_ITEM('',(#170169),#89302) ;
#83586=STYLED_ITEM('',(#170169),#89303) ;
#83587=STYLED_ITEM('',(#170169),#89304) ;
#83588=STYLED_ITEM('',(#170169),#89305) ;
#83589=STYLED_ITEM('',(#170169),#89306) ;
#83590=STYLED_ITEM('',(#170169),#89307) ;
#83591=STYLED_ITEM('',(#170169),#89308) ;
#83592=STYLED_ITEM('',(#170169),#89309) ;
#83593=STYLED_ITEM('',(#170169),#89310) ;
#83594=STYLED_ITEM('',(#170169),#89311) ;
#83595=STYLED_ITEM('',(#170169),#89312) ;
#83596=STYLED_ITEM('',(#170169),#89313) ;
#83597=STYLED_ITEM('',(#170169),#89314) ;
#83598=STYLED_ITEM('',(#170169),#89315) ;
#83599=STYLED_ITEM('',(#170169),#89316) ;
#83600=STYLED_ITEM('',(#170169),#89317) ;
#83601=STYLED_ITEM('',(#170169),#89318) ;
#83602=STYLED_ITEM('',(#170169),#89319) ;
#83603=STYLED_ITEM('',(#170169),#89320) ;
#83604=STYLED_ITEM('',(#170169),#89321) ;
#83605=STYLED_ITEM('',(#170169),#89322) ;
#83606=STYLED_ITEM('',(#170169),#89323) ;
#83607=STYLED_ITEM('',(#170171),#89324) ;
#83608=STYLED_ITEM('',(#170171),#89325) ;
#83609=STYLED_ITEM('',(#170171),#89326) ;
#83610=STYLED_ITEM('',(#170171),#89327) ;
#83611=STYLED_ITEM('',(#170171),#89328) ;
#83612=STYLED_ITEM('',(#170171),#89329) ;
#83613=STYLED_ITEM('',(#170171),#89330) ;
#83614=STYLED_ITEM('',(#170171),#89331) ;
#83615=STYLED_ITEM('',(#170171),#89332) ;
#83616=STYLED_ITEM('',(#170169),#89333) ;
#83617=STYLED_ITEM('',(#170169),#89334) ;
#83618=STYLED_ITEM('',(#170169),#89335) ;
#83619=STYLED_ITEM('',(#170169),#89336) ;
#83620=STYLED_ITEM('',(#170169),#89337) ;
#83621=STYLED_ITEM('',(#170169),#89338) ;
#83622=STYLED_ITEM('',(#170169),#89339) ;
#83623=STYLED_ITEM('',(#170169),#89340) ;
#83624=STYLED_ITEM('',(#170169),#89341) ;
#83625=STYLED_ITEM('',(#170169),#89342) ;
#83626=STYLED_ITEM('',(#170169),#89343) ;
#83627=STYLED_ITEM('',(#170169),#89344) ;
#83628=STYLED_ITEM('',(#170169),#89345) ;
#83629=STYLED_ITEM('',(#170169),#89346) ;
#83630=STYLED_ITEM('',(#170169),#89347) ;
#83631=STYLED_ITEM('',(#170169),#89348) ;
#83632=STYLED_ITEM('',(#170169),#89349) ;
#83633=STYLED_ITEM('',(#170169),#89350) ;
#83634=STYLED_ITEM('',(#170169),#89351) ;
#83635=STYLED_ITEM('',(#170169),#89352) ;
#83636=STYLED_ITEM('',(#170169),#89353) ;
#83637=STYLED_ITEM('',(#170169),#89354) ;
#83638=STYLED_ITEM('',(#170169),#89355) ;
#83639=STYLED_ITEM('',(#170169),#89356) ;
#83640=STYLED_ITEM('',(#170169),#89357) ;
#83641=STYLED_ITEM('',(#170169),#89358) ;
#83642=STYLED_ITEM('',(#170169),#89359) ;
#83643=STYLED_ITEM('',(#170169),#89360) ;
#83644=STYLED_ITEM('',(#170169),#89361) ;
#83645=STYLED_ITEM('',(#170169),#89362) ;
#83646=STYLED_ITEM('',(#170169),#89363) ;
#83647=STYLED_ITEM('',(#170169),#89364) ;
#83648=STYLED_ITEM('',(#170169),#89365) ;
#83649=STYLED_ITEM('',(#170169),#89366) ;
#83650=STYLED_ITEM('',(#170169),#89367) ;
#83651=STYLED_ITEM('',(#170169),#89368) ;
#83652=STYLED_ITEM('',(#170169),#89369) ;
#83653=STYLED_ITEM('',(#170169),#89370) ;
#83654=STYLED_ITEM('',(#170169),#89371) ;
#83655=STYLED_ITEM('',(#170169),#89372) ;
#83656=STYLED_ITEM('',(#170169),#89373) ;
#83657=STYLED_ITEM('',(#170169),#89374) ;
#83658=STYLED_ITEM('',(#170169),#89375) ;
#83659=STYLED_ITEM('',(#170169),#89376) ;
#83660=STYLED_ITEM('',(#170169),#89377) ;
#83661=STYLED_ITEM('',(#170169),#89378) ;
#83662=STYLED_ITEM('',(#170169),#89379) ;
#83663=STYLED_ITEM('',(#170169),#89380) ;
#83664=STYLED_ITEM('',(#170169),#89381) ;
#83665=STYLED_ITEM('',(#170169),#89382) ;
#83666=STYLED_ITEM('',(#170169),#89383) ;
#83667=STYLED_ITEM('',(#170169),#89384) ;
#83668=STYLED_ITEM('',(#170169),#89385) ;
#83669=STYLED_ITEM('',(#170169),#89386) ;
#83670=STYLED_ITEM('',(#170169),#89387) ;
#83671=STYLED_ITEM('',(#170169),#89388) ;
#83672=STYLED_ITEM('',(#170169),#89389) ;
#83673=STYLED_ITEM('',(#170169),#89390) ;
#83674=STYLED_ITEM('',(#170169),#89391) ;
#83675=STYLED_ITEM('',(#170169),#89392) ;
#83676=STYLED_ITEM('',(#170169),#89393) ;
#83677=STYLED_ITEM('',(#170169),#89394) ;
#83678=STYLED_ITEM('',(#170169),#89395) ;
#83679=STYLED_ITEM('',(#170169),#89396) ;
#83680=STYLED_ITEM('',(#170169),#89397) ;
#83681=STYLED_ITEM('',(#170169),#89398) ;
#83682=STYLED_ITEM('',(#170169),#89399) ;
#83683=STYLED_ITEM('',(#170169),#89400) ;
#83684=STYLED_ITEM('',(#170169),#89401) ;
#83685=STYLED_ITEM('',(#170169),#89402) ;
#83686=STYLED_ITEM('',(#170169),#89403) ;
#83687=STYLED_ITEM('',(#170169),#89404) ;
#83688=STYLED_ITEM('',(#170169),#89405) ;
#83689=STYLED_ITEM('',(#170169),#89406) ;
#83690=STYLED_ITEM('',(#170169),#89407) ;
#83691=STYLED_ITEM('',(#170169),#89408) ;
#83692=STYLED_ITEM('',(#170169),#89409) ;
#83693=STYLED_ITEM('',(#170169),#89410) ;
#83694=STYLED_ITEM('',(#170169),#89411) ;
#83695=STYLED_ITEM('',(#170169),#89412) ;
#83696=STYLED_ITEM('',(#170169),#89413) ;
#83697=STYLED_ITEM('',(#170169),#89414) ;
#83698=STYLED_ITEM('',(#170169),#89415) ;
#83699=STYLED_ITEM('',(#170169),#89416) ;
#83700=STYLED_ITEM('',(#170169),#89417) ;
#83701=STYLED_ITEM('',(#170169),#89418) ;
#83702=STYLED_ITEM('',(#170169),#89419) ;
#83703=STYLED_ITEM('',(#170169),#89420) ;
#83704=STYLED_ITEM('',(#170169),#89421) ;
#83705=STYLED_ITEM('',(#170169),#89422) ;
#83706=STYLED_ITEM('',(#170172),#89423) ;
#83707=STYLED_ITEM('',(#170172),#89424) ;
#83708=STYLED_ITEM('',(#170172),#89425) ;
#83709=STYLED_ITEM('',(#170172),#89426) ;
#83710=STYLED_ITEM('',(#170172),#89427) ;
#83711=STYLED_ITEM('',(#170172),#89428) ;
#83712=STYLED_ITEM('',(#170172),#89429) ;
#83713=STYLED_ITEM('',(#170172),#89430) ;
#83714=STYLED_ITEM('',(#170172),#89431) ;
#83715=STYLED_ITEM('',(#170172),#89432) ;
#83716=STYLED_ITEM('',(#170172),#89433) ;
#83717=STYLED_ITEM('',(#170172),#89434) ;
#83718=STYLED_ITEM('',(#170172),#89435) ;
#83719=STYLED_ITEM('',(#170172),#89436) ;
#83720=STYLED_ITEM('',(#170172),#89437) ;
#83721=STYLED_ITEM('',(#170172),#89438) ;
#83722=STYLED_ITEM('',(#170172),#89439) ;
#83723=STYLED_ITEM('',(#170172),#89440) ;
#83724=STYLED_ITEM('',(#170172),#89441) ;
#83725=STYLED_ITEM('',(#170172),#89442) ;
#83726=STYLED_ITEM('',(#170172),#89443) ;
#83727=STYLED_ITEM('',(#170172),#89444) ;
#83728=STYLED_ITEM('',(#170172),#89445) ;
#83729=STYLED_ITEM('',(#170172),#89446) ;
#83730=STYLED_ITEM('',(#170172),#89447) ;
#83731=STYLED_ITEM('',(#170172),#89448) ;
#83732=STYLED_ITEM('',(#170172),#89449) ;
#83733=STYLED_ITEM('',(#170172),#89450) ;
#83734=STYLED_ITEM('',(#170172),#89451) ;
#83735=STYLED_ITEM('',(#170172),#89452) ;
#83736=STYLED_ITEM('',(#170172),#89453) ;
#83737=STYLED_ITEM('',(#170172),#89454) ;
#83738=STYLED_ITEM('',(#170172),#89455) ;
#83739=STYLED_ITEM('',(#170172),#89456) ;
#83740=STYLED_ITEM('',(#170172),#89457) ;
#83741=STYLED_ITEM('',(#170172),#89458) ;
#83742=STYLED_ITEM('',(#170169),#89459) ;
#83743=STYLED_ITEM('',(#170169),#89460) ;
#83744=STYLED_ITEM('',(#170169),#89461) ;
#83745=STYLED_ITEM('',(#170169),#89462) ;
#83746=STYLED_ITEM('',(#170169),#89463) ;
#83747=STYLED_ITEM('',(#170169),#89464) ;
#83748=STYLED_ITEM('',(#170169),#89465) ;
#83749=STYLED_ITEM('',(#170169),#89466) ;
#83750=STYLED_ITEM('',(#170169),#89467) ;
#83751=STYLED_ITEM('',(#170169),#89468) ;
#83752=STYLED_ITEM('',(#170169),#89469) ;
#83753=STYLED_ITEM('',(#170169),#89470) ;
#83754=STYLED_ITEM('',(#170169),#89471) ;
#83755=STYLED_ITEM('',(#170169),#89472) ;
#83756=STYLED_ITEM('',(#170169),#89473) ;
#83757=STYLED_ITEM('',(#170169),#89474) ;
#83758=STYLED_ITEM('',(#170169),#89475) ;
#83759=STYLED_ITEM('',(#170169),#89476) ;
#83760=STYLED_ITEM('',(#170169),#89477) ;
#83761=STYLED_ITEM('',(#170169),#89478) ;
#83762=STYLED_ITEM('',(#170169),#89479) ;
#83763=STYLED_ITEM('',(#170169),#89480) ;
#83764=STYLED_ITEM('',(#170169),#89481) ;
#83765=STYLED_ITEM('',(#170169),#89482) ;
#83766=STYLED_ITEM('',(#170169),#89483) ;
#83767=STYLED_ITEM('',(#170169),#89484) ;
#83768=STYLED_ITEM('',(#170169),#89485) ;
#83769=STYLED_ITEM('',(#170169),#89486) ;
#83770=STYLED_ITEM('',(#170169),#89487) ;
#83771=STYLED_ITEM('',(#170169),#89488) ;
#83772=STYLED_ITEM('',(#170169),#89489) ;
#83773=STYLED_ITEM('',(#170169),#89490) ;
#83774=STYLED_ITEM('',(#170169),#89491) ;
#83775=STYLED_ITEM('',(#170169),#89492) ;
#83776=STYLED_ITEM('',(#170169),#89493) ;
#83777=STYLED_ITEM('',(#170169),#89494) ;
#83778=STYLED_ITEM('',(#170169),#89495) ;
#83779=STYLED_ITEM('',(#170169),#89496) ;
#83780=STYLED_ITEM('',(#170169),#89497) ;
#83781=STYLED_ITEM('',(#170169),#89498) ;
#83782=STYLED_ITEM('',(#170169),#89499) ;
#83783=STYLED_ITEM('',(#170169),#89500) ;
#83784=STYLED_ITEM('',(#170169),#89501) ;
#83785=STYLED_ITEM('',(#170169),#89502) ;
#83786=STYLED_ITEM('',(#170169),#89503) ;
#83787=STYLED_ITEM('',(#170169),#89504) ;
#83788=STYLED_ITEM('',(#170169),#89505) ;
#83789=STYLED_ITEM('',(#170169),#89506) ;
#83790=STYLED_ITEM('',(#170169),#89507) ;
#83791=STYLED_ITEM('',(#170169),#89508) ;
#83792=STYLED_ITEM('',(#170169),#89509) ;
#83793=STYLED_ITEM('',(#170169),#89510) ;
#83794=STYLED_ITEM('',(#170169),#89511) ;
#83795=STYLED_ITEM('',(#170169),#89512) ;
#83796=STYLED_ITEM('',(#170169),#89513) ;
#83797=STYLED_ITEM('',(#170169),#89514) ;
#83798=STYLED_ITEM('',(#170169),#89515) ;
#83799=STYLED_ITEM('',(#170169),#89516) ;
#83800=STYLED_ITEM('',(#170169),#89517) ;
#83801=STYLED_ITEM('',(#170169),#89518) ;
#83802=STYLED_ITEM('',(#170169),#89519) ;
#83803=STYLED_ITEM('',(#170169),#89520) ;
#83804=STYLED_ITEM('',(#170169),#89521) ;
#83805=STYLED_ITEM('',(#170169),#89522) ;
#83806=STYLED_ITEM('',(#170169),#89523) ;
#83807=STYLED_ITEM('',(#170169),#89524) ;
#83808=STYLED_ITEM('',(#170169),#89525) ;
#83809=STYLED_ITEM('',(#170169),#89526) ;
#83810=STYLED_ITEM('',(#170169),#89527) ;
#83811=STYLED_ITEM('',(#170169),#89528) ;
#83812=STYLED_ITEM('',(#170169),#89529) ;
#83813=STYLED_ITEM('',(#170169),#89530) ;
#83814=STYLED_ITEM('',(#170169),#89531) ;
#83815=STYLED_ITEM('',(#170169),#89532) ;
#83816=STYLED_ITEM('',(#170169),#89533) ;
#83817=STYLED_ITEM('',(#170169),#89534) ;
#83818=STYLED_ITEM('',(#170169),#89535) ;
#83819=STYLED_ITEM('',(#170169),#89536) ;
#83820=STYLED_ITEM('',(#170169),#89537) ;
#83821=STYLED_ITEM('',(#170169),#89538) ;
#83822=STYLED_ITEM('',(#170169),#89539) ;
#83823=STYLED_ITEM('',(#170169),#89540) ;
#83824=STYLED_ITEM('',(#170169),#89541) ;
#83825=STYLED_ITEM('',(#170169),#89542) ;
#83826=STYLED_ITEM('',(#170169),#89543) ;
#83827=STYLED_ITEM('',(#170169),#89544) ;
#83828=STYLED_ITEM('',(#170169),#89545) ;
#83829=STYLED_ITEM('',(#170169),#89546) ;
#83830=STYLED_ITEM('',(#170169),#89547) ;
#83831=STYLED_ITEM('',(#170169),#89548) ;
#83832=STYLED_ITEM('',(#170169),#89549) ;
#83833=STYLED_ITEM('',(#170169),#89550) ;
#83834=STYLED_ITEM('',(#170169),#89551) ;
#83835=STYLED_ITEM('',(#170169),#89552) ;
#83836=STYLED_ITEM('',(#170169),#89553) ;
#83837=STYLED_ITEM('',(#170169),#89554) ;
#83838=STYLED_ITEM('',(#170169),#89555) ;
#83839=STYLED_ITEM('',(#170169),#89556) ;
#83840=STYLED_ITEM('',(#170169),#89557) ;
#83841=STYLED_ITEM('',(#170169),#89558) ;
#83842=STYLED_ITEM('',(#170169),#89559) ;
#83843=STYLED_ITEM('',(#170169),#89560) ;
#83844=STYLED_ITEM('',(#170169),#89561) ;
#83845=STYLED_ITEM('',(#170169),#89562) ;
#83846=STYLED_ITEM('',(#170169),#89563) ;
#83847=STYLED_ITEM('',(#170169),#89564) ;
#83848=STYLED_ITEM('',(#170169),#89565) ;
#83849=STYLED_ITEM('',(#170169),#89566) ;
#83850=STYLED_ITEM('',(#170169),#89567) ;
#83851=STYLED_ITEM('',(#170169),#89568) ;
#83852=STYLED_ITEM('',(#170169),#89569) ;
#83853=STYLED_ITEM('',(#170169),#89570) ;
#83854=STYLED_ITEM('',(#170169),#89571) ;
#83855=STYLED_ITEM('',(#170169),#89572) ;
#83856=STYLED_ITEM('',(#170169),#89573) ;
#83857=STYLED_ITEM('',(#170169),#89574) ;
#83858=STYLED_ITEM('',(#170169),#89575) ;
#83859=STYLED_ITEM('',(#170169),#89576) ;
#83860=STYLED_ITEM('',(#170169),#89577) ;
#83861=STYLED_ITEM('',(#170169),#89578) ;
#83862=STYLED_ITEM('',(#170169),#89579) ;
#83863=STYLED_ITEM('',(#170169),#89580) ;
#83864=STYLED_ITEM('',(#170169),#89581) ;
#83865=STYLED_ITEM('',(#170169),#89582) ;
#83866=STYLED_ITEM('',(#170169),#89583) ;
#83867=STYLED_ITEM('',(#170169),#89584) ;
#83868=STYLED_ITEM('',(#170169),#89585) ;
#83869=STYLED_ITEM('',(#170169),#89586) ;
#83870=STYLED_ITEM('',(#170169),#89587) ;
#83871=STYLED_ITEM('',(#170169),#89588) ;
#83872=STYLED_ITEM('',(#170169),#89589) ;
#83873=STYLED_ITEM('',(#170169),#89590) ;
#83874=STYLED_ITEM('',(#170169),#89591) ;
#83875=STYLED_ITEM('',(#170169),#89592) ;
#83876=STYLED_ITEM('',(#170169),#89593) ;
#83877=STYLED_ITEM('',(#170169),#89594) ;
#83878=STYLED_ITEM('',(#170169),#89595) ;
#83879=STYLED_ITEM('',(#170169),#89596) ;
#83880=STYLED_ITEM('',(#170169),#89597) ;
#83881=STYLED_ITEM('',(#170169),#89598) ;
#83882=STYLED_ITEM('',(#170169),#89599) ;
#83883=STYLED_ITEM('',(#170169),#89600) ;
#83884=STYLED_ITEM('',(#170169),#89601) ;
#83885=STYLED_ITEM('',(#170169),#89602) ;
#83886=STYLED_ITEM('',(#170169),#89603) ;
#83887=STYLED_ITEM('',(#170169),#89604) ;
#83888=STYLED_ITEM('',(#170169),#89605) ;
#83889=STYLED_ITEM('',(#170169),#89606) ;
#83890=STYLED_ITEM('',(#170169),#89607) ;
#83891=STYLED_ITEM('',(#170169),#89608) ;
#83892=STYLED_ITEM('',(#170169),#89609) ;
#83893=STYLED_ITEM('',(#170169),#89610) ;
#83894=STYLED_ITEM('',(#170169),#89611) ;
#83895=STYLED_ITEM('',(#170169),#89612) ;
#83896=STYLED_ITEM('',(#170169),#89613) ;
#83897=STYLED_ITEM('',(#170169),#89614) ;
#83898=STYLED_ITEM('',(#170169),#89615) ;
#83899=STYLED_ITEM('',(#170169),#89616) ;
#83900=STYLED_ITEM('',(#170169),#89617) ;
#83901=STYLED_ITEM('',(#170169),#89618) ;
#83902=STYLED_ITEM('',(#170169),#89619) ;
#83903=STYLED_ITEM('',(#170169),#89620) ;
#83904=STYLED_ITEM('',(#170169),#89621) ;
#83905=STYLED_ITEM('',(#170169),#89622) ;
#83906=STYLED_ITEM('',(#170169),#89623) ;
#83907=STYLED_ITEM('',(#170169),#89624) ;
#83908=STYLED_ITEM('',(#170169),#89625) ;
#83909=STYLED_ITEM('',(#170169),#89626) ;
#83910=STYLED_ITEM('',(#170169),#89627) ;
#83911=STYLED_ITEM('',(#170169),#89628) ;
#83912=STYLED_ITEM('',(#170169),#89629) ;
#83913=STYLED_ITEM('',(#170169),#89630) ;
#83914=STYLED_ITEM('',(#170169),#89631) ;
#83915=STYLED_ITEM('',(#170169),#89632) ;
#83916=STYLED_ITEM('',(#170169),#89633) ;
#83917=STYLED_ITEM('',(#170169),#89634) ;
#83918=STYLED_ITEM('',(#170169),#89635) ;
#83919=STYLED_ITEM('',(#170169),#89636) ;
#83920=STYLED_ITEM('',(#170169),#89637) ;
#83921=STYLED_ITEM('',(#170169),#89638) ;
#83922=STYLED_ITEM('',(#170169),#89639) ;
#83923=STYLED_ITEM('',(#170169),#89640) ;
#83924=STYLED_ITEM('',(#170169),#89641) ;
#83925=STYLED_ITEM('',(#170169),#89642) ;
#83926=STYLED_ITEM('',(#170169),#89643) ;
#83927=STYLED_ITEM('',(#170169),#89644) ;
#83928=STYLED_ITEM('',(#170169),#89645) ;
#83929=STYLED_ITEM('',(#170169),#89646) ;
#83930=STYLED_ITEM('',(#170169),#89647) ;
#83931=STYLED_ITEM('',(#170169),#89648) ;
#83932=STYLED_ITEM('',(#170169),#89649) ;
#83933=STYLED_ITEM('',(#170169),#89650) ;
#83934=STYLED_ITEM('',(#170169),#89651) ;
#83935=STYLED_ITEM('',(#170169),#89652) ;
#83936=STYLED_ITEM('',(#170169),#89653) ;
#83937=STYLED_ITEM('',(#170169),#89654) ;
#83938=STYLED_ITEM('',(#170169),#89655) ;
#83939=STYLED_ITEM('',(#170169),#89656) ;
#83940=STYLED_ITEM('',(#170169),#89657) ;
#83941=STYLED_ITEM('',(#170169),#89658) ;
#83942=STYLED_ITEM('',(#170169),#89659) ;
#83943=STYLED_ITEM('',(#170169),#89660) ;
#83944=STYLED_ITEM('',(#170169),#89661) ;
#83945=STYLED_ITEM('',(#170169),#89662) ;
#83946=STYLED_ITEM('',(#170169),#89663) ;
#83947=STYLED_ITEM('',(#170169),#89664) ;
#83948=STYLED_ITEM('',(#170169),#89665) ;
#83949=STYLED_ITEM('',(#170169),#89666) ;
#83950=STYLED_ITEM('',(#170169),#89667) ;
#83951=STYLED_ITEM('',(#170169),#89668) ;
#83952=STYLED_ITEM('',(#170169),#89669) ;
#83953=STYLED_ITEM('',(#170169),#89670) ;
#83954=STYLED_ITEM('',(#170169),#89671) ;
#83955=STYLED_ITEM('',(#170169),#89672) ;
#83956=STYLED_ITEM('',(#170169),#89673) ;
#83957=STYLED_ITEM('',(#170169),#89674) ;
#83958=STYLED_ITEM('',(#170169),#89675) ;
#83959=STYLED_ITEM('',(#170169),#89676) ;
#83960=STYLED_ITEM('',(#170169),#89677) ;
#83961=STYLED_ITEM('',(#170169),#89678) ;
#83962=STYLED_ITEM('',(#170169),#89679) ;
#83963=STYLED_ITEM('',(#170169),#89680) ;
#83964=STYLED_ITEM('',(#170169),#89681) ;
#83965=STYLED_ITEM('',(#170169),#89682) ;
#83966=STYLED_ITEM('',(#170169),#89683) ;
#83967=STYLED_ITEM('',(#170169),#89684) ;
#83968=STYLED_ITEM('',(#170169),#89685) ;
#83969=STYLED_ITEM('',(#170169),#89686) ;
#83970=STYLED_ITEM('',(#170169),#89687) ;
#83971=STYLED_ITEM('',(#170169),#89688) ;
#83972=STYLED_ITEM('',(#170169),#89689) ;
#83973=STYLED_ITEM('',(#170169),#89690) ;
#83974=STYLED_ITEM('',(#170169),#89691) ;
#83975=STYLED_ITEM('',(#170169),#89692) ;
#83976=STYLED_ITEM('',(#170169),#89693) ;
#83977=STYLED_ITEM('',(#170169),#89694) ;
#83978=STYLED_ITEM('',(#170169),#89695) ;
#83979=STYLED_ITEM('',(#170169),#89696) ;
#83980=STYLED_ITEM('',(#170169),#89697) ;
#83981=STYLED_ITEM('',(#170169),#89698) ;
#83982=STYLED_ITEM('',(#170169),#89699) ;
#83983=STYLED_ITEM('',(#170169),#89700) ;
#83984=STYLED_ITEM('',(#170169),#89701) ;
#83985=STYLED_ITEM('',(#170169),#89702) ;
#83986=STYLED_ITEM('',(#170169),#89703) ;
#83987=STYLED_ITEM('',(#170169),#89704) ;
#83988=STYLED_ITEM('',(#170169),#89705) ;
#83989=STYLED_ITEM('',(#170169),#89706) ;
#83990=STYLED_ITEM('',(#170169),#89707) ;
#83991=STYLED_ITEM('',(#170169),#89708) ;
#83992=STYLED_ITEM('',(#170169),#89709) ;
#83993=STYLED_ITEM('',(#170169),#89710) ;
#83994=STYLED_ITEM('',(#170169),#89711) ;
#83995=STYLED_ITEM('',(#170169),#89712) ;
#83996=STYLED_ITEM('',(#170169),#89713) ;
#83997=STYLED_ITEM('',(#170169),#89714) ;
#83998=STYLED_ITEM('',(#170169),#89715) ;
#83999=STYLED_ITEM('',(#170169),#89716) ;
#84000=STYLED_ITEM('',(#170169),#89717) ;
#84001=STYLED_ITEM('',(#170169),#89718) ;
#84002=STYLED_ITEM('',(#170169),#89719) ;
#84003=STYLED_ITEM('',(#170169),#89720) ;
#84004=STYLED_ITEM('',(#170169),#89721) ;
#84005=STYLED_ITEM('',(#170169),#89722) ;
#84006=STYLED_ITEM('',(#170169),#89723) ;
#84007=STYLED_ITEM('',(#170169),#89724) ;
#84008=STYLED_ITEM('',(#170169),#89725) ;
#84009=STYLED_ITEM('',(#170169),#89726) ;
#84010=STYLED_ITEM('',(#170169),#89727) ;
#84011=STYLED_ITEM('',(#170169),#89728) ;
#84012=STYLED_ITEM('',(#170169),#89729) ;
#84013=STYLED_ITEM('',(#170169),#89730) ;
#84014=STYLED_ITEM('',(#170169),#89731) ;
#84015=STYLED_ITEM('',(#170169),#89732) ;
#84016=STYLED_ITEM('',(#170169),#89733) ;
#84017=STYLED_ITEM('',(#170169),#89734) ;
#84018=STYLED_ITEM('',(#170169),#89735) ;
#84019=STYLED_ITEM('',(#170169),#89736) ;
#84020=STYLED_ITEM('',(#170169),#89737) ;
#84021=STYLED_ITEM('',(#170169),#89738) ;
#84022=STYLED_ITEM('',(#170169),#89739) ;
#84023=STYLED_ITEM('',(#170169),#89740) ;
#84024=STYLED_ITEM('',(#170169),#89741) ;
#84025=STYLED_ITEM('',(#170169),#89742) ;
#84026=STYLED_ITEM('',(#170169),#89743) ;
#84027=STYLED_ITEM('',(#170172),#89744) ;
#84028=STYLED_ITEM('',(#170172),#89745) ;
#84029=STYLED_ITEM('',(#170172),#89746) ;
#84030=STYLED_ITEM('',(#170172),#89747) ;
#84031=STYLED_ITEM('',(#170169),#89748) ;
#84032=STYLED_ITEM('',(#170169),#89749) ;
#84033=STYLED_ITEM('',(#170169),#89750) ;
#84034=STYLED_ITEM('',(#170169),#89751) ;
#84035=STYLED_ITEM('',(#170169),#89752) ;
#84036=STYLED_ITEM('',(#170169),#89753) ;
#84037=STYLED_ITEM('',(#170169),#89754) ;
#84038=STYLED_ITEM('',(#170169),#89755) ;
#84039=STYLED_ITEM('',(#170169),#89756) ;
#84040=STYLED_ITEM('',(#170169),#89757) ;
#84041=STYLED_ITEM('',(#170169),#89758) ;
#84042=STYLED_ITEM('',(#170169),#89759) ;
#84043=STYLED_ITEM('',(#170169),#89760) ;
#84044=STYLED_ITEM('',(#170169),#89761) ;
#84045=STYLED_ITEM('',(#170169),#89762) ;
#84046=STYLED_ITEM('',(#170169),#89763) ;
#84047=STYLED_ITEM('',(#170169),#89764) ;
#84048=STYLED_ITEM('',(#170169),#89765) ;
#84049=STYLED_ITEM('',(#170169),#89766) ;
#84050=STYLED_ITEM('',(#170169),#89767) ;
#84051=STYLED_ITEM('',(#170169),#89768) ;
#84052=STYLED_ITEM('',(#170169),#89769) ;
#84053=STYLED_ITEM('',(#170169),#89770) ;
#84054=STYLED_ITEM('',(#170169),#89771) ;
#84055=STYLED_ITEM('',(#170169),#89772) ;
#84056=STYLED_ITEM('',(#170169),#89773) ;
#84057=STYLED_ITEM('',(#170169),#89774) ;
#84058=STYLED_ITEM('',(#170169),#89775) ;
#84059=STYLED_ITEM('',(#170169),#89776) ;
#84060=STYLED_ITEM('',(#170169),#89777) ;
#84061=STYLED_ITEM('',(#170169),#89778) ;
#84062=STYLED_ITEM('',(#170169),#89779) ;
#84063=STYLED_ITEM('',(#170169),#89780) ;
#84064=STYLED_ITEM('',(#170169),#89781) ;
#84065=STYLED_ITEM('',(#170169),#89782) ;
#84066=STYLED_ITEM('',(#170169),#89783) ;
#84067=STYLED_ITEM('',(#170169),#89784) ;
#84068=STYLED_ITEM('',(#170169),#89785) ;
#84069=STYLED_ITEM('',(#170169),#89786) ;
#84070=STYLED_ITEM('',(#170169),#89787) ;
#84071=STYLED_ITEM('',(#170169),#89788) ;
#84072=STYLED_ITEM('',(#170169),#89789) ;
#84073=STYLED_ITEM('',(#170169),#89790) ;
#84074=STYLED_ITEM('',(#170169),#89791) ;
#84075=STYLED_ITEM('',(#170169),#89792) ;
#84076=STYLED_ITEM('',(#170169),#89793) ;
#84077=STYLED_ITEM('',(#170169),#89794) ;
#84078=STYLED_ITEM('',(#170169),#89795) ;
#84079=STYLED_ITEM('',(#170169),#89796) ;
#84080=STYLED_ITEM('',(#170169),#89797) ;
#84081=STYLED_ITEM('',(#170169),#89798) ;
#84082=STYLED_ITEM('',(#170169),#89799) ;
#84083=STYLED_ITEM('',(#170169),#89800) ;
#84084=STYLED_ITEM('',(#170169),#89801) ;
#84085=STYLED_ITEM('',(#170169),#89802) ;
#84086=STYLED_ITEM('',(#170169),#89803) ;
#84087=STYLED_ITEM('',(#170169),#89804) ;
#84088=STYLED_ITEM('',(#170169),#89805) ;
#84089=STYLED_ITEM('',(#170169),#89806) ;
#84090=STYLED_ITEM('',(#170169),#89807) ;
#84091=STYLED_ITEM('',(#170169),#89808) ;
#84092=STYLED_ITEM('',(#170169),#89809) ;
#84093=STYLED_ITEM('',(#170169),#89810) ;
#84094=STYLED_ITEM('',(#170169),#89811) ;
#84095=STYLED_ITEM('',(#170169),#89812) ;
#84096=STYLED_ITEM('',(#170169),#89813) ;
#84097=STYLED_ITEM('',(#170169),#89814) ;
#84098=STYLED_ITEM('',(#170169),#89815) ;
#84099=STYLED_ITEM('',(#170169),#89816) ;
#84100=STYLED_ITEM('',(#170169),#89817) ;
#84101=STYLED_ITEM('',(#170169),#89818) ;
#84102=STYLED_ITEM('',(#170169),#89819) ;
#84103=STYLED_ITEM('',(#170169),#89820) ;
#84104=STYLED_ITEM('',(#170169),#89821) ;
#84105=STYLED_ITEM('',(#170169),#89822) ;
#84106=STYLED_ITEM('',(#170169),#89823) ;
#84107=STYLED_ITEM('',(#170169),#89824) ;
#84108=STYLED_ITEM('',(#170169),#89825) ;
#84109=STYLED_ITEM('',(#170169),#89826) ;
#84110=STYLED_ITEM('',(#170169),#89827) ;
#84111=STYLED_ITEM('',(#170169),#89828) ;
#84112=STYLED_ITEM('',(#170169),#89829) ;
#84113=STYLED_ITEM('',(#170169),#89830) ;
#84114=STYLED_ITEM('',(#170169),#89831) ;
#84115=STYLED_ITEM('',(#170169),#89832) ;
#84116=STYLED_ITEM('',(#170169),#89833) ;
#84117=STYLED_ITEM('',(#170169),#89834) ;
#84118=STYLED_ITEM('',(#170169),#89835) ;
#84119=STYLED_ITEM('',(#170169),#89836) ;
#84120=STYLED_ITEM('',(#170169),#89837) ;
#84121=STYLED_ITEM('',(#170169),#89838) ;
#84122=STYLED_ITEM('',(#170169),#89839) ;
#84123=STYLED_ITEM('',(#170169),#89840) ;
#84124=STYLED_ITEM('',(#170169),#89841) ;
#84125=STYLED_ITEM('',(#170169),#89842) ;
#84126=STYLED_ITEM('',(#170169),#89843) ;
#84127=STYLED_ITEM('',(#170169),#89844) ;
#84128=STYLED_ITEM('',(#170169),#89845) ;
#84129=STYLED_ITEM('',(#170169),#89846) ;
#84130=STYLED_ITEM('',(#170169),#89847) ;
#84131=STYLED_ITEM('',(#170169),#89848) ;
#84132=STYLED_ITEM('',(#170169),#89849) ;
#84133=STYLED_ITEM('',(#170169),#89850) ;
#84134=STYLED_ITEM('',(#170169),#89851) ;
#84135=STYLED_ITEM('',(#170169),#89852) ;
#84136=STYLED_ITEM('',(#170169),#89853) ;
#84137=STYLED_ITEM('',(#170169),#89854) ;
#84138=STYLED_ITEM('',(#170169),#89855) ;
#84139=STYLED_ITEM('',(#170169),#89856) ;
#84140=STYLED_ITEM('',(#170169),#89857) ;
#84141=STYLED_ITEM('',(#170169),#89858) ;
#84142=STYLED_ITEM('',(#170169),#89859) ;
#84143=STYLED_ITEM('',(#170169),#89860) ;
#84144=STYLED_ITEM('',(#170169),#89861) ;
#84145=STYLED_ITEM('',(#170169),#89862) ;
#84146=STYLED_ITEM('',(#170169),#89863) ;
#84147=STYLED_ITEM('',(#170169),#89864) ;
#84148=STYLED_ITEM('',(#170169),#89865) ;
#84149=STYLED_ITEM('',(#170169),#89866) ;
#84150=STYLED_ITEM('',(#170169),#89867) ;
#84151=STYLED_ITEM('',(#170169),#89868) ;
#84152=STYLED_ITEM('',(#170169),#89869) ;
#84153=STYLED_ITEM('',(#170169),#89870) ;
#84154=STYLED_ITEM('',(#170169),#89871) ;
#84155=STYLED_ITEM('',(#170169),#89872) ;
#84156=STYLED_ITEM('',(#170169),#89873) ;
#84157=STYLED_ITEM('',(#170169),#89874) ;
#84158=STYLED_ITEM('',(#170169),#89875) ;
#84159=STYLED_ITEM('',(#170169),#89876) ;
#84160=STYLED_ITEM('',(#170169),#89877) ;
#84161=STYLED_ITEM('',(#170169),#89878) ;
#84162=STYLED_ITEM('',(#170169),#89879) ;
#84163=STYLED_ITEM('',(#170169),#89880) ;
#84164=STYLED_ITEM('',(#170169),#89881) ;
#84165=STYLED_ITEM('',(#170169),#89882) ;
#84166=STYLED_ITEM('',(#170169),#89883) ;
#84167=STYLED_ITEM('',(#170172),#89884) ;
#84168=STYLED_ITEM('',(#170172),#89885) ;
#84169=STYLED_ITEM('',(#170172),#89886) ;
#84170=STYLED_ITEM('',(#170172),#89887) ;
#84171=STYLED_ITEM('',(#170169),#89888) ;
#84172=STYLED_ITEM('',(#170169),#89889) ;
#84173=STYLED_ITEM('',(#170169),#89890) ;
#84174=STYLED_ITEM('',(#170169),#89891) ;
#84175=STYLED_ITEM('',(#170169),#89892) ;
#84176=STYLED_ITEM('',(#170169),#89893) ;
#84177=STYLED_ITEM('',(#170169),#89894) ;
#84178=STYLED_ITEM('',(#170169),#89895) ;
#84179=STYLED_ITEM('',(#170169),#89896) ;
#84180=STYLED_ITEM('',(#170169),#89897) ;
#84181=STYLED_ITEM('',(#170169),#89898) ;
#84182=STYLED_ITEM('',(#170169),#89899) ;
#84183=STYLED_ITEM('',(#170169),#89900) ;
#84184=STYLED_ITEM('',(#170169),#89901) ;
#84185=STYLED_ITEM('',(#170169),#89902) ;
#84186=STYLED_ITEM('',(#170169),#89903) ;
#84187=STYLED_ITEM('',(#170169),#89904) ;
#84188=STYLED_ITEM('',(#170169),#89905) ;
#84189=STYLED_ITEM('',(#170169),#89906) ;
#84190=STYLED_ITEM('',(#170169),#89907) ;
#84191=STYLED_ITEM('',(#170169),#89908) ;
#84192=STYLED_ITEM('',(#170169),#89909) ;
#84193=STYLED_ITEM('',(#170169),#89910) ;
#84194=STYLED_ITEM('',(#170169),#89911) ;
#84195=STYLED_ITEM('',(#170169),#89912) ;
#84196=STYLED_ITEM('',(#170169),#89913) ;
#84197=STYLED_ITEM('',(#170169),#89914) ;
#84198=STYLED_ITEM('',(#170169),#89915) ;
#84199=STYLED_ITEM('',(#170169),#89916) ;
#84200=STYLED_ITEM('',(#170169),#89917) ;
#84201=STYLED_ITEM('',(#170169),#89918) ;
#84202=STYLED_ITEM('',(#170169),#89919) ;
#84203=STYLED_ITEM('',(#170169),#89920) ;
#84204=STYLED_ITEM('',(#170169),#89921) ;
#84205=STYLED_ITEM('',(#170169),#89922) ;
#84206=STYLED_ITEM('',(#170169),#89923) ;
#84207=STYLED_ITEM('',(#170169),#89924) ;
#84208=STYLED_ITEM('',(#170169),#89925) ;
#84209=STYLED_ITEM('',(#170169),#89926) ;
#84210=STYLED_ITEM('',(#170169),#89927) ;
#84211=STYLED_ITEM('',(#170169),#89928) ;
#84212=STYLED_ITEM('',(#170169),#89929) ;
#84213=STYLED_ITEM('',(#170169),#89930) ;
#84214=STYLED_ITEM('',(#170169),#89931) ;
#84215=STYLED_ITEM('',(#170169),#89932) ;
#84216=STYLED_ITEM('',(#170169),#89933) ;
#84217=STYLED_ITEM('',(#170169),#89934) ;
#84218=STYLED_ITEM('',(#170169),#89935) ;
#84219=STYLED_ITEM('',(#170169),#89936) ;
#84220=STYLED_ITEM('',(#170169),#89937) ;
#84221=STYLED_ITEM('',(#170169),#89938) ;
#84222=STYLED_ITEM('',(#170169),#89939) ;
#84223=STYLED_ITEM('',(#170169),#89940) ;
#84224=STYLED_ITEM('',(#170169),#89941) ;
#84225=STYLED_ITEM('',(#170169),#89942) ;
#84226=STYLED_ITEM('',(#170169),#89943) ;
#84227=STYLED_ITEM('',(#170169),#89944) ;
#84228=STYLED_ITEM('',(#170169),#89945) ;
#84229=STYLED_ITEM('',(#170169),#89946) ;
#84230=STYLED_ITEM('',(#170169),#89947) ;
#84231=STYLED_ITEM('',(#170169),#89948) ;
#84232=STYLED_ITEM('',(#170169),#89949) ;
#84233=STYLED_ITEM('',(#170169),#89950) ;
#84234=STYLED_ITEM('',(#170169),#89951) ;
#84235=STYLED_ITEM('',(#170169),#89952) ;
#84236=STYLED_ITEM('',(#170169),#89953) ;
#84237=STYLED_ITEM('',(#170169),#89954) ;
#84238=STYLED_ITEM('',(#170169),#89955) ;
#84239=STYLED_ITEM('',(#170169),#89956) ;
#84240=STYLED_ITEM('',(#170169),#89957) ;
#84241=STYLED_ITEM('',(#170169),#89958) ;
#84242=STYLED_ITEM('',(#170169),#89959) ;
#84243=STYLED_ITEM('',(#170169),#89960) ;
#84244=STYLED_ITEM('',(#170169),#89961) ;
#84245=STYLED_ITEM('',(#170169),#89962) ;
#84246=STYLED_ITEM('',(#170169),#89963) ;
#84247=STYLED_ITEM('',(#170169),#89964) ;
#84248=STYLED_ITEM('',(#170169),#89965) ;
#84249=STYLED_ITEM('',(#170169),#89966) ;
#84250=STYLED_ITEM('',(#170169),#89967) ;
#84251=STYLED_ITEM('',(#170169),#89968) ;
#84252=STYLED_ITEM('',(#170169),#89969) ;
#84253=STYLED_ITEM('',(#170169),#89970) ;
#84254=STYLED_ITEM('',(#170169),#89971) ;
#84255=STYLED_ITEM('',(#170169),#89972) ;
#84256=STYLED_ITEM('',(#170169),#89973) ;
#84257=STYLED_ITEM('',(#170169),#89974) ;
#84258=STYLED_ITEM('',(#170169),#89975) ;
#84259=STYLED_ITEM('',(#170169),#89976) ;
#84260=STYLED_ITEM('',(#170169),#89977) ;
#84261=STYLED_ITEM('',(#170169),#89978) ;
#84262=STYLED_ITEM('',(#170169),#89979) ;
#84263=STYLED_ITEM('',(#170169),#89980) ;
#84264=STYLED_ITEM('',(#170169),#89981) ;
#84265=STYLED_ITEM('',(#170169),#89982) ;
#84266=STYLED_ITEM('',(#170169),#89983) ;
#84267=STYLED_ITEM('',(#170169),#89984) ;
#84268=STYLED_ITEM('',(#170169),#89985) ;
#84269=STYLED_ITEM('',(#170169),#89986) ;
#84270=STYLED_ITEM('',(#170169),#89987) ;
#84271=STYLED_ITEM('',(#170169),#89988) ;
#84272=STYLED_ITEM('',(#170169),#89989) ;
#84273=STYLED_ITEM('',(#170169),#89990) ;
#84274=STYLED_ITEM('',(#170169),#89991) ;
#84275=STYLED_ITEM('',(#170169),#89992) ;
#84276=STYLED_ITEM('',(#170169),#89993) ;
#84277=STYLED_ITEM('',(#170169),#89994) ;
#84278=STYLED_ITEM('',(#170169),#89995) ;
#84279=STYLED_ITEM('',(#170169),#89996) ;
#84280=STYLED_ITEM('',(#170169),#89997) ;
#84281=STYLED_ITEM('',(#170169),#89998) ;
#84282=STYLED_ITEM('',(#170169),#89999) ;
#84283=STYLED_ITEM('',(#170169),#90000) ;
#84284=STYLED_ITEM('',(#170169),#90001) ;
#84285=STYLED_ITEM('',(#170169),#90002) ;
#84286=STYLED_ITEM('',(#170169),#90003) ;
#84287=STYLED_ITEM('',(#170169),#90004) ;
#84288=STYLED_ITEM('',(#170169),#90005) ;
#84289=STYLED_ITEM('',(#170169),#90006) ;
#84290=STYLED_ITEM('',(#170169),#90007) ;
#84291=STYLED_ITEM('',(#170169),#90008) ;
#84292=STYLED_ITEM('',(#170169),#90009) ;
#84293=STYLED_ITEM('',(#170169),#90010) ;
#84294=STYLED_ITEM('',(#170169),#90011) ;
#84295=STYLED_ITEM('',(#170169),#90012) ;
#84296=STYLED_ITEM('',(#170169),#90013) ;
#84297=STYLED_ITEM('',(#170169),#90014) ;
#84298=STYLED_ITEM('',(#170169),#90015) ;
#84299=STYLED_ITEM('',(#170169),#90016) ;
#84300=STYLED_ITEM('',(#170169),#90017) ;
#84301=STYLED_ITEM('',(#170169),#90018) ;
#84302=STYLED_ITEM('',(#170169),#90019) ;
#84303=STYLED_ITEM('',(#170169),#90020) ;
#84304=STYLED_ITEM('',(#170169),#90021) ;
#84305=STYLED_ITEM('',(#170169),#90022) ;
#84306=STYLED_ITEM('',(#170169),#90023) ;
#84307=STYLED_ITEM('',(#170172),#90024) ;
#84308=STYLED_ITEM('',(#170172),#90025) ;
#84309=STYLED_ITEM('',(#170172),#90026) ;
#84310=STYLED_ITEM('',(#170172),#90027) ;
#84311=STYLED_ITEM('',(#170169),#90028) ;
#84312=STYLED_ITEM('',(#170169),#90029) ;
#84313=STYLED_ITEM('',(#170169),#90030) ;
#84314=STYLED_ITEM('',(#170169),#90031) ;
#84315=STYLED_ITEM('',(#170169),#90032) ;
#84316=STYLED_ITEM('',(#170169),#90033) ;
#84317=STYLED_ITEM('',(#170169),#90034) ;
#84318=STYLED_ITEM('',(#170169),#90035) ;
#84319=STYLED_ITEM('',(#170169),#90036) ;
#84320=STYLED_ITEM('',(#170169),#90037) ;
#84321=STYLED_ITEM('',(#170169),#90038) ;
#84322=STYLED_ITEM('',(#170169),#90039) ;
#84323=STYLED_ITEM('',(#170169),#90040) ;
#84324=STYLED_ITEM('',(#170169),#90041) ;
#84325=STYLED_ITEM('',(#170169),#90042) ;
#84326=STYLED_ITEM('',(#170169),#90043) ;
#84327=STYLED_ITEM('',(#170169),#90044) ;
#84328=STYLED_ITEM('',(#170169),#90045) ;
#84329=STYLED_ITEM('',(#170169),#90046) ;
#84330=STYLED_ITEM('',(#170169),#90047) ;
#84331=STYLED_ITEM('',(#170169),#90048) ;
#84332=STYLED_ITEM('',(#170169),#90049) ;
#84333=STYLED_ITEM('',(#170169),#90050) ;
#84334=STYLED_ITEM('',(#170169),#90051) ;
#84335=STYLED_ITEM('',(#170169),#90052) ;
#84336=STYLED_ITEM('',(#170169),#90053) ;
#84337=STYLED_ITEM('',(#170169),#90054) ;
#84338=STYLED_ITEM('',(#170169),#90055) ;
#84339=STYLED_ITEM('',(#170169),#90056) ;
#84340=STYLED_ITEM('',(#170169),#90057) ;
#84341=STYLED_ITEM('',(#170169),#90058) ;
#84342=STYLED_ITEM('',(#170169),#90059) ;
#84343=STYLED_ITEM('',(#170169),#90060) ;
#84344=STYLED_ITEM('',(#170169),#90061) ;
#84345=STYLED_ITEM('',(#170169),#90062) ;
#84346=STYLED_ITEM('',(#170169),#90063) ;
#84347=STYLED_ITEM('',(#170169),#90064) ;
#84348=STYLED_ITEM('',(#170169),#90065) ;
#84349=STYLED_ITEM('',(#170169),#90066) ;
#84350=STYLED_ITEM('',(#170169),#90067) ;
#84351=STYLED_ITEM('',(#170169),#90068) ;
#84352=STYLED_ITEM('',(#170169),#90069) ;
#84353=STYLED_ITEM('',(#170169),#90070) ;
#84354=STYLED_ITEM('',(#170169),#90071) ;
#84355=STYLED_ITEM('',(#170169),#90072) ;
#84356=STYLED_ITEM('',(#170169),#90073) ;
#84357=STYLED_ITEM('',(#170169),#90074) ;
#84358=STYLED_ITEM('',(#170169),#90075) ;
#84359=STYLED_ITEM('',(#170169),#90076) ;
#84360=STYLED_ITEM('',(#170169),#90077) ;
#84361=STYLED_ITEM('',(#170169),#90078) ;
#84362=STYLED_ITEM('',(#170169),#90079) ;
#84363=STYLED_ITEM('',(#170169),#90080) ;
#84364=STYLED_ITEM('',(#170169),#90081) ;
#84365=STYLED_ITEM('',(#170169),#90082) ;
#84366=STYLED_ITEM('',(#170169),#90083) ;
#84367=STYLED_ITEM('',(#170169),#90084) ;
#84368=STYLED_ITEM('',(#170169),#90085) ;
#84369=STYLED_ITEM('',(#170169),#90086) ;
#84370=STYLED_ITEM('',(#170169),#90087) ;
#84371=STYLED_ITEM('',(#170169),#90088) ;
#84372=STYLED_ITEM('',(#170169),#90089) ;
#84373=STYLED_ITEM('',(#170169),#90090) ;
#84374=STYLED_ITEM('',(#170169),#90091) ;
#84375=STYLED_ITEM('',(#170169),#90092) ;
#84376=STYLED_ITEM('',(#170169),#90093) ;
#84377=STYLED_ITEM('',(#170169),#90094) ;
#84378=STYLED_ITEM('',(#170169),#90095) ;
#84379=STYLED_ITEM('',(#170169),#90096) ;
#84380=STYLED_ITEM('',(#170169),#90097) ;
#84381=STYLED_ITEM('',(#170169),#90098) ;
#84382=STYLED_ITEM('',(#170169),#90099) ;
#84383=STYLED_ITEM('',(#170169),#90100) ;
#84384=STYLED_ITEM('',(#170169),#90101) ;
#84385=STYLED_ITEM('',(#170169),#90102) ;
#84386=STYLED_ITEM('',(#170169),#90103) ;
#84387=STYLED_ITEM('',(#170169),#90104) ;
#84388=STYLED_ITEM('',(#170169),#90105) ;
#84389=STYLED_ITEM('',(#170169),#90106) ;
#84390=STYLED_ITEM('',(#170169),#90107) ;
#84391=STYLED_ITEM('',(#170169),#90108) ;
#84392=STYLED_ITEM('',(#170169),#90109) ;
#84393=STYLED_ITEM('',(#170169),#90110) ;
#84394=STYLED_ITEM('',(#170169),#90111) ;
#84395=STYLED_ITEM('',(#170169),#90112) ;
#84396=STYLED_ITEM('',(#170169),#90113) ;
#84397=STYLED_ITEM('',(#170169),#90114) ;
#84398=STYLED_ITEM('',(#170169),#90115) ;
#84399=STYLED_ITEM('',(#170169),#90116) ;
#84400=STYLED_ITEM('',(#170169),#90117) ;
#84401=STYLED_ITEM('',(#170169),#90118) ;
#84402=STYLED_ITEM('',(#170169),#90119) ;
#84403=STYLED_ITEM('',(#170169),#90120) ;
#84404=STYLED_ITEM('',(#170169),#90121) ;
#84405=STYLED_ITEM('',(#170169),#90122) ;
#84406=STYLED_ITEM('',(#170169),#90123) ;
#84407=STYLED_ITEM('',(#170169),#90124) ;
#84408=STYLED_ITEM('',(#170169),#90125) ;
#84409=STYLED_ITEM('',(#170169),#90126) ;
#84410=STYLED_ITEM('',(#170169),#90127) ;
#84411=STYLED_ITEM('',(#170169),#90128) ;
#84412=STYLED_ITEM('',(#170169),#90129) ;
#84413=STYLED_ITEM('',(#170169),#90130) ;
#84414=STYLED_ITEM('',(#170169),#90131) ;
#84415=STYLED_ITEM('',(#170169),#90132) ;
#84416=STYLED_ITEM('',(#170169),#90133) ;
#84417=STYLED_ITEM('',(#170169),#90134) ;
#84418=STYLED_ITEM('',(#170169),#90135) ;
#84419=STYLED_ITEM('',(#170169),#90136) ;
#84420=STYLED_ITEM('',(#170169),#90137) ;
#84421=STYLED_ITEM('',(#170169),#90138) ;
#84422=STYLED_ITEM('',(#170169),#90139) ;
#84423=STYLED_ITEM('',(#170169),#90140) ;
#84424=STYLED_ITEM('',(#170169),#90141) ;
#84425=STYLED_ITEM('',(#170169),#90142) ;
#84426=STYLED_ITEM('',(#170169),#90143) ;
#84427=STYLED_ITEM('',(#170169),#90144) ;
#84428=STYLED_ITEM('',(#170169),#90145) ;
#84429=STYLED_ITEM('',(#170169),#90146) ;
#84430=STYLED_ITEM('',(#170169),#90147) ;
#84431=STYLED_ITEM('',(#170169),#90148) ;
#84432=STYLED_ITEM('',(#170169),#90149) ;
#84433=STYLED_ITEM('',(#170169),#90150) ;
#84434=STYLED_ITEM('',(#170169),#90151) ;
#84435=STYLED_ITEM('',(#170169),#90152) ;
#84436=STYLED_ITEM('',(#170169),#90153) ;
#84437=STYLED_ITEM('',(#170169),#90154) ;
#84438=STYLED_ITEM('',(#170169),#90155) ;
#84439=STYLED_ITEM('',(#170169),#90156) ;
#84440=STYLED_ITEM('',(#170169),#90157) ;
#84441=STYLED_ITEM('',(#170169),#90158) ;
#84442=STYLED_ITEM('',(#170169),#90159) ;
#84443=STYLED_ITEM('',(#170169),#90160) ;
#84444=STYLED_ITEM('',(#170169),#90161) ;
#84445=STYLED_ITEM('',(#170169),#90162) ;
#84446=STYLED_ITEM('',(#170169),#90163) ;
#84447=STYLED_ITEM('',(#170172),#90164) ;
#84448=STYLED_ITEM('',(#170172),#90165) ;
#84449=STYLED_ITEM('',(#170172),#90166) ;
#84450=STYLED_ITEM('',(#170172),#90167) ;
#84451=STYLED_ITEM('',(#170169),#90168) ;
#84452=STYLED_ITEM('',(#170169),#90169) ;
#84453=STYLED_ITEM('',(#170169),#90170) ;
#84454=STYLED_ITEM('',(#170169),#90171) ;
#84455=STYLED_ITEM('',(#170169),#90172) ;
#84456=STYLED_ITEM('',(#170169),#90173) ;
#84457=STYLED_ITEM('',(#170169),#90174) ;
#84458=STYLED_ITEM('',(#170169),#90175) ;
#84459=STYLED_ITEM('',(#170169),#90176) ;
#84460=STYLED_ITEM('',(#170169),#90177) ;
#84461=STYLED_ITEM('',(#170169),#90178) ;
#84462=STYLED_ITEM('',(#170169),#90179) ;
#84463=STYLED_ITEM('',(#170169),#90180) ;
#84464=STYLED_ITEM('',(#170169),#90181) ;
#84465=STYLED_ITEM('',(#170169),#90182) ;
#84466=STYLED_ITEM('',(#170169),#90183) ;
#84467=STYLED_ITEM('',(#170169),#90184) ;
#84468=STYLED_ITEM('',(#170169),#90185) ;
#84469=STYLED_ITEM('',(#170169),#90186) ;
#84470=STYLED_ITEM('',(#170169),#90187) ;
#84471=STYLED_ITEM('',(#170169),#90188) ;
#84472=STYLED_ITEM('',(#170169),#90189) ;
#84473=STYLED_ITEM('',(#170169),#90190) ;
#84474=STYLED_ITEM('',(#170169),#90191) ;
#84475=STYLED_ITEM('',(#170169),#90192) ;
#84476=STYLED_ITEM('',(#170169),#90193) ;
#84477=STYLED_ITEM('',(#170169),#90194) ;
#84478=STYLED_ITEM('',(#170169),#90195) ;
#84479=STYLED_ITEM('',(#170169),#90196) ;
#84480=STYLED_ITEM('',(#170169),#90197) ;
#84481=STYLED_ITEM('',(#170169),#90198) ;
#84482=STYLED_ITEM('',(#170169),#90199) ;
#84483=STYLED_ITEM('',(#170169),#90200) ;
#84484=STYLED_ITEM('',(#170169),#90201) ;
#84485=STYLED_ITEM('',(#170169),#90202) ;
#84486=STYLED_ITEM('',(#170169),#90203) ;
#84487=STYLED_ITEM('',(#170169),#90204) ;
#84488=STYLED_ITEM('',(#170169),#90205) ;
#84489=STYLED_ITEM('',(#170169),#90206) ;
#84490=STYLED_ITEM('',(#170169),#90207) ;
#84491=STYLED_ITEM('',(#170169),#90208) ;
#84492=STYLED_ITEM('',(#170169),#90209) ;
#84493=STYLED_ITEM('',(#170169),#90210) ;
#84494=STYLED_ITEM('',(#170169),#90211) ;
#84495=STYLED_ITEM('',(#170169),#90212) ;
#84496=STYLED_ITEM('',(#170169),#90213) ;
#84497=STYLED_ITEM('',(#170169),#90214) ;
#84498=STYLED_ITEM('',(#170169),#90215) ;
#84499=STYLED_ITEM('',(#170169),#90216) ;
#84500=STYLED_ITEM('',(#170169),#90217) ;
#84501=STYLED_ITEM('',(#170169),#90218) ;
#84502=STYLED_ITEM('',(#170169),#90219) ;
#84503=STYLED_ITEM('',(#170169),#90220) ;
#84504=STYLED_ITEM('',(#170169),#90221) ;
#84505=STYLED_ITEM('',(#170169),#90222) ;
#84506=STYLED_ITEM('',(#170169),#90223) ;
#84507=STYLED_ITEM('',(#170169),#90224) ;
#84508=STYLED_ITEM('',(#170169),#90225) ;
#84509=STYLED_ITEM('',(#170169),#90226) ;
#84510=STYLED_ITEM('',(#170169),#90227) ;
#84511=STYLED_ITEM('',(#170169),#90228) ;
#84512=STYLED_ITEM('',(#170169),#90229) ;
#84513=STYLED_ITEM('',(#170169),#90230) ;
#84514=STYLED_ITEM('',(#170169),#90231) ;
#84515=STYLED_ITEM('',(#170169),#90232) ;
#84516=STYLED_ITEM('',(#170169),#90233) ;
#84517=STYLED_ITEM('',(#170169),#90234) ;
#84518=STYLED_ITEM('',(#170169),#90235) ;
#84519=STYLED_ITEM('',(#170169),#90236) ;
#84520=STYLED_ITEM('',(#170169),#90237) ;
#84521=STYLED_ITEM('',(#170169),#90238) ;
#84522=STYLED_ITEM('',(#170169),#90239) ;
#84523=STYLED_ITEM('',(#170169),#90240) ;
#84524=STYLED_ITEM('',(#170169),#90241) ;
#84525=STYLED_ITEM('',(#170169),#90242) ;
#84526=STYLED_ITEM('',(#170169),#90243) ;
#84527=STYLED_ITEM('',(#170169),#90244) ;
#84528=STYLED_ITEM('',(#170169),#90245) ;
#84529=STYLED_ITEM('',(#170169),#90246) ;
#84530=STYLED_ITEM('',(#170169),#90247) ;
#84531=STYLED_ITEM('',(#170169),#90248) ;
#84532=STYLED_ITEM('',(#170169),#90249) ;
#84533=STYLED_ITEM('',(#170169),#90250) ;
#84534=STYLED_ITEM('',(#170169),#90251) ;
#84535=STYLED_ITEM('',(#170169),#90252) ;
#84536=STYLED_ITEM('',(#170169),#90253) ;
#84537=STYLED_ITEM('',(#170169),#90254) ;
#84538=STYLED_ITEM('',(#170169),#90255) ;
#84539=STYLED_ITEM('',(#170169),#90256) ;
#84540=STYLED_ITEM('',(#170169),#90257) ;
#84541=STYLED_ITEM('',(#170169),#90258) ;
#84542=STYLED_ITEM('',(#170169),#90259) ;
#84543=STYLED_ITEM('',(#170169),#90260) ;
#84544=STYLED_ITEM('',(#170169),#90261) ;
#84545=STYLED_ITEM('',(#170169),#90262) ;
#84546=STYLED_ITEM('',(#170169),#90263) ;
#84547=STYLED_ITEM('',(#170169),#90264) ;
#84548=STYLED_ITEM('',(#170169),#90265) ;
#84549=STYLED_ITEM('',(#170169),#90266) ;
#84550=STYLED_ITEM('',(#170169),#90267) ;
#84551=STYLED_ITEM('',(#170169),#90268) ;
#84552=STYLED_ITEM('',(#170169),#90269) ;
#84553=STYLED_ITEM('',(#170169),#90270) ;
#84554=STYLED_ITEM('',(#170169),#90271) ;
#84555=STYLED_ITEM('',(#170169),#90272) ;
#84556=STYLED_ITEM('',(#170169),#90273) ;
#84557=STYLED_ITEM('',(#170169),#90274) ;
#84558=STYLED_ITEM('',(#170169),#90275) ;
#84559=STYLED_ITEM('',(#170169),#90276) ;
#84560=STYLED_ITEM('',(#170169),#90277) ;
#84561=STYLED_ITEM('',(#170169),#90278) ;
#84562=STYLED_ITEM('',(#170169),#90279) ;
#84563=STYLED_ITEM('',(#170169),#90280) ;
#84564=STYLED_ITEM('',(#170169),#90281) ;
#84565=STYLED_ITEM('',(#170169),#90282) ;
#84566=STYLED_ITEM('',(#170169),#90283) ;
#84567=STYLED_ITEM('',(#170169),#90284) ;
#84568=STYLED_ITEM('',(#170169),#90285) ;
#84569=STYLED_ITEM('',(#170169),#90286) ;
#84570=STYLED_ITEM('',(#170169),#90287) ;
#84571=STYLED_ITEM('',(#170169),#90288) ;
#84572=STYLED_ITEM('',(#170169),#90289) ;
#84573=STYLED_ITEM('',(#170169),#90290) ;
#84574=STYLED_ITEM('',(#170169),#90291) ;
#84575=STYLED_ITEM('',(#170169),#90292) ;
#84576=STYLED_ITEM('',(#170169),#90293) ;
#84577=STYLED_ITEM('',(#170169),#90294) ;
#84578=STYLED_ITEM('',(#170169),#90295) ;
#84579=STYLED_ITEM('',(#170169),#90296) ;
#84580=STYLED_ITEM('',(#170169),#90297) ;
#84581=STYLED_ITEM('',(#170169),#90298) ;
#84582=STYLED_ITEM('',(#170169),#90299) ;
#84583=STYLED_ITEM('',(#170169),#90300) ;
#84584=STYLED_ITEM('',(#170169),#90301) ;
#84585=STYLED_ITEM('',(#170169),#90302) ;
#84586=STYLED_ITEM('',(#170169),#90303) ;
#84587=STYLED_ITEM('',(#170172),#90304) ;
#84588=STYLED_ITEM('',(#170172),#90305) ;
#84589=STYLED_ITEM('',(#170172),#90306) ;
#84590=STYLED_ITEM('',(#170172),#90307) ;
#84591=STYLED_ITEM('',(#170169),#90308) ;
#84592=STYLED_ITEM('',(#170169),#90309) ;
#84593=STYLED_ITEM('',(#170169),#90310) ;
#84594=STYLED_ITEM('',(#170169),#90311) ;
#84595=STYLED_ITEM('',(#170169),#90312) ;
#84596=STYLED_ITEM('',(#170169),#90313) ;
#84597=STYLED_ITEM('',(#170169),#90314) ;
#84598=STYLED_ITEM('',(#170169),#90315) ;
#84599=STYLED_ITEM('',(#170169),#90316) ;
#84600=STYLED_ITEM('',(#170169),#90317) ;
#84601=STYLED_ITEM('',(#170169),#90318) ;
#84602=STYLED_ITEM('',(#170169),#90319) ;
#84603=STYLED_ITEM('',(#170169),#90320) ;
#84604=STYLED_ITEM('',(#170169),#90321) ;
#84605=STYLED_ITEM('',(#170169),#90322) ;
#84606=STYLED_ITEM('',(#170169),#90323) ;
#84607=STYLED_ITEM('',(#170169),#90324) ;
#84608=STYLED_ITEM('',(#170169),#90325) ;
#84609=STYLED_ITEM('',(#170169),#90326) ;
#84610=STYLED_ITEM('',(#170169),#90327) ;
#84611=STYLED_ITEM('',(#170169),#90328) ;
#84612=STYLED_ITEM('',(#170169),#90329) ;
#84613=STYLED_ITEM('',(#170169),#90330) ;
#84614=STYLED_ITEM('',(#170169),#90331) ;
#84615=STYLED_ITEM('',(#170169),#90332) ;
#84616=STYLED_ITEM('',(#170169),#90333) ;
#84617=STYLED_ITEM('',(#170169),#90334) ;
#84618=STYLED_ITEM('',(#170169),#90335) ;
#84619=STYLED_ITEM('',(#170169),#90336) ;
#84620=STYLED_ITEM('',(#170169),#90337) ;
#84621=STYLED_ITEM('',(#170169),#90338) ;
#84622=STYLED_ITEM('',(#170169),#90339) ;
#84623=STYLED_ITEM('',(#170169),#90340) ;
#84624=STYLED_ITEM('',(#170169),#90341) ;
#84625=STYLED_ITEM('',(#170169),#90342) ;
#84626=STYLED_ITEM('',(#170169),#90343) ;
#84627=STYLED_ITEM('',(#170169),#90344) ;
#84628=STYLED_ITEM('',(#170169),#90345) ;
#84629=STYLED_ITEM('',(#170169),#90346) ;
#84630=STYLED_ITEM('',(#170169),#90347) ;
#84631=STYLED_ITEM('',(#170169),#90348) ;
#84632=STYLED_ITEM('',(#170169),#90349) ;
#84633=STYLED_ITEM('',(#170169),#90350) ;
#84634=STYLED_ITEM('',(#170169),#90351) ;
#84635=STYLED_ITEM('',(#170169),#90352) ;
#84636=STYLED_ITEM('',(#170169),#90353) ;
#84637=STYLED_ITEM('',(#170169),#90354) ;
#84638=STYLED_ITEM('',(#170169),#90355) ;
#84639=STYLED_ITEM('',(#170169),#90356) ;
#84640=STYLED_ITEM('',(#170169),#90357) ;
#84641=STYLED_ITEM('',(#170169),#90358) ;
#84642=STYLED_ITEM('',(#170169),#90359) ;
#84643=STYLED_ITEM('',(#170169),#90360) ;
#84644=STYLED_ITEM('',(#170169),#90361) ;
#84645=STYLED_ITEM('',(#170169),#90362) ;
#84646=STYLED_ITEM('',(#170169),#90363) ;
#84647=STYLED_ITEM('',(#170169),#90364) ;
#84648=STYLED_ITEM('',(#170169),#90365) ;
#84649=STYLED_ITEM('',(#170169),#90366) ;
#84650=STYLED_ITEM('',(#170169),#90367) ;
#84651=STYLED_ITEM('',(#170169),#90368) ;
#84652=STYLED_ITEM('',(#170169),#90369) ;
#84653=STYLED_ITEM('',(#170169),#90370) ;
#84654=STYLED_ITEM('',(#170169),#90371) ;
#84655=STYLED_ITEM('',(#170169),#90372) ;
#84656=STYLED_ITEM('',(#170169),#90373) ;
#84657=STYLED_ITEM('',(#170169),#90374) ;
#84658=STYLED_ITEM('',(#170169),#90375) ;
#84659=STYLED_ITEM('',(#170169),#90376) ;
#84660=STYLED_ITEM('',(#170169),#90377) ;
#84661=STYLED_ITEM('',(#170169),#90378) ;
#84662=STYLED_ITEM('',(#170169),#90379) ;
#84663=STYLED_ITEM('',(#170169),#90380) ;
#84664=STYLED_ITEM('',(#170169),#90381) ;
#84665=STYLED_ITEM('',(#170169),#90382) ;
#84666=STYLED_ITEM('',(#170169),#90383) ;
#84667=STYLED_ITEM('',(#170169),#90384) ;
#84668=STYLED_ITEM('',(#170169),#90385) ;
#84669=STYLED_ITEM('',(#170169),#90386) ;
#84670=STYLED_ITEM('',(#170169),#90387) ;
#84671=STYLED_ITEM('',(#170169),#90388) ;
#84672=STYLED_ITEM('',(#170169),#90389) ;
#84673=STYLED_ITEM('',(#170169),#90390) ;
#84674=STYLED_ITEM('',(#170169),#90391) ;
#84675=STYLED_ITEM('',(#170169),#90392) ;
#84676=STYLED_ITEM('',(#170169),#90393) ;
#84677=STYLED_ITEM('',(#170169),#90394) ;
#84678=STYLED_ITEM('',(#170169),#90395) ;
#84679=STYLED_ITEM('',(#170169),#90396) ;
#84680=STYLED_ITEM('',(#170169),#90397) ;
#84681=STYLED_ITEM('',(#170169),#90398) ;
#84682=STYLED_ITEM('',(#170169),#90399) ;
#84683=STYLED_ITEM('',(#170169),#90400) ;
#84684=STYLED_ITEM('',(#170169),#90401) ;
#84685=STYLED_ITEM('',(#170169),#90402) ;
#84686=STYLED_ITEM('',(#170169),#90403) ;
#84687=STYLED_ITEM('',(#170169),#90404) ;
#84688=STYLED_ITEM('',(#170169),#90405) ;
#84689=STYLED_ITEM('',(#170169),#90406) ;
#84690=STYLED_ITEM('',(#170169),#90407) ;
#84691=STYLED_ITEM('',(#170169),#90408) ;
#84692=STYLED_ITEM('',(#170169),#90409) ;
#84693=STYLED_ITEM('',(#170169),#90410) ;
#84694=STYLED_ITEM('',(#170169),#90411) ;
#84695=STYLED_ITEM('',(#170169),#90412) ;
#84696=STYLED_ITEM('',(#170169),#90413) ;
#84697=STYLED_ITEM('',(#170169),#90414) ;
#84698=STYLED_ITEM('',(#170169),#90415) ;
#84699=STYLED_ITEM('',(#170169),#90416) ;
#84700=STYLED_ITEM('',(#170169),#90417) ;
#84701=STYLED_ITEM('',(#170169),#90418) ;
#84702=STYLED_ITEM('',(#170169),#90419) ;
#84703=STYLED_ITEM('',(#170169),#90420) ;
#84704=STYLED_ITEM('',(#170169),#90421) ;
#84705=STYLED_ITEM('',(#170169),#90422) ;
#84706=STYLED_ITEM('',(#170169),#90423) ;
#84707=STYLED_ITEM('',(#170169),#90424) ;
#84708=STYLED_ITEM('',(#170169),#90425) ;
#84709=STYLED_ITEM('',(#170169),#90426) ;
#84710=STYLED_ITEM('',(#170169),#90427) ;
#84711=STYLED_ITEM('',(#170169),#90428) ;
#84712=STYLED_ITEM('',(#170169),#90429) ;
#84713=STYLED_ITEM('',(#170169),#90430) ;
#84714=STYLED_ITEM('',(#170169),#90431) ;
#84715=STYLED_ITEM('',(#170169),#90432) ;
#84716=STYLED_ITEM('',(#170169),#90433) ;
#84717=STYLED_ITEM('',(#170169),#90434) ;
#84718=STYLED_ITEM('',(#170169),#90435) ;
#84719=STYLED_ITEM('',(#170169),#90436) ;
#84720=STYLED_ITEM('',(#170169),#90437) ;
#84721=STYLED_ITEM('',(#170169),#90438) ;
#84722=STYLED_ITEM('',(#170169),#90439) ;
#84723=STYLED_ITEM('',(#170169),#90440) ;
#84724=STYLED_ITEM('',(#170169),#90441) ;
#84725=STYLED_ITEM('',(#170169),#90442) ;
#84726=STYLED_ITEM('',(#170169),#90443) ;
#84727=STYLED_ITEM('',(#170172),#90444) ;
#84728=STYLED_ITEM('',(#170172),#90445) ;
#84729=STYLED_ITEM('',(#170172),#90446) ;
#84730=STYLED_ITEM('',(#170172),#90447) ;
#84731=STYLED_ITEM('',(#170169),#90448) ;
#84732=STYLED_ITEM('',(#170169),#90449) ;
#84733=STYLED_ITEM('',(#170169),#90450) ;
#84734=STYLED_ITEM('',(#170169),#90451) ;
#84735=STYLED_ITEM('',(#170169),#90452) ;
#84736=STYLED_ITEM('',(#170169),#90453) ;
#84737=STYLED_ITEM('',(#170169),#90454) ;
#84738=STYLED_ITEM('',(#170169),#90455) ;
#84739=STYLED_ITEM('',(#170169),#90456) ;
#84740=STYLED_ITEM('',(#170169),#90457) ;
#84741=STYLED_ITEM('',(#170169),#90458) ;
#84742=STYLED_ITEM('',(#170169),#90459) ;
#84743=STYLED_ITEM('',(#170169),#90460) ;
#84744=STYLED_ITEM('',(#170169),#90461) ;
#84745=STYLED_ITEM('',(#170169),#90462) ;
#84746=STYLED_ITEM('',(#170169),#90463) ;
#84747=STYLED_ITEM('',(#170169),#90464) ;
#84748=STYLED_ITEM('',(#170169),#90465) ;
#84749=STYLED_ITEM('',(#170169),#90466) ;
#84750=STYLED_ITEM('',(#170169),#90467) ;
#84751=STYLED_ITEM('',(#170169),#90468) ;
#84752=STYLED_ITEM('',(#170169),#90469) ;
#84753=STYLED_ITEM('',(#170169),#90470) ;
#84754=STYLED_ITEM('',(#170169),#90471) ;
#84755=STYLED_ITEM('',(#170169),#90472) ;
#84756=STYLED_ITEM('',(#170169),#90473) ;
#84757=STYLED_ITEM('',(#170169),#90474) ;
#84758=STYLED_ITEM('',(#170169),#90475) ;
#84759=STYLED_ITEM('',(#170169),#90476) ;
#84760=STYLED_ITEM('',(#170169),#90477) ;
#84761=STYLED_ITEM('',(#170169),#90478) ;
#84762=STYLED_ITEM('',(#170169),#90479) ;
#84763=STYLED_ITEM('',(#170169),#90480) ;
#84764=STYLED_ITEM('',(#170169),#90481) ;
#84765=STYLED_ITEM('',(#170169),#90482) ;
#84766=STYLED_ITEM('',(#170169),#90483) ;
#84767=STYLED_ITEM('',(#170169),#90484) ;
#84768=STYLED_ITEM('',(#170169),#90485) ;
#84769=STYLED_ITEM('',(#170169),#90486) ;
#84770=STYLED_ITEM('',(#170169),#90487) ;
#84771=STYLED_ITEM('',(#170169),#90488) ;
#84772=STYLED_ITEM('',(#170169),#90489) ;
#84773=STYLED_ITEM('',(#170169),#90490) ;
#84774=STYLED_ITEM('',(#170169),#90491) ;
#84775=STYLED_ITEM('',(#170169),#90492) ;
#84776=STYLED_ITEM('',(#170169),#90493) ;
#84777=STYLED_ITEM('',(#170169),#90494) ;
#84778=STYLED_ITEM('',(#170169),#90495) ;
#84779=STYLED_ITEM('',(#170169),#90496) ;
#84780=STYLED_ITEM('',(#170169),#90497) ;
#84781=STYLED_ITEM('',(#170169),#90498) ;
#84782=STYLED_ITEM('',(#170169),#90499) ;
#84783=STYLED_ITEM('',(#170169),#90500) ;
#84784=STYLED_ITEM('',(#170169),#90501) ;
#84785=STYLED_ITEM('',(#170169),#90502) ;
#84786=STYLED_ITEM('',(#170169),#90503) ;
#84787=STYLED_ITEM('',(#170169),#90504) ;
#84788=STYLED_ITEM('',(#170169),#90505) ;
#84789=STYLED_ITEM('',(#170169),#90506) ;
#84790=STYLED_ITEM('',(#170169),#90507) ;
#84791=STYLED_ITEM('',(#170169),#90508) ;
#84792=STYLED_ITEM('',(#170169),#90509) ;
#84793=STYLED_ITEM('',(#170169),#90510) ;
#84794=STYLED_ITEM('',(#170169),#90511) ;
#84795=STYLED_ITEM('',(#170169),#90512) ;
#84796=STYLED_ITEM('',(#170169),#90513) ;
#84797=STYLED_ITEM('',(#170169),#90514) ;
#84798=STYLED_ITEM('',(#170169),#90515) ;
#84799=STYLED_ITEM('',(#170169),#90516) ;
#84800=STYLED_ITEM('',(#170169),#90517) ;
#84801=STYLED_ITEM('',(#170169),#90518) ;
#84802=STYLED_ITEM('',(#170169),#90519) ;
#84803=STYLED_ITEM('',(#170169),#90520) ;
#84804=STYLED_ITEM('',(#170169),#90521) ;
#84805=STYLED_ITEM('',(#170169),#90522) ;
#84806=STYLED_ITEM('',(#170169),#90523) ;
#84807=STYLED_ITEM('',(#170169),#90524) ;
#84808=STYLED_ITEM('',(#170169),#90525) ;
#84809=STYLED_ITEM('',(#170169),#90526) ;
#84810=STYLED_ITEM('',(#170169),#90527) ;
#84811=STYLED_ITEM('',(#170169),#90528) ;
#84812=STYLED_ITEM('',(#170169),#90529) ;
#84813=STYLED_ITEM('',(#170169),#90530) ;
#84814=STYLED_ITEM('',(#170169),#90531) ;
#84815=STYLED_ITEM('',(#170169),#90532) ;
#84816=STYLED_ITEM('',(#170169),#90533) ;
#84817=STYLED_ITEM('',(#170169),#90534) ;
#84818=STYLED_ITEM('',(#170169),#90535) ;
#84819=STYLED_ITEM('',(#170169),#90536) ;
#84820=STYLED_ITEM('',(#170169),#90537) ;
#84821=STYLED_ITEM('',(#170169),#90538) ;
#84822=STYLED_ITEM('',(#170169),#90539) ;
#84823=STYLED_ITEM('',(#170169),#90540) ;
#84824=STYLED_ITEM('',(#170169),#90541) ;
#84825=STYLED_ITEM('',(#170169),#90542) ;
#84826=STYLED_ITEM('',(#170169),#90543) ;
#84827=STYLED_ITEM('',(#170169),#90544) ;
#84828=STYLED_ITEM('',(#170169),#90545) ;
#84829=STYLED_ITEM('',(#170169),#90546) ;
#84830=STYLED_ITEM('',(#170169),#90547) ;
#84831=STYLED_ITEM('',(#170169),#90548) ;
#84832=STYLED_ITEM('',(#170169),#90549) ;
#84833=STYLED_ITEM('',(#170169),#90550) ;
#84834=STYLED_ITEM('',(#170169),#90551) ;
#84835=STYLED_ITEM('',(#170169),#90552) ;
#84836=STYLED_ITEM('',(#170169),#90553) ;
#84837=STYLED_ITEM('',(#170169),#90554) ;
#84838=STYLED_ITEM('',(#170169),#90555) ;
#84839=STYLED_ITEM('',(#170169),#90556) ;
#84840=STYLED_ITEM('',(#170169),#90557) ;
#84841=STYLED_ITEM('',(#170169),#90558) ;
#84842=STYLED_ITEM('',(#170169),#90559) ;
#84843=STYLED_ITEM('',(#170169),#90560) ;
#84844=STYLED_ITEM('',(#170169),#90561) ;
#84845=STYLED_ITEM('',(#170169),#90562) ;
#84846=STYLED_ITEM('',(#170169),#90563) ;
#84847=STYLED_ITEM('',(#170169),#90564) ;
#84848=STYLED_ITEM('',(#170169),#90565) ;
#84849=STYLED_ITEM('',(#170169),#90566) ;
#84850=STYLED_ITEM('',(#170169),#90567) ;
#84851=STYLED_ITEM('',(#170169),#90568) ;
#84852=STYLED_ITEM('',(#170169),#90569) ;
#84853=STYLED_ITEM('',(#170169),#90570) ;
#84854=STYLED_ITEM('',(#170169),#90571) ;
#84855=STYLED_ITEM('',(#170169),#90572) ;
#84856=STYLED_ITEM('',(#170169),#90573) ;
#84857=STYLED_ITEM('',(#170169),#90574) ;
#84858=STYLED_ITEM('',(#170169),#90575) ;
#84859=STYLED_ITEM('',(#170169),#90576) ;
#84860=STYLED_ITEM('',(#170169),#90577) ;
#84861=STYLED_ITEM('',(#170169),#90578) ;
#84862=STYLED_ITEM('',(#170169),#90579) ;
#84863=STYLED_ITEM('',(#170169),#90580) ;
#84864=STYLED_ITEM('',(#170169),#90581) ;
#84865=STYLED_ITEM('',(#170169),#90582) ;
#84866=STYLED_ITEM('',(#170169),#90583) ;
#84867=STYLED_ITEM('',(#170172),#90584) ;
#84868=STYLED_ITEM('',(#170172),#90585) ;
#84869=STYLED_ITEM('',(#170172),#90586) ;
#84870=STYLED_ITEM('',(#170172),#90587) ;
#84871=STYLED_ITEM('',(#170169),#90588) ;
#84872=STYLED_ITEM('',(#170169),#90589) ;
#84873=STYLED_ITEM('',(#170169),#90590) ;
#84874=STYLED_ITEM('',(#170169),#90591) ;
#84875=STYLED_ITEM('',(#170169),#90592) ;
#84876=STYLED_ITEM('',(#170169),#90593) ;
#84877=STYLED_ITEM('',(#170169),#90594) ;
#84878=STYLED_ITEM('',(#170169),#90595) ;
#84879=STYLED_ITEM('',(#170169),#90596) ;
#84880=STYLED_ITEM('',(#170169),#90597) ;
#84881=STYLED_ITEM('',(#170169),#90598) ;
#84882=STYLED_ITEM('',(#170169),#90599) ;
#84883=STYLED_ITEM('',(#170169),#90600) ;
#84884=STYLED_ITEM('',(#170169),#90601) ;
#84885=STYLED_ITEM('',(#170169),#90602) ;
#84886=STYLED_ITEM('',(#170169),#90603) ;
#84887=STYLED_ITEM('',(#170169),#90604) ;
#84888=STYLED_ITEM('',(#170169),#90605) ;
#84889=STYLED_ITEM('',(#170169),#90606) ;
#84890=STYLED_ITEM('',(#170169),#90607) ;
#84891=STYLED_ITEM('',(#170169),#90608) ;
#84892=STYLED_ITEM('',(#170169),#90609) ;
#84893=STYLED_ITEM('',(#170169),#90610) ;
#84894=STYLED_ITEM('',(#170169),#90611) ;
#84895=STYLED_ITEM('',(#170169),#90612) ;
#84896=STYLED_ITEM('',(#170169),#90613) ;
#84897=STYLED_ITEM('',(#170169),#90614) ;
#84898=STYLED_ITEM('',(#170169),#90615) ;
#84899=STYLED_ITEM('',(#170169),#90616) ;
#84900=STYLED_ITEM('',(#170169),#90617) ;
#84901=STYLED_ITEM('',(#170169),#90618) ;
#84902=STYLED_ITEM('',(#170169),#90619) ;
#84903=STYLED_ITEM('',(#170169),#90620) ;
#84904=STYLED_ITEM('',(#170169),#90621) ;
#84905=STYLED_ITEM('',(#170169),#90622) ;
#84906=STYLED_ITEM('',(#170169),#90623) ;
#84907=STYLED_ITEM('',(#170169),#90624) ;
#84908=STYLED_ITEM('',(#170169),#90625) ;
#84909=STYLED_ITEM('',(#170169),#90626) ;
#84910=STYLED_ITEM('',(#170169),#90627) ;
#84911=STYLED_ITEM('',(#170169),#90628) ;
#84912=STYLED_ITEM('',(#170169),#90629) ;
#84913=STYLED_ITEM('',(#170169),#90630) ;
#84914=STYLED_ITEM('',(#170169),#90631) ;
#84915=STYLED_ITEM('',(#170169),#90632) ;
#84916=STYLED_ITEM('',(#170169),#90633) ;
#84917=STYLED_ITEM('',(#170169),#90634) ;
#84918=STYLED_ITEM('',(#170169),#90635) ;
#84919=STYLED_ITEM('',(#170169),#90636) ;
#84920=STYLED_ITEM('',(#170169),#90637) ;
#84921=STYLED_ITEM('',(#170169),#90638) ;
#84922=STYLED_ITEM('',(#170169),#90639) ;
#84923=STYLED_ITEM('',(#170169),#90640) ;
#84924=STYLED_ITEM('',(#170169),#90641) ;
#84925=STYLED_ITEM('',(#170169),#90642) ;
#84926=STYLED_ITEM('',(#170169),#90643) ;
#84927=STYLED_ITEM('',(#170169),#90644) ;
#84928=STYLED_ITEM('',(#170169),#90645) ;
#84929=STYLED_ITEM('',(#170169),#90646) ;
#84930=STYLED_ITEM('',(#170169),#90647) ;
#84931=STYLED_ITEM('',(#170169),#90648) ;
#84932=STYLED_ITEM('',(#170169),#90649) ;
#84933=STYLED_ITEM('',(#170169),#90650) ;
#84934=STYLED_ITEM('',(#170169),#90651) ;
#84935=STYLED_ITEM('',(#170169),#90652) ;
#84936=STYLED_ITEM('',(#170169),#90653) ;
#84937=STYLED_ITEM('',(#170169),#90654) ;
#84938=STYLED_ITEM('',(#170169),#90655) ;
#84939=STYLED_ITEM('',(#170169),#90656) ;
#84940=STYLED_ITEM('',(#170169),#90657) ;
#84941=STYLED_ITEM('',(#170169),#90658) ;
#84942=STYLED_ITEM('',(#170169),#90659) ;
#84943=STYLED_ITEM('',(#170169),#90660) ;
#84944=STYLED_ITEM('',(#170169),#90661) ;
#84945=STYLED_ITEM('',(#170169),#90662) ;
#84946=STYLED_ITEM('',(#170169),#90663) ;
#84947=STYLED_ITEM('',(#170169),#90664) ;
#84948=STYLED_ITEM('',(#170169),#90665) ;
#84949=STYLED_ITEM('',(#170169),#90666) ;
#84950=STYLED_ITEM('',(#170169),#90667) ;
#84951=STYLED_ITEM('',(#170169),#90668) ;
#84952=STYLED_ITEM('',(#170169),#90669) ;
#84953=STYLED_ITEM('',(#170169),#90670) ;
#84954=STYLED_ITEM('',(#170169),#90671) ;
#84955=STYLED_ITEM('',(#170169),#90672) ;
#84956=STYLED_ITEM('',(#170169),#90673) ;
#84957=STYLED_ITEM('',(#170169),#90674) ;
#84958=STYLED_ITEM('',(#170169),#90675) ;
#84959=STYLED_ITEM('',(#170169),#90676) ;
#84960=STYLED_ITEM('',(#170169),#90677) ;
#84961=STYLED_ITEM('',(#170169),#90678) ;
#84962=STYLED_ITEM('',(#170169),#90679) ;
#84963=STYLED_ITEM('',(#170169),#90680) ;
#84964=STYLED_ITEM('',(#170169),#90681) ;
#84965=STYLED_ITEM('',(#170169),#90682) ;
#84966=STYLED_ITEM('',(#170169),#90683) ;
#84967=STYLED_ITEM('',(#170169),#90684) ;
#84968=STYLED_ITEM('',(#170169),#90685) ;
#84969=STYLED_ITEM('',(#170169),#90686) ;
#84970=STYLED_ITEM('',(#170169),#90687) ;
#84971=STYLED_ITEM('',(#170169),#90688) ;
#84972=STYLED_ITEM('',(#170169),#90689) ;
#84973=STYLED_ITEM('',(#170169),#90690) ;
#84974=STYLED_ITEM('',(#170169),#90691) ;
#84975=STYLED_ITEM('',(#170169),#90692) ;
#84976=STYLED_ITEM('',(#170169),#90693) ;
#84977=STYLED_ITEM('',(#170169),#90694) ;
#84978=STYLED_ITEM('',(#170169),#90695) ;
#84979=STYLED_ITEM('',(#170169),#90696) ;
#84980=STYLED_ITEM('',(#170169),#90697) ;
#84981=STYLED_ITEM('',(#170169),#90698) ;
#84982=STYLED_ITEM('',(#170169),#90699) ;
#84983=STYLED_ITEM('',(#170169),#90700) ;
#84984=STYLED_ITEM('',(#170169),#90701) ;
#84985=STYLED_ITEM('',(#170169),#90702) ;
#84986=STYLED_ITEM('',(#170169),#90703) ;
#84987=STYLED_ITEM('',(#170169),#90704) ;
#84988=STYLED_ITEM('',(#170169),#90705) ;
#84989=STYLED_ITEM('',(#170169),#90706) ;
#84990=STYLED_ITEM('',(#170169),#90707) ;
#84991=STYLED_ITEM('',(#170169),#90708) ;
#84992=STYLED_ITEM('',(#170169),#90709) ;
#84993=STYLED_ITEM('',(#170169),#90710) ;
#84994=STYLED_ITEM('',(#170169),#90711) ;
#84995=STYLED_ITEM('',(#170169),#90712) ;
#84996=STYLED_ITEM('',(#170169),#90713) ;
#84997=STYLED_ITEM('',(#170169),#90714) ;
#84998=STYLED_ITEM('',(#170169),#90715) ;
#84999=STYLED_ITEM('',(#170169),#90716) ;
#85000=STYLED_ITEM('',(#170169),#90717) ;
#85001=STYLED_ITEM('',(#170169),#90718) ;
#85002=STYLED_ITEM('',(#170169),#90719) ;
#85003=STYLED_ITEM('',(#170169),#90720) ;
#85004=STYLED_ITEM('',(#170169),#90721) ;
#85005=STYLED_ITEM('',(#170169),#90722) ;
#85006=STYLED_ITEM('',(#170169),#90723) ;
#85007=STYLED_ITEM('',(#170172),#90724) ;
#85008=STYLED_ITEM('',(#170172),#90725) ;
#85009=STYLED_ITEM('',(#170172),#90726) ;
#85010=STYLED_ITEM('',(#170172),#90727) ;
#85011=STYLED_ITEM('',(#170169),#90728) ;
#85012=STYLED_ITEM('',(#170169),#90729) ;
#85013=STYLED_ITEM('',(#170169),#90730) ;
#85014=STYLED_ITEM('',(#170169),#90731) ;
#85015=STYLED_ITEM('',(#170169),#90732) ;
#85016=STYLED_ITEM('',(#170169),#90733) ;
#85017=STYLED_ITEM('',(#170169),#90734) ;
#85018=STYLED_ITEM('',(#170169),#90735) ;
#85019=STYLED_ITEM('',(#170169),#90736) ;
#85020=STYLED_ITEM('',(#170169),#90737) ;
#85021=STYLED_ITEM('',(#170169),#90738) ;
#85022=STYLED_ITEM('',(#170169),#90739) ;
#85023=STYLED_ITEM('',(#170169),#90740) ;
#85024=STYLED_ITEM('',(#170169),#90741) ;
#85025=STYLED_ITEM('',(#170169),#90742) ;
#85026=STYLED_ITEM('',(#170169),#90743) ;
#85027=STYLED_ITEM('',(#170169),#90744) ;
#85028=STYLED_ITEM('',(#170169),#90745) ;
#85029=STYLED_ITEM('',(#170169),#90746) ;
#85030=STYLED_ITEM('',(#170169),#90747) ;
#85031=STYLED_ITEM('',(#170169),#90748) ;
#85032=STYLED_ITEM('',(#170169),#90749) ;
#85033=STYLED_ITEM('',(#170169),#90750) ;
#85034=STYLED_ITEM('',(#170169),#90751) ;
#85035=STYLED_ITEM('',(#170169),#90752) ;
#85036=STYLED_ITEM('',(#170169),#90753) ;
#85037=STYLED_ITEM('',(#170169),#90754) ;
#85038=STYLED_ITEM('',(#170169),#90755) ;
#85039=STYLED_ITEM('',(#170169),#90756) ;
#85040=STYLED_ITEM('',(#170169),#90757) ;
#85041=STYLED_ITEM('',(#170169),#90758) ;
#85042=STYLED_ITEM('',(#170169),#90759) ;
#85043=STYLED_ITEM('',(#170169),#90760) ;
#85044=STYLED_ITEM('',(#170169),#90761) ;
#85045=STYLED_ITEM('',(#170169),#90762) ;
#85046=STYLED_ITEM('',(#170169),#90763) ;
#85047=STYLED_ITEM('',(#170169),#90764) ;
#85048=STYLED_ITEM('',(#170169),#90765) ;
#85049=STYLED_ITEM('',(#170169),#90766) ;
#85050=STYLED_ITEM('',(#170169),#90767) ;
#85051=STYLED_ITEM('',(#170169),#90768) ;
#85052=STYLED_ITEM('',(#170169),#90769) ;
#85053=STYLED_ITEM('',(#170169),#90770) ;
#85054=STYLED_ITEM('',(#170169),#90771) ;
#85055=STYLED_ITEM('',(#170169),#90772) ;
#85056=STYLED_ITEM('',(#170169),#90773) ;
#85057=STYLED_ITEM('',(#170169),#90774) ;
#85058=STYLED_ITEM('',(#170169),#90775) ;
#85059=STYLED_ITEM('',(#170169),#90776) ;
#85060=STYLED_ITEM('',(#170169),#90777) ;
#85061=STYLED_ITEM('',(#170169),#90778) ;
#85062=STYLED_ITEM('',(#170169),#90779) ;
#85063=STYLED_ITEM('',(#170169),#90780) ;
#85064=STYLED_ITEM('',(#170169),#90781) ;
#85065=STYLED_ITEM('',(#170169),#90782) ;
#85066=STYLED_ITEM('',(#170169),#90783) ;
#85067=STYLED_ITEM('',(#170169),#90784) ;
#85068=STYLED_ITEM('',(#170169),#90785) ;
#85069=STYLED_ITEM('',(#170169),#90786) ;
#85070=STYLED_ITEM('',(#170169),#90787) ;
#85071=STYLED_ITEM('',(#170169),#90788) ;
#85072=STYLED_ITEM('',(#170169),#90789) ;
#85073=STYLED_ITEM('',(#170169),#90790) ;
#85074=STYLED_ITEM('',(#170169),#90791) ;
#85075=STYLED_ITEM('',(#170169),#90792) ;
#85076=STYLED_ITEM('',(#170169),#90793) ;
#85077=STYLED_ITEM('',(#170169),#90794) ;
#85078=STYLED_ITEM('',(#170169),#90795) ;
#85079=STYLED_ITEM('',(#170169),#90796) ;
#85080=STYLED_ITEM('',(#170169),#90797) ;
#85081=STYLED_ITEM('',(#170169),#90798) ;
#85082=STYLED_ITEM('',(#170169),#90799) ;
#85083=STYLED_ITEM('',(#170169),#90800) ;
#85084=STYLED_ITEM('',(#170169),#90801) ;
#85085=STYLED_ITEM('',(#170169),#90802) ;
#85086=STYLED_ITEM('',(#170169),#90803) ;
#85087=STYLED_ITEM('',(#170169),#90804) ;
#85088=STYLED_ITEM('',(#170169),#90805) ;
#85089=STYLED_ITEM('',(#170169),#90806) ;
#85090=STYLED_ITEM('',(#170169),#90807) ;
#85091=STYLED_ITEM('',(#170169),#90808) ;
#85092=STYLED_ITEM('',(#170169),#90809) ;
#85093=STYLED_ITEM('',(#170169),#90810) ;
#85094=STYLED_ITEM('',(#170169),#90811) ;
#85095=STYLED_ITEM('',(#170169),#90812) ;
#85096=STYLED_ITEM('',(#170169),#90813) ;
#85097=STYLED_ITEM('',(#170169),#90814) ;
#85098=STYLED_ITEM('',(#170169),#90815) ;
#85099=STYLED_ITEM('',(#170169),#90816) ;
#85100=STYLED_ITEM('',(#170169),#90817) ;
#85101=STYLED_ITEM('',(#170169),#90818) ;
#85102=STYLED_ITEM('',(#170169),#90819) ;
#85103=STYLED_ITEM('',(#170169),#90820) ;
#85104=STYLED_ITEM('',(#170169),#90821) ;
#85105=STYLED_ITEM('',(#170169),#90822) ;
#85106=STYLED_ITEM('',(#170169),#90823) ;
#85107=STYLED_ITEM('',(#170169),#90824) ;
#85108=STYLED_ITEM('',(#170169),#90825) ;
#85109=STYLED_ITEM('',(#170169),#90826) ;
#85110=STYLED_ITEM('',(#170169),#90827) ;
#85111=STYLED_ITEM('',(#170169),#90828) ;
#85112=STYLED_ITEM('',(#170169),#90829) ;
#85113=STYLED_ITEM('',(#170169),#90830) ;
#85114=STYLED_ITEM('',(#170169),#90831) ;
#85115=STYLED_ITEM('',(#170169),#90832) ;
#85116=STYLED_ITEM('',(#170169),#90833) ;
#85117=STYLED_ITEM('',(#170169),#90834) ;
#85118=STYLED_ITEM('',(#170169),#90835) ;
#85119=STYLED_ITEM('',(#170169),#90836) ;
#85120=STYLED_ITEM('',(#170169),#90837) ;
#85121=STYLED_ITEM('',(#170169),#90838) ;
#85122=STYLED_ITEM('',(#170169),#90839) ;
#85123=STYLED_ITEM('',(#170169),#90840) ;
#85124=STYLED_ITEM('',(#170169),#90841) ;
#85125=STYLED_ITEM('',(#170169),#90842) ;
#85126=STYLED_ITEM('',(#170169),#90843) ;
#85127=STYLED_ITEM('',(#170169),#90844) ;
#85128=STYLED_ITEM('',(#170169),#90845) ;
#85129=STYLED_ITEM('',(#170169),#90846) ;
#85130=STYLED_ITEM('',(#170169),#90847) ;
#85131=STYLED_ITEM('',(#170169),#90848) ;
#85132=STYLED_ITEM('',(#170169),#90849) ;
#85133=STYLED_ITEM('',(#170169),#90850) ;
#85134=STYLED_ITEM('',(#170169),#90851) ;
#85135=STYLED_ITEM('',(#170169),#90852) ;
#85136=STYLED_ITEM('',(#170169),#90853) ;
#85137=STYLED_ITEM('',(#170169),#90854) ;
#85138=STYLED_ITEM('',(#170169),#90855) ;
#85139=STYLED_ITEM('',(#170169),#90856) ;
#85140=STYLED_ITEM('',(#170169),#90857) ;
#85141=STYLED_ITEM('',(#170169),#90858) ;
#85142=STYLED_ITEM('',(#170169),#90859) ;
#85143=STYLED_ITEM('',(#170169),#90860) ;
#85144=STYLED_ITEM('',(#170169),#90861) ;
#85145=STYLED_ITEM('',(#170169),#90862) ;
#85146=STYLED_ITEM('',(#170169),#90863) ;
#85147=STYLED_ITEM('',(#170172),#90864) ;
#85148=STYLED_ITEM('',(#170172),#90865) ;
#85149=STYLED_ITEM('',(#170172),#90866) ;
#85150=STYLED_ITEM('',(#170172),#90867) ;
#85151=STYLED_ITEM('',(#170169),#90868) ;
#85152=STYLED_ITEM('',(#170169),#90869) ;
#85153=STYLED_ITEM('',(#170169),#90870) ;
#85154=STYLED_ITEM('',(#170169),#90871) ;
#85155=STYLED_ITEM('',(#170169),#90872) ;
#85156=STYLED_ITEM('',(#170169),#90873) ;
#85157=STYLED_ITEM('',(#170169),#90874) ;
#85158=STYLED_ITEM('',(#170169),#90875) ;
#85159=STYLED_ITEM('',(#170169),#90876) ;
#85160=STYLED_ITEM('',(#170169),#90877) ;
#85161=STYLED_ITEM('',(#170169),#90878) ;
#85162=STYLED_ITEM('',(#170169),#90879) ;
#85163=STYLED_ITEM('',(#170169),#90880) ;
#85164=STYLED_ITEM('',(#170169),#90881) ;
#85165=STYLED_ITEM('',(#170169),#90882) ;
#85166=STYLED_ITEM('',(#170169),#90883) ;
#85167=STYLED_ITEM('',(#170169),#90884) ;
#85168=STYLED_ITEM('',(#170169),#90885) ;
#85169=STYLED_ITEM('',(#170169),#90886) ;
#85170=STYLED_ITEM('',(#170169),#90887) ;
#85171=STYLED_ITEM('',(#170169),#90888) ;
#85172=STYLED_ITEM('',(#170169),#90889) ;
#85173=STYLED_ITEM('',(#170169),#90890) ;
#85174=STYLED_ITEM('',(#170169),#90891) ;
#85175=STYLED_ITEM('',(#170169),#90892) ;
#85176=STYLED_ITEM('',(#170169),#90893) ;
#85177=STYLED_ITEM('',(#170169),#90894) ;
#85178=STYLED_ITEM('',(#170169),#90895) ;
#85179=STYLED_ITEM('',(#170169),#90896) ;
#85180=STYLED_ITEM('',(#170169),#90897) ;
#85181=STYLED_ITEM('',(#170169),#90898) ;
#85182=STYLED_ITEM('',(#170169),#90899) ;
#85183=STYLED_ITEM('',(#170169),#90900) ;
#85184=STYLED_ITEM('',(#170169),#90901) ;
#85185=STYLED_ITEM('',(#170169),#90902) ;
#85186=STYLED_ITEM('',(#170169),#90903) ;
#85187=STYLED_ITEM('',(#170169),#90904) ;
#85188=STYLED_ITEM('',(#170169),#90905) ;
#85189=STYLED_ITEM('',(#170169),#90906) ;
#85190=STYLED_ITEM('',(#170169),#90907) ;
#85191=STYLED_ITEM('',(#170169),#90908) ;
#85192=STYLED_ITEM('',(#170169),#90909) ;
#85193=STYLED_ITEM('',(#170169),#90910) ;
#85194=STYLED_ITEM('',(#170169),#90911) ;
#85195=STYLED_ITEM('',(#170169),#90912) ;
#85196=STYLED_ITEM('',(#170169),#90913) ;
#85197=STYLED_ITEM('',(#170169),#90914) ;
#85198=STYLED_ITEM('',(#170169),#90915) ;
#85199=STYLED_ITEM('',(#170169),#90916) ;
#85200=STYLED_ITEM('',(#170169),#90917) ;
#85201=STYLED_ITEM('',(#170169),#90918) ;
#85202=STYLED_ITEM('',(#170169),#90919) ;
#85203=STYLED_ITEM('',(#170169),#90920) ;
#85204=STYLED_ITEM('',(#170169),#90921) ;
#85205=STYLED_ITEM('',(#170169),#90922) ;
#85206=STYLED_ITEM('',(#170169),#90923) ;
#85207=STYLED_ITEM('',(#170169),#90924) ;
#85208=STYLED_ITEM('',(#170169),#90925) ;
#85209=STYLED_ITEM('',(#170169),#90926) ;
#85210=STYLED_ITEM('',(#170169),#90927) ;
#85211=STYLED_ITEM('',(#170169),#90928) ;
#85212=STYLED_ITEM('',(#170169),#90929) ;
#85213=STYLED_ITEM('',(#170169),#90930) ;
#85214=STYLED_ITEM('',(#170169),#90931) ;
#85215=STYLED_ITEM('',(#170169),#90932) ;
#85216=STYLED_ITEM('',(#170169),#90933) ;
#85217=STYLED_ITEM('',(#170169),#90934) ;
#85218=STYLED_ITEM('',(#170169),#90935) ;
#85219=STYLED_ITEM('',(#170169),#90936) ;
#85220=STYLED_ITEM('',(#170169),#90937) ;
#85221=STYLED_ITEM('',(#170169),#90938) ;
#85222=STYLED_ITEM('',(#170169),#90939) ;
#85223=STYLED_ITEM('',(#170169),#90940) ;
#85224=STYLED_ITEM('',(#170169),#90941) ;
#85225=STYLED_ITEM('',(#170169),#90942) ;
#85226=STYLED_ITEM('',(#170169),#90943) ;
#85227=STYLED_ITEM('',(#170169),#90944) ;
#85228=STYLED_ITEM('',(#170169),#90945) ;
#85229=STYLED_ITEM('',(#170169),#90946) ;
#85230=STYLED_ITEM('',(#170169),#90947) ;
#85231=STYLED_ITEM('',(#170169),#90948) ;
#85232=STYLED_ITEM('',(#170169),#90949) ;
#85233=STYLED_ITEM('',(#170169),#90950) ;
#85234=STYLED_ITEM('',(#170169),#90951) ;
#85235=STYLED_ITEM('',(#170169),#90952) ;
#85236=STYLED_ITEM('',(#170169),#90953) ;
#85237=STYLED_ITEM('',(#170169),#90954) ;
#85238=STYLED_ITEM('',(#170169),#90955) ;
#85239=STYLED_ITEM('',(#170169),#90956) ;
#85240=STYLED_ITEM('',(#170169),#90957) ;
#85241=STYLED_ITEM('',(#170169),#90958) ;
#85242=STYLED_ITEM('',(#170169),#90959) ;
#85243=STYLED_ITEM('',(#170169),#90960) ;
#85244=STYLED_ITEM('',(#170169),#90961) ;
#85245=STYLED_ITEM('',(#170169),#90962) ;
#85246=STYLED_ITEM('',(#170169),#90963) ;
#85247=STYLED_ITEM('',(#170169),#90964) ;
#85248=STYLED_ITEM('',(#170169),#90965) ;
#85249=STYLED_ITEM('',(#170169),#90966) ;
#85250=STYLED_ITEM('',(#170169),#90967) ;
#85251=STYLED_ITEM('',(#170169),#90968) ;
#85252=STYLED_ITEM('',(#170169),#90969) ;
#85253=STYLED_ITEM('',(#170169),#90970) ;
#85254=STYLED_ITEM('',(#170169),#90971) ;
#85255=STYLED_ITEM('',(#170169),#90972) ;
#85256=STYLED_ITEM('',(#170169),#90973) ;
#85257=STYLED_ITEM('',(#170169),#90974) ;
#85258=STYLED_ITEM('',(#170169),#90975) ;
#85259=STYLED_ITEM('',(#170169),#90976) ;
#85260=STYLED_ITEM('',(#170169),#90977) ;
#85261=STYLED_ITEM('',(#170169),#90978) ;
#85262=STYLED_ITEM('',(#170169),#90979) ;
#85263=STYLED_ITEM('',(#170169),#90980) ;
#85264=STYLED_ITEM('',(#170169),#90981) ;
#85265=STYLED_ITEM('',(#170169),#90982) ;
#85266=STYLED_ITEM('',(#170169),#90983) ;
#85267=STYLED_ITEM('',(#170169),#90984) ;
#85268=STYLED_ITEM('',(#170169),#90985) ;
#85269=STYLED_ITEM('',(#170169),#90986) ;
#85270=STYLED_ITEM('',(#170169),#90987) ;
#85271=STYLED_ITEM('',(#170169),#90988) ;
#85272=STYLED_ITEM('',(#170169),#90989) ;
#85273=STYLED_ITEM('',(#170169),#90990) ;
#85274=STYLED_ITEM('',(#170169),#90991) ;
#85275=STYLED_ITEM('',(#170169),#90992) ;
#85276=STYLED_ITEM('',(#170169),#90993) ;
#85277=STYLED_ITEM('',(#170169),#90994) ;
#85278=STYLED_ITEM('',(#170169),#90995) ;
#85279=STYLED_ITEM('',(#170169),#90996) ;
#85280=STYLED_ITEM('',(#170169),#90997) ;
#85281=STYLED_ITEM('',(#170169),#90998) ;
#85282=STYLED_ITEM('',(#170169),#90999) ;
#85283=STYLED_ITEM('',(#170169),#91000) ;
#85284=STYLED_ITEM('',(#170169),#91001) ;
#85285=STYLED_ITEM('',(#170169),#91002) ;
#85286=STYLED_ITEM('',(#170169),#91003) ;
#85287=STYLED_ITEM('',(#170169),#91004) ;
#85288=STYLED_ITEM('',(#170169),#91005) ;
#85289=STYLED_ITEM('',(#170169),#91006) ;
#85290=STYLED_ITEM('',(#170169),#91007) ;
#85291=STYLED_ITEM('',(#170169),#91008) ;
#85292=STYLED_ITEM('',(#170169),#91009) ;
#85293=STYLED_ITEM('',(#170169),#91010) ;
#85294=STYLED_ITEM('',(#170169),#91011) ;
#85295=STYLED_ITEM('',(#170169),#91012) ;
#85296=STYLED_ITEM('',(#170169),#91013) ;
#85297=STYLED_ITEM('',(#170169),#91014) ;
#85298=STYLED_ITEM('',(#170169),#91015) ;
#85299=STYLED_ITEM('',(#170169),#91016) ;
#85300=STYLED_ITEM('',(#170169),#91017) ;
#85301=STYLED_ITEM('',(#170169),#91018) ;
#85302=STYLED_ITEM('',(#170169),#91019) ;
#85303=STYLED_ITEM('',(#170169),#91020) ;
#85304=STYLED_ITEM('',(#170169),#91021) ;
#85305=STYLED_ITEM('',(#170169),#91022) ;
#85306=STYLED_ITEM('',(#170169),#91023) ;
#85307=STYLED_ITEM('',(#170169),#91024) ;
#85308=STYLED_ITEM('',(#170169),#91025) ;
#85309=STYLED_ITEM('',(#170169),#91026) ;
#85310=STYLED_ITEM('',(#170169),#91027) ;
#85311=STYLED_ITEM('',(#170169),#91028) ;
#85312=STYLED_ITEM('',(#170169),#91029) ;
#85313=STYLED_ITEM('',(#170169),#91030) ;
#85314=STYLED_ITEM('',(#170169),#91031) ;
#85315=STYLED_ITEM('',(#170169),#91032) ;
#85316=STYLED_ITEM('',(#170169),#91033) ;
#85317=STYLED_ITEM('',(#170169),#91034) ;
#85318=STYLED_ITEM('',(#170169),#91035) ;
#85319=STYLED_ITEM('',(#170169),#91036) ;
#85320=STYLED_ITEM('',(#170169),#91037) ;
#85321=STYLED_ITEM('',(#170169),#91038) ;
#85322=STYLED_ITEM('',(#170169),#91039) ;
#85323=STYLED_ITEM('',(#170169),#91040) ;
#85324=STYLED_ITEM('',(#170169),#91041) ;
#85325=STYLED_ITEM('',(#170169),#91042) ;
#85326=STYLED_ITEM('',(#170169),#91043) ;
#85327=STYLED_ITEM('',(#170169),#91044) ;
#85328=STYLED_ITEM('',(#170169),#91045) ;
#85329=STYLED_ITEM('',(#170169),#91046) ;
#85330=STYLED_ITEM('',(#170169),#91047) ;
#85331=STYLED_ITEM('',(#170169),#91048) ;
#85332=STYLED_ITEM('',(#170169),#91049) ;
#85333=STYLED_ITEM('',(#170169),#91050) ;
#85334=STYLED_ITEM('',(#170169),#91051) ;
#85335=STYLED_ITEM('',(#170169),#91052) ;
#85336=STYLED_ITEM('',(#170169),#91053) ;
#85337=STYLED_ITEM('',(#170169),#91054) ;
#85338=STYLED_ITEM('',(#170169),#91055) ;
#85339=STYLED_ITEM('',(#170169),#91056) ;
#85340=STYLED_ITEM('',(#170169),#91057) ;
#85341=STYLED_ITEM('',(#170169),#91058) ;
#85342=STYLED_ITEM('',(#170169),#91059) ;
#85343=STYLED_ITEM('',(#170169),#91060) ;
#85344=STYLED_ITEM('',(#170169),#91061) ;
#85345=STYLED_ITEM('',(#170169),#91062) ;
#85346=STYLED_ITEM('',(#170169),#91063) ;
#85347=STYLED_ITEM('',(#170169),#91064) ;
#85348=STYLED_ITEM('',(#170169),#91065) ;
#85349=STYLED_ITEM('',(#170169),#91066) ;
#85350=STYLED_ITEM('',(#170169),#91067) ;
#85351=STYLED_ITEM('',(#170169),#91068) ;
#85352=STYLED_ITEM('',(#170169),#91069) ;
#85353=STYLED_ITEM('',(#170169),#91070) ;
#85354=STYLED_ITEM('',(#170169),#91071) ;
#85355=STYLED_ITEM('',(#170169),#91072) ;
#85356=STYLED_ITEM('',(#170169),#91073) ;
#85357=STYLED_ITEM('',(#170169),#91074) ;
#85358=STYLED_ITEM('',(#170169),#91075) ;
#85359=STYLED_ITEM('',(#170169),#91076) ;
#85360=STYLED_ITEM('',(#170169),#91077) ;
#85361=STYLED_ITEM('',(#170169),#91078) ;
#85362=STYLED_ITEM('',(#170169),#91079) ;
#85363=STYLED_ITEM('',(#170169),#91080) ;
#85364=STYLED_ITEM('',(#170169),#91081) ;
#85365=STYLED_ITEM('',(#170169),#91082) ;
#85366=STYLED_ITEM('',(#170168),#33) ;
#88718=ADVANCED_FACE('',(#20398),#15100,.F.) ;
#88719=ADVANCED_FACE('',(#20399),#79344,.T.) ;
#88720=ADVANCED_FACE('',(#20400),#79345,.T.) ;
#88721=ADVANCED_FACE('',(#20401),#79346,.F.) ;
#88722=ADVANCED_FACE('',(#20402),#79347,.T.) ;
#88723=ADVANCED_FACE('',(#20403),#79348,.F.) ;
#88724=ADVANCED_FACE('',(#20404),#79349,.T.) ;
#88725=ADVANCED_FACE('',(#20405),#79350,.F.) ;
#88726=ADVANCED_FACE('',(#20406),#79351,.T.) ;
#88727=ADVANCED_FACE('',(#20407),#79352,.F.) ;
#88728=ADVANCED_FACE('',(#20408),#79353,.T.) ;
#88729=ADVANCED_FACE('',(#20409),#79354,.F.) ;
#88730=ADVANCED_FACE('',(#20410),#79355,.T.) ;
#88731=ADVANCED_FACE('',(#20411),#79356,.F.) ;
#88732=ADVANCED_FACE('',(#20412),#79357,.T.) ;
#88733=ADVANCED_FACE('',(#20413),#79358,.F.) ;
#88734=ADVANCED_FACE('',(#20414),#79359,.T.) ;
#88735=ADVANCED_FACE('',(#20415),#79360,.F.) ;
#88736=ADVANCED_FACE('',(#20416),#79361,.T.) ;
#88737=ADVANCED_FACE('',(#20417),#79362,.F.) ;
#88738=ADVANCED_FACE('',(#20418),#79363,.T.) ;
#88739=ADVANCED_FACE('',(#20419),#79364,.F.) ;
#88740=ADVANCED_FACE('',(#20420),#15101,.F.) ;
#88741=ADVANCED_FACE('',(#20421),#15102,.F.) ;
#88742=ADVANCED_FACE('',(#20422),#15103,.F.) ;
#88743=ADVANCED_FACE('',(#20423),#15104,.F.) ;
#88744=ADVANCED_FACE('',(#20424),#15105,.F.) ;
#88745=ADVANCED_FACE('',(#20425),#15106,.F.) ;
#88746=ADVANCED_FACE('',(#20426),#15107,.F.) ;
#88747=ADVANCED_FACE('',(#20427),#79365,.F.) ;
#88748=ADVANCED_FACE('',(#20428),#79366,.T.) ;
#88749=ADVANCED_FACE('',(#20429),#79367,.T.) ;
#88750=ADVANCED_FACE('',(#20430),#79368,.F.) ;
#88751=ADVANCED_FACE('',(#20431),#79369,.T.) ;
#88752=ADVANCED_FACE('',(#20432),#79370,.T.) ;
#88753=ADVANCED_FACE('',(#20433),#79371,.F.) ;
#88754=ADVANCED_FACE('',(#20434),#79372,.T.) ;
#88755=ADVANCED_FACE('',(#20435),#79373,.T.) ;
#88756=ADVANCED_FACE('',(#20436),#79374,.F.) ;
#88757=ADVANCED_FACE('',(#20437),#79375,.T.) ;
#88758=ADVANCED_FACE('',(#20438),#79376,.T.) ;
#88759=ADVANCED_FACE('',(#20439),#79377,.F.) ;
#88760=ADVANCED_FACE('',(#20440),#79378,.T.) ;
#88761=ADVANCED_FACE('',(#20441),#79379,.T.) ;
#88762=ADVANCED_FACE('',(#20442),#79380,.F.) ;
#88763=ADVANCED_FACE('',(#20443),#79381,.T.) ;
#88764=ADVANCED_FACE('',(#20444),#79382,.T.) ;
#88765=ADVANCED_FACE('',(#20445),#79383,.F.) ;
#88766=ADVANCED_FACE('',(#20446),#79384,.T.) ;
#88767=ADVANCED_FACE('',(#20447),#79385,.T.) ;
#88768=ADVANCED_FACE('',(#20448),#79386,.F.) ;
#88769=ADVANCED_FACE('',(#20449),#79387,.T.) ;
#88770=ADVANCED_FACE('',(#20450),#79388,.T.) ;
#88771=ADVANCED_FACE('',(#20451),#79389,.F.) ;
#88772=ADVANCED_FACE('',(#20452),#79390,.T.) ;
#88773=ADVANCED_FACE('',(#20453),#79391,.T.) ;
#88774=ADVANCED_FACE('',(#20454),#15108,.F.) ;
#88775=ADVANCED_FACE('',(#20455),#15109,.F.) ;
#88776=ADVANCED_FACE('',(#20456),#15110,.F.) ;
#88777=ADVANCED_FACE('',(#20457),#15111,.F.) ;
#88778=ADVANCED_FACE('',(#20458),#15112,.F.) ;
#88779=ADVANCED_FACE('',(#20459),#15113,.F.) ;
#88780=ADVANCED_FACE('',(#20460),#15114,.F.) ;
#88781=ADVANCED_FACE('',(#20461),#15115,.F.) ;
#88782=ADVANCED_FACE('',(#20462),#15116,.F.) ;
#88783=ADVANCED_FACE('',(#20463),#2420,.F.) ;
#88784=ADVANCED_FACE('',(#20464),#2421,.F.) ;
#88785=ADVANCED_FACE('',(#20465),#2422,.F.) ;
#88786=ADVANCED_FACE('',(#20466),#2423,.F.) ;
#88787=ADVANCED_FACE('',(#20467),#2424,.F.) ;
#88788=ADVANCED_FACE('',(#20468),#2425,.F.) ;
#88789=ADVANCED_FACE('',(#20469),#2426,.F.) ;
#88790=ADVANCED_FACE('',(#20470),#2427,.F.) ;
#88791=ADVANCED_FACE('',(#20471),#2428,.F.) ;
#88792=ADVANCED_FACE('',(#20472),#15117,.F.) ;
#88793=ADVANCED_FACE('',(#20473),#15118,.F.) ;
#88794=ADVANCED_FACE('',(#20474),#15119,.F.) ;
#88795=ADVANCED_FACE('',(#20475),#15120,.F.) ;
#88796=ADVANCED_FACE('',(#20476),#15121,.F.) ;
#88797=ADVANCED_FACE('',(#20477),#15122,.F.) ;
#88798=ADVANCED_FACE('',(#20478),#15123,.F.) ;
#88799=ADVANCED_FACE('',(#20479),#15124,.F.) ;
#88800=ADVANCED_FACE('',(#20480),#15125,.F.) ;
#88801=ADVANCED_FACE('',(#20481),#79392,.F.) ;
#88802=ADVANCED_FACE('',(#20482),#79393,.T.) ;
#88803=ADVANCED_FACE('',(#20483),#79394,.T.) ;
#88804=ADVANCED_FACE('',(#20484),#15126,.F.) ;
#88805=ADVANCED_FACE('',(#20485),#15127,.F.) ;
#88806=ADVANCED_FACE('',(#20486),#15128,.F.) ;
#88807=ADVANCED_FACE('',(#20487),#15129,.F.) ;
#88808=ADVANCED_FACE('',(#20488),#15130,.F.) ;
#88809=ADVANCED_FACE('',(#20489),#2429,.F.) ;
#88810=ADVANCED_FACE('',(#20490),#15131,.F.) ;
#88811=ADVANCED_FACE('',(#20491,#714,#715,#716,#717,#718,#719,#720,#721,
#722,#723,#724,#725,#726,#727,#728,#729,#730,#731,#732,#733),#1513,.T.) ;
#88812=ADVANCED_FACE('',(#20492,#734),#1514,.F.) ;
#88813=ADVANCED_FACE('',(#20493,#735),#1515,.F.) ;
#88814=ADVANCED_FACE('',(#20494,#736),#1516,.F.) ;
#88815=ADVANCED_FACE('',(#20495,#737),#1517,.F.) ;
#88816=ADVANCED_FACE('',(#20496,#738),#1518,.F.) ;
#88817=ADVANCED_FACE('',(#20497,#739),#1519,.F.) ;
#88818=ADVANCED_FACE('',(#20498,#740),#1520,.F.) ;
#88819=ADVANCED_FACE('',(#20499,#741),#1521,.F.) ;
#88820=ADVANCED_FACE('',(#20500,#742),#1522,.F.) ;
#88821=ADVANCED_FACE('',(#20501),#1523,.T.) ;
#88822=ADVANCED_FACE('',(#20502),#1524,.T.) ;
#88823=ADVANCED_FACE('',(#20503),#1525,.T.) ;
#88824=ADVANCED_FACE('',(#20504),#1526,.T.) ;
#88825=ADVANCED_FACE('',(#20505),#1527,.T.) ;
#88826=ADVANCED_FACE('',(#20506),#1528,.T.) ;
#88827=ADVANCED_FACE('',(#20507),#1529,.T.) ;
#88828=ADVANCED_FACE('',(#20508),#1530,.T.) ;
#88829=ADVANCED_FACE('',(#20509),#1531,.T.) ;
#88830=ADVANCED_FACE('',(#20510),#1532,.T.) ;
#88831=ADVANCED_FACE('',(#20511),#1533,.T.) ;
#88832=ADVANCED_FACE('',(#20512),#1534,.T.) ;
#88833=ADVANCED_FACE('',(#20513),#1535,.T.) ;
#88834=ADVANCED_FACE('',(#20514),#1536,.T.) ;
#88835=ADVANCED_FACE('',(#20515),#1537,.T.) ;
#88836=ADVANCED_FACE('',(#20516),#1538,.T.) ;
#88837=ADVANCED_FACE('',(#20517),#1539,.T.) ;
#88838=ADVANCED_FACE('',(#20518),#1540,.T.) ;
#88839=ADVANCED_FACE('',(#20519),#1541,.T.) ;
#88840=ADVANCED_FACE('',(#20520),#1542,.T.) ;
#88841=ADVANCED_FACE('',(#20521),#1543,.T.) ;
#88842=ADVANCED_FACE('',(#20522),#15132,.T.) ;
#88843=ADVANCED_FACE('',(#20523),#15133,.T.) ;
#88844=ADVANCED_FACE('',(#20524,#743,#744,#745,#746,#747,#748,#749,#750,
#751,#752),#1544,.T.) ;
#88845=ADVANCED_FACE('',(#20525,#753),#1545,.F.) ;
#88846=ADVANCED_FACE('',(#20526),#1546,.T.) ;
#88847=ADVANCED_FACE('',(#20527),#1547,.T.) ;
#88848=ADVANCED_FACE('',(#20528),#1548,.T.) ;
#88849=ADVANCED_FACE('',(#20529),#1549,.T.) ;
#88850=ADVANCED_FACE('',(#20530),#1550,.T.) ;
#88851=ADVANCED_FACE('',(#20531),#1551,.T.) ;
#88852=ADVANCED_FACE('',(#20532,#754,#755,#756,#757,#758,#759,#760,#761,
#762,#763),#1552,.T.) ;
#88853=ADVANCED_FACE('',(#20533),#1553,.T.) ;
#88854=ADVANCED_FACE('',(#20534),#1554,.F.) ;
#88855=ADVANCED_FACE('',(#20535),#1555,.F.) ;
#88856=ADVANCED_FACE('',(#20536),#1556,.F.) ;
#88857=ADVANCED_FACE('',(#20537),#1557,.F.) ;
#88858=ADVANCED_FACE('',(#20538),#1558,.F.) ;
#88859=ADVANCED_FACE('',(#20539),#1559,.F.) ;
#88860=ADVANCED_FACE('',(#20540),#1560,.F.) ;
#88861=ADVANCED_FACE('',(#20541),#1561,.T.) ;
#88862=ADVANCED_FACE('',(#20542),#1562,.F.) ;
#88863=ADVANCED_FACE('',(#20543),#1563,.F.) ;
#88864=ADVANCED_FACE('',(#20544),#1564,.F.) ;
#88865=ADVANCED_FACE('',(#20545),#1565,.F.) ;
#88866=ADVANCED_FACE('',(#20546,#764),#1566,.T.) ;
#88867=ADVANCED_FACE('',(#20547),#1567,.T.) ;
#88868=ADVANCED_FACE('',(#20548),#1568,.T.) ;
#88869=ADVANCED_FACE('',(#20549),#1569,.T.) ;
#88870=ADVANCED_FACE('',(#20550),#1570,.T.) ;
#88871=ADVANCED_FACE('',(#20551),#1571,.T.) ;
#88872=ADVANCED_FACE('',(#20552),#1572,.F.) ;
#88873=ADVANCED_FACE('',(#20553),#1573,.F.) ;
#88874=ADVANCED_FACE('',(#20554),#1574,.F.) ;
#88875=ADVANCED_FACE('',(#20555),#1575,.F.) ;
#88876=ADVANCED_FACE('',(#20556),#1576,.F.) ;
#88877=ADVANCED_FACE('',(#20557),#1577,.F.) ;
#88878=ADVANCED_FACE('',(#20558),#1578,.F.) ;
#88879=ADVANCED_FACE('',(#20559),#1579,.F.) ;
#88880=ADVANCED_FACE('',(#20560),#15134,.F.) ;
#88881=ADVANCED_FACE('',(#20561,#765),#1580,.T.) ;
#88882=ADVANCED_FACE('',(#20562),#1581,.T.) ;
#88883=ADVANCED_FACE('',(#20563),#1582,.F.) ;
#88884=ADVANCED_FACE('',(#20564),#1583,.F.) ;
#88885=ADVANCED_FACE('',(#20565),#1584,.F.) ;
#88886=ADVANCED_FACE('',(#20566),#1585,.F.) ;
#88887=ADVANCED_FACE('',(#20567,#766),#1586,.T.) ;
#88888=ADVANCED_FACE('',(#20568),#1587,.T.) ;
#88889=ADVANCED_FACE('',(#20569),#1588,.T.) ;
#88890=ADVANCED_FACE('',(#20570),#1589,.T.) ;
#88891=ADVANCED_FACE('',(#20571),#1590,.T.) ;
#88892=ADVANCED_FACE('',(#20572),#1591,.T.) ;
#88893=ADVANCED_FACE('',(#20573),#1592,.T.) ;
#88894=ADVANCED_FACE('',(#20574),#1593,.F.) ;
#88895=ADVANCED_FACE('',(#20575),#1594,.F.) ;
#88896=ADVANCED_FACE('',(#20576),#1595,.T.) ;
#88897=ADVANCED_FACE('',(#20577),#15135,.T.) ;
#88898=ADVANCED_FACE('',(#20578),#15136,.T.) ;
#88899=ADVANCED_FACE('',(#20579),#1596,.F.) ;
#88900=ADVANCED_FACE('',(#20580),#1597,.F.) ;
#88901=ADVANCED_FACE('',(#20581),#15137,.T.) ;
#88902=ADVANCED_FACE('',(#20582),#15138,.T.) ;
#88903=ADVANCED_FACE('',(#20583),#15139,.T.) ;
#88904=ADVANCED_FACE('',(#20584),#1598,.F.) ;
#88905=ADVANCED_FACE('',(#20585),#15140,.T.) ;
#88906=ADVANCED_FACE('',(#20586),#1599,.F.) ;
#88907=ADVANCED_FACE('',(#20587),#15141,.T.) ;
#88908=ADVANCED_FACE('',(#20588),#1600,.F.) ;
#88909=ADVANCED_FACE('',(#20589),#15142,.T.) ;
#88910=ADVANCED_FACE('',(#20590),#1601,.F.) ;
#88911=ADVANCED_FACE('',(#20591),#1602,.F.) ;
#88912=ADVANCED_FACE('',(#20592),#15143,.T.) ;
#88913=ADVANCED_FACE('',(#20593),#16689,.T.) ;
#88914=ADVANCED_FACE('',(#20594),#15144,.T.) ;
#88915=ADVANCED_FACE('',(#20595),#15145,.T.) ;
#88916=ADVANCED_FACE('',(#20596),#15146,.T.) ;
#88917=ADVANCED_FACE('',(#20597),#15147,.T.) ;
#88918=ADVANCED_FACE('',(#20598),#15148,.T.) ;
#88919=ADVANCED_FACE('',(#20599),#15149,.T.) ;
#88920=ADVANCED_FACE('',(#20600),#16690,.T.) ;
#88921=ADVANCED_FACE('',(#20601),#16691,.T.) ;
#88922=ADVANCED_FACE('',(#20602),#15150,.T.) ;
#88923=ADVANCED_FACE('',(#20603),#16692,.T.) ;
#88924=ADVANCED_FACE('',(#20604),#15151,.T.) ;
#88925=ADVANCED_FACE('',(#20605),#15152,.T.) ;
#88926=ADVANCED_FACE('',(#20606),#15153,.T.) ;
#88927=ADVANCED_FACE('',(#20607),#15154,.T.) ;
#88928=ADVANCED_FACE('',(#20608),#15155,.T.) ;
#88929=ADVANCED_FACE('',(#20609),#15156,.T.) ;
#88930=ADVANCED_FACE('',(#20610),#79395,.T.) ;
#88931=ADVANCED_FACE('',(#20611),#16693,.T.) ;
#88932=ADVANCED_FACE('',(#20612),#16694,.T.) ;
#88933=ADVANCED_FACE('',(#20613),#15157,.F.) ;
#88934=ADVANCED_FACE('',(#20614),#15158,.T.) ;
#88935=ADVANCED_FACE('',(#20615),#15159,.T.) ;
#88936=ADVANCED_FACE('',(#20616),#79396,.T.) ;
#88937=ADVANCED_FACE('',(#20617),#15160,.T.) ;
#88938=ADVANCED_FACE('',(#20618),#16695,.T.) ;
#88939=ADVANCED_FACE('',(#20619),#79397,.T.) ;
#88940=ADVANCED_FACE('',(#20620),#15161,.T.) ;
#88941=ADVANCED_FACE('',(#20621),#15162,.T.) ;
#88942=ADVANCED_FACE('',(#20622),#15163,.T.) ;
#88943=ADVANCED_FACE('',(#20623),#15164,.T.) ;
#88944=ADVANCED_FACE('',(#20624),#16696,.T.) ;
#88945=ADVANCED_FACE('',(#20625),#79398,.F.) ;
#88946=ADVANCED_FACE('',(#20626),#16697,.T.) ;
#88947=ADVANCED_FACE('',(#20627),#15165,.T.) ;
#88948=ADVANCED_FACE('',(#20628),#15166,.T.) ;
#88949=ADVANCED_FACE('',(#20629),#15167,.T.) ;
#88950=ADVANCED_FACE('',(#20630),#79399,.F.) ;
#88951=ADVANCED_FACE('',(#20631),#15168,.F.) ;
#88952=ADVANCED_FACE('',(#20632),#15169,.T.) ;
#88953=ADVANCED_FACE('',(#20633),#16698,.T.) ;
#88954=ADVANCED_FACE('',(#20634),#79400,.F.) ;
#88955=ADVANCED_FACE('',(#20635),#79401,.T.) ;
#88956=ADVANCED_FACE('',(#20636),#15170,.T.) ;
#88957=ADVANCED_FACE('',(#20637),#15171,.F.) ;
#88958=ADVANCED_FACE('',(#20638),#15172,.T.) ;
#88959=ADVANCED_FACE('',(#20639),#15173,.F.) ;
#88960=ADVANCED_FACE('',(#20640),#15174,.F.) ;
#88961=ADVANCED_FACE('',(#20641),#79402,.T.) ;
#88962=ADVANCED_FACE('',(#20642),#16699,.T.) ;
#88963=ADVANCED_FACE('',(#20643),#16700,.F.) ;
#88964=ADVANCED_FACE('',(#20644),#15175,.T.) ;
#88965=ADVANCED_FACE('',(#20645),#15176,.T.) ;
#88966=ADVANCED_FACE('',(#20646),#15177,.T.) ;
#88967=ADVANCED_FACE('',(#20647),#15178,.F.) ;
#88968=ADVANCED_FACE('',(#20648),#16701,.T.) ;
#88969=ADVANCED_FACE('',(#20649),#79403,.F.) ;
#88970=ADVANCED_FACE('',(#20650),#15179,.F.) ;
#88971=ADVANCED_FACE('',(#20651),#15180,.F.) ;
#88972=ADVANCED_FACE('',(#20652),#15181,.T.) ;
#88973=ADVANCED_FACE('',(#20653),#15182,.F.) ;
#88974=ADVANCED_FACE('',(#20654),#16702,.F.) ;
#88975=ADVANCED_FACE('',(#20655),#79404,.F.) ;
#88976=ADVANCED_FACE('',(#20656),#15183,.F.) ;
#88977=ADVANCED_FACE('',(#20657),#79405,.F.) ;
#88978=ADVANCED_FACE('',(#20658),#15184,.F.) ;
#88979=ADVANCED_FACE('',(#20659),#15185,.F.) ;
#88980=ADVANCED_FACE('',(#20660),#79406,.F.) ;
#88981=ADVANCED_FACE('',(#20661),#79407,.F.) ;
#88982=ADVANCED_FACE('',(#20662),#15186,.F.) ;
#88983=ADVANCED_FACE('',(#20663),#15187,.F.) ;
#88984=ADVANCED_FACE('',(#20664),#79408,.F.) ;
#88985=ADVANCED_FACE('',(#20665),#15188,.T.) ;
#88986=ADVANCED_FACE('',(#20666),#79409,.T.) ;
#88987=ADVANCED_FACE('',(#20667),#79410,.T.) ;
#88988=ADVANCED_FACE('',(#20668),#15189,.T.) ;
#88989=ADVANCED_FACE('',(#20669),#15190,.F.) ;
#88990=ADVANCED_FACE('',(#20670),#15191,.F.) ;
#88991=ADVANCED_FACE('',(#20671),#15192,.F.) ;
#88992=ADVANCED_FACE('',(#20672),#15193,.T.) ;
#88993=ADVANCED_FACE('',(#20673),#15194,.T.) ;
#88994=ADVANCED_FACE('',(#20674),#79411,.T.) ;
#88995=ADVANCED_FACE('',(#20675),#16703,.F.) ;
#88996=ADVANCED_FACE('',(#20676),#16704,.F.) ;
#88997=ADVANCED_FACE('',(#20677),#79412,.T.) ;
#88998=ADVANCED_FACE('',(#20678),#15195,.F.) ;
#88999=ADVANCED_FACE('',(#20679),#15196,.F.) ;
#89000=ADVANCED_FACE('',(#20680),#15197,.F.) ;
#89001=ADVANCED_FACE('',(#20681),#15198,.F.) ;
#89002=ADVANCED_FACE('',(#20682),#16705,.F.) ;
#89003=ADVANCED_FACE('',(#20683),#16706,.F.) ;
#89004=ADVANCED_FACE('',(#20684),#15199,.F.) ;
#89005=ADVANCED_FACE('',(#20685),#15200,.T.) ;
#89006=ADVANCED_FACE('',(#20686),#15201,.T.) ;
#89007=ADVANCED_FACE('',(#20687),#15202,.T.) ;
#89008=ADVANCED_FACE('',(#20688),#16707,.T.) ;
#89009=ADVANCED_FACE('',(#20689),#16708,.T.) ;
#89010=ADVANCED_FACE('',(#20690),#15203,.T.) ;
#89011=ADVANCED_FACE('',(#20691),#15204,.T.) ;
#89012=ADVANCED_FACE('',(#20692),#15205,.T.) ;
#89013=ADVANCED_FACE('',(#20693),#15206,.T.) ;
#89014=ADVANCED_FACE('',(#20694),#16709,.T.) ;
#89015=ADVANCED_FACE('',(#20695),#16710,.T.) ;
#89016=ADVANCED_FACE('',(#20696),#15207,.T.) ;
#89017=ADVANCED_FACE('',(#20697),#15208,.F.) ;
#89018=ADVANCED_FACE('',(#20698),#16711,.F.) ;
#89019=ADVANCED_FACE('',(#20699),#15209,.F.) ;
#89020=ADVANCED_FACE('',(#20700),#15210,.F.) ;
#89021=ADVANCED_FACE('',(#20701),#15211,.F.) ;
#89022=ADVANCED_FACE('',(#20702),#128,.T.) ;
#89023=ADVANCED_FACE('',(#20703),#16712,.F.) ;
#89024=ADVANCED_FACE('',(#20704),#15212,.F.) ;
#89025=ADVANCED_FACE('',(#20705),#15213,.F.) ;
#89026=ADVANCED_FACE('',(#20706),#15214,.T.) ;
#89027=ADVANCED_FACE('',(#20707),#15215,.T.) ;
#89028=ADVANCED_FACE('',(#20708),#15216,.F.) ;
#89029=ADVANCED_FACE('',(#20709),#16713,.F.) ;
#89030=ADVANCED_FACE('',(#20710),#129,.T.) ;
#89031=ADVANCED_FACE('',(#20711),#130,.T.) ;
#89032=ADVANCED_FACE('',(#20712),#15217,.F.) ;
#89033=ADVANCED_FACE('',(#20713),#15218,.F.) ;
#89034=ADVANCED_FACE('',(#20714),#15219,.T.) ;
#89035=ADVANCED_FACE('',(#20715),#15220,.T.) ;
#89036=ADVANCED_FACE('',(#20716),#16714,.F.) ;
#89037=ADVANCED_FACE('',(#20717),#131,.T.) ;
#89038=ADVANCED_FACE('',(#20718),#15221,.F.) ;
#89039=ADVANCED_FACE('',(#20719),#15222,.T.) ;
#89040=ADVANCED_FACE('',(#20720),#79413,.T.) ;
#89041=ADVANCED_FACE('',(#20721),#79414,.T.) ;
#89042=ADVANCED_FACE('',(#20722),#15223,.T.) ;
#89043=ADVANCED_FACE('',(#20723),#15224,.F.) ;
#89044=ADVANCED_FACE('',(#20724),#15225,.F.) ;
#89045=ADVANCED_FACE('',(#20725),#15226,.F.) ;
#89046=ADVANCED_FACE('',(#20726),#15227,.T.) ;
#89047=ADVANCED_FACE('',(#20727),#15228,.T.) ;
#89048=ADVANCED_FACE('',(#20728),#79415,.T.) ;
#89049=ADVANCED_FACE('',(#20729),#16715,.F.) ;
#89050=ADVANCED_FACE('',(#20730),#16716,.F.) ;
#89051=ADVANCED_FACE('',(#20731),#79416,.T.) ;
#89052=ADVANCED_FACE('',(#20732),#15229,.F.) ;
#89053=ADVANCED_FACE('',(#20733),#15230,.F.) ;
#89054=ADVANCED_FACE('',(#20734),#15231,.F.) ;
#89055=ADVANCED_FACE('',(#20735),#15232,.F.) ;
#89056=ADVANCED_FACE('',(#20736),#16717,.F.) ;
#89057=ADVANCED_FACE('',(#20737),#16718,.F.) ;
#89058=ADVANCED_FACE('',(#20738),#15233,.F.) ;
#89059=ADVANCED_FACE('',(#20739),#15234,.T.) ;
#89060=ADVANCED_FACE('',(#20740),#15235,.T.) ;
#89061=ADVANCED_FACE('',(#20741),#15236,.T.) ;
#89062=ADVANCED_FACE('',(#20742),#16719,.T.) ;
#89063=ADVANCED_FACE('',(#20743),#16720,.T.) ;
#89064=ADVANCED_FACE('',(#20744),#15237,.T.) ;
#89065=ADVANCED_FACE('',(#20745),#15238,.T.) ;
#89066=ADVANCED_FACE('',(#20746),#15239,.T.) ;
#89067=ADVANCED_FACE('',(#20747),#15240,.T.) ;
#89068=ADVANCED_FACE('',(#20748),#16721,.T.) ;
#89069=ADVANCED_FACE('',(#20749),#16722,.T.) ;
#89070=ADVANCED_FACE('',(#20750),#15241,.T.) ;
#89071=ADVANCED_FACE('',(#20751),#15242,.T.) ;
#89072=ADVANCED_FACE('',(#20752),#16723,.T.) ;
#89073=ADVANCED_FACE('',(#20753),#16724,.T.) ;
#89074=ADVANCED_FACE('',(#20754),#15243,.T.) ;
#89075=ADVANCED_FACE('',(#20755),#15244,.T.) ;
#89076=ADVANCED_FACE('',(#20756),#16725,.T.) ;
#89077=ADVANCED_FACE('',(#20757),#16726,.T.) ;
#89078=ADVANCED_FACE('',(#20758),#15245,.T.) ;
#89079=ADVANCED_FACE('',(#20759),#15246,.T.) ;
#89080=ADVANCED_FACE('',(#20760),#15247,.F.) ;
#89081=ADVANCED_FACE('',(#20761),#15248,.F.) ;
#89082=ADVANCED_FACE('',(#20762),#15249,.T.) ;
#89083=ADVANCED_FACE('',(#20763),#15250,.F.) ;
#89084=ADVANCED_FACE('',(#20764),#79417,.T.) ;
#89085=ADVANCED_FACE('',(#20765),#15251,.T.) ;
#89086=ADVANCED_FACE('',(#20766),#79418,.T.) ;
#89087=ADVANCED_FACE('',(#20767),#79419,.T.) ;
#89088=ADVANCED_FACE('',(#20768),#15252,.T.) ;
#89089=ADVANCED_FACE('',(#20769),#16727,.T.) ;
#89090=ADVANCED_FACE('',(#20770),#79420,.T.) ;
#89091=ADVANCED_FACE('',(#20771),#15253,.T.) ;
#89092=ADVANCED_FACE('',(#20772),#16728,.T.) ;
#89093=ADVANCED_FACE('',(#20773),#79421,.F.) ;
#89094=ADVANCED_FACE('',(#20774),#132,.F.) ;
#89095=ADVANCED_FACE('',(#20775),#79422,.F.) ;
#89096=ADVANCED_FACE('',(#20776),#79423,.F.) ;
#89097=ADVANCED_FACE('',(#20777),#133,.F.) ;
#89098=ADVANCED_FACE('',(#20778),#79424,.F.) ;
#89099=ADVANCED_FACE('',(#20779),#1603,.F.) ;
#89100=ADVANCED_FACE('',(#20780),#1604,.F.) ;
#89101=ADVANCED_FACE('',(#20781),#1605,.F.) ;
#89102=ADVANCED_FACE('',(#20782),#1606,.F.) ;
#89103=ADVANCED_FACE('',(#20783),#1607,.F.) ;
#89104=ADVANCED_FACE('',(#20784),#1608,.F.) ;
#89105=ADVANCED_FACE('',(#20785),#1609,.F.) ;
#89106=ADVANCED_FACE('',(#20786),#1610,.F.) ;
#89107=ADVANCED_FACE('',(#20787),#1611,.F.) ;
#89108=ADVANCED_FACE('',(#20788),#1612,.F.) ;
#89109=ADVANCED_FACE('',(#20789),#1613,.F.) ;
#89110=ADVANCED_FACE('',(#20790),#1614,.F.) ;
#89111=ADVANCED_FACE('',(#20791),#1615,.F.) ;
#89112=ADVANCED_FACE('',(#20792),#1616,.F.) ;
#89113=ADVANCED_FACE('',(#20793),#1617,.F.) ;
#89114=ADVANCED_FACE('',(#20794),#1618,.F.) ;
#89115=ADVANCED_FACE('',(#20795),#1619,.F.) ;
#89116=ADVANCED_FACE('',(#20796),#1620,.F.) ;
#89117=ADVANCED_FACE('',(#20797),#1621,.F.) ;
#89118=ADVANCED_FACE('',(#20798),#1622,.F.) ;
#89119=ADVANCED_FACE('',(#20799),#1623,.F.) ;
#89120=ADVANCED_FACE('',(#20800),#1624,.F.) ;
#89121=ADVANCED_FACE('',(#20801),#1625,.F.) ;
#89122=ADVANCED_FACE('',(#20802),#1626,.F.) ;
#89123=ADVANCED_FACE('',(#20803),#1627,.F.) ;
#89124=ADVANCED_FACE('',(#20804),#1628,.F.) ;
#89125=ADVANCED_FACE('',(#20805),#1629,.F.) ;
#89126=ADVANCED_FACE('',(#20806),#1630,.F.) ;
#89127=ADVANCED_FACE('',(#20807),#1631,.F.) ;
#89128=ADVANCED_FACE('',(#20808),#1632,.F.) ;
#89129=ADVANCED_FACE('',(#20809),#1633,.F.) ;
#89130=ADVANCED_FACE('',(#20810),#1634,.F.) ;
#89131=ADVANCED_FACE('',(#20811),#1635,.F.) ;
#89132=ADVANCED_FACE('',(#20812),#1636,.F.) ;
#89133=ADVANCED_FACE('',(#20813),#1637,.F.) ;
#89134=ADVANCED_FACE('',(#20814),#1638,.F.) ;
#89135=ADVANCED_FACE('',(#20815),#1639,.F.) ;
#89136=ADVANCED_FACE('',(#20816),#1640,.F.) ;
#89137=ADVANCED_FACE('',(#20817),#1641,.F.) ;
#89138=ADVANCED_FACE('',(#20818),#1642,.F.) ;
#89139=ADVANCED_FACE('',(#20819),#1643,.F.) ;
#89140=ADVANCED_FACE('',(#20820),#1644,.F.) ;
#89141=ADVANCED_FACE('',(#20821),#1645,.F.) ;
#89142=ADVANCED_FACE('',(#20822),#1646,.F.) ;
#89143=ADVANCED_FACE('',(#20823),#1647,.F.) ;
#89144=ADVANCED_FACE('',(#20824),#1648,.F.) ;
#89145=ADVANCED_FACE('',(#20825),#1649,.F.) ;
#89146=ADVANCED_FACE('',(#20826),#1650,.F.) ;
#89147=ADVANCED_FACE('',(#20827),#1651,.F.) ;
#89148=ADVANCED_FACE('',(#20828),#1652,.F.) ;
#89149=ADVANCED_FACE('',(#20829),#1653,.F.) ;
#89150=ADVANCED_FACE('',(#20830),#1654,.F.) ;
#89151=ADVANCED_FACE('',(#20831),#1655,.F.) ;
#89152=ADVANCED_FACE('',(#20832),#1656,.F.) ;
#89153=ADVANCED_FACE('',(#20833),#1657,.T.) ;
#89154=ADVANCED_FACE('',(#20834),#1658,.T.) ;
#89155=ADVANCED_FACE('',(#20835),#1659,.T.) ;
#89156=ADVANCED_FACE('',(#20836),#1660,.T.) ;
#89157=ADVANCED_FACE('',(#20837),#1661,.T.) ;
#89158=ADVANCED_FACE('',(#20838),#1662,.T.) ;
#89159=ADVANCED_FACE('',(#20839),#1663,.T.) ;
#89160=ADVANCED_FACE('',(#20840),#1664,.T.) ;
#89161=ADVANCED_FACE('',(#20841),#1665,.T.) ;
#89162=ADVANCED_FACE('',(#20842),#1666,.F.) ;
#89163=ADVANCED_FACE('',(#20843),#1667,.F.) ;
#89164=ADVANCED_FACE('',(#20844),#1668,.F.) ;
#89165=ADVANCED_FACE('',(#20845),#1669,.F.) ;
#89166=ADVANCED_FACE('',(#20846),#1670,.F.) ;
#89167=ADVANCED_FACE('',(#20847),#1671,.F.) ;
#89168=ADVANCED_FACE('',(#20848),#1672,.F.) ;
#89169=ADVANCED_FACE('',(#20849),#1673,.F.) ;
#89170=ADVANCED_FACE('',(#20850),#1674,.F.) ;
#89171=ADVANCED_FACE('',(#20851),#1675,.F.) ;
#89172=ADVANCED_FACE('',(#20852),#1676,.F.) ;
#89173=ADVANCED_FACE('',(#20853),#1677,.F.) ;
#89174=ADVANCED_FACE('',(#20854),#1678,.F.) ;
#89175=ADVANCED_FACE('',(#20855),#1679,.F.) ;
#89176=ADVANCED_FACE('',(#20856),#1680,.F.) ;
#89177=ADVANCED_FACE('',(#20857),#1681,.F.) ;
#89178=ADVANCED_FACE('',(#20858),#1682,.F.) ;
#89179=ADVANCED_FACE('',(#20859),#1683,.F.) ;
#89180=ADVANCED_FACE('',(#20860),#1684,.F.) ;
#89181=ADVANCED_FACE('',(#20861),#1685,.F.) ;
#89182=ADVANCED_FACE('',(#20862),#1686,.F.) ;
#89183=ADVANCED_FACE('',(#20863),#1687,.F.) ;
#89184=ADVANCED_FACE('',(#20864),#1688,.F.) ;
#89185=ADVANCED_FACE('',(#20865),#1689,.F.) ;
#89186=ADVANCED_FACE('',(#20866),#1690,.F.) ;
#89187=ADVANCED_FACE('',(#20867),#1691,.F.) ;
#89188=ADVANCED_FACE('',(#20868),#1692,.F.) ;
#89189=ADVANCED_FACE('',(#20869),#1693,.F.) ;
#89190=ADVANCED_FACE('',(#20870),#1694,.F.) ;
#89191=ADVANCED_FACE('',(#20871),#1695,.F.) ;
#89192=ADVANCED_FACE('',(#20872),#1696,.F.) ;
#89193=ADVANCED_FACE('',(#20873),#1697,.F.) ;
#89194=ADVANCED_FACE('',(#20874),#1698,.F.) ;
#89195=ADVANCED_FACE('',(#20875),#1699,.F.) ;
#89196=ADVANCED_FACE('',(#20876),#1700,.F.) ;
#89197=ADVANCED_FACE('',(#20877),#1701,.F.) ;
#89198=ADVANCED_FACE('',(#20878,#767),#1702,.T.) ;
#89199=ADVANCED_FACE('',(#20879),#1703,.T.) ;
#89200=ADVANCED_FACE('',(#20880),#1704,.T.) ;
#89201=ADVANCED_FACE('',(#20881),#1705,.T.) ;
#89202=ADVANCED_FACE('',(#20882),#1706,.T.) ;
#89203=ADVANCED_FACE('',(#20883,#768),#1707,.T.) ;
#89204=ADVANCED_FACE('',(#20884),#1708,.T.) ;
#89205=ADVANCED_FACE('',(#20885),#1709,.T.) ;
#89206=ADVANCED_FACE('',(#20886),#1710,.T.) ;
#89207=ADVANCED_FACE('',(#20887),#1711,.T.) ;
#89208=ADVANCED_FACE('',(#20888,#769),#1712,.T.) ;
#89209=ADVANCED_FACE('',(#20889),#1713,.T.) ;
#89210=ADVANCED_FACE('',(#20890),#1714,.T.) ;
#89211=ADVANCED_FACE('',(#20891),#1715,.T.) ;
#89212=ADVANCED_FACE('',(#20892),#1716,.T.) ;
#89213=ADVANCED_FACE('',(#20893,#770),#1717,.T.) ;
#89214=ADVANCED_FACE('',(#20894),#1718,.T.) ;
#89215=ADVANCED_FACE('',(#20895),#1719,.T.) ;
#89216=ADVANCED_FACE('',(#20896),#1720,.T.) ;
#89217=ADVANCED_FACE('',(#20897),#1721,.T.) ;
#89218=ADVANCED_FACE('',(#20898,#771),#1722,.T.) ;
#89219=ADVANCED_FACE('',(#20899),#1723,.T.) ;
#89220=ADVANCED_FACE('',(#20900),#1724,.T.) ;
#89221=ADVANCED_FACE('',(#20901),#1725,.T.) ;
#89222=ADVANCED_FACE('',(#20902),#1726,.T.) ;
#89223=ADVANCED_FACE('',(#20903,#772),#1727,.T.) ;
#89224=ADVANCED_FACE('',(#20904),#1728,.T.) ;
#89225=ADVANCED_FACE('',(#20905),#1729,.T.) ;
#89226=ADVANCED_FACE('',(#20906),#1730,.T.) ;
#89227=ADVANCED_FACE('',(#20907),#1731,.T.) ;
#89228=ADVANCED_FACE('',(#20908,#773),#1732,.T.) ;
#89229=ADVANCED_FACE('',(#20909),#1733,.T.) ;
#89230=ADVANCED_FACE('',(#20910),#1734,.T.) ;
#89231=ADVANCED_FACE('',(#20911),#1735,.T.) ;
#89232=ADVANCED_FACE('',(#20912),#1736,.T.) ;
#89233=ADVANCED_FACE('',(#20913,#774),#1737,.T.) ;
#89234=ADVANCED_FACE('',(#20914),#1738,.T.) ;
#89235=ADVANCED_FACE('',(#20915),#1739,.T.) ;
#89236=ADVANCED_FACE('',(#20916),#1740,.T.) ;
#89237=ADVANCED_FACE('',(#20917),#1741,.T.) ;
#89238=ADVANCED_FACE('',(#20918,#775),#1742,.T.) ;
#89239=ADVANCED_FACE('',(#20919),#1743,.T.) ;
#89240=ADVANCED_FACE('',(#20920),#1744,.T.) ;
#89241=ADVANCED_FACE('',(#20921),#1745,.T.) ;
#89242=ADVANCED_FACE('',(#20922),#1746,.T.) ;
#89243=ADVANCED_FACE('',(#20923),#1747,.T.) ;
#89244=ADVANCED_FACE('',(#20924),#1748,.T.) ;
#89245=ADVANCED_FACE('',(#20925),#1749,.T.) ;
#89246=ADVANCED_FACE('',(#20926),#1750,.T.) ;
#89247=ADVANCED_FACE('',(#20927),#1751,.T.) ;
#89248=ADVANCED_FACE('',(#20928),#1752,.T.) ;
#89249=ADVANCED_FACE('',(#20929),#1753,.T.) ;
#89250=ADVANCED_FACE('',(#20930),#1754,.T.) ;
#89251=ADVANCED_FACE('',(#20931),#1755,.T.) ;
#89252=ADVANCED_FACE('',(#20932),#1756,.F.) ;
#89253=ADVANCED_FACE('',(#20933),#1757,.F.) ;
#89254=ADVANCED_FACE('',(#20934),#1758,.F.) ;
#89255=ADVANCED_FACE('',(#20935),#1759,.F.) ;
#89256=ADVANCED_FACE('',(#20936),#1760,.F.) ;
#89257=ADVANCED_FACE('',(#20937),#1761,.F.) ;
#89258=ADVANCED_FACE('',(#20938),#1762,.F.) ;
#89259=ADVANCED_FACE('',(#20939),#1763,.F.) ;
#89260=ADVANCED_FACE('',(#20940),#1764,.F.) ;
#89261=ADVANCED_FACE('',(#20941),#1765,.F.) ;
#89262=ADVANCED_FACE('',(#20942),#1766,.F.) ;
#89263=ADVANCED_FACE('',(#20943),#1767,.F.) ;
#89264=ADVANCED_FACE('',(#20944),#1768,.F.) ;
#89265=ADVANCED_FACE('',(#20945),#1769,.F.) ;
#89266=ADVANCED_FACE('',(#20946),#1770,.F.) ;
#89267=ADVANCED_FACE('',(#20947),#1771,.F.) ;
#89268=ADVANCED_FACE('',(#20948),#1772,.F.) ;
#89269=ADVANCED_FACE('',(#20949),#1773,.F.) ;
#89270=ADVANCED_FACE('',(#20950),#1774,.F.) ;
#89271=ADVANCED_FACE('',(#20951),#1775,.F.) ;
#89272=ADVANCED_FACE('',(#20952),#1776,.F.) ;
#89273=ADVANCED_FACE('',(#20953),#1777,.F.) ;
#89274=ADVANCED_FACE('',(#20954),#1778,.F.) ;
#89275=ADVANCED_FACE('',(#20955),#1779,.F.) ;
#89276=ADVANCED_FACE('',(#20956),#1780,.F.) ;
#89277=ADVANCED_FACE('',(#20957),#1781,.F.) ;
#89278=ADVANCED_FACE('',(#20958),#1782,.F.) ;
#89279=ADVANCED_FACE('',(#20959),#1783,.F.) ;
#89280=ADVANCED_FACE('',(#20960),#1784,.F.) ;
#89281=ADVANCED_FACE('',(#20961),#1785,.F.) ;
#89282=ADVANCED_FACE('',(#20962),#1786,.F.) ;
#89283=ADVANCED_FACE('',(#20963),#1787,.F.) ;
#89284=ADVANCED_FACE('',(#20964),#1788,.F.) ;
#89285=ADVANCED_FACE('',(#20965),#1789,.F.) ;
#89286=ADVANCED_FACE('',(#20966),#1790,.F.) ;
#89287=ADVANCED_FACE('',(#20967),#1791,.F.) ;
#89288=ADVANCED_FACE('',(#20968),#1792,.F.) ;
#89289=ADVANCED_FACE('',(#20969),#1793,.F.) ;
#89290=ADVANCED_FACE('',(#20970),#15254,.F.) ;
#89291=ADVANCED_FACE('',(#20971,#776),#1794,.T.) ;
#89292=ADVANCED_FACE('',(#20972),#1795,.F.) ;
#89293=ADVANCED_FACE('',(#20973),#1796,.F.) ;
#89294=ADVANCED_FACE('',(#20974),#15255,.F.) ;
#89295=ADVANCED_FACE('',(#20975,#777),#1797,.T.) ;
#89296=ADVANCED_FACE('',(#20976),#1798,.F.) ;
#89297=ADVANCED_FACE('',(#20977),#1799,.F.) ;
#89298=ADVANCED_FACE('',(#20978),#15256,.F.) ;
#89299=ADVANCED_FACE('',(#20979,#778),#1800,.T.) ;
#89300=ADVANCED_FACE('',(#20980),#1801,.F.) ;
#89301=ADVANCED_FACE('',(#20981),#1802,.F.) ;
#89302=ADVANCED_FACE('',(#20982),#15257,.F.) ;
#89303=ADVANCED_FACE('',(#20983,#779),#1803,.T.) ;
#89304=ADVANCED_FACE('',(#20984),#1804,.F.) ;
#89305=ADVANCED_FACE('',(#20985),#1805,.F.) ;
#89306=ADVANCED_FACE('',(#20986),#15258,.F.) ;
#89307=ADVANCED_FACE('',(#20987,#780),#1806,.T.) ;
#89308=ADVANCED_FACE('',(#20988),#1807,.F.) ;
#89309=ADVANCED_FACE('',(#20989),#1808,.F.) ;
#89310=ADVANCED_FACE('',(#20990),#15259,.F.) ;
#89311=ADVANCED_FACE('',(#20991,#781),#1809,.T.) ;
#89312=ADVANCED_FACE('',(#20992),#1810,.F.) ;
#89313=ADVANCED_FACE('',(#20993),#1811,.F.) ;
#89314=ADVANCED_FACE('',(#20994),#15260,.F.) ;
#89315=ADVANCED_FACE('',(#20995,#782),#1812,.T.) ;
#89316=ADVANCED_FACE('',(#20996),#1813,.F.) ;
#89317=ADVANCED_FACE('',(#20997),#1814,.F.) ;
#89318=ADVANCED_FACE('',(#20998),#15261,.F.) ;
#89319=ADVANCED_FACE('',(#20999,#783),#1815,.T.) ;
#89320=ADVANCED_FACE('',(#21000),#1816,.F.) ;
#89321=ADVANCED_FACE('',(#21001),#1817,.F.) ;
#89322=ADVANCED_FACE('',(#21002),#15262,.F.) ;
#89323=ADVANCED_FACE('',(#21003,#784),#1818,.T.) ;
#89324=ADVANCED_FACE('',(#21004),#1819,.T.) ;
#89325=ADVANCED_FACE('',(#21005),#1820,.T.) ;
#89326=ADVANCED_FACE('',(#21006),#1821,.T.) ;
#89327=ADVANCED_FACE('',(#21007),#1822,.T.) ;
#89328=ADVANCED_FACE('',(#21008),#1823,.T.) ;
#89329=ADVANCED_FACE('',(#21009),#1824,.T.) ;
#89330=ADVANCED_FACE('',(#21010),#1825,.T.) ;
#89331=ADVANCED_FACE('',(#21011),#1826,.T.) ;
#89332=ADVANCED_FACE('',(#21012),#1827,.T.) ;
#89333=ADVANCED_FACE('',(#21013),#1828,.F.) ;
#89334=ADVANCED_FACE('',(#21014),#1829,.F.) ;
#89335=ADVANCED_FACE('',(#21015),#1830,.F.) ;
#89336=ADVANCED_FACE('',(#21016),#1831,.F.) ;
#89337=ADVANCED_FACE('',(#21017),#1832,.F.) ;
#89338=ADVANCED_FACE('',(#21018),#1833,.F.) ;
#89339=ADVANCED_FACE('',(#21019),#1834,.F.) ;
#89340=ADVANCED_FACE('',(#21020),#1835,.F.) ;
#89341=ADVANCED_FACE('',(#21021),#1836,.F.) ;
#89342=ADVANCED_FACE('',(#21022),#1837,.F.) ;
#89343=ADVANCED_FACE('',(#21023),#1838,.F.) ;
#89344=ADVANCED_FACE('',(#21024),#1839,.F.) ;
#89345=ADVANCED_FACE('',(#21025),#1840,.F.) ;
#89346=ADVANCED_FACE('',(#21026),#1841,.F.) ;
#89347=ADVANCED_FACE('',(#21027),#1842,.F.) ;
#89348=ADVANCED_FACE('',(#21028),#1843,.F.) ;
#89349=ADVANCED_FACE('',(#21029),#1844,.F.) ;
#89350=ADVANCED_FACE('',(#21030),#1845,.F.) ;
#89351=ADVANCED_FACE('',(#21031),#1846,.F.) ;
#89352=ADVANCED_FACE('',(#21032),#1847,.F.) ;
#89353=ADVANCED_FACE('',(#21033),#1848,.F.) ;
#89354=ADVANCED_FACE('',(#21034),#1849,.F.) ;
#89355=ADVANCED_FACE('',(#21035),#1850,.F.) ;
#89356=ADVANCED_FACE('',(#21036),#1851,.F.) ;
#89357=ADVANCED_FACE('',(#21037),#1852,.F.) ;
#89358=ADVANCED_FACE('',(#21038),#1853,.F.) ;
#89359=ADVANCED_FACE('',(#21039),#1854,.F.) ;
#89360=ADVANCED_FACE('',(#21040),#1855,.F.) ;
#89361=ADVANCED_FACE('',(#21041),#1856,.F.) ;
#89362=ADVANCED_FACE('',(#21042),#1857,.F.) ;
#89363=ADVANCED_FACE('',(#21043),#1858,.F.) ;
#89364=ADVANCED_FACE('',(#21044),#1859,.F.) ;
#89365=ADVANCED_FACE('',(#21045),#1860,.F.) ;
#89366=ADVANCED_FACE('',(#21046),#1861,.F.) ;
#89367=ADVANCED_FACE('',(#21047),#1862,.F.) ;
#89368=ADVANCED_FACE('',(#21048),#1863,.F.) ;
#89369=ADVANCED_FACE('',(#21049,#785),#1864,.T.) ;
#89370=ADVANCED_FACE('',(#21050),#1865,.T.) ;
#89371=ADVANCED_FACE('',(#21051),#1866,.T.) ;
#89372=ADVANCED_FACE('',(#21052),#1867,.T.) ;
#89373=ADVANCED_FACE('',(#21053),#1868,.T.) ;
#89374=ADVANCED_FACE('',(#21054,#786),#1869,.T.) ;
#89375=ADVANCED_FACE('',(#21055),#1870,.T.) ;
#89376=ADVANCED_FACE('',(#21056),#1871,.T.) ;
#89377=ADVANCED_FACE('',(#21057),#1872,.T.) ;
#89378=ADVANCED_FACE('',(#21058),#1873,.T.) ;
#89379=ADVANCED_FACE('',(#21059,#787),#1874,.T.) ;
#89380=ADVANCED_FACE('',(#21060),#1875,.T.) ;
#89381=ADVANCED_FACE('',(#21061),#1876,.T.) ;
#89382=ADVANCED_FACE('',(#21062),#1877,.T.) ;
#89383=ADVANCED_FACE('',(#21063),#1878,.T.) ;
#89384=ADVANCED_FACE('',(#21064,#788),#1879,.T.) ;
#89385=ADVANCED_FACE('',(#21065),#1880,.T.) ;
#89386=ADVANCED_FACE('',(#21066),#1881,.T.) ;
#89387=ADVANCED_FACE('',(#21067),#1882,.T.) ;
#89388=ADVANCED_FACE('',(#21068),#1883,.T.) ;
#89389=ADVANCED_FACE('',(#21069,#789),#1884,.T.) ;
#89390=ADVANCED_FACE('',(#21070),#1885,.T.) ;
#89391=ADVANCED_FACE('',(#21071),#1886,.T.) ;
#89392=ADVANCED_FACE('',(#21072),#1887,.T.) ;
#89393=ADVANCED_FACE('',(#21073),#1888,.T.) ;
#89394=ADVANCED_FACE('',(#21074,#790),#1889,.T.) ;
#89395=ADVANCED_FACE('',(#21075),#1890,.T.) ;
#89396=ADVANCED_FACE('',(#21076),#1891,.T.) ;
#89397=ADVANCED_FACE('',(#21077),#1892,.T.) ;
#89398=ADVANCED_FACE('',(#21078),#1893,.T.) ;
#89399=ADVANCED_FACE('',(#21079,#791),#1894,.T.) ;
#89400=ADVANCED_FACE('',(#21080),#1895,.T.) ;
#89401=ADVANCED_FACE('',(#21081),#1896,.T.) ;
#89402=ADVANCED_FACE('',(#21082),#1897,.T.) ;
#89403=ADVANCED_FACE('',(#21083),#1898,.T.) ;
#89404=ADVANCED_FACE('',(#21084,#792),#1899,.T.) ;
#89405=ADVANCED_FACE('',(#21085),#1900,.T.) ;
#89406=ADVANCED_FACE('',(#21086),#1901,.T.) ;
#89407=ADVANCED_FACE('',(#21087),#1902,.T.) ;
#89408=ADVANCED_FACE('',(#21088),#1903,.T.) ;
#89409=ADVANCED_FACE('',(#21089,#793),#1904,.T.) ;
#89410=ADVANCED_FACE('',(#21090),#1905,.T.) ;
#89411=ADVANCED_FACE('',(#21091),#1906,.T.) ;
#89412=ADVANCED_FACE('',(#21092),#1907,.T.) ;
#89413=ADVANCED_FACE('',(#21093),#1908,.T.) ;
#89414=ADVANCED_FACE('',(#21094),#1909,.T.) ;
#89415=ADVANCED_FACE('',(#21095),#1910,.T.) ;
#89416=ADVANCED_FACE('',(#21096),#1911,.T.) ;
#89417=ADVANCED_FACE('',(#21097),#1912,.T.) ;
#89418=ADVANCED_FACE('',(#21098),#1913,.T.) ;
#89419=ADVANCED_FACE('',(#21099),#1914,.T.) ;
#89420=ADVANCED_FACE('',(#21100),#1915,.T.) ;
#89421=ADVANCED_FACE('',(#21101),#1916,.T.) ;
#89422=ADVANCED_FACE('',(#21102),#1917,.T.) ;
#89423=ADVANCED_FACE('',(#21103),#1918,.T.) ;
#89424=ADVANCED_FACE('',(#21104),#1919,.T.) ;
#89425=ADVANCED_FACE('',(#21105),#1920,.T.) ;
#89426=ADVANCED_FACE('',(#21106),#1921,.T.) ;
#89427=ADVANCED_FACE('',(#21107),#1922,.T.) ;
#89428=ADVANCED_FACE('',(#21108),#1923,.T.) ;
#89429=ADVANCED_FACE('',(#21109),#1924,.T.) ;
#89430=ADVANCED_FACE('',(#21110),#1925,.T.) ;
#89431=ADVANCED_FACE('',(#21111),#1926,.T.) ;
#89432=ADVANCED_FACE('',(#21112),#1927,.F.) ;
#89433=ADVANCED_FACE('',(#21113),#1928,.F.) ;
#89434=ADVANCED_FACE('',(#21114),#1929,.T.) ;
#89435=ADVANCED_FACE('',(#21115),#1930,.F.) ;
#89436=ADVANCED_FACE('',(#21116),#1931,.F.) ;
#89437=ADVANCED_FACE('',(#21117),#1932,.T.) ;
#89438=ADVANCED_FACE('',(#21118),#1933,.F.) ;
#89439=ADVANCED_FACE('',(#21119),#1934,.F.) ;
#89440=ADVANCED_FACE('',(#21120),#1935,.T.) ;
#89441=ADVANCED_FACE('',(#21121),#1936,.F.) ;
#89442=ADVANCED_FACE('',(#21122),#1937,.F.) ;
#89443=ADVANCED_FACE('',(#21123),#1938,.T.) ;
#89444=ADVANCED_FACE('',(#21124),#1939,.F.) ;
#89445=ADVANCED_FACE('',(#21125),#1940,.F.) ;
#89446=ADVANCED_FACE('',(#21126),#1941,.T.) ;
#89447=ADVANCED_FACE('',(#21127),#1942,.F.) ;
#89448=ADVANCED_FACE('',(#21128),#1943,.F.) ;
#89449=ADVANCED_FACE('',(#21129),#1944,.T.) ;
#89450=ADVANCED_FACE('',(#21130),#1945,.F.) ;
#89451=ADVANCED_FACE('',(#21131),#1946,.F.) ;
#89452=ADVANCED_FACE('',(#21132),#1947,.T.) ;
#89453=ADVANCED_FACE('',(#21133),#1948,.F.) ;
#89454=ADVANCED_FACE('',(#21134),#1949,.F.) ;
#89455=ADVANCED_FACE('',(#21135),#1950,.T.) ;
#89456=ADVANCED_FACE('',(#21136),#1951,.F.) ;
#89457=ADVANCED_FACE('',(#21137),#1952,.F.) ;
#89458=ADVANCED_FACE('',(#21138),#1953,.T.) ;
#89459=ADVANCED_FACE('',(#21139),#15263,.T.) ;
#89460=ADVANCED_FACE('',(#21140),#1954,.F.) ;
#89461=ADVANCED_FACE('',(#21141),#15264,.T.) ;
#89462=ADVANCED_FACE('',(#21142),#1955,.F.) ;
#89463=ADVANCED_FACE('',(#21143),#15265,.T.) ;
#89464=ADVANCED_FACE('',(#21144),#1956,.F.) ;
#89465=ADVANCED_FACE('',(#21145),#15266,.T.) ;
#89466=ADVANCED_FACE('',(#21146),#1957,.F.) ;
#89467=ADVANCED_FACE('',(#21147),#1958,.F.) ;
#89468=ADVANCED_FACE('',(#21148),#15267,.T.) ;
#89469=ADVANCED_FACE('',(#21149),#1959,.F.) ;
#89470=ADVANCED_FACE('',(#21150),#15268,.T.) ;
#89471=ADVANCED_FACE('',(#21151),#1960,.F.) ;
#89472=ADVANCED_FACE('',(#21152),#15269,.T.) ;
#89473=ADVANCED_FACE('',(#21153),#1961,.F.) ;
#89474=ADVANCED_FACE('',(#21154),#15270,.T.) ;
#89475=ADVANCED_FACE('',(#21155),#1962,.F.) ;
#89476=ADVANCED_FACE('',(#21156),#1963,.F.) ;
#89477=ADVANCED_FACE('',(#21157),#15271,.T.) ;
#89478=ADVANCED_FACE('',(#21158),#1964,.F.) ;
#89479=ADVANCED_FACE('',(#21159),#15272,.T.) ;
#89480=ADVANCED_FACE('',(#21160),#1965,.F.) ;
#89481=ADVANCED_FACE('',(#21161),#15273,.T.) ;
#89482=ADVANCED_FACE('',(#21162),#1966,.F.) ;
#89483=ADVANCED_FACE('',(#21163),#15274,.T.) ;
#89484=ADVANCED_FACE('',(#21164),#1967,.F.) ;
#89485=ADVANCED_FACE('',(#21165),#1968,.F.) ;
#89486=ADVANCED_FACE('',(#21166),#15275,.T.) ;
#89487=ADVANCED_FACE('',(#21167),#1969,.F.) ;
#89488=ADVANCED_FACE('',(#21168),#15276,.T.) ;
#89489=ADVANCED_FACE('',(#21169),#1970,.F.) ;
#89490=ADVANCED_FACE('',(#21170),#15277,.T.) ;
#89491=ADVANCED_FACE('',(#21171),#1971,.F.) ;
#89492=ADVANCED_FACE('',(#21172),#15278,.T.) ;
#89493=ADVANCED_FACE('',(#21173),#1972,.F.) ;
#89494=ADVANCED_FACE('',(#21174),#1973,.F.) ;
#89495=ADVANCED_FACE('',(#21175),#15279,.T.) ;
#89496=ADVANCED_FACE('',(#21176),#1974,.F.) ;
#89497=ADVANCED_FACE('',(#21177),#15280,.T.) ;
#89498=ADVANCED_FACE('',(#21178),#1975,.F.) ;
#89499=ADVANCED_FACE('',(#21179),#15281,.T.) ;
#89500=ADVANCED_FACE('',(#21180),#1976,.F.) ;
#89501=ADVANCED_FACE('',(#21181),#15282,.T.) ;
#89502=ADVANCED_FACE('',(#21182),#1977,.F.) ;
#89503=ADVANCED_FACE('',(#21183),#1978,.F.) ;
#89504=ADVANCED_FACE('',(#21184),#15283,.T.) ;
#89505=ADVANCED_FACE('',(#21185),#1979,.F.) ;
#89506=ADVANCED_FACE('',(#21186),#15284,.T.) ;
#89507=ADVANCED_FACE('',(#21187),#1980,.F.) ;
#89508=ADVANCED_FACE('',(#21188),#15285,.T.) ;
#89509=ADVANCED_FACE('',(#21189),#1981,.F.) ;
#89510=ADVANCED_FACE('',(#21190),#15286,.T.) ;
#89511=ADVANCED_FACE('',(#21191),#1982,.F.) ;
#89512=ADVANCED_FACE('',(#21192),#1983,.F.) ;
#89513=ADVANCED_FACE('',(#21193),#15287,.T.) ;
#89514=ADVANCED_FACE('',(#21194),#1984,.F.) ;
#89515=ADVANCED_FACE('',(#21195),#15288,.T.) ;
#89516=ADVANCED_FACE('',(#21196),#1985,.F.) ;
#89517=ADVANCED_FACE('',(#21197),#15289,.T.) ;
#89518=ADVANCED_FACE('',(#21198),#1986,.F.) ;
#89519=ADVANCED_FACE('',(#21199),#15290,.T.) ;
#89520=ADVANCED_FACE('',(#21200),#1987,.F.) ;
#89521=ADVANCED_FACE('',(#21201),#1988,.F.) ;
#89522=ADVANCED_FACE('',(#21202),#15291,.T.) ;
#89523=ADVANCED_FACE('',(#21203),#1989,.F.) ;
#89524=ADVANCED_FACE('',(#21204),#15292,.T.) ;
#89525=ADVANCED_FACE('',(#21205),#1990,.F.) ;
#89526=ADVANCED_FACE('',(#21206),#15293,.T.) ;
#89527=ADVANCED_FACE('',(#21207),#1991,.F.) ;
#89528=ADVANCED_FACE('',(#21208),#15294,.T.) ;
#89529=ADVANCED_FACE('',(#21209),#1992,.F.) ;
#89530=ADVANCED_FACE('',(#21210),#1993,.F.) ;
#89531=ADVANCED_FACE('',(#21211),#15295,.T.) ;
#89532=ADVANCED_FACE('',(#21212),#1994,.F.) ;
#89533=ADVANCED_FACE('',(#21213),#15296,.T.) ;
#89534=ADVANCED_FACE('',(#21214),#1995,.F.) ;
#89535=ADVANCED_FACE('',(#21215),#15297,.T.) ;
#89536=ADVANCED_FACE('',(#21216),#1996,.F.) ;
#89537=ADVANCED_FACE('',(#21217),#15298,.T.) ;
#89538=ADVANCED_FACE('',(#21218),#1997,.F.) ;
#89539=ADVANCED_FACE('',(#21219),#1998,.F.) ;
#89540=ADVANCED_FACE('',(#21220),#16729,.T.) ;
#89541=ADVANCED_FACE('',(#21221),#79425,.T.) ;
#89542=ADVANCED_FACE('',(#21222),#15299,.T.) ;
#89543=ADVANCED_FACE('',(#21223),#15300,.T.) ;
#89544=ADVANCED_FACE('',(#21224),#15301,.T.) ;
#89545=ADVANCED_FACE('',(#21225),#15302,.T.) ;
#89546=ADVANCED_FACE('',(#21226),#16730,.T.) ;
#89547=ADVANCED_FACE('',(#21227),#79426,.F.) ;
#89548=ADVANCED_FACE('',(#21228),#16731,.T.) ;
#89549=ADVANCED_FACE('',(#21229),#15303,.T.) ;
#89550=ADVANCED_FACE('',(#21230),#15304,.T.) ;
#89551=ADVANCED_FACE('',(#21231),#15305,.T.) ;
#89552=ADVANCED_FACE('',(#21232),#79427,.F.) ;
#89553=ADVANCED_FACE('',(#21233),#15306,.F.) ;
#89554=ADVANCED_FACE('',(#21234),#15307,.T.) ;
#89555=ADVANCED_FACE('',(#21235),#16732,.T.) ;
#89556=ADVANCED_FACE('',(#21236),#79428,.F.) ;
#89557=ADVANCED_FACE('',(#21237),#79429,.T.) ;
#89558=ADVANCED_FACE('',(#21238),#15308,.T.) ;
#89559=ADVANCED_FACE('',(#21239),#15309,.F.) ;
#89560=ADVANCED_FACE('',(#21240),#15310,.T.) ;
#89561=ADVANCED_FACE('',(#21241),#15311,.F.) ;
#89562=ADVANCED_FACE('',(#21242),#15312,.F.) ;
#89563=ADVANCED_FACE('',(#21243),#79430,.T.) ;
#89564=ADVANCED_FACE('',(#21244),#16733,.T.) ;
#89565=ADVANCED_FACE('',(#21245),#16734,.F.) ;
#89566=ADVANCED_FACE('',(#21246),#15313,.T.) ;
#89567=ADVANCED_FACE('',(#21247),#15314,.T.) ;
#89568=ADVANCED_FACE('',(#21248),#15315,.T.) ;
#89569=ADVANCED_FACE('',(#21249),#15316,.F.) ;
#89570=ADVANCED_FACE('',(#21250),#16735,.T.) ;
#89571=ADVANCED_FACE('',(#21251),#79431,.F.) ;
#89572=ADVANCED_FACE('',(#21252),#15317,.F.) ;
#89573=ADVANCED_FACE('',(#21253),#15318,.T.) ;
#89574=ADVANCED_FACE('',(#21254),#15319,.F.) ;
#89575=ADVANCED_FACE('',(#21255),#16736,.F.) ;
#89576=ADVANCED_FACE('',(#21256),#79432,.F.) ;
#89577=ADVANCED_FACE('',(#21257),#15320,.F.) ;
#89578=ADVANCED_FACE('',(#21258),#79433,.F.) ;
#89579=ADVANCED_FACE('',(#21259),#15321,.F.) ;
#89580=ADVANCED_FACE('',(#21260),#15322,.F.) ;
#89581=ADVANCED_FACE('',(#21261),#79434,.F.) ;
#89582=ADVANCED_FACE('',(#21262),#79435,.F.) ;
#89583=ADVANCED_FACE('',(#21263),#15323,.F.) ;
#89584=ADVANCED_FACE('',(#21264),#15324,.F.) ;
#89585=ADVANCED_FACE('',(#21265),#79436,.F.) ;
#89586=ADVANCED_FACE('',(#21266),#15325,.T.) ;
#89587=ADVANCED_FACE('',(#21267),#15326,.T.) ;
#89588=ADVANCED_FACE('',(#21268),#15327,.T.) ;
#89589=ADVANCED_FACE('',(#21269),#15328,.T.) ;
#89590=ADVANCED_FACE('',(#21270),#15329,.T.) ;
#89591=ADVANCED_FACE('',(#21271),#15330,.T.) ;
#89592=ADVANCED_FACE('',(#21272),#15331,.T.) ;
#89593=ADVANCED_FACE('',(#21273),#15332,.T.) ;
#89594=ADVANCED_FACE('',(#21274),#15333,.T.) ;
#89595=ADVANCED_FACE('',(#21275),#15334,.T.) ;
#89596=ADVANCED_FACE('',(#21276),#15335,.T.) ;
#89597=ADVANCED_FACE('',(#21277),#15336,.T.) ;
#89598=ADVANCED_FACE('',(#21278),#15337,.T.) ;
#89599=ADVANCED_FACE('',(#21279),#15338,.T.) ;
#89600=ADVANCED_FACE('',(#21280),#15339,.T.) ;
#89601=ADVANCED_FACE('',(#21281),#15340,.T.) ;
#89602=ADVANCED_FACE('',(#21282),#15341,.T.) ;
#89603=ADVANCED_FACE('',(#21283),#15342,.T.) ;
#89604=ADVANCED_FACE('',(#21284),#15343,.T.) ;
#89605=ADVANCED_FACE('',(#21285),#15344,.T.) ;
#89606=ADVANCED_FACE('',(#21286),#15345,.T.) ;
#89607=ADVANCED_FACE('',(#21287),#15346,.T.) ;
#89608=ADVANCED_FACE('',(#21288),#15347,.T.) ;
#89609=ADVANCED_FACE('',(#21289),#15348,.T.) ;
#89610=ADVANCED_FACE('',(#21290),#15349,.T.) ;
#89611=ADVANCED_FACE('',(#21291),#15350,.T.) ;
#89612=ADVANCED_FACE('',(#21292),#15351,.T.) ;
#89613=ADVANCED_FACE('',(#21293),#15352,.T.) ;
#89614=ADVANCED_FACE('',(#21294),#15353,.T.) ;
#89615=ADVANCED_FACE('',(#21295),#15354,.T.) ;
#89616=ADVANCED_FACE('',(#21296),#15355,.T.) ;
#89617=ADVANCED_FACE('',(#21297),#15356,.T.) ;
#89618=ADVANCED_FACE('',(#21298),#15357,.T.) ;
#89619=ADVANCED_FACE('',(#21299),#79437,.T.) ;
#89620=ADVANCED_FACE('',(#21300),#79438,.T.) ;
#89621=ADVANCED_FACE('',(#21301),#15358,.T.) ;
#89622=ADVANCED_FACE('',(#21302),#15359,.F.) ;
#89623=ADVANCED_FACE('',(#21303),#15360,.F.) ;
#89624=ADVANCED_FACE('',(#21304),#15361,.F.) ;
#89625=ADVANCED_FACE('',(#21305),#15362,.T.) ;
#89626=ADVANCED_FACE('',(#21306),#15363,.T.) ;
#89627=ADVANCED_FACE('',(#21307),#79439,.T.) ;
#89628=ADVANCED_FACE('',(#21308),#16737,.F.) ;
#89629=ADVANCED_FACE('',(#21309),#16738,.F.) ;
#89630=ADVANCED_FACE('',(#21310),#79440,.T.) ;
#89631=ADVANCED_FACE('',(#21311),#15364,.F.) ;
#89632=ADVANCED_FACE('',(#21312),#15365,.F.) ;
#89633=ADVANCED_FACE('',(#21313),#15366,.F.) ;
#89634=ADVANCED_FACE('',(#21314),#15367,.F.) ;
#89635=ADVANCED_FACE('',(#21315),#16739,.F.) ;
#89636=ADVANCED_FACE('',(#21316),#16740,.F.) ;
#89637=ADVANCED_FACE('',(#21317),#15368,.F.) ;
#89638=ADVANCED_FACE('',(#21318),#15369,.T.) ;
#89639=ADVANCED_FACE('',(#21319),#15370,.T.) ;
#89640=ADVANCED_FACE('',(#21320),#15371,.T.) ;
#89641=ADVANCED_FACE('',(#21321),#16741,.T.) ;
#89642=ADVANCED_FACE('',(#21322),#16742,.T.) ;
#89643=ADVANCED_FACE('',(#21323),#15372,.T.) ;
#89644=ADVANCED_FACE('',(#21324),#15373,.T.) ;
#89645=ADVANCED_FACE('',(#21325),#15374,.T.) ;
#89646=ADVANCED_FACE('',(#21326),#15375,.T.) ;
#89647=ADVANCED_FACE('',(#21327),#16743,.T.) ;
#89648=ADVANCED_FACE('',(#21328),#16744,.T.) ;
#89649=ADVANCED_FACE('',(#21329),#15376,.T.) ;
#89650=ADVANCED_FACE('',(#21330),#15377,.F.) ;
#89651=ADVANCED_FACE('',(#21331),#16745,.F.) ;
#89652=ADVANCED_FACE('',(#21332),#15378,.F.) ;
#89653=ADVANCED_FACE('',(#21333),#15379,.F.) ;
#89654=ADVANCED_FACE('',(#21334),#15380,.F.) ;
#89655=ADVANCED_FACE('',(#21335),#134,.T.) ;
#89656=ADVANCED_FACE('',(#21336),#16746,.F.) ;
#89657=ADVANCED_FACE('',(#21337),#15381,.F.) ;
#89658=ADVANCED_FACE('',(#21338),#15382,.F.) ;
#89659=ADVANCED_FACE('',(#21339),#15383,.T.) ;
#89660=ADVANCED_FACE('',(#21340),#15384,.T.) ;
#89661=ADVANCED_FACE('',(#21341),#15385,.F.) ;
#89662=ADVANCED_FACE('',(#21342),#16747,.F.) ;
#89663=ADVANCED_FACE('',(#21343),#135,.T.) ;
#89664=ADVANCED_FACE('',(#21344),#136,.T.) ;
#89665=ADVANCED_FACE('',(#21345),#15386,.F.) ;
#89666=ADVANCED_FACE('',(#21346),#15387,.F.) ;
#89667=ADVANCED_FACE('',(#21347),#15388,.T.) ;
#89668=ADVANCED_FACE('',(#21348),#15389,.T.) ;
#89669=ADVANCED_FACE('',(#21349),#16748,.F.) ;
#89670=ADVANCED_FACE('',(#21350),#137,.T.) ;
#89671=ADVANCED_FACE('',(#21351),#15390,.F.) ;
#89672=ADVANCED_FACE('',(#21352),#15391,.T.) ;
#89673=ADVANCED_FACE('',(#21353),#15392,.T.) ;
#89674=ADVANCED_FACE('',(#21354),#15393,.T.) ;
#89675=ADVANCED_FACE('',(#21355),#15394,.T.) ;
#89676=ADVANCED_FACE('',(#21356),#15395,.T.) ;
#89677=ADVANCED_FACE('',(#21357),#15396,.T.) ;
#89678=ADVANCED_FACE('',(#21358),#15397,.T.) ;
#89679=ADVANCED_FACE('',(#21359),#15398,.T.) ;
#89680=ADVANCED_FACE('',(#21360),#15399,.T.) ;
#89681=ADVANCED_FACE('',(#21361),#15400,.T.) ;
#89682=ADVANCED_FACE('',(#21362),#15401,.T.) ;
#89683=ADVANCED_FACE('',(#21363),#15402,.T.) ;
#89684=ADVANCED_FACE('',(#21364),#15403,.T.) ;
#89685=ADVANCED_FACE('',(#21365),#15404,.T.) ;
#89686=ADVANCED_FACE('',(#21366),#15405,.T.) ;
#89687=ADVANCED_FACE('',(#21367),#15406,.T.) ;
#89688=ADVANCED_FACE('',(#21368),#15407,.T.) ;
#89689=ADVANCED_FACE('',(#21369),#15408,.T.) ;
#89690=ADVANCED_FACE('',(#21370),#15409,.T.) ;
#89691=ADVANCED_FACE('',(#21371),#15410,.T.) ;
#89692=ADVANCED_FACE('',(#21372),#15411,.T.) ;
#89693=ADVANCED_FACE('',(#21373),#15412,.T.) ;
#89694=ADVANCED_FACE('',(#21374),#15413,.T.) ;
#89695=ADVANCED_FACE('',(#21375),#15414,.T.) ;
#89696=ADVANCED_FACE('',(#21376),#15415,.T.) ;
#89697=ADVANCED_FACE('',(#21377),#15416,.T.) ;
#89698=ADVANCED_FACE('',(#21378),#15417,.T.) ;
#89699=ADVANCED_FACE('',(#21379),#15418,.T.) ;
#89700=ADVANCED_FACE('',(#21380),#15419,.T.) ;
#89701=ADVANCED_FACE('',(#21381),#15420,.T.) ;
#89702=ADVANCED_FACE('',(#21382),#15421,.T.) ;
#89703=ADVANCED_FACE('',(#21383),#15422,.T.) ;
#89704=ADVANCED_FACE('',(#21384),#15423,.T.) ;
#89705=ADVANCED_FACE('',(#21385),#79441,.T.) ;
#89706=ADVANCED_FACE('',(#21386),#79442,.T.) ;
#89707=ADVANCED_FACE('',(#21387),#15424,.T.) ;
#89708=ADVANCED_FACE('',(#21388),#15425,.F.) ;
#89709=ADVANCED_FACE('',(#21389),#15426,.F.) ;
#89710=ADVANCED_FACE('',(#21390),#15427,.F.) ;
#89711=ADVANCED_FACE('',(#21391),#15428,.T.) ;
#89712=ADVANCED_FACE('',(#21392),#15429,.T.) ;
#89713=ADVANCED_FACE('',(#21393),#79443,.T.) ;
#89714=ADVANCED_FACE('',(#21394),#16749,.F.) ;
#89715=ADVANCED_FACE('',(#21395),#16750,.F.) ;
#89716=ADVANCED_FACE('',(#21396),#79444,.T.) ;
#89717=ADVANCED_FACE('',(#21397),#15430,.F.) ;
#89718=ADVANCED_FACE('',(#21398),#15431,.F.) ;
#89719=ADVANCED_FACE('',(#21399),#15432,.F.) ;
#89720=ADVANCED_FACE('',(#21400),#15433,.F.) ;
#89721=ADVANCED_FACE('',(#21401),#16751,.F.) ;
#89722=ADVANCED_FACE('',(#21402),#16752,.F.) ;
#89723=ADVANCED_FACE('',(#21403),#15434,.F.) ;
#89724=ADVANCED_FACE('',(#21404),#15435,.T.) ;
#89725=ADVANCED_FACE('',(#21405),#15436,.T.) ;
#89726=ADVANCED_FACE('',(#21406),#15437,.T.) ;
#89727=ADVANCED_FACE('',(#21407),#16753,.T.) ;
#89728=ADVANCED_FACE('',(#21408),#16754,.T.) ;
#89729=ADVANCED_FACE('',(#21409),#15438,.T.) ;
#89730=ADVANCED_FACE('',(#21410),#15439,.T.) ;
#89731=ADVANCED_FACE('',(#21411),#15440,.T.) ;
#89732=ADVANCED_FACE('',(#21412),#15441,.T.) ;
#89733=ADVANCED_FACE('',(#21413),#16755,.T.) ;
#89734=ADVANCED_FACE('',(#21414),#16756,.T.) ;
#89735=ADVANCED_FACE('',(#21415),#15442,.T.) ;
#89736=ADVANCED_FACE('',(#21416),#15443,.T.) ;
#89737=ADVANCED_FACE('',(#21417),#16757,.T.) ;
#89738=ADVANCED_FACE('',(#21418),#16758,.T.) ;
#89739=ADVANCED_FACE('',(#21419),#15444,.T.) ;
#89740=ADVANCED_FACE('',(#21420),#15445,.T.) ;
#89741=ADVANCED_FACE('',(#21421),#16759,.T.) ;
#89742=ADVANCED_FACE('',(#21422),#16760,.T.) ;
#89743=ADVANCED_FACE('',(#21423),#15446,.T.) ;
#89744=ADVANCED_FACE('',(#21424),#15447,.T.) ;
#89745=ADVANCED_FACE('',(#21425),#15448,.F.) ;
#89746=ADVANCED_FACE('',(#21426),#15449,.F.) ;
#89747=ADVANCED_FACE('',(#21427),#15450,.T.) ;
#89748=ADVANCED_FACE('',(#21428),#16761,.T.) ;
#89749=ADVANCED_FACE('',(#21429),#15451,.T.) ;
#89750=ADVANCED_FACE('',(#21430),#15452,.T.) ;
#89751=ADVANCED_FACE('',(#21431),#79445,.T.) ;
#89752=ADVANCED_FACE('',(#21432),#15453,.T.) ;
#89753=ADVANCED_FACE('',(#21433),#16762,.T.) ;
#89754=ADVANCED_FACE('',(#21434),#79446,.F.) ;
#89755=ADVANCED_FACE('',(#21435),#16763,.T.) ;
#89756=ADVANCED_FACE('',(#21436),#15454,.T.) ;
#89757=ADVANCED_FACE('',(#21437),#15455,.T.) ;
#89758=ADVANCED_FACE('',(#21438),#15456,.F.) ;
#89759=ADVANCED_FACE('',(#21439),#79447,.F.) ;
#89760=ADVANCED_FACE('',(#21440),#15457,.T.) ;
#89761=ADVANCED_FACE('',(#21441),#15458,.T.) ;
#89762=ADVANCED_FACE('',(#21442),#15459,.T.) ;
#89763=ADVANCED_FACE('',(#21443),#79448,.T.) ;
#89764=ADVANCED_FACE('',(#21444),#79449,.F.) ;
#89765=ADVANCED_FACE('',(#21445),#16764,.T.) ;
#89766=ADVANCED_FACE('',(#21446),#15460,.F.) ;
#89767=ADVANCED_FACE('',(#21447),#15461,.T.) ;
#89768=ADVANCED_FACE('',(#21448),#15462,.F.) ;
#89769=ADVANCED_FACE('',(#21449),#15463,.T.) ;
#89770=ADVANCED_FACE('',(#21450),#16765,.F.) ;
#89771=ADVANCED_FACE('',(#21451),#16766,.T.) ;
#89772=ADVANCED_FACE('',(#21452),#79450,.T.) ;
#89773=ADVANCED_FACE('',(#21453),#15464,.F.) ;
#89774=ADVANCED_FACE('',(#21454),#15465,.T.) ;
#89775=ADVANCED_FACE('',(#21455),#15466,.T.) ;
#89776=ADVANCED_FACE('',(#21456),#15467,.T.) ;
#89777=ADVANCED_FACE('',(#21457),#79451,.F.) ;
#89778=ADVANCED_FACE('',(#21458),#16767,.T.) ;
#89779=ADVANCED_FACE('',(#21459),#15468,.F.) ;
#89780=ADVANCED_FACE('',(#21460),#15469,.T.) ;
#89781=ADVANCED_FACE('',(#21461),#15470,.F.) ;
#89782=ADVANCED_FACE('',(#21462),#15471,.F.) ;
#89783=ADVANCED_FACE('',(#21463),#79452,.F.) ;
#89784=ADVANCED_FACE('',(#21464),#16768,.F.) ;
#89785=ADVANCED_FACE('',(#21465),#15472,.F.) ;
#89786=ADVANCED_FACE('',(#21466),#138,.F.) ;
#89787=ADVANCED_FACE('',(#21467),#15473,.F.) ;
#89788=ADVANCED_FACE('',(#21468),#139,.F.) ;
#89789=ADVANCED_FACE('',(#21469),#16769,.F.) ;
#89790=ADVANCED_FACE('',(#21470),#140,.F.) ;
#89791=ADVANCED_FACE('',(#21471),#15474,.F.) ;
#89792=ADVANCED_FACE('',(#21472),#15475,.F.) ;
#89793=ADVANCED_FACE('',(#21473),#15476,.F.) ;
#89794=ADVANCED_FACE('',(#21474),#15477,.F.) ;
#89795=ADVANCED_FACE('',(#21475),#16770,.F.) ;
#89796=ADVANCED_FACE('',(#21476),#16771,.F.) ;
#89797=ADVANCED_FACE('',(#21477),#15478,.F.) ;
#89798=ADVANCED_FACE('',(#21478),#15479,.F.) ;
#89799=ADVANCED_FACE('',(#21479),#16772,.F.) ;
#89800=ADVANCED_FACE('',(#21480),#15480,.F.) ;
#89801=ADVANCED_FACE('',(#21481),#141,.F.) ;
#89802=ADVANCED_FACE('',(#21482),#142,.F.) ;
#89803=ADVANCED_FACE('',(#21483),#143,.F.) ;
#89804=ADVANCED_FACE('',(#21484),#15481,.F.) ;
#89805=ADVANCED_FACE('',(#21485),#15482,.F.) ;
#89806=ADVANCED_FACE('',(#21486),#16773,.F.) ;
#89807=ADVANCED_FACE('',(#21487),#15483,.F.) ;
#89808=ADVANCED_FACE('',(#21488),#15484,.F.) ;
#89809=ADVANCED_FACE('',(#21489),#16774,.F.) ;
#89810=ADVANCED_FACE('',(#21490),#15485,.F.) ;
#89811=ADVANCED_FACE('',(#21491),#144,.F.) ;
#89812=ADVANCED_FACE('',(#21492),#145,.F.) ;
#89813=ADVANCED_FACE('',(#21493),#146,.F.) ;
#89814=ADVANCED_FACE('',(#21494),#147,.F.) ;
#89815=ADVANCED_FACE('',(#21495),#15486,.F.) ;
#89816=ADVANCED_FACE('',(#21496),#15487,.F.) ;
#89817=ADVANCED_FACE('',(#21497),#16775,.F.) ;
#89818=ADVANCED_FACE('',(#21498),#15488,.F.) ;
#89819=ADVANCED_FACE('',(#21499),#15489,.F.) ;
#89820=ADVANCED_FACE('',(#21500),#16776,.F.) ;
#89821=ADVANCED_FACE('',(#21501),#15490,.F.) ;
#89822=ADVANCED_FACE('',(#21502),#148,.F.) ;
#89823=ADVANCED_FACE('',(#21503),#149,.F.) ;
#89824=ADVANCED_FACE('',(#21504),#79453,.F.) ;
#89825=ADVANCED_FACE('',(#21505),#15491,.F.) ;
#89826=ADVANCED_FACE('',(#21506),#15492,.F.) ;
#89827=ADVANCED_FACE('',(#21507),#79454,.F.) ;
#89828=ADVANCED_FACE('',(#21508),#79455,.F.) ;
#89829=ADVANCED_FACE('',(#21509),#15493,.F.) ;
#89830=ADVANCED_FACE('',(#21510),#15494,.F.) ;
#89831=ADVANCED_FACE('',(#21511),#79456,.F.) ;
#89832=ADVANCED_FACE('',(#21512),#15495,.T.) ;
#89833=ADVANCED_FACE('',(#21513),#15496,.T.) ;
#89834=ADVANCED_FACE('',(#21514),#15497,.T.) ;
#89835=ADVANCED_FACE('',(#21515),#16777,.T.) ;
#89836=ADVANCED_FACE('',(#21516),#16778,.T.) ;
#89837=ADVANCED_FACE('',(#21517),#15498,.T.) ;
#89838=ADVANCED_FACE('',(#21518),#15499,.T.) ;
#89839=ADVANCED_FACE('',(#21519),#15500,.T.) ;
#89840=ADVANCED_FACE('',(#21520),#15501,.T.) ;
#89841=ADVANCED_FACE('',(#21521),#16779,.T.) ;
#89842=ADVANCED_FACE('',(#21522),#16780,.T.) ;
#89843=ADVANCED_FACE('',(#21523),#15502,.T.) ;
#89844=ADVANCED_FACE('',(#21524),#15503,.T.) ;
#89845=ADVANCED_FACE('',(#21525),#79457,.T.) ;
#89846=ADVANCED_FACE('',(#21526),#79458,.T.) ;
#89847=ADVANCED_FACE('',(#21527),#15504,.T.) ;
#89848=ADVANCED_FACE('',(#21528),#15505,.F.) ;
#89849=ADVANCED_FACE('',(#21529),#15506,.F.) ;
#89850=ADVANCED_FACE('',(#21530),#15507,.F.) ;
#89851=ADVANCED_FACE('',(#21531),#15508,.T.) ;
#89852=ADVANCED_FACE('',(#21532),#15509,.T.) ;
#89853=ADVANCED_FACE('',(#21533),#79459,.T.) ;
#89854=ADVANCED_FACE('',(#21534),#16781,.F.) ;
#89855=ADVANCED_FACE('',(#21535),#16782,.F.) ;
#89856=ADVANCED_FACE('',(#21536),#79460,.T.) ;
#89857=ADVANCED_FACE('',(#21537),#15510,.F.) ;
#89858=ADVANCED_FACE('',(#21538),#15511,.F.) ;
#89859=ADVANCED_FACE('',(#21539),#15512,.F.) ;
#89860=ADVANCED_FACE('',(#21540),#15513,.F.) ;
#89861=ADVANCED_FACE('',(#21541),#16783,.F.) ;
#89862=ADVANCED_FACE('',(#21542),#16784,.F.) ;
#89863=ADVANCED_FACE('',(#21543),#15514,.F.) ;
#89864=ADVANCED_FACE('',(#21544),#15515,.T.) ;
#89865=ADVANCED_FACE('',(#21545),#15516,.T.) ;
#89866=ADVANCED_FACE('',(#21546),#15517,.T.) ;
#89867=ADVANCED_FACE('',(#21547),#16785,.T.) ;
#89868=ADVANCED_FACE('',(#21548),#16786,.T.) ;
#89869=ADVANCED_FACE('',(#21549),#15518,.T.) ;
#89870=ADVANCED_FACE('',(#21550),#15519,.T.) ;
#89871=ADVANCED_FACE('',(#21551),#15520,.T.) ;
#89872=ADVANCED_FACE('',(#21552),#15521,.T.) ;
#89873=ADVANCED_FACE('',(#21553),#16787,.T.) ;
#89874=ADVANCED_FACE('',(#21554),#16788,.T.) ;
#89875=ADVANCED_FACE('',(#21555),#15522,.T.) ;
#89876=ADVANCED_FACE('',(#21556),#15523,.T.) ;
#89877=ADVANCED_FACE('',(#21557),#16789,.T.) ;
#89878=ADVANCED_FACE('',(#21558),#16790,.T.) ;
#89879=ADVANCED_FACE('',(#21559),#15524,.T.) ;
#89880=ADVANCED_FACE('',(#21560),#15525,.T.) ;
#89881=ADVANCED_FACE('',(#21561),#16791,.T.) ;
#89882=ADVANCED_FACE('',(#21562),#16792,.T.) ;
#89883=ADVANCED_FACE('',(#21563),#15526,.T.) ;
#89884=ADVANCED_FACE('',(#21564),#15527,.T.) ;
#89885=ADVANCED_FACE('',(#21565),#15528,.F.) ;
#89886=ADVANCED_FACE('',(#21566),#15529,.F.) ;
#89887=ADVANCED_FACE('',(#21567),#15530,.T.) ;
#89888=ADVANCED_FACE('',(#21568),#16793,.T.) ;
#89889=ADVANCED_FACE('',(#21569),#15531,.T.) ;
#89890=ADVANCED_FACE('',(#21570),#15532,.T.) ;
#89891=ADVANCED_FACE('',(#21571),#79461,.T.) ;
#89892=ADVANCED_FACE('',(#21572),#15533,.T.) ;
#89893=ADVANCED_FACE('',(#21573),#16794,.T.) ;
#89894=ADVANCED_FACE('',(#21574),#79462,.F.) ;
#89895=ADVANCED_FACE('',(#21575),#16795,.T.) ;
#89896=ADVANCED_FACE('',(#21576),#15534,.T.) ;
#89897=ADVANCED_FACE('',(#21577),#15535,.T.) ;
#89898=ADVANCED_FACE('',(#21578),#15536,.F.) ;
#89899=ADVANCED_FACE('',(#21579),#79463,.F.) ;
#89900=ADVANCED_FACE('',(#21580),#15537,.T.) ;
#89901=ADVANCED_FACE('',(#21581),#15538,.T.) ;
#89902=ADVANCED_FACE('',(#21582),#15539,.T.) ;
#89903=ADVANCED_FACE('',(#21583),#79464,.T.) ;
#89904=ADVANCED_FACE('',(#21584),#79465,.F.) ;
#89905=ADVANCED_FACE('',(#21585),#16796,.T.) ;
#89906=ADVANCED_FACE('',(#21586),#15540,.F.) ;
#89907=ADVANCED_FACE('',(#21587),#15541,.T.) ;
#89908=ADVANCED_FACE('',(#21588),#15542,.F.) ;
#89909=ADVANCED_FACE('',(#21589),#15543,.T.) ;
#89910=ADVANCED_FACE('',(#21590),#16797,.F.) ;
#89911=ADVANCED_FACE('',(#21591),#16798,.T.) ;
#89912=ADVANCED_FACE('',(#21592),#79466,.T.) ;
#89913=ADVANCED_FACE('',(#21593),#15544,.F.) ;
#89914=ADVANCED_FACE('',(#21594),#15545,.T.) ;
#89915=ADVANCED_FACE('',(#21595),#15546,.T.) ;
#89916=ADVANCED_FACE('',(#21596),#15547,.T.) ;
#89917=ADVANCED_FACE('',(#21597),#79467,.F.) ;
#89918=ADVANCED_FACE('',(#21598),#16799,.T.) ;
#89919=ADVANCED_FACE('',(#21599),#15548,.F.) ;
#89920=ADVANCED_FACE('',(#21600),#15549,.T.) ;
#89921=ADVANCED_FACE('',(#21601),#15550,.F.) ;
#89922=ADVANCED_FACE('',(#21602),#15551,.F.) ;
#89923=ADVANCED_FACE('',(#21603),#79468,.F.) ;
#89924=ADVANCED_FACE('',(#21604),#16800,.F.) ;
#89925=ADVANCED_FACE('',(#21605),#15552,.F.) ;
#89926=ADVANCED_FACE('',(#21606),#150,.F.) ;
#89927=ADVANCED_FACE('',(#21607),#15553,.F.) ;
#89928=ADVANCED_FACE('',(#21608),#151,.F.) ;
#89929=ADVANCED_FACE('',(#21609),#16801,.F.) ;
#89930=ADVANCED_FACE('',(#21610),#152,.F.) ;
#89931=ADVANCED_FACE('',(#21611),#15554,.F.) ;
#89932=ADVANCED_FACE('',(#21612),#15555,.F.) ;
#89933=ADVANCED_FACE('',(#21613),#15556,.F.) ;
#89934=ADVANCED_FACE('',(#21614),#15557,.F.) ;
#89935=ADVANCED_FACE('',(#21615),#16802,.F.) ;
#89936=ADVANCED_FACE('',(#21616),#16803,.F.) ;
#89937=ADVANCED_FACE('',(#21617),#15558,.F.) ;
#89938=ADVANCED_FACE('',(#21618),#15559,.F.) ;
#89939=ADVANCED_FACE('',(#21619),#16804,.F.) ;
#89940=ADVANCED_FACE('',(#21620),#15560,.F.) ;
#89941=ADVANCED_FACE('',(#21621),#153,.F.) ;
#89942=ADVANCED_FACE('',(#21622),#154,.F.) ;
#89943=ADVANCED_FACE('',(#21623),#155,.F.) ;
#89944=ADVANCED_FACE('',(#21624),#15561,.F.) ;
#89945=ADVANCED_FACE('',(#21625),#15562,.F.) ;
#89946=ADVANCED_FACE('',(#21626),#16805,.F.) ;
#89947=ADVANCED_FACE('',(#21627),#15563,.F.) ;
#89948=ADVANCED_FACE('',(#21628),#15564,.F.) ;
#89949=ADVANCED_FACE('',(#21629),#16806,.F.) ;
#89950=ADVANCED_FACE('',(#21630),#15565,.F.) ;
#89951=ADVANCED_FACE('',(#21631),#156,.F.) ;
#89952=ADVANCED_FACE('',(#21632),#157,.F.) ;
#89953=ADVANCED_FACE('',(#21633),#158,.F.) ;
#89954=ADVANCED_FACE('',(#21634),#159,.F.) ;
#89955=ADVANCED_FACE('',(#21635),#15566,.F.) ;
#89956=ADVANCED_FACE('',(#21636),#15567,.F.) ;
#89957=ADVANCED_FACE('',(#21637),#16807,.F.) ;
#89958=ADVANCED_FACE('',(#21638),#15568,.F.) ;
#89959=ADVANCED_FACE('',(#21639),#15569,.F.) ;
#89960=ADVANCED_FACE('',(#21640),#16808,.F.) ;
#89961=ADVANCED_FACE('',(#21641),#15570,.F.) ;
#89962=ADVANCED_FACE('',(#21642),#160,.F.) ;
#89963=ADVANCED_FACE('',(#21643),#161,.F.) ;
#89964=ADVANCED_FACE('',(#21644),#79469,.F.) ;
#89965=ADVANCED_FACE('',(#21645),#15571,.F.) ;
#89966=ADVANCED_FACE('',(#21646),#15572,.F.) ;
#89967=ADVANCED_FACE('',(#21647),#79470,.F.) ;
#89968=ADVANCED_FACE('',(#21648),#79471,.F.) ;
#89969=ADVANCED_FACE('',(#21649),#15573,.F.) ;
#89970=ADVANCED_FACE('',(#21650),#15574,.F.) ;
#89971=ADVANCED_FACE('',(#21651),#79472,.F.) ;
#89972=ADVANCED_FACE('',(#21652),#15575,.T.) ;
#89973=ADVANCED_FACE('',(#21653),#15576,.T.) ;
#89974=ADVANCED_FACE('',(#21654),#15577,.T.) ;
#89975=ADVANCED_FACE('',(#21655),#16809,.T.) ;
#89976=ADVANCED_FACE('',(#21656),#16810,.T.) ;
#89977=ADVANCED_FACE('',(#21657),#15578,.T.) ;
#89978=ADVANCED_FACE('',(#21658),#15579,.T.) ;
#89979=ADVANCED_FACE('',(#21659),#15580,.T.) ;
#89980=ADVANCED_FACE('',(#21660),#15581,.T.) ;
#89981=ADVANCED_FACE('',(#21661),#16811,.T.) ;
#89982=ADVANCED_FACE('',(#21662),#16812,.T.) ;
#89983=ADVANCED_FACE('',(#21663),#15582,.T.) ;
#89984=ADVANCED_FACE('',(#21664),#15583,.T.) ;
#89985=ADVANCED_FACE('',(#21665),#79473,.T.) ;
#89986=ADVANCED_FACE('',(#21666),#79474,.T.) ;
#89987=ADVANCED_FACE('',(#21667),#15584,.T.) ;
#89988=ADVANCED_FACE('',(#21668),#15585,.F.) ;
#89989=ADVANCED_FACE('',(#21669),#15586,.F.) ;
#89990=ADVANCED_FACE('',(#21670),#15587,.F.) ;
#89991=ADVANCED_FACE('',(#21671),#15588,.T.) ;
#89992=ADVANCED_FACE('',(#21672),#15589,.T.) ;
#89993=ADVANCED_FACE('',(#21673),#79475,.T.) ;
#89994=ADVANCED_FACE('',(#21674),#16813,.F.) ;
#89995=ADVANCED_FACE('',(#21675),#16814,.F.) ;
#89996=ADVANCED_FACE('',(#21676),#79476,.T.) ;
#89997=ADVANCED_FACE('',(#21677),#15590,.F.) ;
#89998=ADVANCED_FACE('',(#21678),#15591,.F.) ;
#89999=ADVANCED_FACE('',(#21679),#15592,.F.) ;
#90000=ADVANCED_FACE('',(#21680),#15593,.F.) ;
#90001=ADVANCED_FACE('',(#21681),#16815,.F.) ;
#90002=ADVANCED_FACE('',(#21682),#16816,.F.) ;
#90003=ADVANCED_FACE('',(#21683),#15594,.F.) ;
#90004=ADVANCED_FACE('',(#21684),#15595,.T.) ;
#90005=ADVANCED_FACE('',(#21685),#15596,.T.) ;
#90006=ADVANCED_FACE('',(#21686),#15597,.T.) ;
#90007=ADVANCED_FACE('',(#21687),#16817,.T.) ;
#90008=ADVANCED_FACE('',(#21688),#16818,.T.) ;
#90009=ADVANCED_FACE('',(#21689),#15598,.T.) ;
#90010=ADVANCED_FACE('',(#21690),#15599,.T.) ;
#90011=ADVANCED_FACE('',(#21691),#15600,.T.) ;
#90012=ADVANCED_FACE('',(#21692),#15601,.T.) ;
#90013=ADVANCED_FACE('',(#21693),#16819,.T.) ;
#90014=ADVANCED_FACE('',(#21694),#16820,.T.) ;
#90015=ADVANCED_FACE('',(#21695),#15602,.T.) ;
#90016=ADVANCED_FACE('',(#21696),#15603,.T.) ;
#90017=ADVANCED_FACE('',(#21697),#16821,.T.) ;
#90018=ADVANCED_FACE('',(#21698),#16822,.T.) ;
#90019=ADVANCED_FACE('',(#21699),#15604,.T.) ;
#90020=ADVANCED_FACE('',(#21700),#15605,.T.) ;
#90021=ADVANCED_FACE('',(#21701),#16823,.T.) ;
#90022=ADVANCED_FACE('',(#21702),#16824,.T.) ;
#90023=ADVANCED_FACE('',(#21703),#15606,.T.) ;
#90024=ADVANCED_FACE('',(#21704),#15607,.T.) ;
#90025=ADVANCED_FACE('',(#21705),#15608,.F.) ;
#90026=ADVANCED_FACE('',(#21706),#15609,.F.) ;
#90027=ADVANCED_FACE('',(#21707),#15610,.T.) ;
#90028=ADVANCED_FACE('',(#21708),#16825,.T.) ;
#90029=ADVANCED_FACE('',(#21709),#15611,.T.) ;
#90030=ADVANCED_FACE('',(#21710),#15612,.T.) ;
#90031=ADVANCED_FACE('',(#21711),#79477,.T.) ;
#90032=ADVANCED_FACE('',(#21712),#15613,.T.) ;
#90033=ADVANCED_FACE('',(#21713),#16826,.T.) ;
#90034=ADVANCED_FACE('',(#21714),#79478,.F.) ;
#90035=ADVANCED_FACE('',(#21715),#16827,.T.) ;
#90036=ADVANCED_FACE('',(#21716),#15614,.T.) ;
#90037=ADVANCED_FACE('',(#21717),#15615,.T.) ;
#90038=ADVANCED_FACE('',(#21718),#15616,.F.) ;
#90039=ADVANCED_FACE('',(#21719),#79479,.F.) ;
#90040=ADVANCED_FACE('',(#21720),#15617,.T.) ;
#90041=ADVANCED_FACE('',(#21721),#15618,.T.) ;
#90042=ADVANCED_FACE('',(#21722),#15619,.T.) ;
#90043=ADVANCED_FACE('',(#21723),#79480,.T.) ;
#90044=ADVANCED_FACE('',(#21724),#79481,.F.) ;
#90045=ADVANCED_FACE('',(#21725),#16828,.T.) ;
#90046=ADVANCED_FACE('',(#21726),#15620,.F.) ;
#90047=ADVANCED_FACE('',(#21727),#15621,.T.) ;
#90048=ADVANCED_FACE('',(#21728),#15622,.F.) ;
#90049=ADVANCED_FACE('',(#21729),#15623,.T.) ;
#90050=ADVANCED_FACE('',(#21730),#16829,.F.) ;
#90051=ADVANCED_FACE('',(#21731),#16830,.T.) ;
#90052=ADVANCED_FACE('',(#21732),#79482,.T.) ;
#90053=ADVANCED_FACE('',(#21733),#15624,.F.) ;
#90054=ADVANCED_FACE('',(#21734),#15625,.T.) ;
#90055=ADVANCED_FACE('',(#21735),#15626,.T.) ;
#90056=ADVANCED_FACE('',(#21736),#15627,.T.) ;
#90057=ADVANCED_FACE('',(#21737),#79483,.F.) ;
#90058=ADVANCED_FACE('',(#21738),#16831,.T.) ;
#90059=ADVANCED_FACE('',(#21739),#15628,.F.) ;
#90060=ADVANCED_FACE('',(#21740),#15629,.T.) ;
#90061=ADVANCED_FACE('',(#21741),#15630,.F.) ;
#90062=ADVANCED_FACE('',(#21742),#15631,.F.) ;
#90063=ADVANCED_FACE('',(#21743),#79484,.F.) ;
#90064=ADVANCED_FACE('',(#21744),#16832,.F.) ;
#90065=ADVANCED_FACE('',(#21745),#15632,.F.) ;
#90066=ADVANCED_FACE('',(#21746),#162,.F.) ;
#90067=ADVANCED_FACE('',(#21747),#15633,.F.) ;
#90068=ADVANCED_FACE('',(#21748),#163,.F.) ;
#90069=ADVANCED_FACE('',(#21749),#16833,.F.) ;
#90070=ADVANCED_FACE('',(#21750),#164,.F.) ;
#90071=ADVANCED_FACE('',(#21751),#15634,.F.) ;
#90072=ADVANCED_FACE('',(#21752),#15635,.F.) ;
#90073=ADVANCED_FACE('',(#21753),#15636,.F.) ;
#90074=ADVANCED_FACE('',(#21754),#15637,.F.) ;
#90075=ADVANCED_FACE('',(#21755),#16834,.F.) ;
#90076=ADVANCED_FACE('',(#21756),#16835,.F.) ;
#90077=ADVANCED_FACE('',(#21757),#15638,.F.) ;
#90078=ADVANCED_FACE('',(#21758),#15639,.F.) ;
#90079=ADVANCED_FACE('',(#21759),#16836,.F.) ;
#90080=ADVANCED_FACE('',(#21760),#15640,.F.) ;
#90081=ADVANCED_FACE('',(#21761),#165,.F.) ;
#90082=ADVANCED_FACE('',(#21762),#166,.F.) ;
#90083=ADVANCED_FACE('',(#21763),#167,.F.) ;
#90084=ADVANCED_FACE('',(#21764),#15641,.F.) ;
#90085=ADVANCED_FACE('',(#21765),#15642,.F.) ;
#90086=ADVANCED_FACE('',(#21766),#16837,.F.) ;
#90087=ADVANCED_FACE('',(#21767),#15643,.F.) ;
#90088=ADVANCED_FACE('',(#21768),#15644,.F.) ;
#90089=ADVANCED_FACE('',(#21769),#16838,.F.) ;
#90090=ADVANCED_FACE('',(#21770),#15645,.F.) ;
#90091=ADVANCED_FACE('',(#21771),#168,.F.) ;
#90092=ADVANCED_FACE('',(#21772),#169,.F.) ;
#90093=ADVANCED_FACE('',(#21773),#170,.F.) ;
#90094=ADVANCED_FACE('',(#21774),#171,.F.) ;
#90095=ADVANCED_FACE('',(#21775),#15646,.F.) ;
#90096=ADVANCED_FACE('',(#21776),#15647,.F.) ;
#90097=ADVANCED_FACE('',(#21777),#16839,.F.) ;
#90098=ADVANCED_FACE('',(#21778),#15648,.F.) ;
#90099=ADVANCED_FACE('',(#21779),#15649,.F.) ;
#90100=ADVANCED_FACE('',(#21780),#16840,.F.) ;
#90101=ADVANCED_FACE('',(#21781),#15650,.F.) ;
#90102=ADVANCED_FACE('',(#21782),#172,.F.) ;
#90103=ADVANCED_FACE('',(#21783),#173,.F.) ;
#90104=ADVANCED_FACE('',(#21784),#79485,.F.) ;
#90105=ADVANCED_FACE('',(#21785),#15651,.F.) ;
#90106=ADVANCED_FACE('',(#21786),#15652,.F.) ;
#90107=ADVANCED_FACE('',(#21787),#79486,.F.) ;
#90108=ADVANCED_FACE('',(#21788),#79487,.F.) ;
#90109=ADVANCED_FACE('',(#21789),#15653,.F.) ;
#90110=ADVANCED_FACE('',(#21790),#15654,.F.) ;
#90111=ADVANCED_FACE('',(#21791),#79488,.F.) ;
#90112=ADVANCED_FACE('',(#21792),#15655,.T.) ;
#90113=ADVANCED_FACE('',(#21793),#15656,.T.) ;
#90114=ADVANCED_FACE('',(#21794),#15657,.T.) ;
#90115=ADVANCED_FACE('',(#21795),#16841,.T.) ;
#90116=ADVANCED_FACE('',(#21796),#16842,.T.) ;
#90117=ADVANCED_FACE('',(#21797),#15658,.T.) ;
#90118=ADVANCED_FACE('',(#21798),#15659,.T.) ;
#90119=ADVANCED_FACE('',(#21799),#15660,.T.) ;
#90120=ADVANCED_FACE('',(#21800),#15661,.T.) ;
#90121=ADVANCED_FACE('',(#21801),#16843,.T.) ;
#90122=ADVANCED_FACE('',(#21802),#16844,.T.) ;
#90123=ADVANCED_FACE('',(#21803),#15662,.T.) ;
#90124=ADVANCED_FACE('',(#21804),#15663,.T.) ;
#90125=ADVANCED_FACE('',(#21805),#79489,.T.) ;
#90126=ADVANCED_FACE('',(#21806),#79490,.T.) ;
#90127=ADVANCED_FACE('',(#21807),#15664,.T.) ;
#90128=ADVANCED_FACE('',(#21808),#15665,.F.) ;
#90129=ADVANCED_FACE('',(#21809),#15666,.F.) ;
#90130=ADVANCED_FACE('',(#21810),#15667,.F.) ;
#90131=ADVANCED_FACE('',(#21811),#15668,.T.) ;
#90132=ADVANCED_FACE('',(#21812),#15669,.T.) ;
#90133=ADVANCED_FACE('',(#21813),#79491,.T.) ;
#90134=ADVANCED_FACE('',(#21814),#16845,.F.) ;
#90135=ADVANCED_FACE('',(#21815),#16846,.F.) ;
#90136=ADVANCED_FACE('',(#21816),#79492,.T.) ;
#90137=ADVANCED_FACE('',(#21817),#15670,.F.) ;
#90138=ADVANCED_FACE('',(#21818),#15671,.F.) ;
#90139=ADVANCED_FACE('',(#21819),#15672,.F.) ;
#90140=ADVANCED_FACE('',(#21820),#15673,.F.) ;
#90141=ADVANCED_FACE('',(#21821),#16847,.F.) ;
#90142=ADVANCED_FACE('',(#21822),#16848,.F.) ;
#90143=ADVANCED_FACE('',(#21823),#15674,.F.) ;
#90144=ADVANCED_FACE('',(#21824),#15675,.T.) ;
#90145=ADVANCED_FACE('',(#21825),#15676,.T.) ;
#90146=ADVANCED_FACE('',(#21826),#15677,.T.) ;
#90147=ADVANCED_FACE('',(#21827),#16849,.T.) ;
#90148=ADVANCED_FACE('',(#21828),#16850,.T.) ;
#90149=ADVANCED_FACE('',(#21829),#15678,.T.) ;
#90150=ADVANCED_FACE('',(#21830),#15679,.T.) ;
#90151=ADVANCED_FACE('',(#21831),#15680,.T.) ;
#90152=ADVANCED_FACE('',(#21832),#15681,.T.) ;
#90153=ADVANCED_FACE('',(#21833),#16851,.T.) ;
#90154=ADVANCED_FACE('',(#21834),#16852,.T.) ;
#90155=ADVANCED_FACE('',(#21835),#15682,.T.) ;
#90156=ADVANCED_FACE('',(#21836),#15683,.T.) ;
#90157=ADVANCED_FACE('',(#21837),#16853,.T.) ;
#90158=ADVANCED_FACE('',(#21838),#16854,.T.) ;
#90159=ADVANCED_FACE('',(#21839),#15684,.T.) ;
#90160=ADVANCED_FACE('',(#21840),#15685,.T.) ;
#90161=ADVANCED_FACE('',(#21841),#16855,.T.) ;
#90162=ADVANCED_FACE('',(#21842),#16856,.T.) ;
#90163=ADVANCED_FACE('',(#21843),#15686,.T.) ;
#90164=ADVANCED_FACE('',(#21844),#15687,.T.) ;
#90165=ADVANCED_FACE('',(#21845),#15688,.F.) ;
#90166=ADVANCED_FACE('',(#21846),#15689,.F.) ;
#90167=ADVANCED_FACE('',(#21847),#15690,.T.) ;
#90168=ADVANCED_FACE('',(#21848),#16857,.T.) ;
#90169=ADVANCED_FACE('',(#21849),#15691,.T.) ;
#90170=ADVANCED_FACE('',(#21850),#15692,.T.) ;
#90171=ADVANCED_FACE('',(#21851),#79493,.T.) ;
#90172=ADVANCED_FACE('',(#21852),#15693,.T.) ;
#90173=ADVANCED_FACE('',(#21853),#16858,.T.) ;
#90174=ADVANCED_FACE('',(#21854),#79494,.F.) ;
#90175=ADVANCED_FACE('',(#21855),#16859,.T.) ;
#90176=ADVANCED_FACE('',(#21856),#15694,.T.) ;
#90177=ADVANCED_FACE('',(#21857),#15695,.T.) ;
#90178=ADVANCED_FACE('',(#21858),#15696,.F.) ;
#90179=ADVANCED_FACE('',(#21859),#79495,.F.) ;
#90180=ADVANCED_FACE('',(#21860),#15697,.T.) ;
#90181=ADVANCED_FACE('',(#21861),#15698,.T.) ;
#90182=ADVANCED_FACE('',(#21862),#15699,.T.) ;
#90183=ADVANCED_FACE('',(#21863),#79496,.T.) ;
#90184=ADVANCED_FACE('',(#21864),#79497,.F.) ;
#90185=ADVANCED_FACE('',(#21865),#16860,.T.) ;
#90186=ADVANCED_FACE('',(#21866),#15700,.F.) ;
#90187=ADVANCED_FACE('',(#21867),#15701,.T.) ;
#90188=ADVANCED_FACE('',(#21868),#15702,.F.) ;
#90189=ADVANCED_FACE('',(#21869),#15703,.T.) ;
#90190=ADVANCED_FACE('',(#21870),#16861,.F.) ;
#90191=ADVANCED_FACE('',(#21871),#16862,.T.) ;
#90192=ADVANCED_FACE('',(#21872),#79498,.T.) ;
#90193=ADVANCED_FACE('',(#21873),#15704,.F.) ;
#90194=ADVANCED_FACE('',(#21874),#15705,.T.) ;
#90195=ADVANCED_FACE('',(#21875),#15706,.T.) ;
#90196=ADVANCED_FACE('',(#21876),#15707,.T.) ;
#90197=ADVANCED_FACE('',(#21877),#79499,.F.) ;
#90198=ADVANCED_FACE('',(#21878),#16863,.T.) ;
#90199=ADVANCED_FACE('',(#21879),#15708,.F.) ;
#90200=ADVANCED_FACE('',(#21880),#15709,.T.) ;
#90201=ADVANCED_FACE('',(#21881),#15710,.F.) ;
#90202=ADVANCED_FACE('',(#21882),#15711,.F.) ;
#90203=ADVANCED_FACE('',(#21883),#79500,.F.) ;
#90204=ADVANCED_FACE('',(#21884),#16864,.F.) ;
#90205=ADVANCED_FACE('',(#21885),#15712,.F.) ;
#90206=ADVANCED_FACE('',(#21886),#174,.F.) ;
#90207=ADVANCED_FACE('',(#21887),#15713,.F.) ;
#90208=ADVANCED_FACE('',(#21888),#175,.F.) ;
#90209=ADVANCED_FACE('',(#21889),#16865,.F.) ;
#90210=ADVANCED_FACE('',(#21890),#176,.F.) ;
#90211=ADVANCED_FACE('',(#21891),#15714,.F.) ;
#90212=ADVANCED_FACE('',(#21892),#15715,.F.) ;
#90213=ADVANCED_FACE('',(#21893),#15716,.F.) ;
#90214=ADVANCED_FACE('',(#21894),#15717,.F.) ;
#90215=ADVANCED_FACE('',(#21895),#16866,.F.) ;
#90216=ADVANCED_FACE('',(#21896),#16867,.F.) ;
#90217=ADVANCED_FACE('',(#21897),#15718,.F.) ;
#90218=ADVANCED_FACE('',(#21898),#15719,.F.) ;
#90219=ADVANCED_FACE('',(#21899),#16868,.F.) ;
#90220=ADVANCED_FACE('',(#21900),#15720,.F.) ;
#90221=ADVANCED_FACE('',(#21901),#177,.F.) ;
#90222=ADVANCED_FACE('',(#21902),#178,.F.) ;
#90223=ADVANCED_FACE('',(#21903),#179,.F.) ;
#90224=ADVANCED_FACE('',(#21904),#15721,.F.) ;
#90225=ADVANCED_FACE('',(#21905),#15722,.F.) ;
#90226=ADVANCED_FACE('',(#21906),#16869,.F.) ;
#90227=ADVANCED_FACE('',(#21907),#15723,.F.) ;
#90228=ADVANCED_FACE('',(#21908),#15724,.F.) ;
#90229=ADVANCED_FACE('',(#21909),#16870,.F.) ;
#90230=ADVANCED_FACE('',(#21910),#15725,.F.) ;
#90231=ADVANCED_FACE('',(#21911),#180,.F.) ;
#90232=ADVANCED_FACE('',(#21912),#181,.F.) ;
#90233=ADVANCED_FACE('',(#21913),#182,.F.) ;
#90234=ADVANCED_FACE('',(#21914),#183,.F.) ;
#90235=ADVANCED_FACE('',(#21915),#15726,.F.) ;
#90236=ADVANCED_FACE('',(#21916),#15727,.F.) ;
#90237=ADVANCED_FACE('',(#21917),#16871,.F.) ;
#90238=ADVANCED_FACE('',(#21918),#15728,.F.) ;
#90239=ADVANCED_FACE('',(#21919),#15729,.F.) ;
#90240=ADVANCED_FACE('',(#21920),#16872,.F.) ;
#90241=ADVANCED_FACE('',(#21921),#15730,.F.) ;
#90242=ADVANCED_FACE('',(#21922),#184,.F.) ;
#90243=ADVANCED_FACE('',(#21923),#185,.F.) ;
#90244=ADVANCED_FACE('',(#21924),#79501,.F.) ;
#90245=ADVANCED_FACE('',(#21925),#15731,.F.) ;
#90246=ADVANCED_FACE('',(#21926),#15732,.F.) ;
#90247=ADVANCED_FACE('',(#21927),#79502,.F.) ;
#90248=ADVANCED_FACE('',(#21928),#79503,.F.) ;
#90249=ADVANCED_FACE('',(#21929),#15733,.F.) ;
#90250=ADVANCED_FACE('',(#21930),#15734,.F.) ;
#90251=ADVANCED_FACE('',(#21931),#79504,.F.) ;
#90252=ADVANCED_FACE('',(#21932),#15735,.T.) ;
#90253=ADVANCED_FACE('',(#21933),#15736,.T.) ;
#90254=ADVANCED_FACE('',(#21934),#15737,.T.) ;
#90255=ADVANCED_FACE('',(#21935),#16873,.T.) ;
#90256=ADVANCED_FACE('',(#21936),#16874,.T.) ;
#90257=ADVANCED_FACE('',(#21937),#15738,.T.) ;
#90258=ADVANCED_FACE('',(#21938),#15739,.T.) ;
#90259=ADVANCED_FACE('',(#21939),#15740,.T.) ;
#90260=ADVANCED_FACE('',(#21940),#15741,.T.) ;
#90261=ADVANCED_FACE('',(#21941),#16875,.T.) ;
#90262=ADVANCED_FACE('',(#21942),#16876,.T.) ;
#90263=ADVANCED_FACE('',(#21943),#15742,.T.) ;
#90264=ADVANCED_FACE('',(#21944),#15743,.T.) ;
#90265=ADVANCED_FACE('',(#21945),#79505,.T.) ;
#90266=ADVANCED_FACE('',(#21946),#79506,.T.) ;
#90267=ADVANCED_FACE('',(#21947),#15744,.T.) ;
#90268=ADVANCED_FACE('',(#21948),#15745,.F.) ;
#90269=ADVANCED_FACE('',(#21949),#15746,.F.) ;
#90270=ADVANCED_FACE('',(#21950),#15747,.F.) ;
#90271=ADVANCED_FACE('',(#21951),#15748,.T.) ;
#90272=ADVANCED_FACE('',(#21952),#15749,.T.) ;
#90273=ADVANCED_FACE('',(#21953),#79507,.T.) ;
#90274=ADVANCED_FACE('',(#21954),#16877,.F.) ;
#90275=ADVANCED_FACE('',(#21955),#16878,.F.) ;
#90276=ADVANCED_FACE('',(#21956),#79508,.T.) ;
#90277=ADVANCED_FACE('',(#21957),#15750,.F.) ;
#90278=ADVANCED_FACE('',(#21958),#15751,.F.) ;
#90279=ADVANCED_FACE('',(#21959),#15752,.F.) ;
#90280=ADVANCED_FACE('',(#21960),#15753,.F.) ;
#90281=ADVANCED_FACE('',(#21961),#16879,.F.) ;
#90282=ADVANCED_FACE('',(#21962),#16880,.F.) ;
#90283=ADVANCED_FACE('',(#21963),#15754,.F.) ;
#90284=ADVANCED_FACE('',(#21964),#15755,.T.) ;
#90285=ADVANCED_FACE('',(#21965),#15756,.T.) ;
#90286=ADVANCED_FACE('',(#21966),#15757,.T.) ;
#90287=ADVANCED_FACE('',(#21967),#16881,.T.) ;
#90288=ADVANCED_FACE('',(#21968),#16882,.T.) ;
#90289=ADVANCED_FACE('',(#21969),#15758,.T.) ;
#90290=ADVANCED_FACE('',(#21970),#15759,.T.) ;
#90291=ADVANCED_FACE('',(#21971),#15760,.T.) ;
#90292=ADVANCED_FACE('',(#21972),#15761,.T.) ;
#90293=ADVANCED_FACE('',(#21973),#16883,.T.) ;
#90294=ADVANCED_FACE('',(#21974),#16884,.T.) ;
#90295=ADVANCED_FACE('',(#21975),#15762,.T.) ;
#90296=ADVANCED_FACE('',(#21976),#15763,.T.) ;
#90297=ADVANCED_FACE('',(#21977),#16885,.T.) ;
#90298=ADVANCED_FACE('',(#21978),#16886,.T.) ;
#90299=ADVANCED_FACE('',(#21979),#15764,.T.) ;
#90300=ADVANCED_FACE('',(#21980),#15765,.T.) ;
#90301=ADVANCED_FACE('',(#21981),#16887,.T.) ;
#90302=ADVANCED_FACE('',(#21982),#16888,.T.) ;
#90303=ADVANCED_FACE('',(#21983),#15766,.T.) ;
#90304=ADVANCED_FACE('',(#21984),#15767,.T.) ;
#90305=ADVANCED_FACE('',(#21985),#15768,.F.) ;
#90306=ADVANCED_FACE('',(#21986),#15769,.F.) ;
#90307=ADVANCED_FACE('',(#21987),#15770,.T.) ;
#90308=ADVANCED_FACE('',(#21988),#16889,.T.) ;
#90309=ADVANCED_FACE('',(#21989),#15771,.T.) ;
#90310=ADVANCED_FACE('',(#21990),#15772,.T.) ;
#90311=ADVANCED_FACE('',(#21991),#79509,.T.) ;
#90312=ADVANCED_FACE('',(#21992),#15773,.T.) ;
#90313=ADVANCED_FACE('',(#21993),#16890,.T.) ;
#90314=ADVANCED_FACE('',(#21994),#79510,.F.) ;
#90315=ADVANCED_FACE('',(#21995),#16891,.T.) ;
#90316=ADVANCED_FACE('',(#21996),#15774,.T.) ;
#90317=ADVANCED_FACE('',(#21997),#15775,.T.) ;
#90318=ADVANCED_FACE('',(#21998),#15776,.F.) ;
#90319=ADVANCED_FACE('',(#21999),#79511,.F.) ;
#90320=ADVANCED_FACE('',(#22000),#15777,.T.) ;
#90321=ADVANCED_FACE('',(#22001),#15778,.T.) ;
#90322=ADVANCED_FACE('',(#22002),#15779,.T.) ;
#90323=ADVANCED_FACE('',(#22003),#79512,.T.) ;
#90324=ADVANCED_FACE('',(#22004),#79513,.F.) ;
#90325=ADVANCED_FACE('',(#22005),#16892,.T.) ;
#90326=ADVANCED_FACE('',(#22006),#15780,.F.) ;
#90327=ADVANCED_FACE('',(#22007),#15781,.T.) ;
#90328=ADVANCED_FACE('',(#22008),#15782,.F.) ;
#90329=ADVANCED_FACE('',(#22009),#15783,.T.) ;
#90330=ADVANCED_FACE('',(#22010),#16893,.F.) ;
#90331=ADVANCED_FACE('',(#22011),#16894,.T.) ;
#90332=ADVANCED_FACE('',(#22012),#79514,.T.) ;
#90333=ADVANCED_FACE('',(#22013),#15784,.F.) ;
#90334=ADVANCED_FACE('',(#22014),#15785,.T.) ;
#90335=ADVANCED_FACE('',(#22015),#15786,.T.) ;
#90336=ADVANCED_FACE('',(#22016),#15787,.T.) ;
#90337=ADVANCED_FACE('',(#22017),#79515,.F.) ;
#90338=ADVANCED_FACE('',(#22018),#16895,.T.) ;
#90339=ADVANCED_FACE('',(#22019),#15788,.F.) ;
#90340=ADVANCED_FACE('',(#22020),#15789,.T.) ;
#90341=ADVANCED_FACE('',(#22021),#15790,.F.) ;
#90342=ADVANCED_FACE('',(#22022),#15791,.F.) ;
#90343=ADVANCED_FACE('',(#22023),#79516,.F.) ;
#90344=ADVANCED_FACE('',(#22024),#16896,.F.) ;
#90345=ADVANCED_FACE('',(#22025),#15792,.F.) ;
#90346=ADVANCED_FACE('',(#22026),#186,.F.) ;
#90347=ADVANCED_FACE('',(#22027),#15793,.F.) ;
#90348=ADVANCED_FACE('',(#22028),#187,.F.) ;
#90349=ADVANCED_FACE('',(#22029),#16897,.F.) ;
#90350=ADVANCED_FACE('',(#22030),#188,.F.) ;
#90351=ADVANCED_FACE('',(#22031),#15794,.F.) ;
#90352=ADVANCED_FACE('',(#22032),#15795,.F.) ;
#90353=ADVANCED_FACE('',(#22033),#15796,.F.) ;
#90354=ADVANCED_FACE('',(#22034),#15797,.F.) ;
#90355=ADVANCED_FACE('',(#22035),#16898,.F.) ;
#90356=ADVANCED_FACE('',(#22036),#16899,.F.) ;
#90357=ADVANCED_FACE('',(#22037),#15798,.F.) ;
#90358=ADVANCED_FACE('',(#22038),#15799,.F.) ;
#90359=ADVANCED_FACE('',(#22039),#16900,.F.) ;
#90360=ADVANCED_FACE('',(#22040),#15800,.F.) ;
#90361=ADVANCED_FACE('',(#22041),#189,.F.) ;
#90362=ADVANCED_FACE('',(#22042),#190,.F.) ;
#90363=ADVANCED_FACE('',(#22043),#191,.F.) ;
#90364=ADVANCED_FACE('',(#22044),#15801,.F.) ;
#90365=ADVANCED_FACE('',(#22045),#15802,.F.) ;
#90366=ADVANCED_FACE('',(#22046),#16901,.F.) ;
#90367=ADVANCED_FACE('',(#22047),#15803,.F.) ;
#90368=ADVANCED_FACE('',(#22048),#15804,.F.) ;
#90369=ADVANCED_FACE('',(#22049),#16902,.F.) ;
#90370=ADVANCED_FACE('',(#22050),#15805,.F.) ;
#90371=ADVANCED_FACE('',(#22051),#192,.F.) ;
#90372=ADVANCED_FACE('',(#22052),#193,.F.) ;
#90373=ADVANCED_FACE('',(#22053),#194,.F.) ;
#90374=ADVANCED_FACE('',(#22054),#195,.F.) ;
#90375=ADVANCED_FACE('',(#22055),#15806,.F.) ;
#90376=ADVANCED_FACE('',(#22056),#15807,.F.) ;
#90377=ADVANCED_FACE('',(#22057),#16903,.F.) ;
#90378=ADVANCED_FACE('',(#22058),#15808,.F.) ;
#90379=ADVANCED_FACE('',(#22059),#15809,.F.) ;
#90380=ADVANCED_FACE('',(#22060),#16904,.F.) ;
#90381=ADVANCED_FACE('',(#22061),#15810,.F.) ;
#90382=ADVANCED_FACE('',(#22062),#196,.F.) ;
#90383=ADVANCED_FACE('',(#22063),#197,.F.) ;
#90384=ADVANCED_FACE('',(#22064),#79517,.F.) ;
#90385=ADVANCED_FACE('',(#22065),#15811,.F.) ;
#90386=ADVANCED_FACE('',(#22066),#15812,.F.) ;
#90387=ADVANCED_FACE('',(#22067),#79518,.F.) ;
#90388=ADVANCED_FACE('',(#22068),#79519,.F.) ;
#90389=ADVANCED_FACE('',(#22069),#15813,.F.) ;
#90390=ADVANCED_FACE('',(#22070),#15814,.F.) ;
#90391=ADVANCED_FACE('',(#22071),#79520,.F.) ;
#90392=ADVANCED_FACE('',(#22072),#15815,.T.) ;
#90393=ADVANCED_FACE('',(#22073),#15816,.T.) ;
#90394=ADVANCED_FACE('',(#22074),#15817,.T.) ;
#90395=ADVANCED_FACE('',(#22075),#16905,.T.) ;
#90396=ADVANCED_FACE('',(#22076),#16906,.T.) ;
#90397=ADVANCED_FACE('',(#22077),#15818,.T.) ;
#90398=ADVANCED_FACE('',(#22078),#15819,.T.) ;
#90399=ADVANCED_FACE('',(#22079),#15820,.T.) ;
#90400=ADVANCED_FACE('',(#22080),#15821,.T.) ;
#90401=ADVANCED_FACE('',(#22081),#16907,.T.) ;
#90402=ADVANCED_FACE('',(#22082),#16908,.T.) ;
#90403=ADVANCED_FACE('',(#22083),#15822,.T.) ;
#90404=ADVANCED_FACE('',(#22084),#15823,.T.) ;
#90405=ADVANCED_FACE('',(#22085),#79521,.T.) ;
#90406=ADVANCED_FACE('',(#22086),#79522,.T.) ;
#90407=ADVANCED_FACE('',(#22087),#15824,.T.) ;
#90408=ADVANCED_FACE('',(#22088),#15825,.F.) ;
#90409=ADVANCED_FACE('',(#22089),#15826,.F.) ;
#90410=ADVANCED_FACE('',(#22090),#15827,.F.) ;
#90411=ADVANCED_FACE('',(#22091),#15828,.T.) ;
#90412=ADVANCED_FACE('',(#22092),#15829,.T.) ;
#90413=ADVANCED_FACE('',(#22093),#79523,.T.) ;
#90414=ADVANCED_FACE('',(#22094),#16909,.F.) ;
#90415=ADVANCED_FACE('',(#22095),#16910,.F.) ;
#90416=ADVANCED_FACE('',(#22096),#79524,.T.) ;
#90417=ADVANCED_FACE('',(#22097),#15830,.F.) ;
#90418=ADVANCED_FACE('',(#22098),#15831,.F.) ;
#90419=ADVANCED_FACE('',(#22099),#15832,.F.) ;
#90420=ADVANCED_FACE('',(#22100),#15833,.F.) ;
#90421=ADVANCED_FACE('',(#22101),#16911,.F.) ;
#90422=ADVANCED_FACE('',(#22102),#16912,.F.) ;
#90423=ADVANCED_FACE('',(#22103),#15834,.F.) ;
#90424=ADVANCED_FACE('',(#22104),#15835,.T.) ;
#90425=ADVANCED_FACE('',(#22105),#15836,.T.) ;
#90426=ADVANCED_FACE('',(#22106),#15837,.T.) ;
#90427=ADVANCED_FACE('',(#22107),#16913,.T.) ;
#90428=ADVANCED_FACE('',(#22108),#16914,.T.) ;
#90429=ADVANCED_FACE('',(#22109),#15838,.T.) ;
#90430=ADVANCED_FACE('',(#22110),#15839,.T.) ;
#90431=ADVANCED_FACE('',(#22111),#15840,.T.) ;
#90432=ADVANCED_FACE('',(#22112),#15841,.T.) ;
#90433=ADVANCED_FACE('',(#22113),#16915,.T.) ;
#90434=ADVANCED_FACE('',(#22114),#16916,.T.) ;
#90435=ADVANCED_FACE('',(#22115),#15842,.T.) ;
#90436=ADVANCED_FACE('',(#22116),#15843,.T.) ;
#90437=ADVANCED_FACE('',(#22117),#16917,.T.) ;
#90438=ADVANCED_FACE('',(#22118),#16918,.T.) ;
#90439=ADVANCED_FACE('',(#22119),#15844,.T.) ;
#90440=ADVANCED_FACE('',(#22120),#15845,.T.) ;
#90441=ADVANCED_FACE('',(#22121),#16919,.T.) ;
#90442=ADVANCED_FACE('',(#22122),#16920,.T.) ;
#90443=ADVANCED_FACE('',(#22123),#15846,.T.) ;
#90444=ADVANCED_FACE('',(#22124),#15847,.T.) ;
#90445=ADVANCED_FACE('',(#22125),#15848,.F.) ;
#90446=ADVANCED_FACE('',(#22126),#15849,.F.) ;
#90447=ADVANCED_FACE('',(#22127),#15850,.T.) ;
#90448=ADVANCED_FACE('',(#22128),#16921,.T.) ;
#90449=ADVANCED_FACE('',(#22129),#15851,.T.) ;
#90450=ADVANCED_FACE('',(#22130),#15852,.T.) ;
#90451=ADVANCED_FACE('',(#22131),#79525,.T.) ;
#90452=ADVANCED_FACE('',(#22132),#15853,.T.) ;
#90453=ADVANCED_FACE('',(#22133),#16922,.T.) ;
#90454=ADVANCED_FACE('',(#22134),#79526,.F.) ;
#90455=ADVANCED_FACE('',(#22135),#16923,.T.) ;
#90456=ADVANCED_FACE('',(#22136),#15854,.T.) ;
#90457=ADVANCED_FACE('',(#22137),#15855,.T.) ;
#90458=ADVANCED_FACE('',(#22138),#15856,.F.) ;
#90459=ADVANCED_FACE('',(#22139),#79527,.F.) ;
#90460=ADVANCED_FACE('',(#22140),#15857,.T.) ;
#90461=ADVANCED_FACE('',(#22141),#15858,.T.) ;
#90462=ADVANCED_FACE('',(#22142),#15859,.T.) ;
#90463=ADVANCED_FACE('',(#22143),#79528,.T.) ;
#90464=ADVANCED_FACE('',(#22144),#79529,.F.) ;
#90465=ADVANCED_FACE('',(#22145),#16924,.T.) ;
#90466=ADVANCED_FACE('',(#22146),#15860,.F.) ;
#90467=ADVANCED_FACE('',(#22147),#15861,.T.) ;
#90468=ADVANCED_FACE('',(#22148),#15862,.F.) ;
#90469=ADVANCED_FACE('',(#22149),#15863,.T.) ;
#90470=ADVANCED_FACE('',(#22150),#16925,.F.) ;
#90471=ADVANCED_FACE('',(#22151),#16926,.T.) ;
#90472=ADVANCED_FACE('',(#22152),#79530,.T.) ;
#90473=ADVANCED_FACE('',(#22153),#15864,.F.) ;
#90474=ADVANCED_FACE('',(#22154),#15865,.T.) ;
#90475=ADVANCED_FACE('',(#22155),#15866,.T.) ;
#90476=ADVANCED_FACE('',(#22156),#15867,.T.) ;
#90477=ADVANCED_FACE('',(#22157),#79531,.F.) ;
#90478=ADVANCED_FACE('',(#22158),#16927,.T.) ;
#90479=ADVANCED_FACE('',(#22159),#15868,.F.) ;
#90480=ADVANCED_FACE('',(#22160),#15869,.T.) ;
#90481=ADVANCED_FACE('',(#22161),#15870,.F.) ;
#90482=ADVANCED_FACE('',(#22162),#15871,.F.) ;
#90483=ADVANCED_FACE('',(#22163),#79532,.F.) ;
#90484=ADVANCED_FACE('',(#22164),#16928,.F.) ;
#90485=ADVANCED_FACE('',(#22165),#15872,.F.) ;
#90486=ADVANCED_FACE('',(#22166),#198,.F.) ;
#90487=ADVANCED_FACE('',(#22167),#15873,.F.) ;
#90488=ADVANCED_FACE('',(#22168),#199,.F.) ;
#90489=ADVANCED_FACE('',(#22169),#16929,.F.) ;
#90490=ADVANCED_FACE('',(#22170),#200,.F.) ;
#90491=ADVANCED_FACE('',(#22171),#15874,.F.) ;
#90492=ADVANCED_FACE('',(#22172),#15875,.F.) ;
#90493=ADVANCED_FACE('',(#22173),#15876,.F.) ;
#90494=ADVANCED_FACE('',(#22174),#15877,.F.) ;
#90495=ADVANCED_FACE('',(#22175),#16930,.F.) ;
#90496=ADVANCED_FACE('',(#22176),#16931,.F.) ;
#90497=ADVANCED_FACE('',(#22177),#15878,.F.) ;
#90498=ADVANCED_FACE('',(#22178),#15879,.F.) ;
#90499=ADVANCED_FACE('',(#22179),#16932,.F.) ;
#90500=ADVANCED_FACE('',(#22180),#15880,.F.) ;
#90501=ADVANCED_FACE('',(#22181),#201,.F.) ;
#90502=ADVANCED_FACE('',(#22182),#202,.F.) ;
#90503=ADVANCED_FACE('',(#22183),#203,.F.) ;
#90504=ADVANCED_FACE('',(#22184),#15881,.F.) ;
#90505=ADVANCED_FACE('',(#22185),#15882,.F.) ;
#90506=ADVANCED_FACE('',(#22186),#16933,.F.) ;
#90507=ADVANCED_FACE('',(#22187),#15883,.F.) ;
#90508=ADVANCED_FACE('',(#22188),#15884,.F.) ;
#90509=ADVANCED_FACE('',(#22189),#16934,.F.) ;
#90510=ADVANCED_FACE('',(#22190),#15885,.F.) ;
#90511=ADVANCED_FACE('',(#22191),#204,.F.) ;
#90512=ADVANCED_FACE('',(#22192),#205,.F.) ;
#90513=ADVANCED_FACE('',(#22193),#206,.F.) ;
#90514=ADVANCED_FACE('',(#22194),#207,.F.) ;
#90515=ADVANCED_FACE('',(#22195),#15886,.F.) ;
#90516=ADVANCED_FACE('',(#22196),#15887,.F.) ;
#90517=ADVANCED_FACE('',(#22197),#16935,.F.) ;
#90518=ADVANCED_FACE('',(#22198),#15888,.F.) ;
#90519=ADVANCED_FACE('',(#22199),#15889,.F.) ;
#90520=ADVANCED_FACE('',(#22200),#16936,.F.) ;
#90521=ADVANCED_FACE('',(#22201),#15890,.F.) ;
#90522=ADVANCED_FACE('',(#22202),#208,.F.) ;
#90523=ADVANCED_FACE('',(#22203),#209,.F.) ;
#90524=ADVANCED_FACE('',(#22204),#79533,.F.) ;
#90525=ADVANCED_FACE('',(#22205),#15891,.F.) ;
#90526=ADVANCED_FACE('',(#22206),#15892,.F.) ;
#90527=ADVANCED_FACE('',(#22207),#79534,.F.) ;
#90528=ADVANCED_FACE('',(#22208),#79535,.F.) ;
#90529=ADVANCED_FACE('',(#22209),#15893,.F.) ;
#90530=ADVANCED_FACE('',(#22210),#15894,.F.) ;
#90531=ADVANCED_FACE('',(#22211),#79536,.F.) ;
#90532=ADVANCED_FACE('',(#22212),#15895,.T.) ;
#90533=ADVANCED_FACE('',(#22213),#15896,.T.) ;
#90534=ADVANCED_FACE('',(#22214),#15897,.T.) ;
#90535=ADVANCED_FACE('',(#22215),#16937,.T.) ;
#90536=ADVANCED_FACE('',(#22216),#16938,.T.) ;
#90537=ADVANCED_FACE('',(#22217),#15898,.T.) ;
#90538=ADVANCED_FACE('',(#22218),#15899,.T.) ;
#90539=ADVANCED_FACE('',(#22219),#15900,.T.) ;
#90540=ADVANCED_FACE('',(#22220),#15901,.T.) ;
#90541=ADVANCED_FACE('',(#22221),#16939,.T.) ;
#90542=ADVANCED_FACE('',(#22222),#16940,.T.) ;
#90543=ADVANCED_FACE('',(#22223),#15902,.T.) ;
#90544=ADVANCED_FACE('',(#22224),#15903,.T.) ;
#90545=ADVANCED_FACE('',(#22225),#79537,.T.) ;
#90546=ADVANCED_FACE('',(#22226),#79538,.T.) ;
#90547=ADVANCED_FACE('',(#22227),#15904,.T.) ;
#90548=ADVANCED_FACE('',(#22228),#15905,.F.) ;
#90549=ADVANCED_FACE('',(#22229),#15906,.F.) ;
#90550=ADVANCED_FACE('',(#22230),#15907,.F.) ;
#90551=ADVANCED_FACE('',(#22231),#15908,.T.) ;
#90552=ADVANCED_FACE('',(#22232),#15909,.T.) ;
#90553=ADVANCED_FACE('',(#22233),#79539,.T.) ;
#90554=ADVANCED_FACE('',(#22234),#16941,.F.) ;
#90555=ADVANCED_FACE('',(#22235),#16942,.F.) ;
#90556=ADVANCED_FACE('',(#22236),#79540,.T.) ;
#90557=ADVANCED_FACE('',(#22237),#15910,.F.) ;
#90558=ADVANCED_FACE('',(#22238),#15911,.F.) ;
#90559=ADVANCED_FACE('',(#22239),#15912,.F.) ;
#90560=ADVANCED_FACE('',(#22240),#15913,.F.) ;
#90561=ADVANCED_FACE('',(#22241),#16943,.F.) ;
#90562=ADVANCED_FACE('',(#22242),#16944,.F.) ;
#90563=ADVANCED_FACE('',(#22243),#15914,.F.) ;
#90564=ADVANCED_FACE('',(#22244),#15915,.T.) ;
#90565=ADVANCED_FACE('',(#22245),#15916,.T.) ;
#90566=ADVANCED_FACE('',(#22246),#15917,.T.) ;
#90567=ADVANCED_FACE('',(#22247),#16945,.T.) ;
#90568=ADVANCED_FACE('',(#22248),#16946,.T.) ;
#90569=ADVANCED_FACE('',(#22249),#15918,.T.) ;
#90570=ADVANCED_FACE('',(#22250),#15919,.T.) ;
#90571=ADVANCED_FACE('',(#22251),#15920,.T.) ;
#90572=ADVANCED_FACE('',(#22252),#15921,.T.) ;
#90573=ADVANCED_FACE('',(#22253),#16947,.T.) ;
#90574=ADVANCED_FACE('',(#22254),#16948,.T.) ;
#90575=ADVANCED_FACE('',(#22255),#15922,.T.) ;
#90576=ADVANCED_FACE('',(#22256),#15923,.T.) ;
#90577=ADVANCED_FACE('',(#22257),#16949,.T.) ;
#90578=ADVANCED_FACE('',(#22258),#16950,.T.) ;
#90579=ADVANCED_FACE('',(#22259),#15924,.T.) ;
#90580=ADVANCED_FACE('',(#22260),#15925,.T.) ;
#90581=ADVANCED_FACE('',(#22261),#16951,.T.) ;
#90582=ADVANCED_FACE('',(#22262),#16952,.T.) ;
#90583=ADVANCED_FACE('',(#22263),#15926,.T.) ;
#90584=ADVANCED_FACE('',(#22264),#15927,.T.) ;
#90585=ADVANCED_FACE('',(#22265),#15928,.F.) ;
#90586=ADVANCED_FACE('',(#22266),#15929,.F.) ;
#90587=ADVANCED_FACE('',(#22267),#15930,.T.) ;
#90588=ADVANCED_FACE('',(#22268),#16953,.T.) ;
#90589=ADVANCED_FACE('',(#22269),#15931,.T.) ;
#90590=ADVANCED_FACE('',(#22270),#15932,.T.) ;
#90591=ADVANCED_FACE('',(#22271),#79541,.T.) ;
#90592=ADVANCED_FACE('',(#22272),#15933,.T.) ;
#90593=ADVANCED_FACE('',(#22273),#16954,.T.) ;
#90594=ADVANCED_FACE('',(#22274),#79542,.F.) ;
#90595=ADVANCED_FACE('',(#22275),#16955,.T.) ;
#90596=ADVANCED_FACE('',(#22276),#15934,.T.) ;
#90597=ADVANCED_FACE('',(#22277),#15935,.T.) ;
#90598=ADVANCED_FACE('',(#22278),#15936,.F.) ;
#90599=ADVANCED_FACE('',(#22279),#79543,.F.) ;
#90600=ADVANCED_FACE('',(#22280),#15937,.T.) ;
#90601=ADVANCED_FACE('',(#22281),#15938,.T.) ;
#90602=ADVANCED_FACE('',(#22282),#15939,.T.) ;
#90603=ADVANCED_FACE('',(#22283),#79544,.T.) ;
#90604=ADVANCED_FACE('',(#22284),#79545,.F.) ;
#90605=ADVANCED_FACE('',(#22285),#16956,.T.) ;
#90606=ADVANCED_FACE('',(#22286),#15940,.F.) ;
#90607=ADVANCED_FACE('',(#22287),#15941,.T.) ;
#90608=ADVANCED_FACE('',(#22288),#15942,.F.) ;
#90609=ADVANCED_FACE('',(#22289),#15943,.T.) ;
#90610=ADVANCED_FACE('',(#22290),#16957,.F.) ;
#90611=ADVANCED_FACE('',(#22291),#16958,.T.) ;
#90612=ADVANCED_FACE('',(#22292),#79546,.T.) ;
#90613=ADVANCED_FACE('',(#22293),#15944,.F.) ;
#90614=ADVANCED_FACE('',(#22294),#15945,.T.) ;
#90615=ADVANCED_FACE('',(#22295),#15946,.T.) ;
#90616=ADVANCED_FACE('',(#22296),#15947,.T.) ;
#90617=ADVANCED_FACE('',(#22297),#79547,.F.) ;
#90618=ADVANCED_FACE('',(#22298),#16959,.T.) ;
#90619=ADVANCED_FACE('',(#22299),#15948,.F.) ;
#90620=ADVANCED_FACE('',(#22300),#15949,.T.) ;
#90621=ADVANCED_FACE('',(#22301),#15950,.F.) ;
#90622=ADVANCED_FACE('',(#22302),#15951,.F.) ;
#90623=ADVANCED_FACE('',(#22303),#79548,.F.) ;
#90624=ADVANCED_FACE('',(#22304),#16960,.F.) ;
#90625=ADVANCED_FACE('',(#22305),#15952,.F.) ;
#90626=ADVANCED_FACE('',(#22306),#210,.F.) ;
#90627=ADVANCED_FACE('',(#22307),#15953,.F.) ;
#90628=ADVANCED_FACE('',(#22308),#211,.F.) ;
#90629=ADVANCED_FACE('',(#22309),#16961,.F.) ;
#90630=ADVANCED_FACE('',(#22310),#212,.F.) ;
#90631=ADVANCED_FACE('',(#22311),#15954,.F.) ;
#90632=ADVANCED_FACE('',(#22312),#15955,.F.) ;
#90633=ADVANCED_FACE('',(#22313),#15956,.F.) ;
#90634=ADVANCED_FACE('',(#22314),#15957,.F.) ;
#90635=ADVANCED_FACE('',(#22315),#16962,.F.) ;
#90636=ADVANCED_FACE('',(#22316),#16963,.F.) ;
#90637=ADVANCED_FACE('',(#22317),#15958,.F.) ;
#90638=ADVANCED_FACE('',(#22318),#15959,.F.) ;
#90639=ADVANCED_FACE('',(#22319),#16964,.F.) ;
#90640=ADVANCED_FACE('',(#22320),#15960,.F.) ;
#90641=ADVANCED_FACE('',(#22321),#213,.F.) ;
#90642=ADVANCED_FACE('',(#22322),#214,.F.) ;
#90643=ADVANCED_FACE('',(#22323),#215,.F.) ;
#90644=ADVANCED_FACE('',(#22324),#15961,.F.) ;
#90645=ADVANCED_FACE('',(#22325),#15962,.F.) ;
#90646=ADVANCED_FACE('',(#22326),#16965,.F.) ;
#90647=ADVANCED_FACE('',(#22327),#15963,.F.) ;
#90648=ADVANCED_FACE('',(#22328),#15964,.F.) ;
#90649=ADVANCED_FACE('',(#22329),#16966,.F.) ;
#90650=ADVANCED_FACE('',(#22330),#15965,.F.) ;
#90651=ADVANCED_FACE('',(#22331),#216,.F.) ;
#90652=ADVANCED_FACE('',(#22332),#217,.F.) ;
#90653=ADVANCED_FACE('',(#22333),#218,.F.) ;
#90654=ADVANCED_FACE('',(#22334),#219,.F.) ;
#90655=ADVANCED_FACE('',(#22335),#15966,.F.) ;
#90656=ADVANCED_FACE('',(#22336),#15967,.F.) ;
#90657=ADVANCED_FACE('',(#22337),#16967,.F.) ;
#90658=ADVANCED_FACE('',(#22338),#15968,.F.) ;
#90659=ADVANCED_FACE('',(#22339),#15969,.F.) ;
#90660=ADVANCED_FACE('',(#22340),#16968,.F.) ;
#90661=ADVANCED_FACE('',(#22341),#15970,.F.) ;
#90662=ADVANCED_FACE('',(#22342),#220,.F.) ;
#90663=ADVANCED_FACE('',(#22343),#221,.F.) ;
#90664=ADVANCED_FACE('',(#22344),#79549,.F.) ;
#90665=ADVANCED_FACE('',(#22345),#15971,.F.) ;
#90666=ADVANCED_FACE('',(#22346),#15972,.F.) ;
#90667=ADVANCED_FACE('',(#22347),#79550,.F.) ;
#90668=ADVANCED_FACE('',(#22348),#79551,.F.) ;
#90669=ADVANCED_FACE('',(#22349),#15973,.F.) ;
#90670=ADVANCED_FACE('',(#22350),#15974,.F.) ;
#90671=ADVANCED_FACE('',(#22351),#79552,.F.) ;
#90672=ADVANCED_FACE('',(#22352),#15975,.T.) ;
#90673=ADVANCED_FACE('',(#22353),#15976,.T.) ;
#90674=ADVANCED_FACE('',(#22354),#15977,.T.) ;
#90675=ADVANCED_FACE('',(#22355),#16969,.T.) ;
#90676=ADVANCED_FACE('',(#22356),#16970,.T.) ;
#90677=ADVANCED_FACE('',(#22357),#15978,.T.) ;
#90678=ADVANCED_FACE('',(#22358),#15979,.T.) ;
#90679=ADVANCED_FACE('',(#22359),#15980,.T.) ;
#90680=ADVANCED_FACE('',(#22360),#15981,.T.) ;
#90681=ADVANCED_FACE('',(#22361),#16971,.T.) ;
#90682=ADVANCED_FACE('',(#22362),#16972,.T.) ;
#90683=ADVANCED_FACE('',(#22363),#15982,.T.) ;
#90684=ADVANCED_FACE('',(#22364),#15983,.T.) ;
#90685=ADVANCED_FACE('',(#22365),#79553,.T.) ;
#90686=ADVANCED_FACE('',(#22366),#79554,.T.) ;
#90687=ADVANCED_FACE('',(#22367),#15984,.T.) ;
#90688=ADVANCED_FACE('',(#22368),#15985,.F.) ;
#90689=ADVANCED_FACE('',(#22369),#15986,.F.) ;
#90690=ADVANCED_FACE('',(#22370),#15987,.F.) ;
#90691=ADVANCED_FACE('',(#22371),#15988,.T.) ;
#90692=ADVANCED_FACE('',(#22372),#15989,.T.) ;
#90693=ADVANCED_FACE('',(#22373),#79555,.T.) ;
#90694=ADVANCED_FACE('',(#22374),#16973,.F.) ;
#90695=ADVANCED_FACE('',(#22375),#16974,.F.) ;
#90696=ADVANCED_FACE('',(#22376),#79556,.T.) ;
#90697=ADVANCED_FACE('',(#22377),#15990,.F.) ;
#90698=ADVANCED_FACE('',(#22378),#15991,.F.) ;
#90699=ADVANCED_FACE('',(#22379),#15992,.F.) ;
#90700=ADVANCED_FACE('',(#22380),#15993,.F.) ;
#90701=ADVANCED_FACE('',(#22381),#16975,.F.) ;
#90702=ADVANCED_FACE('',(#22382),#16976,.F.) ;
#90703=ADVANCED_FACE('',(#22383),#15994,.F.) ;
#90704=ADVANCED_FACE('',(#22384),#15995,.T.) ;
#90705=ADVANCED_FACE('',(#22385),#15996,.T.) ;
#90706=ADVANCED_FACE('',(#22386),#15997,.T.) ;
#90707=ADVANCED_FACE('',(#22387),#16977,.T.) ;
#90708=ADVANCED_FACE('',(#22388),#16978,.T.) ;
#90709=ADVANCED_FACE('',(#22389),#15998,.T.) ;
#90710=ADVANCED_FACE('',(#22390),#15999,.T.) ;
#90711=ADVANCED_FACE('',(#22391),#16000,.T.) ;
#90712=ADVANCED_FACE('',(#22392),#16001,.T.) ;
#90713=ADVANCED_FACE('',(#22393),#16979,.T.) ;
#90714=ADVANCED_FACE('',(#22394),#16980,.T.) ;
#90715=ADVANCED_FACE('',(#22395),#16002,.T.) ;
#90716=ADVANCED_FACE('',(#22396),#16003,.T.) ;
#90717=ADVANCED_FACE('',(#22397),#16981,.T.) ;
#90718=ADVANCED_FACE('',(#22398),#16982,.T.) ;
#90719=ADVANCED_FACE('',(#22399),#16004,.T.) ;
#90720=ADVANCED_FACE('',(#22400),#16005,.T.) ;
#90721=ADVANCED_FACE('',(#22401),#16983,.T.) ;
#90722=ADVANCED_FACE('',(#22402),#16984,.T.) ;
#90723=ADVANCED_FACE('',(#22403),#16006,.T.) ;
#90724=ADVANCED_FACE('',(#22404),#16007,.T.) ;
#90725=ADVANCED_FACE('',(#22405),#16008,.F.) ;
#90726=ADVANCED_FACE('',(#22406),#16009,.F.) ;
#90727=ADVANCED_FACE('',(#22407),#16010,.T.) ;
#90728=ADVANCED_FACE('',(#22408),#16985,.T.) ;
#90729=ADVANCED_FACE('',(#22409),#16011,.T.) ;
#90730=ADVANCED_FACE('',(#22410),#16012,.T.) ;
#90731=ADVANCED_FACE('',(#22411),#79557,.T.) ;
#90732=ADVANCED_FACE('',(#22412),#16013,.T.) ;
#90733=ADVANCED_FACE('',(#22413),#16986,.T.) ;
#90734=ADVANCED_FACE('',(#22414),#79558,.F.) ;
#90735=ADVANCED_FACE('',(#22415),#16987,.T.) ;
#90736=ADVANCED_FACE('',(#22416),#16014,.T.) ;
#90737=ADVANCED_FACE('',(#22417),#16015,.T.) ;
#90738=ADVANCED_FACE('',(#22418),#16016,.F.) ;
#90739=ADVANCED_FACE('',(#22419),#79559,.F.) ;
#90740=ADVANCED_FACE('',(#22420),#16017,.T.) ;
#90741=ADVANCED_FACE('',(#22421),#16018,.T.) ;
#90742=ADVANCED_FACE('',(#22422),#16019,.T.) ;
#90743=ADVANCED_FACE('',(#22423),#79560,.T.) ;
#90744=ADVANCED_FACE('',(#22424),#79561,.F.) ;
#90745=ADVANCED_FACE('',(#22425),#16988,.T.) ;
#90746=ADVANCED_FACE('',(#22426),#16020,.F.) ;
#90747=ADVANCED_FACE('',(#22427),#16021,.T.) ;
#90748=ADVANCED_FACE('',(#22428),#16022,.F.) ;
#90749=ADVANCED_FACE('',(#22429),#16023,.T.) ;
#90750=ADVANCED_FACE('',(#22430),#16989,.F.) ;
#90751=ADVANCED_FACE('',(#22431),#16990,.T.) ;
#90752=ADVANCED_FACE('',(#22432),#79562,.T.) ;
#90753=ADVANCED_FACE('',(#22433),#16024,.F.) ;
#90754=ADVANCED_FACE('',(#22434),#16025,.T.) ;
#90755=ADVANCED_FACE('',(#22435),#16026,.T.) ;
#90756=ADVANCED_FACE('',(#22436),#16027,.T.) ;
#90757=ADVANCED_FACE('',(#22437),#79563,.F.) ;
#90758=ADVANCED_FACE('',(#22438),#16991,.T.) ;
#90759=ADVANCED_FACE('',(#22439),#16028,.F.) ;
#90760=ADVANCED_FACE('',(#22440),#16029,.T.) ;
#90761=ADVANCED_FACE('',(#22441),#16030,.F.) ;
#90762=ADVANCED_FACE('',(#22442),#16031,.F.) ;
#90763=ADVANCED_FACE('',(#22443),#79564,.F.) ;
#90764=ADVANCED_FACE('',(#22444),#16992,.F.) ;
#90765=ADVANCED_FACE('',(#22445),#16032,.F.) ;
#90766=ADVANCED_FACE('',(#22446),#222,.F.) ;
#90767=ADVANCED_FACE('',(#22447),#16033,.F.) ;
#90768=ADVANCED_FACE('',(#22448),#223,.F.) ;
#90769=ADVANCED_FACE('',(#22449),#16993,.F.) ;
#90770=ADVANCED_FACE('',(#22450),#224,.F.) ;
#90771=ADVANCED_FACE('',(#22451),#16034,.F.) ;
#90772=ADVANCED_FACE('',(#22452),#16035,.F.) ;
#90773=ADVANCED_FACE('',(#22453),#16036,.F.) ;
#90774=ADVANCED_FACE('',(#22454),#16037,.F.) ;
#90775=ADVANCED_FACE('',(#22455),#16994,.F.) ;
#90776=ADVANCED_FACE('',(#22456),#16995,.F.) ;
#90777=ADVANCED_FACE('',(#22457),#16038,.F.) ;
#90778=ADVANCED_FACE('',(#22458),#16039,.F.) ;
#90779=ADVANCED_FACE('',(#22459),#16996,.F.) ;
#90780=ADVANCED_FACE('',(#22460),#16040,.F.) ;
#90781=ADVANCED_FACE('',(#22461),#225,.F.) ;
#90782=ADVANCED_FACE('',(#22462),#226,.F.) ;
#90783=ADVANCED_FACE('',(#22463),#227,.F.) ;
#90784=ADVANCED_FACE('',(#22464),#16041,.F.) ;
#90785=ADVANCED_FACE('',(#22465),#16042,.F.) ;
#90786=ADVANCED_FACE('',(#22466),#16997,.F.) ;
#90787=ADVANCED_FACE('',(#22467),#16043,.F.) ;
#90788=ADVANCED_FACE('',(#22468),#16044,.F.) ;
#90789=ADVANCED_FACE('',(#22469),#16998,.F.) ;
#90790=ADVANCED_FACE('',(#22470),#16045,.F.) ;
#90791=ADVANCED_FACE('',(#22471),#228,.F.) ;
#90792=ADVANCED_FACE('',(#22472),#229,.F.) ;
#90793=ADVANCED_FACE('',(#22473),#230,.F.) ;
#90794=ADVANCED_FACE('',(#22474),#231,.F.) ;
#90795=ADVANCED_FACE('',(#22475),#16046,.F.) ;
#90796=ADVANCED_FACE('',(#22476),#16047,.F.) ;
#90797=ADVANCED_FACE('',(#22477),#16999,.F.) ;
#90798=ADVANCED_FACE('',(#22478),#16048,.F.) ;
#90799=ADVANCED_FACE('',(#22479),#16049,.F.) ;
#90800=ADVANCED_FACE('',(#22480),#17000,.F.) ;
#90801=ADVANCED_FACE('',(#22481),#16050,.F.) ;
#90802=ADVANCED_FACE('',(#22482),#232,.F.) ;
#90803=ADVANCED_FACE('',(#22483),#233,.F.) ;
#90804=ADVANCED_FACE('',(#22484),#79565,.F.) ;
#90805=ADVANCED_FACE('',(#22485),#16051,.F.) ;
#90806=ADVANCED_FACE('',(#22486),#16052,.F.) ;
#90807=ADVANCED_FACE('',(#22487),#79566,.F.) ;
#90808=ADVANCED_FACE('',(#22488),#79567,.F.) ;
#90809=ADVANCED_FACE('',(#22489),#16053,.F.) ;
#90810=ADVANCED_FACE('',(#22490),#16054,.F.) ;
#90811=ADVANCED_FACE('',(#22491),#79568,.F.) ;
#90812=ADVANCED_FACE('',(#22492),#16055,.T.) ;
#90813=ADVANCED_FACE('',(#22493),#16056,.T.) ;
#90814=ADVANCED_FACE('',(#22494),#16057,.T.) ;
#90815=ADVANCED_FACE('',(#22495),#17001,.T.) ;
#90816=ADVANCED_FACE('',(#22496),#17002,.T.) ;
#90817=ADVANCED_FACE('',(#22497),#16058,.T.) ;
#90818=ADVANCED_FACE('',(#22498),#16059,.T.) ;
#90819=ADVANCED_FACE('',(#22499),#16060,.T.) ;
#90820=ADVANCED_FACE('',(#22500),#16061,.T.) ;
#90821=ADVANCED_FACE('',(#22501),#17003,.T.) ;
#90822=ADVANCED_FACE('',(#22502),#17004,.T.) ;
#90823=ADVANCED_FACE('',(#22503),#16062,.T.) ;
#90824=ADVANCED_FACE('',(#22504),#16063,.T.) ;
#90825=ADVANCED_FACE('',(#22505),#79569,.T.) ;
#90826=ADVANCED_FACE('',(#22506),#79570,.T.) ;
#90827=ADVANCED_FACE('',(#22507),#16064,.T.) ;
#90828=ADVANCED_FACE('',(#22508),#16065,.F.) ;
#90829=ADVANCED_FACE('',(#22509),#16066,.F.) ;
#90830=ADVANCED_FACE('',(#22510),#16067,.F.) ;
#90831=ADVANCED_FACE('',(#22511),#16068,.T.) ;
#90832=ADVANCED_FACE('',(#22512),#16069,.T.) ;
#90833=ADVANCED_FACE('',(#22513),#79571,.T.) ;
#90834=ADVANCED_FACE('',(#22514),#17005,.F.) ;
#90835=ADVANCED_FACE('',(#22515),#17006,.F.) ;
#90836=ADVANCED_FACE('',(#22516),#79572,.T.) ;
#90837=ADVANCED_FACE('',(#22517),#16070,.F.) ;
#90838=ADVANCED_FACE('',(#22518),#16071,.F.) ;
#90839=ADVANCED_FACE('',(#22519),#16072,.F.) ;
#90840=ADVANCED_FACE('',(#22520),#16073,.F.) ;
#90841=ADVANCED_FACE('',(#22521),#17007,.F.) ;
#90842=ADVANCED_FACE('',(#22522),#17008,.F.) ;
#90843=ADVANCED_FACE('',(#22523),#16074,.F.) ;
#90844=ADVANCED_FACE('',(#22524),#16075,.T.) ;
#90845=ADVANCED_FACE('',(#22525),#16076,.T.) ;
#90846=ADVANCED_FACE('',(#22526),#16077,.T.) ;
#90847=ADVANCED_FACE('',(#22527),#17009,.T.) ;
#90848=ADVANCED_FACE('',(#22528),#17010,.T.) ;
#90849=ADVANCED_FACE('',(#22529),#16078,.T.) ;
#90850=ADVANCED_FACE('',(#22530),#16079,.T.) ;
#90851=ADVANCED_FACE('',(#22531),#16080,.T.) ;
#90852=ADVANCED_FACE('',(#22532),#16081,.T.) ;
#90853=ADVANCED_FACE('',(#22533),#17011,.T.) ;
#90854=ADVANCED_FACE('',(#22534),#17012,.T.) ;
#90855=ADVANCED_FACE('',(#22535),#16082,.T.) ;
#90856=ADVANCED_FACE('',(#22536),#16083,.T.) ;
#90857=ADVANCED_FACE('',(#22537),#17013,.T.) ;
#90858=ADVANCED_FACE('',(#22538),#17014,.T.) ;
#90859=ADVANCED_FACE('',(#22539),#16084,.T.) ;
#90860=ADVANCED_FACE('',(#22540),#16085,.T.) ;
#90861=ADVANCED_FACE('',(#22541),#17015,.T.) ;
#90862=ADVANCED_FACE('',(#22542),#17016,.T.) ;
#90863=ADVANCED_FACE('',(#22543),#16086,.T.) ;
#90864=ADVANCED_FACE('',(#22544),#16087,.T.) ;
#90865=ADVANCED_FACE('',(#22545),#16088,.F.) ;
#90866=ADVANCED_FACE('',(#22546),#16089,.F.) ;
#90867=ADVANCED_FACE('',(#22547),#16090,.T.) ;
#90868=ADVANCED_FACE('',(#22548),#16091,.F.) ;
#90869=ADVANCED_FACE('',(#22549),#16092,.F.) ;
#90870=ADVANCED_FACE('',(#22550),#16093,.F.) ;
#90871=ADVANCED_FACE('',(#22551),#16094,.F.) ;
#90872=ADVANCED_FACE('',(#22552),#16095,.F.) ;
#90873=ADVANCED_FACE('',(#22553),#16096,.F.) ;
#90874=ADVANCED_FACE('',(#22554),#16097,.F.) ;
#90875=ADVANCED_FACE('',(#22555),#16098,.F.) ;
#90876=ADVANCED_FACE('',(#22556),#16099,.F.) ;
#90877=ADVANCED_FACE('',(#22557),#79573,.T.) ;
#90878=ADVANCED_FACE('',(#22558),#16100,.T.) ;
#90879=ADVANCED_FACE('',(#22559),#79574,.T.) ;
#90880=ADVANCED_FACE('',(#22560),#79575,.T.) ;
#90881=ADVANCED_FACE('',(#22561),#79576,.T.) ;
#90882=ADVANCED_FACE('',(#22562),#16101,.T.) ;
#90883=ADVANCED_FACE('',(#22563),#79577,.T.) ;
#90884=ADVANCED_FACE('',(#22564),#79578,.T.) ;
#90885=ADVANCED_FACE('',(#22565),#16102,.T.) ;
#90886=ADVANCED_FACE('',(#22566),#79579,.T.) ;
#90887=ADVANCED_FACE('',(#22567),#79580,.T.) ;
#90888=ADVANCED_FACE('',(#22568),#16103,.T.) ;
#90889=ADVANCED_FACE('',(#22569),#79581,.T.) ;
#90890=ADVANCED_FACE('',(#22570),#79582,.T.) ;
#90891=ADVANCED_FACE('',(#22571),#16104,.T.) ;
#90892=ADVANCED_FACE('',(#22572),#79583,.T.) ;
#90893=ADVANCED_FACE('',(#22573),#79584,.T.) ;
#90894=ADVANCED_FACE('',(#22574),#16105,.T.) ;
#90895=ADVANCED_FACE('',(#22575),#79585,.T.) ;
#90896=ADVANCED_FACE('',(#22576),#79586,.T.) ;
#90897=ADVANCED_FACE('',(#22577),#16106,.T.) ;
#90898=ADVANCED_FACE('',(#22578),#79587,.T.) ;
#90899=ADVANCED_FACE('',(#22579),#79588,.T.) ;
#90900=ADVANCED_FACE('',(#22580),#16107,.T.) ;
#90901=ADVANCED_FACE('',(#22581),#79589,.T.) ;
#90902=ADVANCED_FACE('',(#22582),#16108,.T.) ;
#90903=ADVANCED_FACE('',(#22583),#79590,.T.) ;
#90904=ADVANCED_FACE('',(#22584),#79591,.T.) ;
#90905=ADVANCED_FACE('',(#22585),#16109,.T.) ;
#90906=ADVANCED_FACE('',(#22586),#17017,.T.) ;
#90907=ADVANCED_FACE('',(#22587),#79592,.T.) ;
#90908=ADVANCED_FACE('',(#22588),#16110,.T.) ;
#90909=ADVANCED_FACE('',(#22589),#17018,.T.) ;
#90910=ADVANCED_FACE('',(#22590),#79593,.T.) ;
#90911=ADVANCED_FACE('',(#22591),#16111,.T.) ;
#90912=ADVANCED_FACE('',(#22592),#17019,.T.) ;
#90913=ADVANCED_FACE('',(#22593),#79594,.T.) ;
#90914=ADVANCED_FACE('',(#22594),#16112,.T.) ;
#90915=ADVANCED_FACE('',(#22595),#17020,.T.) ;
#90916=ADVANCED_FACE('',(#22596),#79595,.T.) ;
#90917=ADVANCED_FACE('',(#22597),#16113,.T.) ;
#90918=ADVANCED_FACE('',(#22598),#17021,.T.) ;
#90919=ADVANCED_FACE('',(#22599),#79596,.T.) ;
#90920=ADVANCED_FACE('',(#22600),#16114,.T.) ;
#90921=ADVANCED_FACE('',(#22601),#17022,.T.) ;
#90922=ADVANCED_FACE('',(#22602),#79597,.T.) ;
#90923=ADVANCED_FACE('',(#22603),#16115,.T.) ;
#90924=ADVANCED_FACE('',(#22604),#17023,.T.) ;
#90925=ADVANCED_FACE('',(#22605),#79598,.T.) ;
#90926=ADVANCED_FACE('',(#22606),#16116,.T.) ;
#90927=ADVANCED_FACE('',(#22607),#17024,.T.) ;
#90928=ADVANCED_FACE('',(#22608),#79599,.T.) ;
#90929=ADVANCED_FACE('',(#22609),#16117,.T.) ;
#90930=ADVANCED_FACE('',(#22610),#17025,.T.) ;
#90931=ADVANCED_FACE('',(#22611),#79600,.T.) ;
#90932=ADVANCED_FACE('',(#22612),#16118,.T.) ;
#90933=ADVANCED_FACE('',(#22613),#17026,.T.) ;
#90934=ADVANCED_FACE('',(#22614),#79601,.T.) ;
#90935=ADVANCED_FACE('',(#22615),#16119,.T.) ;
#90936=ADVANCED_FACE('',(#22616),#17027,.T.) ;
#90937=ADVANCED_FACE('',(#22617),#79602,.T.) ;
#90938=ADVANCED_FACE('',(#22618),#16120,.T.) ;
#90939=ADVANCED_FACE('',(#22619),#17028,.T.) ;
#90940=ADVANCED_FACE('',(#22620),#79603,.T.) ;
#90941=ADVANCED_FACE('',(#22621),#16121,.T.) ;
#90942=ADVANCED_FACE('',(#22622),#17029,.T.) ;
#90943=ADVANCED_FACE('',(#22623),#79604,.T.) ;
#90944=ADVANCED_FACE('',(#22624),#16122,.T.) ;
#90945=ADVANCED_FACE('',(#22625),#17030,.T.) ;
#90946=ADVANCED_FACE('',(#22626),#79605,.T.) ;
#90947=ADVANCED_FACE('',(#22627),#16123,.T.) ;
#90948=ADVANCED_FACE('',(#22628),#17031,.T.) ;
#90949=ADVANCED_FACE('',(#22629),#79606,.T.) ;
#90950=ADVANCED_FACE('',(#22630),#16124,.T.) ;
#90951=ADVANCED_FACE('',(#22631),#17032,.T.) ;
#90952=ADVANCED_FACE('',(#22632),#79607,.T.) ;
#90953=ADVANCED_FACE('',(#22633),#16125,.T.) ;
#90954=ADVANCED_FACE('',(#22634),#17033,.T.) ;
#90955=ADVANCED_FACE('',(#22635),#79608,.T.) ;
#90956=ADVANCED_FACE('',(#22636),#16126,.T.) ;
#90957=ADVANCED_FACE('',(#22637),#17034,.T.) ;
#90958=ADVANCED_FACE('',(#22638),#79609,.F.) ;
#90959=ADVANCED_FACE('',(#22639),#234,.F.) ;
#90960=ADVANCED_FACE('',(#22640),#79610,.F.) ;
#90961=ADVANCED_FACE('',(#22641),#79611,.F.) ;
#90962=ADVANCED_FACE('',(#22642),#235,.F.) ;
#90963=ADVANCED_FACE('',(#22643),#79612,.F.) ;
#90964=ADVANCED_FACE('',(#22644),#79613,.F.) ;
#90965=ADVANCED_FACE('',(#22645),#236,.F.) ;
#90966=ADVANCED_FACE('',(#22646),#79614,.F.) ;
#90967=ADVANCED_FACE('',(#22647),#79615,.F.) ;
#90968=ADVANCED_FACE('',(#22648),#237,.F.) ;
#90969=ADVANCED_FACE('',(#22649),#79616,.F.) ;
#90970=ADVANCED_FACE('',(#22650),#79617,.F.) ;
#90971=ADVANCED_FACE('',(#22651),#238,.F.) ;
#90972=ADVANCED_FACE('',(#22652),#79618,.F.) ;
#90973=ADVANCED_FACE('',(#22653),#79619,.F.) ;
#90974=ADVANCED_FACE('',(#22654),#239,.F.) ;
#90975=ADVANCED_FACE('',(#22655),#79620,.F.) ;
#90976=ADVANCED_FACE('',(#22656),#79621,.F.) ;
#90977=ADVANCED_FACE('',(#22657),#240,.F.) ;
#90978=ADVANCED_FACE('',(#22658),#79622,.F.) ;
#90979=ADVANCED_FACE('',(#22659),#79623,.F.) ;
#90980=ADVANCED_FACE('',(#22660),#241,.F.) ;
#90981=ADVANCED_FACE('',(#22661),#79624,.F.) ;
#90982=ADVANCED_FACE('',(#22662),#79625,.F.) ;
#90983=ADVANCED_FACE('',(#22663),#242,.F.) ;
#90984=ADVANCED_FACE('',(#22664),#79626,.F.) ;
#90985=ADVANCED_FACE('',(#22665),#79627,.F.) ;
#90986=ADVANCED_FACE('',(#22666),#243,.F.) ;
#90987=ADVANCED_FACE('',(#22667),#79628,.F.) ;
#90988=ADVANCED_FACE('',(#22668),#79629,.F.) ;
#90989=ADVANCED_FACE('',(#22669),#244,.F.) ;
#90990=ADVANCED_FACE('',(#22670),#79630,.F.) ;
#90991=ADVANCED_FACE('',(#22671),#79631,.F.) ;
#90992=ADVANCED_FACE('',(#22672),#245,.F.) ;
#90993=ADVANCED_FACE('',(#22673),#79632,.F.) ;
#90994=ADVANCED_FACE('',(#22674),#79633,.F.) ;
#90995=ADVANCED_FACE('',(#22675),#246,.F.) ;
#90996=ADVANCED_FACE('',(#22676),#79634,.F.) ;
#90997=ADVANCED_FACE('',(#22677),#79635,.F.) ;
#90998=ADVANCED_FACE('',(#22678),#247,.F.) ;
#90999=ADVANCED_FACE('',(#22679),#79636,.F.) ;
#91000=ADVANCED_FACE('',(#22680),#79637,.F.) ;
#91001=ADVANCED_FACE('',(#22681),#248,.F.) ;
#91002=ADVANCED_FACE('',(#22682),#79638,.F.) ;
#91003=ADVANCED_FACE('',(#22683),#79639,.F.) ;
#91004=ADVANCED_FACE('',(#22684),#249,.F.) ;
#91005=ADVANCED_FACE('',(#22685),#79640,.F.) ;
#91006=ADVANCED_FACE('',(#22686),#79641,.F.) ;
#91007=ADVANCED_FACE('',(#22687),#250,.F.) ;
#91008=ADVANCED_FACE('',(#22688),#79642,.F.) ;
#91009=ADVANCED_FACE('',(#22689),#79643,.F.) ;
#91010=ADVANCED_FACE('',(#22690),#251,.F.) ;
#91011=ADVANCED_FACE('',(#22691),#79644,.F.) ;
#91012=ADVANCED_FACE('',(#22692),#16127,.T.) ;
#91013=ADVANCED_FACE('',(#22693),#16128,.T.) ;
#91014=ADVANCED_FACE('',(#22694),#16129,.T.) ;
#91015=ADVANCED_FACE('',(#22695),#16130,.T.) ;
#91016=ADVANCED_FACE('',(#22696),#16131,.T.) ;
#91017=ADVANCED_FACE('',(#22697),#16132,.T.) ;
#91018=ADVANCED_FACE('',(#22698),#17035,.T.) ;
#91019=ADVANCED_FACE('',(#22699),#16133,.T.) ;
#91020=ADVANCED_FACE('',(#22700),#79645,.T.) ;
#91021=ADVANCED_FACE('',(#22701),#16134,.T.) ;
#91022=ADVANCED_FACE('',(#22702),#17036,.T.) ;
#91023=ADVANCED_FACE('',(#22703),#16135,.T.) ;
#91024=ADVANCED_FACE('',(#22704),#17037,.T.) ;
#91025=ADVANCED_FACE('',(#22705),#16136,.T.) ;
#91026=ADVANCED_FACE('',(#22706),#17038,.T.) ;
#91027=ADVANCED_FACE('',(#22707),#79646,.T.) ;
#91028=ADVANCED_FACE('',(#22708),#16137,.T.) ;
#91029=ADVANCED_FACE('',(#22709),#16138,.T.) ;
#91030=ADVANCED_FACE('',(#22710),#16139,.F.) ;
#91031=ADVANCED_FACE('',(#22711),#17039,.T.) ;
#91032=ADVANCED_FACE('',(#22712),#79647,.F.) ;
#91033=ADVANCED_FACE('',(#22713),#16140,.T.) ;
#91034=ADVANCED_FACE('',(#22714),#16141,.T.) ;
#91035=ADVANCED_FACE('',(#22715),#16142,.F.) ;
#91036=ADVANCED_FACE('',(#22716),#17040,.T.) ;
#91037=ADVANCED_FACE('',(#22717),#252,.F.) ;
#91038=ADVANCED_FACE('',(#22718),#16143,.T.) ;
#91039=ADVANCED_FACE('',(#22719),#253,.F.) ;
#91040=ADVANCED_FACE('',(#22720),#79648,.T.) ;
#91041=ADVANCED_FACE('',(#22721),#254,.F.) ;
#91042=ADVANCED_FACE('',(#22722),#79649,.T.) ;
#91043=ADVANCED_FACE('',(#22723),#255,.F.) ;
#91044=ADVANCED_FACE('',(#22724),#79650,.T.) ;
#91045=ADVANCED_FACE('',(#22725),#256,.F.) ;
#91046=ADVANCED_FACE('',(#22726),#79651,.T.) ;
#91047=ADVANCED_FACE('',(#22727),#257,.F.) ;
#91048=ADVANCED_FACE('',(#22728),#79652,.T.) ;
#91049=ADVANCED_FACE('',(#22729),#258,.F.) ;
#91050=ADVANCED_FACE('',(#22730),#79653,.T.) ;
#91051=ADVANCED_FACE('',(#22731),#259,.F.) ;
#91052=ADVANCED_FACE('',(#22732),#79654,.T.) ;
#91053=ADVANCED_FACE('',(#22733),#260,.F.) ;
#91054=ADVANCED_FACE('',(#22734),#17041,.T.) ;
#91055=ADVANCED_FACE('',(#22735),#79655,.T.) ;
#91056=ADVANCED_FACE('',(#22736),#16144,.T.) ;
#91057=ADVANCED_FACE('',(#22737),#261,.F.) ;
#91058=ADVANCED_FACE('',(#22738),#79656,.T.) ;
#91059=ADVANCED_FACE('',(#22739),#79657,.T.) ;
#91060=ADVANCED_FACE('',(#22740),#16145,.T.) ;
#91061=ADVANCED_FACE('',(#22741),#262,.F.) ;
#91062=ADVANCED_FACE('',(#22742),#17042,.T.) ;
#91063=ADVANCED_FACE('',(#22743),#79658,.T.) ;
#91064=ADVANCED_FACE('',(#22744),#16146,.F.) ;
#91065=ADVANCED_FACE('',(#22745),#16147,.T.) ;
#91066=ADVANCED_FACE('',(#22746),#79659,.F.) ;
#91067=ADVANCED_FACE('',(#22747),#17043,.T.) ;
#91068=ADVANCED_FACE('',(#22748),#16148,.T.) ;
#91069=ADVANCED_FACE('',(#22749),#16149,.T.) ;
#91070=ADVANCED_FACE('',(#22750),#16150,.F.) ;
#91071=ADVANCED_FACE('',(#22751),#16151,.T.) ;
#91072=ADVANCED_FACE('',(#22752),#17044,.T.) ;
#91073=ADVANCED_FACE('',(#22753),#79660,.T.) ;
#91074=ADVANCED_FACE('',(#22754),#16152,.T.) ;
#91075=ADVANCED_FACE('',(#22755),#16153,.T.) ;
#91076=ADVANCED_FACE('',(#22756),#17045,.T.) ;
#91077=ADVANCED_FACE('',(#22757),#16154,.T.) ;
#91078=ADVANCED_FACE('',(#22758),#17046,.T.) ;
#91079=ADVANCED_FACE('',(#22759),#263,.F.) ;
#91080=ADVANCED_FACE('',(#22760),#264,.F.) ;
#91081=ADVANCED_FACE('',(#22761),#265,.F.) ;
#91082=ADVANCED_FACE('',(#22762),#266,.F.) ;
#91087=CLOSED_SHELL('',(#88718,#88719,#88720,#88721,#88722,#88723,#88724,
#88725,#88726,#88727,#88728,#88729,#88730,#88731,#88732,#88733,#88734,#88735,
#88736,#88737,#88738,#88739,#88740,#88741,#88742,#88743,#88744,#88745,#88746,
#88747,#88748,#88749,#88750,#88751,#88752,#88753,#88754,#88755,#88756,#88757,
#88758,#88759,#88760,#88761,#88762,#88763,#88764,#88765,#88766,#88767,#88768,
#88769,#88770,#88771,#88772,#88773,#88774,#88775,#88776,#88777,#88778,#88779,
#88780,#88781,#88782,#88783,#88784,#88785,#88786,#88787,#88788,#88789,#88790,
#88791,#88792,#88793,#88794,#88795,#88796,#88797,#88798,#88799,#88800,#88801,
#88802,#88803,#88804,#88805,#88806,#88807,#88808,#88809,#88810,#88811,#88812,
#88813,#88814,#88815,#88816,#88817,#88818,#88819,#88820,#88821,#88822,#88823,
#88824,#88825,#88826,#88827,#88828,#88829,#88830,#88831,#88832,#88833,#88834,
#88835,#88836,#88837,#88838,#88839,#88840,#88841,#88842,#88843,#88844,#88845,
#88846,#88847,#88848,#88849,#88850,#88851,#88852,#88853,#88854,#88855,#88856,
#88857,#88858,#88859,#88860,#88861,#88862,#88863,#88864,#88865,#88866,#88867,
#88868,#88869,#88870,#88871,#88872,#88873,#88874,#88875,#88876,#88877,#88878,
#88879,#88880,#88881,#88882,#88883,#88884,#88885,#88886,#88887,#88888,#88889,
#88890,#88891,#88892,#88893,#88894,#88895,#88896,#88897,#88898,#88899,#88900,
#88901,#88902,#88903,#88904,#88905,#88906,#88907,#88908,#88909,#88910,#88911,
#88912,#88913,#88914,#88915,#88916,#88917,#88918,#88919,#88920,#88921,#88922,
#88923,#88924,#88925,#88926,#88927,#88928,#88929,#88930,#88931,#88932,#88933,
#88934,#88935,#88936,#88937,#88938,#88939,#88940,#88941,#88942,#88943,#88944,
#88945,#88946,#88947,#88948,#88949,#88950,#88951,#88952,#88953,#88954,#88955,
#88956,#88957,#88958,#88959,#88960,#88961,#88962,#88963,#88964,#88965,#88966,
#88967,#88968,#88969,#88970,#88971,#88972,#88973,#88974,#88975,#88976,#88977,
#88978,#88979,#88980,#88981,#88982,#88983,#88984,#88985,#88986,#88987,#88988,
#88989,#88990,#88991,#88992,#88993,#88994,#88995,#88996,#88997,#88998,#88999,
#89000,#89001,#89002,#89003,#89004,#89005,#89006,#89007,#89008,#89009,#89010,
#89011,#89012,#89013,#89014,#89015,#89016,#89017,#89018,#89019,#89020,#89021,
#89022,#89023,#89024,#89025,#89026,#89027,#89028,#89029,#89030,#89031,#89032,
#89033,#89034,#89035,#89036,#89037,#89038,#89039,#89040,#89041,#89042,#89043,
#89044,#89045,#89046,#89047,#89048,#89049,#89050,#89051,#89052,#89053,#89054,
#89055,#89056,#89057,#89058,#89059,#89060,#89061,#89062,#89063,#89064,#89065,
#89066,#89067,#89068,#89069,#89070,#89071,#89072,#89073,#89074,#89075,#89076,
#89077,#89078,#89079,#89080,#89081,#89082,#89083,#89084,#89085,#89086,#89087,
#89088,#89089,#89090,#89091,#89092,#89093,#89094,#89095,#89096,#89097,#89098,
#89099,#89100,#89101,#89102,#89103,#89104,#89105,#89106,#89107,#89108,#89109,
#89110,#89111,#89112,#89113,#89114,#89115,#89116,#89117,#89118,#89119,#89120,
#89121,#89122,#89123,#89124,#89125,#89126,#89127,#89128,#89129,#89130,#89131,
#89132,#89133,#89134,#89135,#89136,#89137,#89138,#89139,#89140,#89141,#89142,
#89143,#89144,#89145,#89146,#89147,#89148,#89149,#89150,#89151,#89152,#89153,
#89154,#89155,#89156,#89157,#89158,#89159,#89160,#89161,#89162,#89163,#89164,
#89165,#89166,#89167,#89168,#89169,#89170,#89171,#89172,#89173,#89174,#89175,
#89176,#89177,#89178,#89179,#89180,#89181,#89182,#89183,#89184,#89185,#89186,
#89187,#89188,#89189,#89190,#89191,#89192,#89193,#89194,#89195,#89196,#89197,
#89198,#89199,#89200,#89201,#89202,#89203,#89204,#89205,#89206,#89207,#89208,
#89209,#89210,#89211,#89212,#89213,#89214,#89215,#89216,#89217,#89218,#89219,
#89220,#89221,#89222,#89223,#89224,#89225,#89226,#89227,#89228,#89229,#89230,
#89231,#89232,#89233,#89234,#89235,#89236,#89237,#89238,#89239,#89240,#89241,
#89242,#89243,#89244,#89245,#89246,#89247,#89248,#89249,#89250,#89251,#89252,
#89253,#89254,#89255,#89256,#89257,#89258,#89259,#89260,#89261,#89262,#89263,
#89264,#89265,#89266,#89267,#89268,#89269,#89270,#89271,#89272,#89273,#89274,
#89275,#89276,#89277,#89278,#89279,#89280,#89281,#89282,#89283,#89284,#89285,
#89286,#89287,#89288,#89289,#89290,#89291,#89292,#89293,#89294,#89295,#89296,
#89297,#89298,#89299,#89300,#89301,#89302,#89303,#89304,#89305,#89306,#89307,
#89308,#89309,#89310,#89311,#89312,#89313,#89314,#89315,#89316,#89317,#89318,
#89319,#89320,#89321,#89322,#89323,#89324,#89325,#89326,#89327,#89328,#89329,
#89330,#89331,#89332,#89333,#89334,#89335,#89336,#89337,#89338,#89339,#89340,
#89341,#89342,#89343,#89344,#89345,#89346,#89347,#89348,#89349,#89350,#89351,
#89352,#89353,#89354,#89355,#89356,#89357,#89358,#89359,#89360,#89361,#89362,
#89363,#89364,#89365,#89366,#89367,#89368,#89369,#89370,#89371,#89372,#89373,
#89374,#89375,#89376,#89377,#89378,#89379,#89380,#89381,#89382,#89383,#89384,
#89385,#89386,#89387,#89388,#89389,#89390,#89391,#89392,#89393,#89394,#89395,
#89396,#89397,#89398,#89399,#89400,#89401,#89402,#89403,#89404,#89405,#89406,
#89407,#89408,#89409,#89410,#89411,#89412,#89413,#89414,#89415,#89416,#89417,
#89418,#89419,#89420,#89421,#89422,#89423,#89424,#89425,#89426,#89427,#89428,
#89429,#89430,#89431,#89432,#89433,#89434,#89435,#89436,#89437,#89438,#89439,
#89440,#89441,#89442,#89443,#89444,#89445,#89446,#89447,#89448,#89449,#89450,
#89451,#89452,#89453,#89454,#89455,#89456,#89457,#89458,#89459,#89460,#89461,
#89462,#89463,#89464,#89465,#89466,#89467,#89468,#89469,#89470,#89471,#89472,
#89473,#89474,#89475,#89476,#89477,#89478,#89479,#89480,#89481,#89482,#89483,
#89484,#89485,#89486,#89487,#89488,#89489,#89490,#89491,#89492,#89493,#89494,
#89495,#89496,#89497,#89498,#89499,#89500,#89501,#89502,#89503,#89504,#89505,
#89506,#89507,#89508,#89509,#89510,#89511,#89512,#89513,#89514,#89515,#89516,
#89517,#89518,#89519,#89520,#89521,#89522,#89523,#89524,#89525,#89526,#89527,
#89528,#89529,#89530,#89531,#89532,#89533,#89534,#89535,#89536,#89537,#89538,
#89539,#89540,#89541,#89542,#89543,#89544,#89545,#89546,#89547,#89548,#89549,
#89550,#89551,#89552,#89553,#89554,#89555,#89556,#89557,#89558,#89559,#89560,
#89561,#89562,#89563,#89564,#89565,#89566,#89567,#89568,#89569,#89570,#89571,
#89572,#89573,#89574,#89575,#89576,#89577,#89578,#89579,#89580,#89581,#89582,
#89583,#89584,#89585,#89586,#89587,#89588,#89589,#89590,#89591,#89592,#89593,
#89594,#89595,#89596,#89597,#89598,#89599,#89600,#89601,#89602,#89603,#89604,
#89605,#89606,#89607,#89608,#89609,#89610,#89611,#89612,#89613,#89614,#89615,
#89616,#89617,#89618,#89619,#89620,#89621,#89622,#89623,#89624,#89625,#89626,
#89627,#89628,#89629,#89630,#89631,#89632,#89633,#89634,#89635,#89636,#89637,
#89638,#89639,#89640,#89641,#89642,#89643,#89644,#89645,#89646,#89647,#89648,
#89649,#89650,#89651,#89652,#89653,#89654,#89655,#89656,#89657,#89658,#89659,
#89660,#89661,#89662,#89663,#89664,#89665,#89666,#89667,#89668,#89669,#89670,
#89671,#89672,#89673,#89674,#89675,#89676,#89677,#89678,#89679,#89680,#89681,
#89682,#89683,#89684,#89685,#89686,#89687,#89688,#89689,#89690,#89691,#89692,
#89693,#89694,#89695,#89696,#89697,#89698,#89699,#89700,#89701,#89702,#89703,
#89704,#89705,#89706,#89707,#89708,#89709,#89710,#89711,#89712,#89713,#89714,
#89715,#89716,#89717,#89718,#89719,#89720,#89721,#89722,#89723,#89724,#89725,
#89726,#89727,#89728,#89729,#89730,#89731,#89732,#89733,#89734,#89735,#89736,
#89737,#89738,#89739,#89740,#89741,#89742,#89743,#89744,#89745,#89746,#89747,
#89748,#89749,#89750,#89751,#89752,#89753,#89754,#89755,#89756,#89757,#89758,
#89759,#89760,#89761,#89762,#89763,#89764,#89765,#89766,#89767,#89768,#89769,
#89770,#89771,#89772,#89773,#89774,#89775,#89776,#89777,#89778,#89779,#89780,
#89781,#89782,#89783,#89784,#89785,#89786,#89787,#89788,#89789,#89790,#89791,
#89792,#89793,#89794,#89795,#89796,#89797,#89798,#89799,#89800,#89801,#89802,
#89803,#89804,#89805,#89806,#89807,#89808,#89809,#89810,#89811,#89812,#89813,
#89814,#89815,#89816,#89817,#89818,#89819,#89820,#89821,#89822,#89823,#89824,
#89825,#89826,#89827,#89828,#89829,#89830,#89831,#89832,#89833,#89834,#89835,
#89836,#89837,#89838,#89839,#89840,#89841,#89842,#89843,#89844,#89845,#89846,
#89847,#89848,#89849,#89850,#89851,#89852,#89853,#89854,#89855,#89856,#89857,
#89858,#89859,#89860,#89861,#89862,#89863,#89864,#89865,#89866,#89867,#89868,
#89869,#89870,#89871,#89872,#89873,#89874,#89875,#89876,#89877,#89878,#89879,
#89880,#89881,#89882,#89883,#89884,#89885,#89886,#89887,#89888,#89889,#89890,
#89891,#89892,#89893,#89894,#89895,#89896,#89897,#89898,#89899,#89900,#89901,
#89902,#89903,#89904,#89905,#89906,#89907,#89908,#89909,#89910,#89911,#89912,
#89913,#89914,#89915,#89916,#89917,#89918,#89919,#89920,#89921,#89922,#89923,
#89924,#89925,#89926,#89927,#89928,#89929,#89930,#89931,#89932,#89933,#89934,
#89935,#89936,#89937,#89938,#89939,#89940,#89941,#89942,#89943,#89944,#89945,
#89946,#89947,#89948,#89949,#89950,#89951,#89952,#89953,#89954,#89955,#89956,
#89957,#89958,#89959,#89960,#89961,#89962,#89963,#89964,#89965,#89966,#89967,
#89968,#89969,#89970,#89971,#89972,#89973,#89974,#89975,#89976,#89977,#89978,
#89979,#89980,#89981,#89982,#89983,#89984,#89985,#89986,#89987,#89988,#89989,
#89990,#89991,#89992,#89993,#89994,#89995,#89996,#89997,#89998,#89999,#90000,
#90001,#90002,#90003,#90004,#90005,#90006,#90007,#90008,#90009,#90010,#90011,
#90012,#90013,#90014,#90015,#90016,#90017,#90018,#90019,#90020,#90021,#90022,
#90023,#90024,#90025,#90026,#90027,#90028,#90029,#90030,#90031,#90032,#90033,
#90034,#90035,#90036,#90037,#90038,#90039,#90040,#90041,#90042,#90043,#90044,
#90045,#90046,#90047,#90048,#90049,#90050,#90051,#90052,#90053,#90054,#90055,
#90056,#90057,#90058,#90059,#90060,#90061,#90062,#90063,#90064,#90065,#90066,
#90067,#90068,#90069,#90070,#90071,#90072,#90073,#90074,#90075,#90076,#90077,
#90078,#90079,#90080,#90081,#90082,#90083,#90084,#90085,#90086,#90087,#90088,
#90089,#90090,#90091,#90092,#90093,#90094,#90095,#90096,#90097,#90098,#90099,
#90100,#90101,#90102,#90103,#90104,#90105,#90106,#90107,#90108,#90109,#90110,
#90111,#90112,#90113,#90114,#90115,#90116,#90117,#90118,#90119,#90120,#90121,
#90122,#90123,#90124,#90125,#90126,#90127,#90128,#90129,#90130,#90131,#90132,
#90133,#90134,#90135,#90136,#90137,#90138,#90139,#90140,#90141,#90142,#90143,
#90144,#90145,#90146,#90147,#90148,#90149,#90150,#90151,#90152,#90153,#90154,
#90155,#90156,#90157,#90158,#90159,#90160,#90161,#90162,#90163,#90164,#90165,
#90166,#90167,#90168,#90169,#90170,#90171,#90172,#90173,#90174,#90175,#90176,
#90177,#90178,#90179,#90180,#90181,#90182,#90183,#90184,#90185,#90186,#90187,
#90188,#90189,#90190,#90191,#90192,#90193,#90194,#90195,#90196,#90197,#90198,
#90199,#90200,#90201,#90202,#90203,#90204,#90205,#90206,#90207,#90208,#90209,
#90210,#90211,#90212,#90213,#90214,#90215,#90216,#90217,#90218,#90219,#90220,
#90221,#90222,#90223,#90224,#90225,#90226,#90227,#90228,#90229,#90230,#90231,
#90232,#90233,#90234,#90235,#90236,#90237,#90238,#90239,#90240,#90241,#90242,
#90243,#90244,#90245,#90246,#90247,#90248,#90249,#90250,#90251,#90252,#90253,
#90254,#90255,#90256,#90257,#90258,#90259,#90260,#90261,#90262,#90263,#90264,
#90265,#90266,#90267,#90268,#90269,#90270,#90271,#90272,#90273,#90274,#90275,
#90276,#90277,#90278,#90279,#90280,#90281,#90282,#90283,#90284,#90285,#90286,
#90287,#90288,#90289,#90290,#90291,#90292,#90293,#90294,#90295,#90296,#90297,
#90298,#90299,#90300,#90301,#90302,#90303,#90304,#90305,#90306,#90307,#90308,
#90309,#90310,#90311,#90312,#90313,#90314,#90315,#90316,#90317,#90318,#90319,
#90320,#90321,#90322,#90323,#90324,#90325,#90326,#90327,#90328,#90329,#90330,
#90331,#90332,#90333,#90334,#90335,#90336,#90337,#90338,#90339,#90340,#90341,
#90342,#90343,#90344,#90345,#90346,#90347,#90348,#90349,#90350,#90351,#90352,
#90353,#90354,#90355,#90356,#90357,#90358,#90359,#90360,#90361,#90362,#90363,
#90364,#90365,#90366,#90367,#90368,#90369,#90370,#90371,#90372,#90373,#90374,
#90375,#90376,#90377,#90378,#90379,#90380,#90381,#90382,#90383,#90384,#90385,
#90386,#90387,#90388,#90389,#90390,#90391,#90392,#90393,#90394,#90395,#90396,
#90397,#90398,#90399,#90400,#90401,#90402,#90403,#90404,#90405,#90406,#90407,
#90408,#90409,#90410,#90411,#90412,#90413,#90414,#90415,#90416,#90417,#90418,
#90419,#90420,#90421,#90422,#90423,#90424,#90425,#90426,#90427,#90428,#90429,
#90430,#90431,#90432,#90433,#90434,#90435,#90436,#90437,#90438,#90439,#90440,
#90441,#90442,#90443,#90444,#90445,#90446,#90447,#90448,#90449,#90450,#90451,
#90452,#90453,#90454,#90455,#90456,#90457,#90458,#90459,#90460,#90461,#90462,
#90463,#90464,#90465,#90466,#90467,#90468,#90469,#90470,#90471,#90472,#90473,
#90474,#90475,#90476,#90477,#90478,#90479,#90480,#90481,#90482,#90483,#90484,
#90485,#90486,#90487,#90488,#90489,#90490,#90491,#90492,#90493,#90494,#90495,
#90496,#90497,#90498,#90499,#90500,#90501,#90502,#90503,#90504,#90505,#90506,
#90507,#90508,#90509,#90510,#90511,#90512,#90513,#90514,#90515,#90516,#90517,
#90518,#90519,#90520,#90521,#90522,#90523,#90524,#90525,#90526,#90527,#90528,
#90529,#90530,#90531,#90532,#90533,#90534,#90535,#90536,#90537,#90538,#90539,
#90540,#90541,#90542,#90543,#90544,#90545,#90546,#90547,#90548,#90549,#90550,
#90551,#90552,#90553,#90554,#90555,#90556,#90557,#90558,#90559,#90560,#90561,
#90562,#90563,#90564,#90565,#90566,#90567,#90568,#90569,#90570,#90571,#90572,
#90573,#90574,#90575,#90576,#90577,#90578,#90579,#90580,#90581,#90582,#90583,
#90584,#90585,#90586,#90587,#90588,#90589,#90590,#90591,#90592,#90593,#90594,
#90595,#90596,#90597,#90598,#90599,#90600,#90601,#90602,#90603,#90604,#90605,
#90606,#90607,#90608,#90609,#90610,#90611,#90612,#90613,#90614,#90615,#90616,
#90617,#90618,#90619,#90620,#90621,#90622,#90623,#90624,#90625,#90626,#90627,
#90628,#90629,#90630,#90631,#90632,#90633,#90634,#90635,#90636,#90637,#90638,
#90639,#90640,#90641,#90642,#90643,#90644,#90645,#90646,#90647,#90648,#90649,
#90650,#90651,#90652,#90653,#90654,#90655,#90656,#90657,#90658,#90659,#90660,
#90661,#90662,#90663,#90664,#90665,#90666,#90667,#90668,#90669,#90670,#90671,
#90672,#90673,#90674,#90675,#90676,#90677,#90678,#90679,#90680,#90681,#90682,
#90683,#90684,#90685,#90686,#90687,#90688,#90689,#90690,#90691,#90692,#90693,
#90694,#90695,#90696,#90697,#90698,#90699,#90700,#90701,#90702,#90703,#90704,
#90705,#90706,#90707,#90708,#90709,#90710,#90711,#90712,#90713,#90714,#90715,
#90716,#90717,#90718,#90719,#90720,#90721,#90722,#90723,#90724,#90725,#90726,
#90727,#90728,#90729,#90730,#90731,#90732,#90733,#90734,#90735,#90736,#90737,
#90738,#90739,#90740,#90741,#90742,#90743,#90744,#90745,#90746,#90747,#90748,
#90749,#90750,#90751,#90752,#90753,#90754,#90755,#90756,#90757,#90758,#90759,
#90760,#90761,#90762,#90763,#90764,#90765,#90766,#90767,#90768,#90769,#90770,
#90771,#90772,#90773,#90774,#90775,#90776,#90777,#90778,#90779,#90780,#90781,
#90782,#90783,#90784,#90785,#90786,#90787,#90788,#90789,#90790,#90791,#90792,
#90793,#90794,#90795,#90796,#90797,#90798,#90799,#90800,#90801,#90802,#90803,
#90804,#90805,#90806,#90807,#90808,#90809,#90810,#90811,#90812,#90813,#90814,
#90815,#90816,#90817,#90818,#90819,#90820,#90821,#90822,#90823,#90824,#90825,
#90826,#90827,#90828,#90829,#90830,#90831,#90832,#90833,#90834,#90835,#90836,
#90837,#90838,#90839,#90840,#90841,#90842,#90843,#90844,#90845,#90846,#90847,
#90848,#90849,#90850,#90851,#90852,#90853,#90854,#90855,#90856,#90857,#90858,
#90859,#90860,#90861,#90862,#90863,#90864,#90865,#90866,#90867,#90868,#90869,
#90870,#90871,#90872,#90873,#90874,#90875,#90876,#90877,#90878,#90879,#90880,
#90881,#90882,#90883,#90884,#90885,#90886,#90887,#90888,#90889,#90890,#90891,
#90892,#90893,#90894,#90895,#90896,#90897,#90898,#90899,#90900,#90901,#90902,
#90903,#90904,#90905,#90906,#90907,#90908,#90909,#90910,#90911,#90912,#90913,
#90914,#90915,#90916,#90917,#90918,#90919,#90920,#90921,#90922,#90923,#90924,
#90925,#90926,#90927,#90928,#90929,#90930,#90931,#90932,#90933,#90934,#90935,
#90936,#90937,#90938,#90939,#90940,#90941,#90942,#90943,#90944,#90945,#90946,
#90947,#90948,#90949,#90950,#90951,#90952,#90953,#90954,#90955,#90956,#90957,
#90958,#90959,#90960,#90961,#90962,#90963,#90964,#90965,#90966,#90967,#90968,
#90969,#90970,#90971,#90972,#90973,#90974,#90975,#90976,#90977,#90978,#90979,
#90980,#90981,#90982,#90983,#90984,#90985,#90986,#90987,#90988,#90989,#90990,
#90991,#90992,#90993,#90994,#90995,#90996,#90997,#90998,#90999,#91000,#91001,
#91002,#91003,#91004,#91005,#91006,#91007,#91008,#91009,#91010,#91011,#91012,
#91013,#91014,#91015,#91016,#91017,#91018,#91019,#91020,#91021,#91022,#91023,
#91024,#91025,#91026,#91027,#91028,#91029,#91030,#91031,#91032,#91033,#91034,
#91035,#91036,#91037,#91038,#91039,#91040,#91041,#91042,#91043,#91044,#91045,
#91046,#91047,#91048,#91049,#91050,#91051,#91052,#91053,#91054,#91055,#91056,
#91057,#91058,#91059,#91060,#91061,#91062,#91063,#91064,#91065,#91066,#91067,
#91068,#91069,#91070,#91071,#91072,#91073,#91074,#91075,#91076,#91077,#91078,
#91079,#91080,#91081,#91082)) ;
#98151=AXIS2_PLACEMENT_3D('',#152009,#120475,#120476) ;
#98152=AXIS2_PLACEMENT_3D('',#152010,#120477,#120478) ;
#98153=AXIS2_PLACEMENT_3D('',#152013,#120479,#120480) ;
#98154=AXIS2_PLACEMENT_3D('',#152017,#120482,#120483) ;
#98155=AXIS2_PLACEMENT_3D('',#152019,#120485,#120486) ;
#98156=AXIS2_PLACEMENT_3D('',#152022,#120487,#120488) ;
#98157=AXIS2_PLACEMENT_3D('',#152024,#120489,#120490) ;
#98158=AXIS2_PLACEMENT_3D('',#152026,#120491,#120492) ;
#98159=AXIS2_PLACEMENT_3D('',#152027,#120493,#120494) ;
#98160=AXIS2_PLACEMENT_3D('',#152028,#120495,#120496) ;
#98161=AXIS2_PLACEMENT_3D('',#152031,#120497,#120498) ;
#98162=AXIS2_PLACEMENT_3D('',#152033,#120499,#120500) ;
#98163=AXIS2_PLACEMENT_3D('',#152035,#120501,#120502) ;
#98164=AXIS2_PLACEMENT_3D('',#152036,#120503,#120504) ;
#98165=AXIS2_PLACEMENT_3D('',#152037,#120505,#120506) ;
#98166=AXIS2_PLACEMENT_3D('',#152040,#120507,#120508) ;
#98167=AXIS2_PLACEMENT_3D('',#152122,#120509,#120510) ;
#98168=AXIS2_PLACEMENT_3D('',#152173,#120511,#120512) ;
#98169=AXIS2_PLACEMENT_3D('',#152176,#120513,#120514) ;
#98170=AXIS2_PLACEMENT_3D('',#152178,#120515,#120516) ;
#98171=AXIS2_PLACEMENT_3D('',#152180,#120517,#120518) ;
#98172=AXIS2_PLACEMENT_3D('',#152181,#120519,#120520) ;
#98173=AXIS2_PLACEMENT_3D('',#152182,#120521,#120522) ;
#98174=AXIS2_PLACEMENT_3D('',#152184,#120523,#120524) ;
#98175=AXIS2_PLACEMENT_3D('',#152266,#120525,#120526) ;
#98176=AXIS2_PLACEMENT_3D('',#152348,#120527,#120528) ;
#98177=AXIS2_PLACEMENT_3D('',#152351,#120529,#120530) ;
#98178=AXIS2_PLACEMENT_3D('',#152353,#120531,#120532) ;
#98179=AXIS2_PLACEMENT_3D('',#152355,#120533,#120534) ;
#98180=AXIS2_PLACEMENT_3D('',#152356,#120535,#120536) ;
#98181=AXIS2_PLACEMENT_3D('',#152357,#120537,#120538) ;
#98182=AXIS2_PLACEMENT_3D('',#152359,#120539,#120540) ;
#98183=AXIS2_PLACEMENT_3D('',#152444,#120541,#120542) ;
#98184=AXIS2_PLACEMENT_3D('',#152524,#120543,#120544) ;
#98185=AXIS2_PLACEMENT_3D('',#152527,#120545,#120546) ;
#98186=AXIS2_PLACEMENT_3D('',#152529,#120547,#120548) ;
#98187=AXIS2_PLACEMENT_3D('',#152531,#120549,#120550) ;
#98188=AXIS2_PLACEMENT_3D('',#152532,#120551,#120552) ;
#98189=AXIS2_PLACEMENT_3D('',#152533,#120553,#120554) ;
#98190=AXIS2_PLACEMENT_3D('',#152535,#120555,#120556) ;
#98191=AXIS2_PLACEMENT_3D('',#152618,#120557,#120558) ;
#98192=AXIS2_PLACEMENT_3D('',#152700,#120559,#120560) ;
#98193=AXIS2_PLACEMENT_3D('',#152703,#120561,#120562) ;
#98194=AXIS2_PLACEMENT_3D('',#152705,#120563,#120564) ;
#98195=AXIS2_PLACEMENT_3D('',#152707,#120565,#120566) ;
#98196=AXIS2_PLACEMENT_3D('',#152708,#120567,#120568) ;
#98197=AXIS2_PLACEMENT_3D('',#152709,#120569,#120570) ;
#98198=AXIS2_PLACEMENT_3D('',#152711,#120571,#120572) ;
#98199=AXIS2_PLACEMENT_3D('',#152793,#120573,#120574) ;
#98200=AXIS2_PLACEMENT_3D('',#152875,#120575,#120576) ;
#98201=AXIS2_PLACEMENT_3D('',#152878,#120577,#120578) ;
#98202=AXIS2_PLACEMENT_3D('',#152880,#120579,#120580) ;
#98203=AXIS2_PLACEMENT_3D('',#152882,#120581,#120582) ;
#98204=AXIS2_PLACEMENT_3D('',#152883,#120583,#120584) ;
#98205=AXIS2_PLACEMENT_3D('',#152884,#120585,#120586) ;
#98206=AXIS2_PLACEMENT_3D('',#152886,#120587,#120588) ;
#98207=AXIS2_PLACEMENT_3D('',#152968,#120589,#120590) ;
#98208=AXIS2_PLACEMENT_3D('',#153050,#120591,#120592) ;
#98209=AXIS2_PLACEMENT_3D('',#153053,#120593,#120594) ;
#98210=AXIS2_PLACEMENT_3D('',#153055,#120595,#120596) ;
#98211=AXIS2_PLACEMENT_3D('',#153057,#120597,#120598) ;
#98212=AXIS2_PLACEMENT_3D('',#153058,#120599,#120600) ;
#98213=AXIS2_PLACEMENT_3D('',#153059,#120601,#120602) ;
#98214=AXIS2_PLACEMENT_3D('',#153061,#120603,#120604) ;
#98215=AXIS2_PLACEMENT_3D('',#153143,#120605,#120606) ;
#98216=AXIS2_PLACEMENT_3D('',#153225,#120607,#120608) ;
#98217=AXIS2_PLACEMENT_3D('',#153228,#120609,#120610) ;
#98218=AXIS2_PLACEMENT_3D('',#153230,#120611,#120612) ;
#98219=AXIS2_PLACEMENT_3D('',#153232,#120613,#120614) ;
#98220=AXIS2_PLACEMENT_3D('',#153233,#120615,#120616) ;
#98221=AXIS2_PLACEMENT_3D('',#153234,#120617,#120618) ;
#98222=AXIS2_PLACEMENT_3D('',#153236,#120619,#120620) ;
#98223=AXIS2_PLACEMENT_3D('',#153320,#120621,#120622) ;
#98224=AXIS2_PLACEMENT_3D('',#153401,#120623,#120624) ;
#98225=AXIS2_PLACEMENT_3D('',#153404,#120625,#120626) ;
#98226=AXIS2_PLACEMENT_3D('',#153406,#120627,#120628) ;
#98227=AXIS2_PLACEMENT_3D('',#153408,#120629,#120630) ;
#98228=AXIS2_PLACEMENT_3D('',#153409,#120631,#120632) ;
#98229=AXIS2_PLACEMENT_3D('',#153410,#120633,#120634) ;
#98230=AXIS2_PLACEMENT_3D('',#153412,#120635,#120636) ;
#98231=AXIS2_PLACEMENT_3D('',#153495,#120637,#120638) ;
#98232=AXIS2_PLACEMENT_3D('',#153575,#120639,#120640) ;
#98233=AXIS2_PLACEMENT_3D('',#153578,#120641,#120642) ;
#98234=AXIS2_PLACEMENT_3D('',#153580,#120643,#120644) ;
#98235=AXIS2_PLACEMENT_3D('',#153582,#120645,#120646) ;
#98236=AXIS2_PLACEMENT_3D('',#153583,#120647,#120648) ;
#98237=AXIS2_PLACEMENT_3D('',#153584,#120649,#120650) ;
#98238=AXIS2_PLACEMENT_3D('',#153586,#120651,#120652) ;
#98239=AXIS2_PLACEMENT_3D('',#153639,#120653,#120654) ;
#98240=AXIS2_PLACEMENT_3D('',#153719,#120655,#120656) ;
#98241=AXIS2_PLACEMENT_3D('',#153720,#120657,#120658) ;
#98242=AXIS2_PLACEMENT_3D('',#153723,#120661,#120662) ;
#98243=AXIS2_PLACEMENT_3D('',#153724,#120663,#120664) ;
#98244=AXIS2_PLACEMENT_3D('',#153727,#120667,#120668) ;
#98245=AXIS2_PLACEMENT_3D('',#153728,#120669,#120670) ;
#98246=AXIS2_PLACEMENT_3D('',#153731,#120673,#120674) ;
#98247=AXIS2_PLACEMENT_3D('',#153732,#120675,#120676) ;
#98248=AXIS2_PLACEMENT_3D('',#153735,#120679,#120680) ;
#98249=AXIS2_PLACEMENT_3D('',#153736,#120681,#120682) ;
#98250=AXIS2_PLACEMENT_3D('',#153739,#120685,#120686) ;
#98251=AXIS2_PLACEMENT_3D('',#153740,#120687,#120688) ;
#98252=AXIS2_PLACEMENT_3D('',#153743,#120691,#120692) ;
#98253=AXIS2_PLACEMENT_3D('',#153744,#120693,#120694) ;
#98254=AXIS2_PLACEMENT_3D('',#153747,#120697,#120698) ;
#98255=AXIS2_PLACEMENT_3D('',#153749,#120699,#120700) ;
#98256=AXIS2_PLACEMENT_3D('',#153751,#120701,#120702) ;
#98257=AXIS2_PLACEMENT_3D('',#153752,#120703,#120704) ;
#98258=AXIS2_PLACEMENT_3D('',#153753,#120705,#120706) ;
#98259=AXIS2_PLACEMENT_3D('',#153755,#120707,#120708) ;
#98260=AXIS2_PLACEMENT_3D('',#153757,#120709,#120710) ;
#98261=AXIS2_PLACEMENT_3D('',#153758,#120711,#120712) ;
#98262=AXIS2_PLACEMENT_3D('',#153759,#120713,#120714) ;
#98263=AXIS2_PLACEMENT_3D('',#153761,#120715,#120716) ;
#98264=AXIS2_PLACEMENT_3D('',#153763,#120717,#120718) ;
#98265=AXIS2_PLACEMENT_3D('',#153764,#120719,#120720) ;
#98266=AXIS2_PLACEMENT_3D('',#153765,#120721,#120722) ;
#98267=AXIS2_PLACEMENT_3D('',#153767,#120723,#120724) ;
#98268=AXIS2_PLACEMENT_3D('',#153769,#120725,#120726) ;
#98269=AXIS2_PLACEMENT_3D('',#153770,#120727,#120728) ;
#98270=AXIS2_PLACEMENT_3D('',#153771,#120729,#120730) ;
#98271=AXIS2_PLACEMENT_3D('',#153773,#120731,#120732) ;
#98272=AXIS2_PLACEMENT_3D('',#153775,#120733,#120734) ;
#98273=AXIS2_PLACEMENT_3D('',#153776,#120735,#120736) ;
#98274=AXIS2_PLACEMENT_3D('',#153777,#120737,#120738) ;
#98275=AXIS2_PLACEMENT_3D('',#153779,#120739,#120740) ;
#98276=AXIS2_PLACEMENT_3D('',#153781,#120741,#120742) ;
#98277=AXIS2_PLACEMENT_3D('',#153782,#120743,#120744) ;
#98278=AXIS2_PLACEMENT_3D('',#153783,#120745,#120746) ;
#98279=AXIS2_PLACEMENT_3D('',#153785,#120747,#120748) ;
#98280=AXIS2_PLACEMENT_3D('',#153787,#120749,#120750) ;
#98281=AXIS2_PLACEMENT_3D('',#153788,#120751,#120752) ;
#98282=AXIS2_PLACEMENT_3D('',#153789,#120753,#120754) ;
#98283=AXIS2_PLACEMENT_3D('',#153791,#120755,#120756) ;
#98284=AXIS2_PLACEMENT_3D('',#153793,#120757,#120758) ;
#98285=AXIS2_PLACEMENT_3D('',#153794,#120759,#120760) ;
#98286=AXIS2_PLACEMENT_3D('',#153795,#120761,#120762) ;
#98287=AXIS2_PLACEMENT_3D('',#153797,#120763,#120764) ;
#98288=AXIS2_PLACEMENT_3D('',#153799,#120765,#120766) ;
#98289=AXIS2_PLACEMENT_3D('',#153800,#120767,#120768) ;
#98290=AXIS2_PLACEMENT_3D('',#153801,#120769,#120770) ;
#98291=AXIS2_PLACEMENT_3D('',#153803,#120771,#120772) ;
#98292=AXIS2_PLACEMENT_3D('',#153805,#120773,#120774) ;
#98293=AXIS2_PLACEMENT_3D('',#153806,#120775,#120776) ;
#98294=AXIS2_PLACEMENT_3D('',#153807,#120777,#120778) ;
#98295=AXIS2_PLACEMENT_3D('',#153809,#120779,#120780) ;
#98296=AXIS2_PLACEMENT_3D('',#153811,#120781,#120782) ;
#98297=AXIS2_PLACEMENT_3D('',#153812,#120783,#120784) ;
#98298=AXIS2_PLACEMENT_3D('',#153813,#120785,#120786) ;
#98299=AXIS2_PLACEMENT_3D('',#153815,#120787,#120788) ;
#98300=AXIS2_PLACEMENT_3D('',#153817,#120789,#120790) ;
#98301=AXIS2_PLACEMENT_3D('',#153818,#120791,#120792) ;
#98302=AXIS2_PLACEMENT_3D('',#153819,#120793,#120794) ;
#98303=AXIS2_PLACEMENT_3D('',#153821,#120795,#120796) ;
#98304=AXIS2_PLACEMENT_3D('',#153823,#120797,#120798) ;
#98305=AXIS2_PLACEMENT_3D('',#153824,#120799,#120800) ;
#98306=AXIS2_PLACEMENT_3D('',#153825,#120801,#120802) ;
#98307=AXIS2_PLACEMENT_3D('',#153827,#120803,#120804) ;
#98308=AXIS2_PLACEMENT_3D('',#153829,#120805,#120806) ;
#98309=AXIS2_PLACEMENT_3D('',#153830,#120807,#120808) ;
#98310=AXIS2_PLACEMENT_3D('',#153831,#120809,#120810) ;
#98311=AXIS2_PLACEMENT_3D('',#153833,#120811,#120812) ;
#98312=AXIS2_PLACEMENT_3D('',#153835,#120813,#120814) ;
#98313=AXIS2_PLACEMENT_3D('',#153836,#120815,#120816) ;
#98314=AXIS2_PLACEMENT_3D('',#153837,#120817,#120818) ;
#98315=AXIS2_PLACEMENT_3D('',#153839,#120819,#120820) ;
#98316=AXIS2_PLACEMENT_3D('',#153841,#120821,#120822) ;
#98317=AXIS2_PLACEMENT_3D('',#153842,#120823,#120824) ;
#98318=AXIS2_PLACEMENT_3D('',#153843,#120825,#120826) ;
#98319=AXIS2_PLACEMENT_3D('',#153845,#120827,#120828) ;
#98320=AXIS2_PLACEMENT_3D('',#153847,#120829,#120830) ;
#98321=AXIS2_PLACEMENT_3D('',#153848,#120831,#120832) ;
#98322=AXIS2_PLACEMENT_3D('',#153849,#120833,#120834) ;
#98323=AXIS2_PLACEMENT_3D('',#153851,#120835,#120836) ;
#98324=AXIS2_PLACEMENT_3D('',#153853,#120837,#120838) ;
#98325=AXIS2_PLACEMENT_3D('',#153854,#120839,#120840) ;
#98326=AXIS2_PLACEMENT_3D('',#153855,#120841,#120842) ;
#98327=AXIS2_PLACEMENT_3D('',#153857,#120843,#120844) ;
#98328=AXIS2_PLACEMENT_3D('',#153859,#120845,#120846) ;
#98329=AXIS2_PLACEMENT_3D('',#153860,#120847,#120848) ;
#98330=AXIS2_PLACEMENT_3D('',#153861,#120849,#120850) ;
#98331=AXIS2_PLACEMENT_3D('',#153863,#120851,#120852) ;
#98332=AXIS2_PLACEMENT_3D('',#153865,#120853,#120854) ;
#98333=AXIS2_PLACEMENT_3D('',#153866,#120855,#120856) ;
#98334=AXIS2_PLACEMENT_3D('',#153867,#120857,#120858) ;
#98335=AXIS2_PLACEMENT_3D('',#153869,#120859,#120860) ;
#98336=AXIS2_PLACEMENT_3D('',#153871,#120861,#120862) ;
#98337=AXIS2_PLACEMENT_3D('',#153872,#120863,#120864) ;
#98338=AXIS2_PLACEMENT_3D('',#153873,#120865,#120866) ;
#98339=AXIS2_PLACEMENT_3D('',#153875,#120867,#120868) ;
#98340=AXIS2_PLACEMENT_3D('',#153877,#120869,#120870) ;
#98341=AXIS2_PLACEMENT_3D('',#153878,#120871,#120872) ;
#98342=AXIS2_PLACEMENT_3D('',#153879,#120873,#120874) ;
#98343=AXIS2_PLACEMENT_3D('',#153881,#120875,#120876) ;
#98344=AXIS2_PLACEMENT_3D('',#153883,#120877,#120878) ;
#98345=AXIS2_PLACEMENT_3D('',#153884,#120879,#120880) ;
#98346=AXIS2_PLACEMENT_3D('',#153885,#120881,#120882) ;
#98347=AXIS2_PLACEMENT_3D('',#153887,#120883,#120884) ;
#98348=AXIS2_PLACEMENT_3D('',#153889,#120885,#120886) ;
#98349=AXIS2_PLACEMENT_3D('',#153890,#120887,#120888) ;
#98350=AXIS2_PLACEMENT_3D('',#153891,#120889,#120890) ;
#98351=AXIS2_PLACEMENT_3D('',#153893,#120891,#120892) ;
#98352=AXIS2_PLACEMENT_3D('',#153895,#120893,#120894) ;
#98353=AXIS2_PLACEMENT_3D('',#153896,#120895,#120896) ;
#98354=AXIS2_PLACEMENT_3D('',#153897,#120897,#120898) ;
#98355=AXIS2_PLACEMENT_3D('',#153899,#120899,#120900) ;
#98356=AXIS2_PLACEMENT_3D('',#153901,#120901,#120902) ;
#98357=AXIS2_PLACEMENT_3D('',#153902,#120903,#120904) ;
#98358=AXIS2_PLACEMENT_3D('',#153903,#120905,#120906) ;
#98359=AXIS2_PLACEMENT_3D('',#153905,#120907,#120908) ;
#98360=AXIS2_PLACEMENT_3D('',#153907,#120909,#120910) ;
#98361=AXIS2_PLACEMENT_3D('',#153908,#120911,#120912) ;
#98362=AXIS2_PLACEMENT_3D('',#153909,#120913,#120914) ;
#98363=AXIS2_PLACEMENT_3D('',#153912,#120915,#120916) ;
#98364=AXIS2_PLACEMENT_3D('',#153938,#120918,#120919) ;
#98365=AXIS2_PLACEMENT_3D('',#153985,#120921,#120922) ;
#98366=AXIS2_PLACEMENT_3D('',#154011,#120924,#120925) ;
#98367=AXIS2_PLACEMENT_3D('',#154057,#120927,#120928) ;
#98368=AXIS2_PLACEMENT_3D('',#154059,#120930,#120931) ;
#98369=AXIS2_PLACEMENT_3D('',#154062,#120932,#120933) ;
#98370=AXIS2_PLACEMENT_3D('',#154088,#120935,#120936) ;
#98371=AXIS2_PLACEMENT_3D('',#154135,#120938,#120939) ;
#98372=AXIS2_PLACEMENT_3D('',#154161,#120941,#120942) ;
#98373=AXIS2_PLACEMENT_3D('',#154207,#120944,#120945) ;
#98374=AXIS2_PLACEMENT_3D('',#154209,#120947,#120948) ;
#98375=AXIS2_PLACEMENT_3D('',#154212,#120949,#120950) ;
#98376=AXIS2_PLACEMENT_3D('',#154238,#120952,#120953) ;
#98377=AXIS2_PLACEMENT_3D('',#154285,#120955,#120956) ;
#98378=AXIS2_PLACEMENT_3D('',#154311,#120958,#120959) ;
#98379=AXIS2_PLACEMENT_3D('',#154357,#120961,#120962) ;
#98380=AXIS2_PLACEMENT_3D('',#154359,#120964,#120965) ;
#98381=AXIS2_PLACEMENT_3D('',#154362,#120966,#120967) ;
#98382=AXIS2_PLACEMENT_3D('',#154388,#120969,#120970) ;
#98383=AXIS2_PLACEMENT_3D('',#154435,#120972,#120973) ;
#98384=AXIS2_PLACEMENT_3D('',#154461,#120975,#120976) ;
#98385=AXIS2_PLACEMENT_3D('',#154507,#120978,#120979) ;
#98386=AXIS2_PLACEMENT_3D('',#154509,#120981,#120982) ;
#98387=AXIS2_PLACEMENT_3D('',#154512,#120983,#120984) ;
#98388=AXIS2_PLACEMENT_3D('',#154538,#120986,#120987) ;
#98389=AXIS2_PLACEMENT_3D('',#154585,#120989,#120990) ;
#98390=AXIS2_PLACEMENT_3D('',#154611,#120992,#120993) ;
#98391=AXIS2_PLACEMENT_3D('',#154657,#120995,#120996) ;
#98392=AXIS2_PLACEMENT_3D('',#154659,#120998,#120999) ;
#98393=AXIS2_PLACEMENT_3D('',#154662,#121000,#121001) ;
#98394=AXIS2_PLACEMENT_3D('',#154688,#121003,#121004) ;
#98395=AXIS2_PLACEMENT_3D('',#154735,#121006,#121007) ;
#98396=AXIS2_PLACEMENT_3D('',#154761,#121009,#121010) ;
#98397=AXIS2_PLACEMENT_3D('',#154807,#121012,#121013) ;
#98398=AXIS2_PLACEMENT_3D('',#154809,#121015,#121016) ;
#98399=AXIS2_PLACEMENT_3D('',#154812,#121017,#121018) ;
#98400=AXIS2_PLACEMENT_3D('',#154838,#121020,#121021) ;
#98401=AXIS2_PLACEMENT_3D('',#154885,#121023,#121024) ;
#98402=AXIS2_PLACEMENT_3D('',#154911,#121026,#121027) ;
#98403=AXIS2_PLACEMENT_3D('',#154957,#121029,#121030) ;
#98404=AXIS2_PLACEMENT_3D('',#154959,#121032,#121033) ;
#98405=AXIS2_PLACEMENT_3D('',#154962,#121034,#121035) ;
#98406=AXIS2_PLACEMENT_3D('',#154988,#121037,#121038) ;
#98407=AXIS2_PLACEMENT_3D('',#155035,#121040,#121041) ;
#98408=AXIS2_PLACEMENT_3D('',#155061,#121043,#121044) ;
#98409=AXIS2_PLACEMENT_3D('',#155107,#121046,#121047) ;
#98410=AXIS2_PLACEMENT_3D('',#155109,#121049,#121050) ;
#98411=AXIS2_PLACEMENT_3D('',#155112,#121051,#121052) ;
#98412=AXIS2_PLACEMENT_3D('',#155138,#121054,#121055) ;
#98413=AXIS2_PLACEMENT_3D('',#155185,#121057,#121058) ;
#98414=AXIS2_PLACEMENT_3D('',#155211,#121060,#121061) ;
#98415=AXIS2_PLACEMENT_3D('',#155257,#121063,#121064) ;
#98416=AXIS2_PLACEMENT_3D('',#155259,#121066,#121067) ;
#98417=AXIS2_PLACEMENT_3D('',#155261,#121068,#121069) ;
#98418=AXIS2_PLACEMENT_3D('',#155263,#121071,#121072) ;
#98419=AXIS2_PLACEMENT_3D('',#155265,#121073,#121074) ;
#98420=AXIS2_PLACEMENT_3D('',#155267,#121076,#121077) ;
#98421=AXIS2_PLACEMENT_3D('',#155269,#121078,#121079) ;
#98422=AXIS2_PLACEMENT_3D('',#155271,#121081,#121082) ;
#98423=AXIS2_PLACEMENT_3D('',#155273,#121083,#121084) ;
#98424=AXIS2_PLACEMENT_3D('',#155275,#121086,#121087) ;
#98425=AXIS2_PLACEMENT_3D('',#155277,#121088,#121089) ;
#98426=AXIS2_PLACEMENT_3D('',#155279,#121091,#121092) ;
#98427=AXIS2_PLACEMENT_3D('',#155281,#121093,#121094) ;
#98428=AXIS2_PLACEMENT_3D('',#155283,#121096,#121097) ;
#98429=AXIS2_PLACEMENT_3D('',#155285,#121098,#121099) ;
#98430=AXIS2_PLACEMENT_3D('',#155287,#121101,#121102) ;
#98431=AXIS2_PLACEMENT_3D('',#155289,#121103,#121104) ;
#98432=AXIS2_PLACEMENT_3D('',#155291,#121106,#121107) ;
#98433=AXIS2_PLACEMENT_3D('',#155293,#121108,#121109) ;
#98434=AXIS2_PLACEMENT_3D('',#155295,#121111,#121112) ;
#98435=AXIS2_PLACEMENT_3D('',#155297,#121114,#121115) ;
#98436=AXIS2_PLACEMENT_3D('',#155299,#121117,#121118) ;
#98437=AXIS2_PLACEMENT_3D('',#155301,#121120,#121121) ;
#98438=AXIS2_PLACEMENT_3D('',#155303,#121123,#121124) ;
#98439=AXIS2_PLACEMENT_3D('',#155305,#121126,#121127) ;
#98440=AXIS2_PLACEMENT_3D('',#155307,#121129,#121130) ;
#98441=AXIS2_PLACEMENT_3D('',#155309,#121132,#121133) ;
#98442=AXIS2_PLACEMENT_3D('',#155311,#121135,#121136) ;
#98443=AXIS2_PLACEMENT_3D('',#155313,#121138,#121139) ;
#98444=AXIS2_PLACEMENT_3D('',#155315,#121140,#121141) ;
#98445=AXIS2_PLACEMENT_3D('',#155317,#121142,#121143) ;
#98446=AXIS2_PLACEMENT_3D('',#155318,#121144,#121145) ;
#98447=AXIS2_PLACEMENT_3D('',#155319,#121146,#121147) ;
#98448=AXIS2_PLACEMENT_3D('',#155321,#121148,#121149) ;
#98449=AXIS2_PLACEMENT_3D('',#155323,#121150,#121151) ;
#98450=AXIS2_PLACEMENT_3D('',#155324,#121152,#121153) ;
#98451=AXIS2_PLACEMENT_3D('',#155325,#121154,#121155) ;
#98452=AXIS2_PLACEMENT_3D('',#155327,#121156,#121157) ;
#98453=AXIS2_PLACEMENT_3D('',#155329,#121158,#121159) ;
#98454=AXIS2_PLACEMENT_3D('',#155330,#121160,#121161) ;
#98455=AXIS2_PLACEMENT_3D('',#155331,#121162,#121163) ;
#98456=AXIS2_PLACEMENT_3D('',#155332,#121164,#121165) ;
#98457=AXIS2_PLACEMENT_3D('',#155335,#121168,#121169) ;
#98458=AXIS2_PLACEMENT_3D('',#155337,#121170,#121171) ;
#98459=AXIS2_PLACEMENT_3D('',#155340,#121174,#121175) ;
#98460=AXIS2_PLACEMENT_3D('',#155342,#121176,#121177) ;
#98461=AXIS2_PLACEMENT_3D('',#155345,#121180,#121181) ;
#98462=AXIS2_PLACEMENT_3D('',#155346,#121182,#121183) ;
#98463=AXIS2_PLACEMENT_3D('',#155349,#121186,#121187) ;
#98464=AXIS2_PLACEMENT_3D('',#155352,#121188,#121189) ;
#98465=AXIS2_PLACEMENT_3D('',#155378,#121191,#121192) ;
#98466=AXIS2_PLACEMENT_3D('',#155425,#121194,#121195) ;
#98467=AXIS2_PLACEMENT_3D('',#155451,#121197,#121198) ;
#98468=AXIS2_PLACEMENT_3D('',#155497,#121200,#121201) ;
#98469=AXIS2_PLACEMENT_3D('',#155499,#121203,#121204) ;
#98470=AXIS2_PLACEMENT_3D('',#155501,#121205,#121206) ;
#98471=AXIS2_PLACEMENT_3D('',#155503,#121208,#121209) ;
#98472=AXIS2_PLACEMENT_3D('',#155505,#121211,#121212) ;
#98473=AXIS2_PLACEMENT_3D('',#155514,#121217,#121218) ;
#98474=AXIS2_PLACEMENT_3D('',#155515,#121219,#121220) ;
#98475=AXIS2_PLACEMENT_3D('',#155516,#121221,#121222) ;
#98476=AXIS2_PLACEMENT_3D('',#155517,#121223,#121224) ;
#98477=AXIS2_PLACEMENT_3D('',#155518,#121225,#121226) ;
#98478=AXIS2_PLACEMENT_3D('',#155519,#121227,#121228) ;
#98479=AXIS2_PLACEMENT_3D('',#155520,#121229,#121230) ;
#98480=AXIS2_PLACEMENT_3D('',#155521,#121231,#121232) ;
#98481=AXIS2_PLACEMENT_3D('',#155522,#121233,#121234) ;
#98482=AXIS2_PLACEMENT_3D('',#155523,#121235,#121236) ;
#98483=AXIS2_PLACEMENT_3D('',#155531,#121240,#121241) ;
#98484=AXIS2_PLACEMENT_3D('',#155535,#121243,#121244) ;
#98485=AXIS2_PLACEMENT_3D('',#155539,#121246,#121247) ;
#98486=AXIS2_PLACEMENT_3D('',#155543,#121249,#121250) ;
#98487=AXIS2_PLACEMENT_3D('',#155547,#121252,#121253) ;
#98488=AXIS2_PLACEMENT_3D('',#155551,#121255,#121256) ;
#98489=AXIS2_PLACEMENT_3D('',#155555,#121258,#121259) ;
#98490=AXIS2_PLACEMENT_3D('',#155559,#121261,#121262) ;
#98491=AXIS2_PLACEMENT_3D('',#155563,#121264,#121265) ;
#98492=AXIS2_PLACEMENT_3D('',#155567,#121267,#121268) ;
#98493=AXIS2_PLACEMENT_3D('',#155571,#121270,#121271) ;
#98494=AXIS2_PLACEMENT_3D('',#155575,#121273,#121274) ;
#98495=AXIS2_PLACEMENT_3D('',#155579,#121276,#121277) ;
#98496=AXIS2_PLACEMENT_3D('',#155583,#121279,#121280) ;
#98497=AXIS2_PLACEMENT_3D('',#155587,#121282,#121283) ;
#98498=AXIS2_PLACEMENT_3D('',#155591,#121285,#121286) ;
#98499=AXIS2_PLACEMENT_3D('',#155595,#121288,#121289) ;
#98500=AXIS2_PLACEMENT_3D('',#155599,#121291,#121292) ;
#98501=AXIS2_PLACEMENT_3D('',#155603,#121294,#121295) ;
#98502=AXIS2_PLACEMENT_3D('',#155607,#121297,#121298) ;
#98503=AXIS2_PLACEMENT_3D('',#155611,#121300,#121301) ;
#98504=AXIS2_PLACEMENT_3D('',#155615,#121303,#121304) ;
#98505=AXIS2_PLACEMENT_3D('',#155619,#121306,#121307) ;
#98506=AXIS2_PLACEMENT_3D('',#155623,#121309,#121310) ;
#98507=AXIS2_PLACEMENT_3D('',#155627,#121312,#121313) ;
#98508=AXIS2_PLACEMENT_3D('',#155631,#121315,#121316) ;
#98509=AXIS2_PLACEMENT_3D('',#155635,#121318,#121319) ;
#98510=AXIS2_PLACEMENT_3D('',#155639,#121321,#121322) ;
#98511=AXIS2_PLACEMENT_3D('',#155643,#121324,#121325) ;
#98512=AXIS2_PLACEMENT_3D('',#155647,#121327,#121328) ;
#98513=AXIS2_PLACEMENT_3D('',#155651,#121330,#121331) ;
#98514=AXIS2_PLACEMENT_3D('',#155655,#121333,#121334) ;
#98515=AXIS2_PLACEMENT_3D('',#155659,#121336,#121337) ;
#98516=AXIS2_PLACEMENT_3D('',#155663,#121339,#121340) ;
#98517=AXIS2_PLACEMENT_3D('',#155667,#121342,#121343) ;
#98518=AXIS2_PLACEMENT_3D('',#155671,#121345,#121346) ;
#98519=AXIS2_PLACEMENT_3D('',#155675,#121348,#121349) ;
#98520=AXIS2_PLACEMENT_3D('',#155679,#121351,#121352) ;
#98521=AXIS2_PLACEMENT_3D('',#155683,#121354,#121355) ;
#98522=AXIS2_PLACEMENT_3D('',#155687,#121357,#121358) ;
#98523=AXIS2_PLACEMENT_3D('',#155689,#121360,#121361) ;
#98524=AXIS2_PLACEMENT_3D('',#155702,#121367,#121368) ;
#98525=AXIS2_PLACEMENT_3D('',#155706,#121370,#121371) ;
#98526=AXIS2_PLACEMENT_3D('',#155710,#121373,#121374) ;
#98527=AXIS2_PLACEMENT_3D('',#155713,#121376,#121377) ;
#98528=AXIS2_PLACEMENT_3D('',#155714,#121378,#121379) ;
#98529=AXIS2_PLACEMENT_3D('',#155727,#121385,#121386) ;
#98530=AXIS2_PLACEMENT_3D('',#155731,#121388,#121389) ;
#98531=AXIS2_PLACEMENT_3D('',#155735,#121391,#121392) ;
#98532=AXIS2_PLACEMENT_3D('',#155738,#121394,#121395) ;
#98533=AXIS2_PLACEMENT_3D('',#155739,#121396,#121397) ;
#98534=AXIS2_PLACEMENT_3D('',#155752,#121403,#121404) ;
#98535=AXIS2_PLACEMENT_3D('',#155756,#121406,#121407) ;
#98536=AXIS2_PLACEMENT_3D('',#155760,#121409,#121410) ;
#98537=AXIS2_PLACEMENT_3D('',#155763,#121412,#121413) ;
#98538=AXIS2_PLACEMENT_3D('',#155764,#121414,#121415) ;
#98539=AXIS2_PLACEMENT_3D('',#155777,#121421,#121422) ;
#98540=AXIS2_PLACEMENT_3D('',#155781,#121424,#121425) ;
#98541=AXIS2_PLACEMENT_3D('',#155785,#121427,#121428) ;
#98542=AXIS2_PLACEMENT_3D('',#155788,#121430,#121431) ;
#98543=AXIS2_PLACEMENT_3D('',#155789,#121432,#121433) ;
#98544=AXIS2_PLACEMENT_3D('',#155802,#121439,#121440) ;
#98545=AXIS2_PLACEMENT_3D('',#155806,#121442,#121443) ;
#98546=AXIS2_PLACEMENT_3D('',#155810,#121445,#121446) ;
#98547=AXIS2_PLACEMENT_3D('',#155813,#121448,#121449) ;
#98548=AXIS2_PLACEMENT_3D('',#155814,#121450,#121451) ;
#98549=AXIS2_PLACEMENT_3D('',#155827,#121457,#121458) ;
#98550=AXIS2_PLACEMENT_3D('',#155831,#121460,#121461) ;
#98551=AXIS2_PLACEMENT_3D('',#155835,#121463,#121464) ;
#98552=AXIS2_PLACEMENT_3D('',#155838,#121466,#121467) ;
#98553=AXIS2_PLACEMENT_3D('',#155839,#121468,#121469) ;
#98554=AXIS2_PLACEMENT_3D('',#155852,#121475,#121476) ;
#98555=AXIS2_PLACEMENT_3D('',#155856,#121478,#121479) ;
#98556=AXIS2_PLACEMENT_3D('',#155860,#121481,#121482) ;
#98557=AXIS2_PLACEMENT_3D('',#155863,#121484,#121485) ;
#98558=AXIS2_PLACEMENT_3D('',#155864,#121486,#121487) ;
#98559=AXIS2_PLACEMENT_3D('',#155877,#121493,#121494) ;
#98560=AXIS2_PLACEMENT_3D('',#155881,#121496,#121497) ;
#98561=AXIS2_PLACEMENT_3D('',#155885,#121499,#121500) ;
#98562=AXIS2_PLACEMENT_3D('',#155888,#121502,#121503) ;
#98563=AXIS2_PLACEMENT_3D('',#155889,#121504,#121505) ;
#98564=AXIS2_PLACEMENT_3D('',#155902,#121511,#121512) ;
#98565=AXIS2_PLACEMENT_3D('',#155906,#121514,#121515) ;
#98566=AXIS2_PLACEMENT_3D('',#155910,#121517,#121518) ;
#98567=AXIS2_PLACEMENT_3D('',#155913,#121520,#121521) ;
#98568=AXIS2_PLACEMENT_3D('',#155914,#121522,#121523) ;
#98569=AXIS2_PLACEMENT_3D('',#155916,#121525,#121526) ;
#98570=AXIS2_PLACEMENT_3D('',#155918,#121528,#121529) ;
#98571=AXIS2_PLACEMENT_3D('',#155920,#121531,#121532) ;
#98572=AXIS2_PLACEMENT_3D('',#155922,#121534,#121535) ;
#98573=AXIS2_PLACEMENT_3D('',#155924,#121537,#121538) ;
#98574=AXIS2_PLACEMENT_3D('',#155926,#121540,#121541) ;
#98575=AXIS2_PLACEMENT_3D('',#155928,#121543,#121544) ;
#98576=AXIS2_PLACEMENT_3D('',#155930,#121546,#121547) ;
#98577=AXIS2_PLACEMENT_3D('',#155932,#121549,#121550) ;
#98578=AXIS2_PLACEMENT_3D('',#155945,#121556,#121557) ;
#98579=AXIS2_PLACEMENT_3D('',#155947,#121558,#121559) ;
#98580=AXIS2_PLACEMENT_3D('',#155951,#121561,#121562) ;
#98581=AXIS2_PLACEMENT_3D('',#155953,#121563,#121564) ;
#98582=AXIS2_PLACEMENT_3D('',#155957,#121566,#121567) ;
#98583=AXIS2_PLACEMENT_3D('',#155959,#121568,#121569) ;
#98584=AXIS2_PLACEMENT_3D('',#155963,#121571,#121572) ;
#98585=AXIS2_PLACEMENT_3D('',#155965,#121573,#121574) ;
#98586=AXIS2_PLACEMENT_3D('',#155969,#121576,#121577) ;
#98587=AXIS2_PLACEMENT_3D('',#155971,#121578,#121579) ;
#98588=AXIS2_PLACEMENT_3D('',#155975,#121581,#121582) ;
#98589=AXIS2_PLACEMENT_3D('',#155977,#121583,#121584) ;
#98590=AXIS2_PLACEMENT_3D('',#155981,#121586,#121587) ;
#98591=AXIS2_PLACEMENT_3D('',#155983,#121588,#121589) ;
#98592=AXIS2_PLACEMENT_3D('',#155987,#121591,#121592) ;
#98593=AXIS2_PLACEMENT_3D('',#155989,#121593,#121594) ;
#98594=AXIS2_PLACEMENT_3D('',#155993,#121596,#121597) ;
#98595=AXIS2_PLACEMENT_3D('',#155995,#121598,#121599) ;
#98596=AXIS2_PLACEMENT_3D('',#155999,#121601,#121602) ;
#98597=AXIS2_PLACEMENT_3D('',#156001,#121603,#121604) ;
#98598=AXIS2_PLACEMENT_3D('',#156005,#121606,#121607) ;
#98599=AXIS2_PLACEMENT_3D('',#156007,#121608,#121609) ;
#98600=AXIS2_PLACEMENT_3D('',#156011,#121611,#121612) ;
#98601=AXIS2_PLACEMENT_3D('',#156013,#121613,#121614) ;
#98602=AXIS2_PLACEMENT_3D('',#156017,#121616,#121617) ;
#98603=AXIS2_PLACEMENT_3D('',#156019,#121618,#121619) ;
#98604=AXIS2_PLACEMENT_3D('',#156023,#121621,#121622) ;
#98605=AXIS2_PLACEMENT_3D('',#156025,#121623,#121624) ;
#98606=AXIS2_PLACEMENT_3D('',#156029,#121626,#121627) ;
#98607=AXIS2_PLACEMENT_3D('',#156031,#121628,#121629) ;
#98608=AXIS2_PLACEMENT_3D('',#156035,#121631,#121632) ;
#98609=AXIS2_PLACEMENT_3D('',#156037,#121633,#121634) ;
#98610=AXIS2_PLACEMENT_3D('',#156041,#121636,#121637) ;
#98611=AXIS2_PLACEMENT_3D('',#156043,#121638,#121639) ;
#98612=AXIS2_PLACEMENT_3D('',#156047,#121641,#121642) ;
#98613=AXIS2_PLACEMENT_3D('',#156049,#121643,#121644) ;
#98614=AXIS2_PLACEMENT_3D('',#156053,#121646,#121647) ;
#98615=AXIS2_PLACEMENT_3D('',#156055,#121648,#121649) ;
#98616=AXIS2_PLACEMENT_3D('',#156059,#121651,#121652) ;
#98617=AXIS2_PLACEMENT_3D('',#156060,#121653,#121654) ;
#98618=AXIS2_PLACEMENT_3D('',#156061,#121655,#121656) ;
#98619=AXIS2_PLACEMENT_3D('',#156064,#121657,#121658) ;
#98620=AXIS2_PLACEMENT_3D('',#156076,#121664,#121665) ;
#98621=AXIS2_PLACEMENT_3D('',#156077,#121666,#121667) ;
#98622=AXIS2_PLACEMENT_3D('',#156078,#121668,#121669) ;
#98623=AXIS2_PLACEMENT_3D('',#156081,#121670,#121671) ;
#98624=AXIS2_PLACEMENT_3D('',#156093,#121677,#121678) ;
#98625=AXIS2_PLACEMENT_3D('',#156094,#121679,#121680) ;
#98626=AXIS2_PLACEMENT_3D('',#156095,#121681,#121682) ;
#98627=AXIS2_PLACEMENT_3D('',#156098,#121683,#121684) ;
#98628=AXIS2_PLACEMENT_3D('',#156110,#121690,#121691) ;
#98629=AXIS2_PLACEMENT_3D('',#156111,#121692,#121693) ;
#98630=AXIS2_PLACEMENT_3D('',#156112,#121694,#121695) ;
#98631=AXIS2_PLACEMENT_3D('',#156115,#121696,#121697) ;
#98632=AXIS2_PLACEMENT_3D('',#156127,#121703,#121704) ;
#98633=AXIS2_PLACEMENT_3D('',#156128,#121705,#121706) ;
#98634=AXIS2_PLACEMENT_3D('',#156129,#121707,#121708) ;
#98635=AXIS2_PLACEMENT_3D('',#156132,#121709,#121710) ;
#98636=AXIS2_PLACEMENT_3D('',#156144,#121716,#121717) ;
#98637=AXIS2_PLACEMENT_3D('',#156145,#121718,#121719) ;
#98638=AXIS2_PLACEMENT_3D('',#156146,#121720,#121721) ;
#98639=AXIS2_PLACEMENT_3D('',#156149,#121722,#121723) ;
#98640=AXIS2_PLACEMENT_3D('',#156161,#121729,#121730) ;
#98641=AXIS2_PLACEMENT_3D('',#156162,#121731,#121732) ;
#98642=AXIS2_PLACEMENT_3D('',#156163,#121733,#121734) ;
#98643=AXIS2_PLACEMENT_3D('',#156166,#121735,#121736) ;
#98644=AXIS2_PLACEMENT_3D('',#156178,#121742,#121743) ;
#98645=AXIS2_PLACEMENT_3D('',#156179,#121744,#121745) ;
#98646=AXIS2_PLACEMENT_3D('',#156180,#121746,#121747) ;
#98647=AXIS2_PLACEMENT_3D('',#156183,#121748,#121749) ;
#98648=AXIS2_PLACEMENT_3D('',#156195,#121755,#121756) ;
#98649=AXIS2_PLACEMENT_3D('',#156196,#121757,#121758) ;
#98650=AXIS2_PLACEMENT_3D('',#156197,#121759,#121760) ;
#98651=AXIS2_PLACEMENT_3D('',#156200,#121761,#121762) ;
#98652=AXIS2_PLACEMENT_3D('',#156212,#121768,#121769) ;
#98653=AXIS2_PLACEMENT_3D('',#156213,#121770,#121771) ;
#98654=AXIS2_PLACEMENT_3D('',#156214,#121772,#121773) ;
#98655=AXIS2_PLACEMENT_3D('',#156223,#121778,#121779) ;
#98656=AXIS2_PLACEMENT_3D('',#156234,#121784,#121785) ;
#98657=AXIS2_PLACEMENT_3D('',#156238,#121787,#121788) ;
#98658=AXIS2_PLACEMENT_3D('',#156246,#121792,#121793) ;
#98659=AXIS2_PLACEMENT_3D('',#156250,#121795,#121796) ;
#98660=AXIS2_PLACEMENT_3D('',#156258,#121800,#121801) ;
#98661=AXIS2_PLACEMENT_3D('',#156262,#121803,#121804) ;
#98662=AXIS2_PLACEMENT_3D('',#156270,#121808,#121809) ;
#98663=AXIS2_PLACEMENT_3D('',#156274,#121811,#121812) ;
#98664=AXIS2_PLACEMENT_3D('',#156282,#121816,#121817) ;
#98665=AXIS2_PLACEMENT_3D('',#156286,#121819,#121820) ;
#98666=AXIS2_PLACEMENT_3D('',#156294,#121824,#121825) ;
#98667=AXIS2_PLACEMENT_3D('',#156298,#121827,#121828) ;
#98668=AXIS2_PLACEMENT_3D('',#156306,#121832,#121833) ;
#98669=AXIS2_PLACEMENT_3D('',#156310,#121835,#121836) ;
#98670=AXIS2_PLACEMENT_3D('',#156318,#121840,#121841) ;
#98671=AXIS2_PLACEMENT_3D('',#156322,#121843,#121844) ;
#98672=AXIS2_PLACEMENT_3D('',#156330,#121848,#121849) ;
#98673=AXIS2_PLACEMENT_3D('',#156334,#121851,#121852) ;
#98674=AXIS2_PLACEMENT_3D('',#156342,#121856,#121857) ;
#98675=AXIS2_PLACEMENT_3D('',#156346,#121859,#121860) ;
#98676=AXIS2_PLACEMENT_3D('',#156352,#121864,#121865) ;
#98677=AXIS2_PLACEMENT_3D('',#156356,#121867,#121868) ;
#98678=AXIS2_PLACEMENT_3D('',#156357,#121869,#121870) ;
#98679=AXIS2_PLACEMENT_3D('',#156358,#121871,#121872) ;
#98680=AXIS2_PLACEMENT_3D('',#156363,#121874,#121875) ;
#98681=AXIS2_PLACEMENT_3D('',#156364,#121876,#121877) ;
#98682=AXIS2_PLACEMENT_3D('',#156366,#121878,#121879) ;
#98683=AXIS2_PLACEMENT_3D('',#156367,#121880,#121881) ;
#98684=AXIS2_PLACEMENT_3D('',#156368,#121882,#121883) ;
#98685=AXIS2_PLACEMENT_3D('',#156513,#121928,#121929) ;
#98686=AXIS2_PLACEMENT_3D('',#156526,#121935,#121936) ;
#98687=AXIS2_PLACEMENT_3D('',#156530,#121938,#121939) ;
#98688=AXIS2_PLACEMENT_3D('',#156534,#121941,#121942) ;
#98689=AXIS2_PLACEMENT_3D('',#156537,#121944,#121945) ;
#98690=AXIS2_PLACEMENT_3D('',#156538,#121946,#121947) ;
#98691=AXIS2_PLACEMENT_3D('',#156547,#121952,#121953) ;
#98692=AXIS2_PLACEMENT_3D('',#156549,#121955,#121956) ;
#98693=AXIS2_PLACEMENT_3D('',#156560,#121961,#121962) ;
#98694=AXIS2_PLACEMENT_3D('',#156562,#121963,#121964) ;
#98695=AXIS2_PLACEMENT_3D('',#156564,#121965,#121966) ;
#98696=AXIS2_PLACEMENT_3D('',#156566,#121968,#121969) ;
#98697=AXIS2_PLACEMENT_3D('',#156575,#121974,#121975) ;
#98698=AXIS2_PLACEMENT_3D('',#156581,#121979,#121980) ;
#98699=AXIS2_PLACEMENT_3D('',#156590,#121985,#121986) ;
#98700=AXIS2_PLACEMENT_3D('',#156665,#122023,#122024) ;
#98701=AXIS2_PLACEMENT_3D('',#156669,#122026,#122027) ;
#98702=AXIS2_PLACEMENT_3D('',#156673,#122029,#122030) ;
#98703=AXIS2_PLACEMENT_3D('',#156677,#122032,#122033) ;
#98704=AXIS2_PLACEMENT_3D('',#156681,#122035,#122036) ;
#98705=AXIS2_PLACEMENT_3D('',#156685,#122038,#122039) ;
#98706=AXIS2_PLACEMENT_3D('',#156689,#122041,#122042) ;
#98707=AXIS2_PLACEMENT_3D('',#156693,#122044,#122045) ;
#98708=AXIS2_PLACEMENT_3D('',#156695,#122047,#122048) ;
#98709=AXIS2_PLACEMENT_3D('',#156704,#122052,#122053) ;
#98710=AXIS2_PLACEMENT_3D('',#156712,#122057,#122058) ;
#98711=AXIS2_PLACEMENT_3D('',#156722,#122063,#122064) ;
#98712=AXIS2_PLACEMENT_3D('',#156726,#122067,#122068) ;
#98713=AXIS2_PLACEMENT_3D('',#156739,#122074,#122075) ;
#98714=AXIS2_PLACEMENT_3D('',#156749,#122080,#122081) ;
#98715=AXIS2_PLACEMENT_3D('',#156756,#122085,#122086) ;
#98716=AXIS2_PLACEMENT_3D('',#156757,#122087,#122088) ;
#98717=AXIS2_PLACEMENT_3D('',#156766,#122093,#122094) ;
#98718=AXIS2_PLACEMENT_3D('',#156775,#122099,#122100) ;
#98719=AXIS2_PLACEMENT_3D('',#156780,#122102,#122103) ;
#98720=AXIS2_PLACEMENT_3D('',#156784,#122105,#122106) ;
#98721=AXIS2_PLACEMENT_3D('',#156787,#122108,#122109) ;
#98722=AXIS2_PLACEMENT_3D('',#156788,#122110,#122111) ;
#98723=AXIS2_PLACEMENT_3D('',#156789,#122112,#122113) ;
#98724=AXIS2_PLACEMENT_3D('',#156795,#122117,#122118) ;
#98725=AXIS2_PLACEMENT_3D('',#156804,#122123,#122124) ;
#98726=AXIS2_PLACEMENT_3D('',#156814,#122130,#122131) ;
#98727=AXIS2_PLACEMENT_3D('',#156824,#122137,#122138) ;
#98728=AXIS2_PLACEMENT_3D('',#156833,#122143,#122144) ;
#98729=AXIS2_PLACEMENT_3D('',#156842,#122149,#122150) ;
#98730=AXIS2_PLACEMENT_3D('',#156851,#122155,#122156) ;
#98731=AXIS2_PLACEMENT_3D('',#156860,#122161,#122162) ;
#98732=AXIS2_PLACEMENT_3D('',#156873,#122168,#122169) ;
#98733=AXIS2_PLACEMENT_3D('',#156877,#122171,#122172) ;
#98734=AXIS2_PLACEMENT_3D('',#156881,#122174,#122175) ;
#98735=AXIS2_PLACEMENT_3D('',#156884,#122177,#122178) ;
#98736=AXIS2_PLACEMENT_3D('',#156885,#122179,#122180) ;
#98737=AXIS2_PLACEMENT_3D('',#156891,#122184,#122185) ;
#98738=AXIS2_PLACEMENT_3D('',#156897,#122189,#122190) ;
#98739=AXIS2_PLACEMENT_3D('',#156903,#122194,#122195) ;
#98740=AXIS2_PLACEMENT_3D('',#156909,#122199,#122200) ;
#98741=AXIS2_PLACEMENT_3D('',#156918,#122205,#122206) ;
#98742=AXIS2_PLACEMENT_3D('',#156924,#122209,#122210) ;
#98743=AXIS2_PLACEMENT_3D('',#156929,#122213,#122214) ;
#98744=AXIS2_PLACEMENT_3D('',#156933,#122217,#122218) ;
#98745=AXIS2_PLACEMENT_3D('',#156942,#122223,#122224) ;
#98746=AXIS2_PLACEMENT_3D('',#156945,#122225,#122226) ;
#98747=AXIS2_PLACEMENT_3D('',#156947,#122227,#122228) ;
#98748=AXIS2_PLACEMENT_3D('',#156957,#122233,#122234) ;
#98749=AXIS2_PLACEMENT_3D('',#156963,#122238,#122239) ;
#98750=AXIS2_PLACEMENT_3D('',#156972,#122244,#122245) ;
#98751=AXIS2_PLACEMENT_3D('',#156977,#122247,#122248) ;
#98752=AXIS2_PLACEMENT_3D('',#156979,#122249,#122250) ;
#98753=AXIS2_PLACEMENT_3D('',#156987,#122254,#122255) ;
#98754=AXIS2_PLACEMENT_3D('',#156993,#122259,#122260) ;
#98755=AXIS2_PLACEMENT_3D('',#156999,#122264,#122265) ;
#98756=AXIS2_PLACEMENT_3D('',#157008,#122270,#122271) ;
#98757=AXIS2_PLACEMENT_3D('',#157017,#122276,#122277) ;
#98758=AXIS2_PLACEMENT_3D('',#157022,#122279,#122280) ;
#98759=AXIS2_PLACEMENT_3D('',#157025,#122282,#122283) ;
#98760=AXIS2_PLACEMENT_3D('',#157026,#122284,#122285) ;
#98761=AXIS2_PLACEMENT_3D('',#157031,#122287,#122288) ;
#98762=AXIS2_PLACEMENT_3D('',#157039,#122293,#122294) ;
#98763=AXIS2_PLACEMENT_3D('',#157040,#122295,#122296) ;
#98764=AXIS2_PLACEMENT_3D('',#157049,#122301,#122302) ;
#98765=AXIS2_PLACEMENT_3D('',#157058,#122307,#122308) ;
#98766=AXIS2_PLACEMENT_3D('',#157067,#122313,#122314) ;
#98767=AXIS2_PLACEMENT_3D('',#157076,#122319,#122320) ;
#98768=AXIS2_PLACEMENT_3D('',#157089,#122326,#122327) ;
#98769=AXIS2_PLACEMENT_3D('',#157093,#122329,#122330) ;
#98770=AXIS2_PLACEMENT_3D('',#157097,#122332,#122333) ;
#98771=AXIS2_PLACEMENT_3D('',#157100,#122335,#122336) ;
#98772=AXIS2_PLACEMENT_3D('',#157101,#122337,#122338) ;
#98773=AXIS2_PLACEMENT_3D('',#157107,#122342,#122343) ;
#98774=AXIS2_PLACEMENT_3D('',#157113,#122347,#122348) ;
#98775=AXIS2_PLACEMENT_3D('',#157119,#122352,#122353) ;
#98776=AXIS2_PLACEMENT_3D('',#157125,#122357,#122358) ;
#98777=AXIS2_PLACEMENT_3D('',#157134,#122363,#122364) ;
#98778=AXIS2_PLACEMENT_3D('',#157136,#122366,#122367) ;
#98779=AXIS2_PLACEMENT_3D('',#157139,#122370,#122371) ;
#98780=AXIS2_PLACEMENT_3D('',#157142,#122374,#122375) ;
#98781=AXIS2_PLACEMENT_3D('',#157145,#122378,#122379) ;
#98782=AXIS2_PLACEMENT_3D('',#157146,#122380,#122381) ;
#98783=AXIS2_PLACEMENT_3D('',#157147,#122382,#122383) ;
#98784=AXIS2_PLACEMENT_3D('',#157148,#122384,#122385) ;
#98785=AXIS2_PLACEMENT_3D('',#157149,#122386,#122387) ;
#98786=AXIS2_PLACEMENT_3D('',#157155,#122391,#122392) ;
#98787=AXIS2_PLACEMENT_3D('',#157161,#122396,#122397) ;
#98788=AXIS2_PLACEMENT_3D('',#157162,#122398,#122399) ;
#98789=AXIS2_PLACEMENT_3D('',#157163,#122400,#122401) ;
#98790=AXIS2_PLACEMENT_3D('',#157164,#122402,#122403) ;
#98791=AXIS2_PLACEMENT_3D('',#157165,#122404,#122405) ;
#98792=AXIS2_PLACEMENT_3D('',#157170,#122407,#122408) ;
#98793=AXIS2_PLACEMENT_3D('',#157173,#122410,#122411) ;
#98794=AXIS2_PLACEMENT_3D('',#157174,#122412,#122413) ;
#98795=AXIS2_PLACEMENT_3D('',#157180,#122417,#122418) ;
#98796=AXIS2_PLACEMENT_3D('',#157182,#122419,#122420) ;
#98797=AXIS2_PLACEMENT_3D('',#157185,#122422,#122423) ;
#98798=AXIS2_PLACEMENT_3D('',#157186,#122424,#122425) ;
#98799=AXIS2_PLACEMENT_3D('',#157192,#122429,#122430) ;
#98800=AXIS2_PLACEMENT_3D('',#157194,#122431,#122432) ;
#98801=AXIS2_PLACEMENT_3D('',#157197,#122434,#122435) ;
#98802=AXIS2_PLACEMENT_3D('',#157198,#122436,#122437) ;
#98803=AXIS2_PLACEMENT_3D('',#157204,#122441,#122442) ;
#98804=AXIS2_PLACEMENT_3D('',#157206,#122443,#122444) ;
#98805=AXIS2_PLACEMENT_3D('',#157209,#122446,#122447) ;
#98806=AXIS2_PLACEMENT_3D('',#157210,#122448,#122449) ;
#98807=AXIS2_PLACEMENT_3D('',#157213,#122452,#122453) ;
#98808=AXIS2_PLACEMENT_3D('',#157222,#122458,#122459) ;
#98809=AXIS2_PLACEMENT_3D('',#157223,#122460,#122461) ;
#98810=AXIS2_PLACEMENT_3D('',#157224,#122462,#122463) ;
#98811=AXIS2_PLACEMENT_3D('',#157225,#122464,#122465) ;
#98812=AXIS2_PLACEMENT_3D('',#157226,#122466,#122467) ;
#98813=AXIS2_PLACEMENT_3D('',#157227,#122468,#122469) ;
#98814=AXIS2_PLACEMENT_3D('',#157228,#122470,#122471) ;
#98815=AXIS2_PLACEMENT_3D('',#157229,#122472,#122473) ;
#98816=AXIS2_PLACEMENT_3D('',#157230,#122474,#122475) ;
#98817=AXIS2_PLACEMENT_3D('',#157231,#122476,#122477) ;
#98818=AXIS2_PLACEMENT_3D('',#157232,#122478,#122479) ;
#98819=AXIS2_PLACEMENT_3D('',#157233,#122480,#122481) ;
#98820=AXIS2_PLACEMENT_3D('',#157234,#122482,#122483) ;
#98821=AXIS2_PLACEMENT_3D('',#157235,#122484,#122485) ;
#98822=AXIS2_PLACEMENT_3D('',#157236,#122486,#122487) ;
#98823=AXIS2_PLACEMENT_3D('',#157237,#122488,#122489) ;
#98824=AXIS2_PLACEMENT_3D('',#157238,#122490,#122491) ;
#98825=AXIS2_PLACEMENT_3D('',#157239,#122492,#122493) ;
#98826=AXIS2_PLACEMENT_3D('',#157240,#122494,#122495) ;
#98827=AXIS2_PLACEMENT_3D('',#157241,#122496,#122497) ;
#98828=AXIS2_PLACEMENT_3D('',#157243,#122498,#122499) ;
#98829=AXIS2_PLACEMENT_3D('',#157245,#122500,#122501) ;
#98830=AXIS2_PLACEMENT_3D('',#157246,#122502,#122503) ;
#98831=AXIS2_PLACEMENT_3D('',#157247,#122504,#122505) ;
#98832=AXIS2_PLACEMENT_3D('',#157248,#122506,#122507) ;
#98833=AXIS2_PLACEMENT_3D('',#157249,#122508,#122509) ;
#98834=AXIS2_PLACEMENT_3D('',#157250,#122510,#122511) ;
#98835=AXIS2_PLACEMENT_3D('',#157251,#122512,#122513) ;
#98836=AXIS2_PLACEMENT_3D('',#157252,#122514,#122515) ;
#98837=AXIS2_PLACEMENT_3D('',#157253,#122516,#122517) ;
#98838=AXIS2_PLACEMENT_3D('',#157254,#122518,#122519) ;
#98839=AXIS2_PLACEMENT_3D('',#157255,#122520,#122521) ;
#98840=AXIS2_PLACEMENT_3D('',#157256,#122522,#122523) ;
#98841=AXIS2_PLACEMENT_3D('',#157257,#122524,#122525) ;
#98842=AXIS2_PLACEMENT_3D('',#157258,#122526,#122527) ;
#98843=AXIS2_PLACEMENT_3D('',#157260,#122528,#122529) ;
#98844=AXIS2_PLACEMENT_3D('',#157262,#122530,#122531) ;
#98845=AXIS2_PLACEMENT_3D('',#157263,#122532,#122533) ;
#98846=AXIS2_PLACEMENT_3D('',#157264,#122534,#122535) ;
#98847=AXIS2_PLACEMENT_3D('',#157265,#122536,#122537) ;
#98848=AXIS2_PLACEMENT_3D('',#157266,#122538,#122539) ;
#98849=AXIS2_PLACEMENT_3D('',#157267,#122540,#122541) ;
#98850=AXIS2_PLACEMENT_3D('',#157268,#122542,#122543) ;
#98851=AXIS2_PLACEMENT_3D('',#157269,#122544,#122545) ;
#98852=AXIS2_PLACEMENT_3D('',#157270,#122546,#122547) ;
#98853=AXIS2_PLACEMENT_3D('',#157271,#122548,#122549) ;
#98854=AXIS2_PLACEMENT_3D('',#157272,#122550,#122551) ;
#98855=AXIS2_PLACEMENT_3D('',#157273,#122552,#122553) ;
#98856=AXIS2_PLACEMENT_3D('',#157274,#122554,#122555) ;
#98857=AXIS2_PLACEMENT_3D('',#157275,#122556,#122557) ;
#98858=AXIS2_PLACEMENT_3D('',#157276,#122558,#122559) ;
#98859=AXIS2_PLACEMENT_3D('',#157277,#122560,#122561) ;
#98860=AXIS2_PLACEMENT_3D('',#157278,#122562,#122563) ;
#98861=AXIS2_PLACEMENT_3D('',#157279,#122564,#122565) ;
#98862=AXIS2_PLACEMENT_3D('',#157280,#122566,#122567) ;
#98863=AXIS2_PLACEMENT_3D('',#157282,#122568,#122569) ;
#98864=AXIS2_PLACEMENT_3D('',#157283,#122570,#122571) ;
#98865=AXIS2_PLACEMENT_3D('',#157284,#122572,#122573) ;
#98866=AXIS2_PLACEMENT_3D('',#157285,#122574,#122575) ;
#98867=AXIS2_PLACEMENT_3D('',#157286,#122576,#122577) ;
#98868=AXIS2_PLACEMENT_3D('',#157287,#122578,#122579) ;
#98869=AXIS2_PLACEMENT_3D('',#157288,#122580,#122581) ;
#98870=AXIS2_PLACEMENT_3D('',#157290,#122582,#122583) ;
#98871=AXIS2_PLACEMENT_3D('',#157291,#122584,#122585) ;
#98872=AXIS2_PLACEMENT_3D('',#157292,#122586,#122587) ;
#98873=AXIS2_PLACEMENT_3D('',#157293,#122588,#122589) ;
#98874=AXIS2_PLACEMENT_3D('',#157294,#122590,#122591) ;
#98875=AXIS2_PLACEMENT_3D('',#157296,#122592,#122593) ;
#98876=AXIS2_PLACEMENT_3D('',#157298,#122594,#122595) ;
#98877=AXIS2_PLACEMENT_3D('',#157299,#122596,#122597) ;
#98878=AXIS2_PLACEMENT_3D('',#157300,#122598,#122599) ;
#98879=AXIS2_PLACEMENT_3D('',#157301,#122600,#122601) ;
#98880=AXIS2_PLACEMENT_3D('',#157302,#122602,#122603) ;
#98881=AXIS2_PLACEMENT_3D('',#157303,#122604,#122605) ;
#98882=AXIS2_PLACEMENT_3D('',#157304,#122606,#122607) ;
#98883=AXIS2_PLACEMENT_3D('',#157305,#122608,#122609) ;
#98884=AXIS2_PLACEMENT_3D('',#157306,#122610,#122611) ;
#98885=AXIS2_PLACEMENT_3D('',#157307,#122612,#122613) ;
#98886=AXIS2_PLACEMENT_3D('',#157308,#122614,#122615) ;
#98887=AXIS2_PLACEMENT_3D('',#157309,#122616,#122617) ;
#98888=AXIS2_PLACEMENT_3D('',#157310,#122618,#122619) ;
#98889=AXIS2_PLACEMENT_3D('',#157311,#122620,#122621) ;
#98890=AXIS2_PLACEMENT_3D('',#157312,#122622,#122623) ;
#98891=AXIS2_PLACEMENT_3D('',#157313,#122624,#122625) ;
#98892=AXIS2_PLACEMENT_3D('',#157314,#122626,#122627) ;
#98893=AXIS2_PLACEMENT_3D('',#157315,#122628,#122629) ;
#98894=AXIS2_PLACEMENT_3D('',#157316,#122630,#122631) ;
#98895=AXIS2_PLACEMENT_3D('',#157317,#122632,#122633) ;
#98896=AXIS2_PLACEMENT_3D('',#157318,#122634,#122635) ;
#98897=AXIS2_PLACEMENT_3D('',#157319,#122636,#122637) ;
#98898=AXIS2_PLACEMENT_3D('',#157320,#122638,#122639) ;
#98899=AXIS2_PLACEMENT_3D('',#157321,#122640,#122641) ;
#98900=AXIS2_PLACEMENT_3D('',#157322,#122642,#122643) ;
#98901=AXIS2_PLACEMENT_3D('',#157323,#122644,#122645) ;
#98902=AXIS2_PLACEMENT_3D('',#157324,#122646,#122647) ;
#98903=AXIS2_PLACEMENT_3D('',#157325,#122648,#122649) ;
#98904=AXIS2_PLACEMENT_3D('',#157326,#122650,#122651) ;
#98905=AXIS2_PLACEMENT_3D('',#157327,#122652,#122653) ;
#98906=AXIS2_PLACEMENT_3D('',#157328,#122654,#122655) ;
#98907=AXIS2_PLACEMENT_3D('',#157329,#122656,#122657) ;
#98908=AXIS2_PLACEMENT_3D('',#157330,#122658,#122659) ;
#98909=AXIS2_PLACEMENT_3D('',#157331,#122660,#122661) ;
#98910=AXIS2_PLACEMENT_3D('',#157332,#122662,#122663) ;
#98911=AXIS2_PLACEMENT_3D('',#157333,#122664,#122665) ;
#98912=AXIS2_PLACEMENT_3D('',#157334,#122666,#122667) ;
#98913=AXIS2_PLACEMENT_3D('',#157335,#122668,#122669) ;
#98914=AXIS2_PLACEMENT_3D('',#157336,#122670,#122671) ;
#98915=AXIS2_PLACEMENT_3D('',#157337,#122672,#122673) ;
#98916=AXIS2_PLACEMENT_3D('',#157338,#122674,#122675) ;
#98917=AXIS2_PLACEMENT_3D('',#157339,#122676,#122677) ;
#98918=AXIS2_PLACEMENT_3D('',#157340,#122678,#122679) ;
#98919=AXIS2_PLACEMENT_3D('',#157341,#122680,#122681) ;
#98920=AXIS2_PLACEMENT_3D('',#157342,#122682,#122683) ;
#98921=AXIS2_PLACEMENT_3D('',#157343,#122684,#122685) ;
#98922=AXIS2_PLACEMENT_3D('',#157344,#122686,#122687) ;
#98923=AXIS2_PLACEMENT_3D('',#157345,#122688,#122689) ;
#98924=AXIS2_PLACEMENT_3D('',#157346,#122690,#122691) ;
#98925=AXIS2_PLACEMENT_3D('',#157347,#122692,#122693) ;
#98926=AXIS2_PLACEMENT_3D('',#157348,#122694,#122695) ;
#98927=AXIS2_PLACEMENT_3D('',#157349,#122696,#122697) ;
#98928=AXIS2_PLACEMENT_3D('',#157350,#122698,#122699) ;
#98929=AXIS2_PLACEMENT_3D('',#157351,#122700,#122701) ;
#98930=AXIS2_PLACEMENT_3D('',#157352,#122702,#122703) ;
#98931=AXIS2_PLACEMENT_3D('',#157353,#122704,#122705) ;
#98932=AXIS2_PLACEMENT_3D('',#157354,#122706,#122707) ;
#98933=AXIS2_PLACEMENT_3D('',#157355,#122708,#122709) ;
#98934=AXIS2_PLACEMENT_3D('',#157356,#122710,#122711) ;
#98935=AXIS2_PLACEMENT_3D('',#157357,#122712,#122713) ;
#98936=AXIS2_PLACEMENT_3D('',#157358,#122714,#122715) ;
#98937=AXIS2_PLACEMENT_3D('',#157359,#122716,#122717) ;
#98938=AXIS2_PLACEMENT_3D('',#157360,#122718,#122719) ;
#98939=AXIS2_PLACEMENT_3D('',#157361,#122720,#122721) ;
#98940=AXIS2_PLACEMENT_3D('',#157362,#122722,#122723) ;
#98941=AXIS2_PLACEMENT_3D('',#157363,#122724,#122725) ;
#98942=AXIS2_PLACEMENT_3D('',#157364,#122726,#122727) ;
#98943=AXIS2_PLACEMENT_3D('',#157365,#122728,#122729) ;
#98944=AXIS2_PLACEMENT_3D('',#157366,#122730,#122731) ;
#98945=AXIS2_PLACEMENT_3D('',#157367,#122732,#122733) ;
#98946=AXIS2_PLACEMENT_3D('',#157368,#122734,#122735) ;
#98947=AXIS2_PLACEMENT_3D('',#157369,#122736,#122737) ;
#98948=AXIS2_PLACEMENT_3D('',#157370,#122738,#122739) ;
#98949=AXIS2_PLACEMENT_3D('',#157371,#122740,#122741) ;
#98950=AXIS2_PLACEMENT_3D('',#157372,#122742,#122743) ;
#98951=AXIS2_PLACEMENT_3D('',#157373,#122744,#122745) ;
#98952=AXIS2_PLACEMENT_3D('',#157374,#122746,#122747) ;
#98953=AXIS2_PLACEMENT_3D('',#157375,#122748,#122749) ;
#98954=AXIS2_PLACEMENT_3D('',#157376,#122750,#122751) ;
#98955=AXIS2_PLACEMENT_3D('',#157377,#122752,#122753) ;
#98956=AXIS2_PLACEMENT_3D('',#157378,#122754,#122755) ;
#98957=AXIS2_PLACEMENT_3D('',#157379,#122756,#122757) ;
#98958=AXIS2_PLACEMENT_3D('',#157380,#122758,#122759) ;
#98959=AXIS2_PLACEMENT_3D('',#157381,#122760,#122761) ;
#98960=AXIS2_PLACEMENT_3D('',#157382,#122762,#122763) ;
#98961=AXIS2_PLACEMENT_3D('',#157383,#122764,#122765) ;
#98962=AXIS2_PLACEMENT_3D('',#157384,#122766,#122767) ;
#98963=AXIS2_PLACEMENT_3D('',#157385,#122768,#122769) ;
#98964=AXIS2_PLACEMENT_3D('',#157386,#122770,#122771) ;
#98965=AXIS2_PLACEMENT_3D('',#157387,#122772,#122773) ;
#98966=AXIS2_PLACEMENT_3D('',#157388,#122774,#122775) ;
#98967=AXIS2_PLACEMENT_3D('',#157389,#122776,#122777) ;
#98968=AXIS2_PLACEMENT_3D('',#157390,#122778,#122779) ;
#98969=AXIS2_PLACEMENT_3D('',#157391,#122780,#122781) ;
#98970=AXIS2_PLACEMENT_3D('',#157392,#122782,#122783) ;
#98971=AXIS2_PLACEMENT_3D('',#157393,#122784,#122785) ;
#98972=AXIS2_PLACEMENT_3D('',#157394,#122786,#122787) ;
#98973=AXIS2_PLACEMENT_3D('',#157395,#122788,#122789) ;
#98974=AXIS2_PLACEMENT_3D('',#157396,#122790,#122791) ;
#98975=AXIS2_PLACEMENT_3D('',#157397,#122792,#122793) ;
#98976=AXIS2_PLACEMENT_3D('',#157398,#122794,#122795) ;
#98977=AXIS2_PLACEMENT_3D('',#157399,#122796,#122797) ;
#98978=AXIS2_PLACEMENT_3D('',#157400,#122798,#122799) ;
#98979=AXIS2_PLACEMENT_3D('',#157401,#122800,#122801) ;
#98980=AXIS2_PLACEMENT_3D('',#157402,#122802,#122803) ;
#98981=AXIS2_PLACEMENT_3D('',#157403,#122804,#122805) ;
#98982=AXIS2_PLACEMENT_3D('',#157404,#122806,#122807) ;
#98983=AXIS2_PLACEMENT_3D('',#157405,#122808,#122809) ;
#98984=AXIS2_PLACEMENT_3D('',#157406,#122810,#122811) ;
#98985=AXIS2_PLACEMENT_3D('',#157407,#122812,#122813) ;
#98986=AXIS2_PLACEMENT_3D('',#157408,#122814,#122815) ;
#98987=AXIS2_PLACEMENT_3D('',#157409,#122816,#122817) ;
#98988=AXIS2_PLACEMENT_3D('',#157410,#122818,#122819) ;
#98989=AXIS2_PLACEMENT_3D('',#157411,#122820,#122821) ;
#98990=AXIS2_PLACEMENT_3D('',#157412,#122822,#122823) ;
#98991=AXIS2_PLACEMENT_3D('',#157413,#122824,#122825) ;
#98992=AXIS2_PLACEMENT_3D('',#157414,#122826,#122827) ;
#98993=AXIS2_PLACEMENT_3D('',#157415,#122828,#122829) ;
#98994=AXIS2_PLACEMENT_3D('',#157416,#122830,#122831) ;
#98995=AXIS2_PLACEMENT_3D('',#157417,#122832,#122833) ;
#98996=AXIS2_PLACEMENT_3D('',#157418,#122834,#122835) ;
#98997=AXIS2_PLACEMENT_3D('',#157419,#122836,#122837) ;
#98998=AXIS2_PLACEMENT_3D('',#157420,#122838,#122839) ;
#98999=AXIS2_PLACEMENT_3D('',#157421,#122840,#122841) ;
#99000=AXIS2_PLACEMENT_3D('',#157422,#122842,#122843) ;
#99001=AXIS2_PLACEMENT_3D('',#157423,#122844,#122845) ;
#99002=AXIS2_PLACEMENT_3D('',#157424,#122846,#122847) ;
#99003=AXIS2_PLACEMENT_3D('',#157425,#122848,#122849) ;
#99004=AXIS2_PLACEMENT_3D('',#157426,#122850,#122851) ;
#99005=AXIS2_PLACEMENT_3D('',#157427,#122852,#122853) ;
#99006=AXIS2_PLACEMENT_3D('',#157428,#122854,#122855) ;
#99007=AXIS2_PLACEMENT_3D('',#157429,#122856,#122857) ;
#99008=AXIS2_PLACEMENT_3D('',#157430,#122858,#122859) ;
#99009=AXIS2_PLACEMENT_3D('',#157431,#122860,#122861) ;
#99010=AXIS2_PLACEMENT_3D('',#157432,#122862,#122863) ;
#99011=AXIS2_PLACEMENT_3D('',#157433,#122864,#122865) ;
#99012=AXIS2_PLACEMENT_3D('',#157434,#122866,#122867) ;
#99013=AXIS2_PLACEMENT_3D('',#157435,#122868,#122869) ;
#99014=AXIS2_PLACEMENT_3D('',#157436,#122870,#122871) ;
#99015=AXIS2_PLACEMENT_3D('',#157437,#122872,#122873) ;
#99016=AXIS2_PLACEMENT_3D('',#157438,#122874,#122875) ;
#99017=AXIS2_PLACEMENT_3D('',#157439,#122876,#122877) ;
#99018=AXIS2_PLACEMENT_3D('',#157440,#122878,#122879) ;
#99019=AXIS2_PLACEMENT_3D('',#157441,#122880,#122881) ;
#99020=AXIS2_PLACEMENT_3D('',#157442,#122882,#122883) ;
#99021=AXIS2_PLACEMENT_3D('',#157443,#122884,#122885) ;
#99022=AXIS2_PLACEMENT_3D('',#157444,#122886,#122887) ;
#99023=AXIS2_PLACEMENT_3D('',#157445,#122888,#122889) ;
#99024=AXIS2_PLACEMENT_3D('',#157446,#122890,#122891) ;
#99025=AXIS2_PLACEMENT_3D('',#157447,#122892,#122893) ;
#99026=AXIS2_PLACEMENT_3D('',#157448,#122894,#122895) ;
#99027=AXIS2_PLACEMENT_3D('',#157449,#122896,#122897) ;
#99028=AXIS2_PLACEMENT_3D('',#157450,#122898,#122899) ;
#99029=AXIS2_PLACEMENT_3D('',#157451,#122900,#122901) ;
#99030=AXIS2_PLACEMENT_3D('',#157452,#122902,#122903) ;
#99031=AXIS2_PLACEMENT_3D('',#157453,#122904,#122905) ;
#99032=AXIS2_PLACEMENT_3D('',#157454,#122906,#122907) ;
#99033=AXIS2_PLACEMENT_3D('',#157455,#122908,#122909) ;
#99034=AXIS2_PLACEMENT_3D('',#157456,#122910,#122911) ;
#99035=AXIS2_PLACEMENT_3D('',#157457,#122912,#122913) ;
#99036=AXIS2_PLACEMENT_3D('',#157458,#122914,#122915) ;
#99037=AXIS2_PLACEMENT_3D('',#157459,#122916,#122917) ;
#99038=AXIS2_PLACEMENT_3D('',#157460,#122918,#122919) ;
#99039=AXIS2_PLACEMENT_3D('',#157461,#122920,#122921) ;
#99040=AXIS2_PLACEMENT_3D('',#157462,#122922,#122923) ;
#99041=AXIS2_PLACEMENT_3D('',#157463,#122924,#122925) ;
#99042=AXIS2_PLACEMENT_3D('',#157464,#122926,#122927) ;
#99043=AXIS2_PLACEMENT_3D('',#157465,#122928,#122929) ;
#99044=AXIS2_PLACEMENT_3D('',#157466,#122930,#122931) ;
#99045=AXIS2_PLACEMENT_3D('',#157467,#122932,#122933) ;
#99046=AXIS2_PLACEMENT_3D('',#157468,#122934,#122935) ;
#99047=AXIS2_PLACEMENT_3D('',#157469,#122936,#122937) ;
#99048=AXIS2_PLACEMENT_3D('',#157470,#122938,#122939) ;
#99049=AXIS2_PLACEMENT_3D('',#157471,#122940,#122941) ;
#99050=AXIS2_PLACEMENT_3D('',#157472,#122942,#122943) ;
#99051=AXIS2_PLACEMENT_3D('',#157473,#122944,#122945) ;
#99052=AXIS2_PLACEMENT_3D('',#157474,#122946,#122947) ;
#99053=AXIS2_PLACEMENT_3D('',#157475,#122948,#122949) ;
#99054=AXIS2_PLACEMENT_3D('',#157476,#122950,#122951) ;
#99055=AXIS2_PLACEMENT_3D('',#157477,#122952,#122953) ;
#99056=AXIS2_PLACEMENT_3D('',#157478,#122954,#122955) ;
#99057=AXIS2_PLACEMENT_3D('',#157485,#122956,#122957) ;
#99058=AXIS2_PLACEMENT_3D('',#157486,#122958,#122959) ;
#99059=AXIS2_PLACEMENT_3D('',#157487,#122960,#122961) ;
#99060=AXIS2_PLACEMENT_3D('',#157488,#122962,#122963) ;
#99061=AXIS2_PLACEMENT_3D('',#157507,#122964,#122965) ;
#99062=AXIS2_PLACEMENT_3D('',#157508,#122966,#122967) ;
#99063=AXIS2_PLACEMENT_3D('',#157509,#122968,#122969) ;
#99064=AXIS2_PLACEMENT_3D('',#157510,#122970,#122971) ;
#99065=AXIS2_PLACEMENT_3D('',#157511,#122972,#122973) ;
#99066=AXIS2_PLACEMENT_3D('',#157512,#122974,#122975) ;
#99067=AXIS2_PLACEMENT_3D('',#157513,#122976,#122977) ;
#99068=AXIS2_PLACEMENT_3D('',#157520,#122978,#122979) ;
#99069=AXIS2_PLACEMENT_3D('',#157521,#122980,#122981) ;
#99070=AXIS2_PLACEMENT_3D('',#157522,#122982,#122983) ;
#99071=AXIS2_PLACEMENT_3D('',#157523,#122984,#122985) ;
#99072=AXIS2_PLACEMENT_3D('',#157524,#122986,#122987) ;
#99073=AXIS2_PLACEMENT_3D('',#157525,#122988,#122989) ;
#99074=AXIS2_PLACEMENT_3D('',#157526,#122990,#122991) ;
#99075=AXIS2_PLACEMENT_3D('',#157527,#122992,#122993) ;
#99076=AXIS2_PLACEMENT_3D('',#157528,#122994,#122995) ;
#99077=AXIS2_PLACEMENT_3D('',#157547,#122996,#122997) ;
#99078=AXIS2_PLACEMENT_3D('',#157566,#122998,#122999) ;
#99079=AXIS2_PLACEMENT_3D('',#157567,#123000,#123001) ;
#99080=AXIS2_PLACEMENT_3D('',#157568,#123002,#123003) ;
#99081=AXIS2_PLACEMENT_3D('',#157569,#123004,#123005) ;
#99082=AXIS2_PLACEMENT_3D('',#157570,#123006,#123007) ;
#99083=AXIS2_PLACEMENT_3D('',#157571,#123008,#123009) ;
#99084=AXIS2_PLACEMENT_3D('',#157572,#123010,#123011) ;
#99085=AXIS2_PLACEMENT_3D('',#157573,#123012,#123013) ;
#99086=AXIS2_PLACEMENT_3D('',#157574,#123014,#123015) ;
#99087=AXIS2_PLACEMENT_3D('',#157575,#123016,#123017) ;
#99088=AXIS2_PLACEMENT_3D('',#157576,#123018,#123019) ;
#99089=AXIS2_PLACEMENT_3D('',#157595,#123020,#123021) ;
#99090=AXIS2_PLACEMENT_3D('',#157596,#123022,#123023) ;
#99091=AXIS2_PLACEMENT_3D('',#157597,#123024,#123025) ;
#99092=AXIS2_PLACEMENT_3D('',#157598,#123026,#123027) ;
#99093=AXIS2_PLACEMENT_3D('',#157599,#123028,#123029) ;
#99094=AXIS2_PLACEMENT_3D('',#157600,#123030,#123031) ;
#99095=AXIS2_PLACEMENT_3D('',#157601,#123032,#123033) ;
#99096=AXIS2_PLACEMENT_3D('',#157602,#123034,#123035) ;
#99097=AXIS2_PLACEMENT_3D('',#157603,#123036,#123037) ;
#99098=AXIS2_PLACEMENT_3D('',#157604,#123038,#123039) ;
#99099=AXIS2_PLACEMENT_3D('',#157605,#123040,#123041) ;
#99100=AXIS2_PLACEMENT_3D('',#157606,#123042,#123043) ;
#99101=AXIS2_PLACEMENT_3D('',#157607,#123044,#123045) ;
#99102=AXIS2_PLACEMENT_3D('',#157608,#123046,#123047) ;
#99103=AXIS2_PLACEMENT_3D('',#157609,#123048,#123049) ;
#99104=AXIS2_PLACEMENT_3D('',#157610,#123050,#123051) ;
#99105=AXIS2_PLACEMENT_3D('',#157611,#123052,#123053) ;
#99106=AXIS2_PLACEMENT_3D('',#157612,#123054,#123055) ;
#99107=AXIS2_PLACEMENT_3D('',#157613,#123056,#123057) ;
#99108=AXIS2_PLACEMENT_3D('',#157614,#123058,#123059) ;
#99109=AXIS2_PLACEMENT_3D('',#157615,#123060,#123061) ;
#99110=AXIS2_PLACEMENT_3D('',#157616,#123062,#123063) ;
#99111=AXIS2_PLACEMENT_3D('',#157617,#123064,#123065) ;
#99112=AXIS2_PLACEMENT_3D('',#157618,#123066,#123067) ;
#99113=AXIS2_PLACEMENT_3D('',#157619,#123068,#123069) ;
#99114=AXIS2_PLACEMENT_3D('',#157620,#123070,#123071) ;
#99115=AXIS2_PLACEMENT_3D('',#157621,#123072,#123073) ;
#99116=AXIS2_PLACEMENT_3D('',#157622,#123074,#123075) ;
#99117=AXIS2_PLACEMENT_3D('',#157623,#123076,#123077) ;
#99118=AXIS2_PLACEMENT_3D('',#157624,#123078,#123079) ;
#99119=AXIS2_PLACEMENT_3D('',#157625,#123080,#123081) ;
#99120=AXIS2_PLACEMENT_3D('',#157626,#123082,#123083) ;
#99121=AXIS2_PLACEMENT_3D('',#157627,#123084,#123085) ;
#99122=AXIS2_PLACEMENT_3D('',#157628,#123086,#123087) ;
#99123=AXIS2_PLACEMENT_3D('',#157629,#123088,#123089) ;
#99124=AXIS2_PLACEMENT_3D('',#157630,#123090,#123091) ;
#99125=AXIS2_PLACEMENT_3D('',#157631,#123092,#123093) ;
#99126=AXIS2_PLACEMENT_3D('',#157632,#123094,#123095) ;
#99127=AXIS2_PLACEMENT_3D('',#157633,#123096,#123097) ;
#99128=AXIS2_PLACEMENT_3D('',#157634,#123098,#123099) ;
#99129=AXIS2_PLACEMENT_3D('',#157635,#123100,#123101) ;
#99130=AXIS2_PLACEMENT_3D('',#157636,#123102,#123103) ;
#99131=AXIS2_PLACEMENT_3D('',#157637,#123104,#123105) ;
#99132=AXIS2_PLACEMENT_3D('',#157638,#123106,#123107) ;
#99133=AXIS2_PLACEMENT_3D('',#157639,#123108,#123109) ;
#99134=AXIS2_PLACEMENT_3D('',#157640,#123110,#123111) ;
#99135=AXIS2_PLACEMENT_3D('',#157641,#123112,#123113) ;
#99136=AXIS2_PLACEMENT_3D('',#157642,#123114,#123115) ;
#99137=AXIS2_PLACEMENT_3D('',#157643,#123116,#123117) ;
#99138=AXIS2_PLACEMENT_3D('',#157644,#123118,#123119) ;
#99139=AXIS2_PLACEMENT_3D('',#157645,#123120,#123121) ;
#99140=AXIS2_PLACEMENT_3D('',#157646,#123122,#123123) ;
#99141=AXIS2_PLACEMENT_3D('',#157647,#123124,#123125) ;
#99142=AXIS2_PLACEMENT_3D('',#157648,#123126,#123127) ;
#99143=AXIS2_PLACEMENT_3D('',#157649,#123128,#123129) ;
#99144=AXIS2_PLACEMENT_3D('',#157650,#123130,#123131) ;
#99145=AXIS2_PLACEMENT_3D('',#157651,#123132,#123133) ;
#99146=AXIS2_PLACEMENT_3D('',#157652,#123134,#123135) ;
#99147=AXIS2_PLACEMENT_3D('',#157653,#123136,#123137) ;
#99148=AXIS2_PLACEMENT_3D('',#157654,#123138,#123139) ;
#99149=AXIS2_PLACEMENT_3D('',#157655,#123140,#123141) ;
#99150=AXIS2_PLACEMENT_3D('',#157656,#123142,#123143) ;
#99151=AXIS2_PLACEMENT_3D('',#157657,#123144,#123145) ;
#99152=AXIS2_PLACEMENT_3D('',#157658,#123146,#123147) ;
#99153=AXIS2_PLACEMENT_3D('',#157659,#123148,#123149) ;
#99154=AXIS2_PLACEMENT_3D('',#157660,#123150,#123151) ;
#99155=AXIS2_PLACEMENT_3D('',#157661,#123152,#123153) ;
#99156=AXIS2_PLACEMENT_3D('',#157662,#123154,#123155) ;
#99157=AXIS2_PLACEMENT_3D('',#157663,#123156,#123157) ;
#99158=AXIS2_PLACEMENT_3D('',#157664,#123158,#123159) ;
#99159=AXIS2_PLACEMENT_3D('',#157665,#123160,#123161) ;
#99160=AXIS2_PLACEMENT_3D('',#157666,#123162,#123163) ;
#99161=AXIS2_PLACEMENT_3D('',#157667,#123164,#123165) ;
#99162=AXIS2_PLACEMENT_3D('',#157668,#123166,#123167) ;
#99163=AXIS2_PLACEMENT_3D('',#157669,#123168,#123169) ;
#99164=AXIS2_PLACEMENT_3D('',#157670,#123170,#123171) ;
#99165=AXIS2_PLACEMENT_3D('',#157671,#123172,#123173) ;
#99166=AXIS2_PLACEMENT_3D('',#157672,#123174,#123175) ;
#99167=AXIS2_PLACEMENT_3D('',#157673,#123176,#123177) ;
#99168=AXIS2_PLACEMENT_3D('',#157674,#123178,#123179) ;
#99169=AXIS2_PLACEMENT_3D('',#157675,#123180,#123181) ;
#99170=AXIS2_PLACEMENT_3D('',#157676,#123182,#123183) ;
#99171=AXIS2_PLACEMENT_3D('',#157677,#123184,#123185) ;
#99172=AXIS2_PLACEMENT_3D('',#157678,#123186,#123187) ;
#99173=AXIS2_PLACEMENT_3D('',#157679,#123188,#123189) ;
#99174=AXIS2_PLACEMENT_3D('',#157680,#123190,#123191) ;
#99175=AXIS2_PLACEMENT_3D('',#157681,#123192,#123193) ;
#99176=AXIS2_PLACEMENT_3D('',#157682,#123194,#123195) ;
#99177=AXIS2_PLACEMENT_3D('',#157683,#123196,#123197) ;
#99178=AXIS2_PLACEMENT_3D('',#157684,#123198,#123199) ;
#99179=AXIS2_PLACEMENT_3D('',#157685,#123200,#123201) ;
#99180=AXIS2_PLACEMENT_3D('',#157686,#123202,#123203) ;
#99181=AXIS2_PLACEMENT_3D('',#157687,#123204,#123205) ;
#99182=AXIS2_PLACEMENT_3D('',#157688,#123206,#123207) ;
#99183=AXIS2_PLACEMENT_3D('',#157723,#123208,#123209) ;
#99184=AXIS2_PLACEMENT_3D('',#157724,#123210,#123211) ;
#99185=AXIS2_PLACEMENT_3D('',#157726,#123212,#123213) ;
#99186=AXIS2_PLACEMENT_3D('',#157727,#123214,#123215) ;
#99187=AXIS2_PLACEMENT_3D('',#157728,#123216,#123217) ;
#99188=AXIS2_PLACEMENT_3D('',#157755,#123218,#123219) ;
#99189=AXIS2_PLACEMENT_3D('',#157812,#123220,#123221) ;
#99190=AXIS2_PLACEMENT_3D('',#157813,#123222,#123223) ;
#99191=AXIS2_PLACEMENT_3D('',#157814,#123224,#123225) ;
#99192=AXIS2_PLACEMENT_3D('',#157815,#123226,#123227) ;
#99193=AXIS2_PLACEMENT_3D('',#157816,#123228,#123229) ;
#99194=AXIS2_PLACEMENT_3D('',#157817,#123230,#123231) ;
#99195=AXIS2_PLACEMENT_3D('',#157819,#123232,#123233) ;
#99196=AXIS2_PLACEMENT_3D('',#157846,#123234,#123235) ;
#99197=AXIS2_PLACEMENT_3D('',#157847,#123236,#123237) ;
#99198=AXIS2_PLACEMENT_3D('',#157848,#123238,#123239) ;
#99199=AXIS2_PLACEMENT_3D('',#157849,#123240,#123241) ;
#99200=AXIS2_PLACEMENT_3D('',#157850,#123242,#123243) ;
#99201=AXIS2_PLACEMENT_3D('',#157851,#123244,#123245) ;
#99202=AXIS2_PLACEMENT_3D('',#157882,#123246,#123247) ;
#99203=AXIS2_PLACEMENT_3D('',#157883,#123248,#123249) ;
#99204=AXIS2_PLACEMENT_3D('',#157884,#123250,#123251) ;
#99205=AXIS2_PLACEMENT_3D('',#157885,#123252,#123253) ;
#99206=AXIS2_PLACEMENT_3D('',#157916,#123254,#123255) ;
#99207=AXIS2_PLACEMENT_3D('',#157917,#123256,#123257) ;
#99208=AXIS2_PLACEMENT_3D('',#157918,#123258,#123259) ;
#99209=AXIS2_PLACEMENT_3D('',#157927,#123264,#123265) ;
#99210=AXIS2_PLACEMENT_3D('',#157936,#123270,#123271) ;
#99211=AXIS2_PLACEMENT_3D('',#157941,#123273,#123274) ;
#99212=AXIS2_PLACEMENT_3D('',#157945,#123276,#123277) ;
#99213=AXIS2_PLACEMENT_3D('',#157948,#123279,#123280) ;
#99214=AXIS2_PLACEMENT_3D('',#157949,#123281,#123282) ;
#99215=AXIS2_PLACEMENT_3D('',#157950,#123283,#123284) ;
#99216=AXIS2_PLACEMENT_3D('',#157956,#123288,#123289) ;
#99217=AXIS2_PLACEMENT_3D('',#157965,#123294,#123295) ;
#99218=AXIS2_PLACEMENT_3D('',#157974,#123300,#123301) ;
#99219=AXIS2_PLACEMENT_3D('',#157983,#123306,#123307) ;
#99220=AXIS2_PLACEMENT_3D('',#157988,#123309,#123310) ;
#99221=AXIS2_PLACEMENT_3D('',#157992,#123312,#123313) ;
#99222=AXIS2_PLACEMENT_3D('',#157995,#123315,#123316) ;
#99223=AXIS2_PLACEMENT_3D('',#157996,#123317,#123318) ;
#99224=AXIS2_PLACEMENT_3D('',#157997,#123319,#123320) ;
#99225=AXIS2_PLACEMENT_3D('',#158003,#123324,#123325) ;
#99226=AXIS2_PLACEMENT_3D('',#158012,#123330,#123331) ;
#99227=AXIS2_PLACEMENT_3D('',#158021,#123336,#123337) ;
#99228=AXIS2_PLACEMENT_3D('',#158030,#123342,#123343) ;
#99229=AXIS2_PLACEMENT_3D('',#158035,#123345,#123346) ;
#99230=AXIS2_PLACEMENT_3D('',#158039,#123348,#123349) ;
#99231=AXIS2_PLACEMENT_3D('',#158042,#123351,#123352) ;
#99232=AXIS2_PLACEMENT_3D('',#158043,#123353,#123354) ;
#99233=AXIS2_PLACEMENT_3D('',#158044,#123355,#123356) ;
#99234=AXIS2_PLACEMENT_3D('',#158050,#123360,#123361) ;
#99235=AXIS2_PLACEMENT_3D('',#158059,#123366,#123367) ;
#99236=AXIS2_PLACEMENT_3D('',#158068,#123372,#123373) ;
#99237=AXIS2_PLACEMENT_3D('',#158077,#123378,#123379) ;
#99238=AXIS2_PLACEMENT_3D('',#158082,#123381,#123382) ;
#99239=AXIS2_PLACEMENT_3D('',#158086,#123384,#123385) ;
#99240=AXIS2_PLACEMENT_3D('',#158089,#123387,#123388) ;
#99241=AXIS2_PLACEMENT_3D('',#158090,#123389,#123390) ;
#99242=AXIS2_PLACEMENT_3D('',#158091,#123391,#123392) ;
#99243=AXIS2_PLACEMENT_3D('',#158097,#123396,#123397) ;
#99244=AXIS2_PLACEMENT_3D('',#158106,#123402,#123403) ;
#99245=AXIS2_PLACEMENT_3D('',#158115,#123408,#123409) ;
#99246=AXIS2_PLACEMENT_3D('',#158124,#123414,#123415) ;
#99247=AXIS2_PLACEMENT_3D('',#158129,#123417,#123418) ;
#99248=AXIS2_PLACEMENT_3D('',#158133,#123420,#123421) ;
#99249=AXIS2_PLACEMENT_3D('',#158136,#123423,#123424) ;
#99250=AXIS2_PLACEMENT_3D('',#158137,#123425,#123426) ;
#99251=AXIS2_PLACEMENT_3D('',#158138,#123427,#123428) ;
#99252=AXIS2_PLACEMENT_3D('',#158144,#123432,#123433) ;
#99253=AXIS2_PLACEMENT_3D('',#158153,#123438,#123439) ;
#99254=AXIS2_PLACEMENT_3D('',#158162,#123444,#123445) ;
#99255=AXIS2_PLACEMENT_3D('',#158171,#123450,#123451) ;
#99256=AXIS2_PLACEMENT_3D('',#158176,#123453,#123454) ;
#99257=AXIS2_PLACEMENT_3D('',#158180,#123456,#123457) ;
#99258=AXIS2_PLACEMENT_3D('',#158183,#123459,#123460) ;
#99259=AXIS2_PLACEMENT_3D('',#158184,#123461,#123462) ;
#99260=AXIS2_PLACEMENT_3D('',#158185,#123463,#123464) ;
#99261=AXIS2_PLACEMENT_3D('',#158191,#123468,#123469) ;
#99262=AXIS2_PLACEMENT_3D('',#158200,#123474,#123475) ;
#99263=AXIS2_PLACEMENT_3D('',#158209,#123480,#123481) ;
#99264=AXIS2_PLACEMENT_3D('',#158218,#123486,#123487) ;
#99265=AXIS2_PLACEMENT_3D('',#158223,#123489,#123490) ;
#99266=AXIS2_PLACEMENT_3D('',#158227,#123492,#123493) ;
#99267=AXIS2_PLACEMENT_3D('',#158230,#123495,#123496) ;
#99268=AXIS2_PLACEMENT_3D('',#158231,#123497,#123498) ;
#99269=AXIS2_PLACEMENT_3D('',#158232,#123499,#123500) ;
#99270=AXIS2_PLACEMENT_3D('',#158238,#123504,#123505) ;
#99271=AXIS2_PLACEMENT_3D('',#158247,#123510,#123511) ;
#99272=AXIS2_PLACEMENT_3D('',#158256,#123516,#123517) ;
#99273=AXIS2_PLACEMENT_3D('',#158265,#123522,#123523) ;
#99274=AXIS2_PLACEMENT_3D('',#158270,#123525,#123526) ;
#99275=AXIS2_PLACEMENT_3D('',#158274,#123528,#123529) ;
#99276=AXIS2_PLACEMENT_3D('',#158277,#123531,#123532) ;
#99277=AXIS2_PLACEMENT_3D('',#158278,#123533,#123534) ;
#99278=AXIS2_PLACEMENT_3D('',#158279,#123535,#123536) ;
#99279=AXIS2_PLACEMENT_3D('',#158285,#123540,#123541) ;
#99280=AXIS2_PLACEMENT_3D('',#158294,#123546,#123547) ;
#99281=AXIS2_PLACEMENT_3D('',#158303,#123552,#123553) ;
#99282=AXIS2_PLACEMENT_3D('',#158312,#123558,#123559) ;
#99283=AXIS2_PLACEMENT_3D('',#158317,#123561,#123562) ;
#99284=AXIS2_PLACEMENT_3D('',#158321,#123564,#123565) ;
#99285=AXIS2_PLACEMENT_3D('',#158324,#123567,#123568) ;
#99286=AXIS2_PLACEMENT_3D('',#158325,#123569,#123570) ;
#99287=AXIS2_PLACEMENT_3D('',#158326,#123571,#123572) ;
#99288=AXIS2_PLACEMENT_3D('',#158332,#123576,#123577) ;
#99289=AXIS2_PLACEMENT_3D('',#158341,#123582,#123583) ;
#99290=AXIS2_PLACEMENT_3D('',#158351,#123589,#123590) ;
#99291=AXIS2_PLACEMENT_3D('',#158356,#123592,#123593) ;
#99292=AXIS2_PLACEMENT_3D('',#158364,#123598,#123599) ;
#99293=AXIS2_PLACEMENT_3D('',#158365,#123600,#123601) ;
#99294=AXIS2_PLACEMENT_3D('',#158370,#123603,#123604) ;
#99295=AXIS2_PLACEMENT_3D('',#158378,#123609,#123610) ;
#99296=AXIS2_PLACEMENT_3D('',#158379,#123611,#123612) ;
#99297=AXIS2_PLACEMENT_3D('',#158384,#123614,#123615) ;
#99298=AXIS2_PLACEMENT_3D('',#158392,#123620,#123621) ;
#99299=AXIS2_PLACEMENT_3D('',#158393,#123622,#123623) ;
#99300=AXIS2_PLACEMENT_3D('',#158398,#123625,#123626) ;
#99301=AXIS2_PLACEMENT_3D('',#158406,#123631,#123632) ;
#99302=AXIS2_PLACEMENT_3D('',#158407,#123633,#123634) ;
#99303=AXIS2_PLACEMENT_3D('',#158412,#123636,#123637) ;
#99304=AXIS2_PLACEMENT_3D('',#158420,#123642,#123643) ;
#99305=AXIS2_PLACEMENT_3D('',#158421,#123644,#123645) ;
#99306=AXIS2_PLACEMENT_3D('',#158426,#123647,#123648) ;
#99307=AXIS2_PLACEMENT_3D('',#158434,#123653,#123654) ;
#99308=AXIS2_PLACEMENT_3D('',#158435,#123655,#123656) ;
#99309=AXIS2_PLACEMENT_3D('',#158440,#123658,#123659) ;
#99310=AXIS2_PLACEMENT_3D('',#158448,#123664,#123665) ;
#99311=AXIS2_PLACEMENT_3D('',#158449,#123666,#123667) ;
#99312=AXIS2_PLACEMENT_3D('',#158454,#123669,#123670) ;
#99313=AXIS2_PLACEMENT_3D('',#158462,#123675,#123676) ;
#99314=AXIS2_PLACEMENT_3D('',#158463,#123677,#123678) ;
#99315=AXIS2_PLACEMENT_3D('',#158473,#123684,#123685) ;
#99316=AXIS2_PLACEMENT_3D('',#158478,#123687,#123688) ;
#99317=AXIS2_PLACEMENT_3D('',#158486,#123693,#123694) ;
#99318=AXIS2_PLACEMENT_3D('',#158487,#123695,#123696) ;
#99319=AXIS2_PLACEMENT_3D('',#158492,#123698,#123699) ;
#99320=AXIS2_PLACEMENT_3D('',#158500,#123704,#123705) ;
#99321=AXIS2_PLACEMENT_3D('',#158501,#123706,#123707) ;
#99322=AXIS2_PLACEMENT_3D('',#158506,#123709,#123710) ;
#99323=AXIS2_PLACEMENT_3D('',#158514,#123715,#123716) ;
#99324=AXIS2_PLACEMENT_3D('',#158515,#123717,#123718) ;
#99325=AXIS2_PLACEMENT_3D('',#158520,#123720,#123721) ;
#99326=AXIS2_PLACEMENT_3D('',#158528,#123726,#123727) ;
#99327=AXIS2_PLACEMENT_3D('',#158529,#123728,#123729) ;
#99328=AXIS2_PLACEMENT_3D('',#158534,#123731,#123732) ;
#99329=AXIS2_PLACEMENT_3D('',#158542,#123737,#123738) ;
#99330=AXIS2_PLACEMENT_3D('',#158543,#123739,#123740) ;
#99331=AXIS2_PLACEMENT_3D('',#158548,#123742,#123743) ;
#99332=AXIS2_PLACEMENT_3D('',#158556,#123748,#123749) ;
#99333=AXIS2_PLACEMENT_3D('',#158557,#123750,#123751) ;
#99334=AXIS2_PLACEMENT_3D('',#158562,#123753,#123754) ;
#99335=AXIS2_PLACEMENT_3D('',#158570,#123759,#123760) ;
#99336=AXIS2_PLACEMENT_3D('',#158571,#123761,#123762) ;
#99337=AXIS2_PLACEMENT_3D('',#158576,#123764,#123765) ;
#99338=AXIS2_PLACEMENT_3D('',#158584,#123770,#123771) ;
#99339=AXIS2_PLACEMENT_3D('',#158585,#123772,#123773) ;
#99340=AXIS2_PLACEMENT_3D('',#158594,#123778,#123779) ;
#99341=AXIS2_PLACEMENT_3D('',#158603,#123784,#123785) ;
#99342=AXIS2_PLACEMENT_3D('',#158612,#123790,#123791) ;
#99343=AXIS2_PLACEMENT_3D('',#158621,#123796,#123797) ;
#99344=AXIS2_PLACEMENT_3D('',#158630,#123802,#123803) ;
#99345=AXIS2_PLACEMENT_3D('',#158639,#123808,#123809) ;
#99346=AXIS2_PLACEMENT_3D('',#158648,#123814,#123815) ;
#99347=AXIS2_PLACEMENT_3D('',#158657,#123820,#123821) ;
#99348=AXIS2_PLACEMENT_3D('',#158666,#123826,#123827) ;
#99349=AXIS2_PLACEMENT_3D('',#158675,#123832,#123833) ;
#99350=AXIS2_PLACEMENT_3D('',#158684,#123838,#123839) ;
#99351=AXIS2_PLACEMENT_3D('',#158693,#123844,#123845) ;
#99352=AXIS2_PLACEMENT_3D('',#158702,#123850,#123851) ;
#99353=AXIS2_PLACEMENT_3D('',#158711,#123856,#123857) ;
#99354=AXIS2_PLACEMENT_3D('',#158720,#123862,#123863) ;
#99355=AXIS2_PLACEMENT_3D('',#158729,#123868,#123869) ;
#99356=AXIS2_PLACEMENT_3D('',#158738,#123874,#123875) ;
#99357=AXIS2_PLACEMENT_3D('',#158747,#123880,#123881) ;
#99358=AXIS2_PLACEMENT_3D('',#158756,#123886,#123887) ;
#99359=AXIS2_PLACEMENT_3D('',#158765,#123892,#123893) ;
#99360=AXIS2_PLACEMENT_3D('',#158774,#123898,#123899) ;
#99361=AXIS2_PLACEMENT_3D('',#158783,#123904,#123905) ;
#99362=AXIS2_PLACEMENT_3D('',#158792,#123910,#123911) ;
#99363=AXIS2_PLACEMENT_3D('',#158801,#123916,#123917) ;
#99364=AXIS2_PLACEMENT_3D('',#158810,#123922,#123923) ;
#99365=AXIS2_PLACEMENT_3D('',#158819,#123928,#123929) ;
#99366=AXIS2_PLACEMENT_3D('',#158828,#123934,#123935) ;
#99367=AXIS2_PLACEMENT_3D('',#158837,#123940,#123941) ;
#99368=AXIS2_PLACEMENT_3D('',#158846,#123946,#123947) ;
#99369=AXIS2_PLACEMENT_3D('',#158855,#123952,#123953) ;
#99370=AXIS2_PLACEMENT_3D('',#158864,#123958,#123959) ;
#99371=AXIS2_PLACEMENT_3D('',#158873,#123964,#123965) ;
#99372=AXIS2_PLACEMENT_3D('',#158882,#123970,#123971) ;
#99373=AXIS2_PLACEMENT_3D('',#158891,#123976,#123977) ;
#99374=AXIS2_PLACEMENT_3D('',#158900,#123982,#123983) ;
#99375=AXIS2_PLACEMENT_3D('',#158909,#123988,#123989) ;
#99376=AXIS2_PLACEMENT_3D('',#158922,#123995,#123996) ;
#99377=AXIS2_PLACEMENT_3D('',#158926,#123998,#123999) ;
#99378=AXIS2_PLACEMENT_3D('',#158930,#124001,#124002) ;
#99379=AXIS2_PLACEMENT_3D('',#158933,#124004,#124005) ;
#99380=AXIS2_PLACEMENT_3D('',#158934,#124006,#124007) ;
#99381=AXIS2_PLACEMENT_3D('',#158940,#124011,#124012) ;
#99382=AXIS2_PLACEMENT_3D('',#158946,#124016,#124017) ;
#99383=AXIS2_PLACEMENT_3D('',#158952,#124021,#124022) ;
#99384=AXIS2_PLACEMENT_3D('',#158958,#124026,#124027) ;
#99385=AXIS2_PLACEMENT_3D('',#158971,#124033,#124034) ;
#99386=AXIS2_PLACEMENT_3D('',#158975,#124036,#124037) ;
#99387=AXIS2_PLACEMENT_3D('',#158979,#124039,#124040) ;
#99388=AXIS2_PLACEMENT_3D('',#158982,#124042,#124043) ;
#99389=AXIS2_PLACEMENT_3D('',#158983,#124044,#124045) ;
#99390=AXIS2_PLACEMENT_3D('',#158989,#124049,#124050) ;
#99391=AXIS2_PLACEMENT_3D('',#158995,#124054,#124055) ;
#99392=AXIS2_PLACEMENT_3D('',#159001,#124059,#124060) ;
#99393=AXIS2_PLACEMENT_3D('',#159007,#124064,#124065) ;
#99394=AXIS2_PLACEMENT_3D('',#159020,#124071,#124072) ;
#99395=AXIS2_PLACEMENT_3D('',#159024,#124074,#124075) ;
#99396=AXIS2_PLACEMENT_3D('',#159028,#124077,#124078) ;
#99397=AXIS2_PLACEMENT_3D('',#159031,#124080,#124081) ;
#99398=AXIS2_PLACEMENT_3D('',#159032,#124082,#124083) ;
#99399=AXIS2_PLACEMENT_3D('',#159038,#124087,#124088) ;
#99400=AXIS2_PLACEMENT_3D('',#159044,#124092,#124093) ;
#99401=AXIS2_PLACEMENT_3D('',#159050,#124097,#124098) ;
#99402=AXIS2_PLACEMENT_3D('',#159056,#124102,#124103) ;
#99403=AXIS2_PLACEMENT_3D('',#159069,#124109,#124110) ;
#99404=AXIS2_PLACEMENT_3D('',#159073,#124112,#124113) ;
#99405=AXIS2_PLACEMENT_3D('',#159077,#124115,#124116) ;
#99406=AXIS2_PLACEMENT_3D('',#159080,#124118,#124119) ;
#99407=AXIS2_PLACEMENT_3D('',#159081,#124120,#124121) ;
#99408=AXIS2_PLACEMENT_3D('',#159087,#124125,#124126) ;
#99409=AXIS2_PLACEMENT_3D('',#159093,#124130,#124131) ;
#99410=AXIS2_PLACEMENT_3D('',#159099,#124135,#124136) ;
#99411=AXIS2_PLACEMENT_3D('',#159105,#124140,#124141) ;
#99412=AXIS2_PLACEMENT_3D('',#159118,#124147,#124148) ;
#99413=AXIS2_PLACEMENT_3D('',#159122,#124150,#124151) ;
#99414=AXIS2_PLACEMENT_3D('',#159126,#124153,#124154) ;
#99415=AXIS2_PLACEMENT_3D('',#159129,#124156,#124157) ;
#99416=AXIS2_PLACEMENT_3D('',#159130,#124158,#124159) ;
#99417=AXIS2_PLACEMENT_3D('',#159136,#124163,#124164) ;
#99418=AXIS2_PLACEMENT_3D('',#159142,#124168,#124169) ;
#99419=AXIS2_PLACEMENT_3D('',#159148,#124173,#124174) ;
#99420=AXIS2_PLACEMENT_3D('',#159154,#124178,#124179) ;
#99421=AXIS2_PLACEMENT_3D('',#159167,#124185,#124186) ;
#99422=AXIS2_PLACEMENT_3D('',#159171,#124188,#124189) ;
#99423=AXIS2_PLACEMENT_3D('',#159175,#124191,#124192) ;
#99424=AXIS2_PLACEMENT_3D('',#159178,#124194,#124195) ;
#99425=AXIS2_PLACEMENT_3D('',#159179,#124196,#124197) ;
#99426=AXIS2_PLACEMENT_3D('',#159185,#124201,#124202) ;
#99427=AXIS2_PLACEMENT_3D('',#159191,#124206,#124207) ;
#99428=AXIS2_PLACEMENT_3D('',#159197,#124211,#124212) ;
#99429=AXIS2_PLACEMENT_3D('',#159203,#124216,#124217) ;
#99430=AXIS2_PLACEMENT_3D('',#159216,#124223,#124224) ;
#99431=AXIS2_PLACEMENT_3D('',#159220,#124226,#124227) ;
#99432=AXIS2_PLACEMENT_3D('',#159224,#124229,#124230) ;
#99433=AXIS2_PLACEMENT_3D('',#159227,#124232,#124233) ;
#99434=AXIS2_PLACEMENT_3D('',#159228,#124234,#124235) ;
#99435=AXIS2_PLACEMENT_3D('',#159234,#124239,#124240) ;
#99436=AXIS2_PLACEMENT_3D('',#159240,#124244,#124245) ;
#99437=AXIS2_PLACEMENT_3D('',#159246,#124249,#124250) ;
#99438=AXIS2_PLACEMENT_3D('',#159252,#124254,#124255) ;
#99439=AXIS2_PLACEMENT_3D('',#159265,#124261,#124262) ;
#99440=AXIS2_PLACEMENT_3D('',#159269,#124264,#124265) ;
#99441=AXIS2_PLACEMENT_3D('',#159273,#124267,#124268) ;
#99442=AXIS2_PLACEMENT_3D('',#159276,#124270,#124271) ;
#99443=AXIS2_PLACEMENT_3D('',#159277,#124272,#124273) ;
#99444=AXIS2_PLACEMENT_3D('',#159283,#124277,#124278) ;
#99445=AXIS2_PLACEMENT_3D('',#159289,#124282,#124283) ;
#99446=AXIS2_PLACEMENT_3D('',#159295,#124287,#124288) ;
#99447=AXIS2_PLACEMENT_3D('',#159301,#124292,#124293) ;
#99448=AXIS2_PLACEMENT_3D('',#159314,#124299,#124300) ;
#99449=AXIS2_PLACEMENT_3D('',#159318,#124302,#124303) ;
#99450=AXIS2_PLACEMENT_3D('',#159322,#124305,#124306) ;
#99451=AXIS2_PLACEMENT_3D('',#159325,#124308,#124309) ;
#99452=AXIS2_PLACEMENT_3D('',#159326,#124310,#124311) ;
#99453=AXIS2_PLACEMENT_3D('',#159332,#124315,#124316) ;
#99454=AXIS2_PLACEMENT_3D('',#159338,#124320,#124321) ;
#99455=AXIS2_PLACEMENT_3D('',#159344,#124325,#124326) ;
#99456=AXIS2_PLACEMENT_3D('',#159350,#124330,#124331) ;
#99457=AXIS2_PLACEMENT_3D('',#159359,#124336,#124337) ;
#99458=AXIS2_PLACEMENT_3D('',#159368,#124342,#124343) ;
#99459=AXIS2_PLACEMENT_3D('',#159377,#124348,#124349) ;
#99460=AXIS2_PLACEMENT_3D('',#159386,#124354,#124355) ;
#99461=AXIS2_PLACEMENT_3D('',#159395,#124360,#124361) ;
#99462=AXIS2_PLACEMENT_3D('',#159404,#124366,#124367) ;
#99463=AXIS2_PLACEMENT_3D('',#159413,#124372,#124373) ;
#99464=AXIS2_PLACEMENT_3D('',#159422,#124378,#124379) ;
#99465=AXIS2_PLACEMENT_3D('',#159431,#124384,#124385) ;
#99466=AXIS2_PLACEMENT_3D('',#159434,#124386,#124387) ;
#99467=AXIS2_PLACEMENT_3D('',#159436,#124388,#124389) ;
#99468=AXIS2_PLACEMENT_3D('',#159446,#124394,#124395) ;
#99469=AXIS2_PLACEMENT_3D('',#159452,#124399,#124400) ;
#99470=AXIS2_PLACEMENT_3D('',#159461,#124405,#124406) ;
#99471=AXIS2_PLACEMENT_3D('',#159466,#124408,#124409) ;
#99472=AXIS2_PLACEMENT_3D('',#159468,#124410,#124411) ;
#99473=AXIS2_PLACEMENT_3D('',#159476,#124415,#124416) ;
#99474=AXIS2_PLACEMENT_3D('',#159482,#124420,#124421) ;
#99475=AXIS2_PLACEMENT_3D('',#159491,#124426,#124427) ;
#99476=AXIS2_PLACEMENT_3D('',#159494,#124428,#124429) ;
#99477=AXIS2_PLACEMENT_3D('',#159496,#124430,#124431) ;
#99478=AXIS2_PLACEMENT_3D('',#159506,#124436,#124437) ;
#99479=AXIS2_PLACEMENT_3D('',#159512,#124441,#124442) ;
#99480=AXIS2_PLACEMENT_3D('',#159521,#124447,#124448) ;
#99481=AXIS2_PLACEMENT_3D('',#159526,#124450,#124451) ;
#99482=AXIS2_PLACEMENT_3D('',#159528,#124452,#124453) ;
#99483=AXIS2_PLACEMENT_3D('',#159536,#124457,#124458) ;
#99484=AXIS2_PLACEMENT_3D('',#159542,#124462,#124463) ;
#99485=AXIS2_PLACEMENT_3D('',#159551,#124468,#124469) ;
#99486=AXIS2_PLACEMENT_3D('',#159554,#124470,#124471) ;
#99487=AXIS2_PLACEMENT_3D('',#159556,#124472,#124473) ;
#99488=AXIS2_PLACEMENT_3D('',#159566,#124478,#124479) ;
#99489=AXIS2_PLACEMENT_3D('',#159572,#124483,#124484) ;
#99490=AXIS2_PLACEMENT_3D('',#159581,#124489,#124490) ;
#99491=AXIS2_PLACEMENT_3D('',#159586,#124492,#124493) ;
#99492=AXIS2_PLACEMENT_3D('',#159588,#124494,#124495) ;
#99493=AXIS2_PLACEMENT_3D('',#159596,#124499,#124500) ;
#99494=AXIS2_PLACEMENT_3D('',#159602,#124504,#124505) ;
#99495=AXIS2_PLACEMENT_3D('',#159611,#124510,#124511) ;
#99496=AXIS2_PLACEMENT_3D('',#159614,#124512,#124513) ;
#99497=AXIS2_PLACEMENT_3D('',#159616,#124514,#124515) ;
#99498=AXIS2_PLACEMENT_3D('',#159626,#124520,#124521) ;
#99499=AXIS2_PLACEMENT_3D('',#159632,#124525,#124526) ;
#99500=AXIS2_PLACEMENT_3D('',#159641,#124531,#124532) ;
#99501=AXIS2_PLACEMENT_3D('',#159646,#124534,#124535) ;
#99502=AXIS2_PLACEMENT_3D('',#159648,#124536,#124537) ;
#99503=AXIS2_PLACEMENT_3D('',#159656,#124541,#124542) ;
#99504=AXIS2_PLACEMENT_3D('',#159662,#124546,#124547) ;
#99505=AXIS2_PLACEMENT_3D('',#159671,#124552,#124553) ;
#99506=AXIS2_PLACEMENT_3D('',#159674,#124554,#124555) ;
#99507=AXIS2_PLACEMENT_3D('',#159676,#124556,#124557) ;
#99508=AXIS2_PLACEMENT_3D('',#159686,#124562,#124563) ;
#99509=AXIS2_PLACEMENT_3D('',#159692,#124567,#124568) ;
#99510=AXIS2_PLACEMENT_3D('',#159701,#124573,#124574) ;
#99511=AXIS2_PLACEMENT_3D('',#159706,#124576,#124577) ;
#99512=AXIS2_PLACEMENT_3D('',#159708,#124578,#124579) ;
#99513=AXIS2_PLACEMENT_3D('',#159716,#124583,#124584) ;
#99514=AXIS2_PLACEMENT_3D('',#159722,#124588,#124589) ;
#99515=AXIS2_PLACEMENT_3D('',#159731,#124594,#124595) ;
#99516=AXIS2_PLACEMENT_3D('',#159734,#124596,#124597) ;
#99517=AXIS2_PLACEMENT_3D('',#159736,#124598,#124599) ;
#99518=AXIS2_PLACEMENT_3D('',#159746,#124604,#124605) ;
#99519=AXIS2_PLACEMENT_3D('',#159752,#124609,#124610) ;
#99520=AXIS2_PLACEMENT_3D('',#159761,#124615,#124616) ;
#99521=AXIS2_PLACEMENT_3D('',#159766,#124618,#124619) ;
#99522=AXIS2_PLACEMENT_3D('',#159768,#124620,#124621) ;
#99523=AXIS2_PLACEMENT_3D('',#159776,#124625,#124626) ;
#99524=AXIS2_PLACEMENT_3D('',#159782,#124630,#124631) ;
#99525=AXIS2_PLACEMENT_3D('',#159791,#124636,#124637) ;
#99526=AXIS2_PLACEMENT_3D('',#159794,#124638,#124639) ;
#99527=AXIS2_PLACEMENT_3D('',#159796,#124640,#124641) ;
#99528=AXIS2_PLACEMENT_3D('',#159806,#124646,#124647) ;
#99529=AXIS2_PLACEMENT_3D('',#159812,#124651,#124652) ;
#99530=AXIS2_PLACEMENT_3D('',#159821,#124657,#124658) ;
#99531=AXIS2_PLACEMENT_3D('',#159826,#124660,#124661) ;
#99532=AXIS2_PLACEMENT_3D('',#159828,#124662,#124663) ;
#99533=AXIS2_PLACEMENT_3D('',#159836,#124667,#124668) ;
#99534=AXIS2_PLACEMENT_3D('',#159842,#124672,#124673) ;
#99535=AXIS2_PLACEMENT_3D('',#159851,#124678,#124679) ;
#99536=AXIS2_PLACEMENT_3D('',#159854,#124680,#124681) ;
#99537=AXIS2_PLACEMENT_3D('',#159856,#124682,#124683) ;
#99538=AXIS2_PLACEMENT_3D('',#159866,#124688,#124689) ;
#99539=AXIS2_PLACEMENT_3D('',#159872,#124693,#124694) ;
#99540=AXIS2_PLACEMENT_3D('',#159881,#124699,#124700) ;
#99541=AXIS2_PLACEMENT_3D('',#159886,#124702,#124703) ;
#99542=AXIS2_PLACEMENT_3D('',#159888,#124704,#124705) ;
#99543=AXIS2_PLACEMENT_3D('',#159896,#124709,#124710) ;
#99544=AXIS2_PLACEMENT_3D('',#159902,#124714,#124715) ;
#99545=AXIS2_PLACEMENT_3D('',#159911,#124720,#124721) ;
#99546=AXIS2_PLACEMENT_3D('',#159914,#124722,#124723) ;
#99547=AXIS2_PLACEMENT_3D('',#159916,#124724,#124725) ;
#99548=AXIS2_PLACEMENT_3D('',#159926,#124730,#124731) ;
#99549=AXIS2_PLACEMENT_3D('',#159932,#124735,#124736) ;
#99550=AXIS2_PLACEMENT_3D('',#159941,#124741,#124742) ;
#99551=AXIS2_PLACEMENT_3D('',#159946,#124744,#124745) ;
#99552=AXIS2_PLACEMENT_3D('',#159948,#124746,#124747) ;
#99553=AXIS2_PLACEMENT_3D('',#159956,#124751,#124752) ;
#99554=AXIS2_PLACEMENT_3D('',#159962,#124756,#124757) ;
#99555=AXIS2_PLACEMENT_3D('',#159971,#124762,#124763) ;
#99556=AXIS2_PLACEMENT_3D('',#159980,#124768,#124769) ;
#99557=AXIS2_PLACEMENT_3D('',#159989,#124774,#124775) ;
#99558=AXIS2_PLACEMENT_3D('',#159994,#124777,#124778) ;
#99559=AXIS2_PLACEMENT_3D('',#159997,#124780,#124781) ;
#99560=AXIS2_PLACEMENT_3D('',#159998,#124782,#124783) ;
#99561=AXIS2_PLACEMENT_3D('',#160003,#124785,#124786) ;
#99562=AXIS2_PLACEMENT_3D('',#160011,#124791,#124792) ;
#99563=AXIS2_PLACEMENT_3D('',#160020,#124797,#124798) ;
#99564=AXIS2_PLACEMENT_3D('',#160029,#124803,#124804) ;
#99565=AXIS2_PLACEMENT_3D('',#160034,#124806,#124807) ;
#99566=AXIS2_PLACEMENT_3D('',#160037,#124809,#124810) ;
#99567=AXIS2_PLACEMENT_3D('',#160038,#124811,#124812) ;
#99568=AXIS2_PLACEMENT_3D('',#160043,#124814,#124815) ;
#99569=AXIS2_PLACEMENT_3D('',#160051,#124820,#124821) ;
#99570=AXIS2_PLACEMENT_3D('',#160060,#124826,#124827) ;
#99571=AXIS2_PLACEMENT_3D('',#160069,#124832,#124833) ;
#99572=AXIS2_PLACEMENT_3D('',#160074,#124835,#124836) ;
#99573=AXIS2_PLACEMENT_3D('',#160077,#124838,#124839) ;
#99574=AXIS2_PLACEMENT_3D('',#160078,#124840,#124841) ;
#99575=AXIS2_PLACEMENT_3D('',#160083,#124843,#124844) ;
#99576=AXIS2_PLACEMENT_3D('',#160091,#124849,#124850) ;
#99577=AXIS2_PLACEMENT_3D('',#160100,#124855,#124856) ;
#99578=AXIS2_PLACEMENT_3D('',#160109,#124861,#124862) ;
#99579=AXIS2_PLACEMENT_3D('',#160114,#124864,#124865) ;
#99580=AXIS2_PLACEMENT_3D('',#160117,#124867,#124868) ;
#99581=AXIS2_PLACEMENT_3D('',#160118,#124869,#124870) ;
#99582=AXIS2_PLACEMENT_3D('',#160123,#124872,#124873) ;
#99583=AXIS2_PLACEMENT_3D('',#160131,#124878,#124879) ;
#99584=AXIS2_PLACEMENT_3D('',#160140,#124884,#124885) ;
#99585=AXIS2_PLACEMENT_3D('',#160149,#124890,#124891) ;
#99586=AXIS2_PLACEMENT_3D('',#160154,#124893,#124894) ;
#99587=AXIS2_PLACEMENT_3D('',#160157,#124896,#124897) ;
#99588=AXIS2_PLACEMENT_3D('',#160158,#124898,#124899) ;
#99589=AXIS2_PLACEMENT_3D('',#160163,#124901,#124902) ;
#99590=AXIS2_PLACEMENT_3D('',#160171,#124907,#124908) ;
#99591=AXIS2_PLACEMENT_3D('',#160180,#124913,#124914) ;
#99592=AXIS2_PLACEMENT_3D('',#160189,#124919,#124920) ;
#99593=AXIS2_PLACEMENT_3D('',#160194,#124922,#124923) ;
#99594=AXIS2_PLACEMENT_3D('',#160197,#124925,#124926) ;
#99595=AXIS2_PLACEMENT_3D('',#160198,#124927,#124928) ;
#99596=AXIS2_PLACEMENT_3D('',#160203,#124930,#124931) ;
#99597=AXIS2_PLACEMENT_3D('',#160211,#124936,#124937) ;
#99598=AXIS2_PLACEMENT_3D('',#160220,#124942,#124943) ;
#99599=AXIS2_PLACEMENT_3D('',#160229,#124948,#124949) ;
#99600=AXIS2_PLACEMENT_3D('',#160234,#124951,#124952) ;
#99601=AXIS2_PLACEMENT_3D('',#160237,#124954,#124955) ;
#99602=AXIS2_PLACEMENT_3D('',#160238,#124956,#124957) ;
#99603=AXIS2_PLACEMENT_3D('',#160243,#124959,#124960) ;
#99604=AXIS2_PLACEMENT_3D('',#160251,#124965,#124966) ;
#99605=AXIS2_PLACEMENT_3D('',#160260,#124971,#124972) ;
#99606=AXIS2_PLACEMENT_3D('',#160269,#124977,#124978) ;
#99607=AXIS2_PLACEMENT_3D('',#160274,#124980,#124981) ;
#99608=AXIS2_PLACEMENT_3D('',#160277,#124983,#124984) ;
#99609=AXIS2_PLACEMENT_3D('',#160278,#124985,#124986) ;
#99610=AXIS2_PLACEMENT_3D('',#160283,#124988,#124989) ;
#99611=AXIS2_PLACEMENT_3D('',#160291,#124994,#124995) ;
#99612=AXIS2_PLACEMENT_3D('',#160300,#125000,#125001) ;
#99613=AXIS2_PLACEMENT_3D('',#160309,#125006,#125007) ;
#99614=AXIS2_PLACEMENT_3D('',#160314,#125009,#125010) ;
#99615=AXIS2_PLACEMENT_3D('',#160317,#125012,#125013) ;
#99616=AXIS2_PLACEMENT_3D('',#160318,#125014,#125015) ;
#99617=AXIS2_PLACEMENT_3D('',#160323,#125017,#125018) ;
#99618=AXIS2_PLACEMENT_3D('',#160331,#125023,#125024) ;
#99619=AXIS2_PLACEMENT_3D('',#160332,#125025,#125026) ;
#99620=AXIS2_PLACEMENT_3D('',#160333,#125027,#125028) ;
#99621=AXIS2_PLACEMENT_3D('',#160334,#125029,#125030) ;
#99622=AXIS2_PLACEMENT_3D('',#160335,#125031,#125032) ;
#99623=AXIS2_PLACEMENT_3D('',#160336,#125033,#125034) ;
#99624=AXIS2_PLACEMENT_3D('',#160337,#125035,#125036) ;
#99625=AXIS2_PLACEMENT_3D('',#160338,#125037,#125038) ;
#99626=AXIS2_PLACEMENT_3D('',#160339,#125039,#125040) ;
#99627=AXIS2_PLACEMENT_3D('',#160340,#125041,#125042) ;
#99628=AXIS2_PLACEMENT_3D('',#160349,#125047,#125048) ;
#99629=AXIS2_PLACEMENT_3D('',#160358,#125053,#125054) ;
#99630=AXIS2_PLACEMENT_3D('',#160367,#125059,#125060) ;
#99631=AXIS2_PLACEMENT_3D('',#160376,#125065,#125066) ;
#99632=AXIS2_PLACEMENT_3D('',#160385,#125071,#125072) ;
#99633=AXIS2_PLACEMENT_3D('',#160394,#125077,#125078) ;
#99634=AXIS2_PLACEMENT_3D('',#160403,#125083,#125084) ;
#99635=AXIS2_PLACEMENT_3D('',#160412,#125089,#125090) ;
#99636=AXIS2_PLACEMENT_3D('',#160421,#125095,#125096) ;
#99637=AXIS2_PLACEMENT_3D('',#160430,#125101,#125102) ;
#99638=AXIS2_PLACEMENT_3D('',#160439,#125107,#125108) ;
#99639=AXIS2_PLACEMENT_3D('',#160448,#125113,#125114) ;
#99640=AXIS2_PLACEMENT_3D('',#160457,#125119,#125120) ;
#99641=AXIS2_PLACEMENT_3D('',#160466,#125125,#125126) ;
#99642=AXIS2_PLACEMENT_3D('',#160475,#125131,#125132) ;
#99643=AXIS2_PLACEMENT_3D('',#160484,#125137,#125138) ;
#99644=AXIS2_PLACEMENT_3D('',#160493,#125143,#125144) ;
#99645=AXIS2_PLACEMENT_3D('',#160502,#125149,#125150) ;
#99646=AXIS2_PLACEMENT_3D('',#160511,#125155,#125156) ;
#99647=AXIS2_PLACEMENT_3D('',#160520,#125161,#125162) ;
#99648=AXIS2_PLACEMENT_3D('',#160529,#125167,#125168) ;
#99649=AXIS2_PLACEMENT_3D('',#160538,#125173,#125174) ;
#99650=AXIS2_PLACEMENT_3D('',#160547,#125179,#125180) ;
#99651=AXIS2_PLACEMENT_3D('',#160556,#125185,#125186) ;
#99652=AXIS2_PLACEMENT_3D('',#160565,#125191,#125192) ;
#99653=AXIS2_PLACEMENT_3D('',#160574,#125197,#125198) ;
#99654=AXIS2_PLACEMENT_3D('',#160583,#125203,#125204) ;
#99655=AXIS2_PLACEMENT_3D('',#160592,#125209,#125210) ;
#99656=AXIS2_PLACEMENT_3D('',#160601,#125215,#125216) ;
#99657=AXIS2_PLACEMENT_3D('',#160610,#125221,#125222) ;
#99658=AXIS2_PLACEMENT_3D('',#160619,#125227,#125228) ;
#99659=AXIS2_PLACEMENT_3D('',#160628,#125233,#125234) ;
#99660=AXIS2_PLACEMENT_3D('',#160637,#125239,#125240) ;
#99661=AXIS2_PLACEMENT_3D('',#160646,#125245,#125246) ;
#99662=AXIS2_PLACEMENT_3D('',#160655,#125251,#125252) ;
#99663=AXIS2_PLACEMENT_3D('',#160664,#125257,#125258) ;
#99664=AXIS2_PLACEMENT_3D('',#160677,#125264,#125265) ;
#99665=AXIS2_PLACEMENT_3D('',#160681,#125267,#125268) ;
#99666=AXIS2_PLACEMENT_3D('',#160685,#125270,#125271) ;
#99667=AXIS2_PLACEMENT_3D('',#160688,#125273,#125274) ;
#99668=AXIS2_PLACEMENT_3D('',#160689,#125275,#125276) ;
#99669=AXIS2_PLACEMENT_3D('',#160695,#125280,#125281) ;
#99670=AXIS2_PLACEMENT_3D('',#160701,#125285,#125286) ;
#99671=AXIS2_PLACEMENT_3D('',#160707,#125290,#125291) ;
#99672=AXIS2_PLACEMENT_3D('',#160713,#125295,#125296) ;
#99673=AXIS2_PLACEMENT_3D('',#160726,#125302,#125303) ;
#99674=AXIS2_PLACEMENT_3D('',#160730,#125305,#125306) ;
#99675=AXIS2_PLACEMENT_3D('',#160734,#125308,#125309) ;
#99676=AXIS2_PLACEMENT_3D('',#160737,#125311,#125312) ;
#99677=AXIS2_PLACEMENT_3D('',#160738,#125313,#125314) ;
#99678=AXIS2_PLACEMENT_3D('',#160744,#125318,#125319) ;
#99679=AXIS2_PLACEMENT_3D('',#160750,#125323,#125324) ;
#99680=AXIS2_PLACEMENT_3D('',#160756,#125328,#125329) ;
#99681=AXIS2_PLACEMENT_3D('',#160762,#125333,#125334) ;
#99682=AXIS2_PLACEMENT_3D('',#160775,#125340,#125341) ;
#99683=AXIS2_PLACEMENT_3D('',#160779,#125343,#125344) ;
#99684=AXIS2_PLACEMENT_3D('',#160783,#125346,#125347) ;
#99685=AXIS2_PLACEMENT_3D('',#160786,#125349,#125350) ;
#99686=AXIS2_PLACEMENT_3D('',#160787,#125351,#125352) ;
#99687=AXIS2_PLACEMENT_3D('',#160793,#125356,#125357) ;
#99688=AXIS2_PLACEMENT_3D('',#160799,#125361,#125362) ;
#99689=AXIS2_PLACEMENT_3D('',#160805,#125366,#125367) ;
#99690=AXIS2_PLACEMENT_3D('',#160811,#125371,#125372) ;
#99691=AXIS2_PLACEMENT_3D('',#160824,#125378,#125379) ;
#99692=AXIS2_PLACEMENT_3D('',#160828,#125381,#125382) ;
#99693=AXIS2_PLACEMENT_3D('',#160832,#125384,#125385) ;
#99694=AXIS2_PLACEMENT_3D('',#160835,#125387,#125388) ;
#99695=AXIS2_PLACEMENT_3D('',#160836,#125389,#125390) ;
#99696=AXIS2_PLACEMENT_3D('',#160842,#125394,#125395) ;
#99697=AXIS2_PLACEMENT_3D('',#160848,#125399,#125400) ;
#99698=AXIS2_PLACEMENT_3D('',#160854,#125404,#125405) ;
#99699=AXIS2_PLACEMENT_3D('',#160860,#125409,#125410) ;
#99700=AXIS2_PLACEMENT_3D('',#160873,#125416,#125417) ;
#99701=AXIS2_PLACEMENT_3D('',#160877,#125419,#125420) ;
#99702=AXIS2_PLACEMENT_3D('',#160881,#125422,#125423) ;
#99703=AXIS2_PLACEMENT_3D('',#160884,#125425,#125426) ;
#99704=AXIS2_PLACEMENT_3D('',#160885,#125427,#125428) ;
#99705=AXIS2_PLACEMENT_3D('',#160891,#125432,#125433) ;
#99706=AXIS2_PLACEMENT_3D('',#160897,#125437,#125438) ;
#99707=AXIS2_PLACEMENT_3D('',#160903,#125442,#125443) ;
#99708=AXIS2_PLACEMENT_3D('',#160909,#125447,#125448) ;
#99709=AXIS2_PLACEMENT_3D('',#160922,#125454,#125455) ;
#99710=AXIS2_PLACEMENT_3D('',#160926,#125457,#125458) ;
#99711=AXIS2_PLACEMENT_3D('',#160930,#125460,#125461) ;
#99712=AXIS2_PLACEMENT_3D('',#160933,#125463,#125464) ;
#99713=AXIS2_PLACEMENT_3D('',#160934,#125465,#125466) ;
#99714=AXIS2_PLACEMENT_3D('',#160940,#125470,#125471) ;
#99715=AXIS2_PLACEMENT_3D('',#160946,#125475,#125476) ;
#99716=AXIS2_PLACEMENT_3D('',#160952,#125480,#125481) ;
#99717=AXIS2_PLACEMENT_3D('',#160958,#125485,#125486) ;
#99718=AXIS2_PLACEMENT_3D('',#160971,#125492,#125493) ;
#99719=AXIS2_PLACEMENT_3D('',#160975,#125495,#125496) ;
#99720=AXIS2_PLACEMENT_3D('',#160979,#125498,#125499) ;
#99721=AXIS2_PLACEMENT_3D('',#160982,#125501,#125502) ;
#99722=AXIS2_PLACEMENT_3D('',#160983,#125503,#125504) ;
#99723=AXIS2_PLACEMENT_3D('',#160989,#125508,#125509) ;
#99724=AXIS2_PLACEMENT_3D('',#160995,#125513,#125514) ;
#99725=AXIS2_PLACEMENT_3D('',#161001,#125518,#125519) ;
#99726=AXIS2_PLACEMENT_3D('',#161007,#125523,#125524) ;
#99727=AXIS2_PLACEMENT_3D('',#161020,#125530,#125531) ;
#99728=AXIS2_PLACEMENT_3D('',#161024,#125533,#125534) ;
#99729=AXIS2_PLACEMENT_3D('',#161028,#125536,#125537) ;
#99730=AXIS2_PLACEMENT_3D('',#161031,#125539,#125540) ;
#99731=AXIS2_PLACEMENT_3D('',#161032,#125541,#125542) ;
#99732=AXIS2_PLACEMENT_3D('',#161038,#125546,#125547) ;
#99733=AXIS2_PLACEMENT_3D('',#161044,#125551,#125552) ;
#99734=AXIS2_PLACEMENT_3D('',#161050,#125556,#125557) ;
#99735=AXIS2_PLACEMENT_3D('',#161056,#125561,#125562) ;
#99736=AXIS2_PLACEMENT_3D('',#161069,#125568,#125569) ;
#99737=AXIS2_PLACEMENT_3D('',#161073,#125571,#125572) ;
#99738=AXIS2_PLACEMENT_3D('',#161077,#125574,#125575) ;
#99739=AXIS2_PLACEMENT_3D('',#161080,#125577,#125578) ;
#99740=AXIS2_PLACEMENT_3D('',#161081,#125579,#125580) ;
#99741=AXIS2_PLACEMENT_3D('',#161087,#125584,#125585) ;
#99742=AXIS2_PLACEMENT_3D('',#161093,#125589,#125590) ;
#99743=AXIS2_PLACEMENT_3D('',#161099,#125594,#125595) ;
#99744=AXIS2_PLACEMENT_3D('',#161105,#125599,#125600) ;
#99745=AXIS2_PLACEMENT_3D('',#161114,#125605,#125606) ;
#99746=AXIS2_PLACEMENT_3D('',#161123,#125611,#125612) ;
#99747=AXIS2_PLACEMENT_3D('',#161132,#125617,#125618) ;
#99748=AXIS2_PLACEMENT_3D('',#161141,#125623,#125624) ;
#99749=AXIS2_PLACEMENT_3D('',#161150,#125629,#125630) ;
#99750=AXIS2_PLACEMENT_3D('',#161159,#125635,#125636) ;
#99751=AXIS2_PLACEMENT_3D('',#161168,#125641,#125642) ;
#99752=AXIS2_PLACEMENT_3D('',#161177,#125647,#125648) ;
#99753=AXIS2_PLACEMENT_3D('',#161186,#125653,#125654) ;
#99754=AXIS2_PLACEMENT_3D('',#161188,#125656,#125657) ;
#99755=AXIS2_PLACEMENT_3D('',#161190,#125659,#125660) ;
#99756=AXIS2_PLACEMENT_3D('',#161192,#125662,#125663) ;
#99757=AXIS2_PLACEMENT_3D('',#161194,#125665,#125666) ;
#99758=AXIS2_PLACEMENT_3D('',#161196,#125668,#125669) ;
#99759=AXIS2_PLACEMENT_3D('',#161198,#125671,#125672) ;
#99760=AXIS2_PLACEMENT_3D('',#161200,#125674,#125675) ;
#99761=AXIS2_PLACEMENT_3D('',#161202,#125677,#125678) ;
#99762=AXIS2_PLACEMENT_3D('',#161204,#125680,#125681) ;
#99763=AXIS2_PLACEMENT_3D('',#161207,#125684,#125685) ;
#99764=AXIS2_PLACEMENT_3D('',#161210,#125688,#125689) ;
#99765=AXIS2_PLACEMENT_3D('',#161213,#125692,#125693) ;
#99766=AXIS2_PLACEMENT_3D('',#161216,#125696,#125697) ;
#99767=AXIS2_PLACEMENT_3D('',#161219,#125700,#125701) ;
#99768=AXIS2_PLACEMENT_3D('',#161222,#125704,#125705) ;
#99769=AXIS2_PLACEMENT_3D('',#161225,#125708,#125709) ;
#99770=AXIS2_PLACEMENT_3D('',#161228,#125712,#125713) ;
#99771=AXIS2_PLACEMENT_3D('',#161231,#125716,#125717) ;
#99772=AXIS2_PLACEMENT_3D('',#161234,#125720,#125721) ;
#99773=AXIS2_PLACEMENT_3D('',#161237,#125724,#125725) ;
#99774=AXIS2_PLACEMENT_3D('',#161240,#125728,#125729) ;
#99775=AXIS2_PLACEMENT_3D('',#161243,#125732,#125733) ;
#99776=AXIS2_PLACEMENT_3D('',#161246,#125736,#125737) ;
#99777=AXIS2_PLACEMENT_3D('',#161249,#125740,#125741) ;
#99778=AXIS2_PLACEMENT_3D('',#161252,#125744,#125745) ;
#99779=AXIS2_PLACEMENT_3D('',#161255,#125748,#125749) ;
#99780=AXIS2_PLACEMENT_3D('',#161258,#125752,#125753) ;
#99781=AXIS2_PLACEMENT_3D('',#161261,#125756,#125757) ;
#99782=AXIS2_PLACEMENT_3D('',#161264,#125760,#125761) ;
#99783=AXIS2_PLACEMENT_3D('',#161267,#125764,#125765) ;
#99784=AXIS2_PLACEMENT_3D('',#161270,#125768,#125769) ;
#99785=AXIS2_PLACEMENT_3D('',#161273,#125772,#125773) ;
#99786=AXIS2_PLACEMENT_3D('',#161276,#125776,#125777) ;
#99787=AXIS2_PLACEMENT_3D('',#161279,#125780,#125781) ;
#99788=AXIS2_PLACEMENT_3D('',#161282,#125784,#125785) ;
#99789=AXIS2_PLACEMENT_3D('',#161285,#125788,#125789) ;
#99790=AXIS2_PLACEMENT_3D('',#161290,#125791,#125792) ;
#99791=AXIS2_PLACEMENT_3D('',#161293,#125794,#125795) ;
#99792=AXIS2_PLACEMENT_3D('',#161294,#125796,#125797) ;
#99793=AXIS2_PLACEMENT_3D('',#161300,#125801,#125802) ;
#99794=AXIS2_PLACEMENT_3D('',#161302,#125803,#125804) ;
#99795=AXIS2_PLACEMENT_3D('',#161305,#125806,#125807) ;
#99796=AXIS2_PLACEMENT_3D('',#161306,#125808,#125809) ;
#99797=AXIS2_PLACEMENT_3D('',#161312,#125813,#125814) ;
#99798=AXIS2_PLACEMENT_3D('',#161314,#125815,#125816) ;
#99799=AXIS2_PLACEMENT_3D('',#161317,#125818,#125819) ;
#99800=AXIS2_PLACEMENT_3D('',#161318,#125820,#125821) ;
#99801=AXIS2_PLACEMENT_3D('',#161324,#125825,#125826) ;
#99802=AXIS2_PLACEMENT_3D('',#161326,#125827,#125828) ;
#99803=AXIS2_PLACEMENT_3D('',#161329,#125830,#125831) ;
#99804=AXIS2_PLACEMENT_3D('',#161330,#125832,#125833) ;
#99805=AXIS2_PLACEMENT_3D('',#161333,#125836,#125837) ;
#99806=AXIS2_PLACEMENT_3D('',#161342,#125842,#125843) ;
#99807=AXIS2_PLACEMENT_3D('',#161347,#125845,#125846) ;
#99808=AXIS2_PLACEMENT_3D('',#161350,#125848,#125849) ;
#99809=AXIS2_PLACEMENT_3D('',#161351,#125850,#125851) ;
#99810=AXIS2_PLACEMENT_3D('',#161357,#125855,#125856) ;
#99811=AXIS2_PLACEMENT_3D('',#161359,#125857,#125858) ;
#99812=AXIS2_PLACEMENT_3D('',#161362,#125860,#125861) ;
#99813=AXIS2_PLACEMENT_3D('',#161363,#125862,#125863) ;
#99814=AXIS2_PLACEMENT_3D('',#161369,#125867,#125868) ;
#99815=AXIS2_PLACEMENT_3D('',#161371,#125869,#125870) ;
#99816=AXIS2_PLACEMENT_3D('',#161374,#125872,#125873) ;
#99817=AXIS2_PLACEMENT_3D('',#161375,#125874,#125875) ;
#99818=AXIS2_PLACEMENT_3D('',#161381,#125879,#125880) ;
#99819=AXIS2_PLACEMENT_3D('',#161383,#125881,#125882) ;
#99820=AXIS2_PLACEMENT_3D('',#161386,#125884,#125885) ;
#99821=AXIS2_PLACEMENT_3D('',#161387,#125886,#125887) ;
#99822=AXIS2_PLACEMENT_3D('',#161390,#125890,#125891) ;
#99823=AXIS2_PLACEMENT_3D('',#161399,#125896,#125897) ;
#99824=AXIS2_PLACEMENT_3D('',#161404,#125899,#125900) ;
#99825=AXIS2_PLACEMENT_3D('',#161407,#125902,#125903) ;
#99826=AXIS2_PLACEMENT_3D('',#161408,#125904,#125905) ;
#99827=AXIS2_PLACEMENT_3D('',#161414,#125909,#125910) ;
#99828=AXIS2_PLACEMENT_3D('',#161416,#125911,#125912) ;
#99829=AXIS2_PLACEMENT_3D('',#161419,#125914,#125915) ;
#99830=AXIS2_PLACEMENT_3D('',#161420,#125916,#125917) ;
#99831=AXIS2_PLACEMENT_3D('',#161426,#125921,#125922) ;
#99832=AXIS2_PLACEMENT_3D('',#161428,#125923,#125924) ;
#99833=AXIS2_PLACEMENT_3D('',#161431,#125926,#125927) ;
#99834=AXIS2_PLACEMENT_3D('',#161432,#125928,#125929) ;
#99835=AXIS2_PLACEMENT_3D('',#161438,#125933,#125934) ;
#99836=AXIS2_PLACEMENT_3D('',#161440,#125935,#125936) ;
#99837=AXIS2_PLACEMENT_3D('',#161443,#125938,#125939) ;
#99838=AXIS2_PLACEMENT_3D('',#161444,#125940,#125941) ;
#99839=AXIS2_PLACEMENT_3D('',#161447,#125944,#125945) ;
#99840=AXIS2_PLACEMENT_3D('',#161456,#125950,#125951) ;
#99841=AXIS2_PLACEMENT_3D('',#161461,#125953,#125954) ;
#99842=AXIS2_PLACEMENT_3D('',#161464,#125956,#125957) ;
#99843=AXIS2_PLACEMENT_3D('',#161465,#125958,#125959) ;
#99844=AXIS2_PLACEMENT_3D('',#161471,#125963,#125964) ;
#99845=AXIS2_PLACEMENT_3D('',#161473,#125965,#125966) ;
#99846=AXIS2_PLACEMENT_3D('',#161476,#125968,#125969) ;
#99847=AXIS2_PLACEMENT_3D('',#161477,#125970,#125971) ;
#99848=AXIS2_PLACEMENT_3D('',#161483,#125975,#125976) ;
#99849=AXIS2_PLACEMENT_3D('',#161485,#125977,#125978) ;
#99850=AXIS2_PLACEMENT_3D('',#161488,#125980,#125981) ;
#99851=AXIS2_PLACEMENT_3D('',#161489,#125982,#125983) ;
#99852=AXIS2_PLACEMENT_3D('',#161495,#125987,#125988) ;
#99853=AXIS2_PLACEMENT_3D('',#161497,#125989,#125990) ;
#99854=AXIS2_PLACEMENT_3D('',#161500,#125992,#125993) ;
#99855=AXIS2_PLACEMENT_3D('',#161501,#125994,#125995) ;
#99856=AXIS2_PLACEMENT_3D('',#161504,#125998,#125999) ;
#99857=AXIS2_PLACEMENT_3D('',#161513,#126004,#126005) ;
#99858=AXIS2_PLACEMENT_3D('',#161518,#126007,#126008) ;
#99859=AXIS2_PLACEMENT_3D('',#161521,#126010,#126011) ;
#99860=AXIS2_PLACEMENT_3D('',#161522,#126012,#126013) ;
#99861=AXIS2_PLACEMENT_3D('',#161528,#126017,#126018) ;
#99862=AXIS2_PLACEMENT_3D('',#161530,#126019,#126020) ;
#99863=AXIS2_PLACEMENT_3D('',#161533,#126022,#126023) ;
#99864=AXIS2_PLACEMENT_3D('',#161534,#126024,#126025) ;
#99865=AXIS2_PLACEMENT_3D('',#161540,#126029,#126030) ;
#99866=AXIS2_PLACEMENT_3D('',#161542,#126031,#126032) ;
#99867=AXIS2_PLACEMENT_3D('',#161545,#126034,#126035) ;
#99868=AXIS2_PLACEMENT_3D('',#161546,#126036,#126037) ;
#99869=AXIS2_PLACEMENT_3D('',#161552,#126041,#126042) ;
#99870=AXIS2_PLACEMENT_3D('',#161554,#126043,#126044) ;
#99871=AXIS2_PLACEMENT_3D('',#161557,#126046,#126047) ;
#99872=AXIS2_PLACEMENT_3D('',#161558,#126048,#126049) ;
#99873=AXIS2_PLACEMENT_3D('',#161561,#126052,#126053) ;
#99874=AXIS2_PLACEMENT_3D('',#161570,#126058,#126059) ;
#99875=AXIS2_PLACEMENT_3D('',#161575,#126061,#126062) ;
#99876=AXIS2_PLACEMENT_3D('',#161578,#126064,#126065) ;
#99877=AXIS2_PLACEMENT_3D('',#161579,#126066,#126067) ;
#99878=AXIS2_PLACEMENT_3D('',#161585,#126071,#126072) ;
#99879=AXIS2_PLACEMENT_3D('',#161587,#126073,#126074) ;
#99880=AXIS2_PLACEMENT_3D('',#161590,#126076,#126077) ;
#99881=AXIS2_PLACEMENT_3D('',#161591,#126078,#126079) ;
#99882=AXIS2_PLACEMENT_3D('',#161597,#126083,#126084) ;
#99883=AXIS2_PLACEMENT_3D('',#161599,#126085,#126086) ;
#99884=AXIS2_PLACEMENT_3D('',#161602,#126088,#126089) ;
#99885=AXIS2_PLACEMENT_3D('',#161603,#126090,#126091) ;
#99886=AXIS2_PLACEMENT_3D('',#161609,#126095,#126096) ;
#99887=AXIS2_PLACEMENT_3D('',#161611,#126097,#126098) ;
#99888=AXIS2_PLACEMENT_3D('',#161614,#126100,#126101) ;
#99889=AXIS2_PLACEMENT_3D('',#161615,#126102,#126103) ;
#99890=AXIS2_PLACEMENT_3D('',#161618,#126106,#126107) ;
#99891=AXIS2_PLACEMENT_3D('',#161627,#126112,#126113) ;
#99892=AXIS2_PLACEMENT_3D('',#161632,#126115,#126116) ;
#99893=AXIS2_PLACEMENT_3D('',#161635,#126118,#126119) ;
#99894=AXIS2_PLACEMENT_3D('',#161636,#126120,#126121) ;
#99895=AXIS2_PLACEMENT_3D('',#161642,#126125,#126126) ;
#99896=AXIS2_PLACEMENT_3D('',#161644,#126127,#126128) ;
#99897=AXIS2_PLACEMENT_3D('',#161647,#126130,#126131) ;
#99898=AXIS2_PLACEMENT_3D('',#161648,#126132,#126133) ;
#99899=AXIS2_PLACEMENT_3D('',#161654,#126137,#126138) ;
#99900=AXIS2_PLACEMENT_3D('',#161656,#126139,#126140) ;
#99901=AXIS2_PLACEMENT_3D('',#161659,#126142,#126143) ;
#99902=AXIS2_PLACEMENT_3D('',#161660,#126144,#126145) ;
#99903=AXIS2_PLACEMENT_3D('',#161666,#126149,#126150) ;
#99904=AXIS2_PLACEMENT_3D('',#161668,#126151,#126152) ;
#99905=AXIS2_PLACEMENT_3D('',#161671,#126154,#126155) ;
#99906=AXIS2_PLACEMENT_3D('',#161672,#126156,#126157) ;
#99907=AXIS2_PLACEMENT_3D('',#161675,#126160,#126161) ;
#99908=AXIS2_PLACEMENT_3D('',#161684,#126166,#126167) ;
#99909=AXIS2_PLACEMENT_3D('',#161689,#126169,#126170) ;
#99910=AXIS2_PLACEMENT_3D('',#161692,#126172,#126173) ;
#99911=AXIS2_PLACEMENT_3D('',#161693,#126174,#126175) ;
#99912=AXIS2_PLACEMENT_3D('',#161699,#126179,#126180) ;
#99913=AXIS2_PLACEMENT_3D('',#161701,#126181,#126182) ;
#99914=AXIS2_PLACEMENT_3D('',#161704,#126184,#126185) ;
#99915=AXIS2_PLACEMENT_3D('',#161705,#126186,#126187) ;
#99916=AXIS2_PLACEMENT_3D('',#161711,#126191,#126192) ;
#99917=AXIS2_PLACEMENT_3D('',#161713,#126193,#126194) ;
#99918=AXIS2_PLACEMENT_3D('',#161716,#126196,#126197) ;
#99919=AXIS2_PLACEMENT_3D('',#161717,#126198,#126199) ;
#99920=AXIS2_PLACEMENT_3D('',#161723,#126203,#126204) ;
#99921=AXIS2_PLACEMENT_3D('',#161725,#126205,#126206) ;
#99922=AXIS2_PLACEMENT_3D('',#161728,#126208,#126209) ;
#99923=AXIS2_PLACEMENT_3D('',#161729,#126210,#126211) ;
#99924=AXIS2_PLACEMENT_3D('',#161732,#126214,#126215) ;
#99925=AXIS2_PLACEMENT_3D('',#161741,#126220,#126221) ;
#99926=AXIS2_PLACEMENT_3D('',#161746,#126223,#126224) ;
#99927=AXIS2_PLACEMENT_3D('',#161749,#126226,#126227) ;
#99928=AXIS2_PLACEMENT_3D('',#161750,#126228,#126229) ;
#99929=AXIS2_PLACEMENT_3D('',#161756,#126233,#126234) ;
#99930=AXIS2_PLACEMENT_3D('',#161758,#126235,#126236) ;
#99931=AXIS2_PLACEMENT_3D('',#161761,#126238,#126239) ;
#99932=AXIS2_PLACEMENT_3D('',#161762,#126240,#126241) ;
#99933=AXIS2_PLACEMENT_3D('',#161768,#126245,#126246) ;
#99934=AXIS2_PLACEMENT_3D('',#161770,#126247,#126248) ;
#99935=AXIS2_PLACEMENT_3D('',#161773,#126250,#126251) ;
#99936=AXIS2_PLACEMENT_3D('',#161774,#126252,#126253) ;
#99937=AXIS2_PLACEMENT_3D('',#161780,#126257,#126258) ;
#99938=AXIS2_PLACEMENT_3D('',#161782,#126259,#126260) ;
#99939=AXIS2_PLACEMENT_3D('',#161785,#126262,#126263) ;
#99940=AXIS2_PLACEMENT_3D('',#161786,#126264,#126265) ;
#99941=AXIS2_PLACEMENT_3D('',#161789,#126268,#126269) ;
#99942=AXIS2_PLACEMENT_3D('',#161798,#126274,#126275) ;
#99943=AXIS2_PLACEMENT_3D('',#161799,#126276,#126277) ;
#99944=AXIS2_PLACEMENT_3D('',#161800,#126278,#126279) ;
#99945=AXIS2_PLACEMENT_3D('',#161801,#126280,#126281) ;
#99946=AXIS2_PLACEMENT_3D('',#161802,#126282,#126283) ;
#99947=AXIS2_PLACEMENT_3D('',#161803,#126284,#126285) ;
#99948=AXIS2_PLACEMENT_3D('',#161804,#126286,#126287) ;
#99949=AXIS2_PLACEMENT_3D('',#161805,#126288,#126289) ;
#99950=AXIS2_PLACEMENT_3D('',#161806,#126290,#126291) ;
#99951=AXIS2_PLACEMENT_3D('',#161807,#126292,#126293) ;
#99952=AXIS2_PLACEMENT_3D('',#161808,#126294,#126295) ;
#99953=AXIS2_PLACEMENT_3D('',#161809,#126296,#126297) ;
#99954=AXIS2_PLACEMENT_3D('',#161810,#126298,#126299) ;
#99955=AXIS2_PLACEMENT_3D('',#161811,#126300,#126301) ;
#99956=AXIS2_PLACEMENT_3D('',#161812,#126302,#126303) ;
#99957=AXIS2_PLACEMENT_3D('',#161813,#126304,#126305) ;
#99958=AXIS2_PLACEMENT_3D('',#161814,#126306,#126307) ;
#99959=AXIS2_PLACEMENT_3D('',#161815,#126308,#126309) ;
#99960=AXIS2_PLACEMENT_3D('',#161816,#126310,#126311) ;
#99961=AXIS2_PLACEMENT_3D('',#161817,#126312,#126313) ;
#99962=AXIS2_PLACEMENT_3D('',#161818,#126314,#126315) ;
#99963=AXIS2_PLACEMENT_3D('',#161819,#126316,#126317) ;
#99964=AXIS2_PLACEMENT_3D('',#161820,#126318,#126319) ;
#99965=AXIS2_PLACEMENT_3D('',#161821,#126320,#126321) ;
#99966=AXIS2_PLACEMENT_3D('',#161822,#126322,#126323) ;
#99967=AXIS2_PLACEMENT_3D('',#161823,#126324,#126325) ;
#99968=AXIS2_PLACEMENT_3D('',#161824,#126326,#126327) ;
#99969=AXIS2_PLACEMENT_3D('',#161825,#126328,#126329) ;
#99970=AXIS2_PLACEMENT_3D('',#161826,#126330,#126331) ;
#99971=AXIS2_PLACEMENT_3D('',#161827,#126332,#126333) ;
#99972=AXIS2_PLACEMENT_3D('',#161828,#126334,#126335) ;
#99973=AXIS2_PLACEMENT_3D('',#161829,#126336,#126337) ;
#99974=AXIS2_PLACEMENT_3D('',#161830,#126338,#126339) ;
#99975=AXIS2_PLACEMENT_3D('',#161831,#126340,#126341) ;
#99976=AXIS2_PLACEMENT_3D('',#161832,#126342,#126343) ;
#99977=AXIS2_PLACEMENT_3D('',#161833,#126344,#126345) ;
#99978=AXIS2_PLACEMENT_3D('',#161834,#126346,#126347) ;
#99979=AXIS2_PLACEMENT_3D('',#161835,#126348,#126349) ;
#99980=AXIS2_PLACEMENT_3D('',#161836,#126350,#126351) ;
#99981=AXIS2_PLACEMENT_3D('',#161837,#126352,#126353) ;
#99982=AXIS2_PLACEMENT_3D('',#161838,#126354,#126355) ;
#99983=AXIS2_PLACEMENT_3D('',#161839,#126356,#126357) ;
#99984=AXIS2_PLACEMENT_3D('',#161840,#126358,#126359) ;
#99985=AXIS2_PLACEMENT_3D('',#161841,#126360,#126361) ;
#99986=AXIS2_PLACEMENT_3D('',#161842,#126362,#126363) ;
#99987=AXIS2_PLACEMENT_3D('',#161843,#126364,#126365) ;
#99988=AXIS2_PLACEMENT_3D('',#161844,#126366,#126367) ;
#99989=AXIS2_PLACEMENT_3D('',#161845,#126368,#126369) ;
#99990=AXIS2_PLACEMENT_3D('',#161846,#126370,#126371) ;
#99991=AXIS2_PLACEMENT_3D('',#161847,#126372,#126373) ;
#99992=AXIS2_PLACEMENT_3D('',#161848,#126374,#126375) ;
#99993=AXIS2_PLACEMENT_3D('',#161849,#126376,#126377) ;
#99994=AXIS2_PLACEMENT_3D('',#161850,#126378,#126379) ;
#99995=AXIS2_PLACEMENT_3D('',#161851,#126380,#126381) ;
#99996=AXIS2_PLACEMENT_3D('',#161852,#126382,#126383) ;
#99997=AXIS2_PLACEMENT_3D('',#161853,#126384,#126385) ;
#99998=AXIS2_PLACEMENT_3D('',#161854,#126386,#126387) ;
#99999=AXIS2_PLACEMENT_3D('',#161855,#126388,#126389) ;
#100000=AXIS2_PLACEMENT_3D('',#161856,#126390,#126391) ;
#100001=AXIS2_PLACEMENT_3D('',#161857,#126392,#126393) ;
#100002=AXIS2_PLACEMENT_3D('',#161858,#126394,#126395) ;
#100003=AXIS2_PLACEMENT_3D('',#161859,#126396,#126397) ;
#100004=AXIS2_PLACEMENT_3D('',#161860,#126398,#126399) ;
#100005=AXIS2_PLACEMENT_3D('',#161861,#126400,#126401) ;
#100006=AXIS2_PLACEMENT_3D('',#161862,#126402,#126403) ;
#100007=AXIS2_PLACEMENT_3D('',#161863,#126404,#126405) ;
#100008=AXIS2_PLACEMENT_3D('',#161864,#126406,#126407) ;
#100009=AXIS2_PLACEMENT_3D('',#161865,#126408,#126409) ;
#100010=AXIS2_PLACEMENT_3D('',#161866,#126410,#126411) ;
#100011=AXIS2_PLACEMENT_3D('',#161867,#126412,#126413) ;
#100012=AXIS2_PLACEMENT_3D('',#161868,#126414,#126415) ;
#100013=AXIS2_PLACEMENT_3D('',#161869,#126416,#126417) ;
#100014=AXIS2_PLACEMENT_3D('',#161870,#126418,#126419) ;
#100015=AXIS2_PLACEMENT_3D('',#161871,#126420,#126421) ;
#100016=AXIS2_PLACEMENT_3D('',#161872,#126422,#126423) ;
#100017=AXIS2_PLACEMENT_3D('',#161873,#126424,#126425) ;
#100018=AXIS2_PLACEMENT_3D('',#161874,#126426,#126427) ;
#100019=AXIS2_PLACEMENT_3D('',#161875,#126428,#126429) ;
#100020=AXIS2_PLACEMENT_3D('',#161876,#126430,#126431) ;
#100021=AXIS2_PLACEMENT_3D('',#161877,#126432,#126433) ;
#100022=AXIS2_PLACEMENT_3D('',#161878,#126434,#126435) ;
#100023=AXIS2_PLACEMENT_3D('',#161879,#126436,#126437) ;
#100024=AXIS2_PLACEMENT_3D('',#161880,#126438,#126439) ;
#100025=AXIS2_PLACEMENT_3D('',#161881,#126440,#126441) ;
#100026=AXIS2_PLACEMENT_3D('',#161882,#126442,#126443) ;
#100027=AXIS2_PLACEMENT_3D('',#161883,#126444,#126445) ;
#100028=AXIS2_PLACEMENT_3D('',#161884,#126446,#126447) ;
#100029=AXIS2_PLACEMENT_3D('',#161885,#126448,#126449) ;
#100030=AXIS2_PLACEMENT_3D('',#161886,#126450,#126451) ;
#100031=AXIS2_PLACEMENT_3D('',#161887,#126452,#126453) ;
#100032=AXIS2_PLACEMENT_3D('',#161888,#126454,#126455) ;
#100033=AXIS2_PLACEMENT_3D('',#161889,#126456,#126457) ;
#100034=AXIS2_PLACEMENT_3D('',#161890,#126458,#126459) ;
#100035=AXIS2_PLACEMENT_3D('',#161891,#126460,#126461) ;
#100036=AXIS2_PLACEMENT_3D('',#161892,#126462,#126463) ;
#100037=AXIS2_PLACEMENT_3D('',#161893,#126464,#126465) ;
#100038=AXIS2_PLACEMENT_3D('',#161894,#126466,#126467) ;
#100039=AXIS2_PLACEMENT_3D('',#161895,#126468,#126469) ;
#100040=AXIS2_PLACEMENT_3D('',#161896,#126470,#126471) ;
#100041=AXIS2_PLACEMENT_3D('',#161897,#126472,#126473) ;
#100042=AXIS2_PLACEMENT_3D('',#161898,#126474,#126475) ;
#100043=AXIS2_PLACEMENT_3D('',#161899,#126476,#126477) ;
#100044=AXIS2_PLACEMENT_3D('',#161900,#126478,#126479) ;
#100045=AXIS2_PLACEMENT_3D('',#161902,#126480,#126481) ;
#100046=AXIS2_PLACEMENT_3D('',#161932,#126482,#126483) ;
#100047=AXIS2_PLACEMENT_3D('',#161933,#126484,#126485) ;
#100048=AXIS2_PLACEMENT_3D('',#161949,#126486,#126487) ;
#100049=AXIS2_PLACEMENT_3D('',#161951,#126488,#126489) ;
#100050=AXIS2_PLACEMENT_3D('',#161966,#126490,#126491) ;
#100051=AXIS2_PLACEMENT_3D('',#161982,#126492,#126493) ;
#100052=AXIS2_PLACEMENT_3D('',#161984,#126494,#126495) ;
#100053=AXIS2_PLACEMENT_3D('',#161999,#126496,#126497) ;
#100054=AXIS2_PLACEMENT_3D('',#162015,#126498,#126499) ;
#100055=AXIS2_PLACEMENT_3D('',#162017,#126500,#126501) ;
#100056=AXIS2_PLACEMENT_3D('',#162032,#126502,#126503) ;
#100057=AXIS2_PLACEMENT_3D('',#162034,#126504,#126505) ;
#100058=AXIS2_PLACEMENT_3D('',#162064,#126506,#126507) ;
#100059=AXIS2_PLACEMENT_3D('',#162065,#126508,#126509) ;
#100060=AXIS2_PLACEMENT_3D('',#162081,#126510,#126511) ;
#100061=AXIS2_PLACEMENT_3D('',#162083,#126512,#126513) ;
#100062=AXIS2_PLACEMENT_3D('',#162098,#126514,#126515) ;
#100063=AXIS2_PLACEMENT_3D('',#162114,#126516,#126517) ;
#100064=AXIS2_PLACEMENT_3D('',#162116,#126518,#126519) ;
#100065=AXIS2_PLACEMENT_3D('',#162131,#126520,#126521) ;
#100066=AXIS2_PLACEMENT_3D('',#162147,#126522,#126523) ;
#100067=AXIS2_PLACEMENT_3D('',#162149,#126524,#126525) ;
#100068=AXIS2_PLACEMENT_3D('',#162164,#126526,#126527) ;
#100069=AXIS2_PLACEMENT_3D('',#162166,#126528,#126529) ;
#100070=AXIS2_PLACEMENT_3D('',#162196,#126530,#126531) ;
#100071=AXIS2_PLACEMENT_3D('',#162197,#126532,#126533) ;
#100072=AXIS2_PLACEMENT_3D('',#162213,#126534,#126535) ;
#100073=AXIS2_PLACEMENT_3D('',#162215,#126536,#126537) ;
#100074=AXIS2_PLACEMENT_3D('',#162230,#126538,#126539) ;
#100075=AXIS2_PLACEMENT_3D('',#162246,#126540,#126541) ;
#100076=AXIS2_PLACEMENT_3D('',#162248,#126542,#126543) ;
#100077=AXIS2_PLACEMENT_3D('',#162263,#126544,#126545) ;
#100078=AXIS2_PLACEMENT_3D('',#162279,#126546,#126547) ;
#100079=AXIS2_PLACEMENT_3D('',#162281,#126548,#126549) ;
#100080=AXIS2_PLACEMENT_3D('',#162296,#126550,#126551) ;
#100081=AXIS2_PLACEMENT_3D('',#162298,#126552,#126553) ;
#100082=AXIS2_PLACEMENT_3D('',#162328,#126554,#126555) ;
#100083=AXIS2_PLACEMENT_3D('',#162329,#126556,#126557) ;
#100084=AXIS2_PLACEMENT_3D('',#162345,#126558,#126559) ;
#100085=AXIS2_PLACEMENT_3D('',#162347,#126560,#126561) ;
#100086=AXIS2_PLACEMENT_3D('',#162362,#126562,#126563) ;
#100087=AXIS2_PLACEMENT_3D('',#162378,#126564,#126565) ;
#100088=AXIS2_PLACEMENT_3D('',#162380,#126566,#126567) ;
#100089=AXIS2_PLACEMENT_3D('',#162395,#126568,#126569) ;
#100090=AXIS2_PLACEMENT_3D('',#162411,#126570,#126571) ;
#100091=AXIS2_PLACEMENT_3D('',#162413,#126572,#126573) ;
#100092=AXIS2_PLACEMENT_3D('',#162428,#126574,#126575) ;
#100093=AXIS2_PLACEMENT_3D('',#162430,#126576,#126577) ;
#100094=AXIS2_PLACEMENT_3D('',#162460,#126578,#126579) ;
#100095=AXIS2_PLACEMENT_3D('',#162461,#126580,#126581) ;
#100096=AXIS2_PLACEMENT_3D('',#162477,#126582,#126583) ;
#100097=AXIS2_PLACEMENT_3D('',#162479,#126584,#126585) ;
#100098=AXIS2_PLACEMENT_3D('',#162494,#126586,#126587) ;
#100099=AXIS2_PLACEMENT_3D('',#162510,#126588,#126589) ;
#100100=AXIS2_PLACEMENT_3D('',#162512,#126590,#126591) ;
#100101=AXIS2_PLACEMENT_3D('',#162527,#126592,#126593) ;
#100102=AXIS2_PLACEMENT_3D('',#162543,#126594,#126595) ;
#100103=AXIS2_PLACEMENT_3D('',#162545,#126596,#126597) ;
#100104=AXIS2_PLACEMENT_3D('',#162560,#126598,#126599) ;
#100105=AXIS2_PLACEMENT_3D('',#162562,#126600,#126601) ;
#100106=AXIS2_PLACEMENT_3D('',#162592,#126602,#126603) ;
#100107=AXIS2_PLACEMENT_3D('',#162593,#126604,#126605) ;
#100108=AXIS2_PLACEMENT_3D('',#162609,#126606,#126607) ;
#100109=AXIS2_PLACEMENT_3D('',#162611,#126608,#126609) ;
#100110=AXIS2_PLACEMENT_3D('',#162626,#126610,#126611) ;
#100111=AXIS2_PLACEMENT_3D('',#162642,#126612,#126613) ;
#100112=AXIS2_PLACEMENT_3D('',#162644,#126614,#126615) ;
#100113=AXIS2_PLACEMENT_3D('',#162659,#126616,#126617) ;
#100114=AXIS2_PLACEMENT_3D('',#162675,#126618,#126619) ;
#100115=AXIS2_PLACEMENT_3D('',#162677,#126620,#126621) ;
#100116=AXIS2_PLACEMENT_3D('',#162692,#126622,#126623) ;
#100117=AXIS2_PLACEMENT_3D('',#162694,#126624,#126625) ;
#100118=AXIS2_PLACEMENT_3D('',#162724,#126626,#126627) ;
#100119=AXIS2_PLACEMENT_3D('',#162725,#126628,#126629) ;
#100120=AXIS2_PLACEMENT_3D('',#162741,#126630,#126631) ;
#100121=AXIS2_PLACEMENT_3D('',#162743,#126632,#126633) ;
#100122=AXIS2_PLACEMENT_3D('',#162758,#126634,#126635) ;
#100123=AXIS2_PLACEMENT_3D('',#162774,#126636,#126637) ;
#100124=AXIS2_PLACEMENT_3D('',#162776,#126638,#126639) ;
#100125=AXIS2_PLACEMENT_3D('',#162791,#126640,#126641) ;
#100126=AXIS2_PLACEMENT_3D('',#162807,#126642,#126643) ;
#100127=AXIS2_PLACEMENT_3D('',#162809,#126644,#126645) ;
#100128=AXIS2_PLACEMENT_3D('',#162824,#126646,#126647) ;
#100129=AXIS2_PLACEMENT_3D('',#162826,#126648,#126649) ;
#100130=AXIS2_PLACEMENT_3D('',#162856,#126650,#126651) ;
#100131=AXIS2_PLACEMENT_3D('',#162857,#126652,#126653) ;
#100132=AXIS2_PLACEMENT_3D('',#162873,#126654,#126655) ;
#100133=AXIS2_PLACEMENT_3D('',#162875,#126656,#126657) ;
#100134=AXIS2_PLACEMENT_3D('',#162890,#126658,#126659) ;
#100135=AXIS2_PLACEMENT_3D('',#162906,#126660,#126661) ;
#100136=AXIS2_PLACEMENT_3D('',#162908,#126662,#126663) ;
#100137=AXIS2_PLACEMENT_3D('',#162923,#126664,#126665) ;
#100138=AXIS2_PLACEMENT_3D('',#162939,#126666,#126667) ;
#100139=AXIS2_PLACEMENT_3D('',#162941,#126668,#126669) ;
#100140=AXIS2_PLACEMENT_3D('',#162956,#126670,#126671) ;
#100141=AXIS2_PLACEMENT_3D('',#162957,#126672,#126673) ;
#100142=AXIS2_PLACEMENT_3D('',#162958,#126674,#126675) ;
#100143=AXIS2_PLACEMENT_3D('',#162959,#126676,#126677) ;
#100144=AXIS2_PLACEMENT_3D('',#162960,#126678,#126679) ;
#100145=AXIS2_PLACEMENT_3D('',#162961,#126680,#126681) ;
#100146=AXIS2_PLACEMENT_3D('',#162962,#126682,#126683) ;
#100147=AXIS2_PLACEMENT_3D('',#162963,#126684,#126685) ;
#100148=AXIS2_PLACEMENT_3D('',#162964,#126686,#126687) ;
#100149=AXIS2_PLACEMENT_3D('',#162965,#126688,#126689) ;
#100150=AXIS2_PLACEMENT_3D('',#162966,#126690,#126691) ;
#100151=AXIS2_PLACEMENT_3D('',#162967,#126692,#126693) ;
#100152=AXIS2_PLACEMENT_3D('',#162968,#126694,#126695) ;
#100153=AXIS2_PLACEMENT_3D('',#162969,#126696,#126697) ;
#100154=AXIS2_PLACEMENT_3D('',#162970,#126698,#126699) ;
#100155=AXIS2_PLACEMENT_3D('',#162971,#126700,#126701) ;
#100156=AXIS2_PLACEMENT_3D('',#162972,#126702,#126703) ;
#100157=AXIS2_PLACEMENT_3D('',#162973,#126704,#126705) ;
#100158=AXIS2_PLACEMENT_3D('',#162974,#126706,#126707) ;
#100159=AXIS2_PLACEMENT_3D('',#162975,#126708,#126709) ;
#100160=AXIS2_PLACEMENT_3D('',#162976,#126710,#126711) ;
#100161=AXIS2_PLACEMENT_3D('',#162977,#126712,#126713) ;
#100162=AXIS2_PLACEMENT_3D('',#162978,#126714,#126715) ;
#100163=AXIS2_PLACEMENT_3D('',#162979,#126716,#126717) ;
#100164=AXIS2_PLACEMENT_3D('',#162980,#126718,#126719) ;
#100165=AXIS2_PLACEMENT_3D('',#162981,#126720,#126721) ;
#100166=AXIS2_PLACEMENT_3D('',#162982,#126722,#126723) ;
#100167=AXIS2_PLACEMENT_3D('',#162983,#126724,#126725) ;
#100168=AXIS2_PLACEMENT_3D('',#162984,#126726,#126727) ;
#100169=AXIS2_PLACEMENT_3D('',#162985,#126728,#126729) ;
#100170=AXIS2_PLACEMENT_3D('',#162986,#126730,#126731) ;
#100171=AXIS2_PLACEMENT_3D('',#162987,#126732,#126733) ;
#100172=AXIS2_PLACEMENT_3D('',#162988,#126734,#126735) ;
#100173=AXIS2_PLACEMENT_3D('',#162989,#126736,#126737) ;
#100174=AXIS2_PLACEMENT_3D('',#162990,#126738,#126739) ;
#100175=AXIS2_PLACEMENT_3D('',#162991,#126740,#126741) ;
#100176=AXIS2_PLACEMENT_3D('',#162992,#126742,#126743) ;
#100177=AXIS2_PLACEMENT_3D('',#162993,#126744,#126745) ;
#100178=AXIS2_PLACEMENT_3D('',#162994,#126746,#126747) ;
#100179=AXIS2_PLACEMENT_3D('',#162995,#126748,#126749) ;
#100180=AXIS2_PLACEMENT_3D('',#162996,#126750,#126751) ;
#100181=AXIS2_PLACEMENT_3D('',#162997,#126752,#126753) ;
#100182=AXIS2_PLACEMENT_3D('',#162998,#126754,#126755) ;
#100183=AXIS2_PLACEMENT_3D('',#162999,#126756,#126757) ;
#100184=AXIS2_PLACEMENT_3D('',#163000,#126758,#126759) ;
#100185=AXIS2_PLACEMENT_3D('',#163001,#126760,#126761) ;
#100186=AXIS2_PLACEMENT_3D('',#163002,#126762,#126763) ;
#100187=AXIS2_PLACEMENT_3D('',#163003,#126764,#126765) ;
#100188=AXIS2_PLACEMENT_3D('',#163004,#126766,#126767) ;
#100189=AXIS2_PLACEMENT_3D('',#163005,#126768,#126769) ;
#100190=AXIS2_PLACEMENT_3D('',#163006,#126770,#126771) ;
#100191=AXIS2_PLACEMENT_3D('',#163007,#126772,#126773) ;
#100192=AXIS2_PLACEMENT_3D('',#163008,#126774,#126775) ;
#100193=AXIS2_PLACEMENT_3D('',#163009,#126776,#126777) ;
#100194=AXIS2_PLACEMENT_3D('',#163010,#126778,#126779) ;
#100195=AXIS2_PLACEMENT_3D('',#163011,#126780,#126781) ;
#100196=AXIS2_PLACEMENT_3D('',#163012,#126782,#126783) ;
#100197=AXIS2_PLACEMENT_3D('',#163013,#126784,#126785) ;
#100198=AXIS2_PLACEMENT_3D('',#163014,#126786,#126787) ;
#100199=AXIS2_PLACEMENT_3D('',#163015,#126788,#126789) ;
#100200=AXIS2_PLACEMENT_3D('',#163016,#126790,#126791) ;
#100201=AXIS2_PLACEMENT_3D('',#163017,#126792,#126793) ;
#100202=AXIS2_PLACEMENT_3D('',#163018,#126794,#126795) ;
#100203=AXIS2_PLACEMENT_3D('',#163019,#126796,#126797) ;
#100204=AXIS2_PLACEMENT_3D('',#163020,#126798,#126799) ;
#100205=AXIS2_PLACEMENT_3D('',#163021,#126800,#126801) ;
#100206=AXIS2_PLACEMENT_3D('',#163022,#126802,#126803) ;
#100207=AXIS2_PLACEMENT_3D('',#163023,#126804,#126805) ;
#100208=AXIS2_PLACEMENT_3D('',#163024,#126806,#126807) ;
#100209=AXIS2_PLACEMENT_3D('',#163025,#126808,#126809) ;
#100210=AXIS2_PLACEMENT_3D('',#163026,#126810,#126811) ;
#100211=AXIS2_PLACEMENT_3D('',#163027,#126812,#126813) ;
#100212=AXIS2_PLACEMENT_3D('',#163028,#126814,#126815) ;
#100213=AXIS2_PLACEMENT_3D('',#163029,#126816,#126817) ;
#100214=AXIS2_PLACEMENT_3D('',#163036,#126818,#126819) ;
#100215=AXIS2_PLACEMENT_3D('',#163037,#126820,#126821) ;
#100216=AXIS2_PLACEMENT_3D('',#163038,#126822,#126823) ;
#100217=AXIS2_PLACEMENT_3D('',#163039,#126824,#126825) ;
#100218=AXIS2_PLACEMENT_3D('',#163058,#126826,#126827) ;
#100219=AXIS2_PLACEMENT_3D('',#163059,#126828,#126829) ;
#100220=AXIS2_PLACEMENT_3D('',#163060,#126830,#126831) ;
#100221=AXIS2_PLACEMENT_3D('',#163061,#126832,#126833) ;
#100222=AXIS2_PLACEMENT_3D('',#163062,#126834,#126835) ;
#100223=AXIS2_PLACEMENT_3D('',#163063,#126836,#126837) ;
#100224=AXIS2_PLACEMENT_3D('',#163064,#126838,#126839) ;
#100225=AXIS2_PLACEMENT_3D('',#163071,#126840,#126841) ;
#100226=AXIS2_PLACEMENT_3D('',#163072,#126842,#126843) ;
#100227=AXIS2_PLACEMENT_3D('',#163073,#126844,#126845) ;
#100228=AXIS2_PLACEMENT_3D('',#163074,#126846,#126847) ;
#100229=AXIS2_PLACEMENT_3D('',#163075,#126848,#126849) ;
#100230=AXIS2_PLACEMENT_3D('',#163076,#126850,#126851) ;
#100231=AXIS2_PLACEMENT_3D('',#163077,#126852,#126853) ;
#100232=AXIS2_PLACEMENT_3D('',#163078,#126854,#126855) ;
#100233=AXIS2_PLACEMENT_3D('',#163079,#126856,#126857) ;
#100234=AXIS2_PLACEMENT_3D('',#163098,#126858,#126859) ;
#100235=AXIS2_PLACEMENT_3D('',#163117,#126860,#126861) ;
#100236=AXIS2_PLACEMENT_3D('',#163118,#126862,#126863) ;
#100237=AXIS2_PLACEMENT_3D('',#163119,#126864,#126865) ;
#100238=AXIS2_PLACEMENT_3D('',#163120,#126866,#126867) ;
#100239=AXIS2_PLACEMENT_3D('',#163121,#126868,#126869) ;
#100240=AXIS2_PLACEMENT_3D('',#163122,#126870,#126871) ;
#100241=AXIS2_PLACEMENT_3D('',#163123,#126872,#126873) ;
#100242=AXIS2_PLACEMENT_3D('',#163124,#126874,#126875) ;
#100243=AXIS2_PLACEMENT_3D('',#163125,#126876,#126877) ;
#100244=AXIS2_PLACEMENT_3D('',#163126,#126878,#126879) ;
#100245=AXIS2_PLACEMENT_3D('',#163127,#126880,#126881) ;
#100246=AXIS2_PLACEMENT_3D('',#163146,#126882,#126883) ;
#100247=AXIS2_PLACEMENT_3D('',#163147,#126884,#126885) ;
#100248=AXIS2_PLACEMENT_3D('',#163148,#126886,#126887) ;
#100249=AXIS2_PLACEMENT_3D('',#163150,#126888,#126889) ;
#100250=AXIS2_PLACEMENT_3D('',#163151,#126890,#126891) ;
#100251=AXIS2_PLACEMENT_3D('',#163153,#126892,#126893) ;
#100252=AXIS2_PLACEMENT_3D('',#163155,#126894,#126895) ;
#100253=AXIS2_PLACEMENT_3D('',#163156,#126896,#126897) ;
#100254=AXIS2_PLACEMENT_3D('',#163157,#126898,#126899) ;
#100255=AXIS2_PLACEMENT_3D('',#163159,#126900,#126901) ;
#100256=AXIS2_PLACEMENT_3D('',#163160,#126902,#126903) ;
#100257=AXIS2_PLACEMENT_3D('',#163162,#126904,#126905) ;
#100258=AXIS2_PLACEMENT_3D('',#163163,#126906,#126907) ;
#100259=AXIS2_PLACEMENT_3D('',#163164,#126908,#126909) ;
#100260=AXIS2_PLACEMENT_3D('',#163165,#126910,#126911) ;
#100261=AXIS2_PLACEMENT_3D('',#163166,#126912,#126913) ;
#100262=AXIS2_PLACEMENT_3D('',#163167,#126914,#126915) ;
#100263=AXIS2_PLACEMENT_3D('',#163169,#126916,#126917) ;
#100264=AXIS2_PLACEMENT_3D('',#163171,#126918,#126919) ;
#100265=AXIS2_PLACEMENT_3D('',#163172,#126920,#126921) ;
#100266=AXIS2_PLACEMENT_3D('',#163174,#126922,#126923) ;
#100267=AXIS2_PLACEMENT_3D('',#163175,#126924,#126925) ;
#100268=AXIS2_PLACEMENT_3D('',#163176,#126926,#126927) ;
#100269=AXIS2_PLACEMENT_3D('',#163178,#126928,#126929) ;
#100270=AXIS2_PLACEMENT_3D('',#163179,#126930,#126931) ;
#100271=AXIS2_PLACEMENT_3D('',#163181,#126932,#126933) ;
#100272=AXIS2_PLACEMENT_3D('',#163183,#126934,#126935) ;
#100273=AXIS2_PLACEMENT_3D('',#163184,#126936,#126937) ;
#100274=AXIS2_PLACEMENT_3D('',#163185,#126938,#126939) ;
#100275=AXIS2_PLACEMENT_3D('',#163187,#126940,#126941) ;
#100276=AXIS2_PLACEMENT_3D('',#163188,#126942,#126943) ;
#100277=AXIS2_PLACEMENT_3D('',#163190,#126944,#126945) ;
#100278=AXIS2_PLACEMENT_3D('',#163191,#126946,#126947) ;
#100279=AXIS2_PLACEMENT_3D('',#163192,#126948,#126949) ;
#100280=AXIS2_PLACEMENT_3D('',#163193,#126950,#126951) ;
#100281=AXIS2_PLACEMENT_3D('',#163194,#126952,#126953) ;
#100282=AXIS2_PLACEMENT_3D('',#163195,#126954,#126955) ;
#100283=AXIS2_PLACEMENT_3D('',#163197,#126956,#126957) ;
#100284=AXIS2_PLACEMENT_3D('',#163199,#126958,#126959) ;
#100285=AXIS2_PLACEMENT_3D('',#163200,#126960,#126961) ;
#100286=AXIS2_PLACEMENT_3D('',#163202,#126962,#126963) ;
#100287=AXIS2_PLACEMENT_3D('',#163203,#126964,#126965) ;
#100288=AXIS2_PLACEMENT_3D('',#163204,#126966,#126967) ;
#100289=AXIS2_PLACEMENT_3D('',#163206,#126968,#126969) ;
#100290=AXIS2_PLACEMENT_3D('',#163207,#126970,#126971) ;
#100291=AXIS2_PLACEMENT_3D('',#163209,#126972,#126973) ;
#100292=AXIS2_PLACEMENT_3D('',#163211,#126974,#126975) ;
#100293=AXIS2_PLACEMENT_3D('',#163212,#126976,#126977) ;
#100294=AXIS2_PLACEMENT_3D('',#163213,#126978,#126979) ;
#100295=AXIS2_PLACEMENT_3D('',#163215,#126980,#126981) ;
#100296=AXIS2_PLACEMENT_3D('',#163216,#126982,#126983) ;
#100297=AXIS2_PLACEMENT_3D('',#163218,#126984,#126985) ;
#100298=AXIS2_PLACEMENT_3D('',#163219,#126986,#126987) ;
#100299=AXIS2_PLACEMENT_3D('',#163220,#126988,#126989) ;
#100300=AXIS2_PLACEMENT_3D('',#163221,#126990,#126991) ;
#100301=AXIS2_PLACEMENT_3D('',#163222,#126992,#126993) ;
#100302=AXIS2_PLACEMENT_3D('',#163223,#126994,#126995) ;
#100303=AXIS2_PLACEMENT_3D('',#163225,#126996,#126997) ;
#100304=AXIS2_PLACEMENT_3D('',#163227,#126998,#126999) ;
#100305=AXIS2_PLACEMENT_3D('',#163228,#127000,#127001) ;
#100306=AXIS2_PLACEMENT_3D('',#163230,#127002,#127003) ;
#100307=AXIS2_PLACEMENT_3D('',#163231,#127004,#127005) ;
#100308=AXIS2_PLACEMENT_3D('',#163232,#127006,#127007) ;
#100309=AXIS2_PLACEMENT_3D('',#163234,#127008,#127009) ;
#100310=AXIS2_PLACEMENT_3D('',#163235,#127010,#127011) ;
#100311=AXIS2_PLACEMENT_3D('',#163237,#127012,#127013) ;
#100312=AXIS2_PLACEMENT_3D('',#163239,#127014,#127015) ;
#100313=AXIS2_PLACEMENT_3D('',#163240,#127016,#127017) ;
#100314=AXIS2_PLACEMENT_3D('',#163241,#127018,#127019) ;
#100315=AXIS2_PLACEMENT_3D('',#163243,#127020,#127021) ;
#100316=AXIS2_PLACEMENT_3D('',#163244,#127022,#127023) ;
#100317=AXIS2_PLACEMENT_3D('',#163246,#127024,#127025) ;
#100318=AXIS2_PLACEMENT_3D('',#163247,#127026,#127027) ;
#100319=AXIS2_PLACEMENT_3D('',#163248,#127028,#127029) ;
#100320=AXIS2_PLACEMENT_3D('',#163249,#127030,#127031) ;
#100321=AXIS2_PLACEMENT_3D('',#163250,#127032,#127033) ;
#100322=AXIS2_PLACEMENT_3D('',#163251,#127034,#127035) ;
#100323=AXIS2_PLACEMENT_3D('',#163253,#127036,#127037) ;
#100324=AXIS2_PLACEMENT_3D('',#163255,#127038,#127039) ;
#100325=AXIS2_PLACEMENT_3D('',#163256,#127040,#127041) ;
#100326=AXIS2_PLACEMENT_3D('',#163258,#127042,#127043) ;
#100327=AXIS2_PLACEMENT_3D('',#163259,#127044,#127045) ;
#100328=AXIS2_PLACEMENT_3D('',#163260,#127046,#127047) ;
#100329=AXIS2_PLACEMENT_3D('',#163262,#127048,#127049) ;
#100330=AXIS2_PLACEMENT_3D('',#163263,#127050,#127051) ;
#100331=AXIS2_PLACEMENT_3D('',#163265,#127052,#127053) ;
#100332=AXIS2_PLACEMENT_3D('',#163267,#127054,#127055) ;
#100333=AXIS2_PLACEMENT_3D('',#163268,#127056,#127057) ;
#100334=AXIS2_PLACEMENT_3D('',#163269,#127058,#127059) ;
#100335=AXIS2_PLACEMENT_3D('',#163271,#127060,#127061) ;
#100336=AXIS2_PLACEMENT_3D('',#163272,#127062,#127063) ;
#100337=AXIS2_PLACEMENT_3D('',#163274,#127064,#127065) ;
#100338=AXIS2_PLACEMENT_3D('',#163275,#127066,#127067) ;
#100339=AXIS2_PLACEMENT_3D('',#163276,#127068,#127069) ;
#100340=AXIS2_PLACEMENT_3D('',#163277,#127070,#127071) ;
#100341=AXIS2_PLACEMENT_3D('',#163278,#127072,#127073) ;
#100342=AXIS2_PLACEMENT_3D('',#163279,#127074,#127075) ;
#100343=AXIS2_PLACEMENT_3D('',#163281,#127076,#127077) ;
#100344=AXIS2_PLACEMENT_3D('',#163283,#127078,#127079) ;
#100345=AXIS2_PLACEMENT_3D('',#163284,#127080,#127081) ;
#100346=AXIS2_PLACEMENT_3D('',#163286,#127082,#127083) ;
#100347=AXIS2_PLACEMENT_3D('',#163287,#127084,#127085) ;
#100348=AXIS2_PLACEMENT_3D('',#163288,#127086,#127087) ;
#100349=AXIS2_PLACEMENT_3D('',#163290,#127088,#127089) ;
#100350=AXIS2_PLACEMENT_3D('',#163291,#127090,#127091) ;
#100351=AXIS2_PLACEMENT_3D('',#163293,#127092,#127093) ;
#100352=AXIS2_PLACEMENT_3D('',#163295,#127094,#127095) ;
#100353=AXIS2_PLACEMENT_3D('',#163296,#127096,#127097) ;
#100354=AXIS2_PLACEMENT_3D('',#163297,#127098,#127099) ;
#100355=AXIS2_PLACEMENT_3D('',#163299,#127100,#127101) ;
#100356=AXIS2_PLACEMENT_3D('',#163300,#127102,#127103) ;
#100357=AXIS2_PLACEMENT_3D('',#163302,#127104,#127105) ;
#100358=AXIS2_PLACEMENT_3D('',#163303,#127106,#127107) ;
#100359=AXIS2_PLACEMENT_3D('',#163304,#127108,#127109) ;
#100360=AXIS2_PLACEMENT_3D('',#163305,#127110,#127111) ;
#100361=AXIS2_PLACEMENT_3D('',#163306,#127112,#127113) ;
#100362=AXIS2_PLACEMENT_3D('',#163307,#127114,#127115) ;
#100363=AXIS2_PLACEMENT_3D('',#163309,#127116,#127117) ;
#100364=AXIS2_PLACEMENT_3D('',#163311,#127118,#127119) ;
#100365=AXIS2_PLACEMENT_3D('',#163312,#127120,#127121) ;
#100366=AXIS2_PLACEMENT_3D('',#163314,#127122,#127123) ;
#100367=AXIS2_PLACEMENT_3D('',#163315,#127124,#127125) ;
#100368=AXIS2_PLACEMENT_3D('',#163316,#127126,#127127) ;
#100369=AXIS2_PLACEMENT_3D('',#163318,#127128,#127129) ;
#100370=AXIS2_PLACEMENT_3D('',#163319,#127130,#127131) ;
#100371=AXIS2_PLACEMENT_3D('',#163321,#127132,#127133) ;
#100372=AXIS2_PLACEMENT_3D('',#163323,#127134,#127135) ;
#100373=AXIS2_PLACEMENT_3D('',#163324,#127136,#127137) ;
#100374=AXIS2_PLACEMENT_3D('',#163325,#127138,#127139) ;
#100375=AXIS2_PLACEMENT_3D('',#163327,#127140,#127141) ;
#100376=AXIS2_PLACEMENT_3D('',#163328,#127142,#127143) ;
#100377=AXIS2_PLACEMENT_3D('',#163330,#127144,#127145) ;
#100378=AXIS2_PLACEMENT_3D('',#163331,#127146,#127147) ;
#100379=AXIS2_PLACEMENT_3D('',#163332,#127148,#127149) ;
#100380=AXIS2_PLACEMENT_3D('',#163333,#127150,#127151) ;
#100381=AXIS2_PLACEMENT_3D('',#163334,#127152,#127153) ;
#100382=AXIS2_PLACEMENT_3D('',#163335,#127154,#127155) ;
#100383=AXIS2_PLACEMENT_3D('',#163337,#127156,#127157) ;
#100384=AXIS2_PLACEMENT_3D('',#163339,#127158,#127159) ;
#100385=AXIS2_PLACEMENT_3D('',#163340,#127160,#127161) ;
#100386=AXIS2_PLACEMENT_3D('',#163342,#127162,#127163) ;
#100387=AXIS2_PLACEMENT_3D('',#163343,#127164,#127165) ;
#100388=AXIS2_PLACEMENT_3D('',#163344,#127166,#127167) ;
#100389=AXIS2_PLACEMENT_3D('',#163346,#127168,#127169) ;
#100390=AXIS2_PLACEMENT_3D('',#163347,#127170,#127171) ;
#100391=AXIS2_PLACEMENT_3D('',#163349,#127172,#127173) ;
#100392=AXIS2_PLACEMENT_3D('',#163351,#127174,#127175) ;
#100393=AXIS2_PLACEMENT_3D('',#163352,#127176,#127177) ;
#100394=AXIS2_PLACEMENT_3D('',#163353,#127178,#127179) ;
#100395=AXIS2_PLACEMENT_3D('',#163355,#127180,#127181) ;
#100396=AXIS2_PLACEMENT_3D('',#163356,#127182,#127183) ;
#100397=AXIS2_PLACEMENT_3D('',#163358,#127184,#127185) ;
#100398=AXIS2_PLACEMENT_3D('',#163359,#127186,#127187) ;
#100399=AXIS2_PLACEMENT_3D('',#163360,#127188,#127189) ;
#100400=AXIS2_PLACEMENT_3D('',#163361,#127190,#127191) ;
#100401=AXIS2_PLACEMENT_3D('',#163362,#127192,#127193) ;
#100402=AXIS2_PLACEMENT_3D('',#163363,#127194,#127195) ;
#100403=AXIS2_PLACEMENT_3D('',#163365,#127196,#127197) ;
#100404=AXIS2_PLACEMENT_3D('',#163367,#127198,#127199) ;
#100405=AXIS2_PLACEMENT_3D('',#163368,#127200,#127201) ;
#100406=AXIS2_PLACEMENT_3D('',#163370,#127202,#127203) ;
#100407=AXIS2_PLACEMENT_3D('',#163371,#127204,#127205) ;
#100408=AXIS2_PLACEMENT_3D('',#163372,#127206,#127207) ;
#100409=AXIS2_PLACEMENT_3D('',#163373,#127208,#127209) ;
#100410=AXIS2_PLACEMENT_3D('',#163374,#127210,#127211) ;
#100411=AXIS2_PLACEMENT_3D('',#163375,#127212,#127213) ;
#100412=AXIS2_PLACEMENT_3D('',#163376,#127214,#127215) ;
#100413=AXIS2_PLACEMENT_3D('',#163377,#127216,#127217) ;
#100414=AXIS2_PLACEMENT_3D('',#163378,#127218,#127219) ;
#100415=AXIS2_PLACEMENT_3D('',#163379,#127220,#127221) ;
#100416=AXIS2_PLACEMENT_3D('',#163380,#127222,#127223) ;
#100417=AXIS2_PLACEMENT_3D('',#163381,#127224,#127225) ;
#100418=AXIS2_PLACEMENT_3D('',#163382,#127226,#127227) ;
#100419=AXIS2_PLACEMENT_3D('',#163383,#127228,#127229) ;
#100420=AXIS2_PLACEMENT_3D('',#163384,#127230,#127231) ;
#100421=AXIS2_PLACEMENT_3D('',#163385,#127232,#127233) ;
#100422=AXIS2_PLACEMENT_3D('',#163386,#127234,#127235) ;
#100423=AXIS2_PLACEMENT_3D('',#163387,#127236,#127237) ;
#100424=AXIS2_PLACEMENT_3D('',#163388,#127238,#127239) ;
#100425=AXIS2_PLACEMENT_3D('',#163389,#127240,#127241) ;
#100426=AXIS2_PLACEMENT_3D('',#163390,#127242,#127243) ;
#100427=AXIS2_PLACEMENT_3D('',#163391,#127244,#127245) ;
#100428=AXIS2_PLACEMENT_3D('',#163392,#127246,#127247) ;
#100429=AXIS2_PLACEMENT_3D('',#163393,#127248,#127249) ;
#100430=AXIS2_PLACEMENT_3D('',#163394,#127250,#127251) ;
#100431=AXIS2_PLACEMENT_3D('',#163395,#127252,#127253) ;
#100432=AXIS2_PLACEMENT_3D('',#163396,#127254,#127255) ;
#100433=AXIS2_PLACEMENT_3D('',#163397,#127256,#127257) ;
#100434=AXIS2_PLACEMENT_3D('',#163398,#127258,#127259) ;
#100435=AXIS2_PLACEMENT_3D('',#163399,#127260,#127261) ;
#100436=AXIS2_PLACEMENT_3D('',#163400,#127262,#127263) ;
#100437=AXIS2_PLACEMENT_3D('',#163401,#127264,#127265) ;
#100438=AXIS2_PLACEMENT_3D('',#163402,#127266,#127267) ;
#100439=AXIS2_PLACEMENT_3D('',#163403,#127268,#127269) ;
#100440=AXIS2_PLACEMENT_3D('',#163404,#127270,#127271) ;
#100441=AXIS2_PLACEMENT_3D('',#163405,#127272,#127273) ;
#100442=AXIS2_PLACEMENT_3D('',#163406,#127274,#127275) ;
#100443=AXIS2_PLACEMENT_3D('',#163407,#127276,#127277) ;
#100444=AXIS2_PLACEMENT_3D('',#163408,#127278,#127279) ;
#100445=AXIS2_PLACEMENT_3D('',#163409,#127280,#127281) ;
#100446=AXIS2_PLACEMENT_3D('',#163410,#127282,#127283) ;
#100447=AXIS2_PLACEMENT_3D('',#163411,#127284,#127285) ;
#100448=AXIS2_PLACEMENT_3D('',#163412,#127286,#127287) ;
#100449=AXIS2_PLACEMENT_3D('',#163413,#127288,#127289) ;
#100450=AXIS2_PLACEMENT_3D('',#163414,#127290,#127291) ;
#100451=AXIS2_PLACEMENT_3D('',#163415,#127292,#127293) ;
#100452=AXIS2_PLACEMENT_3D('',#163416,#127294,#127295) ;
#100453=AXIS2_PLACEMENT_3D('',#163417,#127296,#127297) ;
#100454=AXIS2_PLACEMENT_3D('',#163418,#127298,#127299) ;
#100455=AXIS2_PLACEMENT_3D('',#163419,#127300,#127301) ;
#100456=AXIS2_PLACEMENT_3D('',#163420,#127302,#127303) ;
#100457=AXIS2_PLACEMENT_3D('',#163421,#127304,#127305) ;
#100458=AXIS2_PLACEMENT_3D('',#163422,#127306,#127307) ;
#100459=AXIS2_PLACEMENT_3D('',#163423,#127308,#127309) ;
#100460=AXIS2_PLACEMENT_3D('',#163424,#127310,#127311) ;
#100461=AXIS2_PLACEMENT_3D('',#163425,#127312,#127313) ;
#100462=AXIS2_PLACEMENT_3D('',#163426,#127314,#127315) ;
#100463=AXIS2_PLACEMENT_3D('',#163427,#127316,#127317) ;
#100464=AXIS2_PLACEMENT_3D('',#163428,#127318,#127319) ;
#100465=AXIS2_PLACEMENT_3D('',#163429,#127320,#127321) ;
#100466=AXIS2_PLACEMENT_3D('',#163430,#127322,#127323) ;
#100467=AXIS2_PLACEMENT_3D('',#163431,#127324,#127325) ;
#100468=AXIS2_PLACEMENT_3D('',#163432,#127326,#127327) ;
#100469=AXIS2_PLACEMENT_3D('',#163433,#127328,#127329) ;
#100470=AXIS2_PLACEMENT_3D('',#163434,#127330,#127331) ;
#100471=AXIS2_PLACEMENT_3D('',#163435,#127332,#127333) ;
#100472=AXIS2_PLACEMENT_3D('',#163436,#127334,#127335) ;
#100473=AXIS2_PLACEMENT_3D('',#163437,#127336,#127337) ;
#100474=AXIS2_PLACEMENT_3D('',#163438,#127338,#127339) ;
#100475=AXIS2_PLACEMENT_3D('',#163439,#127340,#127341) ;
#100476=AXIS2_PLACEMENT_3D('',#163440,#127342,#127343) ;
#100477=AXIS2_PLACEMENT_3D('',#163441,#127344,#127345) ;
#100478=AXIS2_PLACEMENT_3D('',#163442,#127346,#127347) ;
#100479=AXIS2_PLACEMENT_3D('',#163443,#127348,#127349) ;
#100480=AXIS2_PLACEMENT_3D('',#163444,#127350,#127351) ;
#100481=AXIS2_PLACEMENT_3D('',#163445,#127352,#127353) ;
#100482=AXIS2_PLACEMENT_3D('',#163446,#127354,#127355) ;
#100483=AXIS2_PLACEMENT_3D('',#163447,#127356,#127357) ;
#100484=AXIS2_PLACEMENT_3D('',#163448,#127358,#127359) ;
#100485=AXIS2_PLACEMENT_3D('',#163449,#127360,#127361) ;
#100486=AXIS2_PLACEMENT_3D('',#163450,#127362,#127363) ;
#100487=AXIS2_PLACEMENT_3D('',#163451,#127364,#127365) ;
#100488=AXIS2_PLACEMENT_3D('',#163452,#127366,#127367) ;
#100489=AXIS2_PLACEMENT_3D('',#163453,#127368,#127369) ;
#100490=AXIS2_PLACEMENT_3D('',#163454,#127370,#127371) ;
#100491=AXIS2_PLACEMENT_3D('',#163455,#127372,#127373) ;
#100492=AXIS2_PLACEMENT_3D('',#163456,#127374,#127375) ;
#100493=AXIS2_PLACEMENT_3D('',#163457,#127376,#127377) ;
#100494=AXIS2_PLACEMENT_3D('',#163458,#127378,#127379) ;
#100495=AXIS2_PLACEMENT_3D('',#163459,#127380,#127381) ;
#100496=AXIS2_PLACEMENT_3D('',#163460,#127382,#127383) ;
#100497=AXIS2_PLACEMENT_3D('',#163461,#127384,#127385) ;
#100498=AXIS2_PLACEMENT_3D('',#163462,#127386,#127387) ;
#100499=AXIS2_PLACEMENT_3D('',#163463,#127388,#127389) ;
#100500=AXIS2_PLACEMENT_3D('',#163464,#127390,#127391) ;
#100501=AXIS2_PLACEMENT_3D('',#163465,#127392,#127393) ;
#100502=AXIS2_PLACEMENT_3D('',#163466,#127394,#127395) ;
#100503=AXIS2_PLACEMENT_3D('',#163467,#127396,#127397) ;
#100504=AXIS2_PLACEMENT_3D('',#163468,#127398,#127399) ;
#100505=AXIS2_PLACEMENT_3D('',#163469,#127400,#127401) ;
#100506=AXIS2_PLACEMENT_3D('',#163470,#127402,#127403) ;
#100507=AXIS2_PLACEMENT_3D('',#163471,#127404,#127405) ;
#100508=AXIS2_PLACEMENT_3D('',#163472,#127406,#127407) ;
#100509=AXIS2_PLACEMENT_3D('',#163473,#127408,#127409) ;
#100510=AXIS2_PLACEMENT_3D('',#163474,#127410,#127411) ;
#100511=AXIS2_PLACEMENT_3D('',#163475,#127412,#127413) ;
#100512=AXIS2_PLACEMENT_3D('',#163476,#127414,#127415) ;
#100513=AXIS2_PLACEMENT_3D('',#163477,#127416,#127417) ;
#100514=AXIS2_PLACEMENT_3D('',#163478,#127418,#127419) ;
#100515=AXIS2_PLACEMENT_3D('',#163479,#127420,#127421) ;
#100516=AXIS2_PLACEMENT_3D('',#163480,#127422,#127423) ;
#100517=AXIS2_PLACEMENT_3D('',#163481,#127424,#127425) ;
#100518=AXIS2_PLACEMENT_3D('',#163482,#127426,#127427) ;
#100519=AXIS2_PLACEMENT_3D('',#163483,#127428,#127429) ;
#100520=AXIS2_PLACEMENT_3D('',#163484,#127430,#127431) ;
#100521=AXIS2_PLACEMENT_3D('',#163485,#127432,#127433) ;
#100522=AXIS2_PLACEMENT_3D('',#163486,#127434,#127435) ;
#100523=AXIS2_PLACEMENT_3D('',#163487,#127436,#127437) ;
#100524=AXIS2_PLACEMENT_3D('',#163488,#127438,#127439) ;
#100525=AXIS2_PLACEMENT_3D('',#163489,#127440,#127441) ;
#100526=AXIS2_PLACEMENT_3D('',#163490,#127442,#127443) ;
#100527=AXIS2_PLACEMENT_3D('',#163491,#127444,#127445) ;
#100528=AXIS2_PLACEMENT_3D('',#163492,#127446,#127447) ;
#100529=AXIS2_PLACEMENT_3D('',#163493,#127448,#127449) ;
#100530=AXIS2_PLACEMENT_3D('',#163494,#127450,#127451) ;
#100531=AXIS2_PLACEMENT_3D('',#163495,#127452,#127453) ;
#100532=AXIS2_PLACEMENT_3D('',#163496,#127454,#127455) ;
#100533=AXIS2_PLACEMENT_3D('',#163497,#127456,#127457) ;
#100534=AXIS2_PLACEMENT_3D('',#163498,#127458,#127459) ;
#100535=AXIS2_PLACEMENT_3D('',#163499,#127460,#127461) ;
#100536=AXIS2_PLACEMENT_3D('',#163500,#127462,#127463) ;
#100537=AXIS2_PLACEMENT_3D('',#163501,#127464,#127465) ;
#100538=AXIS2_PLACEMENT_3D('',#163502,#127466,#127467) ;
#100539=AXIS2_PLACEMENT_3D('',#163503,#127468,#127469) ;
#100540=AXIS2_PLACEMENT_3D('',#163504,#127470,#127471) ;
#100541=AXIS2_PLACEMENT_3D('',#163505,#127472,#127473) ;
#100542=AXIS2_PLACEMENT_3D('',#163506,#127474,#127475) ;
#100543=AXIS2_PLACEMENT_3D('',#163507,#127476,#127477) ;
#100544=AXIS2_PLACEMENT_3D('',#163508,#127478,#127479) ;
#100545=AXIS2_PLACEMENT_3D('',#163509,#127480,#127481) ;
#100546=AXIS2_PLACEMENT_3D('',#163510,#127482,#127483) ;
#100547=AXIS2_PLACEMENT_3D('',#163511,#127484,#127485) ;
#100548=AXIS2_PLACEMENT_3D('',#163512,#127486,#127487) ;
#100549=AXIS2_PLACEMENT_3D('',#163513,#127488,#127489) ;
#100550=AXIS2_PLACEMENT_3D('',#163514,#127490,#127491) ;
#100551=AXIS2_PLACEMENT_3D('',#163515,#127492,#127493) ;
#100552=AXIS2_PLACEMENT_3D('',#163516,#127494,#127495) ;
#100553=AXIS2_PLACEMENT_3D('',#163517,#127496,#127497) ;
#100554=AXIS2_PLACEMENT_3D('',#163518,#127498,#127499) ;
#100555=AXIS2_PLACEMENT_3D('',#163519,#127500,#127501) ;
#100556=AXIS2_PLACEMENT_3D('',#163520,#127502,#127503) ;
#100557=AXIS2_PLACEMENT_3D('',#163521,#127504,#127505) ;
#100558=AXIS2_PLACEMENT_3D('',#163522,#127506,#127507) ;
#100559=AXIS2_PLACEMENT_3D('',#163523,#127508,#127509) ;
#100560=AXIS2_PLACEMENT_3D('',#163524,#127510,#127511) ;
#100561=AXIS2_PLACEMENT_3D('',#163525,#127512,#127513) ;
#100562=AXIS2_PLACEMENT_3D('',#163526,#127514,#127515) ;
#100563=AXIS2_PLACEMENT_3D('',#163527,#127516,#127517) ;
#100564=AXIS2_PLACEMENT_3D('',#163528,#127518,#127519) ;
#100565=AXIS2_PLACEMENT_3D('',#163529,#127520,#127521) ;
#100566=AXIS2_PLACEMENT_3D('',#163530,#127522,#127523) ;
#100567=AXIS2_PLACEMENT_3D('',#163531,#127524,#127525) ;
#100568=AXIS2_PLACEMENT_3D('',#163532,#127526,#127527) ;
#100569=AXIS2_PLACEMENT_3D('',#163533,#127528,#127529) ;
#100570=AXIS2_PLACEMENT_3D('',#163534,#127530,#127531) ;
#100571=AXIS2_PLACEMENT_3D('',#163535,#127532,#127533) ;
#100572=AXIS2_PLACEMENT_3D('',#163536,#127534,#127535) ;
#100573=AXIS2_PLACEMENT_3D('',#163537,#127536,#127537) ;
#100574=AXIS2_PLACEMENT_3D('',#163538,#127538,#127539) ;
#100575=AXIS2_PLACEMENT_3D('',#163539,#127540,#127541) ;
#100576=AXIS2_PLACEMENT_3D('',#163540,#127542,#127543) ;
#100577=AXIS2_PLACEMENT_3D('',#163541,#127544,#127545) ;
#100578=AXIS2_PLACEMENT_3D('',#163542,#127546,#127547) ;
#100579=AXIS2_PLACEMENT_3D('',#163543,#127548,#127549) ;
#100580=AXIS2_PLACEMENT_3D('',#163544,#127550,#127551) ;
#100581=AXIS2_PLACEMENT_3D('',#163545,#127552,#127553) ;
#100582=AXIS2_PLACEMENT_3D('',#163570,#127554,#127555) ;
#100583=AXIS2_PLACEMENT_3D('',#163571,#127556,#127557) ;
#100584=AXIS2_PLACEMENT_3D('',#163572,#127558,#127559) ;
#100585=AXIS2_PLACEMENT_3D('',#163597,#127560,#127561) ;
#100586=AXIS2_PLACEMENT_3D('',#163598,#127562,#127563) ;
#100587=AXIS2_PLACEMENT_3D('',#163599,#127564,#127565) ;
#100588=AXIS2_PLACEMENT_3D('',#163600,#127566,#127567) ;
#100589=AXIS2_PLACEMENT_3D('',#163625,#127568,#127569) ;
#100590=AXIS2_PLACEMENT_3D('',#163626,#127570,#127571) ;
#100591=AXIS2_PLACEMENT_3D('',#163627,#127572,#127573) ;
#100592=AXIS2_PLACEMENT_3D('',#163628,#127574,#127575) ;
#100593=AXIS2_PLACEMENT_3D('',#163629,#127576,#127577) ;
#100594=AXIS2_PLACEMENT_3D('',#163630,#127578,#127579) ;
#100595=AXIS2_PLACEMENT_3D('',#163631,#127580,#127581) ;
#100596=AXIS2_PLACEMENT_3D('',#163632,#127582,#127583) ;
#100597=AXIS2_PLACEMENT_3D('',#163633,#127584,#127585) ;
#100598=AXIS2_PLACEMENT_3D('',#163634,#127586,#127587) ;
#100599=AXIS2_PLACEMENT_3D('',#163635,#127588,#127589) ;
#100600=AXIS2_PLACEMENT_3D('',#163636,#127590,#127591) ;
#100601=AXIS2_PLACEMENT_3D('',#163637,#127592,#127593) ;
#100602=AXIS2_PLACEMENT_3D('',#163638,#127594,#127595) ;
#100603=AXIS2_PLACEMENT_3D('',#163639,#127596,#127597) ;
#100604=AXIS2_PLACEMENT_3D('',#163640,#127598,#127599) ;
#100605=AXIS2_PLACEMENT_3D('',#163641,#127600,#127601) ;
#100606=AXIS2_PLACEMENT_3D('',#163642,#127602,#127603) ;
#100607=AXIS2_PLACEMENT_3D('',#163643,#127604,#127605) ;
#100608=AXIS2_PLACEMENT_3D('',#163644,#127606,#127607) ;
#100609=AXIS2_PLACEMENT_3D('',#163645,#127608,#127609) ;
#100610=AXIS2_PLACEMENT_3D('',#163694,#127610,#127611) ;
#100611=AXIS2_PLACEMENT_3D('',#163707,#127612,#127613) ;
#100612=AXIS2_PLACEMENT_3D('',#163708,#127614,#127615) ;
#100613=AXIS2_PLACEMENT_3D('',#163709,#127616,#127617) ;
#100614=AXIS2_PLACEMENT_3D('',#163710,#127618,#127619) ;
#100615=AXIS2_PLACEMENT_3D('',#163711,#127620,#127621) ;
#100616=AXIS2_PLACEMENT_3D('',#163712,#127622,#127623) ;
#100617=AXIS2_PLACEMENT_3D('',#163713,#127624,#127625) ;
#100618=AXIS2_PLACEMENT_3D('',#163714,#127626,#127627) ;
#100619=AXIS2_PLACEMENT_3D('',#163715,#127628,#127629) ;
#100620=AXIS2_PLACEMENT_3D('',#163716,#127630,#127631) ;
#100621=AXIS2_PLACEMENT_3D('',#163717,#127632,#127633) ;
#100622=AXIS2_PLACEMENT_3D('',#163718,#127634,#127635) ;
#100623=AXIS2_PLACEMENT_3D('',#163719,#127636,#127637) ;
#100624=AXIS2_PLACEMENT_3D('',#163720,#127638,#127639) ;
#100625=AXIS2_PLACEMENT_3D('',#163721,#127640,#127641) ;
#100626=AXIS2_PLACEMENT_3D('',#163734,#127642,#127643) ;
#100627=AXIS2_PLACEMENT_3D('',#163759,#127644,#127645) ;
#100628=AXIS2_PLACEMENT_3D('',#163772,#127646,#127647) ;
#100629=AXIS2_PLACEMENT_3D('',#163773,#127648,#127649) ;
#100630=AXIS2_PLACEMENT_3D('',#163774,#127650,#127651) ;
#100631=AXIS2_PLACEMENT_3D('',#163775,#127652,#127653) ;
#100632=AXIS2_PLACEMENT_3D('',#163776,#127654,#127655) ;
#100633=AXIS2_PLACEMENT_3D('',#163777,#127656,#127657) ;
#100634=AXIS2_PLACEMENT_3D('',#163778,#127658,#127659) ;
#100635=AXIS2_PLACEMENT_3D('',#163779,#127660,#127661) ;
#100636=AXIS2_PLACEMENT_3D('',#163780,#127662,#127663) ;
#100637=AXIS2_PLACEMENT_3D('',#163781,#127664,#127665) ;
#100638=AXIS2_PLACEMENT_3D('',#163782,#127666,#127667) ;
#100639=AXIS2_PLACEMENT_3D('',#163783,#127668,#127669) ;
#100640=AXIS2_PLACEMENT_3D('',#163784,#127670,#127671) ;
#100641=AXIS2_PLACEMENT_3D('',#163785,#127672,#127673) ;
#100642=AXIS2_PLACEMENT_3D('',#163786,#127674,#127675) ;
#100643=AXIS2_PLACEMENT_3D('',#163799,#127676,#127677) ;
#100644=AXIS2_PLACEMENT_3D('',#163824,#127678,#127679) ;
#100645=AXIS2_PLACEMENT_3D('',#163825,#127680,#127681) ;
#100646=AXIS2_PLACEMENT_3D('',#163826,#127682,#127683) ;
#100647=AXIS2_PLACEMENT_3D('',#163827,#127684,#127685) ;
#100648=AXIS2_PLACEMENT_3D('',#163828,#127686,#127687) ;
#100649=AXIS2_PLACEMENT_3D('',#163829,#127688,#127689) ;
#100650=AXIS2_PLACEMENT_3D('',#163830,#127690,#127691) ;
#100651=AXIS2_PLACEMENT_3D('',#163831,#127692,#127693) ;
#100652=AXIS2_PLACEMENT_3D('',#163832,#127694,#127695) ;
#100653=AXIS2_PLACEMENT_3D('',#163833,#127696,#127697) ;
#100654=AXIS2_PLACEMENT_3D('',#163834,#127698,#127699) ;
#100655=AXIS2_PLACEMENT_3D('',#163835,#127700,#127701) ;
#100656=AXIS2_PLACEMENT_3D('',#163836,#127702,#127703) ;
#100657=AXIS2_PLACEMENT_3D('',#163837,#127704,#127705) ;
#100658=AXIS2_PLACEMENT_3D('',#163838,#127706,#127707) ;
#100659=AXIS2_PLACEMENT_3D('',#163839,#127708,#127709) ;
#100660=AXIS2_PLACEMENT_3D('',#163840,#127710,#127711) ;
#100661=AXIS2_PLACEMENT_3D('',#163841,#127712,#127713) ;
#100662=AXIS2_PLACEMENT_3D('',#163842,#127714,#127715) ;
#100663=AXIS2_PLACEMENT_3D('',#163843,#127716,#127717) ;
#100664=AXIS2_PLACEMENT_3D('',#163844,#127718,#127719) ;
#100665=AXIS2_PLACEMENT_3D('',#163845,#127720,#127721) ;
#100666=AXIS2_PLACEMENT_3D('',#163846,#127722,#127723) ;
#100667=AXIS2_PLACEMENT_3D('',#163847,#127724,#127725) ;
#100668=AXIS2_PLACEMENT_3D('',#163848,#127726,#127727) ;
#100669=AXIS2_PLACEMENT_3D('',#163849,#127728,#127729) ;
#100670=AXIS2_PLACEMENT_3D('',#163850,#127730,#127731) ;
#100671=AXIS2_PLACEMENT_3D('',#163851,#127732,#127733) ;
#100672=AXIS2_PLACEMENT_3D('',#163852,#127734,#127735) ;
#100673=AXIS2_PLACEMENT_3D('',#163853,#127736,#127737) ;
#100674=AXIS2_PLACEMENT_3D('',#163854,#127738,#127739) ;
#100675=AXIS2_PLACEMENT_3D('',#163855,#127740,#127741) ;
#100676=AXIS2_PLACEMENT_3D('',#163856,#127742,#127743) ;
#100677=AXIS2_PLACEMENT_3D('',#163857,#127744,#127745) ;
#100678=AXIS2_PLACEMENT_3D('',#163858,#127746,#127747) ;
#100679=AXIS2_PLACEMENT_3D('',#163859,#127748,#127749) ;
#100680=AXIS2_PLACEMENT_3D('',#163860,#127750,#127751) ;
#100681=AXIS2_PLACEMENT_3D('',#163861,#127752,#127753) ;
#100682=AXIS2_PLACEMENT_3D('',#163862,#127754,#127755) ;
#100683=AXIS2_PLACEMENT_3D('',#163863,#127756,#127757) ;
#100684=AXIS2_PLACEMENT_3D('',#163864,#127758,#127759) ;
#100685=AXIS2_PLACEMENT_3D('',#163865,#127760,#127761) ;
#100686=AXIS2_PLACEMENT_3D('',#163866,#127762,#127763) ;
#100687=AXIS2_PLACEMENT_3D('',#163867,#127764,#127765) ;
#100688=AXIS2_PLACEMENT_3D('',#163868,#127766,#127767) ;
#100689=AXIS2_PLACEMENT_3D('',#163869,#127768,#127769) ;
#100690=AXIS2_PLACEMENT_3D('',#163870,#127770,#127771) ;
#100691=AXIS2_PLACEMENT_3D('',#163871,#127772,#127773) ;
#100692=AXIS2_PLACEMENT_3D('',#163872,#127774,#127775) ;
#100693=AXIS2_PLACEMENT_3D('',#163873,#127776,#127777) ;
#100694=AXIS2_PLACEMENT_3D('',#163874,#127778,#127779) ;
#100695=AXIS2_PLACEMENT_3D('',#163875,#127780,#127781) ;
#100696=AXIS2_PLACEMENT_3D('',#163876,#127782,#127783) ;
#100697=AXIS2_PLACEMENT_3D('',#163877,#127784,#127785) ;
#100698=AXIS2_PLACEMENT_3D('',#163878,#127786,#127787) ;
#100699=AXIS2_PLACEMENT_3D('',#163879,#127788,#127789) ;
#100700=AXIS2_PLACEMENT_3D('',#163880,#127790,#127791) ;
#100701=AXIS2_PLACEMENT_3D('',#163881,#127792,#127793) ;
#100702=AXIS2_PLACEMENT_3D('',#163882,#127794,#127795) ;
#100703=AXIS2_PLACEMENT_3D('',#163883,#127796,#127797) ;
#100704=AXIS2_PLACEMENT_3D('',#163884,#127798,#127799) ;
#100705=AXIS2_PLACEMENT_3D('',#163885,#127800,#127801) ;
#100706=AXIS2_PLACEMENT_3D('',#163886,#127802,#127803) ;
#100707=AXIS2_PLACEMENT_3D('',#163887,#127804,#127805) ;
#100708=AXIS2_PLACEMENT_3D('',#163888,#127806,#127807) ;
#100709=AXIS2_PLACEMENT_3D('',#163889,#127808,#127809) ;
#100710=AXIS2_PLACEMENT_3D('',#163890,#127810,#127811) ;
#100711=AXIS2_PLACEMENT_3D('',#163891,#127812,#127813) ;
#100712=AXIS2_PLACEMENT_3D('',#163892,#127814,#127815) ;
#100713=AXIS2_PLACEMENT_3D('',#163893,#127816,#127817) ;
#100714=AXIS2_PLACEMENT_3D('',#163894,#127818,#127819) ;
#100715=AXIS2_PLACEMENT_3D('',#163895,#127820,#127821) ;
#100716=AXIS2_PLACEMENT_3D('',#163896,#127822,#127823) ;
#100717=AXIS2_PLACEMENT_3D('',#163897,#127824,#127825) ;
#100718=AXIS2_PLACEMENT_3D('',#163898,#127826,#127827) ;
#100719=AXIS2_PLACEMENT_3D('',#163899,#127828,#127829) ;
#100720=AXIS2_PLACEMENT_3D('',#163900,#127830,#127831) ;
#100721=AXIS2_PLACEMENT_3D('',#163901,#127832,#127833) ;
#100722=AXIS2_PLACEMENT_3D('',#163902,#127834,#127835) ;
#100723=AXIS2_PLACEMENT_3D('',#163903,#127836,#127837) ;
#100724=AXIS2_PLACEMENT_3D('',#163904,#127838,#127839) ;
#100725=AXIS2_PLACEMENT_3D('',#163905,#127840,#127841) ;
#100726=AXIS2_PLACEMENT_3D('',#163906,#127842,#127843) ;
#100727=AXIS2_PLACEMENT_3D('',#163907,#127844,#127845) ;
#100728=AXIS2_PLACEMENT_3D('',#163908,#127846,#127847) ;
#100729=AXIS2_PLACEMENT_3D('',#163909,#127848,#127849) ;
#100730=AXIS2_PLACEMENT_3D('',#163910,#127850,#127851) ;
#100731=AXIS2_PLACEMENT_3D('',#163911,#127852,#127853) ;
#100732=AXIS2_PLACEMENT_3D('',#163912,#127854,#127855) ;
#100733=AXIS2_PLACEMENT_3D('',#163913,#127856,#127857) ;
#100734=AXIS2_PLACEMENT_3D('',#163914,#127858,#127859) ;
#100735=AXIS2_PLACEMENT_3D('',#163915,#127860,#127861) ;
#100736=AXIS2_PLACEMENT_3D('',#163916,#127862,#127863) ;
#100737=AXIS2_PLACEMENT_3D('',#163917,#127864,#127865) ;
#100738=AXIS2_PLACEMENT_3D('',#163918,#127866,#127867) ;
#100739=AXIS2_PLACEMENT_3D('',#163919,#127868,#127869) ;
#100740=AXIS2_PLACEMENT_3D('',#163920,#127870,#127871) ;
#100741=AXIS2_PLACEMENT_3D('',#163921,#127872,#127873) ;
#100742=AXIS2_PLACEMENT_3D('',#163922,#127874,#127875) ;
#100743=AXIS2_PLACEMENT_3D('',#163923,#127876,#127877) ;
#100744=AXIS2_PLACEMENT_3D('',#163924,#127878,#127879) ;
#100745=AXIS2_PLACEMENT_3D('',#163925,#127880,#127881) ;
#100746=AXIS2_PLACEMENT_3D('',#163926,#127882,#127883) ;
#100747=AXIS2_PLACEMENT_3D('',#163927,#127884,#127885) ;
#100748=AXIS2_PLACEMENT_3D('',#163928,#127886,#127887) ;
#100749=AXIS2_PLACEMENT_3D('',#163929,#127888,#127889) ;
#100750=AXIS2_PLACEMENT_3D('',#163930,#127890,#127891) ;
#100751=AXIS2_PLACEMENT_3D('',#163931,#127892,#127893) ;
#100752=AXIS2_PLACEMENT_3D('',#163932,#127894,#127895) ;
#100753=AXIS2_PLACEMENT_3D('',#163933,#127896,#127897) ;
#100754=AXIS2_PLACEMENT_3D('',#163934,#127898,#127899) ;
#100755=AXIS2_PLACEMENT_3D('',#163935,#127900,#127901) ;
#100756=AXIS2_PLACEMENT_3D('',#163936,#127902,#127903) ;
#100757=AXIS2_PLACEMENT_3D('',#163937,#127904,#127905) ;
#100758=AXIS2_PLACEMENT_3D('',#163938,#127906,#127907) ;
#100759=AXIS2_PLACEMENT_3D('',#163939,#127908,#127909) ;
#100760=AXIS2_PLACEMENT_3D('',#163940,#127910,#127911) ;
#100761=AXIS2_PLACEMENT_3D('',#163941,#127912,#127913) ;
#100762=AXIS2_PLACEMENT_3D('',#163942,#127914,#127915) ;
#100763=AXIS2_PLACEMENT_3D('',#163943,#127916,#127917) ;
#100764=AXIS2_PLACEMENT_3D('',#163944,#127918,#127919) ;
#100765=AXIS2_PLACEMENT_3D('',#163945,#127920,#127921) ;
#100766=AXIS2_PLACEMENT_3D('',#163946,#127922,#127923) ;
#100767=AXIS2_PLACEMENT_3D('',#163947,#127924,#127925) ;
#100768=AXIS2_PLACEMENT_3D('',#163948,#127926,#127927) ;
#100769=AXIS2_PLACEMENT_3D('',#163949,#127928,#127929) ;
#100770=AXIS2_PLACEMENT_3D('',#163950,#127930,#127931) ;
#100771=AXIS2_PLACEMENT_3D('',#163951,#127932,#127933) ;
#100772=AXIS2_PLACEMENT_3D('',#163952,#127934,#127935) ;
#100773=AXIS2_PLACEMENT_3D('',#163953,#127936,#127937) ;
#100774=AXIS2_PLACEMENT_3D('',#163954,#127938,#127939) ;
#100775=AXIS2_PLACEMENT_3D('',#163955,#127940,#127941) ;
#100776=AXIS2_PLACEMENT_3D('',#163956,#127942,#127943) ;
#100777=AXIS2_PLACEMENT_3D('',#163957,#127944,#127945) ;
#100778=AXIS2_PLACEMENT_3D('',#163958,#127946,#127947) ;
#100779=AXIS2_PLACEMENT_3D('',#163959,#127948,#127949) ;
#100780=AXIS2_PLACEMENT_3D('',#163960,#127950,#127951) ;
#100781=AXIS2_PLACEMENT_3D('',#163961,#127952,#127953) ;
#100782=AXIS2_PLACEMENT_3D('',#163962,#127954,#127955) ;
#100783=AXIS2_PLACEMENT_3D('',#163963,#127956,#127957) ;
#100784=AXIS2_PLACEMENT_3D('',#163964,#127958,#127959) ;
#100785=AXIS2_PLACEMENT_3D('',#163965,#127960,#127961) ;
#100786=AXIS2_PLACEMENT_3D('',#163966,#127962,#127963) ;
#100787=AXIS2_PLACEMENT_3D('',#163967,#127964,#127965) ;
#100788=AXIS2_PLACEMENT_3D('',#163968,#127966,#127967) ;
#100789=AXIS2_PLACEMENT_3D('',#163969,#127968,#127969) ;
#100790=AXIS2_PLACEMENT_3D('',#163970,#127970,#127971) ;
#100791=AXIS2_PLACEMENT_3D('',#163971,#127972,#127973) ;
#100792=AXIS2_PLACEMENT_3D('',#163972,#127974,#127975) ;
#100793=AXIS2_PLACEMENT_3D('',#163973,#127976,#127977) ;
#100794=AXIS2_PLACEMENT_3D('',#163974,#127978,#127979) ;
#100795=AXIS2_PLACEMENT_3D('',#163975,#127980,#127981) ;
#100796=AXIS2_PLACEMENT_3D('',#163976,#127982,#127983) ;
#100797=AXIS2_PLACEMENT_3D('',#163977,#127984,#127985) ;
#100798=AXIS2_PLACEMENT_3D('',#163978,#127986,#127987) ;
#100799=AXIS2_PLACEMENT_3D('',#163979,#127988,#127989) ;
#100800=AXIS2_PLACEMENT_3D('',#163980,#127990,#127991) ;
#100801=AXIS2_PLACEMENT_3D('',#163981,#127992,#127993) ;
#100802=AXIS2_PLACEMENT_3D('',#163982,#127994,#127995) ;
#100803=AXIS2_PLACEMENT_3D('',#163983,#127996,#127997) ;
#100804=AXIS2_PLACEMENT_3D('',#163984,#127998,#127999) ;
#100805=AXIS2_PLACEMENT_3D('',#163985,#128000,#128001) ;
#100806=AXIS2_PLACEMENT_3D('',#163986,#128002,#128003) ;
#100807=AXIS2_PLACEMENT_3D('',#163987,#128004,#128005) ;
#100808=AXIS2_PLACEMENT_3D('',#163988,#128006,#128007) ;
#100809=AXIS2_PLACEMENT_3D('',#163989,#128008,#128009) ;
#100810=AXIS2_PLACEMENT_3D('',#163990,#128010,#128011) ;
#100811=AXIS2_PLACEMENT_3D('',#163991,#128012,#128013) ;
#100812=AXIS2_PLACEMENT_3D('',#163992,#128014,#128015) ;
#100813=AXIS2_PLACEMENT_3D('',#163993,#128016,#128017) ;
#100814=AXIS2_PLACEMENT_3D('',#163994,#128018,#128019) ;
#100815=AXIS2_PLACEMENT_3D('',#163995,#128020,#128021) ;
#100816=AXIS2_PLACEMENT_3D('',#163996,#128022,#128023) ;
#100817=AXIS2_PLACEMENT_3D('',#163997,#128024,#128025) ;
#100818=AXIS2_PLACEMENT_3D('',#163998,#128026,#128027) ;
#100819=AXIS2_PLACEMENT_3D('',#163999,#128028,#128029) ;
#100820=AXIS2_PLACEMENT_3D('',#164000,#128030,#128031) ;
#100821=AXIS2_PLACEMENT_3D('',#164001,#128032,#128033) ;
#100822=AXIS2_PLACEMENT_3D('',#164002,#128034,#128035) ;
#100823=AXIS2_PLACEMENT_3D('',#164003,#128036,#128037) ;
#100824=AXIS2_PLACEMENT_3D('',#164004,#128038,#128039) ;
#100825=AXIS2_PLACEMENT_3D('',#164005,#128040,#128041) ;
#100826=AXIS2_PLACEMENT_3D('',#164006,#128042,#128043) ;
#100827=AXIS2_PLACEMENT_3D('',#164007,#128044,#128045) ;
#100828=AXIS2_PLACEMENT_3D('',#164008,#128046,#128047) ;
#100829=AXIS2_PLACEMENT_3D('',#164009,#128048,#128049) ;
#100830=AXIS2_PLACEMENT_3D('',#164010,#128050,#128051) ;
#100831=AXIS2_PLACEMENT_3D('',#164011,#128052,#128053) ;
#100832=AXIS2_PLACEMENT_3D('',#164012,#128054,#128055) ;
#100833=AXIS2_PLACEMENT_3D('',#164013,#128056,#128057) ;
#100834=AXIS2_PLACEMENT_3D('',#164014,#128058,#128059) ;
#100835=AXIS2_PLACEMENT_3D('',#164015,#128060,#128061) ;
#100836=AXIS2_PLACEMENT_3D('',#164016,#128062,#128063) ;
#100837=AXIS2_PLACEMENT_3D('',#164017,#128064,#128065) ;
#100838=AXIS2_PLACEMENT_3D('',#164018,#128066,#128067) ;
#100839=AXIS2_PLACEMENT_3D('',#164019,#128068,#128069) ;
#100840=AXIS2_PLACEMENT_3D('',#164020,#128070,#128071) ;
#100841=AXIS2_PLACEMENT_3D('',#164021,#128072,#128073) ;
#100842=AXIS2_PLACEMENT_3D('',#164022,#128074,#128075) ;
#100843=AXIS2_PLACEMENT_3D('',#164023,#128076,#128077) ;
#100844=AXIS2_PLACEMENT_3D('',#164024,#128078,#128079) ;
#100845=AXIS2_PLACEMENT_3D('',#164025,#128080,#128081) ;
#100846=AXIS2_PLACEMENT_3D('',#164026,#128082,#128083) ;
#100847=AXIS2_PLACEMENT_3D('',#164027,#128084,#128085) ;
#100848=AXIS2_PLACEMENT_3D('',#164028,#128086,#128087) ;
#100849=AXIS2_PLACEMENT_3D('',#164029,#128088,#128089) ;
#100850=AXIS2_PLACEMENT_3D('',#164030,#128090,#128091) ;
#100851=AXIS2_PLACEMENT_3D('',#164031,#128092,#128093) ;
#100852=AXIS2_PLACEMENT_3D('',#164032,#128094,#128095) ;
#100853=AXIS2_PLACEMENT_3D('',#164033,#128096,#128097) ;
#100854=AXIS2_PLACEMENT_3D('',#164034,#128098,#128099) ;
#100855=AXIS2_PLACEMENT_3D('',#164035,#128100,#128101) ;
#100856=AXIS2_PLACEMENT_3D('',#164036,#128102,#128103) ;
#100857=AXIS2_PLACEMENT_3D('',#164037,#128104,#128105) ;
#100858=AXIS2_PLACEMENT_3D('',#164062,#128106,#128107) ;
#100859=AXIS2_PLACEMENT_3D('',#164063,#128108,#128109) ;
#100860=AXIS2_PLACEMENT_3D('',#164064,#128110,#128111) ;
#100861=AXIS2_PLACEMENT_3D('',#164089,#128112,#128113) ;
#100862=AXIS2_PLACEMENT_3D('',#164090,#128114,#128115) ;
#100863=AXIS2_PLACEMENT_3D('',#164091,#128116,#128117) ;
#100864=AXIS2_PLACEMENT_3D('',#164092,#128118,#128119) ;
#100865=AXIS2_PLACEMENT_3D('',#164117,#128120,#128121) ;
#100866=AXIS2_PLACEMENT_3D('',#164118,#128122,#128123) ;
#100867=AXIS2_PLACEMENT_3D('',#164119,#128124,#128125) ;
#100868=AXIS2_PLACEMENT_3D('',#164120,#128126,#128127) ;
#100869=AXIS2_PLACEMENT_3D('',#164121,#128128,#128129) ;
#100870=AXIS2_PLACEMENT_3D('',#164122,#128130,#128131) ;
#100871=AXIS2_PLACEMENT_3D('',#164123,#128132,#128133) ;
#100872=AXIS2_PLACEMENT_3D('',#164124,#128134,#128135) ;
#100873=AXIS2_PLACEMENT_3D('',#164125,#128136,#128137) ;
#100874=AXIS2_PLACEMENT_3D('',#164126,#128138,#128139) ;
#100875=AXIS2_PLACEMENT_3D('',#164127,#128140,#128141) ;
#100876=AXIS2_PLACEMENT_3D('',#164128,#128142,#128143) ;
#100877=AXIS2_PLACEMENT_3D('',#164129,#128144,#128145) ;
#100878=AXIS2_PLACEMENT_3D('',#164130,#128146,#128147) ;
#100879=AXIS2_PLACEMENT_3D('',#164131,#128148,#128149) ;
#100880=AXIS2_PLACEMENT_3D('',#164132,#128150,#128151) ;
#100881=AXIS2_PLACEMENT_3D('',#164133,#128152,#128153) ;
#100882=AXIS2_PLACEMENT_3D('',#164134,#128154,#128155) ;
#100883=AXIS2_PLACEMENT_3D('',#164135,#128156,#128157) ;
#100884=AXIS2_PLACEMENT_3D('',#164136,#128158,#128159) ;
#100885=AXIS2_PLACEMENT_3D('',#164137,#128160,#128161) ;
#100886=AXIS2_PLACEMENT_3D('',#164186,#128162,#128163) ;
#100887=AXIS2_PLACEMENT_3D('',#164199,#128164,#128165) ;
#100888=AXIS2_PLACEMENT_3D('',#164200,#128166,#128167) ;
#100889=AXIS2_PLACEMENT_3D('',#164201,#128168,#128169) ;
#100890=AXIS2_PLACEMENT_3D('',#164202,#128170,#128171) ;
#100891=AXIS2_PLACEMENT_3D('',#164203,#128172,#128173) ;
#100892=AXIS2_PLACEMENT_3D('',#164204,#128174,#128175) ;
#100893=AXIS2_PLACEMENT_3D('',#164205,#128176,#128177) ;
#100894=AXIS2_PLACEMENT_3D('',#164206,#128178,#128179) ;
#100895=AXIS2_PLACEMENT_3D('',#164207,#128180,#128181) ;
#100896=AXIS2_PLACEMENT_3D('',#164208,#128182,#128183) ;
#100897=AXIS2_PLACEMENT_3D('',#164209,#128184,#128185) ;
#100898=AXIS2_PLACEMENT_3D('',#164210,#128186,#128187) ;
#100899=AXIS2_PLACEMENT_3D('',#164211,#128188,#128189) ;
#100900=AXIS2_PLACEMENT_3D('',#164212,#128190,#128191) ;
#100901=AXIS2_PLACEMENT_3D('',#164213,#128192,#128193) ;
#100902=AXIS2_PLACEMENT_3D('',#164226,#128194,#128195) ;
#100903=AXIS2_PLACEMENT_3D('',#164251,#128196,#128197) ;
#100904=AXIS2_PLACEMENT_3D('',#164264,#128198,#128199) ;
#100905=AXIS2_PLACEMENT_3D('',#164265,#128200,#128201) ;
#100906=AXIS2_PLACEMENT_3D('',#164266,#128202,#128203) ;
#100907=AXIS2_PLACEMENT_3D('',#164267,#128204,#128205) ;
#100908=AXIS2_PLACEMENT_3D('',#164268,#128206,#128207) ;
#100909=AXIS2_PLACEMENT_3D('',#164269,#128208,#128209) ;
#100910=AXIS2_PLACEMENT_3D('',#164270,#128210,#128211) ;
#100911=AXIS2_PLACEMENT_3D('',#164271,#128212,#128213) ;
#100912=AXIS2_PLACEMENT_3D('',#164272,#128214,#128215) ;
#100913=AXIS2_PLACEMENT_3D('',#164273,#128216,#128217) ;
#100914=AXIS2_PLACEMENT_3D('',#164274,#128218,#128219) ;
#100915=AXIS2_PLACEMENT_3D('',#164275,#128220,#128221) ;
#100916=AXIS2_PLACEMENT_3D('',#164276,#128222,#128223) ;
#100917=AXIS2_PLACEMENT_3D('',#164277,#128224,#128225) ;
#100918=AXIS2_PLACEMENT_3D('',#164278,#128226,#128227) ;
#100919=AXIS2_PLACEMENT_3D('',#164291,#128228,#128229) ;
#100920=AXIS2_PLACEMENT_3D('',#164316,#128230,#128231) ;
#100921=AXIS2_PLACEMENT_3D('',#164317,#128232,#128233) ;
#100922=AXIS2_PLACEMENT_3D('',#164318,#128234,#128235) ;
#100923=AXIS2_PLACEMENT_3D('',#164319,#128236,#128237) ;
#100924=AXIS2_PLACEMENT_3D('',#164320,#128238,#128239) ;
#100925=AXIS2_PLACEMENT_3D('',#164321,#128240,#128241) ;
#100926=AXIS2_PLACEMENT_3D('',#164322,#128242,#128243) ;
#100927=AXIS2_PLACEMENT_3D('',#164323,#128244,#128245) ;
#100928=AXIS2_PLACEMENT_3D('',#164324,#128246,#128247) ;
#100929=AXIS2_PLACEMENT_3D('',#164325,#128248,#128249) ;
#100930=AXIS2_PLACEMENT_3D('',#164326,#128250,#128251) ;
#100931=AXIS2_PLACEMENT_3D('',#164327,#128252,#128253) ;
#100932=AXIS2_PLACEMENT_3D('',#164328,#128254,#128255) ;
#100933=AXIS2_PLACEMENT_3D('',#164329,#128256,#128257) ;
#100934=AXIS2_PLACEMENT_3D('',#164330,#128258,#128259) ;
#100935=AXIS2_PLACEMENT_3D('',#164331,#128260,#128261) ;
#100936=AXIS2_PLACEMENT_3D('',#164332,#128262,#128263) ;
#100937=AXIS2_PLACEMENT_3D('',#164333,#128264,#128265) ;
#100938=AXIS2_PLACEMENT_3D('',#164334,#128266,#128267) ;
#100939=AXIS2_PLACEMENT_3D('',#164335,#128268,#128269) ;
#100940=AXIS2_PLACEMENT_3D('',#164336,#128270,#128271) ;
#100941=AXIS2_PLACEMENT_3D('',#164337,#128272,#128273) ;
#100942=AXIS2_PLACEMENT_3D('',#164338,#128274,#128275) ;
#100943=AXIS2_PLACEMENT_3D('',#164339,#128276,#128277) ;
#100944=AXIS2_PLACEMENT_3D('',#164340,#128278,#128279) ;
#100945=AXIS2_PLACEMENT_3D('',#164341,#128280,#128281) ;
#100946=AXIS2_PLACEMENT_3D('',#164342,#128282,#128283) ;
#100947=AXIS2_PLACEMENT_3D('',#164343,#128284,#128285) ;
#100948=AXIS2_PLACEMENT_3D('',#164344,#128286,#128287) ;
#100949=AXIS2_PLACEMENT_3D('',#164345,#128288,#128289) ;
#100950=AXIS2_PLACEMENT_3D('',#164346,#128290,#128291) ;
#100951=AXIS2_PLACEMENT_3D('',#164347,#128292,#128293) ;
#100952=AXIS2_PLACEMENT_3D('',#164348,#128294,#128295) ;
#100953=AXIS2_PLACEMENT_3D('',#164349,#128296,#128297) ;
#100954=AXIS2_PLACEMENT_3D('',#164350,#128298,#128299) ;
#100955=AXIS2_PLACEMENT_3D('',#164351,#128300,#128301) ;
#100956=AXIS2_PLACEMENT_3D('',#164352,#128302,#128303) ;
#100957=AXIS2_PLACEMENT_3D('',#164353,#128304,#128305) ;
#100958=AXIS2_PLACEMENT_3D('',#164354,#128306,#128307) ;
#100959=AXIS2_PLACEMENT_3D('',#164355,#128308,#128309) ;
#100960=AXIS2_PLACEMENT_3D('',#164356,#128310,#128311) ;
#100961=AXIS2_PLACEMENT_3D('',#164357,#128312,#128313) ;
#100962=AXIS2_PLACEMENT_3D('',#164358,#128314,#128315) ;
#100963=AXIS2_PLACEMENT_3D('',#164359,#128316,#128317) ;
#100964=AXIS2_PLACEMENT_3D('',#164360,#128318,#128319) ;
#100965=AXIS2_PLACEMENT_3D('',#164361,#128320,#128321) ;
#100966=AXIS2_PLACEMENT_3D('',#164362,#128322,#128323) ;
#100967=AXIS2_PLACEMENT_3D('',#164363,#128324,#128325) ;
#100968=AXIS2_PLACEMENT_3D('',#164364,#128326,#128327) ;
#100969=AXIS2_PLACEMENT_3D('',#164365,#128328,#128329) ;
#100970=AXIS2_PLACEMENT_3D('',#164366,#128330,#128331) ;
#100971=AXIS2_PLACEMENT_3D('',#164367,#128332,#128333) ;
#100972=AXIS2_PLACEMENT_3D('',#164368,#128334,#128335) ;
#100973=AXIS2_PLACEMENT_3D('',#164369,#128336,#128337) ;
#100974=AXIS2_PLACEMENT_3D('',#164370,#128338,#128339) ;
#100975=AXIS2_PLACEMENT_3D('',#164371,#128340,#128341) ;
#100976=AXIS2_PLACEMENT_3D('',#164372,#128342,#128343) ;
#100977=AXIS2_PLACEMENT_3D('',#164373,#128344,#128345) ;
#100978=AXIS2_PLACEMENT_3D('',#164374,#128346,#128347) ;
#100979=AXIS2_PLACEMENT_3D('',#164375,#128348,#128349) ;
#100980=AXIS2_PLACEMENT_3D('',#164376,#128350,#128351) ;
#100981=AXIS2_PLACEMENT_3D('',#164377,#128352,#128353) ;
#100982=AXIS2_PLACEMENT_3D('',#164378,#128354,#128355) ;
#100983=AXIS2_PLACEMENT_3D('',#164379,#128356,#128357) ;
#100984=AXIS2_PLACEMENT_3D('',#164380,#128358,#128359) ;
#100985=AXIS2_PLACEMENT_3D('',#164381,#128360,#128361) ;
#100986=AXIS2_PLACEMENT_3D('',#164382,#128362,#128363) ;
#100987=AXIS2_PLACEMENT_3D('',#164383,#128364,#128365) ;
#100988=AXIS2_PLACEMENT_3D('',#164384,#128366,#128367) ;
#100989=AXIS2_PLACEMENT_3D('',#164385,#128368,#128369) ;
#100990=AXIS2_PLACEMENT_3D('',#164386,#128370,#128371) ;
#100991=AXIS2_PLACEMENT_3D('',#164387,#128372,#128373) ;
#100992=AXIS2_PLACEMENT_3D('',#164388,#128374,#128375) ;
#100993=AXIS2_PLACEMENT_3D('',#164389,#128376,#128377) ;
#100994=AXIS2_PLACEMENT_3D('',#164390,#128378,#128379) ;
#100995=AXIS2_PLACEMENT_3D('',#164391,#128380,#128381) ;
#100996=AXIS2_PLACEMENT_3D('',#164392,#128382,#128383) ;
#100997=AXIS2_PLACEMENT_3D('',#164393,#128384,#128385) ;
#100998=AXIS2_PLACEMENT_3D('',#164394,#128386,#128387) ;
#100999=AXIS2_PLACEMENT_3D('',#164395,#128388,#128389) ;
#101000=AXIS2_PLACEMENT_3D('',#164396,#128390,#128391) ;
#101001=AXIS2_PLACEMENT_3D('',#164397,#128392,#128393) ;
#101002=AXIS2_PLACEMENT_3D('',#164398,#128394,#128395) ;
#101003=AXIS2_PLACEMENT_3D('',#164399,#128396,#128397) ;
#101004=AXIS2_PLACEMENT_3D('',#164400,#128398,#128399) ;
#101005=AXIS2_PLACEMENT_3D('',#164401,#128400,#128401) ;
#101006=AXIS2_PLACEMENT_3D('',#164402,#128402,#128403) ;
#101007=AXIS2_PLACEMENT_3D('',#164403,#128404,#128405) ;
#101008=AXIS2_PLACEMENT_3D('',#164404,#128406,#128407) ;
#101009=AXIS2_PLACEMENT_3D('',#164405,#128408,#128409) ;
#101010=AXIS2_PLACEMENT_3D('',#164406,#128410,#128411) ;
#101011=AXIS2_PLACEMENT_3D('',#164407,#128412,#128413) ;
#101012=AXIS2_PLACEMENT_3D('',#164408,#128414,#128415) ;
#101013=AXIS2_PLACEMENT_3D('',#164409,#128416,#128417) ;
#101014=AXIS2_PLACEMENT_3D('',#164410,#128418,#128419) ;
#101015=AXIS2_PLACEMENT_3D('',#164411,#128420,#128421) ;
#101016=AXIS2_PLACEMENT_3D('',#164412,#128422,#128423) ;
#101017=AXIS2_PLACEMENT_3D('',#164413,#128424,#128425) ;
#101018=AXIS2_PLACEMENT_3D('',#164414,#128426,#128427) ;
#101019=AXIS2_PLACEMENT_3D('',#164415,#128428,#128429) ;
#101020=AXIS2_PLACEMENT_3D('',#164416,#128430,#128431) ;
#101021=AXIS2_PLACEMENT_3D('',#164417,#128432,#128433) ;
#101022=AXIS2_PLACEMENT_3D('',#164418,#128434,#128435) ;
#101023=AXIS2_PLACEMENT_3D('',#164419,#128436,#128437) ;
#101024=AXIS2_PLACEMENT_3D('',#164420,#128438,#128439) ;
#101025=AXIS2_PLACEMENT_3D('',#164421,#128440,#128441) ;
#101026=AXIS2_PLACEMENT_3D('',#164422,#128442,#128443) ;
#101027=AXIS2_PLACEMENT_3D('',#164423,#128444,#128445) ;
#101028=AXIS2_PLACEMENT_3D('',#164424,#128446,#128447) ;
#101029=AXIS2_PLACEMENT_3D('',#164425,#128448,#128449) ;
#101030=AXIS2_PLACEMENT_3D('',#164426,#128450,#128451) ;
#101031=AXIS2_PLACEMENT_3D('',#164427,#128452,#128453) ;
#101032=AXIS2_PLACEMENT_3D('',#164428,#128454,#128455) ;
#101033=AXIS2_PLACEMENT_3D('',#164429,#128456,#128457) ;
#101034=AXIS2_PLACEMENT_3D('',#164430,#128458,#128459) ;
#101035=AXIS2_PLACEMENT_3D('',#164431,#128460,#128461) ;
#101036=AXIS2_PLACEMENT_3D('',#164432,#128462,#128463) ;
#101037=AXIS2_PLACEMENT_3D('',#164433,#128464,#128465) ;
#101038=AXIS2_PLACEMENT_3D('',#164434,#128466,#128467) ;
#101039=AXIS2_PLACEMENT_3D('',#164435,#128468,#128469) ;
#101040=AXIS2_PLACEMENT_3D('',#164436,#128470,#128471) ;
#101041=AXIS2_PLACEMENT_3D('',#164437,#128472,#128473) ;
#101042=AXIS2_PLACEMENT_3D('',#164438,#128474,#128475) ;
#101043=AXIS2_PLACEMENT_3D('',#164439,#128476,#128477) ;
#101044=AXIS2_PLACEMENT_3D('',#164440,#128478,#128479) ;
#101045=AXIS2_PLACEMENT_3D('',#164441,#128480,#128481) ;
#101046=AXIS2_PLACEMENT_3D('',#164442,#128482,#128483) ;
#101047=AXIS2_PLACEMENT_3D('',#164443,#128484,#128485) ;
#101048=AXIS2_PLACEMENT_3D('',#164444,#128486,#128487) ;
#101049=AXIS2_PLACEMENT_3D('',#164445,#128488,#128489) ;
#101050=AXIS2_PLACEMENT_3D('',#164446,#128490,#128491) ;
#101051=AXIS2_PLACEMENT_3D('',#164447,#128492,#128493) ;
#101052=AXIS2_PLACEMENT_3D('',#164448,#128494,#128495) ;
#101053=AXIS2_PLACEMENT_3D('',#164449,#128496,#128497) ;
#101054=AXIS2_PLACEMENT_3D('',#164450,#128498,#128499) ;
#101055=AXIS2_PLACEMENT_3D('',#164451,#128500,#128501) ;
#101056=AXIS2_PLACEMENT_3D('',#164452,#128502,#128503) ;
#101057=AXIS2_PLACEMENT_3D('',#164453,#128504,#128505) ;
#101058=AXIS2_PLACEMENT_3D('',#164454,#128506,#128507) ;
#101059=AXIS2_PLACEMENT_3D('',#164455,#128508,#128509) ;
#101060=AXIS2_PLACEMENT_3D('',#164456,#128510,#128511) ;
#101061=AXIS2_PLACEMENT_3D('',#164457,#128512,#128513) ;
#101062=AXIS2_PLACEMENT_3D('',#164458,#128514,#128515) ;
#101063=AXIS2_PLACEMENT_3D('',#164459,#128516,#128517) ;
#101064=AXIS2_PLACEMENT_3D('',#164460,#128518,#128519) ;
#101065=AXIS2_PLACEMENT_3D('',#164461,#128520,#128521) ;
#101066=AXIS2_PLACEMENT_3D('',#164462,#128522,#128523) ;
#101067=AXIS2_PLACEMENT_3D('',#164463,#128524,#128525) ;
#101068=AXIS2_PLACEMENT_3D('',#164464,#128526,#128527) ;
#101069=AXIS2_PLACEMENT_3D('',#164465,#128528,#128529) ;
#101070=AXIS2_PLACEMENT_3D('',#164466,#128530,#128531) ;
#101071=AXIS2_PLACEMENT_3D('',#164467,#128532,#128533) ;
#101072=AXIS2_PLACEMENT_3D('',#164468,#128534,#128535) ;
#101073=AXIS2_PLACEMENT_3D('',#164469,#128536,#128537) ;
#101074=AXIS2_PLACEMENT_3D('',#164470,#128538,#128539) ;
#101075=AXIS2_PLACEMENT_3D('',#164471,#128540,#128541) ;
#101076=AXIS2_PLACEMENT_3D('',#164472,#128542,#128543) ;
#101077=AXIS2_PLACEMENT_3D('',#164473,#128544,#128545) ;
#101078=AXIS2_PLACEMENT_3D('',#164474,#128546,#128547) ;
#101079=AXIS2_PLACEMENT_3D('',#164475,#128548,#128549) ;
#101080=AXIS2_PLACEMENT_3D('',#164476,#128550,#128551) ;
#101081=AXIS2_PLACEMENT_3D('',#164477,#128552,#128553) ;
#101082=AXIS2_PLACEMENT_3D('',#164478,#128554,#128555) ;
#101083=AXIS2_PLACEMENT_3D('',#164479,#128556,#128557) ;
#101084=AXIS2_PLACEMENT_3D('',#164480,#128558,#128559) ;
#101085=AXIS2_PLACEMENT_3D('',#164481,#128560,#128561) ;
#101086=AXIS2_PLACEMENT_3D('',#164482,#128562,#128563) ;
#101087=AXIS2_PLACEMENT_3D('',#164483,#128564,#128565) ;
#101088=AXIS2_PLACEMENT_3D('',#164484,#128566,#128567) ;
#101089=AXIS2_PLACEMENT_3D('',#164485,#128568,#128569) ;
#101090=AXIS2_PLACEMENT_3D('',#164486,#128570,#128571) ;
#101091=AXIS2_PLACEMENT_3D('',#164487,#128572,#128573) ;
#101092=AXIS2_PLACEMENT_3D('',#164488,#128574,#128575) ;
#101093=AXIS2_PLACEMENT_3D('',#164489,#128576,#128577) ;
#101094=AXIS2_PLACEMENT_3D('',#164490,#128578,#128579) ;
#101095=AXIS2_PLACEMENT_3D('',#164491,#128580,#128581) ;
#101096=AXIS2_PLACEMENT_3D('',#164492,#128582,#128583) ;
#101097=AXIS2_PLACEMENT_3D('',#164493,#128584,#128585) ;
#101098=AXIS2_PLACEMENT_3D('',#164494,#128586,#128587) ;
#101099=AXIS2_PLACEMENT_3D('',#164495,#128588,#128589) ;
#101100=AXIS2_PLACEMENT_3D('',#164496,#128590,#128591) ;
#101101=AXIS2_PLACEMENT_3D('',#164497,#128592,#128593) ;
#101102=AXIS2_PLACEMENT_3D('',#164498,#128594,#128595) ;
#101103=AXIS2_PLACEMENT_3D('',#164499,#128596,#128597) ;
#101104=AXIS2_PLACEMENT_3D('',#164500,#128598,#128599) ;
#101105=AXIS2_PLACEMENT_3D('',#164501,#128600,#128601) ;
#101106=AXIS2_PLACEMENT_3D('',#164502,#128602,#128603) ;
#101107=AXIS2_PLACEMENT_3D('',#164503,#128604,#128605) ;
#101108=AXIS2_PLACEMENT_3D('',#164504,#128606,#128607) ;
#101109=AXIS2_PLACEMENT_3D('',#164505,#128608,#128609) ;
#101110=AXIS2_PLACEMENT_3D('',#164506,#128610,#128611) ;
#101111=AXIS2_PLACEMENT_3D('',#164507,#128612,#128613) ;
#101112=AXIS2_PLACEMENT_3D('',#164508,#128614,#128615) ;
#101113=AXIS2_PLACEMENT_3D('',#164509,#128616,#128617) ;
#101114=AXIS2_PLACEMENT_3D('',#164510,#128618,#128619) ;
#101115=AXIS2_PLACEMENT_3D('',#164511,#128620,#128621) ;
#101116=AXIS2_PLACEMENT_3D('',#164512,#128622,#128623) ;
#101117=AXIS2_PLACEMENT_3D('',#164513,#128624,#128625) ;
#101118=AXIS2_PLACEMENT_3D('',#164514,#128626,#128627) ;
#101119=AXIS2_PLACEMENT_3D('',#164515,#128628,#128629) ;
#101120=AXIS2_PLACEMENT_3D('',#164516,#128630,#128631) ;
#101121=AXIS2_PLACEMENT_3D('',#164517,#128632,#128633) ;
#101122=AXIS2_PLACEMENT_3D('',#164518,#128634,#128635) ;
#101123=AXIS2_PLACEMENT_3D('',#164519,#128636,#128637) ;
#101124=AXIS2_PLACEMENT_3D('',#164520,#128638,#128639) ;
#101125=AXIS2_PLACEMENT_3D('',#164521,#128640,#128641) ;
#101126=AXIS2_PLACEMENT_3D('',#164522,#128642,#128643) ;
#101127=AXIS2_PLACEMENT_3D('',#164523,#128644,#128645) ;
#101128=AXIS2_PLACEMENT_3D('',#164524,#128646,#128647) ;
#101129=AXIS2_PLACEMENT_3D('',#164525,#128648,#128649) ;
#101130=AXIS2_PLACEMENT_3D('',#164526,#128650,#128651) ;
#101131=AXIS2_PLACEMENT_3D('',#164527,#128652,#128653) ;
#101132=AXIS2_PLACEMENT_3D('',#164528,#128654,#128655) ;
#101133=AXIS2_PLACEMENT_3D('',#164529,#128656,#128657) ;
#101134=AXIS2_PLACEMENT_3D('',#164554,#128658,#128659) ;
#101135=AXIS2_PLACEMENT_3D('',#164555,#128660,#128661) ;
#101136=AXIS2_PLACEMENT_3D('',#164556,#128662,#128663) ;
#101137=AXIS2_PLACEMENT_3D('',#164581,#128664,#128665) ;
#101138=AXIS2_PLACEMENT_3D('',#164582,#128666,#128667) ;
#101139=AXIS2_PLACEMENT_3D('',#164583,#128668,#128669) ;
#101140=AXIS2_PLACEMENT_3D('',#164584,#128670,#128671) ;
#101141=AXIS2_PLACEMENT_3D('',#164609,#128672,#128673) ;
#101142=AXIS2_PLACEMENT_3D('',#164610,#128674,#128675) ;
#101143=AXIS2_PLACEMENT_3D('',#164611,#128676,#128677) ;
#101144=AXIS2_PLACEMENT_3D('',#164612,#128678,#128679) ;
#101145=AXIS2_PLACEMENT_3D('',#164613,#128680,#128681) ;
#101146=AXIS2_PLACEMENT_3D('',#164614,#128682,#128683) ;
#101147=AXIS2_PLACEMENT_3D('',#164615,#128684,#128685) ;
#101148=AXIS2_PLACEMENT_3D('',#164616,#128686,#128687) ;
#101149=AXIS2_PLACEMENT_3D('',#164617,#128688,#128689) ;
#101150=AXIS2_PLACEMENT_3D('',#164618,#128690,#128691) ;
#101151=AXIS2_PLACEMENT_3D('',#164619,#128692,#128693) ;
#101152=AXIS2_PLACEMENT_3D('',#164620,#128694,#128695) ;
#101153=AXIS2_PLACEMENT_3D('',#164621,#128696,#128697) ;
#101154=AXIS2_PLACEMENT_3D('',#164622,#128698,#128699) ;
#101155=AXIS2_PLACEMENT_3D('',#164623,#128700,#128701) ;
#101156=AXIS2_PLACEMENT_3D('',#164624,#128702,#128703) ;
#101157=AXIS2_PLACEMENT_3D('',#164625,#128704,#128705) ;
#101158=AXIS2_PLACEMENT_3D('',#164626,#128706,#128707) ;
#101159=AXIS2_PLACEMENT_3D('',#164627,#128708,#128709) ;
#101160=AXIS2_PLACEMENT_3D('',#164628,#128710,#128711) ;
#101161=AXIS2_PLACEMENT_3D('',#164629,#128712,#128713) ;
#101162=AXIS2_PLACEMENT_3D('',#164678,#128714,#128715) ;
#101163=AXIS2_PLACEMENT_3D('',#164691,#128716,#128717) ;
#101164=AXIS2_PLACEMENT_3D('',#164692,#128718,#128719) ;
#101165=AXIS2_PLACEMENT_3D('',#164693,#128720,#128721) ;
#101166=AXIS2_PLACEMENT_3D('',#164694,#128722,#128723) ;
#101167=AXIS2_PLACEMENT_3D('',#164695,#128724,#128725) ;
#101168=AXIS2_PLACEMENT_3D('',#164696,#128726,#128727) ;
#101169=AXIS2_PLACEMENT_3D('',#164697,#128728,#128729) ;
#101170=AXIS2_PLACEMENT_3D('',#164698,#128730,#128731) ;
#101171=AXIS2_PLACEMENT_3D('',#164699,#128732,#128733) ;
#101172=AXIS2_PLACEMENT_3D('',#164700,#128734,#128735) ;
#101173=AXIS2_PLACEMENT_3D('',#164701,#128736,#128737) ;
#101174=AXIS2_PLACEMENT_3D('',#164702,#128738,#128739) ;
#101175=AXIS2_PLACEMENT_3D('',#164703,#128740,#128741) ;
#101176=AXIS2_PLACEMENT_3D('',#164704,#128742,#128743) ;
#101177=AXIS2_PLACEMENT_3D('',#164705,#128744,#128745) ;
#101178=AXIS2_PLACEMENT_3D('',#164718,#128746,#128747) ;
#101179=AXIS2_PLACEMENT_3D('',#164743,#128748,#128749) ;
#101180=AXIS2_PLACEMENT_3D('',#164756,#128750,#128751) ;
#101181=AXIS2_PLACEMENT_3D('',#164757,#128752,#128753) ;
#101182=AXIS2_PLACEMENT_3D('',#164758,#128754,#128755) ;
#101183=AXIS2_PLACEMENT_3D('',#164759,#128756,#128757) ;
#101184=AXIS2_PLACEMENT_3D('',#164760,#128758,#128759) ;
#101185=AXIS2_PLACEMENT_3D('',#164761,#128760,#128761) ;
#101186=AXIS2_PLACEMENT_3D('',#164762,#128762,#128763) ;
#101187=AXIS2_PLACEMENT_3D('',#164763,#128764,#128765) ;
#101188=AXIS2_PLACEMENT_3D('',#164764,#128766,#128767) ;
#101189=AXIS2_PLACEMENT_3D('',#164765,#128768,#128769) ;
#101190=AXIS2_PLACEMENT_3D('',#164766,#128770,#128771) ;
#101191=AXIS2_PLACEMENT_3D('',#164767,#128772,#128773) ;
#101192=AXIS2_PLACEMENT_3D('',#164768,#128774,#128775) ;
#101193=AXIS2_PLACEMENT_3D('',#164769,#128776,#128777) ;
#101194=AXIS2_PLACEMENT_3D('',#164770,#128778,#128779) ;
#101195=AXIS2_PLACEMENT_3D('',#164783,#128780,#128781) ;
#101196=AXIS2_PLACEMENT_3D('',#164808,#128782,#128783) ;
#101197=AXIS2_PLACEMENT_3D('',#164809,#128784,#128785) ;
#101198=AXIS2_PLACEMENT_3D('',#164810,#128786,#128787) ;
#101199=AXIS2_PLACEMENT_3D('',#164811,#128788,#128789) ;
#101200=AXIS2_PLACEMENT_3D('',#164812,#128790,#128791) ;
#101201=AXIS2_PLACEMENT_3D('',#164813,#128792,#128793) ;
#101202=AXIS2_PLACEMENT_3D('',#164814,#128794,#128795) ;
#101203=AXIS2_PLACEMENT_3D('',#164815,#128796,#128797) ;
#101204=AXIS2_PLACEMENT_3D('',#164816,#128798,#128799) ;
#101205=AXIS2_PLACEMENT_3D('',#164817,#128800,#128801) ;
#101206=AXIS2_PLACEMENT_3D('',#164818,#128802,#128803) ;
#101207=AXIS2_PLACEMENT_3D('',#164819,#128804,#128805) ;
#101208=AXIS2_PLACEMENT_3D('',#164820,#128806,#128807) ;
#101209=AXIS2_PLACEMENT_3D('',#164821,#128808,#128809) ;
#101210=AXIS2_PLACEMENT_3D('',#164822,#128810,#128811) ;
#101211=AXIS2_PLACEMENT_3D('',#164823,#128812,#128813) ;
#101212=AXIS2_PLACEMENT_3D('',#164824,#128814,#128815) ;
#101213=AXIS2_PLACEMENT_3D('',#164825,#128816,#128817) ;
#101214=AXIS2_PLACEMENT_3D('',#164826,#128818,#128819) ;
#101215=AXIS2_PLACEMENT_3D('',#164827,#128820,#128821) ;
#101216=AXIS2_PLACEMENT_3D('',#164828,#128822,#128823) ;
#101217=AXIS2_PLACEMENT_3D('',#164829,#128824,#128825) ;
#101218=AXIS2_PLACEMENT_3D('',#164830,#128826,#128827) ;
#101219=AXIS2_PLACEMENT_3D('',#164831,#128828,#128829) ;
#101220=AXIS2_PLACEMENT_3D('',#164832,#128830,#128831) ;
#101221=AXIS2_PLACEMENT_3D('',#164833,#128832,#128833) ;
#101222=AXIS2_PLACEMENT_3D('',#164834,#128834,#128835) ;
#101223=AXIS2_PLACEMENT_3D('',#164835,#128836,#128837) ;
#101224=AXIS2_PLACEMENT_3D('',#164836,#128838,#128839) ;
#101225=AXIS2_PLACEMENT_3D('',#164837,#128840,#128841) ;
#101226=AXIS2_PLACEMENT_3D('',#164838,#128842,#128843) ;
#101227=AXIS2_PLACEMENT_3D('',#164839,#128844,#128845) ;
#101228=AXIS2_PLACEMENT_3D('',#164840,#128846,#128847) ;
#101229=AXIS2_PLACEMENT_3D('',#164841,#128848,#128849) ;
#101230=AXIS2_PLACEMENT_3D('',#164842,#128850,#128851) ;
#101231=AXIS2_PLACEMENT_3D('',#164843,#128852,#128853) ;
#101232=AXIS2_PLACEMENT_3D('',#164844,#128854,#128855) ;
#101233=AXIS2_PLACEMENT_3D('',#164845,#128856,#128857) ;
#101234=AXIS2_PLACEMENT_3D('',#164846,#128858,#128859) ;
#101235=AXIS2_PLACEMENT_3D('',#164847,#128860,#128861) ;
#101236=AXIS2_PLACEMENT_3D('',#164848,#128862,#128863) ;
#101237=AXIS2_PLACEMENT_3D('',#164849,#128864,#128865) ;
#101238=AXIS2_PLACEMENT_3D('',#164850,#128866,#128867) ;
#101239=AXIS2_PLACEMENT_3D('',#164851,#128868,#128869) ;
#101240=AXIS2_PLACEMENT_3D('',#164852,#128870,#128871) ;
#101241=AXIS2_PLACEMENT_3D('',#164853,#128872,#128873) ;
#101242=AXIS2_PLACEMENT_3D('',#164854,#128874,#128875) ;
#101243=AXIS2_PLACEMENT_3D('',#164855,#128876,#128877) ;
#101244=AXIS2_PLACEMENT_3D('',#164856,#128878,#128879) ;
#101245=AXIS2_PLACEMENT_3D('',#164857,#128880,#128881) ;
#101246=AXIS2_PLACEMENT_3D('',#164858,#128882,#128883) ;
#101247=AXIS2_PLACEMENT_3D('',#164859,#128884,#128885) ;
#101248=AXIS2_PLACEMENT_3D('',#164860,#128886,#128887) ;
#101249=AXIS2_PLACEMENT_3D('',#164861,#128888,#128889) ;
#101250=AXIS2_PLACEMENT_3D('',#164862,#128890,#128891) ;
#101251=AXIS2_PLACEMENT_3D('',#164863,#128892,#128893) ;
#101252=AXIS2_PLACEMENT_3D('',#164864,#128894,#128895) ;
#101253=AXIS2_PLACEMENT_3D('',#164865,#128896,#128897) ;
#101254=AXIS2_PLACEMENT_3D('',#164866,#128898,#128899) ;
#101255=AXIS2_PLACEMENT_3D('',#164867,#128900,#128901) ;
#101256=AXIS2_PLACEMENT_3D('',#164868,#128902,#128903) ;
#101257=AXIS2_PLACEMENT_3D('',#164869,#128904,#128905) ;
#101258=AXIS2_PLACEMENT_3D('',#164870,#128906,#128907) ;
#101259=AXIS2_PLACEMENT_3D('',#164871,#128908,#128909) ;
#101260=AXIS2_PLACEMENT_3D('',#164872,#128910,#128911) ;
#101261=AXIS2_PLACEMENT_3D('',#164873,#128912,#128913) ;
#101262=AXIS2_PLACEMENT_3D('',#164874,#128914,#128915) ;
#101263=AXIS2_PLACEMENT_3D('',#164875,#128916,#128917) ;
#101264=AXIS2_PLACEMENT_3D('',#164876,#128918,#128919) ;
#101265=AXIS2_PLACEMENT_3D('',#164877,#128920,#128921) ;
#101266=AXIS2_PLACEMENT_3D('',#164878,#128922,#128923) ;
#101267=AXIS2_PLACEMENT_3D('',#164879,#128924,#128925) ;
#101268=AXIS2_PLACEMENT_3D('',#164880,#128926,#128927) ;
#101269=AXIS2_PLACEMENT_3D('',#164881,#128928,#128929) ;
#101270=AXIS2_PLACEMENT_3D('',#164882,#128930,#128931) ;
#101271=AXIS2_PLACEMENT_3D('',#164883,#128932,#128933) ;
#101272=AXIS2_PLACEMENT_3D('',#164884,#128934,#128935) ;
#101273=AXIS2_PLACEMENT_3D('',#164885,#128936,#128937) ;
#101274=AXIS2_PLACEMENT_3D('',#164886,#128938,#128939) ;
#101275=AXIS2_PLACEMENT_3D('',#164887,#128940,#128941) ;
#101276=AXIS2_PLACEMENT_3D('',#164888,#128942,#128943) ;
#101277=AXIS2_PLACEMENT_3D('',#164889,#128944,#128945) ;
#101278=AXIS2_PLACEMENT_3D('',#164890,#128946,#128947) ;
#101279=AXIS2_PLACEMENT_3D('',#164891,#128948,#128949) ;
#101280=AXIS2_PLACEMENT_3D('',#164892,#128950,#128951) ;
#101281=AXIS2_PLACEMENT_3D('',#164893,#128952,#128953) ;
#101282=AXIS2_PLACEMENT_3D('',#164894,#128954,#128955) ;
#101283=AXIS2_PLACEMENT_3D('',#164895,#128956,#128957) ;
#101284=AXIS2_PLACEMENT_3D('',#164896,#128958,#128959) ;
#101285=AXIS2_PLACEMENT_3D('',#164897,#128960,#128961) ;
#101286=AXIS2_PLACEMENT_3D('',#164898,#128962,#128963) ;
#101287=AXIS2_PLACEMENT_3D('',#164899,#128964,#128965) ;
#101288=AXIS2_PLACEMENT_3D('',#164900,#128966,#128967) ;
#101289=AXIS2_PLACEMENT_3D('',#164901,#128968,#128969) ;
#101290=AXIS2_PLACEMENT_3D('',#164902,#128970,#128971) ;
#101291=AXIS2_PLACEMENT_3D('',#164903,#128972,#128973) ;
#101292=AXIS2_PLACEMENT_3D('',#164904,#128974,#128975) ;
#101293=AXIS2_PLACEMENT_3D('',#164905,#128976,#128977) ;
#101294=AXIS2_PLACEMENT_3D('',#164906,#128978,#128979) ;
#101295=AXIS2_PLACEMENT_3D('',#164907,#128980,#128981) ;
#101296=AXIS2_PLACEMENT_3D('',#164908,#128982,#128983) ;
#101297=AXIS2_PLACEMENT_3D('',#164909,#128984,#128985) ;
#101298=AXIS2_PLACEMENT_3D('',#164910,#128986,#128987) ;
#101299=AXIS2_PLACEMENT_3D('',#164911,#128988,#128989) ;
#101300=AXIS2_PLACEMENT_3D('',#164912,#128990,#128991) ;
#101301=AXIS2_PLACEMENT_3D('',#164913,#128992,#128993) ;
#101302=AXIS2_PLACEMENT_3D('',#164914,#128994,#128995) ;
#101303=AXIS2_PLACEMENT_3D('',#164915,#128996,#128997) ;
#101304=AXIS2_PLACEMENT_3D('',#164916,#128998,#128999) ;
#101305=AXIS2_PLACEMENT_3D('',#164917,#129000,#129001) ;
#101306=AXIS2_PLACEMENT_3D('',#164918,#129002,#129003) ;
#101307=AXIS2_PLACEMENT_3D('',#164919,#129004,#129005) ;
#101308=AXIS2_PLACEMENT_3D('',#164920,#129006,#129007) ;
#101309=AXIS2_PLACEMENT_3D('',#164921,#129008,#129009) ;
#101310=AXIS2_PLACEMENT_3D('',#164922,#129010,#129011) ;
#101311=AXIS2_PLACEMENT_3D('',#164923,#129012,#129013) ;
#101312=AXIS2_PLACEMENT_3D('',#164924,#129014,#129015) ;
#101313=AXIS2_PLACEMENT_3D('',#164925,#129016,#129017) ;
#101314=AXIS2_PLACEMENT_3D('',#164926,#129018,#129019) ;
#101315=AXIS2_PLACEMENT_3D('',#164927,#129020,#129021) ;
#101316=AXIS2_PLACEMENT_3D('',#164928,#129022,#129023) ;
#101317=AXIS2_PLACEMENT_3D('',#164929,#129024,#129025) ;
#101318=AXIS2_PLACEMENT_3D('',#164930,#129026,#129027) ;
#101319=AXIS2_PLACEMENT_3D('',#164931,#129028,#129029) ;
#101320=AXIS2_PLACEMENT_3D('',#164932,#129030,#129031) ;
#101321=AXIS2_PLACEMENT_3D('',#164933,#129032,#129033) ;
#101322=AXIS2_PLACEMENT_3D('',#164934,#129034,#129035) ;
#101323=AXIS2_PLACEMENT_3D('',#164935,#129036,#129037) ;
#101324=AXIS2_PLACEMENT_3D('',#164936,#129038,#129039) ;
#101325=AXIS2_PLACEMENT_3D('',#164937,#129040,#129041) ;
#101326=AXIS2_PLACEMENT_3D('',#164938,#129042,#129043) ;
#101327=AXIS2_PLACEMENT_3D('',#164939,#129044,#129045) ;
#101328=AXIS2_PLACEMENT_3D('',#164940,#129046,#129047) ;
#101329=AXIS2_PLACEMENT_3D('',#164941,#129048,#129049) ;
#101330=AXIS2_PLACEMENT_3D('',#164942,#129050,#129051) ;
#101331=AXIS2_PLACEMENT_3D('',#164943,#129052,#129053) ;
#101332=AXIS2_PLACEMENT_3D('',#164944,#129054,#129055) ;
#101333=AXIS2_PLACEMENT_3D('',#164945,#129056,#129057) ;
#101334=AXIS2_PLACEMENT_3D('',#164946,#129058,#129059) ;
#101335=AXIS2_PLACEMENT_3D('',#164947,#129060,#129061) ;
#101336=AXIS2_PLACEMENT_3D('',#164948,#129062,#129063) ;
#101337=AXIS2_PLACEMENT_3D('',#164949,#129064,#129065) ;
#101338=AXIS2_PLACEMENT_3D('',#164950,#129066,#129067) ;
#101339=AXIS2_PLACEMENT_3D('',#164951,#129068,#129069) ;
#101340=AXIS2_PLACEMENT_3D('',#164952,#129070,#129071) ;
#101341=AXIS2_PLACEMENT_3D('',#164953,#129072,#129073) ;
#101342=AXIS2_PLACEMENT_3D('',#164954,#129074,#129075) ;
#101343=AXIS2_PLACEMENT_3D('',#164955,#129076,#129077) ;
#101344=AXIS2_PLACEMENT_3D('',#164956,#129078,#129079) ;
#101345=AXIS2_PLACEMENT_3D('',#164957,#129080,#129081) ;
#101346=AXIS2_PLACEMENT_3D('',#164958,#129082,#129083) ;
#101347=AXIS2_PLACEMENT_3D('',#164959,#129084,#129085) ;
#101348=AXIS2_PLACEMENT_3D('',#164960,#129086,#129087) ;
#101349=AXIS2_PLACEMENT_3D('',#164961,#129088,#129089) ;
#101350=AXIS2_PLACEMENT_3D('',#164962,#129090,#129091) ;
#101351=AXIS2_PLACEMENT_3D('',#164963,#129092,#129093) ;
#101352=AXIS2_PLACEMENT_3D('',#164964,#129094,#129095) ;
#101353=AXIS2_PLACEMENT_3D('',#164965,#129096,#129097) ;
#101354=AXIS2_PLACEMENT_3D('',#164966,#129098,#129099) ;
#101355=AXIS2_PLACEMENT_3D('',#164967,#129100,#129101) ;
#101356=AXIS2_PLACEMENT_3D('',#164968,#129102,#129103) ;
#101357=AXIS2_PLACEMENT_3D('',#164969,#129104,#129105) ;
#101358=AXIS2_PLACEMENT_3D('',#164970,#129106,#129107) ;
#101359=AXIS2_PLACEMENT_3D('',#164971,#129108,#129109) ;
#101360=AXIS2_PLACEMENT_3D('',#164972,#129110,#129111) ;
#101361=AXIS2_PLACEMENT_3D('',#164973,#129112,#129113) ;
#101362=AXIS2_PLACEMENT_3D('',#164974,#129114,#129115) ;
#101363=AXIS2_PLACEMENT_3D('',#164975,#129116,#129117) ;
#101364=AXIS2_PLACEMENT_3D('',#164976,#129118,#129119) ;
#101365=AXIS2_PLACEMENT_3D('',#164977,#129120,#129121) ;
#101366=AXIS2_PLACEMENT_3D('',#164978,#129122,#129123) ;
#101367=AXIS2_PLACEMENT_3D('',#164979,#129124,#129125) ;
#101368=AXIS2_PLACEMENT_3D('',#164980,#129126,#129127) ;
#101369=AXIS2_PLACEMENT_3D('',#164981,#129128,#129129) ;
#101370=AXIS2_PLACEMENT_3D('',#164982,#129130,#129131) ;
#101371=AXIS2_PLACEMENT_3D('',#164983,#129132,#129133) ;
#101372=AXIS2_PLACEMENT_3D('',#164984,#129134,#129135) ;
#101373=AXIS2_PLACEMENT_3D('',#164985,#129136,#129137) ;
#101374=AXIS2_PLACEMENT_3D('',#164986,#129138,#129139) ;
#101375=AXIS2_PLACEMENT_3D('',#164987,#129140,#129141) ;
#101376=AXIS2_PLACEMENT_3D('',#164988,#129142,#129143) ;
#101377=AXIS2_PLACEMENT_3D('',#164989,#129144,#129145) ;
#101378=AXIS2_PLACEMENT_3D('',#164990,#129146,#129147) ;
#101379=AXIS2_PLACEMENT_3D('',#164991,#129148,#129149) ;
#101380=AXIS2_PLACEMENT_3D('',#164992,#129150,#129151) ;
#101381=AXIS2_PLACEMENT_3D('',#164993,#129152,#129153) ;
#101382=AXIS2_PLACEMENT_3D('',#164994,#129154,#129155) ;
#101383=AXIS2_PLACEMENT_3D('',#164995,#129156,#129157) ;
#101384=AXIS2_PLACEMENT_3D('',#164996,#129158,#129159) ;
#101385=AXIS2_PLACEMENT_3D('',#164997,#129160,#129161) ;
#101386=AXIS2_PLACEMENT_3D('',#164998,#129162,#129163) ;
#101387=AXIS2_PLACEMENT_3D('',#164999,#129164,#129165) ;
#101388=AXIS2_PLACEMENT_3D('',#165000,#129166,#129167) ;
#101389=AXIS2_PLACEMENT_3D('',#165001,#129168,#129169) ;
#101390=AXIS2_PLACEMENT_3D('',#165002,#129170,#129171) ;
#101391=AXIS2_PLACEMENT_3D('',#165003,#129172,#129173) ;
#101392=AXIS2_PLACEMENT_3D('',#165004,#129174,#129175) ;
#101393=AXIS2_PLACEMENT_3D('',#165005,#129176,#129177) ;
#101394=AXIS2_PLACEMENT_3D('',#165006,#129178,#129179) ;
#101395=AXIS2_PLACEMENT_3D('',#165007,#129180,#129181) ;
#101396=AXIS2_PLACEMENT_3D('',#165008,#129182,#129183) ;
#101397=AXIS2_PLACEMENT_3D('',#165009,#129184,#129185) ;
#101398=AXIS2_PLACEMENT_3D('',#165010,#129186,#129187) ;
#101399=AXIS2_PLACEMENT_3D('',#165011,#129188,#129189) ;
#101400=AXIS2_PLACEMENT_3D('',#165012,#129190,#129191) ;
#101401=AXIS2_PLACEMENT_3D('',#165013,#129192,#129193) ;
#101402=AXIS2_PLACEMENT_3D('',#165014,#129194,#129195) ;
#101403=AXIS2_PLACEMENT_3D('',#165015,#129196,#129197) ;
#101404=AXIS2_PLACEMENT_3D('',#165016,#129198,#129199) ;
#101405=AXIS2_PLACEMENT_3D('',#165017,#129200,#129201) ;
#101406=AXIS2_PLACEMENT_3D('',#165018,#129202,#129203) ;
#101407=AXIS2_PLACEMENT_3D('',#165019,#129204,#129205) ;
#101408=AXIS2_PLACEMENT_3D('',#165020,#129206,#129207) ;
#101409=AXIS2_PLACEMENT_3D('',#165021,#129208,#129209) ;
#101410=AXIS2_PLACEMENT_3D('',#165046,#129210,#129211) ;
#101411=AXIS2_PLACEMENT_3D('',#165047,#129212,#129213) ;
#101412=AXIS2_PLACEMENT_3D('',#165048,#129214,#129215) ;
#101413=AXIS2_PLACEMENT_3D('',#165073,#129216,#129217) ;
#101414=AXIS2_PLACEMENT_3D('',#165074,#129218,#129219) ;
#101415=AXIS2_PLACEMENT_3D('',#165075,#129220,#129221) ;
#101416=AXIS2_PLACEMENT_3D('',#165076,#129222,#129223) ;
#101417=AXIS2_PLACEMENT_3D('',#165101,#129224,#129225) ;
#101418=AXIS2_PLACEMENT_3D('',#165102,#129226,#129227) ;
#101419=AXIS2_PLACEMENT_3D('',#165103,#129228,#129229) ;
#101420=AXIS2_PLACEMENT_3D('',#165104,#129230,#129231) ;
#101421=AXIS2_PLACEMENT_3D('',#165105,#129232,#129233) ;
#101422=AXIS2_PLACEMENT_3D('',#165106,#129234,#129235) ;
#101423=AXIS2_PLACEMENT_3D('',#165107,#129236,#129237) ;
#101424=AXIS2_PLACEMENT_3D('',#165108,#129238,#129239) ;
#101425=AXIS2_PLACEMENT_3D('',#165109,#129240,#129241) ;
#101426=AXIS2_PLACEMENT_3D('',#165110,#129242,#129243) ;
#101427=AXIS2_PLACEMENT_3D('',#165111,#129244,#129245) ;
#101428=AXIS2_PLACEMENT_3D('',#165112,#129246,#129247) ;
#101429=AXIS2_PLACEMENT_3D('',#165113,#129248,#129249) ;
#101430=AXIS2_PLACEMENT_3D('',#165114,#129250,#129251) ;
#101431=AXIS2_PLACEMENT_3D('',#165115,#129252,#129253) ;
#101432=AXIS2_PLACEMENT_3D('',#165116,#129254,#129255) ;
#101433=AXIS2_PLACEMENT_3D('',#165117,#129256,#129257) ;
#101434=AXIS2_PLACEMENT_3D('',#165118,#129258,#129259) ;
#101435=AXIS2_PLACEMENT_3D('',#165119,#129260,#129261) ;
#101436=AXIS2_PLACEMENT_3D('',#165120,#129262,#129263) ;
#101437=AXIS2_PLACEMENT_3D('',#165121,#129264,#129265) ;
#101438=AXIS2_PLACEMENT_3D('',#165170,#129266,#129267) ;
#101439=AXIS2_PLACEMENT_3D('',#165183,#129268,#129269) ;
#101440=AXIS2_PLACEMENT_3D('',#165184,#129270,#129271) ;
#101441=AXIS2_PLACEMENT_3D('',#165185,#129272,#129273) ;
#101442=AXIS2_PLACEMENT_3D('',#165186,#129274,#129275) ;
#101443=AXIS2_PLACEMENT_3D('',#165187,#129276,#129277) ;
#101444=AXIS2_PLACEMENT_3D('',#165188,#129278,#129279) ;
#101445=AXIS2_PLACEMENT_3D('',#165189,#129280,#129281) ;
#101446=AXIS2_PLACEMENT_3D('',#165190,#129282,#129283) ;
#101447=AXIS2_PLACEMENT_3D('',#165191,#129284,#129285) ;
#101448=AXIS2_PLACEMENT_3D('',#165192,#129286,#129287) ;
#101449=AXIS2_PLACEMENT_3D('',#165193,#129288,#129289) ;
#101450=AXIS2_PLACEMENT_3D('',#165194,#129290,#129291) ;
#101451=AXIS2_PLACEMENT_3D('',#165195,#129292,#129293) ;
#101452=AXIS2_PLACEMENT_3D('',#165196,#129294,#129295) ;
#101453=AXIS2_PLACEMENT_3D('',#165197,#129296,#129297) ;
#101454=AXIS2_PLACEMENT_3D('',#165210,#129298,#129299) ;
#101455=AXIS2_PLACEMENT_3D('',#165235,#129300,#129301) ;
#101456=AXIS2_PLACEMENT_3D('',#165248,#129302,#129303) ;
#101457=AXIS2_PLACEMENT_3D('',#165249,#129304,#129305) ;
#101458=AXIS2_PLACEMENT_3D('',#165250,#129306,#129307) ;
#101459=AXIS2_PLACEMENT_3D('',#165251,#129308,#129309) ;
#101460=AXIS2_PLACEMENT_3D('',#165252,#129310,#129311) ;
#101461=AXIS2_PLACEMENT_3D('',#165253,#129312,#129313) ;
#101462=AXIS2_PLACEMENT_3D('',#165254,#129314,#129315) ;
#101463=AXIS2_PLACEMENT_3D('',#165255,#129316,#129317) ;
#101464=AXIS2_PLACEMENT_3D('',#165256,#129318,#129319) ;
#101465=AXIS2_PLACEMENT_3D('',#165257,#129320,#129321) ;
#101466=AXIS2_PLACEMENT_3D('',#165258,#129322,#129323) ;
#101467=AXIS2_PLACEMENT_3D('',#165259,#129324,#129325) ;
#101468=AXIS2_PLACEMENT_3D('',#165260,#129326,#129327) ;
#101469=AXIS2_PLACEMENT_3D('',#165261,#129328,#129329) ;
#101470=AXIS2_PLACEMENT_3D('',#165262,#129330,#129331) ;
#101471=AXIS2_PLACEMENT_3D('',#165275,#129332,#129333) ;
#101472=AXIS2_PLACEMENT_3D('',#165300,#129334,#129335) ;
#101473=AXIS2_PLACEMENT_3D('',#165301,#129336,#129337) ;
#101474=AXIS2_PLACEMENT_3D('',#165302,#129338,#129339) ;
#101475=AXIS2_PLACEMENT_3D('',#165303,#129340,#129341) ;
#101476=AXIS2_PLACEMENT_3D('',#165304,#129342,#129343) ;
#101477=AXIS2_PLACEMENT_3D('',#165305,#129344,#129345) ;
#101478=AXIS2_PLACEMENT_3D('',#165306,#129346,#129347) ;
#101479=AXIS2_PLACEMENT_3D('',#165307,#129348,#129349) ;
#101480=AXIS2_PLACEMENT_3D('',#165308,#129350,#129351) ;
#101481=AXIS2_PLACEMENT_3D('',#165309,#129352,#129353) ;
#101482=AXIS2_PLACEMENT_3D('',#165310,#129354,#129355) ;
#101483=AXIS2_PLACEMENT_3D('',#165311,#129356,#129357) ;
#101484=AXIS2_PLACEMENT_3D('',#165312,#129358,#129359) ;
#101485=AXIS2_PLACEMENT_3D('',#165313,#129360,#129361) ;
#101486=AXIS2_PLACEMENT_3D('',#165314,#129362,#129363) ;
#101487=AXIS2_PLACEMENT_3D('',#165315,#129364,#129365) ;
#101488=AXIS2_PLACEMENT_3D('',#165316,#129366,#129367) ;
#101489=AXIS2_PLACEMENT_3D('',#165317,#129368,#129369) ;
#101490=AXIS2_PLACEMENT_3D('',#165318,#129370,#129371) ;
#101491=AXIS2_PLACEMENT_3D('',#165319,#129372,#129373) ;
#101492=AXIS2_PLACEMENT_3D('',#165320,#129374,#129375) ;
#101493=AXIS2_PLACEMENT_3D('',#165321,#129376,#129377) ;
#101494=AXIS2_PLACEMENT_3D('',#165322,#129378,#129379) ;
#101495=AXIS2_PLACEMENT_3D('',#165323,#129380,#129381) ;
#101496=AXIS2_PLACEMENT_3D('',#165324,#129382,#129383) ;
#101497=AXIS2_PLACEMENT_3D('',#165325,#129384,#129385) ;
#101498=AXIS2_PLACEMENT_3D('',#165326,#129386,#129387) ;
#101499=AXIS2_PLACEMENT_3D('',#165327,#129388,#129389) ;
#101500=AXIS2_PLACEMENT_3D('',#165328,#129390,#129391) ;
#101501=AXIS2_PLACEMENT_3D('',#165329,#129392,#129393) ;
#101502=AXIS2_PLACEMENT_3D('',#165330,#129394,#129395) ;
#101503=AXIS2_PLACEMENT_3D('',#165331,#129396,#129397) ;
#101504=AXIS2_PLACEMENT_3D('',#165332,#129398,#129399) ;
#101505=AXIS2_PLACEMENT_3D('',#165333,#129400,#129401) ;
#101506=AXIS2_PLACEMENT_3D('',#165334,#129402,#129403) ;
#101507=AXIS2_PLACEMENT_3D('',#165335,#129404,#129405) ;
#101508=AXIS2_PLACEMENT_3D('',#165336,#129406,#129407) ;
#101509=AXIS2_PLACEMENT_3D('',#165337,#129408,#129409) ;
#101510=AXIS2_PLACEMENT_3D('',#165338,#129410,#129411) ;
#101511=AXIS2_PLACEMENT_3D('',#165339,#129412,#129413) ;
#101512=AXIS2_PLACEMENT_3D('',#165340,#129414,#129415) ;
#101513=AXIS2_PLACEMENT_3D('',#165341,#129416,#129417) ;
#101514=AXIS2_PLACEMENT_3D('',#165342,#129418,#129419) ;
#101515=AXIS2_PLACEMENT_3D('',#165343,#129420,#129421) ;
#101516=AXIS2_PLACEMENT_3D('',#165344,#129422,#129423) ;
#101517=AXIS2_PLACEMENT_3D('',#165345,#129424,#129425) ;
#101518=AXIS2_PLACEMENT_3D('',#165346,#129426,#129427) ;
#101519=AXIS2_PLACEMENT_3D('',#165347,#129428,#129429) ;
#101520=AXIS2_PLACEMENT_3D('',#165348,#129430,#129431) ;
#101521=AXIS2_PLACEMENT_3D('',#165349,#129432,#129433) ;
#101522=AXIS2_PLACEMENT_3D('',#165350,#129434,#129435) ;
#101523=AXIS2_PLACEMENT_3D('',#165351,#129436,#129437) ;
#101524=AXIS2_PLACEMENT_3D('',#165352,#129438,#129439) ;
#101525=AXIS2_PLACEMENT_3D('',#165353,#129440,#129441) ;
#101526=AXIS2_PLACEMENT_3D('',#165354,#129442,#129443) ;
#101527=AXIS2_PLACEMENT_3D('',#165355,#129444,#129445) ;
#101528=AXIS2_PLACEMENT_3D('',#165356,#129446,#129447) ;
#101529=AXIS2_PLACEMENT_3D('',#165357,#129448,#129449) ;
#101530=AXIS2_PLACEMENT_3D('',#165358,#129450,#129451) ;
#101531=AXIS2_PLACEMENT_3D('',#165359,#129452,#129453) ;
#101532=AXIS2_PLACEMENT_3D('',#165360,#129454,#129455) ;
#101533=AXIS2_PLACEMENT_3D('',#165361,#129456,#129457) ;
#101534=AXIS2_PLACEMENT_3D('',#165362,#129458,#129459) ;
#101535=AXIS2_PLACEMENT_3D('',#165363,#129460,#129461) ;
#101536=AXIS2_PLACEMENT_3D('',#165364,#129462,#129463) ;
#101537=AXIS2_PLACEMENT_3D('',#165365,#129464,#129465) ;
#101538=AXIS2_PLACEMENT_3D('',#165366,#129466,#129467) ;
#101539=AXIS2_PLACEMENT_3D('',#165367,#129468,#129469) ;
#101540=AXIS2_PLACEMENT_3D('',#165368,#129470,#129471) ;
#101541=AXIS2_PLACEMENT_3D('',#165369,#129472,#129473) ;
#101542=AXIS2_PLACEMENT_3D('',#165370,#129474,#129475) ;
#101543=AXIS2_PLACEMENT_3D('',#165371,#129476,#129477) ;
#101544=AXIS2_PLACEMENT_3D('',#165372,#129478,#129479) ;
#101545=AXIS2_PLACEMENT_3D('',#165373,#129480,#129481) ;
#101546=AXIS2_PLACEMENT_3D('',#165374,#129482,#129483) ;
#101547=AXIS2_PLACEMENT_3D('',#165375,#129484,#129485) ;
#101548=AXIS2_PLACEMENT_3D('',#165376,#129486,#129487) ;
#101549=AXIS2_PLACEMENT_3D('',#165377,#129488,#129489) ;
#101550=AXIS2_PLACEMENT_3D('',#165378,#129490,#129491) ;
#101551=AXIS2_PLACEMENT_3D('',#165379,#129492,#129493) ;
#101552=AXIS2_PLACEMENT_3D('',#165380,#129494,#129495) ;
#101553=AXIS2_PLACEMENT_3D('',#165381,#129496,#129497) ;
#101554=AXIS2_PLACEMENT_3D('',#165382,#129498,#129499) ;
#101555=AXIS2_PLACEMENT_3D('',#165383,#129500,#129501) ;
#101556=AXIS2_PLACEMENT_3D('',#165384,#129502,#129503) ;
#101557=AXIS2_PLACEMENT_3D('',#165385,#129504,#129505) ;
#101558=AXIS2_PLACEMENT_3D('',#165386,#129506,#129507) ;
#101559=AXIS2_PLACEMENT_3D('',#165387,#129508,#129509) ;
#101560=AXIS2_PLACEMENT_3D('',#165388,#129510,#129511) ;
#101561=AXIS2_PLACEMENT_3D('',#165389,#129512,#129513) ;
#101562=AXIS2_PLACEMENT_3D('',#165390,#129514,#129515) ;
#101563=AXIS2_PLACEMENT_3D('',#165391,#129516,#129517) ;
#101564=AXIS2_PLACEMENT_3D('',#165392,#129518,#129519) ;
#101565=AXIS2_PLACEMENT_3D('',#165393,#129520,#129521) ;
#101566=AXIS2_PLACEMENT_3D('',#165394,#129522,#129523) ;
#101567=AXIS2_PLACEMENT_3D('',#165395,#129524,#129525) ;
#101568=AXIS2_PLACEMENT_3D('',#165396,#129526,#129527) ;
#101569=AXIS2_PLACEMENT_3D('',#165397,#129528,#129529) ;
#101570=AXIS2_PLACEMENT_3D('',#165398,#129530,#129531) ;
#101571=AXIS2_PLACEMENT_3D('',#165399,#129532,#129533) ;
#101572=AXIS2_PLACEMENT_3D('',#165400,#129534,#129535) ;
#101573=AXIS2_PLACEMENT_3D('',#165401,#129536,#129537) ;
#101574=AXIS2_PLACEMENT_3D('',#165402,#129538,#129539) ;
#101575=AXIS2_PLACEMENT_3D('',#165403,#129540,#129541) ;
#101576=AXIS2_PLACEMENT_3D('',#165404,#129542,#129543) ;
#101577=AXIS2_PLACEMENT_3D('',#165405,#129544,#129545) ;
#101578=AXIS2_PLACEMENT_3D('',#165406,#129546,#129547) ;
#101579=AXIS2_PLACEMENT_3D('',#165407,#129548,#129549) ;
#101580=AXIS2_PLACEMENT_3D('',#165408,#129550,#129551) ;
#101581=AXIS2_PLACEMENT_3D('',#165409,#129552,#129553) ;
#101582=AXIS2_PLACEMENT_3D('',#165410,#129554,#129555) ;
#101583=AXIS2_PLACEMENT_3D('',#165411,#129556,#129557) ;
#101584=AXIS2_PLACEMENT_3D('',#165412,#129558,#129559) ;
#101585=AXIS2_PLACEMENT_3D('',#165413,#129560,#129561) ;
#101586=AXIS2_PLACEMENT_3D('',#165414,#129562,#129563) ;
#101587=AXIS2_PLACEMENT_3D('',#165415,#129564,#129565) ;
#101588=AXIS2_PLACEMENT_3D('',#165416,#129566,#129567) ;
#101589=AXIS2_PLACEMENT_3D('',#165417,#129568,#129569) ;
#101590=AXIS2_PLACEMENT_3D('',#165418,#129570,#129571) ;
#101591=AXIS2_PLACEMENT_3D('',#165419,#129572,#129573) ;
#101592=AXIS2_PLACEMENT_3D('',#165420,#129574,#129575) ;
#101593=AXIS2_PLACEMENT_3D('',#165421,#129576,#129577) ;
#101594=AXIS2_PLACEMENT_3D('',#165422,#129578,#129579) ;
#101595=AXIS2_PLACEMENT_3D('',#165423,#129580,#129581) ;
#101596=AXIS2_PLACEMENT_3D('',#165424,#129582,#129583) ;
#101597=AXIS2_PLACEMENT_3D('',#165425,#129584,#129585) ;
#101598=AXIS2_PLACEMENT_3D('',#165426,#129586,#129587) ;
#101599=AXIS2_PLACEMENT_3D('',#165427,#129588,#129589) ;
#101600=AXIS2_PLACEMENT_3D('',#165428,#129590,#129591) ;
#101601=AXIS2_PLACEMENT_3D('',#165429,#129592,#129593) ;
#101602=AXIS2_PLACEMENT_3D('',#165430,#129594,#129595) ;
#101603=AXIS2_PLACEMENT_3D('',#165431,#129596,#129597) ;
#101604=AXIS2_PLACEMENT_3D('',#165432,#129598,#129599) ;
#101605=AXIS2_PLACEMENT_3D('',#165433,#129600,#129601) ;
#101606=AXIS2_PLACEMENT_3D('',#165434,#129602,#129603) ;
#101607=AXIS2_PLACEMENT_3D('',#165435,#129604,#129605) ;
#101608=AXIS2_PLACEMENT_3D('',#165436,#129606,#129607) ;
#101609=AXIS2_PLACEMENT_3D('',#165437,#129608,#129609) ;
#101610=AXIS2_PLACEMENT_3D('',#165438,#129610,#129611) ;
#101611=AXIS2_PLACEMENT_3D('',#165439,#129612,#129613) ;
#101612=AXIS2_PLACEMENT_3D('',#165440,#129614,#129615) ;
#101613=AXIS2_PLACEMENT_3D('',#165441,#129616,#129617) ;
#101614=AXIS2_PLACEMENT_3D('',#165442,#129618,#129619) ;
#101615=AXIS2_PLACEMENT_3D('',#165443,#129620,#129621) ;
#101616=AXIS2_PLACEMENT_3D('',#165444,#129622,#129623) ;
#101617=AXIS2_PLACEMENT_3D('',#165445,#129624,#129625) ;
#101618=AXIS2_PLACEMENT_3D('',#165446,#129626,#129627) ;
#101619=AXIS2_PLACEMENT_3D('',#165447,#129628,#129629) ;
#101620=AXIS2_PLACEMENT_3D('',#165448,#129630,#129631) ;
#101621=AXIS2_PLACEMENT_3D('',#165449,#129632,#129633) ;
#101622=AXIS2_PLACEMENT_3D('',#165450,#129634,#129635) ;
#101623=AXIS2_PLACEMENT_3D('',#165451,#129636,#129637) ;
#101624=AXIS2_PLACEMENT_3D('',#165452,#129638,#129639) ;
#101625=AXIS2_PLACEMENT_3D('',#165453,#129640,#129641) ;
#101626=AXIS2_PLACEMENT_3D('',#165454,#129642,#129643) ;
#101627=AXIS2_PLACEMENT_3D('',#165455,#129644,#129645) ;
#101628=AXIS2_PLACEMENT_3D('',#165456,#129646,#129647) ;
#101629=AXIS2_PLACEMENT_3D('',#165457,#129648,#129649) ;
#101630=AXIS2_PLACEMENT_3D('',#165458,#129650,#129651) ;
#101631=AXIS2_PLACEMENT_3D('',#165459,#129652,#129653) ;
#101632=AXIS2_PLACEMENT_3D('',#165460,#129654,#129655) ;
#101633=AXIS2_PLACEMENT_3D('',#165461,#129656,#129657) ;
#101634=AXIS2_PLACEMENT_3D('',#165462,#129658,#129659) ;
#101635=AXIS2_PLACEMENT_3D('',#165463,#129660,#129661) ;
#101636=AXIS2_PLACEMENT_3D('',#165464,#129662,#129663) ;
#101637=AXIS2_PLACEMENT_3D('',#165465,#129664,#129665) ;
#101638=AXIS2_PLACEMENT_3D('',#165466,#129666,#129667) ;
#101639=AXIS2_PLACEMENT_3D('',#165467,#129668,#129669) ;
#101640=AXIS2_PLACEMENT_3D('',#165468,#129670,#129671) ;
#101641=AXIS2_PLACEMENT_3D('',#165469,#129672,#129673) ;
#101642=AXIS2_PLACEMENT_3D('',#165470,#129674,#129675) ;
#101643=AXIS2_PLACEMENT_3D('',#165471,#129676,#129677) ;
#101644=AXIS2_PLACEMENT_3D('',#165472,#129678,#129679) ;
#101645=AXIS2_PLACEMENT_3D('',#165473,#129680,#129681) ;
#101646=AXIS2_PLACEMENT_3D('',#165474,#129682,#129683) ;
#101647=AXIS2_PLACEMENT_3D('',#165475,#129684,#129685) ;
#101648=AXIS2_PLACEMENT_3D('',#165476,#129686,#129687) ;
#101649=AXIS2_PLACEMENT_3D('',#165477,#129688,#129689) ;
#101650=AXIS2_PLACEMENT_3D('',#165478,#129690,#129691) ;
#101651=AXIS2_PLACEMENT_3D('',#165479,#129692,#129693) ;
#101652=AXIS2_PLACEMENT_3D('',#165480,#129694,#129695) ;
#101653=AXIS2_PLACEMENT_3D('',#165481,#129696,#129697) ;
#101654=AXIS2_PLACEMENT_3D('',#165482,#129698,#129699) ;
#101655=AXIS2_PLACEMENT_3D('',#165483,#129700,#129701) ;
#101656=AXIS2_PLACEMENT_3D('',#165484,#129702,#129703) ;
#101657=AXIS2_PLACEMENT_3D('',#165485,#129704,#129705) ;
#101658=AXIS2_PLACEMENT_3D('',#165486,#129706,#129707) ;
#101659=AXIS2_PLACEMENT_3D('',#165487,#129708,#129709) ;
#101660=AXIS2_PLACEMENT_3D('',#165488,#129710,#129711) ;
#101661=AXIS2_PLACEMENT_3D('',#165489,#129712,#129713) ;
#101662=AXIS2_PLACEMENT_3D('',#165490,#129714,#129715) ;
#101663=AXIS2_PLACEMENT_3D('',#165491,#129716,#129717) ;
#101664=AXIS2_PLACEMENT_3D('',#165492,#129718,#129719) ;
#101665=AXIS2_PLACEMENT_3D('',#165493,#129720,#129721) ;
#101666=AXIS2_PLACEMENT_3D('',#165494,#129722,#129723) ;
#101667=AXIS2_PLACEMENT_3D('',#165495,#129724,#129725) ;
#101668=AXIS2_PLACEMENT_3D('',#165496,#129726,#129727) ;
#101669=AXIS2_PLACEMENT_3D('',#165497,#129728,#129729) ;
#101670=AXIS2_PLACEMENT_3D('',#165498,#129730,#129731) ;
#101671=AXIS2_PLACEMENT_3D('',#165499,#129732,#129733) ;
#101672=AXIS2_PLACEMENT_3D('',#165500,#129734,#129735) ;
#101673=AXIS2_PLACEMENT_3D('',#165501,#129736,#129737) ;
#101674=AXIS2_PLACEMENT_3D('',#165502,#129738,#129739) ;
#101675=AXIS2_PLACEMENT_3D('',#165503,#129740,#129741) ;
#101676=AXIS2_PLACEMENT_3D('',#165504,#129742,#129743) ;
#101677=AXIS2_PLACEMENT_3D('',#165505,#129744,#129745) ;
#101678=AXIS2_PLACEMENT_3D('',#165506,#129746,#129747) ;
#101679=AXIS2_PLACEMENT_3D('',#165507,#129748,#129749) ;
#101680=AXIS2_PLACEMENT_3D('',#165508,#129750,#129751) ;
#101681=AXIS2_PLACEMENT_3D('',#165509,#129752,#129753) ;
#101682=AXIS2_PLACEMENT_3D('',#165510,#129754,#129755) ;
#101683=AXIS2_PLACEMENT_3D('',#165511,#129756,#129757) ;
#101684=AXIS2_PLACEMENT_3D('',#165512,#129758,#129759) ;
#101685=AXIS2_PLACEMENT_3D('',#165513,#129760,#129761) ;
#101686=AXIS2_PLACEMENT_3D('',#165538,#129762,#129763) ;
#101687=AXIS2_PLACEMENT_3D('',#165539,#129764,#129765) ;
#101688=AXIS2_PLACEMENT_3D('',#165540,#129766,#129767) ;
#101689=AXIS2_PLACEMENT_3D('',#165565,#129768,#129769) ;
#101690=AXIS2_PLACEMENT_3D('',#165566,#129770,#129771) ;
#101691=AXIS2_PLACEMENT_3D('',#165567,#129772,#129773) ;
#101692=AXIS2_PLACEMENT_3D('',#165568,#129774,#129775) ;
#101693=AXIS2_PLACEMENT_3D('',#165593,#129776,#129777) ;
#101694=AXIS2_PLACEMENT_3D('',#165594,#129778,#129779) ;
#101695=AXIS2_PLACEMENT_3D('',#165595,#129780,#129781) ;
#101696=AXIS2_PLACEMENT_3D('',#165596,#129782,#129783) ;
#101697=AXIS2_PLACEMENT_3D('',#165597,#129784,#129785) ;
#101698=AXIS2_PLACEMENT_3D('',#165598,#129786,#129787) ;
#101699=AXIS2_PLACEMENT_3D('',#165599,#129788,#129789) ;
#101700=AXIS2_PLACEMENT_3D('',#165600,#129790,#129791) ;
#101701=AXIS2_PLACEMENT_3D('',#165601,#129792,#129793) ;
#101702=AXIS2_PLACEMENT_3D('',#165602,#129794,#129795) ;
#101703=AXIS2_PLACEMENT_3D('',#165603,#129796,#129797) ;
#101704=AXIS2_PLACEMENT_3D('',#165604,#129798,#129799) ;
#101705=AXIS2_PLACEMENT_3D('',#165605,#129800,#129801) ;
#101706=AXIS2_PLACEMENT_3D('',#165606,#129802,#129803) ;
#101707=AXIS2_PLACEMENT_3D('',#165607,#129804,#129805) ;
#101708=AXIS2_PLACEMENT_3D('',#165608,#129806,#129807) ;
#101709=AXIS2_PLACEMENT_3D('',#165609,#129808,#129809) ;
#101710=AXIS2_PLACEMENT_3D('',#165610,#129810,#129811) ;
#101711=AXIS2_PLACEMENT_3D('',#165611,#129812,#129813) ;
#101712=AXIS2_PLACEMENT_3D('',#165612,#129814,#129815) ;
#101713=AXIS2_PLACEMENT_3D('',#165613,#129816,#129817) ;
#101714=AXIS2_PLACEMENT_3D('',#165662,#129818,#129819) ;
#101715=AXIS2_PLACEMENT_3D('',#165675,#129820,#129821) ;
#101716=AXIS2_PLACEMENT_3D('',#165676,#129822,#129823) ;
#101717=AXIS2_PLACEMENT_3D('',#165677,#129824,#129825) ;
#101718=AXIS2_PLACEMENT_3D('',#165678,#129826,#129827) ;
#101719=AXIS2_PLACEMENT_3D('',#165679,#129828,#129829) ;
#101720=AXIS2_PLACEMENT_3D('',#165680,#129830,#129831) ;
#101721=AXIS2_PLACEMENT_3D('',#165681,#129832,#129833) ;
#101722=AXIS2_PLACEMENT_3D('',#165682,#129834,#129835) ;
#101723=AXIS2_PLACEMENT_3D('',#165683,#129836,#129837) ;
#101724=AXIS2_PLACEMENT_3D('',#165684,#129838,#129839) ;
#101725=AXIS2_PLACEMENT_3D('',#165685,#129840,#129841) ;
#101726=AXIS2_PLACEMENT_3D('',#165686,#129842,#129843) ;
#101727=AXIS2_PLACEMENT_3D('',#165687,#129844,#129845) ;
#101728=AXIS2_PLACEMENT_3D('',#165688,#129846,#129847) ;
#101729=AXIS2_PLACEMENT_3D('',#165689,#129848,#129849) ;
#101730=AXIS2_PLACEMENT_3D('',#165702,#129850,#129851) ;
#101731=AXIS2_PLACEMENT_3D('',#165727,#129852,#129853) ;
#101732=AXIS2_PLACEMENT_3D('',#165740,#129854,#129855) ;
#101733=AXIS2_PLACEMENT_3D('',#165741,#129856,#129857) ;
#101734=AXIS2_PLACEMENT_3D('',#165742,#129858,#129859) ;
#101735=AXIS2_PLACEMENT_3D('',#165743,#129860,#129861) ;
#101736=AXIS2_PLACEMENT_3D('',#165744,#129862,#129863) ;
#101737=AXIS2_PLACEMENT_3D('',#165745,#129864,#129865) ;
#101738=AXIS2_PLACEMENT_3D('',#165746,#129866,#129867) ;
#101739=AXIS2_PLACEMENT_3D('',#165747,#129868,#129869) ;
#101740=AXIS2_PLACEMENT_3D('',#165748,#129870,#129871) ;
#101741=AXIS2_PLACEMENT_3D('',#165749,#129872,#129873) ;
#101742=AXIS2_PLACEMENT_3D('',#165750,#129874,#129875) ;
#101743=AXIS2_PLACEMENT_3D('',#165751,#129876,#129877) ;
#101744=AXIS2_PLACEMENT_3D('',#165752,#129878,#129879) ;
#101745=AXIS2_PLACEMENT_3D('',#165753,#129880,#129881) ;
#101746=AXIS2_PLACEMENT_3D('',#165754,#129882,#129883) ;
#101747=AXIS2_PLACEMENT_3D('',#165767,#129884,#129885) ;
#101748=AXIS2_PLACEMENT_3D('',#165792,#129886,#129887) ;
#101749=AXIS2_PLACEMENT_3D('',#165793,#129888,#129889) ;
#101750=AXIS2_PLACEMENT_3D('',#165794,#129890,#129891) ;
#101751=AXIS2_PLACEMENT_3D('',#165795,#129892,#129893) ;
#101752=AXIS2_PLACEMENT_3D('',#165796,#129894,#129895) ;
#101753=AXIS2_PLACEMENT_3D('',#165797,#129896,#129897) ;
#101754=AXIS2_PLACEMENT_3D('',#165798,#129898,#129899) ;
#101755=AXIS2_PLACEMENT_3D('',#165799,#129900,#129901) ;
#101756=AXIS2_PLACEMENT_3D('',#165800,#129902,#129903) ;
#101757=AXIS2_PLACEMENT_3D('',#165801,#129904,#129905) ;
#101758=AXIS2_PLACEMENT_3D('',#165802,#129906,#129907) ;
#101759=AXIS2_PLACEMENT_3D('',#165803,#129908,#129909) ;
#101760=AXIS2_PLACEMENT_3D('',#165804,#129910,#129911) ;
#101761=AXIS2_PLACEMENT_3D('',#165805,#129912,#129913) ;
#101762=AXIS2_PLACEMENT_3D('',#165806,#129914,#129915) ;
#101763=AXIS2_PLACEMENT_3D('',#165807,#129916,#129917) ;
#101764=AXIS2_PLACEMENT_3D('',#165808,#129918,#129919) ;
#101765=AXIS2_PLACEMENT_3D('',#165809,#129920,#129921) ;
#101766=AXIS2_PLACEMENT_3D('',#165810,#129922,#129923) ;
#101767=AXIS2_PLACEMENT_3D('',#165811,#129924,#129925) ;
#101768=AXIS2_PLACEMENT_3D('',#165812,#129926,#129927) ;
#101769=AXIS2_PLACEMENT_3D('',#165813,#129928,#129929) ;
#101770=AXIS2_PLACEMENT_3D('',#165814,#129930,#129931) ;
#101771=AXIS2_PLACEMENT_3D('',#165815,#129932,#129933) ;
#101772=AXIS2_PLACEMENT_3D('',#165816,#129934,#129935) ;
#101773=AXIS2_PLACEMENT_3D('',#165817,#129936,#129937) ;
#101774=AXIS2_PLACEMENT_3D('',#165818,#129938,#129939) ;
#101775=AXIS2_PLACEMENT_3D('',#165819,#129940,#129941) ;
#101776=AXIS2_PLACEMENT_3D('',#165820,#129942,#129943) ;
#101777=AXIS2_PLACEMENT_3D('',#165821,#129944,#129945) ;
#101778=AXIS2_PLACEMENT_3D('',#165822,#129946,#129947) ;
#101779=AXIS2_PLACEMENT_3D('',#165823,#129948,#129949) ;
#101780=AXIS2_PLACEMENT_3D('',#165824,#129950,#129951) ;
#101781=AXIS2_PLACEMENT_3D('',#165825,#129952,#129953) ;
#101782=AXIS2_PLACEMENT_3D('',#165826,#129954,#129955) ;
#101783=AXIS2_PLACEMENT_3D('',#165827,#129956,#129957) ;
#101784=AXIS2_PLACEMENT_3D('',#165828,#129958,#129959) ;
#101785=AXIS2_PLACEMENT_3D('',#165829,#129960,#129961) ;
#101786=AXIS2_PLACEMENT_3D('',#165830,#129962,#129963) ;
#101787=AXIS2_PLACEMENT_3D('',#165831,#129964,#129965) ;
#101788=AXIS2_PLACEMENT_3D('',#165832,#129966,#129967) ;
#101789=AXIS2_PLACEMENT_3D('',#165833,#129968,#129969) ;
#101790=AXIS2_PLACEMENT_3D('',#165834,#129970,#129971) ;
#101791=AXIS2_PLACEMENT_3D('',#165835,#129972,#129973) ;
#101792=AXIS2_PLACEMENT_3D('',#165836,#129974,#129975) ;
#101793=AXIS2_PLACEMENT_3D('',#165837,#129976,#129977) ;
#101794=AXIS2_PLACEMENT_3D('',#165838,#129978,#129979) ;
#101795=AXIS2_PLACEMENT_3D('',#165839,#129980,#129981) ;
#101796=AXIS2_PLACEMENT_3D('',#165840,#129982,#129983) ;
#101797=AXIS2_PLACEMENT_3D('',#165841,#129984,#129985) ;
#101798=AXIS2_PLACEMENT_3D('',#165842,#129986,#129987) ;
#101799=AXIS2_PLACEMENT_3D('',#165843,#129988,#129989) ;
#101800=AXIS2_PLACEMENT_3D('',#165844,#129990,#129991) ;
#101801=AXIS2_PLACEMENT_3D('',#165845,#129992,#129993) ;
#101802=AXIS2_PLACEMENT_3D('',#165846,#129994,#129995) ;
#101803=AXIS2_PLACEMENT_3D('',#165847,#129996,#129997) ;
#101804=AXIS2_PLACEMENT_3D('',#165848,#129998,#129999) ;
#101805=AXIS2_PLACEMENT_3D('',#165849,#130000,#130001) ;
#101806=AXIS2_PLACEMENT_3D('',#165850,#130002,#130003) ;
#101807=AXIS2_PLACEMENT_3D('',#165851,#130004,#130005) ;
#101808=AXIS2_PLACEMENT_3D('',#165852,#130006,#130007) ;
#101809=AXIS2_PLACEMENT_3D('',#165853,#130008,#130009) ;
#101810=AXIS2_PLACEMENT_3D('',#165854,#130010,#130011) ;
#101811=AXIS2_PLACEMENT_3D('',#165855,#130012,#130013) ;
#101812=AXIS2_PLACEMENT_3D('',#165856,#130014,#130015) ;
#101813=AXIS2_PLACEMENT_3D('',#165857,#130016,#130017) ;
#101814=AXIS2_PLACEMENT_3D('',#165858,#130018,#130019) ;
#101815=AXIS2_PLACEMENT_3D('',#165859,#130020,#130021) ;
#101816=AXIS2_PLACEMENT_3D('',#165860,#130022,#130023) ;
#101817=AXIS2_PLACEMENT_3D('',#165861,#130024,#130025) ;
#101818=AXIS2_PLACEMENT_3D('',#165862,#130026,#130027) ;
#101819=AXIS2_PLACEMENT_3D('',#165863,#130028,#130029) ;
#101820=AXIS2_PLACEMENT_3D('',#165864,#130030,#130031) ;
#101821=AXIS2_PLACEMENT_3D('',#165865,#130032,#130033) ;
#101822=AXIS2_PLACEMENT_3D('',#165866,#130034,#130035) ;
#101823=AXIS2_PLACEMENT_3D('',#165867,#130036,#130037) ;
#101824=AXIS2_PLACEMENT_3D('',#165868,#130038,#130039) ;
#101825=AXIS2_PLACEMENT_3D('',#165869,#130040,#130041) ;
#101826=AXIS2_PLACEMENT_3D('',#165870,#130042,#130043) ;
#101827=AXIS2_PLACEMENT_3D('',#165871,#130044,#130045) ;
#101828=AXIS2_PLACEMENT_3D('',#165872,#130046,#130047) ;
#101829=AXIS2_PLACEMENT_3D('',#165873,#130048,#130049) ;
#101830=AXIS2_PLACEMENT_3D('',#165874,#130050,#130051) ;
#101831=AXIS2_PLACEMENT_3D('',#165875,#130052,#130053) ;
#101832=AXIS2_PLACEMENT_3D('',#165876,#130054,#130055) ;
#101833=AXIS2_PLACEMENT_3D('',#165877,#130056,#130057) ;
#101834=AXIS2_PLACEMENT_3D('',#165878,#130058,#130059) ;
#101835=AXIS2_PLACEMENT_3D('',#165879,#130060,#130061) ;
#101836=AXIS2_PLACEMENT_3D('',#165880,#130062,#130063) ;
#101837=AXIS2_PLACEMENT_3D('',#165881,#130064,#130065) ;
#101838=AXIS2_PLACEMENT_3D('',#165882,#130066,#130067) ;
#101839=AXIS2_PLACEMENT_3D('',#165883,#130068,#130069) ;
#101840=AXIS2_PLACEMENT_3D('',#165884,#130070,#130071) ;
#101841=AXIS2_PLACEMENT_3D('',#165885,#130072,#130073) ;
#101842=AXIS2_PLACEMENT_3D('',#165886,#130074,#130075) ;
#101843=AXIS2_PLACEMENT_3D('',#165887,#130076,#130077) ;
#101844=AXIS2_PLACEMENT_3D('',#165888,#130078,#130079) ;
#101845=AXIS2_PLACEMENT_3D('',#165889,#130080,#130081) ;
#101846=AXIS2_PLACEMENT_3D('',#165890,#130082,#130083) ;
#101847=AXIS2_PLACEMENT_3D('',#165891,#130084,#130085) ;
#101848=AXIS2_PLACEMENT_3D('',#165892,#130086,#130087) ;
#101849=AXIS2_PLACEMENT_3D('',#165893,#130088,#130089) ;
#101850=AXIS2_PLACEMENT_3D('',#165894,#130090,#130091) ;
#101851=AXIS2_PLACEMENT_3D('',#165895,#130092,#130093) ;
#101852=AXIS2_PLACEMENT_3D('',#165896,#130094,#130095) ;
#101853=AXIS2_PLACEMENT_3D('',#165897,#130096,#130097) ;
#101854=AXIS2_PLACEMENT_3D('',#165898,#130098,#130099) ;
#101855=AXIS2_PLACEMENT_3D('',#165899,#130100,#130101) ;
#101856=AXIS2_PLACEMENT_3D('',#165900,#130102,#130103) ;
#101857=AXIS2_PLACEMENT_3D('',#165901,#130104,#130105) ;
#101858=AXIS2_PLACEMENT_3D('',#165902,#130106,#130107) ;
#101859=AXIS2_PLACEMENT_3D('',#165903,#130108,#130109) ;
#101860=AXIS2_PLACEMENT_3D('',#165904,#130110,#130111) ;
#101861=AXIS2_PLACEMENT_3D('',#165905,#130112,#130113) ;
#101862=AXIS2_PLACEMENT_3D('',#165906,#130114,#130115) ;
#101863=AXIS2_PLACEMENT_3D('',#165907,#130116,#130117) ;
#101864=AXIS2_PLACEMENT_3D('',#165908,#130118,#130119) ;
#101865=AXIS2_PLACEMENT_3D('',#165909,#130120,#130121) ;
#101866=AXIS2_PLACEMENT_3D('',#165910,#130122,#130123) ;
#101867=AXIS2_PLACEMENT_3D('',#165911,#130124,#130125) ;
#101868=AXIS2_PLACEMENT_3D('',#165912,#130126,#130127) ;
#101869=AXIS2_PLACEMENT_3D('',#165913,#130128,#130129) ;
#101870=AXIS2_PLACEMENT_3D('',#165914,#130130,#130131) ;
#101871=AXIS2_PLACEMENT_3D('',#165915,#130132,#130133) ;
#101872=AXIS2_PLACEMENT_3D('',#165916,#130134,#130135) ;
#101873=AXIS2_PLACEMENT_3D('',#165917,#130136,#130137) ;
#101874=AXIS2_PLACEMENT_3D('',#165918,#130138,#130139) ;
#101875=AXIS2_PLACEMENT_3D('',#165919,#130140,#130141) ;
#101876=AXIS2_PLACEMENT_3D('',#165920,#130142,#130143) ;
#101877=AXIS2_PLACEMENT_3D('',#165921,#130144,#130145) ;
#101878=AXIS2_PLACEMENT_3D('',#165922,#130146,#130147) ;
#101879=AXIS2_PLACEMENT_3D('',#165923,#130148,#130149) ;
#101880=AXIS2_PLACEMENT_3D('',#165924,#130150,#130151) ;
#101881=AXIS2_PLACEMENT_3D('',#165925,#130152,#130153) ;
#101882=AXIS2_PLACEMENT_3D('',#165926,#130154,#130155) ;
#101883=AXIS2_PLACEMENT_3D('',#165927,#130156,#130157) ;
#101884=AXIS2_PLACEMENT_3D('',#165928,#130158,#130159) ;
#101885=AXIS2_PLACEMENT_3D('',#165929,#130160,#130161) ;
#101886=AXIS2_PLACEMENT_3D('',#165930,#130162,#130163) ;
#101887=AXIS2_PLACEMENT_3D('',#165931,#130164,#130165) ;
#101888=AXIS2_PLACEMENT_3D('',#165932,#130166,#130167) ;
#101889=AXIS2_PLACEMENT_3D('',#165933,#130168,#130169) ;
#101890=AXIS2_PLACEMENT_3D('',#165934,#130170,#130171) ;
#101891=AXIS2_PLACEMENT_3D('',#165935,#130172,#130173) ;
#101892=AXIS2_PLACEMENT_3D('',#165936,#130174,#130175) ;
#101893=AXIS2_PLACEMENT_3D('',#165937,#130176,#130177) ;
#101894=AXIS2_PLACEMENT_3D('',#165938,#130178,#130179) ;
#101895=AXIS2_PLACEMENT_3D('',#165939,#130180,#130181) ;
#101896=AXIS2_PLACEMENT_3D('',#165940,#130182,#130183) ;
#101897=AXIS2_PLACEMENT_3D('',#165941,#130184,#130185) ;
#101898=AXIS2_PLACEMENT_3D('',#165942,#130186,#130187) ;
#101899=AXIS2_PLACEMENT_3D('',#165943,#130188,#130189) ;
#101900=AXIS2_PLACEMENT_3D('',#165944,#130190,#130191) ;
#101901=AXIS2_PLACEMENT_3D('',#165945,#130192,#130193) ;
#101902=AXIS2_PLACEMENT_3D('',#165946,#130194,#130195) ;
#101903=AXIS2_PLACEMENT_3D('',#165947,#130196,#130197) ;
#101904=AXIS2_PLACEMENT_3D('',#165948,#130198,#130199) ;
#101905=AXIS2_PLACEMENT_3D('',#165949,#130200,#130201) ;
#101906=AXIS2_PLACEMENT_3D('',#165950,#130202,#130203) ;
#101907=AXIS2_PLACEMENT_3D('',#165951,#130204,#130205) ;
#101908=AXIS2_PLACEMENT_3D('',#165952,#130206,#130207) ;
#101909=AXIS2_PLACEMENT_3D('',#165953,#130208,#130209) ;
#101910=AXIS2_PLACEMENT_3D('',#165954,#130210,#130211) ;
#101911=AXIS2_PLACEMENT_3D('',#165955,#130212,#130213) ;
#101912=AXIS2_PLACEMENT_3D('',#165956,#130214,#130215) ;
#101913=AXIS2_PLACEMENT_3D('',#165957,#130216,#130217) ;
#101914=AXIS2_PLACEMENT_3D('',#165958,#130218,#130219) ;
#101915=AXIS2_PLACEMENT_3D('',#165959,#130220,#130221) ;
#101916=AXIS2_PLACEMENT_3D('',#165960,#130222,#130223) ;
#101917=AXIS2_PLACEMENT_3D('',#165961,#130224,#130225) ;
#101918=AXIS2_PLACEMENT_3D('',#165962,#130226,#130227) ;
#101919=AXIS2_PLACEMENT_3D('',#165963,#130228,#130229) ;
#101920=AXIS2_PLACEMENT_3D('',#165964,#130230,#130231) ;
#101921=AXIS2_PLACEMENT_3D('',#165965,#130232,#130233) ;
#101922=AXIS2_PLACEMENT_3D('',#165966,#130234,#130235) ;
#101923=AXIS2_PLACEMENT_3D('',#165967,#130236,#130237) ;
#101924=AXIS2_PLACEMENT_3D('',#165968,#130238,#130239) ;
#101925=AXIS2_PLACEMENT_3D('',#165969,#130240,#130241) ;
#101926=AXIS2_PLACEMENT_3D('',#165970,#130242,#130243) ;
#101927=AXIS2_PLACEMENT_3D('',#165971,#130244,#130245) ;
#101928=AXIS2_PLACEMENT_3D('',#165972,#130246,#130247) ;
#101929=AXIS2_PLACEMENT_3D('',#165973,#130248,#130249) ;
#101930=AXIS2_PLACEMENT_3D('',#165974,#130250,#130251) ;
#101931=AXIS2_PLACEMENT_3D('',#165975,#130252,#130253) ;
#101932=AXIS2_PLACEMENT_3D('',#165976,#130254,#130255) ;
#101933=AXIS2_PLACEMENT_3D('',#165977,#130256,#130257) ;
#101934=AXIS2_PLACEMENT_3D('',#165978,#130258,#130259) ;
#101935=AXIS2_PLACEMENT_3D('',#165979,#130260,#130261) ;
#101936=AXIS2_PLACEMENT_3D('',#165980,#130262,#130263) ;
#101937=AXIS2_PLACEMENT_3D('',#165981,#130264,#130265) ;
#101938=AXIS2_PLACEMENT_3D('',#165982,#130266,#130267) ;
#101939=AXIS2_PLACEMENT_3D('',#165983,#130268,#130269) ;
#101940=AXIS2_PLACEMENT_3D('',#165984,#130270,#130271) ;
#101941=AXIS2_PLACEMENT_3D('',#165985,#130272,#130273) ;
#101942=AXIS2_PLACEMENT_3D('',#165986,#130274,#130275) ;
#101943=AXIS2_PLACEMENT_3D('',#165987,#130276,#130277) ;
#101944=AXIS2_PLACEMENT_3D('',#165988,#130278,#130279) ;
#101945=AXIS2_PLACEMENT_3D('',#165989,#130280,#130281) ;
#101946=AXIS2_PLACEMENT_3D('',#165990,#130282,#130283) ;
#101947=AXIS2_PLACEMENT_3D('',#165991,#130284,#130285) ;
#101948=AXIS2_PLACEMENT_3D('',#165992,#130286,#130287) ;
#101949=AXIS2_PLACEMENT_3D('',#165993,#130288,#130289) ;
#101950=AXIS2_PLACEMENT_3D('',#165994,#130290,#130291) ;
#101951=AXIS2_PLACEMENT_3D('',#165995,#130292,#130293) ;
#101952=AXIS2_PLACEMENT_3D('',#165996,#130294,#130295) ;
#101953=AXIS2_PLACEMENT_3D('',#165997,#130296,#130297) ;
#101954=AXIS2_PLACEMENT_3D('',#165998,#130298,#130299) ;
#101955=AXIS2_PLACEMENT_3D('',#165999,#130300,#130301) ;
#101956=AXIS2_PLACEMENT_3D('',#166000,#130302,#130303) ;
#101957=AXIS2_PLACEMENT_3D('',#166001,#130304,#130305) ;
#101958=AXIS2_PLACEMENT_3D('',#166002,#130306,#130307) ;
#101959=AXIS2_PLACEMENT_3D('',#166003,#130308,#130309) ;
#101960=AXIS2_PLACEMENT_3D('',#166004,#130310,#130311) ;
#101961=AXIS2_PLACEMENT_3D('',#166005,#130312,#130313) ;
#101962=AXIS2_PLACEMENT_3D('',#166030,#130314,#130315) ;
#101963=AXIS2_PLACEMENT_3D('',#166031,#130316,#130317) ;
#101964=AXIS2_PLACEMENT_3D('',#166032,#130318,#130319) ;
#101965=AXIS2_PLACEMENT_3D('',#166057,#130320,#130321) ;
#101966=AXIS2_PLACEMENT_3D('',#166058,#130322,#130323) ;
#101967=AXIS2_PLACEMENT_3D('',#166059,#130324,#130325) ;
#101968=AXIS2_PLACEMENT_3D('',#166060,#130326,#130327) ;
#101969=AXIS2_PLACEMENT_3D('',#166085,#130328,#130329) ;
#101970=AXIS2_PLACEMENT_3D('',#166086,#130330,#130331) ;
#101971=AXIS2_PLACEMENT_3D('',#166087,#130332,#130333) ;
#101972=AXIS2_PLACEMENT_3D('',#166088,#130334,#130335) ;
#101973=AXIS2_PLACEMENT_3D('',#166089,#130336,#130337) ;
#101974=AXIS2_PLACEMENT_3D('',#166090,#130338,#130339) ;
#101975=AXIS2_PLACEMENT_3D('',#166091,#130340,#130341) ;
#101976=AXIS2_PLACEMENT_3D('',#166092,#130342,#130343) ;
#101977=AXIS2_PLACEMENT_3D('',#166093,#130344,#130345) ;
#101978=AXIS2_PLACEMENT_3D('',#166094,#130346,#130347) ;
#101979=AXIS2_PLACEMENT_3D('',#166095,#130348,#130349) ;
#101980=AXIS2_PLACEMENT_3D('',#166096,#130350,#130351) ;
#101981=AXIS2_PLACEMENT_3D('',#166097,#130352,#130353) ;
#101982=AXIS2_PLACEMENT_3D('',#166098,#130354,#130355) ;
#101983=AXIS2_PLACEMENT_3D('',#166099,#130356,#130357) ;
#101984=AXIS2_PLACEMENT_3D('',#166100,#130358,#130359) ;
#101985=AXIS2_PLACEMENT_3D('',#166101,#130360,#130361) ;
#101986=AXIS2_PLACEMENT_3D('',#166102,#130362,#130363) ;
#101987=AXIS2_PLACEMENT_3D('',#166103,#130364,#130365) ;
#101988=AXIS2_PLACEMENT_3D('',#166104,#130366,#130367) ;
#101989=AXIS2_PLACEMENT_3D('',#166105,#130368,#130369) ;
#101990=AXIS2_PLACEMENT_3D('',#166154,#130370,#130371) ;
#101991=AXIS2_PLACEMENT_3D('',#166167,#130372,#130373) ;
#101992=AXIS2_PLACEMENT_3D('',#166168,#130374,#130375) ;
#101993=AXIS2_PLACEMENT_3D('',#166169,#130376,#130377) ;
#101994=AXIS2_PLACEMENT_3D('',#166170,#130378,#130379) ;
#101995=AXIS2_PLACEMENT_3D('',#166171,#130380,#130381) ;
#101996=AXIS2_PLACEMENT_3D('',#166172,#130382,#130383) ;
#101997=AXIS2_PLACEMENT_3D('',#166173,#130384,#130385) ;
#101998=AXIS2_PLACEMENT_3D('',#166174,#130386,#130387) ;
#101999=AXIS2_PLACEMENT_3D('',#166175,#130388,#130389) ;
#102000=AXIS2_PLACEMENT_3D('',#166176,#130390,#130391) ;
#102001=AXIS2_PLACEMENT_3D('',#166177,#130392,#130393) ;
#102002=AXIS2_PLACEMENT_3D('',#166178,#130394,#130395) ;
#102003=AXIS2_PLACEMENT_3D('',#166179,#130396,#130397) ;
#102004=AXIS2_PLACEMENT_3D('',#166180,#130398,#130399) ;
#102005=AXIS2_PLACEMENT_3D('',#166181,#130400,#130401) ;
#102006=AXIS2_PLACEMENT_3D('',#166194,#130402,#130403) ;
#102007=AXIS2_PLACEMENT_3D('',#166219,#130404,#130405) ;
#102008=AXIS2_PLACEMENT_3D('',#166232,#130406,#130407) ;
#102009=AXIS2_PLACEMENT_3D('',#166233,#130408,#130409) ;
#102010=AXIS2_PLACEMENT_3D('',#166234,#130410,#130411) ;
#102011=AXIS2_PLACEMENT_3D('',#166235,#130412,#130413) ;
#102012=AXIS2_PLACEMENT_3D('',#166236,#130414,#130415) ;
#102013=AXIS2_PLACEMENT_3D('',#166237,#130416,#130417) ;
#102014=AXIS2_PLACEMENT_3D('',#166238,#130418,#130419) ;
#102015=AXIS2_PLACEMENT_3D('',#166239,#130420,#130421) ;
#102016=AXIS2_PLACEMENT_3D('',#166240,#130422,#130423) ;
#102017=AXIS2_PLACEMENT_3D('',#166241,#130424,#130425) ;
#102018=AXIS2_PLACEMENT_3D('',#166242,#130426,#130427) ;
#102019=AXIS2_PLACEMENT_3D('',#166243,#130428,#130429) ;
#102020=AXIS2_PLACEMENT_3D('',#166244,#130430,#130431) ;
#102021=AXIS2_PLACEMENT_3D('',#166245,#130432,#130433) ;
#102022=AXIS2_PLACEMENT_3D('',#166246,#130434,#130435) ;
#102023=AXIS2_PLACEMENT_3D('',#166259,#130436,#130437) ;
#102024=AXIS2_PLACEMENT_3D('',#166284,#130438,#130439) ;
#102025=AXIS2_PLACEMENT_3D('',#166285,#130440,#130441) ;
#102026=AXIS2_PLACEMENT_3D('',#166286,#130442,#130443) ;
#102027=AXIS2_PLACEMENT_3D('',#166287,#130444,#130445) ;
#102028=AXIS2_PLACEMENT_3D('',#166288,#130446,#130447) ;
#102029=AXIS2_PLACEMENT_3D('',#166289,#130448,#130449) ;
#102030=AXIS2_PLACEMENT_3D('',#166290,#130450,#130451) ;
#102031=AXIS2_PLACEMENT_3D('',#166291,#130452,#130453) ;
#102032=AXIS2_PLACEMENT_3D('',#166292,#130454,#130455) ;
#102033=AXIS2_PLACEMENT_3D('',#166293,#130456,#130457) ;
#102034=AXIS2_PLACEMENT_3D('',#166294,#130458,#130459) ;
#102035=AXIS2_PLACEMENT_3D('',#166295,#130460,#130461) ;
#102036=AXIS2_PLACEMENT_3D('',#166296,#130462,#130463) ;
#102037=AXIS2_PLACEMENT_3D('',#166297,#130464,#130465) ;
#102038=AXIS2_PLACEMENT_3D('',#166298,#130466,#130467) ;
#102039=AXIS2_PLACEMENT_3D('',#166299,#130468,#130469) ;
#102040=AXIS2_PLACEMENT_3D('',#166300,#130470,#130471) ;
#102041=AXIS2_PLACEMENT_3D('',#166301,#130472,#130473) ;
#102042=AXIS2_PLACEMENT_3D('',#166302,#130474,#130475) ;
#102043=AXIS2_PLACEMENT_3D('',#166303,#130476,#130477) ;
#102044=AXIS2_PLACEMENT_3D('',#166304,#130478,#130479) ;
#102045=AXIS2_PLACEMENT_3D('',#166305,#130480,#130481) ;
#102046=AXIS2_PLACEMENT_3D('',#166306,#130482,#130483) ;
#102047=AXIS2_PLACEMENT_3D('',#166307,#130484,#130485) ;
#102048=AXIS2_PLACEMENT_3D('',#166308,#130486,#130487) ;
#102049=AXIS2_PLACEMENT_3D('',#166309,#130488,#130489) ;
#102050=AXIS2_PLACEMENT_3D('',#166310,#130490,#130491) ;
#102051=AXIS2_PLACEMENT_3D('',#166311,#130492,#130493) ;
#102052=AXIS2_PLACEMENT_3D('',#166312,#130494,#130495) ;
#102053=AXIS2_PLACEMENT_3D('',#166313,#130496,#130497) ;
#102054=AXIS2_PLACEMENT_3D('',#166314,#130498,#130499) ;
#102055=AXIS2_PLACEMENT_3D('',#166315,#130500,#130501) ;
#102056=AXIS2_PLACEMENT_3D('',#166316,#130502,#130503) ;
#102057=AXIS2_PLACEMENT_3D('',#166317,#130504,#130505) ;
#102058=AXIS2_PLACEMENT_3D('',#166318,#130506,#130507) ;
#102059=AXIS2_PLACEMENT_3D('',#166319,#130508,#130509) ;
#102060=AXIS2_PLACEMENT_3D('',#166320,#130510,#130511) ;
#102061=AXIS2_PLACEMENT_3D('',#166321,#130512,#130513) ;
#102062=AXIS2_PLACEMENT_3D('',#166322,#130514,#130515) ;
#102063=AXIS2_PLACEMENT_3D('',#166323,#130516,#130517) ;
#102064=AXIS2_PLACEMENT_3D('',#166324,#130518,#130519) ;
#102065=AXIS2_PLACEMENT_3D('',#166325,#130520,#130521) ;
#102066=AXIS2_PLACEMENT_3D('',#166326,#130522,#130523) ;
#102067=AXIS2_PLACEMENT_3D('',#166327,#130524,#130525) ;
#102068=AXIS2_PLACEMENT_3D('',#166328,#130526,#130527) ;
#102069=AXIS2_PLACEMENT_3D('',#166329,#130528,#130529) ;
#102070=AXIS2_PLACEMENT_3D('',#166330,#130530,#130531) ;
#102071=AXIS2_PLACEMENT_3D('',#166331,#130532,#130533) ;
#102072=AXIS2_PLACEMENT_3D('',#166332,#130534,#130535) ;
#102073=AXIS2_PLACEMENT_3D('',#166333,#130536,#130537) ;
#102074=AXIS2_PLACEMENT_3D('',#166334,#130538,#130539) ;
#102075=AXIS2_PLACEMENT_3D('',#166335,#130540,#130541) ;
#102076=AXIS2_PLACEMENT_3D('',#166336,#130542,#130543) ;
#102077=AXIS2_PLACEMENT_3D('',#166337,#130544,#130545) ;
#102078=AXIS2_PLACEMENT_3D('',#166338,#130546,#130547) ;
#102079=AXIS2_PLACEMENT_3D('',#166339,#130548,#130549) ;
#102080=AXIS2_PLACEMENT_3D('',#166340,#130550,#130551) ;
#102081=AXIS2_PLACEMENT_3D('',#166341,#130552,#130553) ;
#102082=AXIS2_PLACEMENT_3D('',#166342,#130554,#130555) ;
#102083=AXIS2_PLACEMENT_3D('',#166343,#130556,#130557) ;
#102084=AXIS2_PLACEMENT_3D('',#166344,#130558,#130559) ;
#102085=AXIS2_PLACEMENT_3D('',#166345,#130560,#130561) ;
#102086=AXIS2_PLACEMENT_3D('',#166346,#130562,#130563) ;
#102087=AXIS2_PLACEMENT_3D('',#166347,#130564,#130565) ;
#102088=AXIS2_PLACEMENT_3D('',#166348,#130566,#130567) ;
#102089=AXIS2_PLACEMENT_3D('',#166349,#130568,#130569) ;
#102090=AXIS2_PLACEMENT_3D('',#166350,#130570,#130571) ;
#102091=AXIS2_PLACEMENT_3D('',#166351,#130572,#130573) ;
#102092=AXIS2_PLACEMENT_3D('',#166352,#130574,#130575) ;
#102093=AXIS2_PLACEMENT_3D('',#166353,#130576,#130577) ;
#102094=AXIS2_PLACEMENT_3D('',#166354,#130578,#130579) ;
#102095=AXIS2_PLACEMENT_3D('',#166355,#130580,#130581) ;
#102096=AXIS2_PLACEMENT_3D('',#166356,#130582,#130583) ;
#102097=AXIS2_PLACEMENT_3D('',#166357,#130584,#130585) ;
#102098=AXIS2_PLACEMENT_3D('',#166358,#130586,#130587) ;
#102099=AXIS2_PLACEMENT_3D('',#166359,#130588,#130589) ;
#102100=AXIS2_PLACEMENT_3D('',#166360,#130590,#130591) ;
#102101=AXIS2_PLACEMENT_3D('',#166361,#130592,#130593) ;
#102102=AXIS2_PLACEMENT_3D('',#166362,#130594,#130595) ;
#102103=AXIS2_PLACEMENT_3D('',#166363,#130596,#130597) ;
#102104=AXIS2_PLACEMENT_3D('',#166364,#130598,#130599) ;
#102105=AXIS2_PLACEMENT_3D('',#166365,#130600,#130601) ;
#102106=AXIS2_PLACEMENT_3D('',#166366,#130602,#130603) ;
#102107=AXIS2_PLACEMENT_3D('',#166367,#130604,#130605) ;
#102108=AXIS2_PLACEMENT_3D('',#166368,#130606,#130607) ;
#102109=AXIS2_PLACEMENT_3D('',#166369,#130608,#130609) ;
#102110=AXIS2_PLACEMENT_3D('',#166370,#130610,#130611) ;
#102111=AXIS2_PLACEMENT_3D('',#166371,#130612,#130613) ;
#102112=AXIS2_PLACEMENT_3D('',#166372,#130614,#130615) ;
#102113=AXIS2_PLACEMENT_3D('',#166373,#130616,#130617) ;
#102114=AXIS2_PLACEMENT_3D('',#166374,#130618,#130619) ;
#102115=AXIS2_PLACEMENT_3D('',#166375,#130620,#130621) ;
#102116=AXIS2_PLACEMENT_3D('',#166376,#130622,#130623) ;
#102117=AXIS2_PLACEMENT_3D('',#166377,#130624,#130625) ;
#102118=AXIS2_PLACEMENT_3D('',#166378,#130626,#130627) ;
#102119=AXIS2_PLACEMENT_3D('',#166379,#130628,#130629) ;
#102120=AXIS2_PLACEMENT_3D('',#166380,#130630,#130631) ;
#102121=AXIS2_PLACEMENT_3D('',#166381,#130632,#130633) ;
#102122=AXIS2_PLACEMENT_3D('',#166382,#130634,#130635) ;
#102123=AXIS2_PLACEMENT_3D('',#166383,#130636,#130637) ;
#102124=AXIS2_PLACEMENT_3D('',#166384,#130638,#130639) ;
#102125=AXIS2_PLACEMENT_3D('',#166385,#130640,#130641) ;
#102126=AXIS2_PLACEMENT_3D('',#166386,#130642,#130643) ;
#102127=AXIS2_PLACEMENT_3D('',#166387,#130644,#130645) ;
#102128=AXIS2_PLACEMENT_3D('',#166388,#130646,#130647) ;
#102129=AXIS2_PLACEMENT_3D('',#166389,#130648,#130649) ;
#102130=AXIS2_PLACEMENT_3D('',#166390,#130650,#130651) ;
#102131=AXIS2_PLACEMENT_3D('',#166391,#130652,#130653) ;
#102132=AXIS2_PLACEMENT_3D('',#166392,#130654,#130655) ;
#102133=AXIS2_PLACEMENT_3D('',#166393,#130656,#130657) ;
#102134=AXIS2_PLACEMENT_3D('',#166394,#130658,#130659) ;
#102135=AXIS2_PLACEMENT_3D('',#166395,#130660,#130661) ;
#102136=AXIS2_PLACEMENT_3D('',#166396,#130662,#130663) ;
#102137=AXIS2_PLACEMENT_3D('',#166397,#130664,#130665) ;
#102138=AXIS2_PLACEMENT_3D('',#166398,#130666,#130667) ;
#102139=AXIS2_PLACEMENT_3D('',#166399,#130668,#130669) ;
#102140=AXIS2_PLACEMENT_3D('',#166400,#130670,#130671) ;
#102141=AXIS2_PLACEMENT_3D('',#166401,#130672,#130673) ;
#102142=AXIS2_PLACEMENT_3D('',#166402,#130674,#130675) ;
#102143=AXIS2_PLACEMENT_3D('',#166403,#130676,#130677) ;
#102144=AXIS2_PLACEMENT_3D('',#166404,#130678,#130679) ;
#102145=AXIS2_PLACEMENT_3D('',#166405,#130680,#130681) ;
#102146=AXIS2_PLACEMENT_3D('',#166406,#130682,#130683) ;
#102147=AXIS2_PLACEMENT_3D('',#166407,#130684,#130685) ;
#102148=AXIS2_PLACEMENT_3D('',#166408,#130686,#130687) ;
#102149=AXIS2_PLACEMENT_3D('',#166409,#130688,#130689) ;
#102150=AXIS2_PLACEMENT_3D('',#166410,#130690,#130691) ;
#102151=AXIS2_PLACEMENT_3D('',#166411,#130692,#130693) ;
#102152=AXIS2_PLACEMENT_3D('',#166412,#130694,#130695) ;
#102153=AXIS2_PLACEMENT_3D('',#166413,#130696,#130697) ;
#102154=AXIS2_PLACEMENT_3D('',#166414,#130698,#130699) ;
#102155=AXIS2_PLACEMENT_3D('',#166415,#130700,#130701) ;
#102156=AXIS2_PLACEMENT_3D('',#166416,#130702,#130703) ;
#102157=AXIS2_PLACEMENT_3D('',#166417,#130704,#130705) ;
#102158=AXIS2_PLACEMENT_3D('',#166418,#130706,#130707) ;
#102159=AXIS2_PLACEMENT_3D('',#166419,#130708,#130709) ;
#102160=AXIS2_PLACEMENT_3D('',#166420,#130710,#130711) ;
#102161=AXIS2_PLACEMENT_3D('',#166421,#130712,#130713) ;
#102162=AXIS2_PLACEMENT_3D('',#166422,#130714,#130715) ;
#102163=AXIS2_PLACEMENT_3D('',#166423,#130716,#130717) ;
#102164=AXIS2_PLACEMENT_3D('',#166424,#130718,#130719) ;
#102165=AXIS2_PLACEMENT_3D('',#166425,#130720,#130721) ;
#102166=AXIS2_PLACEMENT_3D('',#166426,#130722,#130723) ;
#102167=AXIS2_PLACEMENT_3D('',#166427,#130724,#130725) ;
#102168=AXIS2_PLACEMENT_3D('',#166428,#130726,#130727) ;
#102169=AXIS2_PLACEMENT_3D('',#166429,#130728,#130729) ;
#102170=AXIS2_PLACEMENT_3D('',#166430,#130730,#130731) ;
#102171=AXIS2_PLACEMENT_3D('',#166431,#130732,#130733) ;
#102172=AXIS2_PLACEMENT_3D('',#166432,#130734,#130735) ;
#102173=AXIS2_PLACEMENT_3D('',#166433,#130736,#130737) ;
#102174=AXIS2_PLACEMENT_3D('',#166434,#130738,#130739) ;
#102175=AXIS2_PLACEMENT_3D('',#166435,#130740,#130741) ;
#102176=AXIS2_PLACEMENT_3D('',#166436,#130742,#130743) ;
#102177=AXIS2_PLACEMENT_3D('',#166437,#130744,#130745) ;
#102178=AXIS2_PLACEMENT_3D('',#166438,#130746,#130747) ;
#102179=AXIS2_PLACEMENT_3D('',#166439,#130748,#130749) ;
#102180=AXIS2_PLACEMENT_3D('',#166440,#130750,#130751) ;
#102181=AXIS2_PLACEMENT_3D('',#166441,#130752,#130753) ;
#102182=AXIS2_PLACEMENT_3D('',#166442,#130754,#130755) ;
#102183=AXIS2_PLACEMENT_3D('',#166443,#130756,#130757) ;
#102184=AXIS2_PLACEMENT_3D('',#166444,#130758,#130759) ;
#102185=AXIS2_PLACEMENT_3D('',#166445,#130760,#130761) ;
#102186=AXIS2_PLACEMENT_3D('',#166446,#130762,#130763) ;
#102187=AXIS2_PLACEMENT_3D('',#166447,#130764,#130765) ;
#102188=AXIS2_PLACEMENT_3D('',#166448,#130766,#130767) ;
#102189=AXIS2_PLACEMENT_3D('',#166449,#130768,#130769) ;
#102190=AXIS2_PLACEMENT_3D('',#166450,#130770,#130771) ;
#102191=AXIS2_PLACEMENT_3D('',#166451,#130772,#130773) ;
#102192=AXIS2_PLACEMENT_3D('',#166452,#130774,#130775) ;
#102193=AXIS2_PLACEMENT_3D('',#166453,#130776,#130777) ;
#102194=AXIS2_PLACEMENT_3D('',#166454,#130778,#130779) ;
#102195=AXIS2_PLACEMENT_3D('',#166455,#130780,#130781) ;
#102196=AXIS2_PLACEMENT_3D('',#166456,#130782,#130783) ;
#102197=AXIS2_PLACEMENT_3D('',#166457,#130784,#130785) ;
#102198=AXIS2_PLACEMENT_3D('',#166458,#130786,#130787) ;
#102199=AXIS2_PLACEMENT_3D('',#166459,#130788,#130789) ;
#102200=AXIS2_PLACEMENT_3D('',#166460,#130790,#130791) ;
#102201=AXIS2_PLACEMENT_3D('',#166461,#130792,#130793) ;
#102202=AXIS2_PLACEMENT_3D('',#166462,#130794,#130795) ;
#102203=AXIS2_PLACEMENT_3D('',#166463,#130796,#130797) ;
#102204=AXIS2_PLACEMENT_3D('',#166464,#130798,#130799) ;
#102205=AXIS2_PLACEMENT_3D('',#166465,#130800,#130801) ;
#102206=AXIS2_PLACEMENT_3D('',#166466,#130802,#130803) ;
#102207=AXIS2_PLACEMENT_3D('',#166467,#130804,#130805) ;
#102208=AXIS2_PLACEMENT_3D('',#166468,#130806,#130807) ;
#102209=AXIS2_PLACEMENT_3D('',#166469,#130808,#130809) ;
#102210=AXIS2_PLACEMENT_3D('',#166470,#130810,#130811) ;
#102211=AXIS2_PLACEMENT_3D('',#166471,#130812,#130813) ;
#102212=AXIS2_PLACEMENT_3D('',#166472,#130814,#130815) ;
#102213=AXIS2_PLACEMENT_3D('',#166473,#130816,#130817) ;
#102214=AXIS2_PLACEMENT_3D('',#166474,#130818,#130819) ;
#102215=AXIS2_PLACEMENT_3D('',#166475,#130820,#130821) ;
#102216=AXIS2_PLACEMENT_3D('',#166476,#130822,#130823) ;
#102217=AXIS2_PLACEMENT_3D('',#166477,#130824,#130825) ;
#102218=AXIS2_PLACEMENT_3D('',#166478,#130826,#130827) ;
#102219=AXIS2_PLACEMENT_3D('',#166479,#130828,#130829) ;
#102220=AXIS2_PLACEMENT_3D('',#166480,#130830,#130831) ;
#102221=AXIS2_PLACEMENT_3D('',#166481,#130832,#130833) ;
#102222=AXIS2_PLACEMENT_3D('',#166482,#130834,#130835) ;
#102223=AXIS2_PLACEMENT_3D('',#166483,#130836,#130837) ;
#102224=AXIS2_PLACEMENT_3D('',#166484,#130838,#130839) ;
#102225=AXIS2_PLACEMENT_3D('',#166485,#130840,#130841) ;
#102226=AXIS2_PLACEMENT_3D('',#166486,#130842,#130843) ;
#102227=AXIS2_PLACEMENT_3D('',#166487,#130844,#130845) ;
#102228=AXIS2_PLACEMENT_3D('',#166488,#130846,#130847) ;
#102229=AXIS2_PLACEMENT_3D('',#166489,#130848,#130849) ;
#102230=AXIS2_PLACEMENT_3D('',#166490,#130850,#130851) ;
#102231=AXIS2_PLACEMENT_3D('',#166491,#130852,#130853) ;
#102232=AXIS2_PLACEMENT_3D('',#166492,#130854,#130855) ;
#102233=AXIS2_PLACEMENT_3D('',#166493,#130856,#130857) ;
#102234=AXIS2_PLACEMENT_3D('',#166494,#130858,#130859) ;
#102235=AXIS2_PLACEMENT_3D('',#166495,#130860,#130861) ;
#102236=AXIS2_PLACEMENT_3D('',#166496,#130862,#130863) ;
#102237=AXIS2_PLACEMENT_3D('',#166497,#130864,#130865) ;
#102238=AXIS2_PLACEMENT_3D('',#166522,#130866,#130867) ;
#102239=AXIS2_PLACEMENT_3D('',#166523,#130868,#130869) ;
#102240=AXIS2_PLACEMENT_3D('',#166524,#130870,#130871) ;
#102241=AXIS2_PLACEMENT_3D('',#166549,#130872,#130873) ;
#102242=AXIS2_PLACEMENT_3D('',#166550,#130874,#130875) ;
#102243=AXIS2_PLACEMENT_3D('',#166551,#130876,#130877) ;
#102244=AXIS2_PLACEMENT_3D('',#166552,#130878,#130879) ;
#102245=AXIS2_PLACEMENT_3D('',#166577,#130880,#130881) ;
#102246=AXIS2_PLACEMENT_3D('',#166578,#130882,#130883) ;
#102247=AXIS2_PLACEMENT_3D('',#166579,#130884,#130885) ;
#102248=AXIS2_PLACEMENT_3D('',#166580,#130886,#130887) ;
#102249=AXIS2_PLACEMENT_3D('',#166581,#130888,#130889) ;
#102250=AXIS2_PLACEMENT_3D('',#166582,#130890,#130891) ;
#102251=AXIS2_PLACEMENT_3D('',#166583,#130892,#130893) ;
#102252=AXIS2_PLACEMENT_3D('',#166584,#130894,#130895) ;
#102253=AXIS2_PLACEMENT_3D('',#166585,#130896,#130897) ;
#102254=AXIS2_PLACEMENT_3D('',#166586,#130898,#130899) ;
#102255=AXIS2_PLACEMENT_3D('',#166587,#130900,#130901) ;
#102256=AXIS2_PLACEMENT_3D('',#166588,#130902,#130903) ;
#102257=AXIS2_PLACEMENT_3D('',#166589,#130904,#130905) ;
#102258=AXIS2_PLACEMENT_3D('',#166590,#130906,#130907) ;
#102259=AXIS2_PLACEMENT_3D('',#166591,#130908,#130909) ;
#102260=AXIS2_PLACEMENT_3D('',#166592,#130910,#130911) ;
#102261=AXIS2_PLACEMENT_3D('',#166593,#130912,#130913) ;
#102262=AXIS2_PLACEMENT_3D('',#166594,#130914,#130915) ;
#102263=AXIS2_PLACEMENT_3D('',#166595,#130916,#130917) ;
#102264=AXIS2_PLACEMENT_3D('',#166596,#130918,#130919) ;
#102265=AXIS2_PLACEMENT_3D('',#166597,#130920,#130921) ;
#102266=AXIS2_PLACEMENT_3D('',#166646,#130922,#130923) ;
#102267=AXIS2_PLACEMENT_3D('',#166659,#130924,#130925) ;
#102268=AXIS2_PLACEMENT_3D('',#166660,#130926,#130927) ;
#102269=AXIS2_PLACEMENT_3D('',#166661,#130928,#130929) ;
#102270=AXIS2_PLACEMENT_3D('',#166662,#130930,#130931) ;
#102271=AXIS2_PLACEMENT_3D('',#166663,#130932,#130933) ;
#102272=AXIS2_PLACEMENT_3D('',#166664,#130934,#130935) ;
#102273=AXIS2_PLACEMENT_3D('',#166665,#130936,#130937) ;
#102274=AXIS2_PLACEMENT_3D('',#166666,#130938,#130939) ;
#102275=AXIS2_PLACEMENT_3D('',#166667,#130940,#130941) ;
#102276=AXIS2_PLACEMENT_3D('',#166668,#130942,#130943) ;
#102277=AXIS2_PLACEMENT_3D('',#166669,#130944,#130945) ;
#102278=AXIS2_PLACEMENT_3D('',#166670,#130946,#130947) ;
#102279=AXIS2_PLACEMENT_3D('',#166671,#130948,#130949) ;
#102280=AXIS2_PLACEMENT_3D('',#166672,#130950,#130951) ;
#102281=AXIS2_PLACEMENT_3D('',#166673,#130952,#130953) ;
#102282=AXIS2_PLACEMENT_3D('',#166686,#130954,#130955) ;
#102283=AXIS2_PLACEMENT_3D('',#166711,#130956,#130957) ;
#102284=AXIS2_PLACEMENT_3D('',#166724,#130958,#130959) ;
#102285=AXIS2_PLACEMENT_3D('',#166725,#130960,#130961) ;
#102286=AXIS2_PLACEMENT_3D('',#166726,#130962,#130963) ;
#102287=AXIS2_PLACEMENT_3D('',#166727,#130964,#130965) ;
#102288=AXIS2_PLACEMENT_3D('',#166728,#130966,#130967) ;
#102289=AXIS2_PLACEMENT_3D('',#166729,#130968,#130969) ;
#102290=AXIS2_PLACEMENT_3D('',#166730,#130970,#130971) ;
#102291=AXIS2_PLACEMENT_3D('',#166731,#130972,#130973) ;
#102292=AXIS2_PLACEMENT_3D('',#166732,#130974,#130975) ;
#102293=AXIS2_PLACEMENT_3D('',#166733,#130976,#130977) ;
#102294=AXIS2_PLACEMENT_3D('',#166734,#130978,#130979) ;
#102295=AXIS2_PLACEMENT_3D('',#166735,#130980,#130981) ;
#102296=AXIS2_PLACEMENT_3D('',#166736,#130982,#130983) ;
#102297=AXIS2_PLACEMENT_3D('',#166737,#130984,#130985) ;
#102298=AXIS2_PLACEMENT_3D('',#166738,#130986,#130987) ;
#102299=AXIS2_PLACEMENT_3D('',#166751,#130988,#130989) ;
#102300=AXIS2_PLACEMENT_3D('',#166776,#130990,#130991) ;
#102301=AXIS2_PLACEMENT_3D('',#166777,#130992,#130993) ;
#102302=AXIS2_PLACEMENT_3D('',#166778,#130994,#130995) ;
#102303=AXIS2_PLACEMENT_3D('',#166779,#130996,#130997) ;
#102304=AXIS2_PLACEMENT_3D('',#166780,#130998,#130999) ;
#102305=AXIS2_PLACEMENT_3D('',#166781,#131000,#131001) ;
#102306=AXIS2_PLACEMENT_3D('',#166782,#131002,#131003) ;
#102307=AXIS2_PLACEMENT_3D('',#166783,#131004,#131005) ;
#102308=AXIS2_PLACEMENT_3D('',#166784,#131006,#131007) ;
#102309=AXIS2_PLACEMENT_3D('',#166785,#131008,#131009) ;
#102310=AXIS2_PLACEMENT_3D('',#166786,#131010,#131011) ;
#102311=AXIS2_PLACEMENT_3D('',#166787,#131012,#131013) ;
#102312=AXIS2_PLACEMENT_3D('',#166788,#131014,#131015) ;
#102313=AXIS2_PLACEMENT_3D('',#166789,#131016,#131017) ;
#102314=AXIS2_PLACEMENT_3D('',#166790,#131018,#131019) ;
#102315=AXIS2_PLACEMENT_3D('',#166791,#131020,#131021) ;
#102316=AXIS2_PLACEMENT_3D('',#166792,#131022,#131023) ;
#102317=AXIS2_PLACEMENT_3D('',#166793,#131024,#131025) ;
#102318=AXIS2_PLACEMENT_3D('',#166794,#131026,#131027) ;
#102319=AXIS2_PLACEMENT_3D('',#166795,#131028,#131029) ;
#102320=AXIS2_PLACEMENT_3D('',#166796,#131030,#131031) ;
#102321=AXIS2_PLACEMENT_3D('',#166797,#131032,#131033) ;
#102322=AXIS2_PLACEMENT_3D('',#166798,#131034,#131035) ;
#102323=AXIS2_PLACEMENT_3D('',#166799,#131036,#131037) ;
#102324=AXIS2_PLACEMENT_3D('',#166800,#131038,#131039) ;
#102325=AXIS2_PLACEMENT_3D('',#166801,#131040,#131041) ;
#102326=AXIS2_PLACEMENT_3D('',#166802,#131042,#131043) ;
#102327=AXIS2_PLACEMENT_3D('',#166803,#131044,#131045) ;
#102328=AXIS2_PLACEMENT_3D('',#166804,#131046,#131047) ;
#102329=AXIS2_PLACEMENT_3D('',#166805,#131048,#131049) ;
#102330=AXIS2_PLACEMENT_3D('',#166806,#131050,#131051) ;
#102331=AXIS2_PLACEMENT_3D('',#166807,#131052,#131053) ;
#102332=AXIS2_PLACEMENT_3D('',#166808,#131054,#131055) ;
#102333=AXIS2_PLACEMENT_3D('',#166809,#131056,#131057) ;
#102334=AXIS2_PLACEMENT_3D('',#166810,#131058,#131059) ;
#102335=AXIS2_PLACEMENT_3D('',#166811,#131060,#131061) ;
#102336=AXIS2_PLACEMENT_3D('',#166812,#131062,#131063) ;
#102337=AXIS2_PLACEMENT_3D('',#166813,#131064,#131065) ;
#102338=AXIS2_PLACEMENT_3D('',#166814,#131066,#131067) ;
#102339=AXIS2_PLACEMENT_3D('',#166815,#131068,#131069) ;
#102340=AXIS2_PLACEMENT_3D('',#166816,#131070,#131071) ;
#102341=AXIS2_PLACEMENT_3D('',#166817,#131072,#131073) ;
#102342=AXIS2_PLACEMENT_3D('',#166818,#131074,#131075) ;
#102343=AXIS2_PLACEMENT_3D('',#166819,#131076,#131077) ;
#102344=AXIS2_PLACEMENT_3D('',#166820,#131078,#131079) ;
#102345=AXIS2_PLACEMENT_3D('',#166821,#131080,#131081) ;
#102346=AXIS2_PLACEMENT_3D('',#166822,#131082,#131083) ;
#102347=AXIS2_PLACEMENT_3D('',#166823,#131084,#131085) ;
#102348=AXIS2_PLACEMENT_3D('',#166824,#131086,#131087) ;
#102349=AXIS2_PLACEMENT_3D('',#166825,#131088,#131089) ;
#102350=AXIS2_PLACEMENT_3D('',#166826,#131090,#131091) ;
#102351=AXIS2_PLACEMENT_3D('',#166827,#131092,#131093) ;
#102352=AXIS2_PLACEMENT_3D('',#166828,#131094,#131095) ;
#102353=AXIS2_PLACEMENT_3D('',#166829,#131096,#131097) ;
#102354=AXIS2_PLACEMENT_3D('',#166830,#131098,#131099) ;
#102355=AXIS2_PLACEMENT_3D('',#166831,#131100,#131101) ;
#102356=AXIS2_PLACEMENT_3D('',#166832,#131102,#131103) ;
#102357=AXIS2_PLACEMENT_3D('',#166833,#131104,#131105) ;
#102358=AXIS2_PLACEMENT_3D('',#166834,#131106,#131107) ;
#102359=AXIS2_PLACEMENT_3D('',#166835,#131108,#131109) ;
#102360=AXIS2_PLACEMENT_3D('',#166836,#131110,#131111) ;
#102361=AXIS2_PLACEMENT_3D('',#166837,#131112,#131113) ;
#102362=AXIS2_PLACEMENT_3D('',#166838,#131114,#131115) ;
#102363=AXIS2_PLACEMENT_3D('',#166839,#131116,#131117) ;
#102364=AXIS2_PLACEMENT_3D('',#166840,#131118,#131119) ;
#102365=AXIS2_PLACEMENT_3D('',#166841,#131120,#131121) ;
#102366=AXIS2_PLACEMENT_3D('',#166842,#131122,#131123) ;
#102367=AXIS2_PLACEMENT_3D('',#166843,#131124,#131125) ;
#102368=AXIS2_PLACEMENT_3D('',#166844,#131126,#131127) ;
#102369=AXIS2_PLACEMENT_3D('',#166845,#131128,#131129) ;
#102370=AXIS2_PLACEMENT_3D('',#166846,#131130,#131131) ;
#102371=AXIS2_PLACEMENT_3D('',#166847,#131132,#131133) ;
#102372=AXIS2_PLACEMENT_3D('',#166848,#131134,#131135) ;
#102373=AXIS2_PLACEMENT_3D('',#166849,#131136,#131137) ;
#102374=AXIS2_PLACEMENT_3D('',#166850,#131138,#131139) ;
#102375=AXIS2_PLACEMENT_3D('',#166851,#131140,#131141) ;
#102376=AXIS2_PLACEMENT_3D('',#166852,#131142,#131143) ;
#102377=AXIS2_PLACEMENT_3D('',#166853,#131144,#131145) ;
#102378=AXIS2_PLACEMENT_3D('',#166854,#131146,#131147) ;
#102379=AXIS2_PLACEMENT_3D('',#166855,#131148,#131149) ;
#102380=AXIS2_PLACEMENT_3D('',#166856,#131150,#131151) ;
#102381=AXIS2_PLACEMENT_3D('',#166857,#131152,#131153) ;
#102382=AXIS2_PLACEMENT_3D('',#166858,#131154,#131155) ;
#102383=AXIS2_PLACEMENT_3D('',#166859,#131156,#131157) ;
#102384=AXIS2_PLACEMENT_3D('',#166860,#131158,#131159) ;
#102385=AXIS2_PLACEMENT_3D('',#166861,#131160,#131161) ;
#102386=AXIS2_PLACEMENT_3D('',#166862,#131162,#131163) ;
#102387=AXIS2_PLACEMENT_3D('',#166863,#131164,#131165) ;
#102388=AXIS2_PLACEMENT_3D('',#166864,#131166,#131167) ;
#102389=AXIS2_PLACEMENT_3D('',#166865,#131168,#131169) ;
#102390=AXIS2_PLACEMENT_3D('',#166866,#131170,#131171) ;
#102391=AXIS2_PLACEMENT_3D('',#166867,#131172,#131173) ;
#102392=AXIS2_PLACEMENT_3D('',#166868,#131174,#131175) ;
#102393=AXIS2_PLACEMENT_3D('',#166869,#131176,#131177) ;
#102394=AXIS2_PLACEMENT_3D('',#166870,#131178,#131179) ;
#102395=AXIS2_PLACEMENT_3D('',#166871,#131180,#131181) ;
#102396=AXIS2_PLACEMENT_3D('',#166872,#131182,#131183) ;
#102397=AXIS2_PLACEMENT_3D('',#166873,#131184,#131185) ;
#102398=AXIS2_PLACEMENT_3D('',#166874,#131186,#131187) ;
#102399=AXIS2_PLACEMENT_3D('',#166875,#131188,#131189) ;
#102400=AXIS2_PLACEMENT_3D('',#166876,#131190,#131191) ;
#102401=AXIS2_PLACEMENT_3D('',#166877,#131192,#131193) ;
#102402=AXIS2_PLACEMENT_3D('',#166878,#131194,#131195) ;
#102403=AXIS2_PLACEMENT_3D('',#166879,#131196,#131197) ;
#102404=AXIS2_PLACEMENT_3D('',#166880,#131198,#131199) ;
#102405=AXIS2_PLACEMENT_3D('',#166881,#131200,#131201) ;
#102406=AXIS2_PLACEMENT_3D('',#166882,#131202,#131203) ;
#102407=AXIS2_PLACEMENT_3D('',#166883,#131204,#131205) ;
#102408=AXIS2_PLACEMENT_3D('',#166884,#131206,#131207) ;
#102409=AXIS2_PLACEMENT_3D('',#166885,#131208,#131209) ;
#102410=AXIS2_PLACEMENT_3D('',#166886,#131210,#131211) ;
#102411=AXIS2_PLACEMENT_3D('',#166887,#131212,#131213) ;
#102412=AXIS2_PLACEMENT_3D('',#166888,#131214,#131215) ;
#102413=AXIS2_PLACEMENT_3D('',#166889,#131216,#131217) ;
#102414=AXIS2_PLACEMENT_3D('',#166890,#131218,#131219) ;
#102415=AXIS2_PLACEMENT_3D('',#166891,#131220,#131221) ;
#102416=AXIS2_PLACEMENT_3D('',#166892,#131222,#131223) ;
#102417=AXIS2_PLACEMENT_3D('',#166893,#131224,#131225) ;
#102418=AXIS2_PLACEMENT_3D('',#166894,#131226,#131227) ;
#102419=AXIS2_PLACEMENT_3D('',#166895,#131228,#131229) ;
#102420=AXIS2_PLACEMENT_3D('',#166896,#131230,#131231) ;
#102421=AXIS2_PLACEMENT_3D('',#166897,#131232,#131233) ;
#102422=AXIS2_PLACEMENT_3D('',#166898,#131234,#131235) ;
#102423=AXIS2_PLACEMENT_3D('',#166899,#131236,#131237) ;
#102424=AXIS2_PLACEMENT_3D('',#166900,#131238,#131239) ;
#102425=AXIS2_PLACEMENT_3D('',#166901,#131240,#131241) ;
#102426=AXIS2_PLACEMENT_3D('',#166902,#131242,#131243) ;
#102427=AXIS2_PLACEMENT_3D('',#166903,#131244,#131245) ;
#102428=AXIS2_PLACEMENT_3D('',#166904,#131246,#131247) ;
#102429=AXIS2_PLACEMENT_3D('',#166905,#131248,#131249) ;
#102430=AXIS2_PLACEMENT_3D('',#166906,#131250,#131251) ;
#102431=AXIS2_PLACEMENT_3D('',#166907,#131252,#131253) ;
#102432=AXIS2_PLACEMENT_3D('',#166908,#131254,#131255) ;
#102433=AXIS2_PLACEMENT_3D('',#166909,#131256,#131257) ;
#102434=AXIS2_PLACEMENT_3D('',#166910,#131258,#131259) ;
#102435=AXIS2_PLACEMENT_3D('',#166911,#131260,#131261) ;
#102436=AXIS2_PLACEMENT_3D('',#166912,#131262,#131263) ;
#102437=AXIS2_PLACEMENT_3D('',#166913,#131264,#131265) ;
#102438=AXIS2_PLACEMENT_3D('',#166914,#131266,#131267) ;
#102439=AXIS2_PLACEMENT_3D('',#166915,#131268,#131269) ;
#102440=AXIS2_PLACEMENT_3D('',#166916,#131270,#131271) ;
#102441=AXIS2_PLACEMENT_3D('',#166917,#131272,#131273) ;
#102442=AXIS2_PLACEMENT_3D('',#166918,#131274,#131275) ;
#102443=AXIS2_PLACEMENT_3D('',#166919,#131276,#131277) ;
#102444=AXIS2_PLACEMENT_3D('',#166920,#131278,#131279) ;
#102445=AXIS2_PLACEMENT_3D('',#166921,#131280,#131281) ;
#102446=AXIS2_PLACEMENT_3D('',#166922,#131282,#131283) ;
#102447=AXIS2_PLACEMENT_3D('',#166923,#131284,#131285) ;
#102448=AXIS2_PLACEMENT_3D('',#166924,#131286,#131287) ;
#102449=AXIS2_PLACEMENT_3D('',#166925,#131288,#131289) ;
#102450=AXIS2_PLACEMENT_3D('',#166926,#131290,#131291) ;
#102451=AXIS2_PLACEMENT_3D('',#166927,#131292,#131293) ;
#102452=AXIS2_PLACEMENT_3D('',#166928,#131294,#131295) ;
#102453=AXIS2_PLACEMENT_3D('',#166929,#131296,#131297) ;
#102454=AXIS2_PLACEMENT_3D('',#166930,#131298,#131299) ;
#102455=AXIS2_PLACEMENT_3D('',#166931,#131300,#131301) ;
#102456=AXIS2_PLACEMENT_3D('',#166932,#131302,#131303) ;
#102457=AXIS2_PLACEMENT_3D('',#166933,#131304,#131305) ;
#102458=AXIS2_PLACEMENT_3D('',#166934,#131306,#131307) ;
#102459=AXIS2_PLACEMENT_3D('',#166935,#131308,#131309) ;
#102460=AXIS2_PLACEMENT_3D('',#166936,#131310,#131311) ;
#102461=AXIS2_PLACEMENT_3D('',#166937,#131312,#131313) ;
#102462=AXIS2_PLACEMENT_3D('',#166938,#131314,#131315) ;
#102463=AXIS2_PLACEMENT_3D('',#166939,#131316,#131317) ;
#102464=AXIS2_PLACEMENT_3D('',#166940,#131318,#131319) ;
#102465=AXIS2_PLACEMENT_3D('',#166941,#131320,#131321) ;
#102466=AXIS2_PLACEMENT_3D('',#166942,#131322,#131323) ;
#102467=AXIS2_PLACEMENT_3D('',#166943,#131324,#131325) ;
#102468=AXIS2_PLACEMENT_3D('',#166944,#131326,#131327) ;
#102469=AXIS2_PLACEMENT_3D('',#166945,#131328,#131329) ;
#102470=AXIS2_PLACEMENT_3D('',#166946,#131330,#131331) ;
#102471=AXIS2_PLACEMENT_3D('',#166947,#131332,#131333) ;
#102472=AXIS2_PLACEMENT_3D('',#166948,#131334,#131335) ;
#102473=AXIS2_PLACEMENT_3D('',#166949,#131336,#131337) ;
#102474=AXIS2_PLACEMENT_3D('',#166950,#131338,#131339) ;
#102475=AXIS2_PLACEMENT_3D('',#166951,#131340,#131341) ;
#102476=AXIS2_PLACEMENT_3D('',#166952,#131342,#131343) ;
#102477=AXIS2_PLACEMENT_3D('',#166953,#131344,#131345) ;
#102478=AXIS2_PLACEMENT_3D('',#166954,#131346,#131347) ;
#102479=AXIS2_PLACEMENT_3D('',#166955,#131348,#131349) ;
#102480=AXIS2_PLACEMENT_3D('',#166956,#131350,#131351) ;
#102481=AXIS2_PLACEMENT_3D('',#166957,#131352,#131353) ;
#102482=AXIS2_PLACEMENT_3D('',#166958,#131354,#131355) ;
#102483=AXIS2_PLACEMENT_3D('',#166959,#131356,#131357) ;
#102484=AXIS2_PLACEMENT_3D('',#166960,#131358,#131359) ;
#102485=AXIS2_PLACEMENT_3D('',#166961,#131360,#131361) ;
#102486=AXIS2_PLACEMENT_3D('',#166962,#131362,#131363) ;
#102487=AXIS2_PLACEMENT_3D('',#166963,#131364,#131365) ;
#102488=AXIS2_PLACEMENT_3D('',#166964,#131366,#131367) ;
#102489=AXIS2_PLACEMENT_3D('',#166965,#131368,#131369) ;
#102490=AXIS2_PLACEMENT_3D('',#166966,#131370,#131371) ;
#102491=AXIS2_PLACEMENT_3D('',#166967,#131372,#131373) ;
#102492=AXIS2_PLACEMENT_3D('',#166968,#131374,#131375) ;
#102493=AXIS2_PLACEMENT_3D('',#166969,#131376,#131377) ;
#102494=AXIS2_PLACEMENT_3D('',#166970,#131378,#131379) ;
#102495=AXIS2_PLACEMENT_3D('',#166971,#131380,#131381) ;
#102496=AXIS2_PLACEMENT_3D('',#166972,#131382,#131383) ;
#102497=AXIS2_PLACEMENT_3D('',#166973,#131384,#131385) ;
#102498=AXIS2_PLACEMENT_3D('',#166974,#131386,#131387) ;
#102499=AXIS2_PLACEMENT_3D('',#166975,#131388,#131389) ;
#102500=AXIS2_PLACEMENT_3D('',#166976,#131390,#131391) ;
#102501=AXIS2_PLACEMENT_3D('',#166977,#131392,#131393) ;
#102502=AXIS2_PLACEMENT_3D('',#166978,#131394,#131395) ;
#102503=AXIS2_PLACEMENT_3D('',#166979,#131396,#131397) ;
#102504=AXIS2_PLACEMENT_3D('',#166980,#131398,#131399) ;
#102505=AXIS2_PLACEMENT_3D('',#166981,#131400,#131401) ;
#102506=AXIS2_PLACEMENT_3D('',#166982,#131402,#131403) ;
#102507=AXIS2_PLACEMENT_3D('',#166983,#131404,#131405) ;
#102508=AXIS2_PLACEMENT_3D('',#166984,#131406,#131407) ;
#102509=AXIS2_PLACEMENT_3D('',#166985,#131408,#131409) ;
#102510=AXIS2_PLACEMENT_3D('',#166986,#131410,#131411) ;
#102511=AXIS2_PLACEMENT_3D('',#166987,#131412,#131413) ;
#102512=AXIS2_PLACEMENT_3D('',#166988,#131414,#131415) ;
#102513=AXIS2_PLACEMENT_3D('',#166989,#131416,#131417) ;
#102514=AXIS2_PLACEMENT_3D('',#167014,#131418,#131419) ;
#102515=AXIS2_PLACEMENT_3D('',#167015,#131420,#131421) ;
#102516=AXIS2_PLACEMENT_3D('',#167016,#131422,#131423) ;
#102517=AXIS2_PLACEMENT_3D('',#167041,#131424,#131425) ;
#102518=AXIS2_PLACEMENT_3D('',#167042,#131426,#131427) ;
#102519=AXIS2_PLACEMENT_3D('',#167043,#131428,#131429) ;
#102520=AXIS2_PLACEMENT_3D('',#167044,#131430,#131431) ;
#102521=AXIS2_PLACEMENT_3D('',#167069,#131432,#131433) ;
#102522=AXIS2_PLACEMENT_3D('',#167070,#131434,#131435) ;
#102523=AXIS2_PLACEMENT_3D('',#167071,#131436,#131437) ;
#102524=AXIS2_PLACEMENT_3D('',#167072,#131438,#131439) ;
#102525=AXIS2_PLACEMENT_3D('',#167073,#131440,#131441) ;
#102526=AXIS2_PLACEMENT_3D('',#167074,#131442,#131443) ;
#102527=AXIS2_PLACEMENT_3D('',#167075,#131444,#131445) ;
#102528=AXIS2_PLACEMENT_3D('',#167076,#131446,#131447) ;
#102529=AXIS2_PLACEMENT_3D('',#167077,#131448,#131449) ;
#102530=AXIS2_PLACEMENT_3D('',#167078,#131450,#131451) ;
#102531=AXIS2_PLACEMENT_3D('',#167079,#131452,#131453) ;
#102532=AXIS2_PLACEMENT_3D('',#167080,#131454,#131455) ;
#102533=AXIS2_PLACEMENT_3D('',#167081,#131456,#131457) ;
#102534=AXIS2_PLACEMENT_3D('',#167082,#131458,#131459) ;
#102535=AXIS2_PLACEMENT_3D('',#167083,#131460,#131461) ;
#102536=AXIS2_PLACEMENT_3D('',#167084,#131462,#131463) ;
#102537=AXIS2_PLACEMENT_3D('',#167085,#131464,#131465) ;
#102538=AXIS2_PLACEMENT_3D('',#167086,#131466,#131467) ;
#102539=AXIS2_PLACEMENT_3D('',#167087,#131468,#131469) ;
#102540=AXIS2_PLACEMENT_3D('',#167088,#131470,#131471) ;
#102541=AXIS2_PLACEMENT_3D('',#167089,#131472,#131473) ;
#102542=AXIS2_PLACEMENT_3D('',#167138,#131474,#131475) ;
#102543=AXIS2_PLACEMENT_3D('',#167151,#131476,#131477) ;
#102544=AXIS2_PLACEMENT_3D('',#167152,#131478,#131479) ;
#102545=AXIS2_PLACEMENT_3D('',#167153,#131480,#131481) ;
#102546=AXIS2_PLACEMENT_3D('',#167154,#131482,#131483) ;
#102547=AXIS2_PLACEMENT_3D('',#167155,#131484,#131485) ;
#102548=AXIS2_PLACEMENT_3D('',#167156,#131486,#131487) ;
#102549=AXIS2_PLACEMENT_3D('',#167157,#131488,#131489) ;
#102550=AXIS2_PLACEMENT_3D('',#167158,#131490,#131491) ;
#102551=AXIS2_PLACEMENT_3D('',#167159,#131492,#131493) ;
#102552=AXIS2_PLACEMENT_3D('',#167160,#131494,#131495) ;
#102553=AXIS2_PLACEMENT_3D('',#167161,#131496,#131497) ;
#102554=AXIS2_PLACEMENT_3D('',#167162,#131498,#131499) ;
#102555=AXIS2_PLACEMENT_3D('',#167163,#131500,#131501) ;
#102556=AXIS2_PLACEMENT_3D('',#167164,#131502,#131503) ;
#102557=AXIS2_PLACEMENT_3D('',#167165,#131504,#131505) ;
#102558=AXIS2_PLACEMENT_3D('',#167178,#131506,#131507) ;
#102559=AXIS2_PLACEMENT_3D('',#167203,#131508,#131509) ;
#102560=AXIS2_PLACEMENT_3D('',#167216,#131510,#131511) ;
#102561=AXIS2_PLACEMENT_3D('',#167217,#131512,#131513) ;
#102562=AXIS2_PLACEMENT_3D('',#167218,#131514,#131515) ;
#102563=AXIS2_PLACEMENT_3D('',#167219,#131516,#131517) ;
#102564=AXIS2_PLACEMENT_3D('',#167220,#131518,#131519) ;
#102565=AXIS2_PLACEMENT_3D('',#167221,#131520,#131521) ;
#102566=AXIS2_PLACEMENT_3D('',#167222,#131522,#131523) ;
#102567=AXIS2_PLACEMENT_3D('',#167223,#131524,#131525) ;
#102568=AXIS2_PLACEMENT_3D('',#167224,#131526,#131527) ;
#102569=AXIS2_PLACEMENT_3D('',#167225,#131528,#131529) ;
#102570=AXIS2_PLACEMENT_3D('',#167226,#131530,#131531) ;
#102571=AXIS2_PLACEMENT_3D('',#167227,#131532,#131533) ;
#102572=AXIS2_PLACEMENT_3D('',#167228,#131534,#131535) ;
#102573=AXIS2_PLACEMENT_3D('',#167229,#131536,#131537) ;
#102574=AXIS2_PLACEMENT_3D('',#167230,#131538,#131539) ;
#102575=AXIS2_PLACEMENT_3D('',#167243,#131540,#131541) ;
#102576=AXIS2_PLACEMENT_3D('',#167268,#131542,#131543) ;
#102577=AXIS2_PLACEMENT_3D('',#167269,#131544,#131545) ;
#102578=AXIS2_PLACEMENT_3D('',#167270,#131546,#131547) ;
#102579=AXIS2_PLACEMENT_3D('',#167271,#131548,#131549) ;
#102580=AXIS2_PLACEMENT_3D('',#167272,#131550,#131551) ;
#102581=AXIS2_PLACEMENT_3D('',#167273,#131552,#131553) ;
#102582=AXIS2_PLACEMENT_3D('',#167274,#131554,#131555) ;
#102583=AXIS2_PLACEMENT_3D('',#167275,#131556,#131557) ;
#102584=AXIS2_PLACEMENT_3D('',#167276,#131558,#131559) ;
#102585=AXIS2_PLACEMENT_3D('',#167277,#131560,#131561) ;
#102586=AXIS2_PLACEMENT_3D('',#167278,#131562,#131563) ;
#102587=AXIS2_PLACEMENT_3D('',#167279,#131564,#131565) ;
#102588=AXIS2_PLACEMENT_3D('',#167280,#131566,#131567) ;
#102589=AXIS2_PLACEMENT_3D('',#167281,#131568,#131569) ;
#102590=AXIS2_PLACEMENT_3D('',#167282,#131570,#131571) ;
#102591=AXIS2_PLACEMENT_3D('',#167283,#131572,#131573) ;
#102592=AXIS2_PLACEMENT_3D('',#167284,#131574,#131575) ;
#102593=AXIS2_PLACEMENT_3D('',#167285,#131576,#131577) ;
#102594=AXIS2_PLACEMENT_3D('',#167286,#131578,#131579) ;
#102595=AXIS2_PLACEMENT_3D('',#167287,#131580,#131581) ;
#102596=AXIS2_PLACEMENT_3D('',#167288,#131582,#131583) ;
#102597=AXIS2_PLACEMENT_3D('',#167289,#131584,#131585) ;
#102598=AXIS2_PLACEMENT_3D('',#167290,#131586,#131587) ;
#102599=AXIS2_PLACEMENT_3D('',#167291,#131588,#131589) ;
#102600=AXIS2_PLACEMENT_3D('',#167292,#131590,#131591) ;
#102601=AXIS2_PLACEMENT_3D('',#167293,#131592,#131593) ;
#102602=AXIS2_PLACEMENT_3D('',#167294,#131594,#131595) ;
#102603=AXIS2_PLACEMENT_3D('',#167295,#131596,#131597) ;
#102604=AXIS2_PLACEMENT_3D('',#167296,#131598,#131599) ;
#102605=AXIS2_PLACEMENT_3D('',#167297,#131600,#131601) ;
#102606=AXIS2_PLACEMENT_3D('',#167298,#131602,#131603) ;
#102607=AXIS2_PLACEMENT_3D('',#167299,#131604,#131605) ;
#102608=AXIS2_PLACEMENT_3D('',#167300,#131606,#131607) ;
#102609=AXIS2_PLACEMENT_3D('',#167301,#131608,#131609) ;
#102610=AXIS2_PLACEMENT_3D('',#167302,#131610,#131611) ;
#102611=AXIS2_PLACEMENT_3D('',#167303,#131612,#131613) ;
#102612=AXIS2_PLACEMENT_3D('',#167304,#131614,#131615) ;
#102613=AXIS2_PLACEMENT_3D('',#167305,#131616,#131617) ;
#102614=AXIS2_PLACEMENT_3D('',#167306,#131618,#131619) ;
#102615=AXIS2_PLACEMENT_3D('',#167307,#131620,#131621) ;
#102616=AXIS2_PLACEMENT_3D('',#167308,#131622,#131623) ;
#102617=AXIS2_PLACEMENT_3D('',#167309,#131624,#131625) ;
#102618=AXIS2_PLACEMENT_3D('',#167310,#131626,#131627) ;
#102619=AXIS2_PLACEMENT_3D('',#167311,#131628,#131629) ;
#102620=AXIS2_PLACEMENT_3D('',#167312,#131630,#131631) ;
#102621=AXIS2_PLACEMENT_3D('',#167313,#131632,#131633) ;
#102622=AXIS2_PLACEMENT_3D('',#167314,#131634,#131635) ;
#102623=AXIS2_PLACEMENT_3D('',#167315,#131636,#131637) ;
#102624=AXIS2_PLACEMENT_3D('',#167316,#131638,#131639) ;
#102625=AXIS2_PLACEMENT_3D('',#167317,#131640,#131641) ;
#102626=AXIS2_PLACEMENT_3D('',#167318,#131642,#131643) ;
#102627=AXIS2_PLACEMENT_3D('',#167319,#131644,#131645) ;
#102628=AXIS2_PLACEMENT_3D('',#167320,#131646,#131647) ;
#102629=AXIS2_PLACEMENT_3D('',#167321,#131648,#131649) ;
#102630=AXIS2_PLACEMENT_3D('',#167322,#131650,#131651) ;
#102631=AXIS2_PLACEMENT_3D('',#167323,#131652,#131653) ;
#102632=AXIS2_PLACEMENT_3D('',#167324,#131654,#131655) ;
#102633=AXIS2_PLACEMENT_3D('',#167325,#131656,#131657) ;
#102634=AXIS2_PLACEMENT_3D('',#167326,#131658,#131659) ;
#102635=AXIS2_PLACEMENT_3D('',#167327,#131660,#131661) ;
#102636=AXIS2_PLACEMENT_3D('',#167328,#131662,#131663) ;
#102637=AXIS2_PLACEMENT_3D('',#167329,#131664,#131665) ;
#102638=AXIS2_PLACEMENT_3D('',#167330,#131666,#131667) ;
#102639=AXIS2_PLACEMENT_3D('',#167331,#131668,#131669) ;
#102640=AXIS2_PLACEMENT_3D('',#167332,#131670,#131671) ;
#102641=AXIS2_PLACEMENT_3D('',#167333,#131672,#131673) ;
#102642=AXIS2_PLACEMENT_3D('',#167334,#131674,#131675) ;
#102643=AXIS2_PLACEMENT_3D('',#167335,#131676,#131677) ;
#102644=AXIS2_PLACEMENT_3D('',#167336,#131678,#131679) ;
#102645=AXIS2_PLACEMENT_3D('',#167337,#131680,#131681) ;
#102646=AXIS2_PLACEMENT_3D('',#167338,#131682,#131683) ;
#102647=AXIS2_PLACEMENT_3D('',#167339,#131684,#131685) ;
#102648=AXIS2_PLACEMENT_3D('',#167340,#131686,#131687) ;
#102649=AXIS2_PLACEMENT_3D('',#167341,#131688,#131689) ;
#102650=AXIS2_PLACEMENT_3D('',#167342,#131690,#131691) ;
#102651=AXIS2_PLACEMENT_3D('',#167343,#131692,#131693) ;
#102652=AXIS2_PLACEMENT_3D('',#167344,#131694,#131695) ;
#102653=AXIS2_PLACEMENT_3D('',#167345,#131696,#131697) ;
#102654=AXIS2_PLACEMENT_3D('',#167346,#131698,#131699) ;
#102655=AXIS2_PLACEMENT_3D('',#167347,#131700,#131701) ;
#102656=AXIS2_PLACEMENT_3D('',#167348,#131702,#131703) ;
#102657=AXIS2_PLACEMENT_3D('',#167349,#131704,#131705) ;
#102658=AXIS2_PLACEMENT_3D('',#167350,#131706,#131707) ;
#102659=AXIS2_PLACEMENT_3D('',#167351,#131708,#131709) ;
#102660=AXIS2_PLACEMENT_3D('',#167352,#131710,#131711) ;
#102661=AXIS2_PLACEMENT_3D('',#167353,#131712,#131713) ;
#102662=AXIS2_PLACEMENT_3D('',#167354,#131714,#131715) ;
#102663=AXIS2_PLACEMENT_3D('',#167355,#131716,#131717) ;
#102664=AXIS2_PLACEMENT_3D('',#167356,#131718,#131719) ;
#102665=AXIS2_PLACEMENT_3D('',#167357,#131720,#131721) ;
#102666=AXIS2_PLACEMENT_3D('',#167358,#131722,#131723) ;
#102667=AXIS2_PLACEMENT_3D('',#167359,#131724,#131725) ;
#102668=AXIS2_PLACEMENT_3D('',#167360,#131726,#131727) ;
#102669=AXIS2_PLACEMENT_3D('',#167361,#131728,#131729) ;
#102670=AXIS2_PLACEMENT_3D('',#167362,#131730,#131731) ;
#102671=AXIS2_PLACEMENT_3D('',#167363,#131732,#131733) ;
#102672=AXIS2_PLACEMENT_3D('',#167364,#131734,#131735) ;
#102673=AXIS2_PLACEMENT_3D('',#167365,#131736,#131737) ;
#102674=AXIS2_PLACEMENT_3D('',#167366,#131738,#131739) ;
#102675=AXIS2_PLACEMENT_3D('',#167367,#131740,#131741) ;
#102676=AXIS2_PLACEMENT_3D('',#167368,#131742,#131743) ;
#102677=AXIS2_PLACEMENT_3D('',#167369,#131744,#131745) ;
#102678=AXIS2_PLACEMENT_3D('',#167370,#131746,#131747) ;
#102679=AXIS2_PLACEMENT_3D('',#167371,#131748,#131749) ;
#102680=AXIS2_PLACEMENT_3D('',#167372,#131750,#131751) ;
#102681=AXIS2_PLACEMENT_3D('',#167373,#131752,#131753) ;
#102682=AXIS2_PLACEMENT_3D('',#167374,#131754,#131755) ;
#102683=AXIS2_PLACEMENT_3D('',#167375,#131756,#131757) ;
#102684=AXIS2_PLACEMENT_3D('',#167376,#131758,#131759) ;
#102685=AXIS2_PLACEMENT_3D('',#167377,#131760,#131761) ;
#102686=AXIS2_PLACEMENT_3D('',#167378,#131762,#131763) ;
#102687=AXIS2_PLACEMENT_3D('',#167379,#131764,#131765) ;
#102688=AXIS2_PLACEMENT_3D('',#167380,#131766,#131767) ;
#102689=AXIS2_PLACEMENT_3D('',#167381,#131768,#131769) ;
#102690=AXIS2_PLACEMENT_3D('',#167382,#131770,#131771) ;
#102691=AXIS2_PLACEMENT_3D('',#167383,#131772,#131773) ;
#102692=AXIS2_PLACEMENT_3D('',#167384,#131774,#131775) ;
#102693=AXIS2_PLACEMENT_3D('',#167385,#131776,#131777) ;
#102694=AXIS2_PLACEMENT_3D('',#167386,#131778,#131779) ;
#102695=AXIS2_PLACEMENT_3D('',#167387,#131780,#131781) ;
#102696=AXIS2_PLACEMENT_3D('',#167388,#131782,#131783) ;
#102697=AXIS2_PLACEMENT_3D('',#167389,#131784,#131785) ;
#102698=AXIS2_PLACEMENT_3D('',#167390,#131786,#131787) ;
#102699=AXIS2_PLACEMENT_3D('',#167391,#131788,#131789) ;
#102700=AXIS2_PLACEMENT_3D('',#167392,#131790,#131791) ;
#102701=AXIS2_PLACEMENT_3D('',#167393,#131792,#131793) ;
#102702=AXIS2_PLACEMENT_3D('',#167394,#131794,#131795) ;
#102703=AXIS2_PLACEMENT_3D('',#167395,#131796,#131797) ;
#102704=AXIS2_PLACEMENT_3D('',#167396,#131798,#131799) ;
#102705=AXIS2_PLACEMENT_3D('',#167397,#131800,#131801) ;
#102706=AXIS2_PLACEMENT_3D('',#167398,#131802,#131803) ;
#102707=AXIS2_PLACEMENT_3D('',#167399,#131804,#131805) ;
#102708=AXIS2_PLACEMENT_3D('',#167400,#131806,#131807) ;
#102709=AXIS2_PLACEMENT_3D('',#167401,#131808,#131809) ;
#102710=AXIS2_PLACEMENT_3D('',#167402,#131810,#131811) ;
#102711=AXIS2_PLACEMENT_3D('',#167403,#131812,#131813) ;
#102712=AXIS2_PLACEMENT_3D('',#167404,#131814,#131815) ;
#102713=AXIS2_PLACEMENT_3D('',#167405,#131816,#131817) ;
#102714=AXIS2_PLACEMENT_3D('',#167406,#131818,#131819) ;
#102715=AXIS2_PLACEMENT_3D('',#167407,#131820,#131821) ;
#102716=AXIS2_PLACEMENT_3D('',#167408,#131822,#131823) ;
#102717=AXIS2_PLACEMENT_3D('',#167409,#131824,#131825) ;
#102718=AXIS2_PLACEMENT_3D('',#167410,#131826,#131827) ;
#102719=AXIS2_PLACEMENT_3D('',#167411,#131828,#131829) ;
#102720=AXIS2_PLACEMENT_3D('',#167412,#131830,#131831) ;
#102721=AXIS2_PLACEMENT_3D('',#167413,#131832,#131833) ;
#102722=AXIS2_PLACEMENT_3D('',#167414,#131834,#131835) ;
#102723=AXIS2_PLACEMENT_3D('',#167415,#131836,#131837) ;
#102724=AXIS2_PLACEMENT_3D('',#167416,#131838,#131839) ;
#102725=AXIS2_PLACEMENT_3D('',#167417,#131840,#131841) ;
#102726=AXIS2_PLACEMENT_3D('',#167418,#131842,#131843) ;
#102727=AXIS2_PLACEMENT_3D('',#167419,#131844,#131845) ;
#102728=AXIS2_PLACEMENT_3D('',#167420,#131846,#131847) ;
#102729=AXIS2_PLACEMENT_3D('',#167421,#131848,#131849) ;
#102730=AXIS2_PLACEMENT_3D('',#167422,#131850,#131851) ;
#102731=AXIS2_PLACEMENT_3D('',#167423,#131852,#131853) ;
#102732=AXIS2_PLACEMENT_3D('',#167425,#131854,#131855) ;
#102733=AXIS2_PLACEMENT_3D('',#167452,#131856,#131857) ;
#102734=AXIS2_PLACEMENT_3D('',#167453,#131858,#131859) ;
#102735=AXIS2_PLACEMENT_3D('',#167455,#131860,#131861) ;
#102736=AXIS2_PLACEMENT_3D('',#167456,#131862,#131863) ;
#102737=AXIS2_PLACEMENT_3D('',#167457,#131864,#131865) ;
#102738=AXIS2_PLACEMENT_3D('',#167492,#131866,#131867) ;
#102739=AXIS2_PLACEMENT_3D('',#167519,#131868,#131869) ;
#102740=AXIS2_PLACEMENT_3D('',#167521,#131870,#131871) ;
#102741=AXIS2_PLACEMENT_3D('',#167548,#131872,#131873) ;
#102742=AXIS2_PLACEMENT_3D('',#167549,#131874,#131875) ;
#102743=AXIS2_PLACEMENT_3D('',#167551,#131876,#131877) ;
#102744=AXIS2_PLACEMENT_3D('',#167552,#131878,#131879) ;
#102745=AXIS2_PLACEMENT_3D('',#167553,#131880,#131881) ;
#102746=AXIS2_PLACEMENT_3D('',#167588,#131882,#131883) ;
#102747=AXIS2_PLACEMENT_3D('',#167590,#131884,#131885) ;
#102748=AXIS2_PLACEMENT_3D('',#167617,#131886,#131887) ;
#102749=AXIS2_PLACEMENT_3D('',#167618,#131888,#131889) ;
#102750=AXIS2_PLACEMENT_3D('',#167620,#131890,#131891) ;
#102751=AXIS2_PLACEMENT_3D('',#167621,#131892,#131893) ;
#102752=AXIS2_PLACEMENT_3D('',#167622,#131894,#131895) ;
#102753=AXIS2_PLACEMENT_3D('',#167657,#131896,#131897) ;
#102754=AXIS2_PLACEMENT_3D('',#167659,#131898,#131899) ;
#102755=AXIS2_PLACEMENT_3D('',#167686,#131900,#131901) ;
#102756=AXIS2_PLACEMENT_3D('',#167687,#131902,#131903) ;
#102757=AXIS2_PLACEMENT_3D('',#167689,#131904,#131905) ;
#102758=AXIS2_PLACEMENT_3D('',#167690,#131906,#131907) ;
#102759=AXIS2_PLACEMENT_3D('',#167691,#131908,#131909) ;
#102760=AXIS2_PLACEMENT_3D('',#167726,#131910,#131911) ;
#102761=AXIS2_PLACEMENT_3D('',#167728,#131912,#131913) ;
#102762=AXIS2_PLACEMENT_3D('',#167755,#131914,#131915) ;
#102763=AXIS2_PLACEMENT_3D('',#167756,#131916,#131917) ;
#102764=AXIS2_PLACEMENT_3D('',#167758,#131918,#131919) ;
#102765=AXIS2_PLACEMENT_3D('',#167759,#131920,#131921) ;
#102766=AXIS2_PLACEMENT_3D('',#167760,#131922,#131923) ;
#102767=AXIS2_PLACEMENT_3D('',#167795,#131924,#131925) ;
#102768=AXIS2_PLACEMENT_3D('',#167797,#131926,#131927) ;
#102769=AXIS2_PLACEMENT_3D('',#167824,#131928,#131929) ;
#102770=AXIS2_PLACEMENT_3D('',#167825,#131930,#131931) ;
#102771=AXIS2_PLACEMENT_3D('',#167827,#131932,#131933) ;
#102772=AXIS2_PLACEMENT_3D('',#167828,#131934,#131935) ;
#102773=AXIS2_PLACEMENT_3D('',#167829,#131936,#131937) ;
#102774=AXIS2_PLACEMENT_3D('',#167864,#131938,#131939) ;
#102775=AXIS2_PLACEMENT_3D('',#167866,#131940,#131941) ;
#102776=AXIS2_PLACEMENT_3D('',#167893,#131942,#131943) ;
#102777=AXIS2_PLACEMENT_3D('',#167894,#131944,#131945) ;
#102778=AXIS2_PLACEMENT_3D('',#167896,#131946,#131947) ;
#102779=AXIS2_PLACEMENT_3D('',#167897,#131948,#131949) ;
#102780=AXIS2_PLACEMENT_3D('',#167898,#131950,#131951) ;
#102781=AXIS2_PLACEMENT_3D('',#167933,#131952,#131953) ;
#102782=AXIS2_PLACEMENT_3D('',#167935,#131954,#131955) ;
#102783=AXIS2_PLACEMENT_3D('',#167962,#131956,#131957) ;
#102784=AXIS2_PLACEMENT_3D('',#167963,#131958,#131959) ;
#102785=AXIS2_PLACEMENT_3D('',#167965,#131960,#131961) ;
#102786=AXIS2_PLACEMENT_3D('',#167966,#131962,#131963) ;
#102787=AXIS2_PLACEMENT_3D('',#167967,#131964,#131965) ;
#102788=AXIS2_PLACEMENT_3D('',#168002,#131966,#131967) ;
#102789=AXIS2_PLACEMENT_3D('',#168003,#131968,#131969) ;
#102790=AXIS2_PLACEMENT_3D('',#168005,#131970,#131971) ;
#102791=AXIS2_PLACEMENT_3D('',#168006,#131972,#131973) ;
#102792=AXIS2_PLACEMENT_3D('',#168007,#131974,#131975) ;
#102793=AXIS2_PLACEMENT_3D('',#168042,#131976,#131977) ;
#102794=AXIS2_PLACEMENT_3D('',#168099,#131978,#131979) ;
#102795=AXIS2_PLACEMENT_3D('',#168100,#131980,#131981) ;
#102796=AXIS2_PLACEMENT_3D('',#168101,#131982,#131983) ;
#102797=AXIS2_PLACEMENT_3D('',#168102,#131984,#131985) ;
#102798=AXIS2_PLACEMENT_3D('',#168103,#131986,#131987) ;
#102799=AXIS2_PLACEMENT_3D('',#168104,#131988,#131989) ;
#102800=AXIS2_PLACEMENT_3D('',#168106,#131990,#131991) ;
#102801=AXIS2_PLACEMENT_3D('',#168133,#131992,#131993) ;
#102802=AXIS2_PLACEMENT_3D('',#168134,#131994,#131995) ;
#102803=AXIS2_PLACEMENT_3D('',#168135,#131996,#131997) ;
#102804=AXIS2_PLACEMENT_3D('',#168136,#131998,#131999) ;
#102805=AXIS2_PLACEMENT_3D('',#168137,#132000,#132001) ;
#102806=AXIS2_PLACEMENT_3D('',#168194,#132002,#132003) ;
#102807=AXIS2_PLACEMENT_3D('',#168195,#132004,#132005) ;
#102808=AXIS2_PLACEMENT_3D('',#168196,#132006,#132007) ;
#102809=AXIS2_PLACEMENT_3D('',#168197,#132008,#132009) ;
#102810=AXIS2_PLACEMENT_3D('',#168198,#132010,#132011) ;
#102811=AXIS2_PLACEMENT_3D('',#168199,#132012,#132013) ;
#102812=AXIS2_PLACEMENT_3D('',#168201,#132014,#132015) ;
#102813=AXIS2_PLACEMENT_3D('',#168228,#132016,#132017) ;
#102814=AXIS2_PLACEMENT_3D('',#168229,#132018,#132019) ;
#102815=AXIS2_PLACEMENT_3D('',#168230,#132020,#132021) ;
#102816=AXIS2_PLACEMENT_3D('',#168231,#132022,#132023) ;
#102817=AXIS2_PLACEMENT_3D('',#168232,#132024,#132025) ;
#102818=AXIS2_PLACEMENT_3D('',#168289,#132026,#132027) ;
#102819=AXIS2_PLACEMENT_3D('',#168290,#132028,#132029) ;
#102820=AXIS2_PLACEMENT_3D('',#168291,#132030,#132031) ;
#102821=AXIS2_PLACEMENT_3D('',#168292,#132032,#132033) ;
#102822=AXIS2_PLACEMENT_3D('',#168293,#132034,#132035) ;
#102823=AXIS2_PLACEMENT_3D('',#168294,#132036,#132037) ;
#102824=AXIS2_PLACEMENT_3D('',#168296,#132038,#132039) ;
#102825=AXIS2_PLACEMENT_3D('',#168323,#132040,#132041) ;
#102826=AXIS2_PLACEMENT_3D('',#168324,#132042,#132043) ;
#102827=AXIS2_PLACEMENT_3D('',#168325,#132044,#132045) ;
#102828=AXIS2_PLACEMENT_3D('',#168326,#132046,#132047) ;
#102829=AXIS2_PLACEMENT_3D('',#168327,#132048,#132049) ;
#102830=AXIS2_PLACEMENT_3D('',#168384,#132050,#132051) ;
#102831=AXIS2_PLACEMENT_3D('',#168385,#132052,#132053) ;
#102832=AXIS2_PLACEMENT_3D('',#168386,#132054,#132055) ;
#102833=AXIS2_PLACEMENT_3D('',#168387,#132056,#132057) ;
#102834=AXIS2_PLACEMENT_3D('',#168388,#132058,#132059) ;
#102835=AXIS2_PLACEMENT_3D('',#168389,#132060,#132061) ;
#102836=AXIS2_PLACEMENT_3D('',#168391,#132062,#132063) ;
#102837=AXIS2_PLACEMENT_3D('',#168418,#132064,#132065) ;
#102838=AXIS2_PLACEMENT_3D('',#168419,#132066,#132067) ;
#102839=AXIS2_PLACEMENT_3D('',#168420,#132068,#132069) ;
#102840=AXIS2_PLACEMENT_3D('',#168421,#132070,#132071) ;
#102841=AXIS2_PLACEMENT_3D('',#168422,#132072,#132073) ;
#102842=AXIS2_PLACEMENT_3D('',#168479,#132074,#132075) ;
#102843=AXIS2_PLACEMENT_3D('',#168480,#132076,#132077) ;
#102844=AXIS2_PLACEMENT_3D('',#168481,#132078,#132079) ;
#102845=AXIS2_PLACEMENT_3D('',#168482,#132080,#132081) ;
#102846=AXIS2_PLACEMENT_3D('',#168483,#132082,#132083) ;
#102847=AXIS2_PLACEMENT_3D('',#168484,#132084,#132085) ;
#102848=AXIS2_PLACEMENT_3D('',#168486,#132086,#132087) ;
#102849=AXIS2_PLACEMENT_3D('',#168513,#132088,#132089) ;
#102850=AXIS2_PLACEMENT_3D('',#168514,#132090,#132091) ;
#102851=AXIS2_PLACEMENT_3D('',#168515,#132092,#132093) ;
#102852=AXIS2_PLACEMENT_3D('',#168516,#132094,#132095) ;
#102853=AXIS2_PLACEMENT_3D('',#168517,#132096,#132097) ;
#102854=AXIS2_PLACEMENT_3D('',#168574,#132098,#132099) ;
#102855=AXIS2_PLACEMENT_3D('',#168575,#132100,#132101) ;
#102856=AXIS2_PLACEMENT_3D('',#168576,#132102,#132103) ;
#102857=AXIS2_PLACEMENT_3D('',#168577,#132104,#132105) ;
#102858=AXIS2_PLACEMENT_3D('',#168578,#132106,#132107) ;
#102859=AXIS2_PLACEMENT_3D('',#168579,#132108,#132109) ;
#102860=AXIS2_PLACEMENT_3D('',#168581,#132110,#132111) ;
#102861=AXIS2_PLACEMENT_3D('',#168608,#132112,#132113) ;
#102862=AXIS2_PLACEMENT_3D('',#168609,#132114,#132115) ;
#102863=AXIS2_PLACEMENT_3D('',#168610,#132116,#132117) ;
#102864=AXIS2_PLACEMENT_3D('',#168611,#132118,#132119) ;
#102865=AXIS2_PLACEMENT_3D('',#168612,#132120,#132121) ;
#102866=AXIS2_PLACEMENT_3D('',#168669,#132122,#132123) ;
#102867=AXIS2_PLACEMENT_3D('',#168670,#132124,#132125) ;
#102868=AXIS2_PLACEMENT_3D('',#168671,#132126,#132127) ;
#102869=AXIS2_PLACEMENT_3D('',#168672,#132128,#132129) ;
#102870=AXIS2_PLACEMENT_3D('',#168673,#132130,#132131) ;
#102871=AXIS2_PLACEMENT_3D('',#168674,#132132,#132133) ;
#102872=AXIS2_PLACEMENT_3D('',#168676,#132134,#132135) ;
#102873=AXIS2_PLACEMENT_3D('',#168703,#132136,#132137) ;
#102874=AXIS2_PLACEMENT_3D('',#168704,#132138,#132139) ;
#102875=AXIS2_PLACEMENT_3D('',#168705,#132140,#132141) ;
#102876=AXIS2_PLACEMENT_3D('',#168706,#132142,#132143) ;
#102877=AXIS2_PLACEMENT_3D('',#168707,#132144,#132145) ;
#102878=AXIS2_PLACEMENT_3D('',#168764,#132146,#132147) ;
#102879=AXIS2_PLACEMENT_3D('',#168765,#132148,#132149) ;
#102880=AXIS2_PLACEMENT_3D('',#168766,#132150,#132151) ;
#102881=AXIS2_PLACEMENT_3D('',#168767,#132152,#132153) ;
#102882=AXIS2_PLACEMENT_3D('',#168768,#132154,#132155) ;
#102883=AXIS2_PLACEMENT_3D('',#168769,#132156,#132157) ;
#102884=AXIS2_PLACEMENT_3D('',#168771,#132158,#132159) ;
#102885=AXIS2_PLACEMENT_3D('',#168798,#132160,#132161) ;
#102886=AXIS2_PLACEMENT_3D('',#168799,#132162,#132163) ;
#102887=AXIS2_PLACEMENT_3D('',#168800,#132164,#132165) ;
#102888=AXIS2_PLACEMENT_3D('',#168801,#132166,#132167) ;
#102889=AXIS2_PLACEMENT_3D('',#168802,#132168,#132169) ;
#102890=AXIS2_PLACEMENT_3D('',#168859,#132170,#132171) ;
#102891=AXIS2_PLACEMENT_3D('',#168860,#132172,#132173) ;
#102892=AXIS2_PLACEMENT_3D('',#168861,#132174,#132175) ;
#102893=AXIS2_PLACEMENT_3D('',#168862,#132176,#132177) ;
#102894=AXIS2_PLACEMENT_3D('',#168863,#132178,#132179) ;
#102895=AXIS2_PLACEMENT_3D('',#168864,#132180,#132181) ;
#102896=AXIS2_PLACEMENT_3D('',#168866,#132182,#132183) ;
#102897=AXIS2_PLACEMENT_3D('',#168893,#132184,#132185) ;
#102898=AXIS2_PLACEMENT_3D('',#168894,#132186,#132187) ;
#102899=AXIS2_PLACEMENT_3D('',#168895,#132188,#132189) ;
#102900=AXIS2_PLACEMENT_3D('',#168896,#132190,#132191) ;
#102901=AXIS2_PLACEMENT_3D('',#168897,#132192,#132193) ;
#102902=AXIS2_PLACEMENT_3D('',#168898,#132194,#132195) ;
#102903=AXIS2_PLACEMENT_3D('',#168929,#132196,#132197) ;
#102904=AXIS2_PLACEMENT_3D('',#168930,#132198,#132199) ;
#102905=AXIS2_PLACEMENT_3D('',#168931,#132200,#132201) ;
#102906=AXIS2_PLACEMENT_3D('',#168932,#132202,#132203) ;
#102907=AXIS2_PLACEMENT_3D('',#168963,#132204,#132205) ;
#102908=AXIS2_PLACEMENT_3D('',#168964,#132206,#132207) ;
#102909=AXIS2_PLACEMENT_3D('',#168965,#132208,#132209) ;
#102910=AXIS2_PLACEMENT_3D('',#168966,#132210,#132211) ;
#102911=AXIS2_PLACEMENT_3D('',#168997,#132212,#132213) ;
#102912=AXIS2_PLACEMENT_3D('',#168998,#132214,#132215) ;
#102913=AXIS2_PLACEMENT_3D('',#168999,#132216,#132217) ;
#102914=AXIS2_PLACEMENT_3D('',#169000,#132218,#132219) ;
#102915=AXIS2_PLACEMENT_3D('',#169031,#132220,#132221) ;
#102916=AXIS2_PLACEMENT_3D('',#169032,#132222,#132223) ;
#102917=AXIS2_PLACEMENT_3D('',#169033,#132224,#132225) ;
#102918=AXIS2_PLACEMENT_3D('',#169034,#132226,#132227) ;
#102919=AXIS2_PLACEMENT_3D('',#169065,#132228,#132229) ;
#102920=AXIS2_PLACEMENT_3D('',#169066,#132230,#132231) ;
#102921=AXIS2_PLACEMENT_3D('',#169067,#132232,#132233) ;
#102922=AXIS2_PLACEMENT_3D('',#169068,#132234,#132235) ;
#102923=AXIS2_PLACEMENT_3D('',#169099,#132236,#132237) ;
#102924=AXIS2_PLACEMENT_3D('',#169100,#132238,#132239) ;
#102925=AXIS2_PLACEMENT_3D('',#169101,#132240,#132241) ;
#102926=AXIS2_PLACEMENT_3D('',#169102,#132242,#132243) ;
#102927=AXIS2_PLACEMENT_3D('',#169133,#132244,#132245) ;
#102928=AXIS2_PLACEMENT_3D('',#169134,#132246,#132247) ;
#102929=AXIS2_PLACEMENT_3D('',#169135,#132248,#132249) ;
#102930=AXIS2_PLACEMENT_3D('',#169136,#132250,#132251) ;
#102931=AXIS2_PLACEMENT_3D('',#169167,#132252,#132253) ;
#102932=AXIS2_PLACEMENT_3D('',#169168,#132254,#132255) ;
#102933=AXIS2_PLACEMENT_3D('',#169169,#132256,#132257) ;
#102934=AXIS2_PLACEMENT_3D('',#169170,#132258,#132259) ;
#102935=AXIS2_PLACEMENT_3D('',#169201,#132260,#132261) ;
#102936=AXIS2_PLACEMENT_3D('',#169202,#132262,#132263) ;
#102937=AXIS2_PLACEMENT_3D('',#169203,#132264,#132265) ;
#102938=AXIS2_PLACEMENT_3D('',#169204,#132266,#132267) ;
#102939=AXIS2_PLACEMENT_3D('',#169235,#132268,#132269) ;
#102940=AXIS2_PLACEMENT_3D('',#169236,#132270,#132271) ;
#102941=AXIS2_PLACEMENT_3D('',#169237,#132272,#132273) ;
#102942=AXIS2_PLACEMENT_3D('',#169238,#132274,#132275) ;
#102943=AXIS2_PLACEMENT_3D('',#169269,#132276,#132277) ;
#102944=AXIS2_PLACEMENT_3D('',#169270,#132278,#132279) ;
#102945=AXIS2_PLACEMENT_3D('',#169271,#132280,#132281) ;
#102946=AXIS2_PLACEMENT_3D('',#169272,#132282,#132283) ;
#102947=AXIS2_PLACEMENT_3D('',#169303,#132284,#132285) ;
#102948=AXIS2_PLACEMENT_3D('',#169304,#132286,#132287) ;
#102949=AXIS2_PLACEMENT_3D('',#169305,#132288,#132289) ;
#102950=AXIS2_PLACEMENT_3D('',#169306,#132290,#132291) ;
#102951=AXIS2_PLACEMENT_3D('',#169337,#132292,#132293) ;
#102952=AXIS2_PLACEMENT_3D('',#169338,#132294,#132295) ;
#102953=AXIS2_PLACEMENT_3D('',#169339,#132296,#132297) ;
#102954=AXIS2_PLACEMENT_3D('',#169340,#132298,#132299) ;
#102955=AXIS2_PLACEMENT_3D('',#169371,#132300,#132301) ;
#102956=AXIS2_PLACEMENT_3D('',#169372,#132302,#132303) ;
#102957=AXIS2_PLACEMENT_3D('',#169373,#132304,#132305) ;
#102958=AXIS2_PLACEMENT_3D('',#169374,#132306,#132307) ;
#102959=AXIS2_PLACEMENT_3D('',#169405,#132308,#132309) ;
#102960=AXIS2_PLACEMENT_3D('',#169406,#132310,#132311) ;
#102961=AXIS2_PLACEMENT_3D('',#169407,#132312,#132313) ;
#102962=AXIS2_PLACEMENT_3D('',#169408,#132314,#132315) ;
#102963=AXIS2_PLACEMENT_3D('',#169439,#132316,#132317) ;
#102964=AXIS2_PLACEMENT_3D('',#169440,#132318,#132319) ;
#102965=AXIS2_PLACEMENT_3D('',#169441,#132320,#132321) ;
#102966=AXIS2_PLACEMENT_3D('',#169442,#132322,#132323) ;
#102967=AXIS2_PLACEMENT_3D('',#169473,#132324,#132325) ;
#102968=AXIS2_PLACEMENT_3D('',#169474,#132326,#132327) ;
#102969=AXIS2_PLACEMENT_3D('',#169475,#132328,#132329) ;
#102970=AXIS2_PLACEMENT_3D('',#169476,#132330,#132331) ;
#102971=AXIS2_PLACEMENT_3D('',#169507,#132332,#132333) ;
#102972=AXIS2_PLACEMENT_3D('',#169508,#132334,#132335) ;
#102973=AXIS2_PLACEMENT_3D('',#169509,#132336,#132337) ;
#102974=AXIS2_PLACEMENT_3D('',#169510,#132338,#132339) ;
#102975=AXIS2_PLACEMENT_3D('',#169511,#132340,#132341) ;
#102976=AXIS2_PLACEMENT_3D('',#169512,#132342,#132343) ;
#102977=AXIS2_PLACEMENT_3D('',#169513,#132344,#132345) ;
#102978=AXIS2_PLACEMENT_3D('',#169514,#132346,#132347) ;
#102979=AXIS2_PLACEMENT_3D('',#169515,#132348,#132349) ;
#102980=AXIS2_PLACEMENT_3D('',#169516,#132350,#132351) ;
#102981=AXIS2_PLACEMENT_3D('',#169517,#132352,#132353) ;
#102982=AXIS2_PLACEMENT_3D('',#169518,#132354,#132355) ;
#102983=AXIS2_PLACEMENT_3D('',#169519,#132356,#132357) ;
#102984=AXIS2_PLACEMENT_3D('',#169520,#132358,#132359) ;
#102985=AXIS2_PLACEMENT_3D('',#169521,#132360,#132361) ;
#102986=AXIS2_PLACEMENT_3D('',#169522,#132362,#132363) ;
#102987=AXIS2_PLACEMENT_3D('',#169523,#132364,#132365) ;
#102988=AXIS2_PLACEMENT_3D('',#169524,#132366,#132367) ;
#102989=AXIS2_PLACEMENT_3D('',#169525,#132368,#132369) ;
#102990=AXIS2_PLACEMENT_3D('',#169526,#132370,#132371) ;
#102991=AXIS2_PLACEMENT_3D('',#169527,#132372,#132373) ;
#102992=AXIS2_PLACEMENT_3D('',#169528,#132374,#132375) ;
#102993=AXIS2_PLACEMENT_3D('',#169529,#132376,#132377) ;
#102994=AXIS2_PLACEMENT_3D('',#169530,#132378,#132379) ;
#102995=AXIS2_PLACEMENT_3D('',#169531,#132380,#132381) ;
#102996=AXIS2_PLACEMENT_3D('',#169532,#132382,#132383) ;
#102997=AXIS2_PLACEMENT_3D('',#169533,#132384,#132385) ;
#102998=AXIS2_PLACEMENT_3D('',#169534,#132386,#132387) ;
#102999=AXIS2_PLACEMENT_3D('',#169535,#132388,#132389) ;
#103000=AXIS2_PLACEMENT_3D('',#169536,#132390,#132391) ;
#103001=AXIS2_PLACEMENT_3D('',#169537,#132392,#132393) ;
#103002=AXIS2_PLACEMENT_3D('',#169538,#132394,#132395) ;
#103003=AXIS2_PLACEMENT_3D('',#169539,#132396,#132397) ;
#103004=AXIS2_PLACEMENT_3D('',#169540,#132398,#132399) ;
#103005=AXIS2_PLACEMENT_3D('',#169541,#132400,#132401) ;
#103006=AXIS2_PLACEMENT_3D('',#169542,#132402,#132403) ;
#103007=AXIS2_PLACEMENT_3D('',#169543,#132404,#132405) ;
#103008=AXIS2_PLACEMENT_3D('',#169544,#132406,#132407) ;
#103009=AXIS2_PLACEMENT_3D('',#169545,#132408,#132409) ;
#103010=AXIS2_PLACEMENT_3D('',#169546,#132410,#132411) ;
#103011=AXIS2_PLACEMENT_3D('',#169547,#132412,#132413) ;
#103012=AXIS2_PLACEMENT_3D('',#169548,#132414,#132415) ;
#103013=AXIS2_PLACEMENT_3D('',#169549,#132416,#132417) ;
#103014=AXIS2_PLACEMENT_3D('',#169550,#132418,#132419) ;
#103015=AXIS2_PLACEMENT_3D('',#169551,#132420,#132421) ;
#103016=AXIS2_PLACEMENT_3D('',#169552,#132422,#132423) ;
#103017=AXIS2_PLACEMENT_3D('',#169553,#132424,#132425) ;
#103018=AXIS2_PLACEMENT_3D('',#169554,#132426,#132427) ;
#103019=AXIS2_PLACEMENT_3D('',#169555,#132428,#132429) ;
#103020=AXIS2_PLACEMENT_3D('',#169556,#132430,#132431) ;
#103021=AXIS2_PLACEMENT_3D('',#169557,#132432,#132433) ;
#103022=AXIS2_PLACEMENT_3D('',#169608,#132434,#132435) ;
#103023=AXIS2_PLACEMENT_3D('',#169609,#132436,#132437) ;
#103024=AXIS2_PLACEMENT_3D('',#169640,#132438,#132439) ;
#103025=AXIS2_PLACEMENT_3D('',#169671,#132440,#132441) ;
#103026=AXIS2_PLACEMENT_3D('',#169702,#132442,#132443) ;
#103027=AXIS2_PLACEMENT_3D('',#169733,#132444,#132445) ;
#103028=AXIS2_PLACEMENT_3D('',#169764,#132446,#132447) ;
#103029=AXIS2_PLACEMENT_3D('',#169795,#132448,#132449) ;
#103030=AXIS2_PLACEMENT_3D('',#169826,#132450,#132451) ;
#103031=AXIS2_PLACEMENT_3D('',#169857,#132452,#132453) ;
#103032=AXIS2_PLACEMENT_3D('',#169888,#132454,#132455) ;
#103033=AXIS2_PLACEMENT_3D('',#169889,#132456,#132457) ;
#103034=AXIS2_PLACEMENT_3D('',#169890,#132458,#132459) ;
#103035=AXIS2_PLACEMENT_3D('',#169891,#132460,#132461) ;
#103036=AXIS2_PLACEMENT_3D('',#169892,#132462,#132463) ;
#103037=AXIS2_PLACEMENT_3D('',#169923,#132464,#132465) ;
#103038=AXIS2_PLACEMENT_3D('',#169924,#132466,#132467) ;
#103039=AXIS2_PLACEMENT_3D('',#169925,#132468,#132469) ;
#103040=AXIS2_PLACEMENT_3D('',#169926,#132470,#132471) ;
#103041=AXIS2_PLACEMENT_3D('',#169927,#132472,#132473) ;
#103042=AXIS2_PLACEMENT_3D('',#170008,#132474,#132475) ;
#103043=AXIS2_PLACEMENT_3D('',#170009,#132476,#132477) ;
#103044=AXIS2_PLACEMENT_3D('',#170010,#132478,#132479) ;
#103045=AXIS2_PLACEMENT_3D('',#170011,#132480,#132481) ;
#103046=AXIS2_PLACEMENT_3D('',#170012,#132482,#132483) ;
#103047=AXIS2_PLACEMENT_3D('',#170013,#132484,#132485) ;
#103048=AXIS2_PLACEMENT_3D('',#170014,#132486,#132487) ;
#103049=AXIS2_PLACEMENT_3D('',#170015,#132488,#132489) ;
#103050=AXIS2_PLACEMENT_3D('',#170016,#132490,#132491) ;
#103051=AXIS2_PLACEMENT_3D('',#170017,#132492,#132493) ;
#103052=AXIS2_PLACEMENT_3D('',#170018,#132494,#132495) ;
#103053=AXIS2_PLACEMENT_3D('',#170019,#132496,#132497) ;
#103054=AXIS2_PLACEMENT_3D('',#170020,#132498,#132499) ;
#103055=AXIS2_PLACEMENT_3D('',#170021,#132500,#132501) ;
#103056=AXIS2_PLACEMENT_3D('',#170022,#132502,#132503) ;
#103057=AXIS2_PLACEMENT_3D('',#170023,#132504,#132505) ;
#103058=AXIS2_PLACEMENT_3D('',#170024,#132506,#132507) ;
#103059=AXIS2_PLACEMENT_3D('',#170025,#132508,#132509) ;
#103060=AXIS2_PLACEMENT_3D('',#170026,#132510,#132511) ;
#103061=AXIS2_PLACEMENT_3D('',#170027,#132512,#132513) ;
#103062=AXIS2_PLACEMENT_3D('',#170028,#132514,#132515) ;
#103063=AXIS2_PLACEMENT_3D('',#170029,#132516,#132517) ;
#103064=AXIS2_PLACEMENT_3D('',#170030,#132518,#132519) ;
#103065=AXIS2_PLACEMENT_3D('',#170031,#132520,#132521) ;
#103066=AXIS2_PLACEMENT_3D('',#170032,#132522,#132523) ;
#103067=AXIS2_PLACEMENT_3D('',#170033,#132524,#132525) ;
#103068=AXIS2_PLACEMENT_3D('',#170034,#132526,#132527) ;
#103069=AXIS2_PLACEMENT_3D('',#170035,#132528,#132529) ;
#103070=AXIS2_PLACEMENT_3D('',#170036,#132530,#132531) ;
#103071=AXIS2_PLACEMENT_3D('',#170037,#132532,#132533) ;
#103072=AXIS2_PLACEMENT_3D('',#170038,#132534,#132535) ;
#103073=AXIS2_PLACEMENT_3D('',#170039,#132536,#132537) ;
#103074=AXIS2_PLACEMENT_3D('',#170040,#132538,#132539) ;
#103075=AXIS2_PLACEMENT_3D('',#170065,#132540,#132541) ;
#103076=AXIS2_PLACEMENT_3D('',#170102,#132542,#132543) ;
#120475=DIRECTION('axis',(0.,0.,1.)) ;
#120476=DIRECTION('refdir',(1.,0.,0.)) ;
#120477=DIRECTION('center_axis',(0.,0.,1.)) ;
#120478=DIRECTION('ref_axis',(1.,0.,0.)) ;
#120479=DIRECTION('center_axis',(0.,0.,1.)) ;
#120480=DIRECTION('ref_axis',(1.,0.,0.)) ;
#120481=DIRECTION('',(0.,0.,-1.)) ;
#120482=DIRECTION('center_axis',(0.,0.,1.)) ;
#120483=DIRECTION('ref_axis',(1.,0.,0.)) ;
#120484=DIRECTION('',(0.,0.,1.)) ;
#120485=DIRECTION('center_axis',(-1.31418445149758E-16,1.,0.)) ;
#120486=DIRECTION('ref_axis',(-1.,0.,0.)) ;
#120487=DIRECTION('center_axis',(1.31418445149758E-16,-1.,0.)) ;
#120488=DIRECTION('ref_axis',(-1.,-1.31418445149758E-16,0.)) ;
#120489=DIRECTION('center_axis',(1.,0.,-2.16840434497101E-15)) ;
#120490=DIRECTION('ref_axis',(-2.16840434497101E-15,0.,-1.)) ;
#120491=DIRECTION('center_axis',(-1.31418445149758E-16,1.,0.)) ;
#120492=DIRECTION('ref_axis',(-1.,-1.31418445149758E-16,0.)) ;
#120493=DIRECTION('center_axis',(-0.641814420963378,0.,0.766859993117025)) ;
#120494=DIRECTION('ref_axis',(0.766859993117025,0.,0.641814420963378)) ;
#120495=DIRECTION('center_axis',(-1.31418445149758E-16,1.,0.)) ;
#120496=DIRECTION('ref_axis',(-1.,0.,0.)) ;
#120497=DIRECTION('center_axis',(1.31418445149758E-16,-1.,0.)) ;
#120498=DIRECTION('ref_axis',(-1.,-1.31418445149758E-16,0.)) ;
#120499=DIRECTION('center_axis',(0.823067492614529,0.,0.567943573430699)) ;
#120500=DIRECTION('ref_axis',(0.567943573430699,0.,-0.823067492614529)) ;
#120501=DIRECTION('center_axis',(-1.31418445149758E-16,1.,0.)) ;
#120502=DIRECTION('ref_axis',(-1.,-1.31418445149758E-16,0.)) ;
#120503=DIRECTION('center_axis',(-0.823067492614536,0.,0.56794357343069)) ;
#120504=DIRECTION('ref_axis',(0.56794357343069,0.,0.823067492614536)) ;
#120505=DIRECTION('center_axis',(7.81406971160724E-17,-1.,0.)) ;
#120506=DIRECTION('ref_axis',(1.,0.,0.)) ;
#120507=DIRECTION('center_axis',(7.81406971160724E-17,-1.,0.)) ;
#120508=DIRECTION('ref_axis',(1.,7.81406971160724E-17,0.)) ;
#120509=DIRECTION('center_axis',(-7.81406971160724E-17,1.,0.)) ;
#120510=DIRECTION('ref_axis',(1.,7.81406971160724E-17,-2.66453525910038E-15)) ;
#120511=DIRECTION('center_axis',(-1.31418445149758E-16,1.,0.)) ;
#120512=DIRECTION('ref_axis',(-1.,0.,0.)) ;
#120513=DIRECTION('center_axis',(1.31418445149758E-16,-1.,0.)) ;
#120514=DIRECTION('ref_axis',(-1.,-1.31418445149758E-16,0.)) ;
#120515=DIRECTION('center_axis',(0.823067492614528,-1.78474312718973E-15,
0.567943573430701)) ;
#120516=DIRECTION('ref_axis',(0.567943573430701,-3.32899177295693E-30,-0.823067492614528)) ;
#120517=DIRECTION('center_axis',(-1.31418445149758E-16,1.,0.)) ;
#120518=DIRECTION('ref_axis',(-1.,-1.31418445149758E-16,0.)) ;
#120519=DIRECTION('center_axis',(-0.823067492614537,0.,0.567943573430688)) ;
#120520=DIRECTION('ref_axis',(0.567943573430688,0.,0.823067492614537)) ;
#120521=DIRECTION('center_axis',(7.81406971160724E-17,-1.,0.)) ;
#120522=DIRECTION('ref_axis',(1.,0.,0.)) ;
#120523=DIRECTION('center_axis',(7.81406971160724E-17,-1.,0.)) ;
#120524=DIRECTION('ref_axis',(1.,7.81406971160724E-17,0.)) ;
#120525=DIRECTION('center_axis',(-7.81406971160724E-17,1.,0.)) ;
#120526=DIRECTION('ref_axis',(1.,7.81406971160724E-17,-1.73472347597681E-15)) ;
#120527=DIRECTION('center_axis',(-1.31418445149758E-16,1.,0.)) ;
#120528=DIRECTION('ref_axis',(-1.,0.,0.)) ;
#120529=DIRECTION('center_axis',(1.31418445149758E-16,-1.,0.)) ;
#120530=DIRECTION('ref_axis',(-1.,-1.31418445149758E-16,0.)) ;
#120531=DIRECTION('center_axis',(0.823067492614537,-3.5694862543795E-15,
0.567943573430688)) ;
#120532=DIRECTION('ref_axis',(0.567943573430688,-6.20058923363573E-30,-0.823067492614537)) ;
#120533=DIRECTION('center_axis',(-1.31418445149758E-16,1.,0.)) ;
#120534=DIRECTION('ref_axis',(-1.,-1.31418445149758E-16,0.)) ;
#120535=DIRECTION('center_axis',(-0.823067492614537,0.,0.567943573430688)) ;
#120536=DIRECTION('ref_axis',(0.567943573430688,0.,0.823067492614537)) ;
#120537=DIRECTION('center_axis',(7.81406971160724E-17,-1.,0.)) ;
#120538=DIRECTION('ref_axis',(1.,0.,0.)) ;
#120539=DIRECTION('center_axis',(7.81406971160724E-17,-1.,0.)) ;
#120540=DIRECTION('ref_axis',(1.,7.81406971160724E-17,0.)) ;
#120541=DIRECTION('center_axis',(-7.81406971160724E-17,1.,0.)) ;
#120542=DIRECTION('ref_axis',(1.,7.81406971160724E-17,-1.92747052886312E-15)) ;
#120543=DIRECTION('center_axis',(-1.31418445149758E-16,1.,0.)) ;
#120544=DIRECTION('ref_axis',(-1.,0.,0.)) ;
#120545=DIRECTION('center_axis',(1.31418445149758E-16,-1.,0.)) ;
#120546=DIRECTION('ref_axis',(-1.,-1.31418445149758E-16,0.)) ;
#120547=DIRECTION('center_axis',(0.823067492614537,-3.5694862543795E-15,
0.567943573430688)) ;
#120548=DIRECTION('ref_axis',(0.567943573430688,-6.20058923363573E-30,-0.823067492614537)) ;
#120549=DIRECTION('center_axis',(-1.31418445149758E-16,1.,0.)) ;
#120550=DIRECTION('ref_axis',(-1.,-1.31418445149758E-16,0.)) ;
#120551=DIRECTION('center_axis',(-0.823067492614537,0.,0.567943573430688)) ;
#120552=DIRECTION('ref_axis',(0.567943573430688,0.,0.823067492614537)) ;
#120553=DIRECTION('center_axis',(7.81406971160724E-17,-1.,0.)) ;
#120554=DIRECTION('ref_axis',(1.,0.,0.)) ;
#120555=DIRECTION('center_axis',(7.81406971160724E-17,-1.,0.)) ;
#120556=DIRECTION('ref_axis',(1.,7.81406971160724E-17,0.)) ;
#120557=DIRECTION('center_axis',(-7.81406971160724E-17,1.,0.)) ;
#120558=DIRECTION('ref_axis',(1.,7.81406971160724E-17,-1.5419764230905E-15)) ;
#120559=DIRECTION('center_axis',(-1.31418445149758E-16,1.,0.)) ;
#120560=DIRECTION('ref_axis',(-1.,0.,0.)) ;
#120561=DIRECTION('center_axis',(1.31418445149758E-16,-1.,0.)) ;
#120562=DIRECTION('ref_axis',(-1.,-1.31418445149758E-16,0.)) ;
#120563=DIRECTION('center_axis',(0.823067492614531,3.56948625437948E-15,
0.567943573430696)) ;
#120564=DIRECTION('ref_axis',(0.567943573430696,-1.85164162127997E-29,-0.823067492614531)) ;
#120565=DIRECTION('center_axis',(-1.31418445149758E-16,1.,0.)) ;
#120566=DIRECTION('ref_axis',(-1.,-1.31418445149758E-16,0.)) ;
#120567=DIRECTION('center_axis',(-0.823067492614531,-5.35422938156922E-15,
0.567943573430696)) ;
#120568=DIRECTION('ref_axis',(0.567943573430696,-2.86909128817562E-29,0.823067492614531)) ;
#120569=DIRECTION('center_axis',(7.81406971160724E-17,-1.,0.)) ;
#120570=DIRECTION('ref_axis',(1.,0.,0.)) ;
#120571=DIRECTION('center_axis',(7.81406971160724E-17,-1.,0.)) ;
#120572=DIRECTION('ref_axis',(1.,7.81406971160724E-17,0.)) ;
#120573=DIRECTION('center_axis',(-7.81406971160724E-17,1.,0.)) ;
#120574=DIRECTION('ref_axis',(1.,7.81406971160724E-17,-1.5419764230905E-15)) ;
#120575=DIRECTION('center_axis',(-1.31418445149758E-16,1.,0.)) ;
#120576=DIRECTION('ref_axis',(-1.,0.,0.)) ;
#120577=DIRECTION('center_axis',(1.31418445149758E-16,-1.,0.)) ;
#120578=DIRECTION('ref_axis',(-1.,-1.31418445149758E-16,0.)) ;
#120579=DIRECTION('center_axis',(0.823067492614531,3.56948625437948E-15,
0.567943573430696)) ;
#120580=DIRECTION('ref_axis',(0.567943573430696,-1.85164162127997E-29,-0.823067492614531)) ;
#120581=DIRECTION('center_axis',(-1.31418445149758E-16,1.,0.)) ;
#120582=DIRECTION('ref_axis',(-1.,-1.31418445149758E-16,0.)) ;
#120583=DIRECTION('center_axis',(-0.823067492614531,-5.35422938156922E-15,
0.567943573430696)) ;
#120584=DIRECTION('ref_axis',(0.567943573430696,-2.86909128817562E-29,0.823067492614531)) ;
#120585=DIRECTION('center_axis',(7.81406971160724E-17,-1.,0.)) ;
#120586=DIRECTION('ref_axis',(1.,0.,0.)) ;
#120587=DIRECTION('center_axis',(7.81406971160724E-17,-1.,0.)) ;
#120588=DIRECTION('ref_axis',(1.,7.81406971160724E-17,0.)) ;
#120589=DIRECTION('center_axis',(-7.81406971160724E-17,1.,0.)) ;
#120590=DIRECTION('ref_axis',(1.,7.81406971160724E-17,-1.5419764230905E-15)) ;
#120591=DIRECTION('center_axis',(-1.31418445149758E-16,1.,0.)) ;
#120592=DIRECTION('ref_axis',(-1.,0.,0.)) ;
#120593=DIRECTION('center_axis',(1.31418445149758E-16,-1.,0.)) ;
#120594=DIRECTION('ref_axis',(-1.,-1.31418445149758E-16,0.)) ;
#120595=DIRECTION('center_axis',(0.823067492614531,3.56948625437948E-15,
0.567943573430696)) ;
#120596=DIRECTION('ref_axis',(0.567943573430696,-1.85164162127997E-29,-0.823067492614531)) ;
#120597=DIRECTION('center_axis',(-1.31418445149758E-16,1.,0.)) ;
#120598=DIRECTION('ref_axis',(-1.,-1.31418445149758E-16,0.)) ;
#120599=DIRECTION('center_axis',(-0.823067492614531,-5.35422938156922E-15,
0.567943573430696)) ;
#120600=DIRECTION('ref_axis',(0.567943573430696,-2.86909128817562E-29,0.823067492614531)) ;
#120601=DIRECTION('center_axis',(7.81406971160724E-17,-1.,0.)) ;
#120602=DIRECTION('ref_axis',(1.,0.,0.)) ;
#120603=DIRECTION('center_axis',(7.81406971160724E-17,-1.,0.)) ;
#120604=DIRECTION('ref_axis',(1.,7.81406971160724E-17,0.)) ;
#120605=DIRECTION('center_axis',(-7.81406971160724E-17,1.,0.)) ;
#120606=DIRECTION('ref_axis',(1.,7.81406971160724E-17,-1.5419764230905E-15)) ;
#120607=DIRECTION('center_axis',(-1.31418445149758E-16,1.,0.)) ;
#120608=DIRECTION('ref_axis',(-1.,0.,0.)) ;
#120609=DIRECTION('center_axis',(1.31418445149758E-16,-1.,0.)) ;
#120610=DIRECTION('ref_axis',(-1.,-1.31418445149758E-16,0.)) ;
#120611=DIRECTION('center_axis',(0.823067492614531,3.56948625437948E-15,
0.567943573430696)) ;
#120612=DIRECTION('ref_axis',(0.567943573430696,-1.85164162127997E-29,-0.823067492614531)) ;
#120613=DIRECTION('center_axis',(-1.31418445149758E-16,1.,0.)) ;
#120614=DIRECTION('ref_axis',(-1.,-1.31418445149758E-16,0.)) ;
#120615=DIRECTION('center_axis',(-0.823067492614531,0.,0.567943573430696)) ;
#120616=DIRECTION('ref_axis',(0.567943573430696,0.,0.823067492614531)) ;
#120617=DIRECTION('center_axis',(7.81406971160724E-17,-1.,0.)) ;
#120618=DIRECTION('ref_axis',(1.,0.,0.)) ;
#120619=DIRECTION('center_axis',(7.81406971160724E-17,-1.,0.)) ;
#120620=DIRECTION('ref_axis',(1.,7.81406971160724E-17,0.)) ;
#120621=DIRECTION('center_axis',(-7.81406971160724E-17,1.,0.)) ;
#120622=DIRECTION('ref_axis',(1.,7.81406971160724E-17,-1.5419764230905E-15)) ;
#120623=DIRECTION('center_axis',(-1.31418445149758E-16,1.,0.)) ;
#120624=DIRECTION('ref_axis',(-1.,0.,0.)) ;
#120625=DIRECTION('center_axis',(1.31418445149758E-16,-1.,0.)) ;
#120626=DIRECTION('ref_axis',(-1.,-1.31418445149758E-16,0.)) ;
#120627=DIRECTION('center_axis',(0.823067492614489,5.35422938156894E-15,
0.567943573430758)) ;
#120628=DIRECTION('ref_axis',(0.567943573430758,1.07515500753245E-30,-0.823067492614489)) ;
#120629=DIRECTION('center_axis',(-1.31418445149758E-16,1.,0.)) ;
#120630=DIRECTION('ref_axis',(-1.,-1.31418445149758E-16,0.)) ;
#120631=DIRECTION('center_axis',(-0.823067492614541,1.24932018903283E-14,
0.567943573430683)) ;
#120632=DIRECTION('ref_axis',(0.567943573430683,-1.12678102635321E-28,0.823067492614541)) ;
#120633=DIRECTION('center_axis',(7.81406971160724E-17,-1.,0.)) ;
#120634=DIRECTION('ref_axis',(1.,0.,0.)) ;
#120635=DIRECTION('center_axis',(7.81406971160724E-17,-1.,0.)) ;
#120636=DIRECTION('ref_axis',(1.,7.81406971160724E-17,0.)) ;
#120637=DIRECTION('center_axis',(-7.81406971160724E-17,1.,0.)) ;
#120638=DIRECTION('ref_axis',(1.,7.81406971160724E-17,4.62592926927148E-15)) ;
#120639=DIRECTION('center_axis',(-1.31418445149758E-16,1.,0.)) ;
#120640=DIRECTION('ref_axis',(-1.,0.,0.)) ;
#120641=DIRECTION('center_axis',(1.31418445149758E-16,-1.,0.)) ;
#120642=DIRECTION('ref_axis',(-1.,-1.31418445149758E-16,0.)) ;
#120643=DIRECTION('center_axis',(0.641814420963294,9.74199225357299E-15,
0.766859993117096)) ;
#120644=DIRECTION('ref_axis',(0.766859993117096,-8.05387548571638E-29,-0.641814420963294)) ;
#120645=DIRECTION('center_axis',(-1.31418445149758E-16,1.,0.)) ;
#120646=DIRECTION('ref_axis',(-1.,-1.31418445149758E-16,0.)) ;
#120647=DIRECTION('center_axis',(-1.,0.,0.)) ;
#120648=DIRECTION('ref_axis',(0.,0.,1.)) ;
#120649=DIRECTION('center_axis',(7.81406971160724E-17,-1.,0.)) ;
#120650=DIRECTION('ref_axis',(1.,0.,0.)) ;
#120651=DIRECTION('center_axis',(7.81406971160724E-17,-1.,0.)) ;
#120652=DIRECTION('ref_axis',(1.,7.81406971160724E-17,0.)) ;
#120653=DIRECTION('center_axis',(-7.81406971160724E-17,1.,0.)) ;
#120654=DIRECTION('ref_axis',(1.,7.81406971160724E-17,-3.08395284618099E-15)) ;
#120655=DIRECTION('center_axis',(1.31418445149758E-16,1.,0.)) ;
#120656=DIRECTION('ref_axis',(-1.,1.31418445149758E-16,0.)) ;
#120657=DIRECTION('center_axis',(0.,-1.,0.)) ;
#120658=DIRECTION('ref_axis',(0.,0.,-1.)) ;
#120659=DIRECTION('',(1.31418445149758E-16,1.,0.)) ;
#120660=DIRECTION('',(1.31418445149758E-16,1.,0.)) ;
#120661=DIRECTION('center_axis',(1.31418445149758E-16,1.,0.)) ;
#120662=DIRECTION('ref_axis',(-1.,1.31418445149758E-16,0.)) ;
#120663=DIRECTION('center_axis',(0.,-1.,0.)) ;
#120664=DIRECTION('ref_axis',(0.,0.,-1.)) ;
#120665=DIRECTION('',(1.31418445149758E-16,1.,0.)) ;
#120666=DIRECTION('',(1.31418445149758E-16,1.,0.)) ;
#120667=DIRECTION('center_axis',(1.31418445149758E-16,1.,0.)) ;
#120668=DIRECTION('ref_axis',(-1.,1.31418445149758E-16,0.)) ;
#120669=DIRECTION('center_axis',(0.,-1.,0.)) ;
#120670=DIRECTION('ref_axis',(0.,0.,-1.)) ;
#120671=DIRECTION('',(1.31418445149758E-16,1.,0.)) ;
#120672=DIRECTION('',(1.31418445149758E-16,1.,0.)) ;
#120673=DIRECTION('center_axis',(1.31418445149758E-16,1.,0.)) ;
#120674=DIRECTION('ref_axis',(-1.,1.31418445149758E-16,0.)) ;
#120675=DIRECTION('center_axis',(0.,-1.,0.)) ;
#120676=DIRECTION('ref_axis',(0.,0.,-1.)) ;
#120677=DIRECTION('',(1.31418445149758E-16,1.,0.)) ;
#120678=DIRECTION('',(1.31418445149758E-16,1.,0.)) ;
#120679=DIRECTION('center_axis',(1.31418445149758E-16,1.,0.)) ;
#120680=DIRECTION('ref_axis',(-1.,1.31418445149758E-16,0.)) ;
#120681=DIRECTION('center_axis',(1.18364427747299E-14,-1.,8.16753384930027E-15)) ;
#120682=DIRECTION('ref_axis',(1.,1.18364427747299E-14,1.31368283683801E-29)) ;
#120683=DIRECTION('',(1.31418445149758E-16,1.,0.)) ;
#120684=DIRECTION('',(1.31418445149758E-16,1.,0.)) ;
#120685=DIRECTION('center_axis',(1.31418445149758E-16,1.,0.)) ;
#120686=DIRECTION('ref_axis',(-1.,1.31418445149758E-16,0.)) ;
#120687=DIRECTION('center_axis',(-1.18364427747301E-14,-1.,-8.16753384930045E-15)) ;
#120688=DIRECTION('ref_axis',(1.,-1.18364427747301E-14,1.31368283683791E-29)) ;
#120689=DIRECTION('',(1.31418445149758E-16,1.,0.)) ;
#120690=DIRECTION('',(1.31418445149758E-16,1.,0.)) ;
#120691=DIRECTION('center_axis',(1.31418445149758E-16,1.,0.)) ;
#120692=DIRECTION('ref_axis',(-1.,1.31418445149758E-16,0.)) ;
#120693=DIRECTION('center_axis',(0.,-1.,0.)) ;
#120694=DIRECTION('ref_axis',(0.,0.,-1.)) ;
#120695=DIRECTION('',(1.31418445149758E-16,1.,0.)) ;
#120696=DIRECTION('',(1.31418445149758E-16,1.,0.)) ;
#120697=DIRECTION('center_axis',(1.,0.,0.)) ;
#120698=DIRECTION('ref_axis',(0.,0.,-1.)) ;
#120699=DIRECTION('center_axis',(1.,0.,0.)) ;
#120700=DIRECTION('ref_axis',(0.,0.,-1.)) ;
#120701=DIRECTION('center_axis',(0.,1.,1.22464679914736E-16)) ;
#120702=DIRECTION('ref_axis',(0.,-1.22464679914736E-16,1.)) ;
#120703=DIRECTION('center_axis',(-1.,0.,0.)) ;
#120704=DIRECTION('ref_axis',(0.,0.,-1.)) ;
#120705=DIRECTION('center_axis',(-1.31418445149758E-16,1.,0.)) ;
#120706=DIRECTION('ref_axis',(-1.,0.,0.)) ;
#120707=DIRECTION('center_axis',(-1.31418445149758E-16,1.,0.)) ;
#120708=DIRECTION('ref_axis',(-1.,-1.31418445149758E-16,0.)) ;
#120709=DIRECTION('center_axis',(0.,0.,-1.)) ;
#120710=DIRECTION('ref_axis',(1.,0.,0.)) ;
#120711=DIRECTION('center_axis',(1.31418445149758E-16,-1.,0.)) ;
#120712=DIRECTION('ref_axis',(-1.,-1.31418445149758E-16,0.)) ;
#120713=DIRECTION('center_axis',(1.,0.,0.)) ;
#120714=DIRECTION('ref_axis',(0.,0.,-1.)) ;
#120715=DIRECTION('center_axis',(1.,0.,0.)) ;
#120716=DIRECTION('ref_axis',(0.,0.,-1.)) ;
#120717=DIRECTION('center_axis',(0.,-1.,-1.22464679914735E-16)) ;
#120718=DIRECTION('ref_axis',(0.,-1.22464679914735E-16,1.)) ;
#120719=DIRECTION('center_axis',(-1.,0.,0.)) ;
#120720=DIRECTION('ref_axis',(0.,0.,-1.)) ;
#120721=DIRECTION('center_axis',(1.,0.,0.)) ;
#120722=DIRECTION('ref_axis',(0.,0.,-1.)) ;
#120723=DIRECTION('center_axis',(1.,0.,0.)) ;
#120724=DIRECTION('ref_axis',(0.,0.,-1.)) ;
#120725=DIRECTION('center_axis',(0.,1.,1.22464679914735E-16)) ;
#120726=DIRECTION('ref_axis',(0.,-1.22464679914735E-16,1.)) ;
#120727=DIRECTION('center_axis',(-1.,0.,0.)) ;
#120728=DIRECTION('ref_axis',(0.,0.,-1.)) ;
#120729=DIRECTION('center_axis',(-1.31418445149758E-16,1.,0.)) ;
#120730=DIRECTION('ref_axis',(-1.,0.,0.)) ;
#120731=DIRECTION('center_axis',(-1.31418445149758E-16,1.,0.)) ;
#120732=DIRECTION('ref_axis',(-1.,-1.31418445149758E-16,0.)) ;
#120733=DIRECTION('center_axis',(0.,0.,-1.)) ;
#120734=DIRECTION('ref_axis',(1.,0.,0.)) ;
#120735=DIRECTION('center_axis',(1.31418445149758E-16,-1.,0.)) ;
#120736=DIRECTION('ref_axis',(-1.,-1.31418445149758E-16,0.)) ;
#120737=DIRECTION('center_axis',(1.,0.,0.)) ;
#120738=DIRECTION('ref_axis',(0.,0.,-1.)) ;
#120739=DIRECTION('center_axis',(1.,0.,0.)) ;
#120740=DIRECTION('ref_axis',(0.,0.,-1.)) ;
#120741=DIRECTION('center_axis',(0.,-1.,-1.22464679914735E-16)) ;
#120742=DIRECTION('ref_axis',(0.,-1.22464679914735E-16,1.)) ;
#120743=DIRECTION('center_axis',(-1.,0.,0.)) ;
#120744=DIRECTION('ref_axis',(0.,0.,-1.)) ;
#120745=DIRECTION('center_axis',(1.,0.,0.)) ;
#120746=DIRECTION('ref_axis',(0.,0.,-1.)) ;
#120747=DIRECTION('center_axis',(1.,0.,0.)) ;
#120748=DIRECTION('ref_axis',(0.,0.,-1.)) ;
#120749=DIRECTION('center_axis',(0.,1.,1.22464679914735E-16)) ;
#120750=DIRECTION('ref_axis',(0.,-1.22464679914735E-16,1.)) ;
#120751=DIRECTION('center_axis',(-1.,0.,0.)) ;
#120752=DIRECTION('ref_axis',(0.,0.,-1.)) ;
#120753=DIRECTION('center_axis',(-1.31418445149758E-16,1.,0.)) ;
#120754=DIRECTION('ref_axis',(-1.,0.,0.)) ;
#120755=DIRECTION('center_axis',(-1.31418445149758E-16,1.,0.)) ;
#120756=DIRECTION('ref_axis',(-1.,-1.31418445149758E-16,0.)) ;
#120757=DIRECTION('center_axis',(0.,0.,-1.)) ;
#120758=DIRECTION('ref_axis',(1.,0.,0.)) ;
#120759=DIRECTION('center_axis',(1.31418445149758E-16,-1.,0.)) ;
#120760=DIRECTION('ref_axis',(-1.,-1.31418445149758E-16,0.)) ;
#120761=DIRECTION('center_axis',(1.,0.,0.)) ;
#120762=DIRECTION('ref_axis',(0.,0.,-1.)) ;
#120763=DIRECTION('center_axis',(1.,0.,0.)) ;
#120764=DIRECTION('ref_axis',(0.,0.,-1.)) ;
#120765=DIRECTION('center_axis',(0.,-1.,-1.22464679914735E-16)) ;
#120766=DIRECTION('ref_axis',(0.,-1.22464679914735E-16,1.)) ;
#120767=DIRECTION('center_axis',(-1.,0.,0.)) ;
#120768=DIRECTION('ref_axis',(0.,0.,-1.)) ;
#120769=DIRECTION('center_axis',(1.,0.,0.)) ;
#120770=DIRECTION('ref_axis',(0.,0.,-1.)) ;
#120771=DIRECTION('center_axis',(1.,0.,0.)) ;
#120772=DIRECTION('ref_axis',(0.,0.,-1.)) ;
#120773=DIRECTION('center_axis',(0.,1.,1.22464679914735E-16)) ;
#120774=DIRECTION('ref_axis',(0.,-1.22464679914735E-16,1.)) ;
#120775=DIRECTION('center_axis',(-1.,0.,0.)) ;
#120776=DIRECTION('ref_axis',(0.,0.,-1.)) ;
#120777=DIRECTION('center_axis',(-1.31418445149758E-16,1.,0.)) ;
#120778=DIRECTION('ref_axis',(-1.,0.,0.)) ;
#120779=DIRECTION('center_axis',(-1.31418445149758E-16,1.,0.)) ;
#120780=DIRECTION('ref_axis',(-1.,-1.31418445149758E-16,0.)) ;
#120781=DIRECTION('center_axis',(0.,0.,-1.)) ;
#120782=DIRECTION('ref_axis',(1.,0.,0.)) ;
#120783=DIRECTION('center_axis',(1.31418445149758E-16,-1.,0.)) ;
#120784=DIRECTION('ref_axis',(-1.,-1.31418445149758E-16,0.)) ;
#120785=DIRECTION('center_axis',(1.,0.,0.)) ;
#120786=DIRECTION('ref_axis',(0.,0.,-1.)) ;
#120787=DIRECTION('center_axis',(1.,0.,0.)) ;
#120788=DIRECTION('ref_axis',(0.,0.,-1.)) ;
#120789=DIRECTION('center_axis',(0.,-1.,-1.22464679914735E-16)) ;
#120790=DIRECTION('ref_axis',(0.,-1.22464679914735E-16,1.)) ;
#120791=DIRECTION('center_axis',(-1.,0.,0.)) ;
#120792=DIRECTION('ref_axis',(0.,0.,-1.)) ;
#120793=DIRECTION('center_axis',(1.,0.,0.)) ;
#120794=DIRECTION('ref_axis',(0.,0.,-1.)) ;
#120795=DIRECTION('center_axis',(1.,0.,0.)) ;
#120796=DIRECTION('ref_axis',(0.,0.,-1.)) ;
#120797=DIRECTION('center_axis',(0.,1.,1.22464679914735E-16)) ;
#120798=DIRECTION('ref_axis',(0.,-1.22464679914735E-16,1.)) ;
#120799=DIRECTION('center_axis',(-1.,0.,0.)) ;
#120800=DIRECTION('ref_axis',(0.,0.,-1.)) ;
#120801=DIRECTION('center_axis',(-1.31418445149758E-16,1.,0.)) ;
#120802=DIRECTION('ref_axis',(-1.,0.,0.)) ;
#120803=DIRECTION('center_axis',(-1.31418445149758E-16,1.,0.)) ;
#120804=DIRECTION('ref_axis',(-1.,-1.31418445149758E-16,0.)) ;
#120805=DIRECTION('center_axis',(0.,0.,-1.)) ;
#120806=DIRECTION('ref_axis',(1.,0.,0.)) ;
#120807=DIRECTION('center_axis',(1.31418445149758E-16,-1.,0.)) ;
#120808=DIRECTION('ref_axis',(-1.,-1.31418445149758E-16,0.)) ;
#120809=DIRECTION('center_axis',(1.,0.,0.)) ;
#120810=DIRECTION('ref_axis',(0.,0.,-1.)) ;
#120811=DIRECTION('center_axis',(1.,0.,0.)) ;
#120812=DIRECTION('ref_axis',(0.,0.,-1.)) ;
#120813=DIRECTION('center_axis',(0.,-1.,-1.22464679914735E-16)) ;
#120814=DIRECTION('ref_axis',(0.,-1.22464679914735E-16,1.)) ;
#120815=DIRECTION('center_axis',(-1.,0.,0.)) ;
#120816=DIRECTION('ref_axis',(0.,0.,-1.)) ;
#120817=DIRECTION('center_axis',(1.,0.,0.)) ;
#120818=DIRECTION('ref_axis',(0.,0.,-1.)) ;
#120819=DIRECTION('center_axis',(1.,0.,0.)) ;
#120820=DIRECTION('ref_axis',(0.,0.,-1.)) ;
#120821=DIRECTION('center_axis',(0.,1.,1.22464679914735E-16)) ;
#120822=DIRECTION('ref_axis',(0.,-1.22464679914735E-16,1.)) ;
#120823=DIRECTION('center_axis',(-1.,0.,0.)) ;
#120824=DIRECTION('ref_axis',(0.,0.,-1.)) ;
#120825=DIRECTION('center_axis',(-1.31418445149758E-16,1.,0.)) ;
#120826=DIRECTION('ref_axis',(-1.,0.,0.)) ;
#120827=DIRECTION('center_axis',(-1.31418445149758E-16,1.,0.)) ;
#120828=DIRECTION('ref_axis',(-1.,-1.31418445149758E-16,0.)) ;
#120829=DIRECTION('center_axis',(0.,0.,-1.)) ;
#120830=DIRECTION('ref_axis',(1.,0.,0.)) ;
#120831=DIRECTION('center_axis',(1.31418445149758E-16,-1.,0.)) ;
#120832=DIRECTION('ref_axis',(-1.,-1.31418445149758E-16,0.)) ;
#120833=DIRECTION('center_axis',(1.,0.,0.)) ;
#120834=DIRECTION('ref_axis',(0.,0.,-1.)) ;
#120835=DIRECTION('center_axis',(1.,0.,0.)) ;
#120836=DIRECTION('ref_axis',(0.,0.,-1.)) ;
#120837=DIRECTION('center_axis',(0.,-1.,-1.22464679914735E-16)) ;
#120838=DIRECTION('ref_axis',(0.,-1.22464679914735E-16,1.)) ;
#120839=DIRECTION('center_axis',(-1.,0.,0.)) ;
#120840=DIRECTION('ref_axis',(0.,0.,-1.)) ;
#120841=DIRECTION('center_axis',(1.,0.,0.)) ;
#120842=DIRECTION('ref_axis',(0.,0.,-1.)) ;
#120843=DIRECTION('center_axis',(1.,0.,0.)) ;
#120844=DIRECTION('ref_axis',(0.,0.,-1.)) ;
#120845=DIRECTION('center_axis',(0.,1.,1.22464679914735E-16)) ;
#120846=DIRECTION('ref_axis',(0.,-1.22464679914735E-16,1.)) ;
#120847=DIRECTION('center_axis',(-1.,0.,0.)) ;
#120848=DIRECTION('ref_axis',(0.,0.,-1.)) ;
#120849=DIRECTION('center_axis',(-1.31418445149758E-16,1.,0.)) ;
#120850=DIRECTION('ref_axis',(-1.,0.,0.)) ;
#120851=DIRECTION('center_axis',(-1.31418445149758E-16,1.,0.)) ;
#120852=DIRECTION('ref_axis',(-1.,-1.31418445149758E-16,0.)) ;
#120853=DIRECTION('center_axis',(0.,0.,-1.)) ;
#120854=DIRECTION('ref_axis',(1.,0.,0.)) ;
#120855=DIRECTION('center_axis',(1.31418445149758E-16,-1.,0.)) ;
#120856=DIRECTION('ref_axis',(-1.,-1.31418445149758E-16,0.)) ;
#120857=DIRECTION('center_axis',(1.,0.,0.)) ;
#120858=DIRECTION('ref_axis',(0.,0.,-1.)) ;
#120859=DIRECTION('center_axis',(1.,0.,0.)) ;
#120860=DIRECTION('ref_axis',(0.,0.,-1.)) ;
#120861=DIRECTION('center_axis',(0.,-1.,-1.22464679914735E-16)) ;
#120862=DIRECTION('ref_axis',(0.,-1.22464679914735E-16,1.)) ;
#120863=DIRECTION('center_axis',(-1.,0.,0.)) ;
#120864=DIRECTION('ref_axis',(0.,0.,-1.)) ;
#120865=DIRECTION('center_axis',(1.,0.,0.)) ;
#120866=DIRECTION('ref_axis',(0.,0.,-1.)) ;
#120867=DIRECTION('center_axis',(1.,0.,0.)) ;
#120868=DIRECTION('ref_axis',(0.,0.,-1.)) ;
#120869=DIRECTION('center_axis',(0.,1.,1.22464679914735E-16)) ;
#120870=DIRECTION('ref_axis',(0.,-1.22464679914735E-16,1.)) ;
#120871=DIRECTION('center_axis',(-1.,0.,0.)) ;
#120872=DIRECTION('ref_axis',(0.,0.,-1.)) ;
#120873=DIRECTION('center_axis',(-1.31418445149758E-16,1.,0.)) ;
#120874=DIRECTION('ref_axis',(-1.,0.,0.)) ;
#120875=DIRECTION('center_axis',(-1.31418445149758E-16,1.,0.)) ;
#120876=DIRECTION('ref_axis',(-1.,-1.31418445149758E-16,0.)) ;
#120877=DIRECTION('center_axis',(0.,0.,-1.)) ;
#120878=DIRECTION('ref_axis',(1.,0.,0.)) ;
#120879=DIRECTION('center_axis',(1.31418445149758E-16,-1.,0.)) ;
#120880=DIRECTION('ref_axis',(-1.,-1.31418445149758E-16,0.)) ;
#120881=DIRECTION('center_axis',(1.,0.,0.)) ;
#120882=DIRECTION('ref_axis',(0.,0.,-1.)) ;
#120883=DIRECTION('center_axis',(1.,0.,0.)) ;
#120884=DIRECTION('ref_axis',(0.,0.,-1.)) ;
#120885=DIRECTION('center_axis',(0.,-1.,-1.22464679914735E-16)) ;
#120886=DIRECTION('ref_axis',(0.,-1.22464679914735E-16,1.)) ;
#120887=DIRECTION('center_axis',(-1.,0.,0.)) ;
#120888=DIRECTION('ref_axis',(0.,0.,-1.)) ;
#120889=DIRECTION('center_axis',(1.,0.,0.)) ;
#120890=DIRECTION('ref_axis',(0.,0.,-1.)) ;
#120891=DIRECTION('center_axis',(1.,0.,0.)) ;
#120892=DIRECTION('ref_axis',(0.,0.,-1.)) ;
#120893=DIRECTION('center_axis',(0.,1.,1.22464679914735E-16)) ;
#120894=DIRECTION('ref_axis',(0.,-1.22464679914735E-16,1.)) ;
#120895=DIRECTION('center_axis',(-1.,0.,0.)) ;
#120896=DIRECTION('ref_axis',(0.,0.,-1.)) ;
#120897=DIRECTION('center_axis',(-1.31418445149758E-16,1.,0.)) ;
#120898=DIRECTION('ref_axis',(-1.,0.,0.)) ;
#120899=DIRECTION('center_axis',(-1.31418445149758E-16,1.,0.)) ;
#120900=DIRECTION('ref_axis',(-1.,-1.31418445149758E-16,0.)) ;
#120901=DIRECTION('center_axis',(0.,0.,-1.)) ;
#120902=DIRECTION('ref_axis',(1.,0.,0.)) ;
#120903=DIRECTION('center_axis',(1.31418445149758E-16,-1.,0.)) ;
#120904=DIRECTION('ref_axis',(-1.,-1.31418445149758E-16,0.)) ;
#120905=DIRECTION('center_axis',(1.,0.,0.)) ;
#120906=DIRECTION('ref_axis',(0.,0.,-1.)) ;
#120907=DIRECTION('center_axis',(1.,0.,0.)) ;
#120908=DIRECTION('ref_axis',(0.,0.,-1.)) ;
#120909=DIRECTION('center_axis',(0.,-1.,-1.22464679914735E-16)) ;
#120910=DIRECTION('ref_axis',(0.,-1.22464679914735E-16,1.)) ;
#120911=DIRECTION('center_axis',(-1.,0.,0.)) ;
#120912=DIRECTION('ref_axis',(0.,0.,-1.)) ;
#120913=DIRECTION('center_axis',(1.31418445149758E-16,1.,0.)) ;
#120914=DIRECTION('ref_axis',(-1.,1.31418445149758E-16,0.)) ;
#120915=DIRECTION('center_axis',(1.31418445149758E-16,1.,0.)) ;
#120916=DIRECTION('ref_axis',(-1.,1.31418445149758E-16,0.)) ;
#120917=DIRECTION('',(1.31418445149758E-16,1.,0.)) ;
#120918=DIRECTION('center_axis',(1.31418445149758E-16,1.,0.)) ;
#120919=DIRECTION('ref_axis',(-1.,1.31418445149758E-16,0.)) ;
#120920=DIRECTION('',(1.31418445149758E-16,1.,0.)) ;
#120921=DIRECTION('center_axis',(1.31418445149758E-16,1.,0.)) ;
#120922=DIRECTION('ref_axis',(-1.,1.31418445149758E-16,0.)) ;
#120923=DIRECTION('',(1.31418445149758E-16,1.,0.)) ;
#120924=DIRECTION('center_axis',(1.31418445149758E-16,1.,0.)) ;
#120925=DIRECTION('ref_axis',(-1.,1.31418445149758E-16,0.)) ;
#120926=DIRECTION('',(1.31418445149758E-16,1.,0.)) ;
#120927=DIRECTION('center_axis',(1.31418445149758E-16,1.,0.)) ;
#120928=DIRECTION('ref_axis',(-1.,1.31418445149758E-16,0.)) ;
#120929=DIRECTION('',(1.31418445149758E-16,1.,0.)) ;
#120930=DIRECTION('center_axis',(1.31418445149758E-16,1.,0.)) ;
#120931=DIRECTION('ref_axis',(-1.,1.31418445149758E-16,0.)) ;
#120932=DIRECTION('center_axis',(1.31418445149758E-16,1.,0.)) ;
#120933=DIRECTION('ref_axis',(-1.,1.31418445149758E-16,0.)) ;
#120934=DIRECTION('',(1.31418445149758E-16,1.,0.)) ;
#120935=DIRECTION('center_axis',(1.31418445149758E-16,1.,0.)) ;
#120936=DIRECTION('ref_axis',(-1.,1.31418445149758E-16,0.)) ;
#120937=DIRECTION('',(1.31418445149758E-16,1.,0.)) ;
#120938=DIRECTION('center_axis',(1.31418445149758E-16,1.,0.)) ;
#120939=DIRECTION('ref_axis',(-1.,1.31418445149758E-16,0.)) ;
#120940=DIRECTION('',(1.31418445149758E-16,1.,0.)) ;
#120941=DIRECTION('center_axis',(1.31418445149758E-16,1.,0.)) ;
#120942=DIRECTION('ref_axis',(-1.,1.31418445149758E-16,0.)) ;
#120943=DIRECTION('',(1.31418445149758E-16,1.,0.)) ;
#120944=DIRECTION('center_axis',(1.31418445149758E-16,1.,0.)) ;
#120945=DIRECTION('ref_axis',(-1.,1.31418445149758E-16,0.)) ;
#120946=DIRECTION('',(1.31418445149758E-16,1.,0.)) ;
#120947=DIRECTION('center_axis',(1.31418445149758E-16,1.,0.)) ;
#120948=DIRECTION('ref_axis',(-1.,1.31418445149758E-16,0.)) ;
#120949=DIRECTION('center_axis',(1.31418445149758E-16,1.,0.)) ;
#120950=DIRECTION('ref_axis',(-1.,1.31418445149758E-16,0.)) ;
#120951=DIRECTION('',(1.31418445149758E-16,1.,0.)) ;
#120952=DIRECTION('center_axis',(1.31418445149758E-16,1.,0.)) ;
#120953=DIRECTION('ref_axis',(-1.,1.31418445149758E-16,0.)) ;
#120954=DIRECTION('',(1.31418445149758E-16,1.,0.)) ;
#120955=DIRECTION('center_axis',(1.31418445149758E-16,1.,0.)) ;
#120956=DIRECTION('ref_axis',(-1.,1.31418445149758E-16,0.)) ;
#120957=DIRECTION('',(1.31418445149758E-16,1.,0.)) ;
#120958=DIRECTION('center_axis',(1.31418445149758E-16,1.,0.)) ;
#120959=DIRECTION('ref_axis',(-1.,1.31418445149758E-16,0.)) ;
#120960=DIRECTION('',(1.31418445149758E-16,1.,0.)) ;
#120961=DIRECTION('center_axis',(1.31418445149758E-16,1.,0.)) ;
#120962=DIRECTION('ref_axis',(-1.,1.31418445149758E-16,0.)) ;
#120963=DIRECTION('',(1.31418445149758E-16,1.,0.)) ;
#120964=DIRECTION('center_axis',(1.31418445149758E-16,1.,0.)) ;
#120965=DIRECTION('ref_axis',(-1.,1.31418445149758E-16,0.)) ;
#120966=DIRECTION('center_axis',(1.31418445149758E-16,1.,0.)) ;
#120967=DIRECTION('ref_axis',(-1.,1.31418445149758E-16,0.)) ;
#120968=DIRECTION('',(1.31418445149758E-16,1.,0.)) ;
#120969=DIRECTION('center_axis',(1.31418445149758E-16,1.,0.)) ;
#120970=DIRECTION('ref_axis',(-1.,1.31418445149758E-16,0.)) ;
#120971=DIRECTION('',(1.31418445149758E-16,1.,0.)) ;
#120972=DIRECTION('center_axis',(1.31418445149758E-16,1.,0.)) ;
#120973=DIRECTION('ref_axis',(-1.,1.31418445149758E-16,0.)) ;
#120974=DIRECTION('',(1.31418445149758E-16,1.,0.)) ;
#120975=DIRECTION('center_axis',(1.31418445149758E-16,1.,0.)) ;
#120976=DIRECTION('ref_axis',(-1.,1.31418445149758E-16,0.)) ;
#120977=DIRECTION('',(1.31418445149758E-16,1.,0.)) ;
#120978=DIRECTION('center_axis',(1.31418445149758E-16,1.,0.)) ;
#120979=DIRECTION('ref_axis',(-1.,1.31418445149758E-16,0.)) ;
#120980=DIRECTION('',(1.31418445149758E-16,1.,0.)) ;
#120981=DIRECTION('center_axis',(1.31418445149758E-16,1.,0.)) ;
#120982=DIRECTION('ref_axis',(-1.,1.31418445149758E-16,0.)) ;
#120983=DIRECTION('center_axis',(1.31418445149758E-16,1.,0.)) ;
#120984=DIRECTION('ref_axis',(-1.,1.31418445149758E-16,0.)) ;
#120985=DIRECTION('',(1.31418445149758E-16,1.,0.)) ;
#120986=DIRECTION('center_axis',(1.31418445149758E-16,1.,0.)) ;
#120987=DIRECTION('ref_axis',(-1.,1.31418445149758E-16,0.)) ;
#120988=DIRECTION('',(1.31418445149758E-16,1.,0.)) ;
#120989=DIRECTION('center_axis',(1.31418445149758E-16,1.,0.)) ;
#120990=DIRECTION('ref_axis',(-1.,1.31418445149758E-16,0.)) ;
#120991=DIRECTION('',(1.31418445149758E-16,1.,0.)) ;
#120992=DIRECTION('center_axis',(1.31418445149758E-16,1.,0.)) ;
#120993=DIRECTION('ref_axis',(-1.,1.31418445149758E-16,0.)) ;
#120994=DIRECTION('',(1.31418445149758E-16,1.,0.)) ;
#120995=DIRECTION('center_axis',(1.31418445149758E-16,1.,0.)) ;
#120996=DIRECTION('ref_axis',(-1.,1.31418445149758E-16,0.)) ;
#120997=DIRECTION('',(1.31418445149758E-16,1.,0.)) ;
#120998=DIRECTION('center_axis',(1.31418445149758E-16,1.,0.)) ;
#120999=DIRECTION('ref_axis',(-1.,1.31418445149758E-16,0.)) ;
#121000=DIRECTION('center_axis',(1.31418445149758E-16,1.,0.)) ;
#121001=DIRECTION('ref_axis',(-1.,1.31418445149758E-16,0.)) ;
#121002=DIRECTION('',(1.31418445149758E-16,1.,0.)) ;
#121003=DIRECTION('center_axis',(1.31418445149758E-16,1.,0.)) ;
#121004=DIRECTION('ref_axis',(-1.,1.31418445149758E-16,0.)) ;
#121005=DIRECTION('',(1.31418445149758E-16,1.,0.)) ;
#121006=DIRECTION('center_axis',(1.31418445149758E-16,1.,0.)) ;
#121007=DIRECTION('ref_axis',(-1.,1.31418445149758E-16,0.)) ;
#121008=DIRECTION('',(1.31418445149758E-16,1.,0.)) ;
#121009=DIRECTION('center_axis',(1.31418445149758E-16,1.,0.)) ;
#121010=DIRECTION('ref_axis',(-1.,1.31418445149758E-16,0.)) ;
#121011=DIRECTION('',(1.31418445149758E-16,1.,0.)) ;
#121012=DIRECTION('center_axis',(1.31418445149758E-16,1.,0.)) ;
#121013=DIRECTION('ref_axis',(-1.,1.31418445149758E-16,0.)) ;
#121014=DIRECTION('',(1.31418445149758E-16,1.,0.)) ;
#121015=DIRECTION('center_axis',(1.31418445149758E-16,1.,0.)) ;
#121016=DIRECTION('ref_axis',(-1.,1.31418445149758E-16,0.)) ;
#121017=DIRECTION('center_axis',(1.31418445149758E-16,1.,0.)) ;
#121018=DIRECTION('ref_axis',(-1.,1.31418445149758E-16,0.)) ;
#121019=DIRECTION('',(1.31418445149758E-16,1.,0.)) ;
#121020=DIRECTION('center_axis',(1.31418445149758E-16,1.,0.)) ;
#121021=DIRECTION('ref_axis',(-1.,1.31418445149758E-16,0.)) ;
#121022=DIRECTION('',(1.31418445149758E-16,1.,0.)) ;
#121023=DIRECTION('center_axis',(1.31418445149758E-16,1.,0.)) ;
#121024=DIRECTION('ref_axis',(-1.,1.31418445149758E-16,0.)) ;
#121025=DIRECTION('',(1.31418445149758E-16,1.,0.)) ;
#121026=DIRECTION('center_axis',(1.31418445149758E-16,1.,0.)) ;
#121027=DIRECTION('ref_axis',(-1.,1.31418445149758E-16,0.)) ;
#121028=DIRECTION('',(1.31418445149758E-16,1.,0.)) ;
#121029=DIRECTION('center_axis',(1.31418445149758E-16,1.,0.)) ;
#121030=DIRECTION('ref_axis',(-1.,1.31418445149758E-16,0.)) ;
#121031=DIRECTION('',(1.31418445149758E-16,1.,0.)) ;
#121032=DIRECTION('center_axis',(1.31418445149758E-16,1.,0.)) ;
#121033=DIRECTION('ref_axis',(-1.,1.31418445149758E-16,0.)) ;
#121034=DIRECTION('center_axis',(1.31418445149758E-16,1.,0.)) ;
#121035=DIRECTION('ref_axis',(-1.,1.31418445149758E-16,0.)) ;
#121036=DIRECTION('',(1.31418445149758E-16,1.,0.)) ;
#121037=DIRECTION('center_axis',(1.31418445149758E-16,1.,0.)) ;
#121038=DIRECTION('ref_axis',(-1.,1.31418445149758E-16,0.)) ;
#121039=DIRECTION('',(1.31418445149758E-16,1.,0.)) ;
#121040=DIRECTION('center_axis',(1.31418445149758E-16,1.,0.)) ;
#121041=DIRECTION('ref_axis',(-1.,1.31418445149758E-16,0.)) ;
#121042=DIRECTION('',(1.31418445149758E-16,1.,0.)) ;
#121043=DIRECTION('center_axis',(1.31418445149758E-16,1.,0.)) ;
#121044=DIRECTION('ref_axis',(-1.,1.31418445149758E-16,0.)) ;
#121045=DIRECTION('',(1.31418445149758E-16,1.,0.)) ;
#121046=DIRECTION('center_axis',(1.31418445149758E-16,1.,0.)) ;
#121047=DIRECTION('ref_axis',(-1.,1.31418445149758E-16,0.)) ;
#121048=DIRECTION('',(1.31418445149758E-16,1.,0.)) ;
#121049=DIRECTION('center_axis',(1.31418445149758E-16,1.,0.)) ;
#121050=DIRECTION('ref_axis',(-1.,1.31418445149758E-16,0.)) ;
#121051=DIRECTION('center_axis',(1.31418445149758E-16,1.,0.)) ;
#121052=DIRECTION('ref_axis',(-1.,1.31418445149758E-16,0.)) ;
#121053=DIRECTION('',(1.31418445149758E-16,1.,0.)) ;
#121054=DIRECTION('center_axis',(1.31418445149758E-16,1.,0.)) ;
#121055=DIRECTION('ref_axis',(-1.,1.31418445149758E-16,0.)) ;
#121056=DIRECTION('',(1.31418445149758E-16,1.,0.)) ;
#121057=DIRECTION('center_axis',(1.31418445149758E-16,1.,0.)) ;
#121058=DIRECTION('ref_axis',(-1.,1.31418445149758E-16,0.)) ;
#121059=DIRECTION('',(1.31418445149758E-16,1.,0.)) ;
#121060=DIRECTION('center_axis',(1.31418445149758E-16,1.,0.)) ;
#121061=DIRECTION('ref_axis',(-1.,1.31418445149758E-16,0.)) ;
#121062=DIRECTION('',(1.31418445149758E-16,1.,0.)) ;
#121063=DIRECTION('center_axis',(1.31418445149758E-16,1.,0.)) ;
#121064=DIRECTION('ref_axis',(-1.,1.31418445149758E-16,0.)) ;
#121065=DIRECTION('',(1.31418445149758E-16,1.,0.)) ;
#121066=DIRECTION('center_axis',(1.,0.,0.)) ;
#121067=DIRECTION('ref_axis',(0.,0.,-1.)) ;
#121068=DIRECTION('center_axis',(1.,0.,0.)) ;
#121069=DIRECTION('ref_axis',(0.,0.,-1.)) ;
#121070=DIRECTION('',(0.707106781186546,-8.65956056235495E-17,0.707106781186549)) ;
#121071=DIRECTION('center_axis',(1.,0.,0.)) ;
#121072=DIRECTION('ref_axis',(0.,0.,-1.)) ;
#121073=DIRECTION('center_axis',(1.,0.,0.)) ;
#121074=DIRECTION('ref_axis',(0.,0.,-1.)) ;
#121075=DIRECTION('',(0.707106781186546,-8.65956056235495E-17,0.707106781186549)) ;
#121076=DIRECTION('center_axis',(1.,0.,0.)) ;
#121077=DIRECTION('ref_axis',(0.,0.,-1.)) ;
#121078=DIRECTION('center_axis',(1.,0.,0.)) ;
#121079=DIRECTION('ref_axis',(0.,0.,-1.)) ;
#121080=DIRECTION('',(0.707106781186546,-8.65956056235495E-17,0.707106781186549)) ;
#121081=DIRECTION('center_axis',(1.,0.,0.)) ;
#121082=DIRECTION('ref_axis',(0.,0.,-1.)) ;
#121083=DIRECTION('center_axis',(1.,0.,0.)) ;
#121084=DIRECTION('ref_axis',(0.,0.,-1.)) ;
#121085=DIRECTION('',(0.707106781186546,-8.65956056235495E-17,0.707106781186549)) ;
#121086=DIRECTION('center_axis',(1.,0.,0.)) ;
#121087=DIRECTION('ref_axis',(0.,0.,-1.)) ;
#121088=DIRECTION('center_axis',(1.,0.,0.)) ;
#121089=DIRECTION('ref_axis',(0.,0.,-1.)) ;
#121090=DIRECTION('',(0.707106781186546,-8.65956056235495E-17,0.707106781186549)) ;
#121091=DIRECTION('center_axis',(1.,0.,0.)) ;
#121092=DIRECTION('ref_axis',(0.,0.,-1.)) ;
#121093=DIRECTION('center_axis',(1.,0.,0.)) ;
#121094=DIRECTION('ref_axis',(0.,0.,-1.)) ;
#121095=DIRECTION('',(0.707106781186546,-8.65956056235495E-17,0.707106781186549)) ;
#121096=DIRECTION('center_axis',(1.,0.,0.)) ;
#121097=DIRECTION('ref_axis',(0.,0.,-1.)) ;
#121098=DIRECTION('center_axis',(1.,0.,0.)) ;
#121099=DIRECTION('ref_axis',(0.,0.,-1.)) ;
#121100=DIRECTION('',(0.707106781186546,-8.65956056235495E-17,0.707106781186549)) ;
#121101=DIRECTION('center_axis',(1.,0.,0.)) ;
#121102=DIRECTION('ref_axis',(0.,0.,-1.)) ;
#121103=DIRECTION('center_axis',(1.,0.,0.)) ;
#121104=DIRECTION('ref_axis',(0.,0.,-1.)) ;
#121105=DIRECTION('',(0.707106781186546,-8.65956056235495E-17,0.707106781186549)) ;
#121106=DIRECTION('center_axis',(1.,0.,0.)) ;
#121107=DIRECTION('ref_axis',(0.,0.,-1.)) ;
#121108=DIRECTION('center_axis',(1.,0.,0.)) ;
#121109=DIRECTION('ref_axis',(0.,0.,-1.)) ;
#121110=DIRECTION('',(0.707106781186546,-8.65956056235495E-17,0.707106781186549)) ;
#121111=DIRECTION('center_axis',(1.,0.,0.)) ;
#121112=DIRECTION('ref_axis',(0.,0.,-1.)) ;
#121113=DIRECTION('',(1.,0.,0.)) ;
#121114=DIRECTION('center_axis',(1.,0.,0.)) ;
#121115=DIRECTION('ref_axis',(0.,0.,-1.)) ;
#121116=DIRECTION('',(1.,0.,0.)) ;
#121117=DIRECTION('center_axis',(1.,0.,0.)) ;
#121118=DIRECTION('ref_axis',(0.,0.,-1.)) ;
#121119=DIRECTION('',(1.,0.,0.)) ;
#121120=DIRECTION('center_axis',(1.,0.,0.)) ;
#121121=DIRECTION('ref_axis',(0.,0.,-1.)) ;
#121122=DIRECTION('',(1.,0.,0.)) ;
#121123=DIRECTION('center_axis',(1.,0.,0.)) ;
#121124=DIRECTION('ref_axis',(0.,0.,-1.)) ;
#121125=DIRECTION('',(1.,0.,0.)) ;
#121126=DIRECTION('center_axis',(1.,0.,0.)) ;
#121127=DIRECTION('ref_axis',(0.,0.,-1.)) ;
#121128=DIRECTION('',(1.,0.,0.)) ;
#121129=DIRECTION('center_axis',(1.,0.,0.)) ;
#121130=DIRECTION('ref_axis',(0.,0.,-1.)) ;
#121131=DIRECTION('',(1.,0.,0.)) ;
#121132=DIRECTION('center_axis',(1.,0.,0.)) ;
#121133=DIRECTION('ref_axis',(0.,0.,-1.)) ;
#121134=DIRECTION('',(1.,0.,0.)) ;
#121135=DIRECTION('center_axis',(1.,0.,0.)) ;
#121136=DIRECTION('ref_axis',(0.,0.,-1.)) ;
#121137=DIRECTION('',(1.,0.,0.)) ;
#121138=DIRECTION('center_axis',(1.,0.,0.)) ;
#121139=DIRECTION('ref_axis',(0.,0.,-1.)) ;
#121140=DIRECTION('center_axis',(1.,0.,0.)) ;
#121141=DIRECTION('ref_axis',(0.,0.,-1.)) ;
#121142=DIRECTION('center_axis',(0.,1.,1.22464679914735E-16)) ;
#121143=DIRECTION('ref_axis',(0.,-1.22464679914735E-16,1.)) ;
#121144=DIRECTION('center_axis',(-1.,0.,0.)) ;
#121145=DIRECTION('ref_axis',(0.,0.,-1.)) ;
#121146=DIRECTION('center_axis',(-1.31418445149758E-16,1.,0.)) ;
#121147=DIRECTION('ref_axis',(-1.,0.,0.)) ;
#121148=DIRECTION('center_axis',(-1.31418445149758E-16,1.,0.)) ;
#121149=DIRECTION('ref_axis',(-1.,-1.31418445149758E-16,0.)) ;
#121150=DIRECTION('center_axis',(-1.22464679914735E-16,-1.60941178201573E-32,
-1.)) ;
#121151=DIRECTION('ref_axis',(1.,0.,-1.22464679914735E-16)) ;
#121152=DIRECTION('center_axis',(1.31418445149758E-16,-1.,0.)) ;
#121153=DIRECTION('ref_axis',(-1.,-1.31418445149758E-16,0.)) ;
#121154=DIRECTION('center_axis',(1.,0.,0.)) ;
#121155=DIRECTION('ref_axis',(0.,0.,-1.)) ;
#121156=DIRECTION('center_axis',(1.,0.,0.)) ;
#121157=DIRECTION('ref_axis',(0.,0.,-1.)) ;
#121158=DIRECTION('center_axis',(0.,-1.,-1.22464679914735E-16)) ;
#121159=DIRECTION('ref_axis',(0.,-1.22464679914735E-16,1.)) ;
#121160=DIRECTION('center_axis',(-1.,0.,0.)) ;
#121161=DIRECTION('ref_axis',(0.,0.,-1.)) ;
#121162=DIRECTION('center_axis',(-1.31418445149758E-16,1.,0.)) ;
#121163=DIRECTION('ref_axis',(-1.,-1.31418445149758E-16,0.)) ;
#121164=DIRECTION('center_axis',(0.,-1.,0.)) ;
#121165=DIRECTION('ref_axis',(0.,0.,-1.)) ;
#121166=DIRECTION('',(-1.31418445149758E-16,1.,0.)) ;
#121167=DIRECTION('',(-1.31418445149758E-16,1.,0.)) ;
#121168=DIRECTION('center_axis',(-1.31418445149758E-16,1.,0.)) ;
#121169=DIRECTION('ref_axis',(-1.,-1.31418445149758E-16,0.)) ;
#121170=DIRECTION('center_axis',(-5.62625979646468E-15,-1.,-6.72243160618769E-15)) ;
#121171=DIRECTION('ref_axis',(3.86570035924698E-42,6.72243160618769E-15,
-1.)) ;
#121172=DIRECTION('',(-1.31418445149758E-16,1.,0.)) ;
#121173=DIRECTION('',(-1.31418445149758E-16,1.,0.)) ;
#121174=DIRECTION('center_axis',(1.31418445149758E-16,1.,0.)) ;
#121175=DIRECTION('ref_axis',(-1.,1.31418445149758E-16,0.)) ;
#121176=DIRECTION('center_axis',(8.7661785287084E-15,-1.,0.)) ;
#121177=DIRECTION('ref_axis',(1.,8.7661785287084E-15,0.)) ;
#121178=DIRECTION('',(1.31418445149758E-16,1.,0.)) ;
#121179=DIRECTION('',(1.31418445149758E-16,1.,0.)) ;
#121180=DIRECTION('center_axis',(1.31418445149758E-16,1.,0.)) ;
#121181=DIRECTION('ref_axis',(-1.,1.31418445149758E-16,0.)) ;
#121182=DIRECTION('center_axis',(0.,-1.,0.)) ;
#121183=DIRECTION('ref_axis',(0.,0.,-1.)) ;
#121184=DIRECTION('',(1.31418445149758E-16,1.,0.)) ;
#121185=DIRECTION('',(1.31418445149758E-16,1.,0.)) ;
#121186=DIRECTION('center_axis',(1.31418445149758E-16,1.,0.)) ;
#121187=DIRECTION('ref_axis',(-1.,1.31418445149758E-16,0.)) ;
#121188=DIRECTION('center_axis',(1.31418445149758E-16,1.,0.)) ;
#121189=DIRECTION('ref_axis',(-1.,1.31418445149758E-16,0.)) ;
#121190=DIRECTION('',(1.31418445149758E-16,1.,0.)) ;
#121191=DIRECTION('center_axis',(1.31418445149758E-16,1.,0.)) ;
#121192=DIRECTION('ref_axis',(-1.,1.31418445149758E-16,0.)) ;
#121193=DIRECTION('',(1.31418445149758E-16,1.,0.)) ;
#121194=DIRECTION('center_axis',(1.31418445149758E-16,1.,0.)) ;
#121195=DIRECTION('ref_axis',(-1.,1.31418445149758E-16,0.)) ;
#121196=DIRECTION('',(1.31418445149758E-16,1.,0.)) ;
#121197=DIRECTION('center_axis',(1.31418445149758E-16,1.,0.)) ;
#121198=DIRECTION('ref_axis',(-1.,1.31418445149758E-16,0.)) ;
#121199=DIRECTION('',(1.31418445149758E-16,1.,0.)) ;
#121200=DIRECTION('center_axis',(1.31418445149758E-16,1.,0.)) ;
#121201=DIRECTION('ref_axis',(-1.,1.31418445149758E-16,0.)) ;
#121202=DIRECTION('',(1.31418445149758E-16,1.,0.)) ;
#121203=DIRECTION('center_axis',(1.,0.,0.)) ;
#121204=DIRECTION('ref_axis',(0.,0.,-1.)) ;
#121205=DIRECTION('center_axis',(1.,0.,0.)) ;
#121206=DIRECTION('ref_axis',(0.,0.,-1.)) ;
#121207=DIRECTION('',(0.707106781186546,-8.65956056235495E-17,0.707106781186549)) ;
#121208=DIRECTION('center_axis',(1.,0.,0.)) ;
#121209=DIRECTION('ref_axis',(0.,0.,-1.)) ;
#121210=DIRECTION('',(1.,0.,0.)) ;
#121211=DIRECTION('center_axis',(-1.31418445149758E-16,1.,0.)) ;
#121212=DIRECTION('ref_axis',(-1.,-1.31418445149758E-16,0.)) ;
#121213=DIRECTION('',(0.,0.,1.)) ;
#121214=DIRECTION('',(1.,1.31418445149758E-16,0.)) ;
#121215=DIRECTION('',(0.,0.,-1.)) ;
#121216=DIRECTION('',(-1.,-1.31418445149758E-16,-5.2561455487295E-16)) ;
#121217=DIRECTION('center_axis',(-1.31418445149758E-16,1.,0.)) ;
#121218=DIRECTION('ref_axis',(-1.,-1.31418445149758E-16,0.)) ;
#121219=DIRECTION('center_axis',(-1.31418445149758E-16,1.,0.)) ;
#121220=DIRECTION('ref_axis',(-1.,-1.31418445149758E-16,0.)) ;
#121221=DIRECTION('center_axis',(-1.31418445149758E-16,1.,0.)) ;
#121222=DIRECTION('ref_axis',(-1.,-1.31418445149758E-16,0.)) ;
#121223=DIRECTION('center_axis',(-1.31418445149758E-16,1.,0.)) ;
#121224=DIRECTION('ref_axis',(-1.,-1.31418445149758E-16,0.)) ;
#121225=DIRECTION('center_axis',(-1.31418445149758E-16,1.,0.)) ;
#121226=DIRECTION('ref_axis',(-1.,-1.31418445149758E-16,0.)) ;
#121227=DIRECTION('center_axis',(-1.31418445149758E-16,1.,0.)) ;
#121228=DIRECTION('ref_axis',(-1.,-1.31418445149758E-16,0.)) ;
#121229=DIRECTION('center_axis',(-1.31418445149758E-16,1.,0.)) ;
#121230=DIRECTION('ref_axis',(-1.,-1.31418445149758E-16,0.)) ;
#121231=DIRECTION('center_axis',(-1.31418445149758E-16,1.,0.)) ;
#121232=DIRECTION('ref_axis',(-1.,-1.31418445149758E-16,0.)) ;
#121233=DIRECTION('center_axis',(-1.31418445149758E-16,1.,0.)) ;
#121234=DIRECTION('ref_axis',(-1.,-1.31418445149758E-16,0.)) ;
#121235=DIRECTION('center_axis',(-1.31418445149758E-16,1.,0.)) ;
#121236=DIRECTION('ref_axis',(-1.,-1.31418445149758E-16,0.)) ;
#121237=DIRECTION('',(1.,1.31418445149758E-16,0.)) ;
#121238=DIRECTION('',(0.,0.,-1.)) ;
#121239=DIRECTION('',(-1.,-1.31418445149758E-16,0.)) ;
#121240=DIRECTION('center_axis',(-1.31418445149758E-16,1.,0.)) ;
#121241=DIRECTION('ref_axis',(-1.,-1.31418445149758E-16,0.)) ;
#121242=DIRECTION('',(-1.,-1.31418445149758E-16,-2.16840434497101E-16)) ;
#121243=DIRECTION('center_axis',(-1.31418445149758E-16,1.,0.)) ;
#121244=DIRECTION('ref_axis',(-1.,-1.31418445149758E-16,0.)) ;
#121245=DIRECTION('',(-4.33680868994202E-16,-5.69936654944139E-32,-1.)) ;
#121246=DIRECTION('center_axis',(-1.31418445149758E-16,1.,0.)) ;
#121247=DIRECTION('ref_axis',(-1.,-1.31418445149758E-16,0.)) ;
#121248=DIRECTION('',(1.,1.31418445149758E-16,-2.16840434497101E-16)) ;
#121249=DIRECTION('center_axis',(-1.31418445149758E-16,1.,0.)) ;
#121250=DIRECTION('ref_axis',(-1.,-1.31418445149758E-16,0.)) ;
#121251=DIRECTION('',(2.16840434497101E-16,2.8496832747207E-32,1.)) ;
#121252=DIRECTION('center_axis',(-1.31418445149758E-16,1.,0.)) ;
#121253=DIRECTION('ref_axis',(-1.,-1.31418445149758E-16,0.)) ;
#121254=DIRECTION('',(-1.,-1.31418445149758E-16,-2.16840434497101E-16)) ;
#121255=DIRECTION('center_axis',(-1.31418445149758E-16,1.,0.)) ;
#121256=DIRECTION('ref_axis',(-1.,-1.31418445149758E-16,0.)) ;
#121257=DIRECTION('',(-4.33680868994202E-16,-5.69936654944139E-32,-1.)) ;
#121258=DIRECTION('center_axis',(-1.31418445149758E-16,1.,0.)) ;
#121259=DIRECTION('ref_axis',(-1.,-1.31418445149758E-16,0.)) ;
#121260=DIRECTION('',(1.,1.31418445149758E-16,-2.16840434497101E-16)) ;
#121261=DIRECTION('center_axis',(-1.31418445149758E-16,1.,0.)) ;
#121262=DIRECTION('ref_axis',(-1.,-1.31418445149758E-16,0.)) ;
#121263=DIRECTION('',(2.16840434497101E-16,2.8496832747207E-32,1.)) ;
#121264=DIRECTION('center_axis',(-1.31418445149758E-16,1.,0.)) ;
#121265=DIRECTION('ref_axis',(-1.,-1.31418445149758E-16,0.)) ;
#121266=DIRECTION('',(-1.,-1.31418445149758E-16,-2.16840434497101E-16)) ;
#121267=DIRECTION('center_axis',(-1.31418445149758E-16,1.,0.)) ;
#121268=DIRECTION('ref_axis',(-1.,-1.31418445149758E-16,0.)) ;
#121269=DIRECTION('',(-4.33680868994202E-16,-5.69936654944139E-32,-1.)) ;
#121270=DIRECTION('center_axis',(-1.31418445149758E-16,1.,0.)) ;
#121271=DIRECTION('ref_axis',(-1.,-1.31418445149758E-16,0.)) ;
#121272=DIRECTION('',(1.,1.31418445149758E-16,-2.16840434497101E-16)) ;
#121273=DIRECTION('center_axis',(-1.31418445149758E-16,1.,0.)) ;
#121274=DIRECTION('ref_axis',(-1.,-1.31418445149758E-16,0.)) ;
#121275=DIRECTION('',(2.16840434497101E-16,2.8496832747207E-32,1.)) ;
#121276=DIRECTION('center_axis',(-1.31418445149758E-16,1.,0.)) ;
#121277=DIRECTION('ref_axis',(-1.,-1.31418445149758E-16,0.)) ;
#121278=DIRECTION('',(-1.,-1.31418445149758E-16,-2.16840434497101E-16)) ;
#121279=DIRECTION('center_axis',(-1.31418445149758E-16,1.,0.)) ;
#121280=DIRECTION('ref_axis',(-1.,-1.31418445149758E-16,0.)) ;
#121281=DIRECTION('',(-4.33680868994202E-16,-5.69936654944139E-32,-1.)) ;
#121282=DIRECTION('center_axis',(-1.31418445149758E-16,1.,0.)) ;
#121283=DIRECTION('ref_axis',(-1.,-1.31418445149758E-16,0.)) ;
#121284=DIRECTION('',(1.,1.31418445149758E-16,-2.16840434497101E-16)) ;
#121285=DIRECTION('center_axis',(-1.31418445149758E-16,1.,0.)) ;
#121286=DIRECTION('ref_axis',(-1.,-1.31418445149758E-16,0.)) ;
#121287=DIRECTION('',(2.16840434497101E-16,2.8496832747207E-32,1.)) ;
#121288=DIRECTION('center_axis',(-1.31418445149758E-16,1.,0.)) ;
#121289=DIRECTION('ref_axis',(-1.,-1.31418445149758E-16,0.)) ;
#121290=DIRECTION('',(-1.,-1.31418445149758E-16,-2.16840434497101E-16)) ;
#121291=DIRECTION('center_axis',(-1.31418445149758E-16,1.,0.)) ;
#121292=DIRECTION('ref_axis',(-1.,-1.31418445149758E-16,0.)) ;
#121293=DIRECTION('',(-4.33680868994202E-16,-5.69936654944139E-32,-1.)) ;
#121294=DIRECTION('center_axis',(-1.31418445149758E-16,1.,0.)) ;
#121295=DIRECTION('ref_axis',(-1.,-1.31418445149758E-16,0.)) ;
#121296=DIRECTION('',(1.,1.31418445149758E-16,-2.16840434497101E-16)) ;
#121297=DIRECTION('center_axis',(-1.31418445149758E-16,1.,0.)) ;
#121298=DIRECTION('ref_axis',(-1.,-1.31418445149758E-16,0.)) ;
#121299=DIRECTION('',(2.16840434497101E-16,2.8496832747207E-32,1.)) ;
#121300=DIRECTION('center_axis',(-1.31418445149758E-16,1.,0.)) ;
#121301=DIRECTION('ref_axis',(-1.,-1.31418445149758E-16,0.)) ;
#121302=DIRECTION('',(-1.,-1.31418445149758E-16,-2.16840434497101E-16)) ;
#121303=DIRECTION('center_axis',(-1.31418445149758E-16,1.,0.)) ;
#121304=DIRECTION('ref_axis',(-1.,-1.31418445149758E-16,0.)) ;
#121305=DIRECTION('',(-4.33680868994202E-16,-5.69936654944139E-32,-1.)) ;
#121306=DIRECTION('center_axis',(-1.31418445149758E-16,1.,0.)) ;
#121307=DIRECTION('ref_axis',(-1.,-1.31418445149758E-16,0.)) ;
#121308=DIRECTION('',(1.,1.31418445149758E-16,-2.16840434497101E-16)) ;
#121309=DIRECTION('center_axis',(-1.31418445149758E-16,1.,0.)) ;
#121310=DIRECTION('ref_axis',(-1.,-1.31418445149758E-16,0.)) ;
#121311=DIRECTION('',(2.16840434497101E-16,2.8496832747207E-32,1.)) ;
#121312=DIRECTION('center_axis',(-1.31418445149758E-16,1.,0.)) ;
#121313=DIRECTION('ref_axis',(-1.,-1.31418445149758E-16,0.)) ;
#121314=DIRECTION('',(-1.,-1.31418445149758E-16,-2.16840434497101E-16)) ;
#121315=DIRECTION('center_axis',(-1.31418445149758E-16,1.,0.)) ;
#121316=DIRECTION('ref_axis',(-1.,-1.31418445149758E-16,0.)) ;
#121317=DIRECTION('',(-4.33680868994202E-16,-5.69936654944139E-32,-1.)) ;
#121318=DIRECTION('center_axis',(-1.31418445149758E-16,1.,0.)) ;
#121319=DIRECTION('ref_axis',(-1.,-1.31418445149758E-16,0.)) ;
#121320=DIRECTION('',(1.,1.31418445149758E-16,-2.16840434497101E-16)) ;
#121321=DIRECTION('center_axis',(-1.31418445149758E-16,1.,0.)) ;
#121322=DIRECTION('ref_axis',(-1.,-1.31418445149758E-16,0.)) ;
#121323=DIRECTION('',(2.16840434497101E-16,2.8496832747207E-32,1.)) ;
#121324=DIRECTION('center_axis',(-1.31418445149758E-16,1.,0.)) ;
#121325=DIRECTION('ref_axis',(-1.,-1.31418445149758E-16,0.)) ;
#121326=DIRECTION('',(-1.,-1.31418445149758E-16,-2.16840434497101E-16)) ;
#121327=DIRECTION('center_axis',(-1.31418445149758E-16,1.,0.)) ;
#121328=DIRECTION('ref_axis',(-1.,-1.31418445149758E-16,0.)) ;
#121329=DIRECTION('',(-4.33680868994202E-16,-5.69936654944139E-32,-1.)) ;
#121330=DIRECTION('center_axis',(-1.31418445149758E-16,1.,0.)) ;
#121331=DIRECTION('ref_axis',(-1.,-1.31418445149758E-16,0.)) ;
#121332=DIRECTION('',(1.,1.31418445149758E-16,-2.16840434497101E-16)) ;
#121333=DIRECTION('center_axis',(-1.31418445149758E-16,1.,0.)) ;
#121334=DIRECTION('ref_axis',(-1.,-1.31418445149758E-16,0.)) ;
#121335=DIRECTION('',(2.16840434497101E-16,2.8496832747207E-32,1.)) ;
#121336=DIRECTION('center_axis',(-1.31418445149758E-16,1.,0.)) ;
#121337=DIRECTION('ref_axis',(-1.,-1.31418445149758E-16,0.)) ;
#121338=DIRECTION('',(-1.,-1.31418445149758E-16,-2.16840434497101E-16)) ;
#121339=DIRECTION('center_axis',(-1.31418445149758E-16,1.,0.)) ;
#121340=DIRECTION('ref_axis',(-1.,-1.31418445149758E-16,0.)) ;
#121341=DIRECTION('',(-4.33680868994202E-16,-5.69936654944139E-32,-1.)) ;
#121342=DIRECTION('center_axis',(-1.31418445149758E-16,1.,0.)) ;
#121343=DIRECTION('ref_axis',(-1.,-1.31418445149758E-16,0.)) ;
#121344=DIRECTION('',(1.,1.31418445149758E-16,-2.16840434497101E-16)) ;
#121345=DIRECTION('center_axis',(-1.31418445149758E-16,1.,0.)) ;
#121346=DIRECTION('ref_axis',(-1.,-1.31418445149758E-16,0.)) ;
#121347=DIRECTION('',(2.16840434497101E-16,2.8496832747207E-32,1.)) ;
#121348=DIRECTION('center_axis',(-1.31418445149758E-16,1.,0.)) ;
#121349=DIRECTION('ref_axis',(-1.,-1.31418445149758E-16,0.)) ;
#121350=DIRECTION('',(-1.,-1.31418445149758E-16,-2.16840434497101E-16)) ;
#121351=DIRECTION('center_axis',(-1.31418445149758E-16,1.,0.)) ;
#121352=DIRECTION('ref_axis',(-1.,-1.31418445149758E-16,0.)) ;
#121353=DIRECTION('',(-4.33680868994202E-16,-5.69936654944139E-32,-1.)) ;
#121354=DIRECTION('center_axis',(-1.31418445149758E-16,1.,0.)) ;
#121355=DIRECTION('ref_axis',(-1.,-1.31418445149758E-16,0.)) ;
#121356=DIRECTION('',(1.,1.31418445149758E-16,-2.16840434497101E-16)) ;
#121357=DIRECTION('center_axis',(-1.31418445149758E-16,1.,0.)) ;
#121358=DIRECTION('ref_axis',(-1.,-1.31418445149758E-16,0.)) ;
#121359=DIRECTION('',(2.16840434497101E-16,2.8496832747207E-32,1.)) ;
#121360=DIRECTION('center_axis',(0.,-1.,0.)) ;
#121361=DIRECTION('ref_axis',(0.,0.,-1.)) ;
#121362=DIRECTION('',(0.,0.,-1.)) ;
#121363=DIRECTION('',(-1.,0.,-7.01133629567814E-33)) ;
#121364=DIRECTION('',(0.,0.,1.)) ;
#121365=DIRECTION('',(1.,0.,-7.01133629567814E-33)) ;
#121366=DIRECTION('',(0.,0.,1.)) ;
#121367=DIRECTION('center_axis',(0.,-1.,0.)) ;
#121368=DIRECTION('ref_axis',(0.,0.,-1.)) ;
#121369=DIRECTION('',(-1.,0.,0.)) ;
#121370=DIRECTION('center_axis',(0.,-1.,0.)) ;
#121371=DIRECTION('ref_axis',(0.,0.,-1.)) ;
#121372=DIRECTION('',(0.,0.,-1.)) ;
#121373=DIRECTION('center_axis',(0.,-1.,0.)) ;
#121374=DIRECTION('ref_axis',(0.,0.,-1.)) ;
#121375=DIRECTION('',(1.,0.,0.)) ;
#121376=DIRECTION('center_axis',(0.,-1.,0.)) ;
#121377=DIRECTION('ref_axis',(0.,0.,-1.)) ;
#121378=DIRECTION('center_axis',(0.,-1.,0.)) ;
#121379=DIRECTION('ref_axis',(0.,0.,-1.)) ;
#121380=DIRECTION('',(0.,0.,-1.)) ;
#121381=DIRECTION('',(-1.,0.,-7.01133629567814E-33)) ;
#121382=DIRECTION('',(0.,0.,1.)) ;
#121383=DIRECTION('',(1.,0.,-7.01133629567814E-33)) ;
#121384=DIRECTION('',(0.,0.,1.)) ;
#121385=DIRECTION('center_axis',(0.,-1.,0.)) ;
#121386=DIRECTION('ref_axis',(0.,0.,-1.)) ;
#121387=DIRECTION('',(-1.,0.,0.)) ;
#121388=DIRECTION('center_axis',(0.,-1.,0.)) ;
#121389=DIRECTION('ref_axis',(0.,0.,-1.)) ;
#121390=DIRECTION('',(0.,0.,-1.)) ;
#121391=DIRECTION('center_axis',(0.,-1.,0.)) ;
#121392=DIRECTION('ref_axis',(0.,0.,-1.)) ;
#121393=DIRECTION('',(1.,0.,0.)) ;
#121394=DIRECTION('center_axis',(0.,-1.,0.)) ;
#121395=DIRECTION('ref_axis',(0.,0.,-1.)) ;
#121396=DIRECTION('center_axis',(0.,-1.,0.)) ;
#121397=DIRECTION('ref_axis',(0.,0.,-1.)) ;
#121398=DIRECTION('',(0.,0.,-1.)) ;
#121399=DIRECTION('',(-1.,0.,-7.01133629567814E-33)) ;
#121400=DIRECTION('',(0.,0.,1.)) ;
#121401=DIRECTION('',(1.,0.,-7.01133629567814E-33)) ;
#121402=DIRECTION('',(0.,0.,1.)) ;
#121403=DIRECTION('center_axis',(0.,-1.,0.)) ;
#121404=DIRECTION('ref_axis',(0.,0.,-1.)) ;
#121405=DIRECTION('',(-1.,0.,0.)) ;
#121406=DIRECTION('center_axis',(0.,-1.,0.)) ;
#121407=DIRECTION('ref_axis',(0.,0.,-1.)) ;
#121408=DIRECTION('',(0.,0.,-1.)) ;
#121409=DIRECTION('center_axis',(0.,-1.,0.)) ;
#121410=DIRECTION('ref_axis',(0.,0.,-1.)) ;
#121411=DIRECTION('',(1.,0.,0.)) ;
#121412=DIRECTION('center_axis',(0.,-1.,0.)) ;
#121413=DIRECTION('ref_axis',(0.,0.,-1.)) ;
#121414=DIRECTION('center_axis',(0.,-1.,0.)) ;
#121415=DIRECTION('ref_axis',(0.,0.,-1.)) ;
#121416=DIRECTION('',(0.,0.,-1.)) ;
#121417=DIRECTION('',(-1.,0.,-7.01133629567814E-33)) ;
#121418=DIRECTION('',(0.,0.,1.)) ;
#121419=DIRECTION('',(1.,0.,-7.01133629567814E-33)) ;
#121420=DIRECTION('',(0.,0.,1.)) ;
#121421=DIRECTION('center_axis',(0.,-1.,0.)) ;
#121422=DIRECTION('ref_axis',(0.,0.,-1.)) ;
#121423=DIRECTION('',(-1.,0.,0.)) ;
#121424=DIRECTION('center_axis',(0.,-1.,0.)) ;
#121425=DIRECTION('ref_axis',(0.,0.,-1.)) ;
#121426=DIRECTION('',(0.,0.,-1.)) ;
#121427=DIRECTION('center_axis',(0.,-1.,0.)) ;
#121428=DIRECTION('ref_axis',(0.,0.,-1.)) ;
#121429=DIRECTION('',(1.,0.,0.)) ;
#121430=DIRECTION('center_axis',(0.,-1.,0.)) ;
#121431=DIRECTION('ref_axis',(0.,0.,-1.)) ;
#121432=DIRECTION('center_axis',(0.,-1.,0.)) ;
#121433=DIRECTION('ref_axis',(0.,0.,-1.)) ;
#121434=DIRECTION('',(0.,0.,-1.)) ;
#121435=DIRECTION('',(-1.,0.,-7.01133629567814E-33)) ;
#121436=DIRECTION('',(0.,0.,1.)) ;
#121437=DIRECTION('',(1.,0.,-7.01133629567814E-33)) ;
#121438=DIRECTION('',(0.,0.,1.)) ;
#121439=DIRECTION('center_axis',(0.,-1.,0.)) ;
#121440=DIRECTION('ref_axis',(0.,0.,-1.)) ;
#121441=DIRECTION('',(-1.,0.,0.)) ;
#121442=DIRECTION('center_axis',(0.,-1.,0.)) ;
#121443=DIRECTION('ref_axis',(0.,0.,-1.)) ;
#121444=DIRECTION('',(0.,0.,-1.)) ;
#121445=DIRECTION('center_axis',(0.,-1.,0.)) ;
#121446=DIRECTION('ref_axis',(0.,0.,-1.)) ;
#121447=DIRECTION('',(1.,0.,0.)) ;
#121448=DIRECTION('center_axis',(0.,-1.,0.)) ;
#121449=DIRECTION('ref_axis',(0.,0.,-1.)) ;
#121450=DIRECTION('center_axis',(0.,-1.,0.)) ;
#121451=DIRECTION('ref_axis',(0.,0.,-1.)) ;
#121452=DIRECTION('',(0.,0.,-1.)) ;
#121453=DIRECTION('',(-1.,0.,-7.01133629567814E-33)) ;
#121454=DIRECTION('',(0.,0.,1.)) ;
#121455=DIRECTION('',(1.,0.,-7.01133629567814E-33)) ;
#121456=DIRECTION('',(0.,0.,1.)) ;
#121457=DIRECTION('center_axis',(0.,-1.,0.)) ;
#121458=DIRECTION('ref_axis',(0.,0.,-1.)) ;
#121459=DIRECTION('',(-1.,0.,0.)) ;
#121460=DIRECTION('center_axis',(0.,-1.,0.)) ;
#121461=DIRECTION('ref_axis',(0.,0.,-1.)) ;
#121462=DIRECTION('',(0.,0.,-1.)) ;
#121463=DIRECTION('center_axis',(0.,-1.,0.)) ;
#121464=DIRECTION('ref_axis',(0.,0.,-1.)) ;
#121465=DIRECTION('',(1.,0.,0.)) ;
#121466=DIRECTION('center_axis',(0.,-1.,0.)) ;
#121467=DIRECTION('ref_axis',(0.,0.,-1.)) ;
#121468=DIRECTION('center_axis',(0.,-1.,0.)) ;
#121469=DIRECTION('ref_axis',(0.,0.,-1.)) ;
#121470=DIRECTION('',(0.,0.,-1.)) ;
#121471=DIRECTION('',(-1.,0.,-7.01133629567814E-33)) ;
#121472=DIRECTION('',(0.,0.,1.)) ;
#121473=DIRECTION('',(1.,0.,-7.01133629567814E-33)) ;
#121474=DIRECTION('',(0.,0.,1.)) ;
#121475=DIRECTION('center_axis',(0.,-1.,0.)) ;
#121476=DIRECTION('ref_axis',(0.,0.,-1.)) ;
#121477=DIRECTION('',(-1.,0.,0.)) ;
#121478=DIRECTION('center_axis',(0.,-1.,0.)) ;
#121479=DIRECTION('ref_axis',(0.,0.,-1.)) ;
#121480=DIRECTION('',(0.,0.,-1.)) ;
#121481=DIRECTION('center_axis',(0.,-1.,0.)) ;
#121482=DIRECTION('ref_axis',(0.,0.,-1.)) ;
#121483=DIRECTION('',(1.,0.,0.)) ;
#121484=DIRECTION('center_axis',(0.,-1.,0.)) ;
#121485=DIRECTION('ref_axis',(0.,0.,-1.)) ;
#121486=DIRECTION('center_axis',(0.,-1.,0.)) ;
#121487=DIRECTION('ref_axis',(0.,0.,-1.)) ;
#121488=DIRECTION('',(0.,0.,-1.)) ;
#121489=DIRECTION('',(-1.,0.,-7.01133629567814E-33)) ;
#121490=DIRECTION('',(0.,0.,1.)) ;
#121491=DIRECTION('',(1.,0.,-7.01133629567814E-33)) ;
#121492=DIRECTION('',(0.,0.,1.)) ;
#121493=DIRECTION('center_axis',(0.,-1.,0.)) ;
#121494=DIRECTION('ref_axis',(0.,0.,-1.)) ;
#121495=DIRECTION('',(-1.,0.,0.)) ;
#121496=DIRECTION('center_axis',(0.,-1.,0.)) ;
#121497=DIRECTION('ref_axis',(0.,0.,-1.)) ;
#121498=DIRECTION('',(0.,0.,-1.)) ;
#121499=DIRECTION('center_axis',(0.,-1.,0.)) ;
#121500=DIRECTION('ref_axis',(0.,0.,-1.)) ;
#121501=DIRECTION('',(1.,0.,0.)) ;
#121502=DIRECTION('center_axis',(0.,-1.,0.)) ;
#121503=DIRECTION('ref_axis',(0.,0.,-1.)) ;
#121504=DIRECTION('center_axis',(0.,-1.,0.)) ;
#121505=DIRECTION('ref_axis',(0.,0.,-1.)) ;
#121506=DIRECTION('',(0.,0.,-1.)) ;
#121507=DIRECTION('',(-1.,0.,-7.01133629567814E-33)) ;
#121508=DIRECTION('',(0.,0.,1.)) ;
#121509=DIRECTION('',(1.,0.,-7.01133629567814E-33)) ;
#121510=DIRECTION('',(0.,0.,1.)) ;
#121511=DIRECTION('center_axis',(0.,-1.,0.)) ;
#121512=DIRECTION('ref_axis',(0.,0.,-1.)) ;
#121513=DIRECTION('',(-1.,0.,0.)) ;
#121514=DIRECTION('center_axis',(0.,-1.,0.)) ;
#121515=DIRECTION('ref_axis',(0.,0.,-1.)) ;
#121516=DIRECTION('',(0.,0.,-1.)) ;
#121517=DIRECTION('center_axis',(0.,-1.,0.)) ;
#121518=DIRECTION('ref_axis',(0.,0.,-1.)) ;
#121519=DIRECTION('',(1.,0.,0.)) ;
#121520=DIRECTION('center_axis',(0.,-1.,0.)) ;
#121521=DIRECTION('ref_axis',(0.,0.,-1.)) ;
#121522=DIRECTION('center_axis',(1.31418445149758E-16,1.,0.)) ;
#121523=DIRECTION('ref_axis',(-1.,1.31418445149758E-16,0.)) ;
#121524=DIRECTION('',(0.422618261740697,-5.55398348498559E-17,-0.906307787036651)) ;
#121525=DIRECTION('center_axis',(1.31418445149758E-16,1.,0.)) ;
#121526=DIRECTION('ref_axis',(-1.,1.31418445149758E-16,0.)) ;
#121527=DIRECTION('',(0.422618261740697,-5.55398348498559E-17,-0.906307787036651)) ;
#121528=DIRECTION('center_axis',(1.31418445149758E-16,1.,0.)) ;
#121529=DIRECTION('ref_axis',(-1.,1.31418445149758E-16,0.)) ;
#121530=DIRECTION('',(0.422618261740697,-5.55398348498559E-17,-0.906307787036651)) ;
#121531=DIRECTION('center_axis',(1.31418445149758E-16,1.,0.)) ;
#121532=DIRECTION('ref_axis',(-1.,1.31418445149758E-16,0.)) ;
#121533=DIRECTION('',(0.422618261740697,-5.55398348498559E-17,-0.906307787036651)) ;
#121534=DIRECTION('center_axis',(1.31418445149758E-16,1.,0.)) ;
#121535=DIRECTION('ref_axis',(-1.,1.31418445149758E-16,0.)) ;
#121536=DIRECTION('',(0.422618261740697,-5.55398348498559E-17,-0.906307787036651)) ;
#121537=DIRECTION('center_axis',(1.31418445149758E-16,1.,0.)) ;
#121538=DIRECTION('ref_axis',(-1.,1.31418445149758E-16,0.)) ;
#121539=DIRECTION('',(0.422618261740697,-5.55398348498559E-17,-0.906307787036651)) ;
#121540=DIRECTION('center_axis',(1.31418445149758E-16,1.,0.)) ;
#121541=DIRECTION('ref_axis',(-1.,1.31418445149758E-16,0.)) ;
#121542=DIRECTION('',(0.422618261740697,-5.55398348498559E-17,-0.906307787036651)) ;
#121543=DIRECTION('center_axis',(1.31418445149758E-16,1.,0.)) ;
#121544=DIRECTION('ref_axis',(-1.,1.31418445149758E-16,0.)) ;
#121545=DIRECTION('',(0.422618261740697,-5.55398348498559E-17,-0.906307787036651)) ;
#121546=DIRECTION('center_axis',(1.31418445149758E-16,1.,0.)) ;
#121547=DIRECTION('ref_axis',(-1.,1.31418445149758E-16,0.)) ;
#121548=DIRECTION('',(0.422618261740697,-5.55398348498559E-17,-0.906307787036651)) ;
#121549=DIRECTION('center_axis',(1.,0.,0.)) ;
#121550=DIRECTION('ref_axis',(0.,0.,-1.)) ;
#121551=DIRECTION('',(0.,-4.8455963016112E-16,-1.)) ;
#121552=DIRECTION('',(0.,1.,0.)) ;
#121553=DIRECTION('',(0.,0.,1.)) ;
#121554=DIRECTION('',(0.,-1.,0.)) ;
#121555=DIRECTION('',(0.,4.8455963016112E-16,-1.)) ;
#121556=DIRECTION('center_axis',(-1.,0.,0.)) ;
#121557=DIRECTION('ref_axis',(0.,2.16840434497101E-15,-1.)) ;
#121558=DIRECTION('center_axis',(-1.,0.,0.)) ;
#121559=DIRECTION('ref_axis',(0.,0.,-1.)) ;
#121560=DIRECTION('',(0.,0.,-1.)) ;
#121561=DIRECTION('center_axis',(-1.,0.,0.)) ;
#121562=DIRECTION('ref_axis',(0.,-2.16840434497101E-15,-1.)) ;
#121563=DIRECTION('center_axis',(-1.,0.,0.)) ;
#121564=DIRECTION('ref_axis',(0.,-3.25260651745651E-15,-1.)) ;
#121565=DIRECTION('',(0.,-4.8455963016112E-16,-1.)) ;
#121566=DIRECTION('center_axis',(-1.,0.,0.)) ;
#121567=DIRECTION('ref_axis',(0.,1.0842021724855E-15,-1.)) ;
#121568=DIRECTION('center_axis',(-1.,0.,0.)) ;
#121569=DIRECTION('ref_axis',(0.,0.,-1.)) ;
#121570=DIRECTION('',(0.,0.,-1.)) ;
#121571=DIRECTION('center_axis',(-1.,0.,0.)) ;
#121572=DIRECTION('ref_axis',(0.,-2.16840434497101E-15,-1.)) ;
#121573=DIRECTION('center_axis',(-1.,0.,0.)) ;
#121574=DIRECTION('ref_axis',(0.,3.25260651745652E-15,-1.)) ;
#121575=DIRECTION('',(0.,-4.8455963016112E-16,-1.)) ;
#121576=DIRECTION('center_axis',(-1.,0.,0.)) ;
#121577=DIRECTION('ref_axis',(0.,2.16840434497101E-15,-1.)) ;
#121578=DIRECTION('center_axis',(-1.,0.,0.)) ;
#121579=DIRECTION('ref_axis',(0.,0.,-1.)) ;
#121580=DIRECTION('',(0.,0.,-1.)) ;
#121581=DIRECTION('center_axis',(-1.,0.,0.)) ;
#121582=DIRECTION('ref_axis',(0.,3.25260651745651E-15,-1.)) ;
#121583=DIRECTION('center_axis',(-1.,0.,0.)) ;
#121584=DIRECTION('ref_axis',(0.,-7.58941520739851E-15,-1.)) ;
#121585=DIRECTION('',(0.,-4.8455963016112E-16,-1.)) ;
#121586=DIRECTION('center_axis',(-1.,0.,0.)) ;
#121587=DIRECTION('ref_axis',(0.,1.0842021724855E-15,-1.)) ;
#121588=DIRECTION('center_axis',(-1.,0.,0.)) ;
#121589=DIRECTION('ref_axis',(0.,1.19262238973405E-14,-1.)) ;
#121590=DIRECTION('',(0.,0.,-1.)) ;
#121591=DIRECTION('center_axis',(-1.,0.,0.)) ;
#121592=DIRECTION('ref_axis',(0.,2.168404344971E-15,-1.)) ;
#121593=DIRECTION('center_axis',(-1.,0.,0.)) ;
#121594=DIRECTION('ref_axis',(0.,1.0842021724855E-15,-1.)) ;
#121595=DIRECTION('',(0.,-4.8455963016112E-16,-1.)) ;
#121596=DIRECTION('center_axis',(-1.,0.,0.)) ;
#121597=DIRECTION('ref_axis',(0.,1.0842021724855E-15,-1.)) ;
#121598=DIRECTION('center_axis',(-1.,0.,0.)) ;
#121599=DIRECTION('ref_axis',(0.,1.19262238973405E-14,-1.)) ;
#121600=DIRECTION('',(0.,0.,-1.)) ;
#121601=DIRECTION('center_axis',(-1.,0.,0.)) ;
#121602=DIRECTION('ref_axis',(0.,2.16840434497102E-15,-1.)) ;
#121603=DIRECTION('center_axis',(-1.,0.,0.)) ;
#121604=DIRECTION('ref_axis',(0.,1.08420217248551E-15,-1.)) ;
#121605=DIRECTION('',(0.,-4.8455963016112E-16,-1.)) ;
#121606=DIRECTION('center_axis',(-1.,0.,0.)) ;
#121607=DIRECTION('ref_axis',(0.,1.08420217248551E-15,-1.)) ;
#121608=DIRECTION('center_axis',(-1.,0.,0.)) ;
#121609=DIRECTION('ref_axis',(0.,1.19262238973406E-14,-1.)) ;
#121610=DIRECTION('',(0.,0.,-1.)) ;
#121611=DIRECTION('center_axis',(-1.,0.,0.)) ;
#121612=DIRECTION('ref_axis',(0.,2.16840434497102E-15,-1.)) ;
#121613=DIRECTION('center_axis',(-1.,0.,0.)) ;
#121614=DIRECTION('ref_axis',(0.,1.08420217248551E-15,-1.)) ;
#121615=DIRECTION('',(0.,-4.8455963016112E-16,-1.)) ;
#121616=DIRECTION('center_axis',(-1.,0.,0.)) ;
#121617=DIRECTION('ref_axis',(0.,1.08420217248551E-15,-1.)) ;
#121618=DIRECTION('center_axis',(-1.,0.,0.)) ;
#121619=DIRECTION('ref_axis',(0.,1.19262238973406E-14,-1.)) ;
#121620=DIRECTION('',(0.,0.,-1.)) ;
#121621=DIRECTION('center_axis',(-1.,0.,0.)) ;
#121622=DIRECTION('ref_axis',(0.,2.16840434497102E-15,-1.)) ;
#121623=DIRECTION('center_axis',(-1.,0.,0.)) ;
#121624=DIRECTION('ref_axis',(0.,1.08420217248551E-15,-1.)) ;
#121625=DIRECTION('',(0.,-4.8455963016112E-16,-1.)) ;
#121626=DIRECTION('center_axis',(-1.,0.,0.)) ;
#121627=DIRECTION('ref_axis',(0.,1.08420217248551E-15,-1.)) ;
#121628=DIRECTION('center_axis',(-1.,0.,0.)) ;
#121629=DIRECTION('ref_axis',(0.,1.19262238973406E-14,-1.)) ;
#121630=DIRECTION('',(0.,0.,-1.)) ;
#121631=DIRECTION('center_axis',(-1.,0.,0.)) ;
#121632=DIRECTION('ref_axis',(0.,2.16840434497102E-15,-1.)) ;
#121633=DIRECTION('center_axis',(-1.,0.,0.)) ;
#121634=DIRECTION('ref_axis',(0.,1.08420217248551E-15,-1.)) ;
#121635=DIRECTION('',(0.,-4.8455963016112E-16,-1.)) ;
#121636=DIRECTION('center_axis',(-1.,0.,0.)) ;
#121637=DIRECTION('ref_axis',(0.,1.08420217248551E-15,-1.)) ;
#121638=DIRECTION('center_axis',(-1.,0.,0.)) ;
#121639=DIRECTION('ref_axis',(0.,1.19262238973406E-14,-1.)) ;
#121640=DIRECTION('',(0.,0.,-1.)) ;
#121641=DIRECTION('center_axis',(-1.,0.,0.)) ;
#121642=DIRECTION('ref_axis',(0.,2.16840434497102E-15,-1.)) ;
#121643=DIRECTION('center_axis',(-1.,0.,0.)) ;
#121644=DIRECTION('ref_axis',(0.,0.,-1.)) ;
#121645=DIRECTION('',(0.,-4.8455963016112E-16,-1.)) ;
#121646=DIRECTION('center_axis',(-1.,0.,0.)) ;
#121647=DIRECTION('ref_axis',(0.,-2.16840434497102E-15,-1.)) ;
#121648=DIRECTION('center_axis',(-1.,0.,0.)) ;
#121649=DIRECTION('ref_axis',(0.,-3.25260651745653E-15,-1.)) ;
#121650=DIRECTION('',(0.,0.,-1.)) ;
#121651=DIRECTION('center_axis',(-1.,0.,0.)) ;
#121652=DIRECTION('ref_axis',(0.,2.16840434497102E-15,-1.)) ;
#121653=DIRECTION('center_axis',(-1.,0.,0.)) ;
#121654=DIRECTION('ref_axis',(0.,0.,-1.)) ;
#121655=DIRECTION('center_axis',(1.,0.,0.)) ;
#121656=DIRECTION('ref_axis',(0.,0.,-1.)) ;
#121657=DIRECTION('center_axis',(1.,0.,0.)) ;
#121658=DIRECTION('ref_axis',(0.,0.,-1.)) ;
#121659=DIRECTION('',(0.,0.,1.)) ;
#121660=DIRECTION('',(0.,-1.,-8.9727076343628E-17)) ;
#121661=DIRECTION('',(0.,0.,-1.)) ;
#121662=DIRECTION('',(0.,1.,-8.9727076343628E-17)) ;
#121663=DIRECTION('',(0.,0.,1.)) ;
#121664=DIRECTION('center_axis',(1.,0.,0.)) ;
#121665=DIRECTION('ref_axis',(0.,0.,-1.)) ;
#121666=DIRECTION('center_axis',(1.,0.,0.)) ;
#121667=DIRECTION('ref_axis',(0.,0.,-1.)) ;
#121668=DIRECTION('center_axis',(1.,0.,0.)) ;
#121669=DIRECTION('ref_axis',(0.,0.,-1.)) ;
#121670=DIRECTION('center_axis',(1.,0.,0.)) ;
#121671=DIRECTION('ref_axis',(0.,0.,-1.)) ;
#121672=DIRECTION('',(0.,0.,1.)) ;
#121673=DIRECTION('',(0.,-1.,-8.9727076343628E-17)) ;
#121674=DIRECTION('',(0.,0.,-1.)) ;
#121675=DIRECTION('',(0.,1.,-8.9727076343628E-17)) ;
#121676=DIRECTION('',(0.,0.,1.)) ;
#121677=DIRECTION('center_axis',(1.,0.,0.)) ;
#121678=DIRECTION('ref_axis',(0.,0.,-1.)) ;
#121679=DIRECTION('center_axis',(1.,0.,0.)) ;
#121680=DIRECTION('ref_axis',(0.,0.,-1.)) ;
#121681=DIRECTION('center_axis',(1.,0.,0.)) ;
#121682=DIRECTION('ref_axis',(0.,0.,-1.)) ;
#121683=DIRECTION('center_axis',(1.,0.,0.)) ;
#121684=DIRECTION('ref_axis',(0.,0.,-1.)) ;
#121685=DIRECTION('',(0.,0.,1.)) ;
#121686=DIRECTION('',(0.,-1.,-8.9727076343628E-17)) ;
#121687=DIRECTION('',(0.,0.,-1.)) ;
#121688=DIRECTION('',(0.,1.,-8.9727076343628E-17)) ;
#121689=DIRECTION('',(0.,0.,1.)) ;
#121690=DIRECTION('center_axis',(1.,0.,0.)) ;
#121691=DIRECTION('ref_axis',(0.,0.,-1.)) ;
#121692=DIRECTION('center_axis',(1.,0.,0.)) ;
#121693=DIRECTION('ref_axis',(0.,0.,-1.)) ;
#121694=DIRECTION('center_axis',(1.,0.,0.)) ;
#121695=DIRECTION('ref_axis',(0.,0.,-1.)) ;
#121696=DIRECTION('center_axis',(1.,0.,0.)) ;
#121697=DIRECTION('ref_axis',(0.,0.,-1.)) ;
#121698=DIRECTION('',(0.,0.,1.)) ;
#121699=DIRECTION('',(0.,-1.,-8.9727076343628E-17)) ;
#121700=DIRECTION('',(0.,0.,-1.)) ;
#121701=DIRECTION('',(0.,1.,-8.9727076343628E-17)) ;
#121702=DIRECTION('',(0.,0.,1.)) ;
#121703=DIRECTION('center_axis',(1.,0.,0.)) ;
#121704=DIRECTION('ref_axis',(0.,0.,-1.)) ;
#121705=DIRECTION('center_axis',(1.,0.,0.)) ;
#121706=DIRECTION('ref_axis',(0.,0.,-1.)) ;
#121707=DIRECTION('center_axis',(1.,0.,0.)) ;
#121708=DIRECTION('ref_axis',(0.,0.,-1.)) ;
#121709=DIRECTION('center_axis',(1.,0.,0.)) ;
#121710=DIRECTION('ref_axis',(0.,0.,-1.)) ;
#121711=DIRECTION('',(0.,0.,1.)) ;
#121712=DIRECTION('',(0.,-1.,-8.9727076343628E-17)) ;
#121713=DIRECTION('',(0.,0.,-1.)) ;
#121714=DIRECTION('',(0.,1.,-8.9727076343628E-17)) ;
#121715=DIRECTION('',(0.,0.,1.)) ;
#121716=DIRECTION('center_axis',(1.,0.,0.)) ;
#121717=DIRECTION('ref_axis',(0.,0.,-1.)) ;
#121718=DIRECTION('center_axis',(1.,0.,0.)) ;
#121719=DIRECTION('ref_axis',(0.,0.,-1.)) ;
#121720=DIRECTION('center_axis',(1.,0.,0.)) ;
#121721=DIRECTION('ref_axis',(0.,0.,-1.)) ;
#121722=DIRECTION('center_axis',(1.,0.,0.)) ;
#121723=DIRECTION('ref_axis',(0.,0.,-1.)) ;
#121724=DIRECTION('',(0.,0.,1.)) ;
#121725=DIRECTION('',(0.,-1.,-8.9727076343628E-17)) ;
#121726=DIRECTION('',(0.,0.,-1.)) ;
#121727=DIRECTION('',(0.,1.,-8.9727076343628E-17)) ;
#121728=DIRECTION('',(0.,0.,1.)) ;
#121729=DIRECTION('center_axis',(1.,0.,0.)) ;
#121730=DIRECTION('ref_axis',(0.,0.,-1.)) ;
#121731=DIRECTION('center_axis',(1.,0.,0.)) ;
#121732=DIRECTION('ref_axis',(0.,0.,-1.)) ;
#121733=DIRECTION('center_axis',(1.,0.,0.)) ;
#121734=DIRECTION('ref_axis',(0.,0.,-1.)) ;
#121735=DIRECTION('center_axis',(1.,0.,0.)) ;
#121736=DIRECTION('ref_axis',(0.,0.,-1.)) ;
#121737=DIRECTION('',(0.,0.,1.)) ;
#121738=DIRECTION('',(0.,-1.,-8.9727076343628E-17)) ;
#121739=DIRECTION('',(0.,0.,-1.)) ;
#121740=DIRECTION('',(0.,1.,-8.9727076343628E-17)) ;
#121741=DIRECTION('',(0.,0.,1.)) ;
#121742=DIRECTION('center_axis',(1.,0.,0.)) ;
#121743=DIRECTION('ref_axis',(0.,0.,-1.)) ;
#121744=DIRECTION('center_axis',(1.,0.,0.)) ;
#121745=DIRECTION('ref_axis',(0.,0.,-1.)) ;
#121746=DIRECTION('center_axis',(1.,0.,0.)) ;
#121747=DIRECTION('ref_axis',(0.,0.,-1.)) ;
#121748=DIRECTION('center_axis',(1.,0.,0.)) ;
#121749=DIRECTION('ref_axis',(0.,0.,-1.)) ;
#121750=DIRECTION('',(0.,0.,1.)) ;
#121751=DIRECTION('',(0.,-1.,-8.9727076343628E-17)) ;
#121752=DIRECTION('',(0.,0.,-1.)) ;
#121753=DIRECTION('',(0.,1.,-8.9727076343628E-17)) ;
#121754=DIRECTION('',(0.,0.,1.)) ;
#121755=DIRECTION('center_axis',(1.,0.,0.)) ;
#121756=DIRECTION('ref_axis',(0.,0.,-1.)) ;
#121757=DIRECTION('center_axis',(1.,0.,0.)) ;
#121758=DIRECTION('ref_axis',(0.,0.,-1.)) ;
#121759=DIRECTION('center_axis',(1.,0.,0.)) ;
#121760=DIRECTION('ref_axis',(0.,0.,-1.)) ;
#121761=DIRECTION('center_axis',(1.,0.,0.)) ;
#121762=DIRECTION('ref_axis',(0.,0.,-1.)) ;
#121763=DIRECTION('',(0.,0.,1.)) ;
#121764=DIRECTION('',(0.,-1.,-8.9727076343628E-17)) ;
#121765=DIRECTION('',(0.,0.,-1.)) ;
#121766=DIRECTION('',(0.,1.,-8.9727076343628E-17)) ;
#121767=DIRECTION('',(0.,0.,1.)) ;
#121768=DIRECTION('center_axis',(1.,0.,0.)) ;
#121769=DIRECTION('ref_axis',(0.,0.,-1.)) ;
#121770=DIRECTION('center_axis',(1.,0.,0.)) ;
#121771=DIRECTION('ref_axis',(0.,0.,-1.)) ;
#121772=DIRECTION('center_axis',(1.,7.81406971160724E-17,0.)) ;
#121773=DIRECTION('ref_axis',(-7.81406971160724E-17,1.,0.)) ;
#121774=DIRECTION('',(-7.81406971160724E-17,1.,0.)) ;
#121775=DIRECTION('',(0.,0.,1.)) ;
#121776=DIRECTION('',(7.81406971160724E-17,-1.,0.)) ;
#121777=DIRECTION('',(0.,0.,-1.)) ;
#121778=DIRECTION('center_axis',(1.,7.81406971160724E-17,0.)) ;
#121779=DIRECTION('ref_axis',(-7.81406971160724E-17,1.,0.)) ;
#121780=DIRECTION('',(0.,0.,-1.)) ;
#121781=DIRECTION('',(-7.81406971160724E-17,1.,0.)) ;
#121782=DIRECTION('',(-3.78638272950961E-32,4.8455963016112E-16,1.)) ;
#121783=DIRECTION('',(7.81406971160724E-17,-1.,8.9727076343628E-17)) ;
#121784=DIRECTION('center_axis',(1.,7.81406971160724E-17,0.)) ;
#121785=DIRECTION('ref_axis',(-7.81406971160724E-17,1.,0.)) ;
#121786=DIRECTION('',(0.,0.,1.)) ;
#121787=DIRECTION('center_axis',(1.,7.81406971160724E-17,0.)) ;
#121788=DIRECTION('ref_axis',(-7.81406971160724E-17,1.,0.)) ;
#121789=DIRECTION('',(-7.81406971160724E-17,1.,8.9727076343628E-17)) ;
#121790=DIRECTION('',(-3.78638272950961E-32,4.8455963016112E-16,1.)) ;
#121791=DIRECTION('',(7.81406971160724E-17,-1.,8.9727076343628E-17)) ;
#121792=DIRECTION('center_axis',(1.,7.81406971160724E-17,0.)) ;
#121793=DIRECTION('ref_axis',(-7.81406971160724E-17,1.,0.)) ;
#121794=DIRECTION('',(0.,0.,1.)) ;
#121795=DIRECTION('center_axis',(1.,7.81406971160724E-17,0.)) ;
#121796=DIRECTION('ref_axis',(-7.81406971160724E-17,1.,0.)) ;
#121797=DIRECTION('',(-7.81406971160724E-17,1.,8.9727076343628E-17)) ;
#121798=DIRECTION('',(-3.78638272950961E-32,4.8455963016112E-16,1.)) ;
#121799=DIRECTION('',(7.81406971160724E-17,-1.,8.9727076343628E-17)) ;
#121800=DIRECTION('center_axis',(1.,7.81406971160724E-17,0.)) ;
#121801=DIRECTION('ref_axis',(-7.81406971160724E-17,1.,0.)) ;
#121802=DIRECTION('',(0.,0.,1.)) ;
#121803=DIRECTION('center_axis',(1.,7.81406971160724E-17,0.)) ;
#121804=DIRECTION('ref_axis',(-7.81406971160724E-17,1.,0.)) ;
#121805=DIRECTION('',(-7.81406971160724E-17,1.,8.9727076343628E-17)) ;
#121806=DIRECTION('',(-3.78638272950961E-32,4.8455963016112E-16,1.)) ;
#121807=DIRECTION('',(7.81406971160724E-17,-1.,8.9727076343628E-17)) ;
#121808=DIRECTION('center_axis',(1.,7.81406971160724E-17,0.)) ;
#121809=DIRECTION('ref_axis',(-7.81406971160724E-17,1.,0.)) ;
#121810=DIRECTION('',(0.,0.,1.)) ;
#121811=DIRECTION('center_axis',(1.,7.81406971160724E-17,0.)) ;
#121812=DIRECTION('ref_axis',(-7.81406971160724E-17,1.,0.)) ;
#121813=DIRECTION('',(-7.81406971160724E-17,1.,8.9727076343628E-17)) ;
#121814=DIRECTION('',(-3.78638272950961E-32,4.8455963016112E-16,1.)) ;
#121815=DIRECTION('',(7.81406971160724E-17,-1.,8.9727076343628E-17)) ;
#121816=DIRECTION('center_axis',(1.,7.81406971160724E-17,0.)) ;
#121817=DIRECTION('ref_axis',(-7.81406971160724E-17,1.,0.)) ;
#121818=DIRECTION('',(0.,0.,1.)) ;
#121819=DIRECTION('center_axis',(1.,7.81406971160724E-17,0.)) ;
#121820=DIRECTION('ref_axis',(-7.81406971160724E-17,1.,0.)) ;
#121821=DIRECTION('',(-7.81406971160724E-17,1.,8.9727076343628E-17)) ;
#121822=DIRECTION('',(-3.78638272950961E-32,4.8455963016112E-16,1.)) ;
#121823=DIRECTION('',(7.81406971160724E-17,-1.,8.9727076343628E-17)) ;
#121824=DIRECTION('center_axis',(1.,7.81406971160724E-17,0.)) ;
#121825=DIRECTION('ref_axis',(-7.81406971160724E-17,1.,0.)) ;
#121826=DIRECTION('',(0.,0.,1.)) ;
#121827=DIRECTION('center_axis',(1.,7.81406971160724E-17,0.)) ;
#121828=DIRECTION('ref_axis',(-7.81406971160724E-17,1.,0.)) ;
#121829=DIRECTION('',(-7.81406971160724E-17,1.,8.9727076343628E-17)) ;
#121830=DIRECTION('',(-3.78638272950961E-32,4.8455963016112E-16,1.)) ;
#121831=DIRECTION('',(7.81406971160724E-17,-1.,8.9727076343628E-17)) ;
#121832=DIRECTION('center_axis',(1.,7.81406971160724E-17,0.)) ;
#121833=DIRECTION('ref_axis',(-7.81406971160724E-17,1.,0.)) ;
#121834=DIRECTION('',(0.,0.,1.)) ;
#121835=DIRECTION('center_axis',(1.,7.81406971160724E-17,0.)) ;
#121836=DIRECTION('ref_axis',(-7.81406971160724E-17,1.,0.)) ;
#121837=DIRECTION('',(-7.81406971160724E-17,1.,8.9727076343628E-17)) ;
#121838=DIRECTION('',(-3.78638272950961E-32,4.8455963016112E-16,1.)) ;
#121839=DIRECTION('',(7.81406971160724E-17,-1.,8.9727076343628E-17)) ;
#121840=DIRECTION('center_axis',(1.,7.81406971160724E-17,0.)) ;
#121841=DIRECTION('ref_axis',(-7.81406971160724E-17,1.,0.)) ;
#121842=DIRECTION('',(0.,0.,1.)) ;
#121843=DIRECTION('center_axis',(1.,7.81406971160724E-17,0.)) ;
#121844=DIRECTION('ref_axis',(-7.81406971160724E-17,1.,0.)) ;
#121845=DIRECTION('',(-7.81406971160724E-17,1.,8.9727076343628E-17)) ;
#121846=DIRECTION('',(-3.78638272950961E-32,4.8455963016112E-16,1.)) ;
#121847=DIRECTION('',(7.81406971160724E-17,-1.,8.9727076343628E-17)) ;
#121848=DIRECTION('center_axis',(1.,7.81406971160724E-17,0.)) ;
#121849=DIRECTION('ref_axis',(-7.81406971160724E-17,1.,0.)) ;
#121850=DIRECTION('',(0.,0.,1.)) ;
#121851=DIRECTION('center_axis',(1.,7.81406971160724E-17,0.)) ;
#121852=DIRECTION('ref_axis',(-7.81406971160724E-17,1.,0.)) ;
#121853=DIRECTION('',(-7.81406971160724E-17,1.,8.9727076343628E-17)) ;
#121854=DIRECTION('',(-3.78638272950961E-32,4.8455963016112E-16,1.)) ;
#121855=DIRECTION('',(7.81406971160724E-17,-1.,8.9727076343628E-17)) ;
#121856=DIRECTION('center_axis',(1.,7.81406971160724E-17,0.)) ;
#121857=DIRECTION('ref_axis',(-7.81406971160724E-17,1.,0.)) ;
#121858=DIRECTION('',(0.,0.,1.)) ;
#121859=DIRECTION('center_axis',(1.,7.81406971160724E-17,0.)) ;
#121860=DIRECTION('ref_axis',(-7.81406971160724E-17,1.,0.)) ;
#121861=DIRECTION('',(-7.81406971160724E-17,1.,8.9727076343628E-17)) ;
#121862=DIRECTION('',(3.78638272950961E-32,-4.8455963016112E-16,1.)) ;
#121863=DIRECTION('',(7.81406971160724E-17,-1.,0.)) ;
#121864=DIRECTION('center_axis',(0.,0.,-1.)) ;
#121865=DIRECTION('ref_axis',(-1.,0.,0.)) ;
#121866=DIRECTION('',(0.,0.,-1.)) ;
#121867=DIRECTION('center_axis',(0.,0.,-1.)) ;
#121868=DIRECTION('ref_axis',(-1.,0.,0.)) ;
#121869=DIRECTION('center_axis',(0.,0.,1.)) ;
#121870=DIRECTION('ref_axis',(-1.,0.,0.)) ;
#121871=DIRECTION('center_axis',(0.,4.8455963016112E-16,1.)) ;
#121872=DIRECTION('ref_axis',(0.,-1.,4.8455963016112E-16)) ;
#121873=DIRECTION('',(0.,4.8455963016112E-16,1.)) ;
#121874=DIRECTION('center_axis',(0.,0.,-1.)) ;
#121875=DIRECTION('ref_axis',(-1.,0.,0.)) ;
#121876=DIRECTION('center_axis',(0.,0.,-1.)) ;
#121877=DIRECTION('ref_axis',(-1.,0.,0.)) ;
#121878=DIRECTION('center_axis',(0.,0.,1.)) ;
#121879=DIRECTION('ref_axis',(1.,0.,0.)) ;
#121880=DIRECTION('center_axis',(0.,0.,1.)) ;
#121881=DIRECTION('ref_axis',(1.,0.,0.)) ;
#121882=DIRECTION('center_axis',(-1.,-2.47817639425258E-16,0.)) ;
#121883=DIRECTION('ref_axis',(2.47817639425258E-16,-1.,0.)) ;
#121884=DIRECTION('',(2.47817639425258E-16,-1.,0.)) ;
#121885=DIRECTION('',(0.,0.,1.)) ;
#121886=DIRECTION('',(-2.47817639425258E-16,1.,0.)) ;
#121887=DIRECTION('',(0.,0.,-1.)) ;
#121888=DIRECTION('',(0.,0.,-1.)) ;
#121889=DIRECTION('',(-2.47817639425258E-16,1.,0.)) ;
#121890=DIRECTION('',(0.,0.,1.)) ;
#121891=DIRECTION('',(2.47817639425258E-16,-1.,0.)) ;
#121892=DIRECTION('',(0.,0.,-1.)) ;
#121893=DIRECTION('',(-2.47817639425258E-16,1.,0.)) ;
#121894=DIRECTION('',(0.,0.,1.)) ;
#121895=DIRECTION('',(2.47817639425258E-16,-1.,0.)) ;
#121896=DIRECTION('',(0.,0.,-1.)) ;
#121897=DIRECTION('',(-2.47817639425258E-16,1.,0.)) ;
#121898=DIRECTION('',(0.,0.,1.)) ;
#121899=DIRECTION('',(2.47817639425258E-16,-1.,0.)) ;
#121900=DIRECTION('',(0.,0.,-1.)) ;
#121901=DIRECTION('',(-2.47817639425258E-16,1.,0.)) ;
#121902=DIRECTION('',(0.,0.,1.)) ;
#121903=DIRECTION('',(2.47817639425258E-16,-1.,0.)) ;
#121904=DIRECTION('',(0.,0.,-1.)) ;
#121905=DIRECTION('',(-2.47817639425258E-16,1.,0.)) ;
#121906=DIRECTION('',(0.,0.,1.)) ;
#121907=DIRECTION('',(2.47817639425258E-16,-1.,0.)) ;
#121908=DIRECTION('',(0.,0.,-1.)) ;
#121909=DIRECTION('',(-2.47817639425258E-16,1.,0.)) ;
#121910=DIRECTION('',(0.,0.,1.)) ;
#121911=DIRECTION('',(2.47817639425258E-16,-1.,0.)) ;
#121912=DIRECTION('',(0.,0.,-1.)) ;
#121913=DIRECTION('',(-2.47817639425258E-16,1.,0.)) ;
#121914=DIRECTION('',(0.,0.,1.)) ;
#121915=DIRECTION('',(2.47817639425258E-16,-1.,0.)) ;
#121916=DIRECTION('',(0.,0.,-1.)) ;
#121917=DIRECTION('',(-2.47817639425258E-16,1.,0.)) ;
#121918=DIRECTION('',(0.,0.,1.)) ;
#121919=DIRECTION('',(2.47817639425258E-16,-1.,0.)) ;
#121920=DIRECTION('',(0.,0.,-1.)) ;
#121921=DIRECTION('',(-2.47817639425258E-16,1.,0.)) ;
#121922=DIRECTION('',(0.,0.,1.)) ;
#121923=DIRECTION('',(2.47817639425258E-16,-1.,0.)) ;
#121924=DIRECTION('',(0.,0.,-1.)) ;
#121925=DIRECTION('',(-2.47817639425258E-16,1.,0.)) ;
#121926=DIRECTION('',(0.,0.,1.)) ;
#121927=DIRECTION('',(2.47817639425258E-16,-1.,0.)) ;
#121928=DIRECTION('center_axis',(0.,-1.,0.)) ;
#121929=DIRECTION('ref_axis',(0.,0.,-1.)) ;
#121930=DIRECTION('',(0.,0.,-1.)) ;
#121931=DIRECTION('',(-1.,0.,-7.01133629567814E-33)) ;
#121932=DIRECTION('',(0.,0.,1.)) ;
#121933=DIRECTION('',(1.,0.,-7.01133629567814E-33)) ;
#121934=DIRECTION('',(0.,0.,1.)) ;
#121935=DIRECTION('center_axis',(0.,-1.,0.)) ;
#121936=DIRECTION('ref_axis',(0.,0.,-1.)) ;
#121937=DIRECTION('',(-1.,0.,0.)) ;
#121938=DIRECTION('center_axis',(0.,-1.,0.)) ;
#121939=DIRECTION('ref_axis',(0.,0.,-1.)) ;
#121940=DIRECTION('',(0.,0.,-1.)) ;
#121941=DIRECTION('center_axis',(0.,-1.,0.)) ;
#121942=DIRECTION('ref_axis',(0.,0.,-1.)) ;
#121943=DIRECTION('',(1.,0.,0.)) ;
#121944=DIRECTION('center_axis',(0.,-1.,0.)) ;
#121945=DIRECTION('ref_axis',(0.,0.,-1.)) ;
#121946=DIRECTION('center_axis',(1.,7.81406971160724E-17,0.)) ;
#121947=DIRECTION('ref_axis',(-7.81406971160724E-17,1.,0.)) ;
#121948=DIRECTION('',(-7.81406971160724E-17,1.,-1.10147335281612E-31)) ;
#121949=DIRECTION('',(0.,0.,1.)) ;
#121950=DIRECTION('',(7.81406971160724E-17,-1.,0.)) ;
#121951=DIRECTION('',(0.,0.,-1.)) ;
#121952=DIRECTION('center_axis',(1.31418445149758E-16,1.,0.)) ;
#121953=DIRECTION('ref_axis',(-1.,1.31418445149758E-16,0.)) ;
#121954=DIRECTION('',(0.422618261740697,-5.55398348498559E-17,-0.906307787036651)) ;
#121955=DIRECTION('center_axis',(1.,0.,0.)) ;
#121956=DIRECTION('ref_axis',(0.,0.,-1.)) ;
#121957=DIRECTION('',(0.,-1.,-8.9727076343628E-17)) ;
#121958=DIRECTION('',(0.,0.,-1.)) ;
#121959=DIRECTION('',(0.,1.,-8.9727076343628E-17)) ;
#121960=DIRECTION('',(0.,0.,1.)) ;
#121961=DIRECTION('center_axis',(1.,0.,0.)) ;
#121962=DIRECTION('ref_axis',(0.,0.,-1.)) ;
#121963=DIRECTION('center_axis',(1.,0.,0.)) ;
#121964=DIRECTION('ref_axis',(0.,0.,-1.)) ;
#121965=DIRECTION('center_axis',(1.,0.,0.)) ;
#121966=DIRECTION('ref_axis',(0.,0.,-1.)) ;
#121967=DIRECTION('',(0.,0.,1.)) ;
#121968=DIRECTION('center_axis',(0.,1.,0.)) ;
#121969=DIRECTION('ref_axis',(0.,0.,1.)) ;
#121970=DIRECTION('',(0.,0.,-1.)) ;
#121971=DIRECTION('',(-1.,0.,0.)) ;
#121972=DIRECTION('',(0.,0.,1.)) ;
#121973=DIRECTION('',(1.,0.,0.)) ;
#121974=DIRECTION('center_axis',(-0.89708903366019,0.441849822549049,0.)) ;
#121975=DIRECTION('ref_axis',(-0.441849822549049,-0.89708903366019,0.)) ;
#121976=DIRECTION('',(0.441849822549049,0.89708903366019,0.)) ;
#121977=DIRECTION('',(-0.441849822549049,-0.89708903366019,0.)) ;
#121978=DIRECTION('',(0.,0.,1.)) ;
#121979=DIRECTION('center_axis',(-1.,0.,0.)) ;
#121980=DIRECTION('ref_axis',(0.,0.,1.)) ;
#121981=DIRECTION('',(0.,-1.,0.)) ;
#121982=DIRECTION('',(0.,0.,1.)) ;
#121983=DIRECTION('',(0.,1.,0.)) ;
#121984=DIRECTION('',(0.,0.,-1.)) ;
#121985=DIRECTION('center_axis',(0.,-1.,0.)) ;
#121986=DIRECTION('ref_axis',(0.,0.,-1.)) ;
#121987=DIRECTION('',(1.,0.,0.)) ;
#121988=DIRECTION('',(0.,0.,1.)) ;
#121989=DIRECTION('',(-1.,0.,0.)) ;
#121990=DIRECTION('',(0.,0.,-1.)) ;
#121991=DIRECTION('',(0.,0.,1.)) ;
#121992=DIRECTION('',(1.,0.,-2.16840434497101E-16)) ;
#121993=DIRECTION('',(2.16840434497101E-16,0.,-1.)) ;
#121994=DIRECTION('',(-1.,0.,-2.16840434497101E-16)) ;
#121995=DIRECTION('',(0.,0.,1.)) ;
#121996=DIRECTION('',(1.,0.,-2.16840434497101E-16)) ;
#121997=DIRECTION('',(2.16840434497101E-16,0.,-1.)) ;
#121998=DIRECTION('',(-1.,0.,-2.16840434497101E-16)) ;
#121999=DIRECTION('',(0.,0.,1.)) ;
#122000=DIRECTION('',(1.,0.,-2.16840434497101E-16)) ;
#122001=DIRECTION('',(2.16840434497101E-16,0.,-1.)) ;
#122002=DIRECTION('',(-1.,0.,-2.16840434497101E-16)) ;
#122003=DIRECTION('',(0.,0.,1.)) ;
#122004=DIRECTION('',(1.,0.,-2.16840434497101E-16)) ;
#122005=DIRECTION('',(2.16840434497101E-16,0.,-1.)) ;
#122006=DIRECTION('',(-1.,0.,-2.16840434497101E-16)) ;
#122007=DIRECTION('',(0.,0.,1.)) ;
#122008=DIRECTION('',(1.,0.,-2.16840434497101E-16)) ;
#122009=DIRECTION('',(2.16840434497101E-16,0.,-1.)) ;
#122010=DIRECTION('',(-1.,0.,-2.16840434497101E-16)) ;
#122011=DIRECTION('',(0.,0.,1.)) ;
#122012=DIRECTION('',(1.,0.,-2.16840434497101E-16)) ;
#122013=DIRECTION('',(2.16840434497101E-16,0.,-1.)) ;
#122014=DIRECTION('',(-1.,0.,-2.16840434497101E-16)) ;
#122015=DIRECTION('',(0.,0.,1.)) ;
#122016=DIRECTION('',(1.,0.,-2.16840434497101E-16)) ;
#122017=DIRECTION('',(2.16840434497101E-16,0.,-1.)) ;
#122018=DIRECTION('',(-1.,0.,-2.16840434497101E-16)) ;
#122019=DIRECTION('',(0.,0.,1.)) ;
#122020=DIRECTION('',(1.,0.,-2.16840434497101E-16)) ;
#122021=DIRECTION('',(2.16840434497101E-16,0.,-1.)) ;
#122022=DIRECTION('',(-1.,0.,-2.16840434497101E-16)) ;
#122023=DIRECTION('center_axis',(0.,-1.,0.)) ;
#122024=DIRECTION('ref_axis',(0.,0.,-1.)) ;
#122025=DIRECTION('',(-1.,0.,-2.16840434497101E-16)) ;
#122026=DIRECTION('center_axis',(0.,-1.,0.)) ;
#122027=DIRECTION('ref_axis',(0.,0.,-1.)) ;
#122028=DIRECTION('',(0.,0.,1.)) ;
#122029=DIRECTION('center_axis',(0.,-1.,0.)) ;
#122030=DIRECTION('ref_axis',(0.,0.,-1.)) ;
#122031=DIRECTION('',(1.,0.,-2.16840434497101E-16)) ;
#122032=DIRECTION('center_axis',(0.,-1.,0.)) ;
#122033=DIRECTION('ref_axis',(0.,0.,-1.)) ;
#122034=DIRECTION('',(2.16840434497101E-16,0.,-1.)) ;
#122035=DIRECTION('center_axis',(0.,-1.,0.)) ;
#122036=DIRECTION('ref_axis',(0.,0.,-1.)) ;
#122037=DIRECTION('',(-1.,0.,-2.16840434497101E-16)) ;
#122038=DIRECTION('center_axis',(0.,-1.,0.)) ;
#122039=DIRECTION('ref_axis',(0.,0.,-1.)) ;
#122040=DIRECTION('',(0.,0.,1.)) ;
#122041=DIRECTION('center_axis',(0.,-1.,0.)) ;
#122042=DIRECTION('ref_axis',(0.,0.,-1.)) ;
#122043=DIRECTION('',(1.,0.,-2.16840434497101E-16)) ;
#122044=DIRECTION('center_axis',(0.,-1.,0.)) ;
#122045=DIRECTION('ref_axis',(0.,0.,-1.)) ;
#122046=DIRECTION('',(2.16840434497101E-16,0.,-1.)) ;
#122047=DIRECTION('center_axis',(0.,0.,-1.)) ;
#122048=DIRECTION('ref_axis',(-1.,0.,0.)) ;
#122049=DIRECTION('',(0.,1.,0.)) ;
#122050=DIRECTION('',(1.,1.31418445149758E-16,0.)) ;
#122051=DIRECTION('',(7.81406971160724E-17,-1.,0.)) ;
#122052=DIRECTION('center_axis',(0.,0.,-1.)) ;
#122053=DIRECTION('ref_axis',(-1.,0.,0.)) ;
#122054=DIRECTION('',(1.,7.81406971160724E-17,0.)) ;
#122055=DIRECTION('',(0.,-1.,0.)) ;
#122056=DIRECTION('',(-1.,-7.81406971160724E-17,0.)) ;
#122057=DIRECTION('center_axis',(0.,0.,1.)) ;
#122058=DIRECTION('ref_axis',(-1.,-3.25260651745651E-15,0.)) ;
#122059=DIRECTION('',(7.81406971160724E-17,-1.,0.)) ;
#122060=DIRECTION('',(-1.,0.,0.)) ;
#122061=DIRECTION('',(-2.47817639425258E-16,1.,0.)) ;
#122062=DIRECTION('',(1.,0.,0.)) ;
#122063=DIRECTION('center_axis',(0.,0.,-1.)) ;
#122064=DIRECTION('ref_axis',(-1.,0.,0.)) ;
#122065=DIRECTION('',(0.441849822549049,0.89708903366019,0.)) ;
#122066=DIRECTION('',(-1.,0.,0.)) ;
#122067=DIRECTION('center_axis',(0.,0.,-1.)) ;
#122068=DIRECTION('ref_axis',(-1.,0.,0.)) ;
#122069=DIRECTION('',(-7.81406971160724E-17,1.,0.)) ;
#122070=DIRECTION('',(-1.,-1.31418445149758E-16,0.)) ;
#122071=DIRECTION('',(0.,-1.,0.)) ;
#122072=DIRECTION('',(1.,0.,0.)) ;
#122073=DIRECTION('',(-0.441849822549049,-0.89708903366019,0.)) ;
#122074=DIRECTION('center_axis',(0.,0.,1.)) ;
#122075=DIRECTION('ref_axis',(-1.,0.,0.)) ;
#122076=DIRECTION('',(-1.,0.,0.)) ;
#122077=DIRECTION('',(2.47817639425258E-16,-1.,0.)) ;
#122078=DIRECTION('',(1.,0.,0.)) ;
#122079=DIRECTION('',(-7.81406971160724E-17,1.,0.)) ;
#122080=DIRECTION('center_axis',(0.,0.,-1.)) ;
#122081=DIRECTION('ref_axis',(-1.,0.,0.)) ;
#122082=DIRECTION('',(1.,7.81406971160724E-17,0.)) ;
#122083=DIRECTION('',(0.,1.,0.)) ;
#122084=DIRECTION('',(-1.,-7.81406971160724E-17,0.)) ;
#122085=DIRECTION('center_axis',(0.,0.,1.)) ;
#122086=DIRECTION('ref_axis',(-1.,0.,0.)) ;
#122087=DIRECTION('center_axis',(0.,0.,-1.)) ;
#122088=DIRECTION('ref_axis',(-1.,0.,0.)) ;
#122089=DIRECTION('',(0.970142500145333,0.24253562503633,0.)) ;
#122090=DIRECTION('',(0.,1.,0.)) ;
#122091=DIRECTION('',(-0.707106781186548,0.707106781186547,0.)) ;
#122092=DIRECTION('',(2.47817639425258E-16,-1.,0.)) ;
#122093=DIRECTION('center_axis',(0.432731067584771,0.,-0.901523057468274)) ;
#122094=DIRECTION('ref_axis',(-0.901523057468274,0.,-0.432731067584771)) ;
#122095=DIRECTION('',(0.,-1.,0.)) ;
#122096=DIRECTION('',(0.879462917689188,0.219865729422294,0.42214220049081)) ;
#122097=DIRECTION('',(0.,1.,0.)) ;
#122098=DIRECTION('',(-0.669589480006975,0.669589480006975,-0.321402950403348)) ;
#122099=DIRECTION('center_axis',(1.,0.,0.)) ;
#122100=DIRECTION('ref_axis',(0.,0.,-1.)) ;
#122101=DIRECTION('',(0.,0.,-1.)) ;
#122102=DIRECTION('center_axis',(-1.,-1.41117851341148E-14,1.31136401905241E-14)) ;
#122103=DIRECTION('ref_axis',(-1.81493914443541E-14,0.461934418837058,-0.886914084166933)) ;
#122104=DIRECTION('',(0.,1.,0.)) ;
#122105=DIRECTION('center_axis',(-1.,0.,0.)) ;
#122106=DIRECTION('ref_axis',(0.,0.901523057468499,0.432731067584301)) ;
#122107=DIRECTION('',(0.,0.,-1.)) ;
#122108=DIRECTION('center_axis',(-1.,-1.26549640056948E-14,1.61343974433662E-14)) ;
#122109=DIRECTION('ref_axis',(-1.83905968730662E-14,0.901523057468445,-0.432731067584414)) ;
#122110=DIRECTION('center_axis',(-1.,-1.41117851341149E-14,-1.31136401905241E-14)) ;
#122111=DIRECTION('ref_axis',(1.81493914443479E-14,-0.4619344188362,-0.88691408416738)) ;
#122112=DIRECTION('center_axis',(0.432731067584771,0.,0.901523057468274)) ;
#122113=DIRECTION('ref_axis',(0.901523057468274,0.,-0.432731067584771)) ;
#122114=DIRECTION('',(-0.879462917689188,-0.219865729422294,0.42214220049081)) ;
#122115=DIRECTION('',(0.,1.,0.)) ;
#122116=DIRECTION('',(0.669589480006975,-0.669589480006975,-0.321402950403348)) ;
#122117=DIRECTION('center_axis',(0.,0.,1.)) ;
#122118=DIRECTION('ref_axis',(1.,0.,0.)) ;
#122119=DIRECTION('',(0.,-1.,0.)) ;
#122120=DIRECTION('',(-0.970142500145333,-0.24253562503633,0.)) ;
#122121=DIRECTION('',(-2.47817639425258E-16,1.,0.)) ;
#122122=DIRECTION('',(0.707106781186548,-0.707106781186547,0.)) ;
#122123=DIRECTION('center_axis',(0.24253562503633,-0.970142500145333,0.)) ;
#122124=DIRECTION('ref_axis',(0.,0.,1.)) ;
#122125=DIRECTION('',(0.970142500145333,0.24253562503633,0.)) ;
#122126=DIRECTION('',(0.879462917689188,0.219865729422294,-0.42214220049081)) ;
#122127=DIRECTION('',(-0.879462917689188,-0.219865729422294,-0.42214220049081)) ;
#122128=DIRECTION('',(-0.970142500145333,-0.24253562503633,0.)) ;
#122129=DIRECTION('',(0.,0.,1.)) ;
#122130=DIRECTION('center_axis',(-0.707106781186547,-0.707106781186548,
0.)) ;
#122131=DIRECTION('ref_axis',(0.,0.,-1.)) ;
#122132=DIRECTION('',(0.707106781186548,-0.707106781186547,0.)) ;
#122133=DIRECTION('',(0.669589480006975,-0.669589480006975,0.321402950403348)) ;
#122134=DIRECTION('',(-0.669589480006975,0.669589480006975,0.321402950403348)) ;
#122135=DIRECTION('',(-0.707106781186548,0.707106781186547,0.)) ;
#122136=DIRECTION('',(0.,0.,-1.)) ;
#122137=DIRECTION('center_axis',(1.,0.,2.16840434497101E-16)) ;
#122138=DIRECTION('ref_axis',(2.16840434497101E-16,0.,-1.)) ;
#122139=DIRECTION('',(2.16840434497101E-16,0.,-1.)) ;
#122140=DIRECTION('',(0.,-1.,0.)) ;
#122141=DIRECTION('',(-2.16840434497101E-16,0.,1.)) ;
#122142=DIRECTION('',(0.,1.,0.)) ;
#122143=DIRECTION('center_axis',(2.16840434497101E-16,0.,-1.)) ;
#122144=DIRECTION('ref_axis',(-1.,0.,-2.16840434497101E-16)) ;
#122145=DIRECTION('',(-1.,0.,-2.16840434497101E-16)) ;
#122146=DIRECTION('',(0.,-1.,0.)) ;
#122147=DIRECTION('',(1.,0.,2.16840434497101E-16)) ;
#122148=DIRECTION('',(0.,1.,0.)) ;
#122149=DIRECTION('center_axis',(-1.,0.,0.)) ;
#122150=DIRECTION('ref_axis',(0.,0.,1.)) ;
#122151=DIRECTION('',(0.,1.,0.)) ;
#122152=DIRECTION('',(0.,0.,1.)) ;
#122153=DIRECTION('',(0.,-1.,0.)) ;
#122154=DIRECTION('',(0.,0.,-1.)) ;
#122155=DIRECTION('center_axis',(2.16840434497101E-16,0.,1.)) ;
#122156=DIRECTION('ref_axis',(1.,0.,-2.16840434497101E-16)) ;
#122157=DIRECTION('',(0.,1.,0.)) ;
#122158=DIRECTION('',(1.,0.,-2.16840434497101E-16)) ;
#122159=DIRECTION('',(0.,-1.,0.)) ;
#122160=DIRECTION('',(-1.,0.,2.16840434497101E-16)) ;
#122161=DIRECTION('center_axis',(0.,-1.,0.)) ;
#122162=DIRECTION('ref_axis',(0.,0.,-1.)) ;
#122163=DIRECTION('',(0.,0.,-1.)) ;
#122164=DIRECTION('',(1.,0.,2.16840434497101E-16)) ;
#122165=DIRECTION('',(-2.16840434497101E-16,0.,1.)) ;
#122166=DIRECTION('',(-1.,0.,2.16840434497101E-16)) ;
#122167=DIRECTION('',(1.,0.,0.)) ;
#122168=DIRECTION('center_axis',(0.,1.,0.)) ;
#122169=DIRECTION('ref_axis',(0.,0.,-1.)) ;
#122170=DIRECTION('',(0.,0.,-1.)) ;
#122171=DIRECTION('center_axis',(0.,1.,0.)) ;
#122172=DIRECTION('ref_axis',(0.,0.,-1.)) ;
#122173=DIRECTION('',(-1.,0.,0.)) ;
#122174=DIRECTION('center_axis',(0.,1.,0.)) ;
#122175=DIRECTION('ref_axis',(0.,0.,-1.)) ;
#122176=DIRECTION('',(0.,0.,1.)) ;
#122177=DIRECTION('center_axis',(0.,1.,0.)) ;
#122178=DIRECTION('ref_axis',(0.,0.,-1.)) ;
#122179=DIRECTION('center_axis',(1.,0.,0.)) ;
#122180=DIRECTION('ref_axis',(0.,0.,-1.)) ;
#122181=DIRECTION('',(0.,-1.,0.)) ;
#122182=DIRECTION('',(0.,0.,-1.)) ;
#122183=DIRECTION('',(0.,1.,0.)) ;
#122184=DIRECTION('center_axis',(0.,0.,-1.)) ;
#122185=DIRECTION('ref_axis',(-1.,0.,0.)) ;
#122186=DIRECTION('',(0.,-1.,0.)) ;
#122187=DIRECTION('',(-1.,0.,0.)) ;
#122188=DIRECTION('',(0.,1.,0.)) ;
#122189=DIRECTION('center_axis',(-1.,0.,0.)) ;
#122190=DIRECTION('ref_axis',(0.,0.,1.)) ;
#122191=DIRECTION('',(0.,0.,1.)) ;
#122192=DIRECTION('',(0.,1.,0.)) ;
#122193=DIRECTION('',(0.,-1.,0.)) ;
#122194=DIRECTION('center_axis',(0.,0.,1.)) ;
#122195=DIRECTION('ref_axis',(1.,0.,0.)) ;
#122196=DIRECTION('',(0.,-1.,0.)) ;
#122197=DIRECTION('',(1.,0.,0.)) ;
#122198=DIRECTION('',(0.,1.,0.)) ;
#122199=DIRECTION('center_axis',(0.,-1.,0.)) ;
#122200=DIRECTION('ref_axis',(0.,0.,-1.)) ;
#122201=DIRECTION('',(-1.,0.,0.)) ;
#122202=DIRECTION('',(0.,0.,-1.)) ;
#122203=DIRECTION('',(1.,0.,0.)) ;
#122204=DIRECTION('',(0.,0.,1.)) ;
#122205=DIRECTION('center_axis',(7.81406971160724E-17,-1.,0.)) ;
#122206=DIRECTION('ref_axis',(1.,7.81406971160724E-17,0.)) ;
#122207=DIRECTION('',(-1.,-7.81406971160724E-17,0.)) ;
#122208=DIRECTION('',(0.,0.,1.)) ;
#122209=DIRECTION('center_axis',(-7.81406971160724E-17,1.,0.)) ;
#122210=DIRECTION('ref_axis',(1.,7.81406971160724E-17,0.)) ;
#122211=DIRECTION('',(-1.,-7.81406971160724E-17,0.)) ;
#122212=DIRECTION('',(1.,7.81406971160724E-17,5.2561455487295E-16)) ;
#122213=DIRECTION('center_axis',(-7.81406971160724E-17,1.,0.)) ;
#122214=DIRECTION('ref_axis',(1.,7.81406971160724E-17,0.)) ;
#122215=DIRECTION('',(0.,0.,1.)) ;
#122216=DIRECTION('',(1.,7.81406971160724E-17,0.)) ;
#122217=DIRECTION('center_axis',(-7.81406971160724E-17,1.,4.8455963016112E-16)) ;
#122218=DIRECTION('ref_axis',(-2.5241768025713E-48,-4.8455963016112E-16,
1.)) ;
#122219=DIRECTION('',(0.,-4.8455963016112E-16,1.)) ;
#122220=DIRECTION('',(-1.,-7.81406971160724E-17,0.)) ;
#122221=DIRECTION('',(-3.78638272950961E-32,4.8455963016112E-16,-1.)) ;
#122222=DIRECTION('',(1.,7.81406971160724E-17,0.)) ;
#122223=DIRECTION('center_axis',(-7.01133629567814E-33,8.97270763436279E-17,
-1.)) ;
#122224=DIRECTION('ref_axis',(-6.83680877694706E-64,1.,8.97270763436279E-17)) ;
#122225=DIRECTION('center_axis',(-7.01133629567814E-33,8.97270763436279E-17,
-1.)) ;
#122226=DIRECTION('ref_axis',(6.29106707073161E-49,1.,8.97270763436279E-17)) ;
#122227=DIRECTION('center_axis',(-7.01133629567814E-33,8.97270763436279E-17,
-1.)) ;
#122228=DIRECTION('ref_axis',(6.29106707073161E-49,1.,8.97270763436279E-17)) ;
#122229=DIRECTION('',(-1.,-7.81406971160724E-17,0.)) ;
#122230=DIRECTION('',(7.81406971160724E-17,-1.,-8.9727076343628E-17)) ;
#122231=DIRECTION('',(1.,7.81406971160724E-17,0.)) ;
#122232=DIRECTION('',(0.,1.,8.9727076343628E-17)) ;
#122233=DIRECTION('center_axis',(7.01133629567814E-33,-8.97270763436279E-17,
1.)) ;
#122234=DIRECTION('ref_axis',(6.29106707073161E-49,1.,8.97270763436279E-17)) ;
#122235=DIRECTION('',(1.,0.,-7.01133629567814E-33)) ;
#122236=DIRECTION('',(0.,1.,8.9727076343628E-17)) ;
#122237=DIRECTION('',(-1.,0.,7.01133629567814E-33)) ;
#122238=DIRECTION('center_axis',(-7.81406971160724E-17,1.,0.)) ;
#122239=DIRECTION('ref_axis',(-1.,-7.81406971160724E-17,0.)) ;
#122240=DIRECTION('',(-1.,-7.81406971160724E-17,0.)) ;
#122241=DIRECTION('',(0.,0.,-1.)) ;
#122242=DIRECTION('',(1.,7.81406971160724E-17,0.)) ;
#122243=DIRECTION('',(0.,0.,1.)) ;
#122244=DIRECTION('center_axis',(-7.01133629567814E-33,8.97270763436279E-17,
1.)) ;
#122245=DIRECTION('ref_axis',(6.83680877694706E-64,-1.,8.97270763436279E-17)) ;
#122246=DIRECTION('',(1.,7.81406971160724E-17,0.)) ;
#122247=DIRECTION('center_axis',(-7.01133629567814E-33,8.97270763436279E-17,
1.)) ;
#122248=DIRECTION('ref_axis',(-6.29106707073161E-49,-1.,8.97270763436279E-17)) ;
#122249=DIRECTION('center_axis',(-7.01133629567814E-33,8.97270763436279E-17,
1.)) ;
#122250=DIRECTION('ref_axis',(-6.29106707073161E-49,-1.,8.97270763436279E-17)) ;
#122251=DIRECTION('',(1.,0.,7.01133629567814E-33)) ;
#122252=DIRECTION('',(0.,-1.,8.9727076343628E-17)) ;
#122253=DIRECTION('',(-1.,0.,-7.01133629567814E-33)) ;
#122254=DIRECTION('center_axis',(7.01133629567814E-33,-8.97270763436279E-17,
-1.)) ;
#122255=DIRECTION('ref_axis',(-6.29106707073161E-49,-1.,8.97270763436279E-17)) ;
#122256=DIRECTION('',(0.,-1.,8.9727076343628E-17)) ;
#122257=DIRECTION('',(-1.,-7.81406971160724E-17,0.)) ;
#122258=DIRECTION('',(-7.81406971160724E-17,1.,-8.9727076343628E-17)) ;
#122259=DIRECTION('center_axis',(-7.81406971160724E-17,1.,-4.8455963016112E-16)) ;
#122260=DIRECTION('ref_axis',(2.5241768025713E-48,4.8455963016112E-16,1.)) ;
#122261=DIRECTION('',(1.,7.81406971160724E-17,0.)) ;
#122262=DIRECTION('',(-1.,-7.81406971160724E-17,0.)) ;
#122263=DIRECTION('',(3.78638272950961E-32,-4.8455963016112E-16,-1.)) ;
#122264=DIRECTION('center_axis',(0.,1.,0.)) ;
#122265=DIRECTION('ref_axis',(0.,0.,1.)) ;
#122266=DIRECTION('',(-1.,0.,0.)) ;
#122267=DIRECTION('',(0.,0.,-1.)) ;
#122268=DIRECTION('',(1.,0.,7.01133629567814E-33)) ;
#122269=DIRECTION('',(0.,0.,1.)) ;
#122270=DIRECTION('center_axis',(0.,1.,0.)) ;
#122271=DIRECTION('ref_axis',(0.,0.,1.)) ;
#122272=DIRECTION('',(-1.,0.,7.01133629567814E-33)) ;
#122273=DIRECTION('',(0.,0.,-1.)) ;
#122274=DIRECTION('',(1.,0.,0.)) ;
#122275=DIRECTION('',(0.,0.,1.)) ;
#122276=DIRECTION('center_axis',(-1.,0.,0.)) ;
#122277=DIRECTION('ref_axis',(0.,0.,1.)) ;
#122278=DIRECTION('',(-1.,0.,0.)) ;
#122279=DIRECTION('center_axis',(-1.,0.,0.)) ;
#122280=DIRECTION('ref_axis',(0.,0.,-1.)) ;
#122281=DIRECTION('',(1.,0.,0.)) ;
#122282=DIRECTION('center_axis',(1.,0.,0.)) ;
#122283=DIRECTION('ref_axis',(0.,0.,-1.)) ;
#122284=DIRECTION('center_axis',(1.,0.,0.)) ;
#122285=DIRECTION('ref_axis',(0.,0.,-1.)) ;
#122286=DIRECTION('',(0.,0.,-1.)) ;
#122287=DIRECTION('center_axis',(-1.,0.,0.)) ;
#122288=DIRECTION('ref_axis',(0.,0.,-1.)) ;
#122289=DIRECTION('',(0.,0.,-1.)) ;
#122290=DIRECTION('',(0.,1.,-8.9727076343628E-17)) ;
#122291=DIRECTION('',(0.,0.,1.)) ;
#122292=DIRECTION('',(0.,-1.,-8.9727076343628E-17)) ;
#122293=DIRECTION('center_axis',(1.,0.,0.)) ;
#122294=DIRECTION('ref_axis',(0.,0.,-1.)) ;
#122295=DIRECTION('center_axis',(1.,-1.31418445149758E-16,-2.16840434497101E-16)) ;
#122296=DIRECTION('ref_axis',(-2.16840434497101E-16,0.,-1.)) ;
#122297=DIRECTION('',(2.16840434497101E-16,0.,1.)) ;
#122298=DIRECTION('',(1.31418445149758E-16,1.,0.)) ;
#122299=DIRECTION('',(-2.16840434497101E-16,-2.8496832747207E-32,-1.)) ;
#122300=DIRECTION('',(-1.31418445149758E-16,-1.,0.)) ;
#122301=DIRECTION('center_axis',(-2.16840434497101E-16,2.8496832747207E-32,
1.)) ;
#122302=DIRECTION('ref_axis',(1.,4.92915281362991E-64,2.16840434497101E-16)) ;
#122303=DIRECTION('',(1.,1.31418445149758E-16,2.16840434497101E-16)) ;
#122304=DIRECTION('',(-1.31418445149758E-16,-1.,0.)) ;
#122305=DIRECTION('',(-1.,0.,-2.16840434497101E-16)) ;
#122306=DIRECTION('',(1.31418445149758E-16,1.,0.)) ;
#122307=DIRECTION('center_axis',(-1.,1.31418445149758E-16,4.33680868994202E-16)) ;
#122308=DIRECTION('ref_axis',(4.33680868994202E-16,0.,1.)) ;
#122309=DIRECTION('',(-1.31418445149758E-16,-1.,0.)) ;
#122310=DIRECTION('',(-4.33680868994202E-16,0.,-1.)) ;
#122311=DIRECTION('',(1.31418445149758E-16,1.,0.)) ;
#122312=DIRECTION('',(4.33680868994202E-16,5.69936654944139E-32,1.)) ;
#122313=DIRECTION('center_axis',(-2.16840434497101E-16,2.8496832747207E-32,
-1.)) ;
#122314=DIRECTION('ref_axis',(-1.,-4.92915281362991E-64,2.16840434497101E-16)) ;
#122315=DIRECTION('',(1.,0.,-2.16840434497101E-16)) ;
#122316=DIRECTION('',(1.31418445149758E-16,1.,0.)) ;
#122317=DIRECTION('',(-1.,-1.31418445149758E-16,2.16840434497101E-16)) ;
#122318=DIRECTION('',(-1.31418445149758E-16,-1.,0.)) ;
#122319=DIRECTION('center_axis',(0.,1.,0.)) ;
#122320=DIRECTION('ref_axis',(0.,0.,1.)) ;
#122321=DIRECTION('',(4.33680868994202E-16,0.,1.)) ;
#122322=DIRECTION('',(1.,0.,2.16840434497101E-16)) ;
#122323=DIRECTION('',(-2.16840434497101E-16,0.,-1.)) ;
#122324=DIRECTION('',(-1.,0.,2.16840434497101E-16)) ;
#122325=DIRECTION('',(1.,0.,0.)) ;
#122326=DIRECTION('center_axis',(0.,-1.,0.)) ;
#122327=DIRECTION('ref_axis',(0.,0.,1.)) ;
#122328=DIRECTION('',(0.,0.,1.)) ;
#122329=DIRECTION('center_axis',(0.,-1.,0.)) ;
#122330=DIRECTION('ref_axis',(0.,0.,1.)) ;
#122331=DIRECTION('',(-1.,0.,0.)) ;
#122332=DIRECTION('center_axis',(0.,-1.,0.)) ;
#122333=DIRECTION('ref_axis',(0.,0.,1.)) ;
#122334=DIRECTION('',(0.,0.,-1.)) ;
#122335=DIRECTION('center_axis',(0.,-1.,0.)) ;
#122336=DIRECTION('ref_axis',(0.,0.,1.)) ;
#122337=DIRECTION('center_axis',(1.,0.,0.)) ;
#122338=DIRECTION('ref_axis',(0.,0.,-1.)) ;
#122339=DIRECTION('',(0.,0.,1.)) ;
#122340=DIRECTION('',(0.,-1.,0.)) ;
#122341=DIRECTION('',(0.,1.,0.)) ;
#122342=DIRECTION('center_axis',(0.,0.,1.)) ;
#122343=DIRECTION('ref_axis',(1.,0.,0.)) ;
#122344=DIRECTION('',(-1.,0.,0.)) ;
#122345=DIRECTION('',(0.,-1.,0.)) ;
#122346=DIRECTION('',(0.,1.,0.)) ;
#122347=DIRECTION('center_axis',(-1.,0.,0.)) ;
#122348=DIRECTION('ref_axis',(0.,0.,1.)) ;
#122349=DIRECTION('',(0.,1.,0.)) ;
#122350=DIRECTION('',(0.,0.,-1.)) ;
#122351=DIRECTION('',(0.,-1.,0.)) ;
#122352=DIRECTION('center_axis',(0.,0.,-1.)) ;
#122353=DIRECTION('ref_axis',(-1.,0.,0.)) ;
#122354=DIRECTION('',(1.,0.,0.)) ;
#122355=DIRECTION('',(0.,-1.,0.)) ;
#122356=DIRECTION('',(0.,1.,0.)) ;
#122357=DIRECTION('center_axis',(0.,1.,0.)) ;
#122358=DIRECTION('ref_axis',(0.,0.,1.)) ;
#122359=DIRECTION('',(-1.,0.,0.)) ;
#122360=DIRECTION('',(0.,0.,1.)) ;
#122361=DIRECTION('',(1.,0.,0.)) ;
#122362=DIRECTION('',(0.,0.,-1.)) ;
#122363=DIRECTION('center_axis',(1.31418445149758E-16,1.,0.)) ;
#122364=DIRECTION('ref_axis',(-1.,1.31418445149758E-16,0.)) ;
#122365=DIRECTION('',(-0.422618261740697,5.55398348498559E-17,0.906307787036651)) ;
#122366=DIRECTION('center_axis',(0.906307787036651,-1.19105560199475E-16,
0.422618261740697)) ;
#122367=DIRECTION('ref_axis',(0.422618261740697,-9.57222084411175E-33,-0.906307787036651)) ;
#122368=DIRECTION('',(0.422618261740697,-5.55398348498559E-17,-0.906307787036651)) ;
#122369=DIRECTION('',(-0.422618261740697,5.55398348498559E-17,0.906307787036651)) ;
#122370=DIRECTION('center_axis',(-0.906307787036651,1.19105560199475E-16,
-0.422618261740697)) ;
#122371=DIRECTION('ref_axis',(-0.422618261740697,9.57222084411175E-33,0.906307787036651)) ;
#122372=DIRECTION('',(0.422618261740697,-5.55398348498559E-17,-0.906307787036651)) ;
#122373=DIRECTION('',(-0.422618261740697,5.55398348498559E-17,0.906307787036651)) ;
#122374=DIRECTION('center_axis',(1.31418445149758E-16,1.,0.)) ;
#122375=DIRECTION('ref_axis',(-1.,1.31418445149758E-16,0.)) ;
#122376=DIRECTION('',(0.422618261740697,-5.55398348498559E-17,-0.906307787036651)) ;
#122377=DIRECTION('',(-0.422618261740697,5.55398348498559E-17,0.906307787036651)) ;
#122378=DIRECTION('center_axis',(1.31418445149758E-16,1.,0.)) ;
#122379=DIRECTION('ref_axis',(1.,-1.31418445149758E-16,-1.22464679914735E-16)) ;
#122380=DIRECTION('center_axis',(1.31418445149758E-16,-1.,0.)) ;
#122381=DIRECTION('ref_axis',(-1.,-1.31418445149758E-16,0.)) ;
#122382=DIRECTION('center_axis',(1.31418445149758E-16,1.,0.)) ;
#122383=DIRECTION('ref_axis',(0.990906098224775,-1.30223338718113E-16,-0.134555209861798)) ;
#122384=DIRECTION('center_axis',(1.31418445149758E-16,-1.,0.)) ;
#122385=DIRECTION('ref_axis',(-1.,-1.31418445149758E-16,8.88178419700125E-16)) ;
#122386=DIRECTION('center_axis',(-5.2561455487295E-16,6.90754475494854E-32,
1.)) ;
#122387=DIRECTION('ref_axis',(1.,-1.65558275742919E-64,5.2561455487295E-16)) ;
#122388=DIRECTION('',(1.,1.31418445149758E-16,5.2561455487295E-16)) ;
#122389=DIRECTION('',(7.81406971160724E-17,-1.,1.10147335281612E-31)) ;
#122390=DIRECTION('',(-1.,-7.81406971160724E-17,-5.2561455487295E-16)) ;
#122391=DIRECTION('center_axis',(0.,0.,-1.)) ;
#122392=DIRECTION('ref_axis',(-1.,0.,0.)) ;
#122393=DIRECTION('',(-7.81406971160724E-17,1.,0.)) ;
#122394=DIRECTION('',(-1.,-1.31418445149758E-16,0.)) ;
#122395=DIRECTION('',(1.,7.81406971160724E-17,0.)) ;
#122396=DIRECTION('center_axis',(-1.31418445149758E-16,1.,0.)) ;
#122397=DIRECTION('ref_axis',(0.990906098224775,1.30223338718113E-16,0.134555209861799)) ;
#122398=DIRECTION('center_axis',(1.31418445149758E-16,-1.,0.)) ;
#122399=DIRECTION('ref_axis',(-1.,-1.31418445149758E-16,0.)) ;
#122400=DIRECTION('center_axis',(-1.31418445149758E-16,1.,0.)) ;
#122401=DIRECTION('ref_axis',(1.,1.31418445149758E-16,7.6571373978539E-16)) ;
#122402=DIRECTION('center_axis',(1.31418445149758E-16,-1.,0.)) ;
#122403=DIRECTION('ref_axis',(-1.,-1.31418445149758E-16,-1.54197642309049E-15)) ;
#122404=DIRECTION('center_axis',(0.,-1.,0.)) ;
#122405=DIRECTION('ref_axis',(0.,0.,-1.)) ;
#122406=DIRECTION('',(0.,-1.,0.)) ;
#122407=DIRECTION('center_axis',(0.,1.,0.)) ;
#122408=DIRECTION('ref_axis',(5.20417042793044E-14,0.,-1.)) ;
#122409=DIRECTION('',(0.,-1.,0.)) ;
#122410=DIRECTION('center_axis',(0.,-1.,0.)) ;
#122411=DIRECTION('ref_axis',(0.,0.,-1.)) ;
#122412=DIRECTION('center_axis',(0.,0.,1.)) ;
#122413=DIRECTION('ref_axis',(1.,0.,0.)) ;
#122414=DIRECTION('',(-1.,0.,0.)) ;
#122415=DIRECTION('',(0.,-1.,0.)) ;
#122416=DIRECTION('',(1.,0.,0.)) ;
#122417=DIRECTION('center_axis',(0.,-1.,0.)) ;
#122418=DIRECTION('ref_axis',(0.,0.,-1.)) ;
#122419=DIRECTION('center_axis',(0.,1.,0.)) ;
#122420=DIRECTION('ref_axis',(0.,0.,-1.)) ;
#122421=DIRECTION('',(0.,-1.,0.)) ;
#122422=DIRECTION('center_axis',(0.,-1.,0.)) ;
#122423=DIRECTION('ref_axis',(0.,0.,-1.)) ;
#122424=DIRECTION('center_axis',(1.,0.,0.)) ;
#122425=DIRECTION('ref_axis',(0.,0.,-1.)) ;
#122426=DIRECTION('',(0.,0.,1.)) ;
#122427=DIRECTION('',(0.,-1.,0.)) ;
#122428=DIRECTION('',(0.,0.,-1.)) ;
#122429=DIRECTION('center_axis',(0.,-1.,0.)) ;
#122430=DIRECTION('ref_axis',(0.,0.,-1.)) ;
#122431=DIRECTION('center_axis',(0.,1.,0.)) ;
#122432=DIRECTION('ref_axis',(0.,0.,-1.)) ;
#122433=DIRECTION('',(0.,-1.,0.)) ;
#122434=DIRECTION('center_axis',(0.,-1.,0.)) ;
#122435=DIRECTION('ref_axis',(0.,0.,-1.)) ;
#122436=DIRECTION('center_axis',(0.,0.,-1.)) ;
#122437=DIRECTION('ref_axis',(-1.,0.,0.)) ;
#122438=DIRECTION('',(1.,0.,0.)) ;
#122439=DIRECTION('',(0.,-1.,0.)) ;
#122440=DIRECTION('',(-1.,0.,0.)) ;
#122441=DIRECTION('center_axis',(0.,-1.,0.)) ;
#122442=DIRECTION('ref_axis',(0.,0.,-1.)) ;
#122443=DIRECTION('center_axis',(0.,1.,0.)) ;
#122444=DIRECTION('ref_axis',(0.,0.,-1.)) ;
#122445=DIRECTION('',(0.,-1.,0.)) ;
#122446=DIRECTION('center_axis',(0.,-1.,0.)) ;
#122447=DIRECTION('ref_axis',(0.,0.,-1.)) ;
#122448=DIRECTION('center_axis',(-1.,0.,0.)) ;
#122449=DIRECTION('ref_axis',(0.,0.,1.)) ;
#122450=DIRECTION('',(0.,0.,1.)) ;
#122451=DIRECTION('',(0.,0.,-1.)) ;
#122452=DIRECTION('center_axis',(0.,-1.,0.)) ;
#122453=DIRECTION('ref_axis',(0.,0.,-1.)) ;
#122454=DIRECTION('',(1.,0.,0.)) ;
#122455=DIRECTION('',(0.,0.,-1.)) ;
#122456=DIRECTION('',(-1.,0.,0.)) ;
#122457=DIRECTION('',(0.,0.,1.)) ;
#122458=DIRECTION('center_axis',(-1.,0.,0.)) ;
#122459=DIRECTION('ref_axis',(0.,0.,1.)) ;
#122460=DIRECTION('center_axis',(-1.,0.,0.)) ;
#122461=DIRECTION('ref_axis',(0.,0.,1.)) ;
#122462=DIRECTION('center_axis',(-1.,0.,0.)) ;
#122463=DIRECTION('ref_axis',(0.,0.,1.)) ;
#122464=DIRECTION('center_axis',(0.,1.,0.)) ;
#122465=DIRECTION('ref_axis',(1.,0.,0.)) ;
#122466=DIRECTION('center_axis',(0.,0.,-1.)) ;
#122467=DIRECTION('ref_axis',(1.,0.,0.)) ;
#122468=DIRECTION('center_axis',(0.,1.,0.)) ;
#122469=DIRECTION('ref_axis',(0.,0.,-1.)) ;
#122470=DIRECTION('center_axis',(0.,0.,1.)) ;
#122471=DIRECTION('ref_axis',(1.,0.,0.)) ;
#122472=DIRECTION('center_axis',(0.,0.,1.)) ;
#122473=DIRECTION('ref_axis',(1.,0.,0.)) ;
#122474=DIRECTION('center_axis',(0.,0.,-1.)) ;
#122475=DIRECTION('ref_axis',(1.,0.,0.)) ;
#122476=DIRECTION('center_axis',(-2.47817639425258E-16,1.,0.)) ;
#122477=DIRECTION('ref_axis',(-1.,-2.47817639425258E-16,0.)) ;
#122478=DIRECTION('center_axis',(0.,1.,0.)) ;
#122479=DIRECTION('ref_axis',(0.,0.,1.)) ;
#122480=DIRECTION('center_axis',(0.,0.,1.)) ;
#122481=DIRECTION('ref_axis',(1.,0.,0.)) ;
#122482=DIRECTION('center_axis',(0.,0.,-1.)) ;
#122483=DIRECTION('ref_axis',(-1.,0.,0.)) ;
#122484=DIRECTION('center_axis',(1.,0.,0.)) ;
#122485=DIRECTION('ref_axis',(0.,0.,-1.)) ;
#122486=DIRECTION('center_axis',(-1.,0.,0.)) ;
#122487=DIRECTION('ref_axis',(0.,0.,-1.)) ;
#122488=DIRECTION('center_axis',(-1.,0.,0.)) ;
#122489=DIRECTION('ref_axis',(0.,0.,1.)) ;
#122490=DIRECTION('center_axis',(0.,1.,0.)) ;
#122491=DIRECTION('ref_axis',(0.,0.,1.)) ;
#122492=DIRECTION('center_axis',(0.,-1.,0.)) ;
#122493=DIRECTION('ref_axis',(0.,0.,1.)) ;
#122494=DIRECTION('center_axis',(0.,-1.,0.)) ;
#122495=DIRECTION('ref_axis',(0.,0.,-1.)) ;
#122496=DIRECTION('center_axis',(-1.,0.,0.)) ;
#122497=DIRECTION('ref_axis',(0.,0.,1.)) ;
#122498=DIRECTION('center_axis',(-1.,0.,0.)) ;
#122499=DIRECTION('ref_axis',(0.,0.,1.)) ;
#122500=DIRECTION('center_axis',(-0.297047844549207,0.954862596423522,-1.49073359128363E-13)) ;
#122501=DIRECTION('ref_axis',(0.954691435265115,0.296994598089069,-0.0189333604346236)) ;
#122502=DIRECTION('center_axis',(-0.297047844549074,0.954862596423564,-1.68658673018685E-12)) ;
#122503=DIRECTION('ref_axis',(0.95457509154025,0.296958404763534,0.0245377352504246)) ;
#122504=DIRECTION('center_axis',(0.,1.,0.)) ;
#122505=DIRECTION('ref_axis',(1.,0.,0.)) ;
#122506=DIRECTION('center_axis',(0.,0.,-1.)) ;
#122507=DIRECTION('ref_axis',(1.,0.,0.)) ;
#122508=DIRECTION('center_axis',(1.,0.,0.)) ;
#122509=DIRECTION('ref_axis',(0.,0.,1.)) ;
#122510=DIRECTION('center_axis',(0.,1.,0.)) ;
#122511=DIRECTION('ref_axis',(1.,0.,0.)) ;
#122512=DIRECTION('center_axis',(0.,1.,0.)) ;
#122513=DIRECTION('ref_axis',(0.,0.,-1.)) ;
#122514=DIRECTION('center_axis',(0.,0.,1.)) ;
#122515=DIRECTION('ref_axis',(1.,0.,0.)) ;
#122516=DIRECTION('center_axis',(0.,0.,-1.)) ;
#122517=DIRECTION('ref_axis',(1.,0.,0.)) ;
#122518=DIRECTION('center_axis',(0.,0.,1.)) ;
#122519=DIRECTION('ref_axis',(1.,0.,0.)) ;
#122520=DIRECTION('center_axis',(0.,0.,1.)) ;
#122521=DIRECTION('ref_axis',(1.,0.,0.)) ;
#122522=DIRECTION('center_axis',(0.,0.,-1.)) ;
#122523=DIRECTION('ref_axis',(1.,0.,0.)) ;
#122524=DIRECTION('center_axis',(-0.527647792165807,0.849457787212664,0.00304551577146026)) ;
#122525=DIRECTION('ref_axis',(0.709569539673246,0.438778321275517,0.551348032685832)) ;
#122526=DIRECTION('center_axis',(0.441849822549049,0.89708903366019,0.)) ;
#122527=DIRECTION('ref_axis',(-0.89708903366019,0.441849822549049,0.)) ;
#122528=DIRECTION('center_axis',(0.725180709343317,-0.688554584578773,0.00235007486622799)) ;
#122529=DIRECTION('ref_axis',(0.688552674549923,0.725184403719161,0.00167181716517875)) ;
#122530=DIRECTION('center_axis',(0.725344906601501,-0.688385623360064,4.29369716312682E-6)) ;
#122531=DIRECTION('ref_axis',(0.688335104937436,0.725291600262751,-0.0121193192493712)) ;
#122532=DIRECTION('center_axis',(0.725299716569783,-0.688423829426493,-0.00359891949834901)) ;
#122533=DIRECTION('ref_axis',(0.688175169518926,0.724874796156686,0.0311683485991717)) ;
#122534=DIRECTION('center_axis',(-0.441849822549049,-0.89708903366019,0.)) ;
#122535=DIRECTION('ref_axis',(0.89708903366019,-0.441849822549049,0.)) ;
#122536=DIRECTION('center_axis',(1.,0.,0.)) ;
#122537=DIRECTION('ref_axis',(0.,0.,-1.)) ;
#122538=DIRECTION('center_axis',(1.,0.,0.)) ;
#122539=DIRECTION('ref_axis',(0.,0.,-1.)) ;
#122540=DIRECTION('center_axis',(0.,0.,1.)) ;
#122541=DIRECTION('ref_axis',(1.,0.,0.)) ;
#122542=DIRECTION('center_axis',(0.,0.,-1.)) ;
#122543=DIRECTION('ref_axis',(-1.,0.,0.)) ;
#122544=DIRECTION('center_axis',(2.47817639425258E-16,-1.,0.)) ;
#122545=DIRECTION('ref_axis',(1.,2.47817639425258E-16,0.)) ;
#122546=DIRECTION('center_axis',(0.,1.,0.)) ;
#122547=DIRECTION('ref_axis',(0.,0.,1.)) ;
#122548=DIRECTION('center_axis',(0.,-1.,0.)) ;
#122549=DIRECTION('ref_axis',(0.,0.,-1.)) ;
#122550=DIRECTION('center_axis',(0.,-1.,0.)) ;
#122551=DIRECTION('ref_axis',(0.,0.,-1.)) ;
#122552=DIRECTION('center_axis',(0.,-1.,0.)) ;
#122553=DIRECTION('ref_axis',(0.,0.,-1.)) ;
#122554=DIRECTION('center_axis',(0.,0.,1.)) ;
#122555=DIRECTION('ref_axis',(1.,0.,0.)) ;
#122556=DIRECTION('center_axis',(0.,0.,-1.)) ;
#122557=DIRECTION('ref_axis',(-1.,0.,0.)) ;
#122558=DIRECTION('center_axis',(0.,0.,-1.)) ;
#122559=DIRECTION('ref_axis',(-1.,0.,0.)) ;
#122560=DIRECTION('center_axis',(0.,0.,1.)) ;
#122561=DIRECTION('ref_axis',(-1.,0.,0.)) ;
#122562=DIRECTION('center_axis',(0.,1.,0.)) ;
#122563=DIRECTION('ref_axis',(1.,0.,0.)) ;
#122564=DIRECTION('center_axis',(1.,0.,0.)) ;
#122565=DIRECTION('ref_axis',(0.,0.,1.)) ;
#122566=DIRECTION('center_axis',(0.,0.,1.)) ;
#122567=DIRECTION('ref_axis',(1.,0.,0.)) ;
#122568=DIRECTION('center_axis',(1.,0.,0.)) ;
#122569=DIRECTION('ref_axis',(0.,0.,1.)) ;
#122570=DIRECTION('center_axis',(-0.527646808997082,0.849458398917494,-0.00304523623449406)) ;
#122571=DIRECTION('ref_axis',(0.786342490392807,0.487079579861469,-0.380024960607608)) ;
#122572=DIRECTION('center_axis',(0.,0.,-1.)) ;
#122573=DIRECTION('ref_axis',(-1.,0.,0.)) ;
#122574=DIRECTION('center_axis',(0.,0.,1.)) ;
#122575=DIRECTION('ref_axis',(-1.,0.,0.)) ;
#122576=DIRECTION('center_axis',(-1.,0.,0.)) ;
#122577=DIRECTION('ref_axis',(0.,0.,1.)) ;
#122578=DIRECTION('center_axis',(1.,0.,0.)) ;
#122579=DIRECTION('ref_axis',(0.,0.,-1.)) ;
#122580=DIRECTION('center_axis',(1.,0.,0.)) ;
#122581=DIRECTION('ref_axis',(0.,0.,-1.)) ;
#122582=DIRECTION('center_axis',(-0.297273799163877,0.954789382784888,-0.00235007487718195)) ;
#122583=DIRECTION('ref_axis',(0.954791853023049,0.297270453338573,-0.00167181718241995)) ;
#122584=DIRECTION('center_axis',(-0.297049675376424,0.954862026860596,-4.29369625967978E-6)) ;
#122585=DIRECTION('ref_axis',(0.954791884772883,0.297027909249879,0.012119319225527)) ;
#122586=DIRECTION('center_axis',(0.,0.,-1.)) ;
#122587=DIRECTION('ref_axis',(-1.,0.,0.)) ;
#122588=DIRECTION('center_axis',(0.441849822549049,0.89708903366019,-9.72625879207272E-16)) ;
#122589=DIRECTION('ref_axis',(0.89708903366019,-0.441849822549049,3.9032054237323E-31)) ;
#122590=DIRECTION('center_axis',(-0.441849822549049,-0.89708903366019,0.)) ;
#122591=DIRECTION('ref_axis',(0.89708903366019,-0.441849822549049,0.)) ;
#122592=DIRECTION('center_axis',(0.724093759486039,-0.689695657773317,0.00285081076274628)) ;
#122593=DIRECTION('ref_axis',(0.681728923122044,0.715090798805641,-0.154566570908355)) ;
#122594=DIRECTION('center_axis',(0.725345269034699,-0.688385241474045,-3.11468975456184E-6)) ;
#122595=DIRECTION('ref_axis',(0.688334826632565,0.725292092601058,0.0121056538482987)) ;
#122596=DIRECTION('center_axis',(0.725180989991168,-0.688554302427288,-0.0023461381674182)) ;
#122597=DIRECTION('ref_axis',(0.688552456842981,0.725184663578072,-0.00164860142364575)) ;
#122598=DIRECTION('center_axis',(0.,1.,0.)) ;
#122599=DIRECTION('ref_axis',(1.,0.,0.)) ;
#122600=DIRECTION('center_axis',(-2.05998412772247E-14,0.,-1.)) ;
#122601=DIRECTION('ref_axis',(1.,0.,-2.05998412772247E-14)) ;
#122602=DIRECTION('center_axis',(0.,0.514231796959122,0.857651245551589)) ;
#122603=DIRECTION('ref_axis',(0.,0.857651245551589,-0.514231796959122)) ;
#122604=DIRECTION('center_axis',(-1.,0.,0.)) ;
#122605=DIRECTION('ref_axis',(0.,0.,-1.)) ;
#122606=DIRECTION('center_axis',(1.,0.,0.)) ;
#122607=DIRECTION('ref_axis',(0.,0.,-1.)) ;
#122608=DIRECTION('center_axis',(-2.24981196193434E-14,-0.514231796959101,
0.857651245551602)) ;
#122609=DIRECTION('ref_axis',(1.43956865771859E-30,-0.857651245551602,-0.514231796959101)) ;
#122610=DIRECTION('center_axis',(-1.,0.,0.)) ;
#122611=DIRECTION('ref_axis',(0.,0.,1.)) ;
#122612=DIRECTION('center_axis',(-1.,0.,0.)) ;
#122613=DIRECTION('ref_axis',(0.,0.,-1.)) ;
#122614=DIRECTION('center_axis',(0.,0.,1.)) ;
#122615=DIRECTION('ref_axis',(1.,0.,0.)) ;
#122616=DIRECTION('center_axis',(0.,0.,-1.)) ;
#122617=DIRECTION('ref_axis',(-1.,0.,0.)) ;
#122618=DIRECTION('center_axis',(0.,-1.,8.97270763436279E-17)) ;
#122619=DIRECTION('ref_axis',(0.,-8.97270763436279E-17,-1.)) ;
#122620=DIRECTION('center_axis',(0.,-1.,8.97270763436279E-17)) ;
#122621=DIRECTION('ref_axis',(0.,-8.97270763436279E-17,-1.)) ;
#122622=DIRECTION('center_axis',(0.,-1.,0.)) ;
#122623=DIRECTION('ref_axis',(0.,0.,-1.)) ;
#122624=DIRECTION('center_axis',(0.,0.,-1.)) ;
#122625=DIRECTION('ref_axis',(-1.,0.,0.)) ;
#122626=DIRECTION('center_axis',(0.,0.,1.)) ;
#122627=DIRECTION('ref_axis',(-1.,0.,0.)) ;
#122628=DIRECTION('center_axis',(0.,0.,-1.)) ;
#122629=DIRECTION('ref_axis',(-1.,0.,0.)) ;
#122630=DIRECTION('center_axis',(0.,1.,0.)) ;
#122631=DIRECTION('ref_axis',(1.,0.,0.)) ;
#122632=DIRECTION('center_axis',(-1.,0.,0.)) ;
#122633=DIRECTION('ref_axis',(0.,0.,-1.)) ;
#122634=DIRECTION('center_axis',(0.,-1.84314369322536E-14,1.)) ;
#122635=DIRECTION('ref_axis',(0.,1.,1.84314369322536E-14)) ;
#122636=DIRECTION('center_axis',(1.,0.,0.)) ;
#122637=DIRECTION('ref_axis',(0.,0.,-1.)) ;
#122638=DIRECTION('center_axis',(0.,0.,1.)) ;
#122639=DIRECTION('ref_axis',(-1.,0.,0.)) ;
#122640=DIRECTION('center_axis',(0.,-0.514231796959101,-0.857651245551602)) ;
#122641=DIRECTION('ref_axis',(0.,-0.857651245551602,0.514231796959101)) ;
#122642=DIRECTION('center_axis',(0.,1.,0.)) ;
#122643=DIRECTION('ref_axis',(1.,0.,0.)) ;
#122644=DIRECTION('center_axis',(-1.,0.,0.)) ;
#122645=DIRECTION('ref_axis',(0.,0.,-1.)) ;
#122646=DIRECTION('center_axis',(0.,1.,8.97270763436279E-17)) ;
#122647=DIRECTION('ref_axis',(0.,-8.97270763436279E-17,1.)) ;
#122648=DIRECTION('center_axis',(0.,-1.,-8.97270763436279E-17)) ;
#122649=DIRECTION('ref_axis',(0.,-8.97270763436279E-17,1.)) ;
#122650=DIRECTION('center_axis',(0.,-1.,0.)) ;
#122651=DIRECTION('ref_axis',(0.,0.,-1.)) ;
#122652=DIRECTION('center_axis',(0.,0.,1.)) ;
#122653=DIRECTION('ref_axis',(1.,0.,0.)) ;
#122654=DIRECTION('center_axis',(-2.16840434497102E-15,0.,1.)) ;
#122655=DIRECTION('ref_axis',(1.,0.,2.16840434497102E-15)) ;
#122656=DIRECTION('center_axis',(-1.,0.,0.)) ;
#122657=DIRECTION('ref_axis',(0.,0.,1.)) ;
#122658=DIRECTION('center_axis',(-1.,0.,0.)) ;
#122659=DIRECTION('ref_axis',(0.,0.,-1.)) ;
#122660=DIRECTION('center_axis',(1.,0.,0.)) ;
#122661=DIRECTION('ref_axis',(0.,0.,-1.)) ;
#122662=DIRECTION('center_axis',(0.,0.514231796959101,-0.857651245551602)) ;
#122663=DIRECTION('ref_axis',(0.,0.857651245551602,0.514231796959101)) ;
#122664=DIRECTION('center_axis',(0.,0.,-1.)) ;
#122665=DIRECTION('ref_axis',(-1.,0.,0.)) ;
#122666=DIRECTION('center_axis',(-7.01133629567814E-33,8.97270763436279E-17,
1.)) ;
#122667=DIRECTION('ref_axis',(-6.29106707073161E-49,-1.,8.97270763436279E-17)) ;
#122668=DIRECTION('center_axis',(-1.,0.,-7.01133629567814E-33)) ;
#122669=DIRECTION('ref_axis',(-7.01133629567814E-33,0.,1.)) ;
#122670=DIRECTION('center_axis',(-1.,0.,0.)) ;
#122671=DIRECTION('ref_axis',(0.,0.,1.)) ;
#122672=DIRECTION('center_axis',(0.,1.,0.)) ;
#122673=DIRECTION('ref_axis',(1.,0.,0.)) ;
#122674=DIRECTION('center_axis',(-1.,0.,0.)) ;
#122675=DIRECTION('ref_axis',(0.,0.,-1.)) ;
#122676=DIRECTION('center_axis',(1.,0.,0.)) ;
#122677=DIRECTION('ref_axis',(0.,0.,-1.)) ;
#122678=DIRECTION('center_axis',(0.,0.,-1.)) ;
#122679=DIRECTION('ref_axis',(1.,0.,0.)) ;
#122680=DIRECTION('center_axis',(-7.01133629567814E-33,8.97270763436279E-17,
1.)) ;
#122681=DIRECTION('ref_axis',(0.,-1.,0.)) ;
#122682=DIRECTION('center_axis',(0.,-1.,0.)) ;
#122683=DIRECTION('ref_axis',(0.,0.,1.)) ;
#122684=DIRECTION('center_axis',(-1.,0.,7.01133629567814E-33)) ;
#122685=DIRECTION('ref_axis',(7.01133629567814E-33,0.,1.)) ;
#122686=DIRECTION('center_axis',(-1.,0.,0.)) ;
#122687=DIRECTION('ref_axis',(0.,0.,1.)) ;
#122688=DIRECTION('center_axis',(0.,0.,-1.)) ;
#122689=DIRECTION('ref_axis',(-1.,0.,0.)) ;
#122690=DIRECTION('center_axis',(-7.01133629567814E-33,8.97270763436279E-17,
-1.)) ;
#122691=DIRECTION('ref_axis',(6.29106707073161E-49,1.,8.97270763436279E-17)) ;
#122692=DIRECTION('center_axis',(0.,-1.,8.97270763436279E-17)) ;
#122693=DIRECTION('ref_axis',(0.,-8.97270763436279E-17,-1.)) ;
#122694=DIRECTION('center_axis',(0.,-1.,0.)) ;
#122695=DIRECTION('ref_axis',(0.,0.,-1.)) ;
#122696=DIRECTION('center_axis',(1.,7.81406971160724E-17,0.)) ;
#122697=DIRECTION('ref_axis',(-7.81406971160724E-17,1.,0.)) ;
#122698=DIRECTION('center_axis',(1.,0.,0.)) ;
#122699=DIRECTION('ref_axis',(0.,0.,-1.)) ;
#122700=DIRECTION('center_axis',(1.,0.,0.)) ;
#122701=DIRECTION('ref_axis',(0.,0.,-1.)) ;
#122702=DIRECTION('center_axis',(3.78638272950961E-32,-4.8455963016112E-16,
-1.)) ;
#122703=DIRECTION('ref_axis',(1.83472821505963E-47,1.,-4.8455963016112E-16)) ;
#122704=DIRECTION('center_axis',(0.,0.,-1.)) ;
#122705=DIRECTION('ref_axis',(-1.,0.,0.)) ;
#122706=DIRECTION('center_axis',(0.,0.,1.)) ;
#122707=DIRECTION('ref_axis',(1.,0.,0.)) ;
#122708=DIRECTION('center_axis',(-7.01133629567814E-33,8.97270763436279E-17,
-1.)) ;
#122709=DIRECTION('ref_axis',(0.,1.,0.)) ;
#122710=DIRECTION('center_axis',(0.,-1.,0.)) ;
#122711=DIRECTION('ref_axis',(0.,0.,1.)) ;
#122712=DIRECTION('center_axis',(0.,1.,0.)) ;
#122713=DIRECTION('ref_axis',(1.,0.,0.)) ;
#122714=DIRECTION('center_axis',(-1.,0.,0.)) ;
#122715=DIRECTION('ref_axis',(0.,0.,-1.)) ;
#122716=DIRECTION('center_axis',(0.,0.,1.)) ;
#122717=DIRECTION('ref_axis',(-1.,0.,0.)) ;
#122718=DIRECTION('center_axis',(0.,1.,0.)) ;
#122719=DIRECTION('ref_axis',(1.,0.,0.)) ;
#122720=DIRECTION('center_axis',(0.,1.,0.)) ;
#122721=DIRECTION('ref_axis',(0.,0.,-1.)) ;
#122722=DIRECTION('center_axis',(0.,1.,8.97270763436279E-17)) ;
#122723=DIRECTION('ref_axis',(0.,-8.97270763436279E-17,1.)) ;
#122724=DIRECTION('center_axis',(0.,-1.,0.)) ;
#122725=DIRECTION('ref_axis',(0.,0.,-1.)) ;
#122726=DIRECTION('center_axis',(0.,0.,1.)) ;
#122727=DIRECTION('ref_axis',(1.,0.,0.)) ;
#122728=DIRECTION('center_axis',(0.,0.,1.)) ;
#122729=DIRECTION('ref_axis',(1.,0.,0.)) ;
#122730=DIRECTION('center_axis',(-1.,-7.81406971160724E-17,0.)) ;
#122731=DIRECTION('ref_axis',(7.81406971160724E-17,-1.,0.)) ;
#122732=DIRECTION('center_axis',(-1.,-7.81406971160724E-17,0.)) ;
#122733=DIRECTION('ref_axis',(-7.81406971160724E-17,1.,0.)) ;
#122734=DIRECTION('center_axis',(-7.81406971160724E-17,1.,-8.97270763436279E-17)) ;
#122735=DIRECTION('ref_axis',(-7.01133629567814E-33,8.97270763436279E-17,
1.)) ;
#122736=DIRECTION('center_axis',(0.,1.,0.)) ;
#122737=DIRECTION('ref_axis',(0.,0.,1.)) ;
#122738=DIRECTION('center_axis',(0.,1.,0.)) ;
#122739=DIRECTION('ref_axis',(1.,0.,0.)) ;
#122740=DIRECTION('center_axis',(-1.,0.,0.)) ;
#122741=DIRECTION('ref_axis',(0.,0.,-1.)) ;
#122742=DIRECTION('center_axis',(1.,7.81406971160724E-17,0.)) ;
#122743=DIRECTION('ref_axis',(0.,1.,0.)) ;
#122744=DIRECTION('center_axis',(0.,0.,-1.)) ;
#122745=DIRECTION('ref_axis',(1.,0.,0.)) ;
#122746=DIRECTION('center_axis',(-3.78638272950961E-32,4.8455963016112E-16,
-1.)) ;
#122747=DIRECTION('ref_axis',(1.83472821505963E-47,1.,4.8455963016112E-16)) ;
#122748=DIRECTION('center_axis',(0.,0.,1.)) ;
#122749=DIRECTION('ref_axis',(-1.,1.30104260698261E-14,0.)) ;
#122750=DIRECTION('center_axis',(0.,0.,1.)) ;
#122751=DIRECTION('ref_axis',(1.,0.,0.)) ;
#122752=DIRECTION('center_axis',(1.,7.81406971160724E-17,0.)) ;
#122753=DIRECTION('ref_axis',(-7.81406971160724E-17,1.,0.)) ;
#122754=DIRECTION('center_axis',(1.,0.,0.)) ;
#122755=DIRECTION('ref_axis',(0.,0.,-1.)) ;
#122756=DIRECTION('center_axis',(1.,0.,0.)) ;
#122757=DIRECTION('ref_axis',(0.,0.,-1.)) ;
#122758=DIRECTION('center_axis',(-1.,-7.81406971160724E-17,0.)) ;
#122759=DIRECTION('ref_axis',(7.81406971160724E-17,-1.,0.)) ;
#122760=DIRECTION('center_axis',(-1.,-7.81406971160724E-17,0.)) ;
#122761=DIRECTION('ref_axis',(-7.81406971160724E-17,1.,0.)) ;
#122762=DIRECTION('center_axis',(0.,0.,-1.)) ;
#122763=DIRECTION('ref_axis',(-1.,0.,0.)) ;
#122764=DIRECTION('center_axis',(0.,0.,-1.)) ;
#122765=DIRECTION('ref_axis',(-1.,0.,0.)) ;
#122766=DIRECTION('center_axis',(0.,1.,0.)) ;
#122767=DIRECTION('ref_axis',(1.,0.,0.)) ;
#122768=DIRECTION('center_axis',(0.,1.,0.)) ;
#122769=DIRECTION('ref_axis',(0.,0.,-1.)) ;
#122770=DIRECTION('center_axis',(1.,7.81406971160724E-17,0.)) ;
#122771=DIRECTION('ref_axis',(0.,1.,0.)) ;
#122772=DIRECTION('center_axis',(0.,-1.,0.)) ;
#122773=DIRECTION('ref_axis',(0.,0.,1.)) ;
#122774=DIRECTION('center_axis',(7.81406971160724E-17,-1.,-8.97270763436279E-17)) ;
#122775=DIRECTION('ref_axis',(-7.01133629567814E-33,8.97270763436279E-17,
-1.)) ;
#122776=DIRECTION('center_axis',(0.,-1.,0.)) ;
#122777=DIRECTION('ref_axis',(0.,0.,-1.)) ;
#122778=DIRECTION('center_axis',(-1.,0.,-8.67361737988403E-15)) ;
#122779=DIRECTION('ref_axis',(-8.67361737988403E-15,0.,1.)) ;
#122780=DIRECTION('center_axis',(-5.96311194867026E-15,5.96311194867028E-15,
-1.)) ;
#122781=DIRECTION('ref_axis',(0.,1.,5.96311194867028E-15)) ;
#122782=DIRECTION('center_axis',(0.,0.,-1.)) ;
#122783=DIRECTION('ref_axis',(-1.,0.,0.)) ;
#122784=DIRECTION('center_axis',(0.,6.50521303491304E-15,-1.)) ;
#122785=DIRECTION('ref_axis',(0.,1.,6.50521303491304E-15)) ;
#122786=DIRECTION('center_axis',(1.,0.,0.)) ;
#122787=DIRECTION('ref_axis',(0.,0.,-1.)) ;
#122788=DIRECTION('center_axis',(-1.,0.,0.)) ;
#122789=DIRECTION('ref_axis',(0.,0.,1.)) ;
#122790=DIRECTION('center_axis',(0.,-1.,0.)) ;
#122791=DIRECTION('ref_axis',(0.,0.,-1.)) ;
#122792=DIRECTION('center_axis',(-1.,0.,0.)) ;
#122793=DIRECTION('ref_axis',(0.,0.,1.)) ;
#122794=DIRECTION('center_axis',(0.,-1.,0.)) ;
#122795=DIRECTION('ref_axis',(0.,0.,-1.)) ;
#122796=DIRECTION('center_axis',(6.50521303491295E-15,0.,-1.)) ;
#122797=DIRECTION('ref_axis',(-1.,0.,-6.50521303491295E-15)) ;
#122798=DIRECTION('center_axis',(-1.,0.,0.)) ;
#122799=DIRECTION('ref_axis',(0.,0.,1.)) ;
#122800=DIRECTION('center_axis',(-1.,1.73472347597681E-14,0.)) ;
#122801=DIRECTION('ref_axis',(-1.73472347597681E-14,-1.,0.)) ;
#122802=DIRECTION('center_axis',(0.,0.,1.)) ;
#122803=DIRECTION('ref_axis',(1.,0.,0.)) ;
#122804=DIRECTION('center_axis',(-7.04731412115582E-15,0.,-1.)) ;
#122805=DIRECTION('ref_axis',(-1.,0.,7.04731412115582E-15)) ;
#122806=DIRECTION('center_axis',(0.,-1.,0.)) ;
#122807=DIRECTION('ref_axis',(0.,0.,-1.)) ;
#122808=DIRECTION('center_axis',(1.,0.,-2.16840434497101E-16)) ;
#122809=DIRECTION('ref_axis',(-2.16840434497101E-16,0.,-1.)) ;
#122810=DIRECTION('center_axis',(1.,0.,0.)) ;
#122811=DIRECTION('ref_axis',(0.,0.,-1.)) ;
#122812=DIRECTION('center_axis',(-1.,0.,0.)) ;
#122813=DIRECTION('ref_axis',(0.,0.,1.)) ;
#122814=DIRECTION('center_axis',(0.,-1.,0.)) ;
#122815=DIRECTION('ref_axis',(0.,0.,-1.)) ;
#122816=DIRECTION('center_axis',(0.,0.,-1.)) ;
#122817=DIRECTION('ref_axis',(1.,0.,0.)) ;
#122818=DIRECTION('center_axis',(0.,-1.,0.)) ;
#122819=DIRECTION('ref_axis',(0.,0.,-1.)) ;
#122820=DIRECTION('center_axis',(0.,-1.,0.)) ;
#122821=DIRECTION('ref_axis',(0.,0.,-1.)) ;
#122822=DIRECTION('center_axis',(0.,-1.,0.)) ;
#122823=DIRECTION('ref_axis',(0.,0.,-1.)) ;
#122824=DIRECTION('center_axis',(0.,0.,-1.)) ;
#122825=DIRECTION('ref_axis',(1.,0.,0.)) ;
#122826=DIRECTION('center_axis',(0.,0.,1.)) ;
#122827=DIRECTION('ref_axis',(1.,0.,0.)) ;
#122828=DIRECTION('center_axis',(0.,0.,-1.)) ;
#122829=DIRECTION('ref_axis',(-1.,0.,0.)) ;
#122830=DIRECTION('center_axis',(0.,1.,0.)) ;
#122831=DIRECTION('ref_axis',(0.,0.,1.)) ;
#122832=DIRECTION('center_axis',(0.,-1.,0.)) ;
#122833=DIRECTION('ref_axis',(0.,0.,-1.)) ;
#122834=DIRECTION('center_axis',(-1.,0.,2.16840434497101E-16)) ;
#122835=DIRECTION('ref_axis',(2.16840434497101E-16,0.,1.)) ;
#122836=DIRECTION('center_axis',(-1.,0.,0.)) ;
#122837=DIRECTION('ref_axis',(0.,0.,1.)) ;
#122838=DIRECTION('center_axis',(1.,0.,0.)) ;
#122839=DIRECTION('ref_axis',(0.,0.,-1.)) ;
#122840=DIRECTION('center_axis',(0.,1.,0.)) ;
#122841=DIRECTION('ref_axis',(0.,0.,1.)) ;
#122842=DIRECTION('center_axis',(0.,-1.,0.)) ;
#122843=DIRECTION('ref_axis',(0.,0.,-1.)) ;
#122844=DIRECTION('center_axis',(2.16840434497101E-16,0.,-1.)) ;
#122845=DIRECTION('ref_axis',(-1.,0.,-2.16840434497101E-16)) ;
#122846=DIRECTION('center_axis',(0.,0.,-1.)) ;
#122847=DIRECTION('ref_axis',(-1.,0.,0.)) ;
#122848=DIRECTION('center_axis',(-1.,0.,-2.16840434497101E-16)) ;
#122849=DIRECTION('ref_axis',(-2.16840434497101E-16,0.,1.)) ;
#122850=DIRECTION('center_axis',(-1.,0.,0.)) ;
#122851=DIRECTION('ref_axis',(0.,0.,1.)) ;
#122852=DIRECTION('center_axis',(1.,0.,0.)) ;
#122853=DIRECTION('ref_axis',(0.,0.,-1.)) ;
#122854=DIRECTION('center_axis',(0.,-1.,0.)) ;
#122855=DIRECTION('ref_axis',(0.,0.,-1.)) ;
#122856=DIRECTION('center_axis',(0.,-1.,0.)) ;
#122857=DIRECTION('ref_axis',(0.,0.,-1.)) ;
#122858=DIRECTION('center_axis',(0.,1.,0.)) ;
#122859=DIRECTION('ref_axis',(1.,0.,0.)) ;
#122860=DIRECTION('center_axis',(0.,0.,1.)) ;
#122861=DIRECTION('ref_axis',(-1.,0.,0.)) ;
#122862=DIRECTION('center_axis',(0.,1.,0.)) ;
#122863=DIRECTION('ref_axis',(1.,0.,0.)) ;
#122864=DIRECTION('center_axis',(0.,0.,1.)) ;
#122865=DIRECTION('ref_axis',(-1.,0.,0.)) ;
#122866=DIRECTION('center_axis',(0.,-1.,0.)) ;
#122867=DIRECTION('ref_axis',(0.,0.,-1.)) ;
#122868=DIRECTION('center_axis',(0.,-1.,0.)) ;
#122869=DIRECTION('ref_axis',(0.,0.,-1.)) ;
#122870=DIRECTION('center_axis',(0.,1.,0.)) ;
#122871=DIRECTION('ref_axis',(0.,0.,1.)) ;
#122872=DIRECTION('center_axis',(0.,-1.,0.)) ;
#122873=DIRECTION('ref_axis',(0.,0.,-1.)) ;
#122874=DIRECTION('center_axis',(0.,0.,-1.)) ;
#122875=DIRECTION('ref_axis',(-1.,0.,0.)) ;
#122876=DIRECTION('center_axis',(0.,0.,1.)) ;
#122877=DIRECTION('ref_axis',(1.,0.,0.)) ;
#122878=DIRECTION('center_axis',(-2.16840434497101E-16,0.,1.)) ;
#122879=DIRECTION('ref_axis',(1.,0.,2.16840434497101E-16)) ;
#122880=DIRECTION('center_axis',(0.,0.,1.)) ;
#122881=DIRECTION('ref_axis',(1.,0.,0.)) ;
#122882=DIRECTION('center_axis',(0.,1.,0.)) ;
#122883=DIRECTION('ref_axis',(0.,0.,1.)) ;
#122884=DIRECTION('center_axis',(0.,-1.,0.)) ;
#122885=DIRECTION('ref_axis',(0.,0.,-1.)) ;
#122886=DIRECTION('center_axis',(0.,1.,0.)) ;
#122887=DIRECTION('ref_axis',(1.,0.,0.)) ;
#122888=DIRECTION('center_axis',(-1.,0.,0.)) ;
#122889=DIRECTION('ref_axis',(0.,0.,-1.)) ;
#122890=DIRECTION('center_axis',(0.,1.,0.)) ;
#122891=DIRECTION('ref_axis',(1.,0.,0.)) ;
#122892=DIRECTION('center_axis',(1.,0.,0.)) ;
#122893=DIRECTION('ref_axis',(0.,0.,1.)) ;
#122894=DIRECTION('center_axis',(1.,0.,2.16840434497101E-16)) ;
#122895=DIRECTION('ref_axis',(2.16840434497101E-16,0.,-1.)) ;
#122896=DIRECTION('center_axis',(0.,-1.,0.)) ;
#122897=DIRECTION('ref_axis',(0.,0.,-1.)) ;
#122898=DIRECTION('center_axis',(0.,-1.,0.)) ;
#122899=DIRECTION('ref_axis',(0.,0.,-1.)) ;
#122900=DIRECTION('center_axis',(0.,0.,1.)) ;
#122901=DIRECTION('ref_axis',(1.,0.,0.)) ;
#122902=DIRECTION('center_axis',(0.,0.,-1.)) ;
#122903=DIRECTION('ref_axis',(-1.,0.,0.)) ;
#122904=DIRECTION('center_axis',(0.,0.,1.)) ;
#122905=DIRECTION('ref_axis',(1.,0.,0.)) ;
#122906=DIRECTION('center_axis',(0.,-1.,0.)) ;
#122907=DIRECTION('ref_axis',(0.,0.,-1.)) ;
#122908=DIRECTION('center_axis',(0.,-1.,0.)) ;
#122909=DIRECTION('ref_axis',(0.,0.,-1.)) ;
#122910=DIRECTION('center_axis',(0.,1.,0.)) ;
#122911=DIRECTION('ref_axis',(1.,0.,0.)) ;
#122912=DIRECTION('center_axis',(-1.,0.,0.)) ;
#122913=DIRECTION('ref_axis',(0.,0.,-1.)) ;
#122914=DIRECTION('center_axis',(0.,1.,0.)) ;
#122915=DIRECTION('ref_axis',(1.,0.,0.)) ;
#122916=DIRECTION('center_axis',(-1.,0.,0.)) ;
#122917=DIRECTION('ref_axis',(0.,0.,-1.)) ;
#122918=DIRECTION('center_axis',(0.,-1.,0.)) ;
#122919=DIRECTION('ref_axis',(0.,0.,-1.)) ;
#122920=DIRECTION('center_axis',(0.,-1.,0.)) ;
#122921=DIRECTION('ref_axis',(0.,0.,-1.)) ;
#122922=DIRECTION('center_axis',(-1.,0.,0.)) ;
#122923=DIRECTION('ref_axis',(0.,0.,1.)) ;
#122924=DIRECTION('center_axis',(-1.,0.,0.)) ;
#122925=DIRECTION('ref_axis',(0.,0.,1.)) ;
#122926=DIRECTION('center_axis',(1.,0.,0.)) ;
#122927=DIRECTION('ref_axis',(0.,0.,-1.)) ;
#122928=DIRECTION('center_axis',(-1.,0.,0.)) ;
#122929=DIRECTION('ref_axis',(0.,0.,1.)) ;
#122930=DIRECTION('center_axis',(0.,-1.,0.)) ;
#122931=DIRECTION('ref_axis',(0.,0.,-1.)) ;
#122932=DIRECTION('center_axis',(0.,-1.,0.)) ;
#122933=DIRECTION('ref_axis',(0.,0.,-1.)) ;
#122934=DIRECTION('center_axis',(0.,1.,0.)) ;
#122935=DIRECTION('ref_axis',(1.,0.,0.)) ;
#122936=DIRECTION('center_axis',(0.,0.,-1.)) ;
#122937=DIRECTION('ref_axis',(1.,0.,0.)) ;
#122938=DIRECTION('center_axis',(0.,1.,0.)) ;
#122939=DIRECTION('ref_axis',(1.,0.,0.)) ;
#122940=DIRECTION('center_axis',(0.,0.,1.)) ;
#122941=DIRECTION('ref_axis',(-1.,0.,0.)) ;
#122942=DIRECTION('center_axis',(0.,0.,-1.)) ;
#122943=DIRECTION('ref_axis',(-1.,0.,0.)) ;
#122944=DIRECTION('center_axis',(-0.669589480006975,0.669589480006975,-0.321402950403348)) ;
#122945=DIRECTION('ref_axis',(-0.707106781186547,-0.707106781186548,-3.60611190025948E-16)) ;
#122946=DIRECTION('center_axis',(0.669589480006972,-0.66958948000698,0.321402950403345)) ;
#122947=DIRECTION('ref_axis',(0.707106781186552,0.707106781186543,5.47414022772576E-16)) ;
#122948=DIRECTION('center_axis',(0.,1.,0.)) ;
#122949=DIRECTION('ref_axis',(1.,0.,0.)) ;
#122950=DIRECTION('center_axis',(-5.0109744998751E-15,1.,0.)) ;
#122951=DIRECTION('ref_axis',(1.,5.0109744998751E-15,-4.33680868994201E-15)) ;
#122952=DIRECTION('center_axis',(0.707106781186548,-0.707106781186548,-4.59988025005012E-15)) ;
#122953=DIRECTION('ref_axis',(-0.707106781186548,-0.707106781186548,-1.2354148483551E-31)) ;
#122954=DIRECTION('center_axis',(-0.707106781186548,0.707106781186547,0.)) ;
#122955=DIRECTION('ref_axis',(-0.707106781186547,-0.707106781186548,0.)) ;
#122956=DIRECTION('center_axis',(0.,-1.,0.)) ;
#122957=DIRECTION('ref_axis',(0.,0.,-1.)) ;
#122958=DIRECTION('center_axis',(0.,1.,0.)) ;
#122959=DIRECTION('ref_axis',(0.,0.,1.)) ;
#122960=DIRECTION('center_axis',(-0.879462917689188,-0.219865729422294,
-0.42214220049081)) ;
#122961=DIRECTION('ref_axis',(-0.432731067584771,-3.91091346796197E-16,
0.901523057468274)) ;
#122962=DIRECTION('center_axis',(0.879462917689189,0.219865729422295,0.422142200490807)) ;
#122963=DIRECTION('ref_axis',(0.432731067584768,-3.18283478174207E-16,-0.901523057468275)) ;
#122964=DIRECTION('center_axis',(0.,-1.,0.)) ;
#122965=DIRECTION('ref_axis',(0.,0.,1.)) ;
#122966=DIRECTION('center_axis',(0.,0.,1.)) ;
#122967=DIRECTION('ref_axis',(-1.,0.,0.)) ;
#122968=DIRECTION('center_axis',(0.,1.,0.)) ;
#122969=DIRECTION('ref_axis',(1.,0.,0.)) ;
#122970=DIRECTION('center_axis',(0.970142500145333,0.242535625036331,0.)) ;
#122971=DIRECTION('ref_axis',(0.242535625036331,-0.970142500145332,0.)) ;
#122972=DIRECTION('center_axis',(0.669589480006975,-0.669589480006975,-0.321402950403348)) ;
#122973=DIRECTION('ref_axis',(0.707106781186547,0.707106781186548,-3.60611190025948E-16)) ;
#122974=DIRECTION('center_axis',(0.669589480006975,-0.669589480006975,-0.321402950403349)) ;
#122975=DIRECTION('ref_axis',(0.707106781186548,0.707106781186547,2.25891969505504E-16)) ;
#122976=DIRECTION('center_axis',(0.707106781186548,-0.707106781186547,0.)) ;
#122977=DIRECTION('ref_axis',(0.707106781186547,0.707106781186548,0.)) ;
#122978=DIRECTION('center_axis',(-0.707106781186542,0.707106781186553,0.)) ;
#122979=DIRECTION('ref_axis',(-0.707106781186553,-0.707106781186542,0.)) ;
#122980=DIRECTION('center_axis',(0.,0.,1.)) ;
#122981=DIRECTION('ref_axis',(1.,0.,0.)) ;
#122982=DIRECTION('center_axis',(0.,0.,1.)) ;
#122983=DIRECTION('ref_axis',(1.,0.,0.)) ;
#122984=DIRECTION('center_axis',(2.47817639425258E-16,-1.,0.)) ;
#122985=DIRECTION('ref_axis',(1.,2.47817639425258E-16,0.)) ;
#122986=DIRECTION('center_axis',(0.,-1.,0.)) ;
#122987=DIRECTION('ref_axis',(0.,0.,-1.)) ;
#122988=DIRECTION('center_axis',(-0.970142500145333,-0.24253562503633,0.)) ;
#122989=DIRECTION('ref_axis',(0.24253562503633,-0.970142500145333,0.)) ;
#122990=DIRECTION('center_axis',(0.976187060183959,-0.216930457818629,3.32210494350328E-14)) ;
#122991=DIRECTION('ref_axis',(0.216930457818629,0.976187060183959,-2.9855370908175E-12)) ;
#122992=DIRECTION('center_axis',(0.,1.,0.)) ;
#122993=DIRECTION('ref_axis',(1.,0.,0.)) ;
#122994=DIRECTION('center_axis',(2.71050543121376E-14,1.,-1.3010426069826E-14)) ;
#122995=DIRECTION('ref_axis',(1.,-2.71050543121376E-14,2.16840434497099E-15)) ;
#122996=DIRECTION('center_axis',(0.,-1.,0.)) ;
#122997=DIRECTION('ref_axis',(0.,0.,1.)) ;
#122998=DIRECTION('center_axis',(0.,0.,1.)) ;
#122999=DIRECTION('ref_axis',(-1.,8.67361737988401E-15,0.)) ;
#123000=DIRECTION('center_axis',(0.879462917689188,0.219865729422294,-0.42214220049081)) ;
#123001=DIRECTION('ref_axis',(-0.432731067584771,-3.91091346796197E-16,
-0.901523057468274)) ;
#123002=DIRECTION('center_axis',(0.879462917689188,0.219865729422296,-0.422142200490809)) ;
#123003=DIRECTION('ref_axis',(-0.43273106758477,-9.90395117542237E-17,-0.901523057468274)) ;
#123004=DIRECTION('center_axis',(0.,-1.,0.)) ;
#123005=DIRECTION('ref_axis',(0.,0.,-1.)) ;
#123006=DIRECTION('center_axis',(2.00438979995004E-14,1.,0.)) ;
#123007=DIRECTION('ref_axis',(-1.,2.00438979995004E-14,0.)) ;
#123008=DIRECTION('center_axis',(2.47817639425258E-16,-1.,0.)) ;
#123009=DIRECTION('ref_axis',(1.,2.47817639425258E-16,0.)) ;
#123010=DIRECTION('center_axis',(0.,-1.,0.)) ;
#123011=DIRECTION('ref_axis',(0.,0.,-1.)) ;
#123012=DIRECTION('center_axis',(0.,0.,1.)) ;
#123013=DIRECTION('ref_axis',(1.,0.,0.)) ;
#123014=DIRECTION('center_axis',(0.,0.,1.)) ;
#123015=DIRECTION('ref_axis',(1.,0.,0.)) ;
#123016=DIRECTION('center_axis',(0.,1.,0.)) ;
#123017=DIRECTION('ref_axis',(1.,0.,0.)) ;
#123018=DIRECTION('center_axis',(0.970142500145333,0.242535625036331,0.)) ;
#123019=DIRECTION('ref_axis',(0.242535625036331,-0.970142500145332,0.)) ;
#123020=DIRECTION('center_axis',(-0.97618706018396,0.216930457818626,3.48715666902613E-14)) ;
#123021=DIRECTION('ref_axis',(0.216930457818626,0.97618706018396,1.89720090087137E-12)) ;
#123022=DIRECTION('center_axis',(0.970142500145333,0.24253562503633,0.)) ;
#123023=DIRECTION('ref_axis',(-0.24253562503633,0.970142500145333,0.)) ;
#123024=DIRECTION('center_axis',(1.,1.31418445149758E-16,-2.16840434497101E-16)) ;
#123025=DIRECTION('ref_axis',(-2.16840434497101E-16,-2.8496832747207E-32,
-1.)) ;
#123026=DIRECTION('center_axis',(1.,0.,0.)) ;
#123027=DIRECTION('ref_axis',(0.,0.,-1.)) ;
#123028=DIRECTION('center_axis',(-1.,0.,0.)) ;
#123029=DIRECTION('ref_axis',(0.,0.,1.)) ;
#123030=DIRECTION('center_axis',(-1.31418445149758E-16,1.,0.)) ;
#123031=DIRECTION('ref_axis',(-1.,0.,0.)) ;
#123032=DIRECTION('center_axis',(0.,0.,1.)) ;
#123033=DIRECTION('ref_axis',(-1.,0.,0.)) ;
#123034=DIRECTION('center_axis',(-1.31418445149758E-16,1.,0.)) ;
#123035=DIRECTION('ref_axis',(-1.,-1.31418445149758E-16,0.)) ;
#123036=DIRECTION('center_axis',(-1.31418445149758E-16,1.,0.)) ;
#123037=DIRECTION('ref_axis',(-1.,0.,0.)) ;
#123038=DIRECTION('center_axis',(-1.31418445149758E-16,1.,0.)) ;
#123039=DIRECTION('ref_axis',(-1.,-1.31418445149758E-16,0.)) ;
#123040=DIRECTION('center_axis',(0.,0.,1.)) ;
#123041=DIRECTION('ref_axis',(-1.,0.,0.)) ;
#123042=DIRECTION('center_axis',(-4.33680868994202E-16,-5.69936654944139E-32,
-1.)) ;
#123043=DIRECTION('ref_axis',(-1.,2.47170623787823E-47,4.33680868994202E-16)) ;
#123044=DIRECTION('center_axis',(0.,0.,1.)) ;
#123045=DIRECTION('ref_axis',(1.,0.,0.)) ;
#123046=DIRECTION('center_axis',(-1.31418445149758E-16,-1.,0.)) ;
#123047=DIRECTION('ref_axis',(1.,-1.31418445149758E-16,0.)) ;
#123048=DIRECTION('center_axis',(0.,1.,0.)) ;
#123049=DIRECTION('ref_axis',(0.,0.,1.)) ;
#123050=DIRECTION('center_axis',(-1.,0.,2.16840434497101E-16)) ;
#123051=DIRECTION('ref_axis',(2.16840434497101E-16,0.,1.)) ;
#123052=DIRECTION('center_axis',(-1.,0.,0.)) ;
#123053=DIRECTION('ref_axis',(0.,0.,1.)) ;
#123054=DIRECTION('center_axis',(1.,0.,0.)) ;
#123055=DIRECTION('ref_axis',(0.,0.,-1.)) ;
#123056=DIRECTION('center_axis',(-1.31418445149758E-16,-1.,0.)) ;
#123057=DIRECTION('ref_axis',(1.,-1.31418445149758E-16,0.)) ;
#123058=DIRECTION('center_axis',(0.,1.,0.)) ;
#123059=DIRECTION('ref_axis',(0.,0.,1.)) ;
#123060=DIRECTION('center_axis',(2.16840434497101E-16,2.8496832747207E-32,
1.)) ;
#123061=DIRECTION('ref_axis',(1.,-6.17926559469557E-48,-2.16840434497101E-16)) ;
#123062=DIRECTION('center_axis',(0.,0.,1.)) ;
#123063=DIRECTION('ref_axis',(1.,0.,0.)) ;
#123064=DIRECTION('center_axis',(-1.,-1.31418445149758E-16,-2.16840434497101E-16)) ;
#123065=DIRECTION('ref_axis',(-2.16840434497101E-16,-2.8496832747207E-32,
1.)) ;
#123066=DIRECTION('center_axis',(-1.,0.,0.)) ;
#123067=DIRECTION('ref_axis',(0.,0.,1.)) ;
#123068=DIRECTION('center_axis',(1.,0.,0.)) ;
#123069=DIRECTION('ref_axis',(0.,0.,-1.)) ;
#123070=DIRECTION('center_axis',(-1.31418445149758E-16,1.,0.)) ;
#123071=DIRECTION('ref_axis',(-1.,0.,0.)) ;
#123072=DIRECTION('center_axis',(-1.31418445149758E-16,1.,0.)) ;
#123073=DIRECTION('ref_axis',(-1.,-1.31418445149758E-16,0.)) ;
#123074=DIRECTION('center_axis',(0.,1.,0.)) ;
#123075=DIRECTION('ref_axis',(1.,0.,0.)) ;
#123076=DIRECTION('center_axis',(0.,0.,-1.)) ;
#123077=DIRECTION('ref_axis',(1.,0.,0.)) ;
#123078=DIRECTION('center_axis',(0.,1.,0.)) ;
#123079=DIRECTION('ref_axis',(1.,0.,0.)) ;
#123080=DIRECTION('center_axis',(0.,0.,-1.)) ;
#123081=DIRECTION('ref_axis',(1.,0.,0.)) ;
#123082=DIRECTION('center_axis',(-1.31418445149758E-16,1.,0.)) ;
#123083=DIRECTION('ref_axis',(-1.,0.,0.)) ;
#123084=DIRECTION('center_axis',(-1.31418445149758E-16,1.,0.)) ;
#123085=DIRECTION('ref_axis',(-1.,-1.31418445149758E-16,0.)) ;
#123086=DIRECTION('center_axis',(-1.31418445149758E-16,-1.,0.)) ;
#123087=DIRECTION('ref_axis',(1.,-1.31418445149758E-16,0.)) ;
#123088=DIRECTION('center_axis',(0.,1.,0.)) ;
#123089=DIRECTION('ref_axis',(0.,0.,1.)) ;
#123090=DIRECTION('center_axis',(4.33680868994202E-16,0.,1.)) ;
#123091=DIRECTION('ref_axis',(1.,0.,-4.33680868994202E-16)) ;
#123092=DIRECTION('center_axis',(0.,0.,-1.)) ;
#123093=DIRECTION('ref_axis',(-1.,0.,0.)) ;
#123094=DIRECTION('center_axis',(-2.16840434497101E-16,0.,-1.)) ;
#123095=DIRECTION('ref_axis',(-1.,0.,2.16840434497101E-16)) ;
#123096=DIRECTION('center_axis',(0.,0.,-1.)) ;
#123097=DIRECTION('ref_axis',(-1.,0.,0.)) ;
#123098=DIRECTION('center_axis',(-1.31418445149758E-16,-1.,0.)) ;
#123099=DIRECTION('ref_axis',(1.,-1.31418445149758E-16,0.)) ;
#123100=DIRECTION('center_axis',(0.,1.,0.)) ;
#123101=DIRECTION('ref_axis',(0.,0.,1.)) ;
#123102=DIRECTION('center_axis',(0.,1.,0.)) ;
#123103=DIRECTION('ref_axis',(1.,0.,0.)) ;
#123104=DIRECTION('center_axis',(-1.,0.,0.)) ;
#123105=DIRECTION('ref_axis',(0.,0.,-1.)) ;
#123106=DIRECTION('center_axis',(0.,1.,0.)) ;
#123107=DIRECTION('ref_axis',(1.,0.,0.)) ;
#123108=DIRECTION('center_axis',(1.,0.,0.)) ;
#123109=DIRECTION('ref_axis',(0.,0.,1.)) ;
#123110=DIRECTION('center_axis',(1.,0.,2.16840434497101E-16)) ;
#123111=DIRECTION('ref_axis',(2.16840434497101E-16,0.,-1.)) ;
#123112=DIRECTION('center_axis',(0.,1.,0.)) ;
#123113=DIRECTION('ref_axis',(0.,0.,1.)) ;
#123114=DIRECTION('center_axis',(0.,1.,0.)) ;
#123115=DIRECTION('ref_axis',(0.,0.,1.)) ;
#123116=DIRECTION('center_axis',(0.,0.,-1.)) ;
#123117=DIRECTION('ref_axis',(-1.,0.,0.)) ;
#123118=DIRECTION('center_axis',(0.,0.,1.)) ;
#123119=DIRECTION('ref_axis',(1.,0.,0.)) ;
#123120=DIRECTION('center_axis',(0.,0.,-1.)) ;
#123121=DIRECTION('ref_axis',(-1.,0.,0.)) ;
#123122=DIRECTION('center_axis',(0.,1.,0.)) ;
#123123=DIRECTION('ref_axis',(0.,0.,1.)) ;
#123124=DIRECTION('center_axis',(0.,1.,0.)) ;
#123125=DIRECTION('ref_axis',(0.,0.,1.)) ;
#123126=DIRECTION('center_axis',(0.,1.,0.)) ;
#123127=DIRECTION('ref_axis',(1.,0.,0.)) ;
#123128=DIRECTION('center_axis',(-1.,0.,0.)) ;
#123129=DIRECTION('ref_axis',(0.,0.,-1.)) ;
#123130=DIRECTION('center_axis',(0.,1.,0.)) ;
#123131=DIRECTION('ref_axis',(1.,0.,0.)) ;
#123132=DIRECTION('center_axis',(-1.,0.,0.)) ;
#123133=DIRECTION('ref_axis',(0.,0.,-1.)) ;
#123134=DIRECTION('center_axis',(0.,1.,0.)) ;
#123135=DIRECTION('ref_axis',(0.,0.,1.)) ;
#123136=DIRECTION('center_axis',(0.,1.,0.)) ;
#123137=DIRECTION('ref_axis',(0.,0.,1.)) ;
#123138=DIRECTION('center_axis',(-1.,0.,0.)) ;
#123139=DIRECTION('ref_axis',(0.,0.,1.)) ;
#123140=DIRECTION('center_axis',(-1.,0.,0.)) ;
#123141=DIRECTION('ref_axis',(0.,0.,1.)) ;
#123142=DIRECTION('center_axis',(1.,0.,0.)) ;
#123143=DIRECTION('ref_axis',(0.,0.,-1.)) ;
#123144=DIRECTION('center_axis',(-1.,0.,0.)) ;
#123145=DIRECTION('ref_axis',(0.,0.,1.)) ;
#123146=DIRECTION('center_axis',(0.,1.,0.)) ;
#123147=DIRECTION('ref_axis',(0.,0.,1.)) ;
#123148=DIRECTION('center_axis',(0.,1.,0.)) ;
#123149=DIRECTION('ref_axis',(0.,0.,1.)) ;
#123150=DIRECTION('center_axis',(0.,1.,0.)) ;
#123151=DIRECTION('ref_axis',(1.,0.,0.)) ;
#123152=DIRECTION('center_axis',(0.,0.,1.)) ;
#123153=DIRECTION('ref_axis',(-1.,0.,0.)) ;
#123154=DIRECTION('center_axis',(0.,1.,0.)) ;
#123155=DIRECTION('ref_axis',(1.,0.,0.)) ;
#123156=DIRECTION('center_axis',(0.,0.,-1.)) ;
#123157=DIRECTION('ref_axis',(1.,0.,0.)) ;
#123158=DIRECTION('center_axis',(0.,0.,1.)) ;
#123159=DIRECTION('ref_axis',(1.,0.,0.)) ;
#123160=DIRECTION('center_axis',(0.,0.,1.)) ;
#123161=DIRECTION('ref_axis',(1.,0.,0.)) ;
#123162=DIRECTION('center_axis',(0.,0.,-1.)) ;
#123163=DIRECTION('ref_axis',(-1.,0.,0.)) ;
#123164=DIRECTION('center_axis',(-6.50521303491301E-15,0.,1.)) ;
#123165=DIRECTION('ref_axis',(1.,0.,6.50521303491301E-15)) ;
#123166=DIRECTION('center_axis',(1.,0.,0.)) ;
#123167=DIRECTION('ref_axis',(0.,0.,-1.)) ;
#123168=DIRECTION('center_axis',(1.,0.,0.)) ;
#123169=DIRECTION('ref_axis',(0.,0.,-1.)) ;
#123170=DIRECTION('center_axis',(1.,0.,0.)) ;
#123171=DIRECTION('ref_axis',(0.,0.,-1.)) ;
#123172=DIRECTION('center_axis',(1.,-1.41059322098675E-29,8.67361737988404E-15)) ;
#123173=DIRECTION('ref_axis',(8.67361737988404E-15,0.,-1.)) ;
#123174=DIRECTION('center_axis',(1.,0.,0.)) ;
#123175=DIRECTION('ref_axis',(0.,0.,-1.)) ;
#123176=DIRECTION('center_axis',(1.,0.,1.73472347597681E-14)) ;
#123177=DIRECTION('ref_axis',(1.73472347597681E-14,0.,-1.)) ;
#123178=DIRECTION('center_axis',(-1.,0.,0.)) ;
#123179=DIRECTION('ref_axis',(0.,0.,1.)) ;
#123180=DIRECTION('center_axis',(1.,0.,0.)) ;
#123181=DIRECTION('ref_axis',(0.,0.,-1.)) ;
#123182=DIRECTION('center_axis',(1.,0.,0.)) ;
#123183=DIRECTION('ref_axis',(0.,0.,-1.)) ;
#123184=DIRECTION('center_axis',(-7.04731412115582E-15,0.,-1.)) ;
#123185=DIRECTION('ref_axis',(-1.,0.,7.04731412115582E-15)) ;
#123186=DIRECTION('center_axis',(1.,0.,0.)) ;
#123187=DIRECTION('ref_axis',(0.,0.,-1.)) ;
#123188=DIRECTION('center_axis',(-6.50521303491307E-15,0.,1.)) ;
#123189=DIRECTION('ref_axis',(1.,0.,6.50521303491307E-15)) ;
#123190=DIRECTION('center_axis',(0.,0.,-1.)) ;
#123191=DIRECTION('ref_axis',(-1.,0.,0.)) ;
#123192=DIRECTION('center_axis',(-0.422618261740697,5.55398348498559E-17,
0.906307787036651)) ;
#123193=DIRECTION('ref_axis',(0.906307787036651,-7.29829988871486E-33,0.422618261740697)) ;
#123194=DIRECTION('center_axis',(0.422618261740697,-5.55398348498559E-17,
-0.906307787036651)) ;
#123195=DIRECTION('ref_axis',(-0.906307787036651,1.61222584863515E-33,-0.422618261740697)) ;
#123196=DIRECTION('center_axis',(-0.422618261740697,5.55398348498559E-17,
0.906307787036651)) ;
#123197=DIRECTION('ref_axis',(0.906307787036651,-1.61222584863515E-33,0.422618261740697)) ;
#123198=DIRECTION('center_axis',(0.422618261740697,-5.55398348498559E-17,
-0.906307787036651)) ;
#123199=DIRECTION('ref_axis',(-0.906307787036651,1.03797877997344E-32,-0.422618261740697)) ;
#123200=DIRECTION('center_axis',(0.,0.,1.)) ;
#123201=DIRECTION('ref_axis',(1.,0.,0.)) ;
#123202=DIRECTION('center_axis',(7.01133629567814E-33,-8.97270763436279E-17,
-1.)) ;
#123203=DIRECTION('ref_axis',(-6.29106707073161E-49,-1.,8.97270763436279E-17)) ;
#123204=DIRECTION('center_axis',(7.01133629567814E-33,-8.97270763436279E-17,
1.)) ;
#123205=DIRECTION('ref_axis',(6.29106707073161E-49,1.,8.97270763436279E-17)) ;
#123206=DIRECTION('center_axis',(1.,0.,0.)) ;
#123207=DIRECTION('ref_axis',(0.,0.,-1.)) ;
#123208=DIRECTION('center_axis',(0.,-4.8455963016112E-16,1.)) ;
#123209=DIRECTION('ref_axis',(0.,-1.,-4.8455963016112E-16)) ;
#123210=DIRECTION('center_axis',(0.,4.8455963016112E-16,-1.)) ;
#123211=DIRECTION('ref_axis',(0.,-1.,-4.8455963016112E-16)) ;
#123212=DIRECTION('center_axis',(0.,0.,-1.)) ;
#123213=DIRECTION('ref_axis',(-1.,0.,0.)) ;
#123214=DIRECTION('center_axis',(0.,0.,-1.)) ;
#123215=DIRECTION('ref_axis',(-1.,0.,0.)) ;
#123216=DIRECTION('center_axis',(1.,0.,0.)) ;
#123217=DIRECTION('ref_axis',(0.,0.,-1.)) ;
#123218=DIRECTION('center_axis',(-7.01133629567814E-33,8.97270763436279E-17,
1.)) ;
#123219=DIRECTION('ref_axis',(0.,-1.,0.)) ;
#123220=DIRECTION('center_axis',(1.,0.,0.)) ;
#123221=DIRECTION('ref_axis',(0.,0.,-1.)) ;
#123222=DIRECTION('center_axis',(-1.,0.,-7.01133629567814E-33)) ;
#123223=DIRECTION('ref_axis',(-7.01133629567814E-33,0.,1.)) ;
#123224=DIRECTION('center_axis',(1.,0.,0.)) ;
#123225=DIRECTION('ref_axis',(0.,0.,-1.)) ;
#123226=DIRECTION('center_axis',(1.,0.,0.)) ;
#123227=DIRECTION('ref_axis',(0.,0.,-1.)) ;
#123228=DIRECTION('center_axis',(0.,1.,0.)) ;
#123229=DIRECTION('ref_axis',(1.,0.,0.)) ;
#123230=DIRECTION('center_axis',(-7.01133629567814E-33,8.97270763436279E-17,
-1.)) ;
#123231=DIRECTION('ref_axis',(0.,1.,0.)) ;
#123232=DIRECTION('center_axis',(1.,0.,0.)) ;
#123233=DIRECTION('ref_axis',(0.,0.,-1.)) ;
#123234=DIRECTION('center_axis',(-1.,0.,7.01133629567814E-33)) ;
#123235=DIRECTION('ref_axis',(7.01133629567814E-33,0.,1.)) ;
#123236=DIRECTION('center_axis',(1.,0.,0.)) ;
#123237=DIRECTION('ref_axis',(0.,0.,-1.)) ;
#123238=DIRECTION('center_axis',(1.,0.,0.)) ;
#123239=DIRECTION('ref_axis',(0.,0.,-1.)) ;
#123240=DIRECTION('center_axis',(0.,1.,0.)) ;
#123241=DIRECTION('ref_axis',(1.,0.,0.)) ;
#123242=DIRECTION('center_axis',(1.,0.,0.)) ;
#123243=DIRECTION('ref_axis',(0.,0.,-1.)) ;
#123244=DIRECTION('center_axis',(0.,0.5,0.866025403784439)) ;
#123245=DIRECTION('ref_axis',(0.,-0.866025403784439,0.5)) ;
#123246=DIRECTION('center_axis',(0.866025403784441,0.499999999999997,-2.168404344971E-15)) ;
#123247=DIRECTION('ref_axis',(-0.499999999999997,0.866025403784441,-1.29696145180704E-31)) ;
#123248=DIRECTION('center_axis',(-7.01133629567814E-33,8.97270763436279E-17,
1.)) ;
#123249=DIRECTION('ref_axis',(0.,-1.,0.)) ;
#123250=DIRECTION('center_axis',(1.,0.,0.)) ;
#123251=DIRECTION('ref_axis',(0.,0.,-1.)) ;
#123252=DIRECTION('center_axis',(-2.16840434497101E-15,0.499999999999998,
-0.86602540378444)) ;
#123253=DIRECTION('ref_axis',(-3.01985296231538E-32,0.86602540378444,0.499999999999998)) ;
#123254=DIRECTION('center_axis',(0.866025403784439,0.5,0.)) ;
#123255=DIRECTION('ref_axis',(-0.5,0.866025403784439,0.)) ;
#123256=DIRECTION('center_axis',(-7.01133629567814E-33,8.97270763436279E-17,
-1.)) ;
#123257=DIRECTION('ref_axis',(0.,1.,0.)) ;
#123258=DIRECTION('center_axis',(0.,0.,-1.)) ;
#123259=DIRECTION('ref_axis',(-1.,0.,0.)) ;
#123260=DIRECTION('',(2.47817639425258E-16,-1.,0.)) ;
#123261=DIRECTION('',(0.970142500145333,0.24253562503633,0.)) ;
#123262=DIRECTION('',(0.,1.,0.)) ;
#123263=DIRECTION('',(-0.707106781186549,0.707106781186546,0.)) ;
#123264=DIRECTION('center_axis',(0.432731067584771,0.,-0.901523057468274)) ;
#123265=DIRECTION('ref_axis',(-0.901523057468274,0.,-0.432731067584771)) ;
#123266=DIRECTION('',(0.,-1.,0.)) ;
#123267=DIRECTION('',(0.879462917689188,0.219865729422294,0.42214220049081)) ;
#123268=DIRECTION('',(0.,1.,0.)) ;
#123269=DIRECTION('',(-0.669589480006976,0.669589480006974,-0.321402950403348)) ;
#123270=DIRECTION('center_axis',(1.,0.,0.)) ;
#123271=DIRECTION('ref_axis',(0.,0.,-1.)) ;
#123272=DIRECTION('',(0.,0.,-1.)) ;
#123273=DIRECTION('center_axis',(-1.,0.,0.)) ;
#123274=DIRECTION('ref_axis',(0.,0.461934418836862,-0.886914084167035)) ;
#123275=DIRECTION('',(0.,1.,0.)) ;
#123276=DIRECTION('center_axis',(-1.,-2.53099280113937E-14,-3.2268794886738E-14)) ;
#123277=DIRECTION('ref_axis',(-3.67811937460755E-14,0.901523057469949,0.432731067581281)) ;
#123278=DIRECTION('',(0.,0.,-1.)) ;
#123279=DIRECTION('center_axis',(-1.,-2.53099280113875E-14,3.22687948867301E-14)) ;
#123280=DIRECTION('ref_axis',(-3.67811937461193E-14,0.901523057468688,-0.432731067583908)) ;
#123281=DIRECTION('center_axis',(-1.,2.82235702682257E-14,2.6227280381046E-14)) ;
#123282=DIRECTION('ref_axis',(-3.62987828887412E-14,-0.461934418839581,
-0.886914084165619)) ;
#123283=DIRECTION('center_axis',(0.432731067584771,0.,0.901523057468274)) ;
#123284=DIRECTION('ref_axis',(0.901523057468274,0.,-0.432731067584771)) ;
#123285=DIRECTION('',(-0.879462917689188,-0.219865729422294,0.42214220049081)) ;
#123286=DIRECTION('',(0.,1.,0.)) ;
#123287=DIRECTION('',(0.669589480006976,-0.669589480006974,-0.321402950403348)) ;
#123288=DIRECTION('center_axis',(0.,0.,1.)) ;
#123289=DIRECTION('ref_axis',(1.,0.,0.)) ;
#123290=DIRECTION('',(-2.47817639425258E-16,1.,0.)) ;
#123291=DIRECTION('',(0.707106781186549,-0.707106781186546,0.)) ;
#123292=DIRECTION('',(0.,-1.,0.)) ;
#123293=DIRECTION('',(-0.970142500145333,-0.24253562503633,0.)) ;
#123294=DIRECTION('center_axis',(0.,0.,-1.)) ;
#123295=DIRECTION('ref_axis',(-1.,0.,0.)) ;
#123296=DIRECTION('',(2.47817639425258E-16,-1.,0.)) ;
#123297=DIRECTION('',(0.970142500145333,0.24253562503633,0.)) ;
#123298=DIRECTION('',(0.,1.,0.)) ;
#123299=DIRECTION('',(-0.707106781186549,0.707106781186546,0.)) ;
#123300=DIRECTION('center_axis',(0.432731067584771,0.,-0.901523057468274)) ;
#123301=DIRECTION('ref_axis',(-0.901523057468274,0.,-0.432731067584771)) ;
#123302=DIRECTION('',(0.,-1.,0.)) ;
#123303=DIRECTION('',(0.879462917689188,0.219865729422294,0.42214220049081)) ;
#123304=DIRECTION('',(0.,1.,0.)) ;
#123305=DIRECTION('',(-0.669589480006976,0.669589480006974,-0.321402950403348)) ;
#123306=DIRECTION('center_axis',(1.,0.,0.)) ;
#123307=DIRECTION('ref_axis',(0.,0.,-1.)) ;
#123308=DIRECTION('',(0.,0.,-1.)) ;
#123309=DIRECTION('center_axis',(-1.,1.4111785134113E-14,-1.31136401905232E-14)) ;
#123310=DIRECTION('ref_axis',(1.814939144438E-14,0.461934418840836,-0.886914084164965)) ;
#123311=DIRECTION('',(0.,1.,0.)) ;
#123312=DIRECTION('center_axis',(-1.,0.,0.)) ;
#123313=DIRECTION('ref_axis',(0.,0.901523057470446,0.432731067580246)) ;
#123314=DIRECTION('',(0.,0.,-1.)) ;
#123315=DIRECTION('center_axis',(-1.,-2.53099280113875E-14,3.22687948867301E-14)) ;
#123316=DIRECTION('ref_axis',(-3.6781193746113E-14,0.901523057468839,-0.432731067583594)) ;
#123317=DIRECTION('center_axis',(-1.,2.82235702682248E-14,2.6227280381044E-14)) ;
#123318=DIRECTION('ref_axis',(-3.62987828887609E-14,-0.46193441884108,-0.886914084164838)) ;
#123319=DIRECTION('center_axis',(0.432731067584771,0.,0.901523057468274)) ;
#123320=DIRECTION('ref_axis',(0.901523057468274,0.,-0.432731067584771)) ;
#123321=DIRECTION('',(-0.879462917689188,-0.219865729422294,0.42214220049081)) ;
#123322=DIRECTION('',(0.,1.,0.)) ;
#123323=DIRECTION('',(0.669589480006976,-0.669589480006974,-0.321402950403348)) ;
#123324=DIRECTION('center_axis',(0.,0.,1.)) ;
#123325=DIRECTION('ref_axis',(1.,0.,0.)) ;
#123326=DIRECTION('',(-2.47817639425258E-16,1.,0.)) ;
#123327=DIRECTION('',(0.707106781186549,-0.707106781186546,0.)) ;
#123328=DIRECTION('',(0.,-1.,0.)) ;
#123329=DIRECTION('',(-0.970142500145333,-0.24253562503633,0.)) ;
#123330=DIRECTION('center_axis',(0.,0.,-1.)) ;
#123331=DIRECTION('ref_axis',(-1.,0.,0.)) ;
#123332=DIRECTION('',(2.47817639425258E-16,-1.,0.)) ;
#123333=DIRECTION('',(0.970142500145333,0.24253562503633,0.)) ;
#123334=DIRECTION('',(0.,1.,0.)) ;
#123335=DIRECTION('',(-0.707106781186549,0.707106781186546,0.)) ;
#123336=DIRECTION('center_axis',(0.432731067584771,0.,-0.901523057468274)) ;
#123337=DIRECTION('ref_axis',(-0.901523057468274,0.,-0.432731067584771)) ;
#123338=DIRECTION('',(0.,-1.,0.)) ;
#123339=DIRECTION('',(0.879462917689188,0.219865729422294,0.42214220049081)) ;
#123340=DIRECTION('',(0.,1.,0.)) ;
#123341=DIRECTION('',(-0.669589480006976,0.669589480006974,-0.321402950403348)) ;
#123342=DIRECTION('center_axis',(1.,0.,0.)) ;
#123343=DIRECTION('ref_axis',(0.,0.,-1.)) ;
#123344=DIRECTION('',(0.,0.,-1.)) ;
#123345=DIRECTION('center_axis',(-1.,1.4111785134113E-14,-1.31136401905232E-14)) ;
#123346=DIRECTION('ref_axis',(1.81493914443659E-14,0.461934418838905,-0.886914084165971)) ;
#123347=DIRECTION('',(0.,1.,0.)) ;
#123348=DIRECTION('center_axis',(-1.,0.,0.)) ;
#123349=DIRECTION('ref_axis',(0.,0.901523057469797,0.432731067581597)) ;
#123350=DIRECTION('',(0.,0.,-1.)) ;
#123351=DIRECTION('center_axis',(-1.,0.,0.)) ;
#123352=DIRECTION('ref_axis',(0.,0.901523057468153,-0.432731067585023)) ;
#123353=DIRECTION('center_axis',(-1.,1.41117851341127E-14,1.31136401905217E-14)) ;
#123354=DIRECTION('ref_axis',(-1.8149391444346E-14,-0.461934418836372,-0.88691408416729)) ;
#123355=DIRECTION('center_axis',(0.432731067584771,0.,0.901523057468274)) ;
#123356=DIRECTION('ref_axis',(0.901523057468274,0.,-0.432731067584771)) ;
#123357=DIRECTION('',(-0.879462917689188,-0.219865729422294,0.42214220049081)) ;
#123358=DIRECTION('',(0.,1.,0.)) ;
#123359=DIRECTION('',(0.669589480006976,-0.669589480006974,-0.321402950403348)) ;
#123360=DIRECTION('center_axis',(0.,0.,1.)) ;
#123361=DIRECTION('ref_axis',(1.,0.,0.)) ;
#123362=DIRECTION('',(-2.47817639425258E-16,1.,0.)) ;
#123363=DIRECTION('',(0.707106781186549,-0.707106781186546,0.)) ;
#123364=DIRECTION('',(0.,-1.,0.)) ;
#123365=DIRECTION('',(-0.970142500145333,-0.24253562503633,0.)) ;
#123366=DIRECTION('center_axis',(0.,0.,-1.)) ;
#123367=DIRECTION('ref_axis',(-1.,0.,0.)) ;
#123368=DIRECTION('',(2.47817639425258E-16,-1.,0.)) ;
#123369=DIRECTION('',(0.970142500145333,0.24253562503633,0.)) ;
#123370=DIRECTION('',(0.,1.,0.)) ;
#123371=DIRECTION('',(-0.707106781186549,0.707106781186546,0.)) ;
#123372=DIRECTION('center_axis',(0.432731067584771,0.,-0.901523057468274)) ;
#123373=DIRECTION('ref_axis',(-0.901523057468274,0.,-0.432731067584771)) ;
#123374=DIRECTION('',(0.,-1.,0.)) ;
#123375=DIRECTION('',(0.879462917689188,0.219865729422294,0.42214220049081)) ;
#123376=DIRECTION('',(0.,1.,0.)) ;
#123377=DIRECTION('',(-0.669589480006976,0.669589480006974,-0.321402950403348)) ;
#123378=DIRECTION('center_axis',(1.,0.,0.)) ;
#123379=DIRECTION('ref_axis',(0.,0.,-1.)) ;
#123380=DIRECTION('',(0.,0.,-1.)) ;
#123381=DIRECTION('center_axis',(-1.,1.41117851341151E-14,-1.3113640190524E-14)) ;
#123382=DIRECTION('ref_axis',(1.81493914443558E-14,0.461934418837284,-0.886914084166815)) ;
#123383=DIRECTION('',(0.,1.,0.)) ;
#123384=DIRECTION('center_axis',(-1.,0.,0.)) ;
#123385=DIRECTION('ref_axis',(0.,0.901523057469908,0.432731067581367)) ;
#123386=DIRECTION('',(0.,0.,-1.)) ;
#123387=DIRECTION('center_axis',(-1.,0.,0.)) ;
#123388=DIRECTION('ref_axis',(0.,0.90152305746791,-0.432731067585528)) ;
#123389=DIRECTION('center_axis',(-1.,1.41117851341131E-14,1.31136401905226E-14)) ;
#123390=DIRECTION('ref_axis',(-1.8149391444372E-14,-0.461934418839798,-0.886914084165506)) ;
#123391=DIRECTION('center_axis',(0.432731067584771,0.,0.901523057468274)) ;
#123392=DIRECTION('ref_axis',(0.901523057468274,0.,-0.432731067584771)) ;
#123393=DIRECTION('',(-0.879462917689188,-0.219865729422294,0.42214220049081)) ;
#123394=DIRECTION('',(0.,1.,0.)) ;
#123395=DIRECTION('',(0.669589480006976,-0.669589480006974,-0.321402950403348)) ;
#123396=DIRECTION('center_axis',(0.,0.,1.)) ;
#123397=DIRECTION('ref_axis',(1.,0.,0.)) ;
#123398=DIRECTION('',(-2.47817639425258E-16,1.,0.)) ;
#123399=DIRECTION('',(0.707106781186549,-0.707106781186546,0.)) ;
#123400=DIRECTION('',(0.,-1.,0.)) ;
#123401=DIRECTION('',(-0.970142500145333,-0.24253562503633,0.)) ;
#123402=DIRECTION('center_axis',(0.,0.,-1.)) ;
#123403=DIRECTION('ref_axis',(-1.,0.,0.)) ;
#123404=DIRECTION('',(2.47817639425258E-16,-1.,0.)) ;
#123405=DIRECTION('',(0.970142500145333,0.24253562503633,0.)) ;
#123406=DIRECTION('',(0.,1.,0.)) ;
#123407=DIRECTION('',(-0.707106781186549,0.707106781186546,0.)) ;
#123408=DIRECTION('center_axis',(0.432731067584771,0.,-0.901523057468274)) ;
#123409=DIRECTION('ref_axis',(-0.901523057468274,0.,-0.432731067584771)) ;
#123410=DIRECTION('',(0.,-1.,0.)) ;
#123411=DIRECTION('',(0.879462917689188,0.219865729422294,0.42214220049081)) ;
#123412=DIRECTION('',(0.,1.,0.)) ;
#123413=DIRECTION('',(-0.669589480006976,0.669589480006974,-0.321402950403348)) ;
#123414=DIRECTION('center_axis',(1.,0.,0.)) ;
#123415=DIRECTION('ref_axis',(0.,0.,-1.)) ;
#123416=DIRECTION('',(0.,0.,-1.)) ;
#123417=DIRECTION('center_axis',(-1.,1.4111785134114E-14,-1.31136401905236E-14)) ;
#123418=DIRECTION('ref_axis',(1.81493914443555E-14,0.461934418837353,-0.886914084166779)) ;
#123419=DIRECTION('',(0.,1.,0.)) ;
#123420=DIRECTION('center_axis',(-1.,0.,0.)) ;
#123421=DIRECTION('ref_axis',(0.,0.901523057469398,0.432731067582429)) ;
#123422=DIRECTION('',(0.,0.,-1.)) ;
#123423=DIRECTION('center_axis',(-1.,0.,0.)) ;
#123424=DIRECTION('ref_axis',(0.,0.901523057469399,-0.432731067582427)) ;
#123425=DIRECTION('center_axis',(-1.,2.82235702682282E-14,2.62272803810477E-14)) ;
#123426=DIRECTION('ref_axis',(-3.62987828887127E-14,-0.461934418837437,
-0.886914084166736)) ;
#123427=DIRECTION('center_axis',(0.432731067584771,0.,0.901523057468274)) ;
#123428=DIRECTION('ref_axis',(0.901523057468274,0.,-0.432731067584771)) ;
#123429=DIRECTION('',(-0.879462917689188,-0.219865729422294,0.42214220049081)) ;
#123430=DIRECTION('',(0.,1.,0.)) ;
#123431=DIRECTION('',(0.669589480006976,-0.669589480006974,-0.321402950403348)) ;
#123432=DIRECTION('center_axis',(0.,0.,1.)) ;
#123433=DIRECTION('ref_axis',(1.,0.,0.)) ;
#123434=DIRECTION('',(-2.47817639425258E-16,1.,0.)) ;
#123435=DIRECTION('',(0.707106781186549,-0.707106781186546,0.)) ;
#123436=DIRECTION('',(0.,-1.,0.)) ;
#123437=DIRECTION('',(-0.970142500145333,-0.24253562503633,0.)) ;
#123438=DIRECTION('center_axis',(0.,0.,-1.)) ;
#123439=DIRECTION('ref_axis',(-1.,0.,0.)) ;
#123440=DIRECTION('',(2.47817639425258E-16,-1.,0.)) ;
#123441=DIRECTION('',(0.970142500145333,0.24253562503633,0.)) ;
#123442=DIRECTION('',(0.,1.,0.)) ;
#123443=DIRECTION('',(-0.707106781186549,0.707106781186546,0.)) ;
#123444=DIRECTION('center_axis',(0.432731067584771,0.,-0.901523057468274)) ;
#123445=DIRECTION('ref_axis',(-0.901523057468274,0.,-0.432731067584771)) ;
#123446=DIRECTION('',(0.,-1.,0.)) ;
#123447=DIRECTION('',(0.879462917689188,0.219865729422294,0.42214220049081)) ;
#123448=DIRECTION('',(0.,1.,0.)) ;
#123449=DIRECTION('',(-0.669589480006976,0.669589480006974,-0.321402950403348)) ;
#123450=DIRECTION('center_axis',(1.,0.,0.)) ;
#123451=DIRECTION('ref_axis',(0.,0.,-1.)) ;
#123452=DIRECTION('',(0.,0.,-1.)) ;
#123453=DIRECTION('center_axis',(-1.,0.,0.)) ;
#123454=DIRECTION('ref_axis',(0.,0.4619344188388,-0.886914084166026)) ;
#123455=DIRECTION('',(0.,1.,0.)) ;
#123456=DIRECTION('center_axis',(-1.,0.,0.)) ;
#123457=DIRECTION('ref_axis',(0.,0.901523057467731,0.432731067585901)) ;
#123458=DIRECTION('',(0.,0.,-1.)) ;
#123459=DIRECTION('center_axis',(-1.,0.,0.)) ;
#123460=DIRECTION('ref_axis',(0.,0.901523057469231,-0.432731067582777)) ;
#123461=DIRECTION('center_axis',(-1.,2.82235702682263E-14,2.62272803810454E-14)) ;
#123462=DIRECTION('ref_axis',(-3.62987828886724E-14,-0.461934418834871,
-0.886914084168072)) ;
#123463=DIRECTION('center_axis',(0.432731067584771,0.,0.901523057468274)) ;
#123464=DIRECTION('ref_axis',(0.901523057468274,0.,-0.432731067584771)) ;
#123465=DIRECTION('',(-0.879462917689188,-0.219865729422294,0.42214220049081)) ;
#123466=DIRECTION('',(0.,1.,0.)) ;
#123467=DIRECTION('',(0.669589480006976,-0.669589480006974,-0.321402950403348)) ;
#123468=DIRECTION('center_axis',(0.,0.,1.)) ;
#123469=DIRECTION('ref_axis',(1.,0.,0.)) ;
#123470=DIRECTION('',(-2.47817639425258E-16,1.,0.)) ;
#123471=DIRECTION('',(0.707106781186549,-0.707106781186546,0.)) ;
#123472=DIRECTION('',(0.,-1.,0.)) ;
#123473=DIRECTION('',(-0.970142500145333,-0.24253562503633,0.)) ;
#123474=DIRECTION('center_axis',(0.,0.,-1.)) ;
#123475=DIRECTION('ref_axis',(-1.,0.,0.)) ;
#123476=DIRECTION('',(2.47817639425258E-16,-1.,0.)) ;
#123477=DIRECTION('',(0.970142500145333,0.24253562503633,0.)) ;
#123478=DIRECTION('',(0.,1.,0.)) ;
#123479=DIRECTION('',(-0.707106781186549,0.707106781186546,0.)) ;
#123480=DIRECTION('center_axis',(0.432731067584771,0.,-0.901523057468274)) ;
#123481=DIRECTION('ref_axis',(-0.901523057468274,0.,-0.432731067584771)) ;
#123482=DIRECTION('',(0.,-1.,0.)) ;
#123483=DIRECTION('',(0.879462917689188,0.219865729422294,0.42214220049081)) ;
#123484=DIRECTION('',(0.,1.,0.)) ;
#123485=DIRECTION('',(-0.669589480006976,0.669589480006974,-0.321402950403348)) ;
#123486=DIRECTION('center_axis',(1.,0.,0.)) ;
#123487=DIRECTION('ref_axis',(0.,0.,-1.)) ;
#123488=DIRECTION('',(0.,0.,-1.)) ;
#123489=DIRECTION('center_axis',(-1.,0.,0.)) ;
#123490=DIRECTION('ref_axis',(0.,0.461934418836445,-0.886914084167252)) ;
#123491=DIRECTION('',(0.,1.,0.)) ;
#123492=DIRECTION('center_axis',(-1.,0.,0.)) ;
#123493=DIRECTION('ref_axis',(0.,0.901523057468085,0.432731067585165)) ;
#123494=DIRECTION('',(0.,0.,-1.)) ;
#123495=DIRECTION('center_axis',(-1.,0.,0.)) ;
#123496=DIRECTION('ref_axis',(0.,0.901523057468215,-0.432731067584893)) ;
#123497=DIRECTION('center_axis',(-1.,2.82235702682288E-14,2.62272803810472E-14)) ;
#123498=DIRECTION('ref_axis',(-3.62987828886828E-14,-0.461934418835395,
-0.886914084167799)) ;
#123499=DIRECTION('center_axis',(0.432731067584771,0.,0.901523057468274)) ;
#123500=DIRECTION('ref_axis',(0.901523057468274,0.,-0.432731067584771)) ;
#123501=DIRECTION('',(-0.879462917689188,-0.219865729422294,0.42214220049081)) ;
#123502=DIRECTION('',(0.,1.,0.)) ;
#123503=DIRECTION('',(0.669589480006976,-0.669589480006974,-0.321402950403348)) ;
#123504=DIRECTION('center_axis',(0.,0.,1.)) ;
#123505=DIRECTION('ref_axis',(1.,0.,0.)) ;
#123506=DIRECTION('',(-2.47817639425258E-16,1.,0.)) ;
#123507=DIRECTION('',(0.707106781186549,-0.707106781186546,0.)) ;
#123508=DIRECTION('',(0.,-1.,0.)) ;
#123509=DIRECTION('',(-0.970142500145333,-0.24253562503633,0.)) ;
#123510=DIRECTION('center_axis',(0.,0.,-1.)) ;
#123511=DIRECTION('ref_axis',(-1.,0.,0.)) ;
#123512=DIRECTION('',(2.47817639425258E-16,-1.,0.)) ;
#123513=DIRECTION('',(0.970142500145333,0.24253562503633,0.)) ;
#123514=DIRECTION('',(0.,1.,0.)) ;
#123515=DIRECTION('',(-0.707106781186549,0.707106781186546,0.)) ;
#123516=DIRECTION('center_axis',(0.432731067584771,0.,-0.901523057468274)) ;
#123517=DIRECTION('ref_axis',(-0.901523057468274,0.,-0.432731067584771)) ;
#123518=DIRECTION('',(0.,-1.,0.)) ;
#123519=DIRECTION('',(0.879462917689188,0.219865729422294,0.42214220049081)) ;
#123520=DIRECTION('',(0.,1.,0.)) ;
#123521=DIRECTION('',(-0.669589480006976,0.669589480006974,-0.321402950403348)) ;
#123522=DIRECTION('center_axis',(1.,0.,0.)) ;
#123523=DIRECTION('ref_axis',(0.,0.,-1.)) ;
#123524=DIRECTION('',(0.,0.,-1.)) ;
#123525=DIRECTION('center_axis',(-1.,0.,0.)) ;
#123526=DIRECTION('ref_axis',(0.,0.461934418837712,-0.886914084166592)) ;
#123527=DIRECTION('',(0.,1.,0.)) ;
#123528=DIRECTION('center_axis',(-1.,0.,0.)) ;
#123529=DIRECTION('ref_axis',(0.,0.901523057468494,0.432731067584312)) ;
#123530=DIRECTION('',(0.,0.,-1.)) ;
#123531=DIRECTION('center_axis',(-1.,0.,0.)) ;
#123532=DIRECTION('ref_axis',(0.,0.901523057467713,-0.43273106758594)) ;
#123533=DIRECTION('center_axis',(-1.,2.82235702682276E-14,2.62272803810463E-14)) ;
#123534=DIRECTION('ref_axis',(-3.62987828887053E-14,-0.461934418837035,
-0.886914084166945)) ;
#123535=DIRECTION('center_axis',(0.432731067584771,0.,0.901523057468274)) ;
#123536=DIRECTION('ref_axis',(0.901523057468274,0.,-0.432731067584771)) ;
#123537=DIRECTION('',(-0.879462917689188,-0.219865729422294,0.42214220049081)) ;
#123538=DIRECTION('',(0.,1.,0.)) ;
#123539=DIRECTION('',(0.669589480006976,-0.669589480006974,-0.321402950403348)) ;
#123540=DIRECTION('center_axis',(0.,0.,1.)) ;
#123541=DIRECTION('ref_axis',(1.,0.,0.)) ;
#123542=DIRECTION('',(-2.47817639425258E-16,1.,0.)) ;
#123543=DIRECTION('',(0.707106781186549,-0.707106781186546,0.)) ;
#123544=DIRECTION('',(0.,-1.,0.)) ;
#123545=DIRECTION('',(-0.970142500145333,-0.24253562503633,0.)) ;
#123546=DIRECTION('center_axis',(0.,0.,-1.)) ;
#123547=DIRECTION('ref_axis',(-1.,0.,0.)) ;
#123548=DIRECTION('',(0.970142500145333,0.24253562503633,0.)) ;
#123549=DIRECTION('',(0.,1.,0.)) ;
#123550=DIRECTION('',(-0.707106781186549,0.707106781186546,0.)) ;
#123551=DIRECTION('',(2.47817639425258E-16,-1.,0.)) ;
#123552=DIRECTION('center_axis',(0.432731067584771,0.,-0.901523057468274)) ;
#123553=DIRECTION('ref_axis',(-0.901523057468274,0.,-0.432731067584771)) ;
#123554=DIRECTION('',(0.,-1.,0.)) ;
#123555=DIRECTION('',(0.879462917689188,0.219865729422294,0.42214220049081)) ;
#123556=DIRECTION('',(0.,1.,0.)) ;
#123557=DIRECTION('',(-0.669589480006976,0.669589480006974,-0.321402950403348)) ;
#123558=DIRECTION('center_axis',(1.,0.,0.)) ;
#123559=DIRECTION('ref_axis',(0.,0.,-1.)) ;
#123560=DIRECTION('',(0.,0.,-1.)) ;
#123561=DIRECTION('center_axis',(-1.,-1.41117851341144E-14,1.31136401905238E-14)) ;
#123562=DIRECTION('ref_axis',(-1.81493914443513E-14,0.461934418836728,-0.886914084167105)) ;
#123563=DIRECTION('',(0.,1.,0.)) ;
#123564=DIRECTION('center_axis',(-1.,0.,0.)) ;
#123565=DIRECTION('ref_axis',(0.,0.901523057468354,0.432731067584604)) ;
#123566=DIRECTION('',(0.,0.,-1.)) ;
#123567=DIRECTION('center_axis',(-1.,0.,0.)) ;
#123568=DIRECTION('ref_axis',(0.,0.901523057468327,-0.43273106758466)) ;
#123569=DIRECTION('center_axis',(-1.,0.,0.)) ;
#123570=DIRECTION('ref_axis',(0.,-0.461934418836997,-0.886914084166965)) ;
#123571=DIRECTION('center_axis',(0.432731067584771,0.,0.901523057468274)) ;
#123572=DIRECTION('ref_axis',(0.901523057468274,0.,-0.432731067584771)) ;
#123573=DIRECTION('',(-0.879462917689188,-0.219865729422294,0.42214220049081)) ;
#123574=DIRECTION('',(0.,1.,0.)) ;
#123575=DIRECTION('',(0.669589480006976,-0.669589480006974,-0.321402950403348)) ;
#123576=DIRECTION('center_axis',(0.,0.,1.)) ;
#123577=DIRECTION('ref_axis',(1.,0.,0.)) ;
#123578=DIRECTION('',(0.,-1.,0.)) ;
#123579=DIRECTION('',(-0.970142500145333,-0.24253562503633,0.)) ;
#123580=DIRECTION('',(-2.47817639425258E-16,1.,0.)) ;
#123581=DIRECTION('',(0.707106781186549,-0.707106781186546,0.)) ;
#123582=DIRECTION('center_axis',(0.24253562503633,-0.970142500145333,0.)) ;
#123583=DIRECTION('ref_axis',(0.,0.,1.)) ;
#123584=DIRECTION('',(0.970142500145333,0.24253562503633,0.)) ;
#123585=DIRECTION('',(0.879462917689188,0.219865729422294,-0.42214220049081)) ;
#123586=DIRECTION('',(-0.879462917689188,-0.219865729422294,-0.42214220049081)) ;
#123587=DIRECTION('',(-0.970142500145333,-0.24253562503633,0.)) ;
#123588=DIRECTION('',(0.,0.,1.)) ;
#123589=DIRECTION('center_axis',(0.24253562503633,-0.970142500145333,0.)) ;
#123590=DIRECTION('ref_axis',(0.,0.,1.)) ;
#123591=DIRECTION('',(0.,0.,1.)) ;
#123592=DIRECTION('center_axis',(0.242535625036292,-0.970142500145342,-1.75219879118722E-13)) ;
#123593=DIRECTION('ref_axis',(0.965295032173275,0.241323758043293,-0.0998415978711228)) ;
#123594=DIRECTION('',(0.970142500145333,0.24253562503633,0.)) ;
#123595=DIRECTION('',(0.879462917689188,0.219865729422294,-0.42214220049081)) ;
#123596=DIRECTION('',(-0.879462917689188,-0.219865729422294,-0.42214220049081)) ;
#123597=DIRECTION('',(-0.970142500145333,-0.24253562503633,0.)) ;
#123598=DIRECTION('center_axis',(0.24253562503623,-0.970142500145358,7.11740252775332E-13)) ;
#123599=DIRECTION('ref_axis',(0.965295032194209,0.241323758048516,0.0998415976561007)) ;
#123600=DIRECTION('center_axis',(0.24253562503633,-0.970142500145333,0.)) ;
#123601=DIRECTION('ref_axis',(0.,0.,1.)) ;
#123602=DIRECTION('',(0.,0.,1.)) ;
#123603=DIRECTION('center_axis',(0.242535625036328,-0.970142500145333,9.12301849944342E-14)) ;
#123604=DIRECTION('ref_axis',(0.965295032195861,0.241323758048951,-0.0998415976390787)) ;
#123605=DIRECTION('',(0.970142500145333,0.24253562503633,0.)) ;
#123606=DIRECTION('',(0.879462917689188,0.219865729422294,-0.42214220049081)) ;
#123607=DIRECTION('',(-0.879462917689188,-0.219865729422294,-0.42214220049081)) ;
#123608=DIRECTION('',(-0.970142500145333,-0.24253562503633,0.)) ;
#123609=DIRECTION('center_axis',(0.242535625036328,-0.970142500145333,-9.12301849944342E-14)) ;
#123610=DIRECTION('ref_axis',(0.96529503220126,0.2413237580503,0.0998415975836097)) ;
#123611=DIRECTION('center_axis',(0.24253562503633,-0.970142500145333,0.)) ;
#123612=DIRECTION('ref_axis',(0.,0.,1.)) ;
#123613=DIRECTION('',(0.,0.,1.)) ;
#123614=DIRECTION('center_axis',(0.242535625036292,-0.970142500145342,-1.75943928203529E-13)) ;
#123615=DIRECTION('ref_axis',(0.965295032208283,0.241323758052046,-0.0998415975114907)) ;
#123616=DIRECTION('',(0.970142500145333,0.24253562503633,0.)) ;
#123617=DIRECTION('',(0.879462917689188,0.219865729422294,-0.42214220049081)) ;
#123618=DIRECTION('',(-0.879462917689188,-0.219865729422294,-0.42214220049081)) ;
#123619=DIRECTION('',(-0.970142500145333,-0.24253562503633,0.)) ;
#123620=DIRECTION('center_axis',(0.242535625036312,-0.970142500145337,-2.89619634903271E-15)) ;
#123621=DIRECTION('ref_axis',(0.965295032130061,0.241323758032493,0.0998415983150268)) ;
#123622=DIRECTION('center_axis',(0.24253562503633,-0.970142500145333,0.)) ;
#123623=DIRECTION('ref_axis',(0.,0.,1.)) ;
#123624=DIRECTION('',(0.,0.,1.)) ;
#123625=DIRECTION('center_axis',(0.24253562503623,-0.970142500145358,-7.11016203688594E-13)) ;
#123626=DIRECTION('ref_axis',(0.9652950321316,0.241323758032864,-0.0998415982992527)) ;
#123627=DIRECTION('',(0.970142500145333,0.24253562503633,0.)) ;
#123628=DIRECTION('',(0.879462917689188,0.219865729422294,-0.42214220049081)) ;
#123629=DIRECTION('',(-0.879462917689188,-0.219865729422294,-0.42214220049081)) ;
#123630=DIRECTION('',(-0.970142500145333,-0.24253562503633,0.)) ;
#123631=DIRECTION('center_axis',(0.242535625036245,-0.970142500145354,6.23406264128872E-13)) ;
#123632=DIRECTION('ref_axis',(0.965295032139512,0.241323758034849,0.0998415982179547)) ;
#123633=DIRECTION('center_axis',(0.24253562503633,-0.970142500145333,0.)) ;
#123634=DIRECTION('ref_axis',(0.,0.,1.)) ;
#123635=DIRECTION('',(0.,0.,1.)) ;
#123636=DIRECTION('center_axis',(0.24253562503623,-0.970142500145358,-7.11740252775329E-13)) ;
#123637=DIRECTION('ref_axis',(0.965295032122132,0.241323758030497,-0.0998415983965105)) ;
#123638=DIRECTION('',(0.970142500145333,0.24253562503633,0.)) ;
#123639=DIRECTION('',(0.879462917689188,0.219865729422294,-0.42214220049081)) ;
#123640=DIRECTION('',(-0.879462917689188,-0.219865729422294,-0.42214220049081)) ;
#123641=DIRECTION('',(-0.970142500145333,-0.24253562503633,0.)) ;
#123642=DIRECTION('center_axis',(0.242535625036312,-0.970142500145337,-2.89619634903485E-15)) ;
#123643=DIRECTION('ref_axis',(0.965295032134543,0.241323758033613,0.099841598268988)) ;
#123644=DIRECTION('center_axis',(0.24253562503633,-0.970142500145333,0.)) ;
#123645=DIRECTION('ref_axis',(0.,0.,1.)) ;
#123646=DIRECTION('',(0.,0.,1.)) ;
#123647=DIRECTION('center_axis',(0.242535625036328,-0.970142500145333,2.72966505896118E-13)) ;
#123648=DIRECTION('ref_axis',(0.965295032107306,0.241323758026793,-0.0998415985488062)) ;
#123649=DIRECTION('',(0.970142500145333,0.24253562503633,0.)) ;
#123650=DIRECTION('',(0.879462917689188,0.219865729422294,-0.42214220049081)) ;
#123651=DIRECTION('',(-0.879462917689188,-0.219865729422294,-0.42214220049081)) ;
#123652=DIRECTION('',(-0.970142500145333,-0.24253562503633,0.)) ;
#123653=DIRECTION('center_axis',(0.242535625036224,-0.970142500145359,8.01522339595377E-13)) ;
#123654=DIRECTION('ref_axis',(0.965295032121958,0.241323758030457,0.0998415983982931)) ;
#123655=DIRECTION('center_axis',(0.24253562503633,-0.970142500145333,0.)) ;
#123656=DIRECTION('ref_axis',(0.,0.,1.)) ;
#123657=DIRECTION('',(0.,0.,1.)) ;
#123658=DIRECTION('center_axis',(0.24253562503623,-0.970142500145358,-5.30003931873337E-13)) ;
#123659=DIRECTION('ref_axis',(0.965295032137309,0.241323758034273,-0.0998415982406524)) ;
#123660=DIRECTION('',(0.970142500145333,0.24253562503633,0.)) ;
#123661=DIRECTION('',(0.879462917689188,0.219865729422294,-0.42214220049081)) ;
#123662=DIRECTION('',(-0.879462917689188,-0.219865729422294,-0.42214220049081)) ;
#123663=DIRECTION('',(-0.970142500145333,-0.24253562503633,0.)) ;
#123664=DIRECTION('center_axis',(0.242535625036302,-0.97014250014534,-4.34429452349234E-15)) ;
#123665=DIRECTION('ref_axis',(0.965295032195617,0.241323758048871,0.0998415976416312)) ;
#123666=DIRECTION('center_axis',(0.24253562503633,-0.970142500145333,0.)) ;
#123667=DIRECTION('ref_axis',(0.,0.,1.)) ;
#123668=DIRECTION('',(0.,0.,1.)) ;
#123669=DIRECTION('center_axis',(0.242535625036271,-0.970142500145347,-3.54784052751878E-13)) ;
#123670=DIRECTION('ref_axis',(0.965295032201922,0.241323758050452,-0.0998415975768464)) ;
#123671=DIRECTION('',(0.970142500145333,0.24253562503633,0.)) ;
#123672=DIRECTION('',(0.879462917689188,0.219865729422294,-0.42214220049081)) ;
#123673=DIRECTION('',(-0.879462917689188,-0.219865729422294,-0.42214220049081)) ;
#123674=DIRECTION('',(-0.970142500145333,-0.24253562503633,0.)) ;
#123675=DIRECTION('center_axis',(0.242535625036271,-0.970142500145347,3.54784052753445E-13)) ;
#123676=DIRECTION('ref_axis',(0.965295032195717,0.2413237580489,0.0998415976405848)) ;
#123677=DIRECTION('center_axis',(-0.707106781186546,-0.707106781186549,
0.)) ;
#123678=DIRECTION('ref_axis',(0.,0.,-1.)) ;
#123679=DIRECTION('',(0.707106781186549,-0.707106781186546,0.)) ;
#123680=DIRECTION('',(0.669589480006976,-0.669589480006974,0.321402950403348)) ;
#123681=DIRECTION('',(-0.669589480006976,0.669589480006974,0.321402950403348)) ;
#123682=DIRECTION('',(-0.707106781186549,0.707106781186546,0.)) ;
#123683=DIRECTION('',(0.,0.,-1.)) ;
#123684=DIRECTION('center_axis',(-0.707106781186546,-0.707106781186549,
0.)) ;
#123685=DIRECTION('ref_axis',(0.,0.,-1.)) ;
#123686=DIRECTION('',(0.,0.,-1.)) ;
#123687=DIRECTION('center_axis',(0.707106781186535,0.70710678118656,4.97855948833419E-14)) ;
#123688=DIRECTION('ref_axis',(0.704497887013011,-0.704497887012992,0.0858222254921949)) ;
#123689=DIRECTION('',(0.707106781186549,-0.707106781186546,0.)) ;
#123690=DIRECTION('',(0.669589480006976,-0.669589480006974,0.321402950403348)) ;
#123691=DIRECTION('',(-0.669589480006976,0.669589480006974,0.321402950403348)) ;
#123692=DIRECTION('',(-0.707106781186549,0.707106781186546,0.)) ;
#123693=DIRECTION('center_axis',(0.707106781186531,0.707106781186564,-8.40823380250688E-14)) ;
#123694=DIRECTION('ref_axis',(0.704497887012093,-0.70449788701207,-0.0858222255072959)) ;
#123695=DIRECTION('center_axis',(-0.707106781186546,-0.707106781186549,
0.)) ;
#123696=DIRECTION('ref_axis',(0.,0.,-1.)) ;
#123697=DIRECTION('',(0.,0.,-1.)) ;
#123698=DIRECTION('center_axis',(0.707106781186544,0.707106781186551,7.74442587073954E-15)) ;
#123699=DIRECTION('ref_axis',(0.70449788701354,-0.704497887013534,0.0858222254834004)) ;
#123700=DIRECTION('',(0.707106781186549,-0.707106781186546,0.)) ;
#123701=DIRECTION('',(0.669589480006976,-0.669589480006974,0.321402950403348)) ;
#123702=DIRECTION('',(-0.669589480006976,0.669589480006974,0.321402950403348)) ;
#123703=DIRECTION('',(-0.707106781186549,0.707106781186546,0.)) ;
#123704=DIRECTION('center_axis',(0.707106781186537,0.707106781186558,-6.25085802423985E-14)) ;
#123705=DIRECTION('ref_axis',(0.704497887013265,-0.704497887013252,-0.0858222254879714)) ;
#123706=DIRECTION('center_axis',(-0.707106781186546,-0.707106781186549,
0.)) ;
#123707=DIRECTION('ref_axis',(0.,0.,-1.)) ;
#123708=DIRECTION('',(0.,0.,-1.)) ;
#123709=DIRECTION('center_axis',(0.707106781186549,0.707106781186546,1.65951982944667E-15)) ;
#123710=DIRECTION('ref_axis',(0.704497887013534,-0.704497887013537,0.0858222254834207)) ;
#123711=DIRECTION('',(0.707106781186549,-0.707106781186546,0.)) ;
#123712=DIRECTION('',(0.669589480006976,-0.669589480006974,0.321402950403348)) ;
#123713=DIRECTION('',(-0.669589480006976,0.669589480006974,0.321402950403348)) ;
#123714=DIRECTION('',(-0.707106781186549,0.707106781186546,0.)) ;
#123715=DIRECTION('center_axis',(0.707106781186547,0.707106781186548,-7.1912525942593E-15)) ;
#123716=DIRECTION('ref_axis',(0.704497887013064,-0.704497887013064,-0.0858222254911589)) ;
#123717=DIRECTION('center_axis',(-0.707106781186546,-0.707106781186549,
0.)) ;
#123718=DIRECTION('ref_axis',(0.,0.,-1.)) ;
#123719=DIRECTION('',(0.,0.,-1.)) ;
#123720=DIRECTION('center_axis',(0.707106781186549,0.707106781186546,4.42538621185838E-15)) ;
#123721=DIRECTION('ref_axis',(0.70449788701323,-0.704497887013233,0.0858222254884169)) ;
#123722=DIRECTION('',(0.707106781186549,-0.707106781186546,0.)) ;
#123723=DIRECTION('',(0.669589480006976,-0.669589480006974,0.321402950403348)) ;
#123724=DIRECTION('',(-0.669589480006976,0.669589480006974,0.321402950403348)) ;
#123725=DIRECTION('',(-0.707106781186549,0.707106781186546,0.)) ;
#123726=DIRECTION('center_axis',(0.707106781186555,0.70710678118654,3.31903965888224E-14)) ;
#123727=DIRECTION('ref_axis',(0.704497887013092,-0.704497887013103,-0.0858222254906087)) ;
#123728=DIRECTION('center_axis',(-0.707106781186546,-0.707106781186549,
0.)) ;
#123729=DIRECTION('ref_axis',(0.,0.,-1.)) ;
#123730=DIRECTION('',(0.,0.,-1.)) ;
#123731=DIRECTION('center_axis',(0.707106781186558,0.707106781186537,-5.75300207541695E-14)) ;
#123732=DIRECTION('ref_axis',(0.704497887013391,-0.704497887013405,0.0858222254856872)) ;
#123733=DIRECTION('',(0.707106781186549,-0.707106781186546,0.)) ;
#123734=DIRECTION('',(0.669589480006976,-0.669589480006974,0.321402950403348)) ;
#123735=DIRECTION('',(-0.669589480006976,0.669589480006974,0.321402950403348)) ;
#123736=DIRECTION('',(-0.707106781186549,0.707106781186546,0.)) ;
#123737=DIRECTION('center_axis',(0.707106781186548,0.707106781186547,-3.87221293536151E-15)) ;
#123738=DIRECTION('ref_axis',(0.704497887013335,-0.704497887013336,-0.0858222254867023)) ;
#123739=DIRECTION('center_axis',(-0.707106781186546,-0.707106781186549,
0.)) ;
#123740=DIRECTION('ref_axis',(0.,0.,-1.)) ;
#123741=DIRECTION('',(0.,0.,-1.)) ;
#123742=DIRECTION('center_axis',(0.707106781186543,0.707106781186552,1.7701544847441E-14)) ;
#123743=DIRECTION('ref_axis',(0.704497887012761,-0.704497887012754,0.0858222254962028)) ;
#123744=DIRECTION('',(0.707106781186549,-0.707106781186546,0.)) ;
#123745=DIRECTION('',(0.669589480006976,-0.669589480006974,0.321402950403348)) ;
#123746=DIRECTION('',(-0.669589480006976,0.669589480006974,0.321402950403348)) ;
#123747=DIRECTION('',(-0.707106781186549,0.707106781186546,0.)) ;
#123748=DIRECTION('center_axis',(0.707106781186551,0.707106781186544,1.82547181238502E-14)) ;
#123749=DIRECTION('ref_axis',(0.704497887013145,-0.70449788701315,-0.0858222254897919)) ;
#123750=DIRECTION('center_axis',(-0.707106781186546,-0.707106781186549,
0.)) ;
#123751=DIRECTION('ref_axis',(0.,0.,-1.)) ;
#123752=DIRECTION('',(0.,0.,-1.)) ;
#123753=DIRECTION('center_axis',(0.707106781186541,0.707106781186554,2.26801043356451E-14)) ;
#123754=DIRECTION('ref_axis',(0.704497887008924,-0.704497887008914,0.0858222255592156)) ;
#123755=DIRECTION('',(0.707106781186549,-0.707106781186546,0.)) ;
#123756=DIRECTION('',(0.669589480006976,-0.669589480006974,0.321402950403348)) ;
#123757=DIRECTION('',(-0.669589480006976,0.669589480006974,0.321402950403348)) ;
#123758=DIRECTION('',(-0.707106781186549,0.707106781186546,0.)) ;
#123759=DIRECTION('center_axis',(0.707106781186548,0.707106781186547,6.63807931776562E-15)) ;
#123760=DIRECTION('ref_axis',(0.704497887012742,-0.704497887012742,-0.0858222254964534)) ;
#123761=DIRECTION('center_axis',(-0.707106781186546,-0.707106781186549,
0.)) ;
#123762=DIRECTION('ref_axis',(0.,0.,-1.)) ;
#123763=DIRECTION('',(0.,0.,-1.)) ;
#123764=DIRECTION('center_axis',(0.707106781186546,0.707106781186549,-1.6595198294363E-15)) ;
#123765=DIRECTION('ref_axis',(0.704497887009798,-0.704497887009795,0.0858222255448097)) ;
#123766=DIRECTION('',(0.707106781186549,-0.707106781186546,0.)) ;
#123767=DIRECTION('',(0.669589480006976,-0.669589480006974,0.321402950403348)) ;
#123768=DIRECTION('',(-0.669589480006976,0.669589480006974,0.321402950403348)) ;
#123769=DIRECTION('',(-0.707106781186549,0.707106781186546,0.)) ;
#123770=DIRECTION('center_axis',(0.707106781186546,0.707106781186549,-9.40394570014366E-15)) ;
#123771=DIRECTION('ref_axis',(0.704497887009107,-0.704497887009105,-0.0858222255561507)) ;
#123772=DIRECTION('center_axis',(1.,0.,2.16840434497101E-16)) ;
#123773=DIRECTION('ref_axis',(2.16840434497101E-16,0.,-1.)) ;
#123774=DIRECTION('',(-2.16840434497101E-16,0.,1.)) ;
#123775=DIRECTION('',(0.,1.,0.)) ;
#123776=DIRECTION('',(2.16840434497101E-16,0.,-1.)) ;
#123777=DIRECTION('',(0.,-1.,0.)) ;
#123778=DIRECTION('center_axis',(2.16840434497101E-16,0.,-1.)) ;
#123779=DIRECTION('ref_axis',(-1.,0.,-2.16840434497101E-16)) ;
#123780=DIRECTION('',(-1.,0.,-2.16840434497101E-16)) ;
#123781=DIRECTION('',(0.,-1.,0.)) ;
#123782=DIRECTION('',(1.,0.,2.16840434497101E-16)) ;
#123783=DIRECTION('',(0.,1.,0.)) ;
#123784=DIRECTION('center_axis',(-1.,0.,0.)) ;
#123785=DIRECTION('ref_axis',(0.,0.,1.)) ;
#123786=DIRECTION('',(0.,0.,-1.)) ;
#123787=DIRECTION('',(0.,1.,0.)) ;
#123788=DIRECTION('',(0.,0.,1.)) ;
#123789=DIRECTION('',(0.,-1.,0.)) ;
#123790=DIRECTION('center_axis',(2.16840434497101E-16,0.,1.)) ;
#123791=DIRECTION('ref_axis',(1.,0.,-2.16840434497101E-16)) ;
#123792=DIRECTION('',(-1.,0.,2.16840434497101E-16)) ;
#123793=DIRECTION('',(0.,1.,0.)) ;
#123794=DIRECTION('',(1.,0.,-2.16840434497101E-16)) ;
#123795=DIRECTION('',(0.,-1.,0.)) ;
#123796=DIRECTION('center_axis',(1.,0.,2.16840434497101E-16)) ;
#123797=DIRECTION('ref_axis',(2.16840434497101E-16,0.,-1.)) ;
#123798=DIRECTION('',(-2.16840434497101E-16,0.,1.)) ;
#123799=DIRECTION('',(0.,1.,0.)) ;
#123800=DIRECTION('',(2.16840434497101E-16,0.,-1.)) ;
#123801=DIRECTION('',(0.,-1.,0.)) ;
#123802=DIRECTION('center_axis',(2.16840434497101E-16,0.,-1.)) ;
#123803=DIRECTION('ref_axis',(-1.,0.,-2.16840434497101E-16)) ;
#123804=DIRECTION('',(-1.,0.,-2.16840434497101E-16)) ;
#123805=DIRECTION('',(0.,-1.,0.)) ;
#123806=DIRECTION('',(1.,0.,2.16840434497101E-16)) ;
#123807=DIRECTION('',(0.,1.,0.)) ;
#123808=DIRECTION('center_axis',(-1.,0.,0.)) ;
#123809=DIRECTION('ref_axis',(0.,0.,1.)) ;
#123810=DIRECTION('',(0.,0.,-1.)) ;
#123811=DIRECTION('',(0.,1.,0.)) ;
#123812=DIRECTION('',(0.,0.,1.)) ;
#123813=DIRECTION('',(0.,-1.,0.)) ;
#123814=DIRECTION('center_axis',(2.16840434497101E-16,0.,1.)) ;
#123815=DIRECTION('ref_axis',(1.,0.,-2.16840434497101E-16)) ;
#123816=DIRECTION('',(-1.,0.,2.16840434497101E-16)) ;
#123817=DIRECTION('',(0.,1.,0.)) ;
#123818=DIRECTION('',(1.,0.,-2.16840434497101E-16)) ;
#123819=DIRECTION('',(0.,-1.,0.)) ;
#123820=DIRECTION('center_axis',(1.,0.,2.16840434497101E-16)) ;
#123821=DIRECTION('ref_axis',(2.16840434497101E-16,0.,-1.)) ;
#123822=DIRECTION('',(-2.16840434497101E-16,0.,1.)) ;
#123823=DIRECTION('',(0.,1.,0.)) ;
#123824=DIRECTION('',(2.16840434497101E-16,0.,-1.)) ;
#123825=DIRECTION('',(0.,-1.,0.)) ;
#123826=DIRECTION('center_axis',(2.16840434497101E-16,0.,-1.)) ;
#123827=DIRECTION('ref_axis',(-1.,0.,-2.16840434497101E-16)) ;
#123828=DIRECTION('',(-1.,0.,-2.16840434497101E-16)) ;
#123829=DIRECTION('',(0.,-1.,0.)) ;
#123830=DIRECTION('',(1.,0.,2.16840434497101E-16)) ;
#123831=DIRECTION('',(0.,1.,0.)) ;
#123832=DIRECTION('center_axis',(-1.,0.,0.)) ;
#123833=DIRECTION('ref_axis',(0.,0.,1.)) ;
#123834=DIRECTION('',(0.,0.,-1.)) ;
#123835=DIRECTION('',(0.,1.,0.)) ;
#123836=DIRECTION('',(0.,0.,1.)) ;
#123837=DIRECTION('',(0.,-1.,0.)) ;
#123838=DIRECTION('center_axis',(2.16840434497101E-16,0.,1.)) ;
#123839=DIRECTION('ref_axis',(1.,0.,-2.16840434497101E-16)) ;
#123840=DIRECTION('',(-1.,0.,2.16840434497101E-16)) ;
#123841=DIRECTION('',(0.,1.,0.)) ;
#123842=DIRECTION('',(1.,0.,-2.16840434497101E-16)) ;
#123843=DIRECTION('',(0.,-1.,0.)) ;
#123844=DIRECTION('center_axis',(1.,0.,2.16840434497101E-16)) ;
#123845=DIRECTION('ref_axis',(2.16840434497101E-16,0.,-1.)) ;
#123846=DIRECTION('',(-2.16840434497101E-16,0.,1.)) ;
#123847=DIRECTION('',(0.,1.,0.)) ;
#123848=DIRECTION('',(2.16840434497101E-16,0.,-1.)) ;
#123849=DIRECTION('',(0.,-1.,0.)) ;
#123850=DIRECTION('center_axis',(2.16840434497101E-16,0.,-1.)) ;
#123851=DIRECTION('ref_axis',(-1.,0.,-2.16840434497101E-16)) ;
#123852=DIRECTION('',(-1.,0.,-2.16840434497101E-16)) ;
#123853=DIRECTION('',(0.,-1.,0.)) ;
#123854=DIRECTION('',(1.,0.,2.16840434497101E-16)) ;
#123855=DIRECTION('',(0.,1.,0.)) ;
#123856=DIRECTION('center_axis',(-1.,0.,0.)) ;
#123857=DIRECTION('ref_axis',(0.,0.,1.)) ;
#123858=DIRECTION('',(0.,0.,-1.)) ;
#123859=DIRECTION('',(0.,1.,0.)) ;
#123860=DIRECTION('',(0.,0.,1.)) ;
#123861=DIRECTION('',(0.,-1.,0.)) ;
#123862=DIRECTION('center_axis',(2.16840434497101E-16,0.,1.)) ;
#123863=DIRECTION('ref_axis',(1.,0.,-2.16840434497101E-16)) ;
#123864=DIRECTION('',(-1.,0.,2.16840434497101E-16)) ;
#123865=DIRECTION('',(0.,1.,0.)) ;
#123866=DIRECTION('',(1.,0.,-2.16840434497101E-16)) ;
#123867=DIRECTION('',(0.,-1.,0.)) ;
#123868=DIRECTION('center_axis',(1.,0.,2.16840434497101E-16)) ;
#123869=DIRECTION('ref_axis',(2.16840434497101E-16,0.,-1.)) ;
#123870=DIRECTION('',(-2.16840434497101E-16,0.,1.)) ;
#123871=DIRECTION('',(0.,1.,0.)) ;
#123872=DIRECTION('',(2.16840434497101E-16,0.,-1.)) ;
#123873=DIRECTION('',(0.,-1.,0.)) ;
#123874=DIRECTION('center_axis',(2.16840434497101E-16,0.,-1.)) ;
#123875=DIRECTION('ref_axis',(-1.,0.,-2.16840434497101E-16)) ;
#123876=DIRECTION('',(-1.,0.,-2.16840434497101E-16)) ;
#123877=DIRECTION('',(0.,-1.,0.)) ;
#123878=DIRECTION('',(1.,0.,2.16840434497101E-16)) ;
#123879=DIRECTION('',(0.,1.,0.)) ;
#123880=DIRECTION('center_axis',(-1.,0.,0.)) ;
#123881=DIRECTION('ref_axis',(0.,0.,1.)) ;
#123882=DIRECTION('',(0.,0.,-1.)) ;
#123883=DIRECTION('',(0.,1.,0.)) ;
#123884=DIRECTION('',(0.,0.,1.)) ;
#123885=DIRECTION('',(0.,-1.,0.)) ;
#123886=DIRECTION('center_axis',(2.16840434497101E-16,0.,1.)) ;
#123887=DIRECTION('ref_axis',(1.,0.,-2.16840434497101E-16)) ;
#123888=DIRECTION('',(-1.,0.,2.16840434497101E-16)) ;
#123889=DIRECTION('',(0.,1.,0.)) ;
#123890=DIRECTION('',(1.,0.,-2.16840434497101E-16)) ;
#123891=DIRECTION('',(0.,-1.,0.)) ;
#123892=DIRECTION('center_axis',(1.,0.,2.16840434497101E-16)) ;
#123893=DIRECTION('ref_axis',(2.16840434497101E-16,0.,-1.)) ;
#123894=DIRECTION('',(-2.16840434497101E-16,0.,1.)) ;
#123895=DIRECTION('',(0.,1.,0.)) ;
#123896=DIRECTION('',(2.16840434497101E-16,0.,-1.)) ;
#123897=DIRECTION('',(0.,-1.,0.)) ;
#123898=DIRECTION('center_axis',(2.16840434497101E-16,0.,-1.)) ;
#123899=DIRECTION('ref_axis',(-1.,0.,-2.16840434497101E-16)) ;
#123900=DIRECTION('',(-1.,0.,-2.16840434497101E-16)) ;
#123901=DIRECTION('',(0.,-1.,0.)) ;
#123902=DIRECTION('',(1.,0.,2.16840434497101E-16)) ;
#123903=DIRECTION('',(0.,1.,0.)) ;
#123904=DIRECTION('center_axis',(-1.,0.,0.)) ;
#123905=DIRECTION('ref_axis',(0.,0.,1.)) ;
#123906=DIRECTION('',(0.,0.,-1.)) ;
#123907=DIRECTION('',(0.,1.,0.)) ;
#123908=DIRECTION('',(0.,0.,1.)) ;
#123909=DIRECTION('',(0.,-1.,0.)) ;
#123910=DIRECTION('center_axis',(2.16840434497101E-16,0.,1.)) ;
#123911=DIRECTION('ref_axis',(1.,0.,-2.16840434497101E-16)) ;
#123912=DIRECTION('',(-1.,0.,2.16840434497101E-16)) ;
#123913=DIRECTION('',(0.,1.,0.)) ;
#123914=DIRECTION('',(1.,0.,-2.16840434497101E-16)) ;
#123915=DIRECTION('',(0.,-1.,0.)) ;
#123916=DIRECTION('center_axis',(1.,0.,2.16840434497101E-16)) ;
#123917=DIRECTION('ref_axis',(2.16840434497101E-16,0.,-1.)) ;
#123918=DIRECTION('',(-2.16840434497101E-16,0.,1.)) ;
#123919=DIRECTION('',(0.,1.,0.)) ;
#123920=DIRECTION('',(2.16840434497101E-16,0.,-1.)) ;
#123921=DIRECTION('',(0.,-1.,0.)) ;
#123922=DIRECTION('center_axis',(2.16840434497101E-16,0.,-1.)) ;
#123923=DIRECTION('ref_axis',(-1.,0.,-2.16840434497101E-16)) ;
#123924=DIRECTION('',(-1.,0.,-2.16840434497101E-16)) ;
#123925=DIRECTION('',(0.,-1.,0.)) ;
#123926=DIRECTION('',(1.,0.,2.16840434497101E-16)) ;
#123927=DIRECTION('',(0.,1.,0.)) ;
#123928=DIRECTION('center_axis',(-1.,0.,0.)) ;
#123929=DIRECTION('ref_axis',(0.,0.,1.)) ;
#123930=DIRECTION('',(0.,0.,-1.)) ;
#123931=DIRECTION('',(0.,1.,0.)) ;
#123932=DIRECTION('',(0.,0.,1.)) ;
#123933=DIRECTION('',(0.,-1.,0.)) ;
#123934=DIRECTION('center_axis',(2.16840434497101E-16,0.,1.)) ;
#123935=DIRECTION('ref_axis',(1.,0.,-2.16840434497101E-16)) ;
#123936=DIRECTION('',(-1.,0.,2.16840434497101E-16)) ;
#123937=DIRECTION('',(0.,1.,0.)) ;
#123938=DIRECTION('',(1.,0.,-2.16840434497101E-16)) ;
#123939=DIRECTION('',(0.,-1.,0.)) ;
#123940=DIRECTION('center_axis',(1.,0.,2.16840434497101E-16)) ;
#123941=DIRECTION('ref_axis',(2.16840434497101E-16,0.,-1.)) ;
#123942=DIRECTION('',(-2.16840434497101E-16,0.,1.)) ;
#123943=DIRECTION('',(0.,1.,0.)) ;
#123944=DIRECTION('',(2.16840434497101E-16,0.,-1.)) ;
#123945=DIRECTION('',(0.,-1.,0.)) ;
#123946=DIRECTION('center_axis',(2.16840434497101E-16,0.,-1.)) ;
#123947=DIRECTION('ref_axis',(-1.,0.,-2.16840434497101E-16)) ;
#123948=DIRECTION('',(-1.,0.,-2.16840434497101E-16)) ;
#123949=DIRECTION('',(0.,-1.,0.)) ;
#123950=DIRECTION('',(1.,0.,2.16840434497101E-16)) ;
#123951=DIRECTION('',(0.,1.,0.)) ;
#123952=DIRECTION('center_axis',(-1.,0.,0.)) ;
#123953=DIRECTION('ref_axis',(0.,0.,1.)) ;
#123954=DIRECTION('',(0.,0.,-1.)) ;
#123955=DIRECTION('',(0.,1.,0.)) ;
#123956=DIRECTION('',(0.,0.,1.)) ;
#123957=DIRECTION('',(0.,-1.,0.)) ;
#123958=DIRECTION('center_axis',(2.16840434497101E-16,0.,1.)) ;
#123959=DIRECTION('ref_axis',(1.,0.,-2.16840434497101E-16)) ;
#123960=DIRECTION('',(-1.,0.,2.16840434497101E-16)) ;
#123961=DIRECTION('',(0.,1.,0.)) ;
#123962=DIRECTION('',(1.,0.,-2.16840434497101E-16)) ;
#123963=DIRECTION('',(0.,-1.,0.)) ;
#123964=DIRECTION('center_axis',(1.,0.,2.16840434497101E-16)) ;
#123965=DIRECTION('ref_axis',(2.16840434497101E-16,0.,-1.)) ;
#123966=DIRECTION('',(2.16840434497101E-16,0.,-1.)) ;
#123967=DIRECTION('',(0.,-1.,0.)) ;
#123968=DIRECTION('',(-2.16840434497101E-16,0.,1.)) ;
#123969=DIRECTION('',(0.,1.,0.)) ;
#123970=DIRECTION('center_axis',(2.16840434497101E-16,0.,-1.)) ;
#123971=DIRECTION('ref_axis',(-1.,0.,-2.16840434497101E-16)) ;
#123972=DIRECTION('',(-1.,0.,-2.16840434497101E-16)) ;
#123973=DIRECTION('',(0.,-1.,0.)) ;
#123974=DIRECTION('',(1.,0.,2.16840434497101E-16)) ;
#123975=DIRECTION('',(0.,1.,0.)) ;
#123976=DIRECTION('center_axis',(-1.,0.,0.)) ;
#123977=DIRECTION('ref_axis',(0.,0.,1.)) ;
#123978=DIRECTION('',(0.,1.,0.)) ;
#123979=DIRECTION('',(0.,0.,1.)) ;
#123980=DIRECTION('',(0.,-1.,0.)) ;
#123981=DIRECTION('',(0.,0.,-1.)) ;
#123982=DIRECTION('center_axis',(2.16840434497101E-16,0.,1.)) ;
#123983=DIRECTION('ref_axis',(1.,0.,-2.16840434497101E-16)) ;
#123984=DIRECTION('',(0.,1.,0.)) ;
#123985=DIRECTION('',(1.,0.,-2.16840434497101E-16)) ;
#123986=DIRECTION('',(0.,-1.,0.)) ;
#123987=DIRECTION('',(-1.,0.,2.16840434497101E-16)) ;
#123988=DIRECTION('center_axis',(0.,-1.,0.)) ;
#123989=DIRECTION('ref_axis',(0.,0.,-1.)) ;
#123990=DIRECTION('',(0.,0.,-1.)) ;
#123991=DIRECTION('',(1.,0.,2.16840434497101E-16)) ;
#123992=DIRECTION('',(-2.16840434497101E-16,0.,1.)) ;
#123993=DIRECTION('',(-1.,0.,2.16840434497101E-16)) ;
#123994=DIRECTION('',(1.,0.,0.)) ;
#123995=DIRECTION('center_axis',(0.,1.,0.)) ;
#123996=DIRECTION('ref_axis',(0.,0.,-1.)) ;
#123997=DIRECTION('',(0.,0.,-1.)) ;
#123998=DIRECTION('center_axis',(0.,1.,0.)) ;
#123999=DIRECTION('ref_axis',(0.,0.,-1.)) ;
#124000=DIRECTION('',(-1.,0.,0.)) ;
#124001=DIRECTION('center_axis',(0.,1.,0.)) ;
#124002=DIRECTION('ref_axis',(0.,0.,-1.)) ;
#124003=DIRECTION('',(0.,0.,1.)) ;
#124004=DIRECTION('center_axis',(0.,1.,0.)) ;
#124005=DIRECTION('ref_axis',(0.,0.,-1.)) ;
#124006=DIRECTION('center_axis',(1.,0.,0.)) ;
#124007=DIRECTION('ref_axis',(0.,0.,-1.)) ;
#124008=DIRECTION('',(0.,-1.,0.)) ;
#124009=DIRECTION('',(0.,0.,-1.)) ;
#124010=DIRECTION('',(0.,1.,0.)) ;
#124011=DIRECTION('center_axis',(0.,0.,-1.)) ;
#124012=DIRECTION('ref_axis',(-1.,0.,0.)) ;
#124013=DIRECTION('',(0.,-1.,0.)) ;
#124014=DIRECTION('',(-1.,0.,0.)) ;
#124015=DIRECTION('',(0.,1.,0.)) ;
#124016=DIRECTION('center_axis',(-1.,0.,0.)) ;
#124017=DIRECTION('ref_axis',(0.,0.,1.)) ;
#124018=DIRECTION('',(0.,0.,1.)) ;
#124019=DIRECTION('',(0.,1.,0.)) ;
#124020=DIRECTION('',(0.,-1.,0.)) ;
#124021=DIRECTION('center_axis',(0.,0.,1.)) ;
#124022=DIRECTION('ref_axis',(1.,0.,0.)) ;
#124023=DIRECTION('',(0.,-1.,0.)) ;
#124024=DIRECTION('',(1.,0.,0.)) ;
#124025=DIRECTION('',(0.,1.,0.)) ;
#124026=DIRECTION('center_axis',(0.,-1.,0.)) ;
#124027=DIRECTION('ref_axis',(0.,0.,-1.)) ;
#124028=DIRECTION('',(0.,0.,-1.)) ;
#124029=DIRECTION('',(1.,0.,2.16840434497101E-16)) ;
#124030=DIRECTION('',(-2.16840434497101E-16,0.,1.)) ;
#124031=DIRECTION('',(-1.,0.,2.16840434497101E-16)) ;
#124032=DIRECTION('',(1.,0.,0.)) ;
#124033=DIRECTION('center_axis',(0.,1.,0.)) ;
#124034=DIRECTION('ref_axis',(0.,0.,-1.)) ;
#124035=DIRECTION('',(0.,0.,-1.)) ;
#124036=DIRECTION('center_axis',(0.,1.,0.)) ;
#124037=DIRECTION('ref_axis',(0.,0.,-1.)) ;
#124038=DIRECTION('',(-1.,0.,0.)) ;
#124039=DIRECTION('center_axis',(0.,1.,0.)) ;
#124040=DIRECTION('ref_axis',(0.,0.,-1.)) ;
#124041=DIRECTION('',(0.,0.,1.)) ;
#124042=DIRECTION('center_axis',(0.,1.,0.)) ;
#124043=DIRECTION('ref_axis',(0.,0.,-1.)) ;
#124044=DIRECTION('center_axis',(1.,0.,0.)) ;
#124045=DIRECTION('ref_axis',(0.,0.,-1.)) ;
#124046=DIRECTION('',(0.,-1.,0.)) ;
#124047=DIRECTION('',(0.,0.,-1.)) ;
#124048=DIRECTION('',(0.,1.,0.)) ;
#124049=DIRECTION('center_axis',(0.,0.,-1.)) ;
#124050=DIRECTION('ref_axis',(-1.,0.,0.)) ;
#124051=DIRECTION('',(0.,-1.,0.)) ;
#124052=DIRECTION('',(-1.,0.,0.)) ;
#124053=DIRECTION('',(0.,1.,0.)) ;
#124054=DIRECTION('center_axis',(-1.,0.,0.)) ;
#124055=DIRECTION('ref_axis',(0.,0.,1.)) ;
#124056=DIRECTION('',(0.,0.,1.)) ;
#124057=DIRECTION('',(0.,1.,0.)) ;
#124058=DIRECTION('',(0.,-1.,0.)) ;
#124059=DIRECTION('center_axis',(0.,0.,1.)) ;
#124060=DIRECTION('ref_axis',(1.,0.,0.)) ;
#124061=DIRECTION('',(0.,-1.,0.)) ;
#124062=DIRECTION('',(1.,0.,0.)) ;
#124063=DIRECTION('',(0.,1.,0.)) ;
#124064=DIRECTION('center_axis',(0.,-1.,0.)) ;
#124065=DIRECTION('ref_axis',(0.,0.,-1.)) ;
#124066=DIRECTION('',(0.,0.,-1.)) ;
#124067=DIRECTION('',(1.,0.,2.16840434497101E-16)) ;
#124068=DIRECTION('',(-2.16840434497101E-16,0.,1.)) ;
#124069=DIRECTION('',(-1.,0.,2.16840434497101E-16)) ;
#124070=DIRECTION('',(1.,0.,0.)) ;
#124071=DIRECTION('center_axis',(0.,1.,0.)) ;
#124072=DIRECTION('ref_axis',(0.,0.,-1.)) ;
#124073=DIRECTION('',(0.,0.,-1.)) ;
#124074=DIRECTION('center_axis',(0.,1.,0.)) ;
#124075=DIRECTION('ref_axis',(0.,0.,-1.)) ;
#124076=DIRECTION('',(-1.,0.,0.)) ;
#124077=DIRECTION('center_axis',(0.,1.,0.)) ;
#124078=DIRECTION('ref_axis',(0.,0.,-1.)) ;
#124079=DIRECTION('',(0.,0.,1.)) ;
#124080=DIRECTION('center_axis',(0.,1.,0.)) ;
#124081=DIRECTION('ref_axis',(0.,0.,-1.)) ;
#124082=DIRECTION('center_axis',(1.,0.,0.)) ;
#124083=DIRECTION('ref_axis',(0.,0.,-1.)) ;
#124084=DIRECTION('',(0.,-1.,0.)) ;
#124085=DIRECTION('',(0.,0.,-1.)) ;
#124086=DIRECTION('',(0.,1.,0.)) ;
#124087=DIRECTION('center_axis',(0.,0.,-1.)) ;
#124088=DIRECTION('ref_axis',(-1.,0.,0.)) ;
#124089=DIRECTION('',(0.,-1.,0.)) ;
#124090=DIRECTION('',(-1.,0.,0.)) ;
#124091=DIRECTION('',(0.,1.,0.)) ;
#124092=DIRECTION('center_axis',(-1.,0.,0.)) ;
#124093=DIRECTION('ref_axis',(0.,0.,1.)) ;
#124094=DIRECTION('',(0.,0.,1.)) ;
#124095=DIRECTION('',(0.,1.,0.)) ;
#124096=DIRECTION('',(0.,-1.,0.)) ;
#124097=DIRECTION('center_axis',(0.,0.,1.)) ;
#124098=DIRECTION('ref_axis',(1.,0.,0.)) ;
#124099=DIRECTION('',(0.,-1.,0.)) ;
#124100=DIRECTION('',(1.,0.,0.)) ;
#124101=DIRECTION('',(0.,1.,0.)) ;
#124102=DIRECTION('center_axis',(0.,-1.,0.)) ;
#124103=DIRECTION('ref_axis',(0.,0.,-1.)) ;
#124104=DIRECTION('',(0.,0.,-1.)) ;
#124105=DIRECTION('',(1.,0.,2.16840434497101E-16)) ;
#124106=DIRECTION('',(-2.16840434497101E-16,0.,1.)) ;
#124107=DIRECTION('',(-1.,0.,2.16840434497101E-16)) ;
#124108=DIRECTION('',(1.,0.,0.)) ;
#124109=DIRECTION('center_axis',(0.,1.,0.)) ;
#124110=DIRECTION('ref_axis',(0.,0.,-1.)) ;
#124111=DIRECTION('',(0.,0.,-1.)) ;
#124112=DIRECTION('center_axis',(0.,1.,0.)) ;
#124113=DIRECTION('ref_axis',(0.,0.,-1.)) ;
#124114=DIRECTION('',(-1.,0.,0.)) ;
#124115=DIRECTION('center_axis',(0.,1.,0.)) ;
#124116=DIRECTION('ref_axis',(0.,0.,-1.)) ;
#124117=DIRECTION('',(0.,0.,1.)) ;
#124118=DIRECTION('center_axis',(0.,1.,0.)) ;
#124119=DIRECTION('ref_axis',(0.,0.,-1.)) ;
#124120=DIRECTION('center_axis',(1.,0.,0.)) ;
#124121=DIRECTION('ref_axis',(0.,0.,-1.)) ;
#124122=DIRECTION('',(0.,-1.,0.)) ;
#124123=DIRECTION('',(0.,0.,-1.)) ;
#124124=DIRECTION('',(0.,1.,0.)) ;
#124125=DIRECTION('center_axis',(0.,0.,-1.)) ;
#124126=DIRECTION('ref_axis',(-1.,0.,0.)) ;
#124127=DIRECTION('',(0.,-1.,0.)) ;
#124128=DIRECTION('',(-1.,0.,0.)) ;
#124129=DIRECTION('',(0.,1.,0.)) ;
#124130=DIRECTION('center_axis',(-1.,0.,0.)) ;
#124131=DIRECTION('ref_axis',(0.,0.,1.)) ;
#124132=DIRECTION('',(0.,0.,1.)) ;
#124133=DIRECTION('',(0.,1.,0.)) ;
#124134=DIRECTION('',(0.,-1.,0.)) ;
#124135=DIRECTION('center_axis',(0.,0.,1.)) ;
#124136=DIRECTION('ref_axis',(1.,0.,0.)) ;
#124137=DIRECTION('',(0.,-1.,0.)) ;
#124138=DIRECTION('',(1.,0.,0.)) ;
#124139=DIRECTION('',(0.,1.,0.)) ;
#124140=DIRECTION('center_axis',(0.,-1.,0.)) ;
#124141=DIRECTION('ref_axis',(0.,0.,-1.)) ;
#124142=DIRECTION('',(0.,0.,-1.)) ;
#124143=DIRECTION('',(1.,0.,2.16840434497101E-16)) ;
#124144=DIRECTION('',(-2.16840434497101E-16,0.,1.)) ;
#124145=DIRECTION('',(-1.,0.,2.16840434497101E-16)) ;
#124146=DIRECTION('',(1.,0.,0.)) ;
#124147=DIRECTION('center_axis',(0.,1.,0.)) ;
#124148=DIRECTION('ref_axis',(0.,0.,-1.)) ;
#124149=DIRECTION('',(0.,0.,-1.)) ;
#124150=DIRECTION('center_axis',(0.,1.,0.)) ;
#124151=DIRECTION('ref_axis',(0.,0.,-1.)) ;
#124152=DIRECTION('',(-1.,0.,0.)) ;
#124153=DIRECTION('center_axis',(0.,1.,0.)) ;
#124154=DIRECTION('ref_axis',(0.,0.,-1.)) ;
#124155=DIRECTION('',(0.,0.,1.)) ;
#124156=DIRECTION('center_axis',(0.,1.,0.)) ;
#124157=DIRECTION('ref_axis',(0.,0.,-1.)) ;
#124158=DIRECTION('center_axis',(1.,0.,0.)) ;
#124159=DIRECTION('ref_axis',(0.,0.,-1.)) ;
#124160=DIRECTION('',(0.,-1.,0.)) ;
#124161=DIRECTION('',(0.,0.,-1.)) ;
#124162=DIRECTION('',(0.,1.,0.)) ;
#124163=DIRECTION('center_axis',(0.,0.,-1.)) ;
#124164=DIRECTION('ref_axis',(-1.,0.,0.)) ;
#124165=DIRECTION('',(0.,-1.,0.)) ;
#124166=DIRECTION('',(-1.,0.,0.)) ;
#124167=DIRECTION('',(0.,1.,0.)) ;
#124168=DIRECTION('center_axis',(-1.,0.,0.)) ;
#124169=DIRECTION('ref_axis',(0.,0.,1.)) ;
#124170=DIRECTION('',(0.,0.,1.)) ;
#124171=DIRECTION('',(0.,1.,0.)) ;
#124172=DIRECTION('',(0.,-1.,0.)) ;
#124173=DIRECTION('center_axis',(0.,0.,1.)) ;
#124174=DIRECTION('ref_axis',(1.,0.,0.)) ;
#124175=DIRECTION('',(0.,-1.,0.)) ;
#124176=DIRECTION('',(1.,0.,0.)) ;
#124177=DIRECTION('',(0.,1.,0.)) ;
#124178=DIRECTION('center_axis',(0.,-1.,0.)) ;
#124179=DIRECTION('ref_axis',(0.,0.,-1.)) ;
#124180=DIRECTION('',(0.,0.,-1.)) ;
#124181=DIRECTION('',(1.,0.,2.16840434497101E-16)) ;
#124182=DIRECTION('',(-2.16840434497101E-16,0.,1.)) ;
#124183=DIRECTION('',(-1.,0.,2.16840434497101E-16)) ;
#124184=DIRECTION('',(1.,0.,0.)) ;
#124185=DIRECTION('center_axis',(0.,1.,0.)) ;
#124186=DIRECTION('ref_axis',(0.,0.,-1.)) ;
#124187=DIRECTION('',(0.,0.,-1.)) ;
#124188=DIRECTION('center_axis',(0.,1.,0.)) ;
#124189=DIRECTION('ref_axis',(0.,0.,-1.)) ;
#124190=DIRECTION('',(-1.,0.,0.)) ;
#124191=DIRECTION('center_axis',(0.,1.,0.)) ;
#124192=DIRECTION('ref_axis',(0.,0.,-1.)) ;
#124193=DIRECTION('',(0.,0.,1.)) ;
#124194=DIRECTION('center_axis',(0.,1.,0.)) ;
#124195=DIRECTION('ref_axis',(0.,0.,-1.)) ;
#124196=DIRECTION('center_axis',(1.,0.,0.)) ;
#124197=DIRECTION('ref_axis',(0.,0.,-1.)) ;
#124198=DIRECTION('',(0.,-1.,0.)) ;
#124199=DIRECTION('',(0.,0.,-1.)) ;
#124200=DIRECTION('',(0.,1.,0.)) ;
#124201=DIRECTION('center_axis',(0.,0.,-1.)) ;
#124202=DIRECTION('ref_axis',(-1.,0.,0.)) ;
#124203=DIRECTION('',(0.,-1.,0.)) ;
#124204=DIRECTION('',(-1.,0.,0.)) ;
#124205=DIRECTION('',(0.,1.,0.)) ;
#124206=DIRECTION('center_axis',(-1.,0.,0.)) ;
#124207=DIRECTION('ref_axis',(0.,0.,1.)) ;
#124208=DIRECTION('',(0.,0.,1.)) ;
#124209=DIRECTION('',(0.,1.,0.)) ;
#124210=DIRECTION('',(0.,-1.,0.)) ;
#124211=DIRECTION('center_axis',(0.,0.,1.)) ;
#124212=DIRECTION('ref_axis',(1.,0.,0.)) ;
#124213=DIRECTION('',(0.,-1.,0.)) ;
#124214=DIRECTION('',(1.,0.,0.)) ;
#124215=DIRECTION('',(0.,1.,0.)) ;
#124216=DIRECTION('center_axis',(0.,-1.,0.)) ;
#124217=DIRECTION('ref_axis',(0.,0.,-1.)) ;
#124218=DIRECTION('',(0.,0.,-1.)) ;
#124219=DIRECTION('',(1.,0.,2.16840434497101E-16)) ;
#124220=DIRECTION('',(-2.16840434497101E-16,0.,1.)) ;
#124221=DIRECTION('',(-1.,0.,2.16840434497101E-16)) ;
#124222=DIRECTION('',(1.,0.,0.)) ;
#124223=DIRECTION('center_axis',(0.,1.,0.)) ;
#124224=DIRECTION('ref_axis',(0.,0.,-1.)) ;
#124225=DIRECTION('',(0.,0.,-1.)) ;
#124226=DIRECTION('center_axis',(0.,1.,0.)) ;
#124227=DIRECTION('ref_axis',(0.,0.,-1.)) ;
#124228=DIRECTION('',(-1.,0.,0.)) ;
#124229=DIRECTION('center_axis',(0.,1.,0.)) ;
#124230=DIRECTION('ref_axis',(0.,0.,-1.)) ;
#124231=DIRECTION('',(0.,0.,1.)) ;
#124232=DIRECTION('center_axis',(0.,1.,0.)) ;
#124233=DIRECTION('ref_axis',(0.,0.,-1.)) ;
#124234=DIRECTION('center_axis',(1.,0.,0.)) ;
#124235=DIRECTION('ref_axis',(0.,0.,-1.)) ;
#124236=DIRECTION('',(0.,-1.,0.)) ;
#124237=DIRECTION('',(0.,0.,-1.)) ;
#124238=DIRECTION('',(0.,1.,0.)) ;
#124239=DIRECTION('center_axis',(0.,0.,-1.)) ;
#124240=DIRECTION('ref_axis',(-1.,0.,0.)) ;
#124241=DIRECTION('',(0.,-1.,0.)) ;
#124242=DIRECTION('',(-1.,0.,0.)) ;
#124243=DIRECTION('',(0.,1.,0.)) ;
#124244=DIRECTION('center_axis',(-1.,0.,0.)) ;
#124245=DIRECTION('ref_axis',(0.,0.,1.)) ;
#124246=DIRECTION('',(0.,0.,1.)) ;
#124247=DIRECTION('',(0.,1.,0.)) ;
#124248=DIRECTION('',(0.,-1.,0.)) ;
#124249=DIRECTION('center_axis',(0.,0.,1.)) ;
#124250=DIRECTION('ref_axis',(1.,0.,0.)) ;
#124251=DIRECTION('',(0.,-1.,0.)) ;
#124252=DIRECTION('',(1.,0.,0.)) ;
#124253=DIRECTION('',(0.,1.,0.)) ;
#124254=DIRECTION('center_axis',(0.,-1.,0.)) ;
#124255=DIRECTION('ref_axis',(0.,0.,-1.)) ;
#124256=DIRECTION('',(0.,0.,-1.)) ;
#124257=DIRECTION('',(1.,0.,2.16840434497101E-16)) ;
#124258=DIRECTION('',(-2.16840434497101E-16,0.,1.)) ;
#124259=DIRECTION('',(-1.,0.,2.16840434497101E-16)) ;
#124260=DIRECTION('',(1.,0.,0.)) ;
#124261=DIRECTION('center_axis',(0.,1.,0.)) ;
#124262=DIRECTION('ref_axis',(0.,0.,-1.)) ;
#124263=DIRECTION('',(0.,0.,-1.)) ;
#124264=DIRECTION('center_axis',(0.,1.,0.)) ;
#124265=DIRECTION('ref_axis',(0.,0.,-1.)) ;
#124266=DIRECTION('',(-1.,0.,0.)) ;
#124267=DIRECTION('center_axis',(0.,1.,0.)) ;
#124268=DIRECTION('ref_axis',(0.,0.,-1.)) ;
#124269=DIRECTION('',(0.,0.,1.)) ;
#124270=DIRECTION('center_axis',(0.,1.,0.)) ;
#124271=DIRECTION('ref_axis',(0.,0.,-1.)) ;
#124272=DIRECTION('center_axis',(1.,0.,0.)) ;
#124273=DIRECTION('ref_axis',(0.,0.,-1.)) ;
#124274=DIRECTION('',(0.,-1.,0.)) ;
#124275=DIRECTION('',(0.,0.,-1.)) ;
#124276=DIRECTION('',(0.,1.,0.)) ;
#124277=DIRECTION('center_axis',(0.,0.,-1.)) ;
#124278=DIRECTION('ref_axis',(-1.,0.,0.)) ;
#124279=DIRECTION('',(0.,-1.,0.)) ;
#124280=DIRECTION('',(-1.,0.,0.)) ;
#124281=DIRECTION('',(0.,1.,0.)) ;
#124282=DIRECTION('center_axis',(-1.,0.,0.)) ;
#124283=DIRECTION('ref_axis',(0.,0.,1.)) ;
#124284=DIRECTION('',(0.,0.,1.)) ;
#124285=DIRECTION('',(0.,1.,0.)) ;
#124286=DIRECTION('',(0.,-1.,0.)) ;
#124287=DIRECTION('center_axis',(0.,0.,1.)) ;
#124288=DIRECTION('ref_axis',(1.,0.,0.)) ;
#124289=DIRECTION('',(0.,-1.,0.)) ;
#124290=DIRECTION('',(1.,0.,0.)) ;
#124291=DIRECTION('',(0.,1.,0.)) ;
#124292=DIRECTION('center_axis',(0.,-1.,0.)) ;
#124293=DIRECTION('ref_axis',(0.,0.,-1.)) ;
#124294=DIRECTION('',(0.,0.,-1.)) ;
#124295=DIRECTION('',(1.,0.,2.16840434497101E-16)) ;
#124296=DIRECTION('',(-2.16840434497101E-16,0.,1.)) ;
#124297=DIRECTION('',(-1.,0.,2.16840434497101E-16)) ;
#124298=DIRECTION('',(1.,0.,0.)) ;
#124299=DIRECTION('center_axis',(0.,1.,0.)) ;
#124300=DIRECTION('ref_axis',(0.,0.,-1.)) ;
#124301=DIRECTION('',(0.,0.,-1.)) ;
#124302=DIRECTION('center_axis',(0.,1.,0.)) ;
#124303=DIRECTION('ref_axis',(0.,0.,-1.)) ;
#124304=DIRECTION('',(-1.,0.,0.)) ;
#124305=DIRECTION('center_axis',(0.,1.,0.)) ;
#124306=DIRECTION('ref_axis',(0.,0.,-1.)) ;
#124307=DIRECTION('',(0.,0.,1.)) ;
#124308=DIRECTION('center_axis',(0.,1.,0.)) ;
#124309=DIRECTION('ref_axis',(0.,0.,-1.)) ;
#124310=DIRECTION('center_axis',(1.,0.,0.)) ;
#124311=DIRECTION('ref_axis',(0.,0.,-1.)) ;
#124312=DIRECTION('',(0.,-1.,0.)) ;
#124313=DIRECTION('',(0.,0.,-1.)) ;
#124314=DIRECTION('',(0.,1.,0.)) ;
#124315=DIRECTION('center_axis',(0.,0.,-1.)) ;
#124316=DIRECTION('ref_axis',(-1.,0.,0.)) ;
#124317=DIRECTION('',(0.,-1.,0.)) ;
#124318=DIRECTION('',(-1.,0.,0.)) ;
#124319=DIRECTION('',(0.,1.,0.)) ;
#124320=DIRECTION('center_axis',(-1.,0.,0.)) ;
#124321=DIRECTION('ref_axis',(0.,0.,1.)) ;
#124322=DIRECTION('',(0.,0.,1.)) ;
#124323=DIRECTION('',(0.,1.,0.)) ;
#124324=DIRECTION('',(0.,-1.,0.)) ;
#124325=DIRECTION('center_axis',(0.,0.,1.)) ;
#124326=DIRECTION('ref_axis',(1.,0.,0.)) ;
#124327=DIRECTION('',(0.,-1.,0.)) ;
#124328=DIRECTION('',(1.,0.,0.)) ;
#124329=DIRECTION('',(0.,1.,0.)) ;
#124330=DIRECTION('center_axis',(0.,-1.,0.)) ;
#124331=DIRECTION('ref_axis',(0.,0.,-1.)) ;
#124332=DIRECTION('',(-1.,0.,0.)) ;
#124333=DIRECTION('',(0.,0.,-1.)) ;
#124334=DIRECTION('',(1.,0.,0.)) ;
#124335=DIRECTION('',(0.,0.,1.)) ;
#124336=DIRECTION('center_axis',(0.,-1.,0.)) ;
#124337=DIRECTION('ref_axis',(0.,0.,-1.)) ;
#124338=DIRECTION('',(-1.,0.,0.)) ;
#124339=DIRECTION('',(0.,0.,-1.)) ;
#124340=DIRECTION('',(1.,0.,0.)) ;
#124341=DIRECTION('',(0.,0.,1.)) ;
#124342=DIRECTION('center_axis',(0.,-1.,0.)) ;
#124343=DIRECTION('ref_axis',(0.,0.,-1.)) ;
#124344=DIRECTION('',(-1.,0.,0.)) ;
#124345=DIRECTION('',(0.,0.,-1.)) ;
#124346=DIRECTION('',(1.,0.,0.)) ;
#124347=DIRECTION('',(0.,0.,1.)) ;
#124348=DIRECTION('center_axis',(0.,-1.,0.)) ;
#124349=DIRECTION('ref_axis',(0.,0.,-1.)) ;
#124350=DIRECTION('',(-1.,0.,0.)) ;
#124351=DIRECTION('',(0.,0.,-1.)) ;
#124352=DIRECTION('',(1.,0.,0.)) ;
#124353=DIRECTION('',(0.,0.,1.)) ;
#124354=DIRECTION('center_axis',(0.,-1.,0.)) ;
#124355=DIRECTION('ref_axis',(0.,0.,-1.)) ;
#124356=DIRECTION('',(-1.,0.,0.)) ;
#124357=DIRECTION('',(0.,0.,-1.)) ;
#124358=DIRECTION('',(1.,0.,0.)) ;
#124359=DIRECTION('',(0.,0.,1.)) ;
#124360=DIRECTION('center_axis',(0.,-1.,0.)) ;
#124361=DIRECTION('ref_axis',(0.,0.,-1.)) ;
#124362=DIRECTION('',(-1.,0.,0.)) ;
#124363=DIRECTION('',(0.,0.,-1.)) ;
#124364=DIRECTION('',(1.,0.,0.)) ;
#124365=DIRECTION('',(0.,0.,1.)) ;
#124366=DIRECTION('center_axis',(0.,-1.,0.)) ;
#124367=DIRECTION('ref_axis',(0.,0.,-1.)) ;
#124368=DIRECTION('',(-1.,0.,0.)) ;
#124369=DIRECTION('',(0.,0.,-1.)) ;
#124370=DIRECTION('',(1.,0.,0.)) ;
#124371=DIRECTION('',(0.,0.,1.)) ;
#124372=DIRECTION('center_axis',(0.,-1.,0.)) ;
#124373=DIRECTION('ref_axis',(0.,0.,-1.)) ;
#124374=DIRECTION('',(-1.,0.,0.)) ;
#124375=DIRECTION('',(0.,0.,-1.)) ;
#124376=DIRECTION('',(1.,0.,0.)) ;
#124377=DIRECTION('',(0.,0.,1.)) ;
#124378=DIRECTION('center_axis',(0.,-1.,0.)) ;
#124379=DIRECTION('ref_axis',(0.,0.,-1.)) ;
#124380=DIRECTION('',(-1.,0.,0.)) ;
#124381=DIRECTION('',(0.,0.,-1.)) ;
#124382=DIRECTION('',(1.,0.,0.)) ;
#124383=DIRECTION('',(0.,0.,1.)) ;
#124384=DIRECTION('center_axis',(-7.01133629567814E-33,8.97270763436279E-17,
-1.)) ;
#124385=DIRECTION('ref_axis',(-6.83680877694706E-64,1.,8.97270763436279E-17)) ;
#124386=DIRECTION('center_axis',(-7.01133629567814E-33,8.97270763436279E-17,
-1.)) ;
#124387=DIRECTION('ref_axis',(6.29106707073161E-49,1.,8.97270763436279E-17)) ;
#124388=DIRECTION('center_axis',(-7.01133629567814E-33,8.97270763436279E-17,
-1.)) ;
#124389=DIRECTION('ref_axis',(6.29106707073161E-49,1.,8.97270763436279E-17)) ;
#124390=DIRECTION('',(-1.,-7.81406971160724E-17,0.)) ;
#124391=DIRECTION('',(7.81406971160724E-17,-1.,-8.9727076343628E-17)) ;
#124392=DIRECTION('',(1.,7.81406971160724E-17,0.)) ;
#124393=DIRECTION('',(0.,1.,8.9727076343628E-17)) ;
#124394=DIRECTION('center_axis',(7.01133629567814E-33,-8.97270763436279E-17,
1.)) ;
#124395=DIRECTION('ref_axis',(6.29106707073161E-49,1.,8.97270763436279E-17)) ;
#124396=DIRECTION('',(1.,0.,-7.01133629567814E-33)) ;
#124397=DIRECTION('',(0.,1.,8.9727076343628E-17)) ;
#124398=DIRECTION('',(-1.,0.,7.01133629567814E-33)) ;
#124399=DIRECTION('center_axis',(-7.81406971160724E-17,1.,0.)) ;
#124400=DIRECTION('ref_axis',(-1.,-7.81406971160724E-17,0.)) ;
#124401=DIRECTION('',(-1.,-7.81406971160724E-17,0.)) ;
#124402=DIRECTION('',(0.,0.,-1.)) ;
#124403=DIRECTION('',(1.,7.81406971160724E-17,0.)) ;
#124404=DIRECTION('',(0.,0.,1.)) ;
#124405=DIRECTION('center_axis',(-7.01133629567814E-33,8.97270763436279E-17,
1.)) ;
#124406=DIRECTION('ref_axis',(6.83680877694706E-64,-1.,8.97270763436279E-17)) ;
#124407=DIRECTION('',(1.,7.81406971160724E-17,0.)) ;
#124408=DIRECTION('center_axis',(-7.01133629567814E-33,8.97270763436279E-17,
1.)) ;
#124409=DIRECTION('ref_axis',(-6.29106707073161E-49,-1.,8.97270763436279E-17)) ;
#124410=DIRECTION('center_axis',(-7.01133629567814E-33,8.97270763436279E-17,
1.)) ;
#124411=DIRECTION('ref_axis',(-6.29106707073161E-49,-1.,8.97270763436279E-17)) ;
#124412=DIRECTION('',(1.,0.,7.01133629567814E-33)) ;
#124413=DIRECTION('',(0.,-1.,8.9727076343628E-17)) ;
#124414=DIRECTION('',(-1.,0.,-7.01133629567814E-33)) ;
#124415=DIRECTION('center_axis',(7.01133629567814E-33,-8.97270763436279E-17,
-1.)) ;
#124416=DIRECTION('ref_axis',(-6.29106707073161E-49,-1.,8.97270763436279E-17)) ;
#124417=DIRECTION('',(0.,-1.,8.9727076343628E-17)) ;
#124418=DIRECTION('',(-1.,-7.81406971160724E-17,0.)) ;
#124419=DIRECTION('',(-7.81406971160724E-17,1.,-8.9727076343628E-17)) ;
#124420=DIRECTION('center_axis',(-7.81406971160724E-17,1.,-4.8455963016112E-16)) ;
#124421=DIRECTION('ref_axis',(2.5241768025713E-48,4.8455963016112E-16,1.)) ;
#124422=DIRECTION('',(1.,7.81406971160724E-17,0.)) ;
#124423=DIRECTION('',(0.,4.8455963016112E-16,1.)) ;
#124424=DIRECTION('',(-1.,-7.81406971160724E-17,0.)) ;
#124425=DIRECTION('',(3.78638272950961E-32,-4.8455963016112E-16,-1.)) ;
#124426=DIRECTION('center_axis',(-7.01133629567814E-33,8.97270763436279E-17,
-1.)) ;
#124427=DIRECTION('ref_axis',(-6.83680877694706E-64,1.,8.97270763436279E-17)) ;
#124428=DIRECTION('center_axis',(-7.01133629567814E-33,8.97270763436279E-17,
-1.)) ;
#124429=DIRECTION('ref_axis',(6.29106707073161E-49,1.,8.97270763436279E-17)) ;
#124430=DIRECTION('center_axis',(-7.01133629567814E-33,8.97270763436279E-17,
-1.)) ;
#124431=DIRECTION('ref_axis',(6.29106707073161E-49,1.,8.97270763436279E-17)) ;
#124432=DIRECTION('',(-1.,-7.81406971160724E-17,0.)) ;
#124433=DIRECTION('',(7.81406971160724E-17,-1.,-8.9727076343628E-17)) ;
#124434=DIRECTION('',(1.,7.81406971160724E-17,0.)) ;
#124435=DIRECTION('',(0.,1.,8.9727076343628E-17)) ;
#124436=DIRECTION('center_axis',(7.01133629567814E-33,-8.97270763436279E-17,
1.)) ;
#124437=DIRECTION('ref_axis',(6.29106707073161E-49,1.,8.97270763436279E-17)) ;
#124438=DIRECTION('',(1.,0.,-7.01133629567814E-33)) ;
#124439=DIRECTION('',(0.,1.,8.9727076343628E-17)) ;
#124440=DIRECTION('',(-1.,0.,7.01133629567814E-33)) ;
#124441=DIRECTION('center_axis',(-7.81406971160724E-17,1.,0.)) ;
#124442=DIRECTION('ref_axis',(-1.,-7.81406971160724E-17,0.)) ;
#124443=DIRECTION('',(-1.,-7.81406971160724E-17,0.)) ;
#124444=DIRECTION('',(0.,0.,-1.)) ;
#124445=DIRECTION('',(1.,7.81406971160724E-17,0.)) ;
#124446=DIRECTION('',(0.,0.,1.)) ;
#124447=DIRECTION('center_axis',(-7.01133629567814E-33,8.97270763436279E-17,
1.)) ;
#124448=DIRECTION('ref_axis',(6.83680877694706E-64,-1.,8.97270763436279E-17)) ;
#124449=DIRECTION('',(1.,7.81406971160724E-17,0.)) ;
#124450=DIRECTION('center_axis',(-7.01133629567814E-33,8.97270763436279E-17,
1.)) ;
#124451=DIRECTION('ref_axis',(-6.29106707073161E-49,-1.,8.97270763436279E-17)) ;
#124452=DIRECTION('center_axis',(-7.01133629567814E-33,8.97270763436279E-17,
1.)) ;
#124453=DIRECTION('ref_axis',(-6.29106707073161E-49,-1.,8.97270763436279E-17)) ;
#124454=DIRECTION('',(1.,0.,7.01133629567814E-33)) ;
#124455=DIRECTION('',(0.,-1.,8.9727076343628E-17)) ;
#124456=DIRECTION('',(-1.,0.,-7.01133629567814E-33)) ;
#124457=DIRECTION('center_axis',(7.01133629567814E-33,-8.97270763436279E-17,
-1.)) ;
#124458=DIRECTION('ref_axis',(-6.29106707073161E-49,-1.,8.97270763436279E-17)) ;
#124459=DIRECTION('',(0.,-1.,8.9727076343628E-17)) ;
#124460=DIRECTION('',(-1.,-7.81406971160724E-17,0.)) ;
#124461=DIRECTION('',(-7.81406971160724E-17,1.,-8.9727076343628E-17)) ;
#124462=DIRECTION('center_axis',(-7.81406971160724E-17,1.,-4.8455963016112E-16)) ;
#124463=DIRECTION('ref_axis',(2.5241768025713E-48,4.8455963016112E-16,1.)) ;
#124464=DIRECTION('',(1.,7.81406971160724E-17,0.)) ;
#124465=DIRECTION('',(0.,4.8455963016112E-16,1.)) ;
#124466=DIRECTION('',(-1.,-7.81406971160724E-17,0.)) ;
#124467=DIRECTION('',(3.78638272950961E-32,-4.8455963016112E-16,-1.)) ;
#124468=DIRECTION('center_axis',(-7.01133629567814E-33,8.97270763436279E-17,
-1.)) ;
#124469=DIRECTION('ref_axis',(-6.83680877694706E-64,1.,8.97270763436279E-17)) ;
#124470=DIRECTION('center_axis',(-7.01133629567814E-33,8.97270763436279E-17,
-1.)) ;
#124471=DIRECTION('ref_axis',(6.29106707073161E-49,1.,8.97270763436279E-17)) ;
#124472=DIRECTION('center_axis',(-7.01133629567814E-33,8.97270763436279E-17,
-1.)) ;
#124473=DIRECTION('ref_axis',(6.29106707073161E-49,1.,8.97270763436279E-17)) ;
#124474=DIRECTION('',(-1.,-7.81406971160724E-17,0.)) ;
#124475=DIRECTION('',(7.81406971160724E-17,-1.,-8.9727076343628E-17)) ;
#124476=DIRECTION('',(1.,7.81406971160724E-17,0.)) ;
#124477=DIRECTION('',(0.,1.,8.9727076343628E-17)) ;
#124478=DIRECTION('center_axis',(7.01133629567814E-33,-8.97270763436279E-17,
1.)) ;
#124479=DIRECTION('ref_axis',(6.29106707073161E-49,1.,8.97270763436279E-17)) ;
#124480=DIRECTION('',(1.,0.,-7.01133629567814E-33)) ;
#124481=DIRECTION('',(0.,1.,8.9727076343628E-17)) ;
#124482=DIRECTION('',(-1.,0.,7.01133629567814E-33)) ;
#124483=DIRECTION('center_axis',(-7.81406971160724E-17,1.,0.)) ;
#124484=DIRECTION('ref_axis',(-1.,-7.81406971160724E-17,0.)) ;
#124485=DIRECTION('',(-1.,-7.81406971160724E-17,0.)) ;
#124486=DIRECTION('',(0.,0.,-1.)) ;
#124487=DIRECTION('',(1.,7.81406971160724E-17,0.)) ;
#124488=DIRECTION('',(0.,0.,1.)) ;
#124489=DIRECTION('center_axis',(-7.01133629567814E-33,8.97270763436279E-17,
1.)) ;
#124490=DIRECTION('ref_axis',(6.83680877694706E-64,-1.,8.97270763436279E-17)) ;
#124491=DIRECTION('',(1.,7.81406971160724E-17,0.)) ;
#124492=DIRECTION('center_axis',(-7.01133629567814E-33,8.97270763436279E-17,
1.)) ;
#124493=DIRECTION('ref_axis',(-6.29106707073161E-49,-1.,8.97270763436279E-17)) ;
#124494=DIRECTION('center_axis',(-7.01133629567814E-33,8.97270763436279E-17,
1.)) ;
#124495=DIRECTION('ref_axis',(-6.29106707073161E-49,-1.,8.97270763436279E-17)) ;
#124496=DIRECTION('',(1.,0.,7.01133629567814E-33)) ;
#124497=DIRECTION('',(0.,-1.,8.9727076343628E-17)) ;
#124498=DIRECTION('',(-1.,0.,-7.01133629567814E-33)) ;
#124499=DIRECTION('center_axis',(7.01133629567814E-33,-8.97270763436279E-17,
-1.)) ;
#124500=DIRECTION('ref_axis',(-6.29106707073161E-49,-1.,8.97270763436279E-17)) ;
#124501=DIRECTION('',(0.,-1.,8.9727076343628E-17)) ;
#124502=DIRECTION('',(-1.,-7.81406971160724E-17,0.)) ;
#124503=DIRECTION('',(-7.81406971160724E-17,1.,-8.9727076343628E-17)) ;
#124504=DIRECTION('center_axis',(-7.81406971160724E-17,1.,-4.8455963016112E-16)) ;
#124505=DIRECTION('ref_axis',(2.5241768025713E-48,4.8455963016112E-16,1.)) ;
#124506=DIRECTION('',(1.,7.81406971160724E-17,0.)) ;
#124507=DIRECTION('',(0.,4.8455963016112E-16,1.)) ;
#124508=DIRECTION('',(-1.,-7.81406971160724E-17,0.)) ;
#124509=DIRECTION('',(3.78638272950961E-32,-4.8455963016112E-16,-1.)) ;
#124510=DIRECTION('center_axis',(-7.01133629567814E-33,8.97270763436279E-17,
-1.)) ;
#124511=DIRECTION('ref_axis',(-6.83680877694706E-64,1.,8.97270763436279E-17)) ;
#124512=DIRECTION('center_axis',(-7.01133629567814E-33,8.97270763436279E-17,
-1.)) ;
#124513=DIRECTION('ref_axis',(6.29106707073161E-49,1.,8.97270763436279E-17)) ;
#124514=DIRECTION('center_axis',(-7.01133629567814E-33,8.97270763436279E-17,
-1.)) ;
#124515=DIRECTION('ref_axis',(6.29106707073161E-49,1.,8.97270763436279E-17)) ;
#124516=DIRECTION('',(-1.,-7.81406971160724E-17,0.)) ;
#124517=DIRECTION('',(7.81406971160724E-17,-1.,-8.9727076343628E-17)) ;
#124518=DIRECTION('',(1.,7.81406971160724E-17,0.)) ;
#124519=DIRECTION('',(0.,1.,8.9727076343628E-17)) ;
#124520=DIRECTION('center_axis',(7.01133629567814E-33,-8.97270763436279E-17,
1.)) ;
#124521=DIRECTION('ref_axis',(6.29106707073161E-49,1.,8.97270763436279E-17)) ;
#124522=DIRECTION('',(1.,0.,-7.01133629567814E-33)) ;
#124523=DIRECTION('',(0.,1.,8.9727076343628E-17)) ;
#124524=DIRECTION('',(-1.,0.,7.01133629567814E-33)) ;
#124525=DIRECTION('center_axis',(-7.81406971160724E-17,1.,0.)) ;
#124526=DIRECTION('ref_axis',(-1.,-7.81406971160724E-17,0.)) ;
#124527=DIRECTION('',(-1.,-7.81406971160724E-17,0.)) ;
#124528=DIRECTION('',(0.,0.,-1.)) ;
#124529=DIRECTION('',(1.,7.81406971160724E-17,0.)) ;
#124530=DIRECTION('',(0.,0.,1.)) ;
#124531=DIRECTION('center_axis',(-7.01133629567814E-33,8.97270763436279E-17,
1.)) ;
#124532=DIRECTION('ref_axis',(6.83680877694706E-64,-1.,8.97270763436279E-17)) ;
#124533=DIRECTION('',(1.,7.81406971160724E-17,0.)) ;
#124534=DIRECTION('center_axis',(-7.01133629567814E-33,8.97270763436279E-17,
1.)) ;
#124535=DIRECTION('ref_axis',(-6.29106707073161E-49,-1.,8.97270763436279E-17)) ;
#124536=DIRECTION('center_axis',(-7.01133629567814E-33,8.97270763436279E-17,
1.)) ;
#124537=DIRECTION('ref_axis',(-6.29106707073161E-49,-1.,8.97270763436279E-17)) ;
#124538=DIRECTION('',(1.,0.,7.01133629567814E-33)) ;
#124539=DIRECTION('',(0.,-1.,8.9727076343628E-17)) ;
#124540=DIRECTION('',(-1.,0.,-7.01133629567814E-33)) ;
#124541=DIRECTION('center_axis',(7.01133629567814E-33,-8.97270763436279E-17,
-1.)) ;
#124542=DIRECTION('ref_axis',(-6.29106707073161E-49,-1.,8.97270763436279E-17)) ;
#124543=DIRECTION('',(0.,-1.,8.9727076343628E-17)) ;
#124544=DIRECTION('',(-1.,-7.81406971160724E-17,0.)) ;
#124545=DIRECTION('',(-7.81406971160724E-17,1.,-8.9727076343628E-17)) ;
#124546=DIRECTION('center_axis',(-7.81406971160724E-17,1.,-4.8455963016112E-16)) ;
#124547=DIRECTION('ref_axis',(2.5241768025713E-48,4.8455963016112E-16,1.)) ;
#124548=DIRECTION('',(1.,7.81406971160724E-17,0.)) ;
#124549=DIRECTION('',(0.,4.8455963016112E-16,1.)) ;
#124550=DIRECTION('',(-1.,-7.81406971160724E-17,0.)) ;
#124551=DIRECTION('',(3.78638272950961E-32,-4.8455963016112E-16,-1.)) ;
#124552=DIRECTION('center_axis',(-7.01133629567814E-33,8.97270763436279E-17,
-1.)) ;
#124553=DIRECTION('ref_axis',(-6.83680877694706E-64,1.,8.97270763436279E-17)) ;
#124554=DIRECTION('center_axis',(-7.01133629567814E-33,8.97270763436279E-17,
-1.)) ;
#124555=DIRECTION('ref_axis',(6.29106707073161E-49,1.,8.97270763436279E-17)) ;
#124556=DIRECTION('center_axis',(-7.01133629567814E-33,8.97270763436279E-17,
-1.)) ;
#124557=DIRECTION('ref_axis',(6.29106707073161E-49,1.,8.97270763436279E-17)) ;
#124558=DIRECTION('',(-1.,-7.81406971160724E-17,0.)) ;
#124559=DIRECTION('',(7.81406971160724E-17,-1.,-8.9727076343628E-17)) ;
#124560=DIRECTION('',(1.,7.81406971160724E-17,0.)) ;
#124561=DIRECTION('',(0.,1.,8.9727076343628E-17)) ;
#124562=DIRECTION('center_axis',(7.01133629567814E-33,-8.97270763436279E-17,
1.)) ;
#124563=DIRECTION('ref_axis',(6.29106707073161E-49,1.,8.97270763436279E-17)) ;
#124564=DIRECTION('',(1.,0.,-7.01133629567814E-33)) ;
#124565=DIRECTION('',(0.,1.,8.9727076343628E-17)) ;
#124566=DIRECTION('',(-1.,0.,7.01133629567814E-33)) ;
#124567=DIRECTION('center_axis',(-7.81406971160724E-17,1.,0.)) ;
#124568=DIRECTION('ref_axis',(-1.,-7.81406971160724E-17,0.)) ;
#124569=DIRECTION('',(-1.,-7.81406971160724E-17,0.)) ;
#124570=DIRECTION('',(0.,0.,-1.)) ;
#124571=DIRECTION('',(1.,7.81406971160724E-17,0.)) ;
#124572=DIRECTION('',(0.,0.,1.)) ;
#124573=DIRECTION('center_axis',(-7.01133629567814E-33,8.97270763436279E-17,
1.)) ;
#124574=DIRECTION('ref_axis',(6.83680877694706E-64,-1.,8.97270763436279E-17)) ;
#124575=DIRECTION('',(1.,7.81406971160724E-17,0.)) ;
#124576=DIRECTION('center_axis',(-7.01133629567814E-33,8.97270763436279E-17,
1.)) ;
#124577=DIRECTION('ref_axis',(-6.29106707073161E-49,-1.,8.97270763436279E-17)) ;
#124578=DIRECTION('center_axis',(-7.01133629567814E-33,8.97270763436279E-17,
1.)) ;
#124579=DIRECTION('ref_axis',(-6.29106707073161E-49,-1.,8.97270763436279E-17)) ;
#124580=DIRECTION('',(1.,0.,7.01133629567814E-33)) ;
#124581=DIRECTION('',(0.,-1.,8.9727076343628E-17)) ;
#124582=DIRECTION('',(-1.,0.,-7.01133629567814E-33)) ;
#124583=DIRECTION('center_axis',(7.01133629567814E-33,-8.97270763436279E-17,
-1.)) ;
#124584=DIRECTION('ref_axis',(-6.29106707073161E-49,-1.,8.97270763436279E-17)) ;
#124585=DIRECTION('',(0.,-1.,8.9727076343628E-17)) ;
#124586=DIRECTION('',(-1.,-7.81406971160724E-17,0.)) ;
#124587=DIRECTION('',(-7.81406971160724E-17,1.,-8.9727076343628E-17)) ;
#124588=DIRECTION('center_axis',(-7.81406971160724E-17,1.,-4.8455963016112E-16)) ;
#124589=DIRECTION('ref_axis',(2.5241768025713E-48,4.8455963016112E-16,1.)) ;
#124590=DIRECTION('',(1.,7.81406971160724E-17,0.)) ;
#124591=DIRECTION('',(0.,4.8455963016112E-16,1.)) ;
#124592=DIRECTION('',(-1.,-7.81406971160724E-17,0.)) ;
#124593=DIRECTION('',(3.78638272950961E-32,-4.8455963016112E-16,-1.)) ;
#124594=DIRECTION('center_axis',(-7.01133629567814E-33,8.97270763436279E-17,
-1.)) ;
#124595=DIRECTION('ref_axis',(-6.83680877694706E-64,1.,8.97270763436279E-17)) ;
#124596=DIRECTION('center_axis',(-7.01133629567814E-33,8.97270763436279E-17,
-1.)) ;
#124597=DIRECTION('ref_axis',(6.29106707073161E-49,1.,8.97270763436279E-17)) ;
#124598=DIRECTION('center_axis',(-7.01133629567814E-33,8.97270763436279E-17,
-1.)) ;
#124599=DIRECTION('ref_axis',(6.29106707073161E-49,1.,8.97270763436279E-17)) ;
#124600=DIRECTION('',(-1.,-7.81406971160724E-17,0.)) ;
#124601=DIRECTION('',(7.81406971160724E-17,-1.,-8.9727076343628E-17)) ;
#124602=DIRECTION('',(1.,7.81406971160724E-17,0.)) ;
#124603=DIRECTION('',(0.,1.,8.9727076343628E-17)) ;
#124604=DIRECTION('center_axis',(7.01133629567814E-33,-8.97270763436279E-17,
1.)) ;
#124605=DIRECTION('ref_axis',(6.29106707073161E-49,1.,8.97270763436279E-17)) ;
#124606=DIRECTION('',(1.,0.,-7.01133629567814E-33)) ;
#124607=DIRECTION('',(0.,1.,8.9727076343628E-17)) ;
#124608=DIRECTION('',(-1.,0.,7.01133629567814E-33)) ;
#124609=DIRECTION('center_axis',(-7.81406971160724E-17,1.,0.)) ;
#124610=DIRECTION('ref_axis',(-1.,-7.81406971160724E-17,0.)) ;
#124611=DIRECTION('',(-1.,-7.81406971160724E-17,0.)) ;
#124612=DIRECTION('',(0.,0.,-1.)) ;
#124613=DIRECTION('',(1.,7.81406971160724E-17,0.)) ;
#124614=DIRECTION('',(0.,0.,1.)) ;
#124615=DIRECTION('center_axis',(-7.01133629567814E-33,8.97270763436279E-17,
1.)) ;
#124616=DIRECTION('ref_axis',(6.83680877694706E-64,-1.,8.97270763436279E-17)) ;
#124617=DIRECTION('',(1.,7.81406971160724E-17,0.)) ;
#124618=DIRECTION('center_axis',(-7.01133629567814E-33,8.97270763436279E-17,
1.)) ;
#124619=DIRECTION('ref_axis',(-6.29106707073161E-49,-1.,8.97270763436279E-17)) ;
#124620=DIRECTION('center_axis',(-7.01133629567814E-33,8.97270763436279E-17,
1.)) ;
#124621=DIRECTION('ref_axis',(-6.29106707073161E-49,-1.,8.97270763436279E-17)) ;
#124622=DIRECTION('',(1.,0.,7.01133629567814E-33)) ;
#124623=DIRECTION('',(0.,-1.,8.9727076343628E-17)) ;
#124624=DIRECTION('',(-1.,0.,-7.01133629567814E-33)) ;
#124625=DIRECTION('center_axis',(7.01133629567814E-33,-8.97270763436279E-17,
-1.)) ;
#124626=DIRECTION('ref_axis',(-6.29106707073161E-49,-1.,8.97270763436279E-17)) ;
#124627=DIRECTION('',(0.,-1.,8.9727076343628E-17)) ;
#124628=DIRECTION('',(-1.,-7.81406971160724E-17,0.)) ;
#124629=DIRECTION('',(-7.81406971160724E-17,1.,-8.9727076343628E-17)) ;
#124630=DIRECTION('center_axis',(-7.81406971160724E-17,1.,-4.8455963016112E-16)) ;
#124631=DIRECTION('ref_axis',(2.5241768025713E-48,4.8455963016112E-16,1.)) ;
#124632=DIRECTION('',(1.,7.81406971160724E-17,0.)) ;
#124633=DIRECTION('',(0.,4.8455963016112E-16,1.)) ;
#124634=DIRECTION('',(-1.,-7.81406971160724E-17,0.)) ;
#124635=DIRECTION('',(3.78638272950961E-32,-4.8455963016112E-16,-1.)) ;
#124636=DIRECTION('center_axis',(-7.01133629567814E-33,8.97270763436279E-17,
-1.)) ;
#124637=DIRECTION('ref_axis',(-6.83680877694706E-64,1.,8.97270763436279E-17)) ;
#124638=DIRECTION('center_axis',(-7.01133629567814E-33,8.97270763436279E-17,
-1.)) ;
#124639=DIRECTION('ref_axis',(6.29106707073161E-49,1.,8.97270763436279E-17)) ;
#124640=DIRECTION('center_axis',(-7.01133629567814E-33,8.97270763436279E-17,
-1.)) ;
#124641=DIRECTION('ref_axis',(6.29106707073161E-49,1.,8.97270763436279E-17)) ;
#124642=DIRECTION('',(-1.,-7.81406971160724E-17,0.)) ;
#124643=DIRECTION('',(7.81406971160724E-17,-1.,-8.9727076343628E-17)) ;
#124644=DIRECTION('',(1.,7.81406971160724E-17,0.)) ;
#124645=DIRECTION('',(0.,1.,8.9727076343628E-17)) ;
#124646=DIRECTION('center_axis',(7.01133629567814E-33,-8.97270763436279E-17,
1.)) ;
#124647=DIRECTION('ref_axis',(6.29106707073161E-49,1.,8.97270763436279E-17)) ;
#124648=DIRECTION('',(1.,0.,-7.01133629567814E-33)) ;
#124649=DIRECTION('',(0.,1.,8.9727076343628E-17)) ;
#124650=DIRECTION('',(-1.,0.,7.01133629567814E-33)) ;
#124651=DIRECTION('center_axis',(-7.81406971160724E-17,1.,0.)) ;
#124652=DIRECTION('ref_axis',(-1.,-7.81406971160724E-17,0.)) ;
#124653=DIRECTION('',(-1.,-7.81406971160724E-17,0.)) ;
#124654=DIRECTION('',(0.,0.,-1.)) ;
#124655=DIRECTION('',(1.,7.81406971160724E-17,0.)) ;
#124656=DIRECTION('',(0.,0.,1.)) ;
#124657=DIRECTION('center_axis',(-7.01133629567814E-33,8.97270763436279E-17,
1.)) ;
#124658=DIRECTION('ref_axis',(6.83680877694706E-64,-1.,8.97270763436279E-17)) ;
#124659=DIRECTION('',(1.,7.81406971160724E-17,0.)) ;
#124660=DIRECTION('center_axis',(-7.01133629567814E-33,8.97270763436279E-17,
1.)) ;
#124661=DIRECTION('ref_axis',(-6.29106707073161E-49,-1.,8.97270763436279E-17)) ;
#124662=DIRECTION('center_axis',(-7.01133629567814E-33,8.97270763436279E-17,
1.)) ;
#124663=DIRECTION('ref_axis',(-6.29106707073161E-49,-1.,8.97270763436279E-17)) ;
#124664=DIRECTION('',(1.,0.,7.01133629567814E-33)) ;
#124665=DIRECTION('',(0.,-1.,8.9727076343628E-17)) ;
#124666=DIRECTION('',(-1.,0.,-7.01133629567814E-33)) ;
#124667=DIRECTION('center_axis',(7.01133629567814E-33,-8.97270763436279E-17,
-1.)) ;
#124668=DIRECTION('ref_axis',(-6.29106707073161E-49,-1.,8.97270763436279E-17)) ;
#124669=DIRECTION('',(0.,-1.,8.9727076343628E-17)) ;
#124670=DIRECTION('',(-1.,-7.81406971160724E-17,0.)) ;
#124671=DIRECTION('',(-7.81406971160724E-17,1.,-8.9727076343628E-17)) ;
#124672=DIRECTION('center_axis',(-7.81406971160724E-17,1.,-4.8455963016112E-16)) ;
#124673=DIRECTION('ref_axis',(2.5241768025713E-48,4.8455963016112E-16,1.)) ;
#124674=DIRECTION('',(1.,7.81406971160724E-17,0.)) ;
#124675=DIRECTION('',(0.,4.8455963016112E-16,1.)) ;
#124676=DIRECTION('',(-1.,-7.81406971160724E-17,0.)) ;
#124677=DIRECTION('',(3.78638272950961E-32,-4.8455963016112E-16,-1.)) ;
#124678=DIRECTION('center_axis',(-7.01133629567814E-33,8.97270763436279E-17,
-1.)) ;
#124679=DIRECTION('ref_axis',(-6.83680877694706E-64,1.,8.97270763436279E-17)) ;
#124680=DIRECTION('center_axis',(-7.01133629567814E-33,8.97270763436279E-17,
-1.)) ;
#124681=DIRECTION('ref_axis',(6.29106707073161E-49,1.,8.97270763436279E-17)) ;
#124682=DIRECTION('center_axis',(-7.01133629567814E-33,8.97270763436279E-17,
-1.)) ;
#124683=DIRECTION('ref_axis',(6.29106707073161E-49,1.,8.97270763436279E-17)) ;
#124684=DIRECTION('',(-1.,-7.81406971160724E-17,0.)) ;
#124685=DIRECTION('',(7.81406971160724E-17,-1.,-8.9727076343628E-17)) ;
#124686=DIRECTION('',(1.,7.81406971160724E-17,0.)) ;
#124687=DIRECTION('',(0.,1.,8.9727076343628E-17)) ;
#124688=DIRECTION('center_axis',(7.01133629567814E-33,-8.97270763436279E-17,
1.)) ;
#124689=DIRECTION('ref_axis',(6.29106707073161E-49,1.,8.97270763436279E-17)) ;
#124690=DIRECTION('',(1.,0.,-7.01133629567814E-33)) ;
#124691=DIRECTION('',(0.,1.,8.9727076343628E-17)) ;
#124692=DIRECTION('',(-1.,0.,7.01133629567814E-33)) ;
#124693=DIRECTION('center_axis',(-7.81406971160724E-17,1.,0.)) ;
#124694=DIRECTION('ref_axis',(-1.,-7.81406971160724E-17,0.)) ;
#124695=DIRECTION('',(-1.,-7.81406971160724E-17,0.)) ;
#124696=DIRECTION('',(0.,0.,-1.)) ;
#124697=DIRECTION('',(1.,7.81406971160724E-17,0.)) ;
#124698=DIRECTION('',(0.,0.,1.)) ;
#124699=DIRECTION('center_axis',(-7.01133629567814E-33,8.97270763436279E-17,
1.)) ;
#124700=DIRECTION('ref_axis',(6.83680877694706E-64,-1.,8.97270763436279E-17)) ;
#124701=DIRECTION('',(1.,7.81406971160724E-17,0.)) ;
#124702=DIRECTION('center_axis',(-7.01133629567814E-33,8.97270763436279E-17,
1.)) ;
#124703=DIRECTION('ref_axis',(-6.29106707073161E-49,-1.,8.97270763436279E-17)) ;
#124704=DIRECTION('center_axis',(-7.01133629567814E-33,8.97270763436279E-17,
1.)) ;
#124705=DIRECTION('ref_axis',(-6.29106707073161E-49,-1.,8.97270763436279E-17)) ;
#124706=DIRECTION('',(1.,0.,7.01133629567814E-33)) ;
#124707=DIRECTION('',(0.,-1.,8.9727076343628E-17)) ;
#124708=DIRECTION('',(-1.,0.,-7.01133629567814E-33)) ;
#124709=DIRECTION('center_axis',(7.01133629567814E-33,-8.97270763436279E-17,
-1.)) ;
#124710=DIRECTION('ref_axis',(-6.29106707073161E-49,-1.,8.97270763436279E-17)) ;
#124711=DIRECTION('',(0.,-1.,8.9727076343628E-17)) ;
#124712=DIRECTION('',(-1.,-7.81406971160724E-17,0.)) ;
#124713=DIRECTION('',(-7.81406971160724E-17,1.,-8.9727076343628E-17)) ;
#124714=DIRECTION('center_axis',(-7.81406971160724E-17,1.,-4.8455963016112E-16)) ;
#124715=DIRECTION('ref_axis',(2.5241768025713E-48,4.8455963016112E-16,1.)) ;
#124716=DIRECTION('',(1.,7.81406971160724E-17,0.)) ;
#124717=DIRECTION('',(0.,4.8455963016112E-16,1.)) ;
#124718=DIRECTION('',(-1.,-7.81406971160724E-17,0.)) ;
#124719=DIRECTION('',(3.78638272950961E-32,-4.8455963016112E-16,-1.)) ;
#124720=DIRECTION('center_axis',(-7.01133629567814E-33,8.97270763436279E-17,
-1.)) ;
#124721=DIRECTION('ref_axis',(-6.83680877694706E-64,1.,8.97270763436279E-17)) ;
#124722=DIRECTION('center_axis',(-7.01133629567814E-33,8.97270763436279E-17,
-1.)) ;
#124723=DIRECTION('ref_axis',(6.29106707073161E-49,1.,8.97270763436279E-17)) ;
#124724=DIRECTION('center_axis',(-7.01133629567814E-33,8.97270763436279E-17,
-1.)) ;
#124725=DIRECTION('ref_axis',(6.29106707073161E-49,1.,8.97270763436279E-17)) ;
#124726=DIRECTION('',(-1.,-7.81406971160724E-17,0.)) ;
#124727=DIRECTION('',(7.81406971160724E-17,-1.,-8.9727076343628E-17)) ;
#124728=DIRECTION('',(1.,7.81406971160724E-17,0.)) ;
#124729=DIRECTION('',(0.,1.,8.9727076343628E-17)) ;
#124730=DIRECTION('center_axis',(7.01133629567814E-33,-8.97270763436279E-17,
1.)) ;
#124731=DIRECTION('ref_axis',(6.29106707073161E-49,1.,8.97270763436279E-17)) ;
#124732=DIRECTION('',(1.,0.,-7.01133629567814E-33)) ;
#124733=DIRECTION('',(0.,1.,8.9727076343628E-17)) ;
#124734=DIRECTION('',(-1.,0.,7.01133629567814E-33)) ;
#124735=DIRECTION('center_axis',(-7.81406971160724E-17,1.,0.)) ;
#124736=DIRECTION('ref_axis',(-1.,-7.81406971160724E-17,0.)) ;
#124737=DIRECTION('',(-1.,-7.81406971160724E-17,0.)) ;
#124738=DIRECTION('',(0.,0.,-1.)) ;
#124739=DIRECTION('',(1.,7.81406971160724E-17,0.)) ;
#124740=DIRECTION('',(0.,0.,1.)) ;
#124741=DIRECTION('center_axis',(-7.01133629567814E-33,8.97270763436279E-17,
1.)) ;
#124742=DIRECTION('ref_axis',(6.83680877694706E-64,-1.,8.97270763436279E-17)) ;
#124743=DIRECTION('',(1.,7.81406971160724E-17,0.)) ;
#124744=DIRECTION('center_axis',(-7.01133629567814E-33,8.97270763436279E-17,
1.)) ;
#124745=DIRECTION('ref_axis',(-6.29106707073161E-49,-1.,8.97270763436279E-17)) ;
#124746=DIRECTION('center_axis',(-7.01133629567814E-33,8.97270763436279E-17,
1.)) ;
#124747=DIRECTION('ref_axis',(-6.29106707073161E-49,-1.,8.97270763436279E-17)) ;
#124748=DIRECTION('',(1.,0.,7.01133629567814E-33)) ;
#124749=DIRECTION('',(0.,-1.,8.9727076343628E-17)) ;
#124750=DIRECTION('',(-1.,0.,-7.01133629567814E-33)) ;
#124751=DIRECTION('center_axis',(7.01133629567814E-33,-8.97270763436279E-17,
-1.)) ;
#124752=DIRECTION('ref_axis',(-6.29106707073161E-49,-1.,8.97270763436279E-17)) ;
#124753=DIRECTION('',(0.,-1.,8.9727076343628E-17)) ;
#124754=DIRECTION('',(-1.,-7.81406971160724E-17,0.)) ;
#124755=DIRECTION('',(-7.81406971160724E-17,1.,-8.9727076343628E-17)) ;
#124756=DIRECTION('center_axis',(-7.81406971160724E-17,1.,-4.8455963016112E-16)) ;
#124757=DIRECTION('ref_axis',(2.5241768025713E-48,4.8455963016112E-16,1.)) ;
#124758=DIRECTION('',(3.78638272950961E-32,-4.8455963016112E-16,-1.)) ;
#124759=DIRECTION('',(1.,7.81406971160724E-17,0.)) ;
#124760=DIRECTION('',(0.,4.8455963016112E-16,1.)) ;
#124761=DIRECTION('',(-1.,-7.81406971160724E-17,0.)) ;
#124762=DIRECTION('center_axis',(0.,1.,0.)) ;
#124763=DIRECTION('ref_axis',(0.,0.,1.)) ;
#124764=DIRECTION('',(-1.,0.,0.)) ;
#124765=DIRECTION('',(0.,0.,-1.)) ;
#124766=DIRECTION('',(1.,0.,7.01133629567814E-33)) ;
#124767=DIRECTION('',(0.,0.,1.)) ;
#124768=DIRECTION('center_axis',(0.,1.,0.)) ;
#124769=DIRECTION('ref_axis',(0.,0.,1.)) ;
#124770=DIRECTION('',(-1.,0.,7.01133629567814E-33)) ;
#124771=DIRECTION('',(0.,0.,-1.)) ;
#124772=DIRECTION('',(1.,0.,0.)) ;
#124773=DIRECTION('',(0.,0.,1.)) ;
#124774=DIRECTION('center_axis',(-1.,0.,0.)) ;
#124775=DIRECTION('ref_axis',(0.,0.,1.)) ;
#124776=DIRECTION('',(-1.,0.,0.)) ;
#124777=DIRECTION('center_axis',(-1.,0.,0.)) ;
#124778=DIRECTION('ref_axis',(0.,7.85535158932893E-16,-1.)) ;
#124779=DIRECTION('',(1.,0.,0.)) ;
#124780=DIRECTION('center_axis',(1.,0.,0.)) ;
#124781=DIRECTION('ref_axis',(0.,0.,-1.)) ;
#124782=DIRECTION('center_axis',(1.,0.,0.)) ;
#124783=DIRECTION('ref_axis',(0.,0.,-1.)) ;
#124784=DIRECTION('',(0.,0.,-1.)) ;
#124785=DIRECTION('center_axis',(-1.,0.,0.)) ;
#124786=DIRECTION('ref_axis',(0.,0.,-1.)) ;
#124787=DIRECTION('',(0.,0.,-1.)) ;
#124788=DIRECTION('',(0.,1.,-8.9727076343628E-17)) ;
#124789=DIRECTION('',(0.,0.,1.)) ;
#124790=DIRECTION('',(0.,-1.,-8.9727076343628E-17)) ;
#124791=DIRECTION('center_axis',(0.,1.,0.)) ;
#124792=DIRECTION('ref_axis',(0.,0.,1.)) ;
#124793=DIRECTION('',(-1.,0.,0.)) ;
#124794=DIRECTION('',(0.,0.,-1.)) ;
#124795=DIRECTION('',(1.,0.,7.01133629567814E-33)) ;
#124796=DIRECTION('',(0.,0.,1.)) ;
#124797=DIRECTION('center_axis',(0.,1.,0.)) ;
#124798=DIRECTION('ref_axis',(0.,0.,1.)) ;
#124799=DIRECTION('',(-1.,0.,7.01133629567814E-33)) ;
#124800=DIRECTION('',(0.,0.,-1.)) ;
#124801=DIRECTION('',(1.,0.,0.)) ;
#124802=DIRECTION('',(0.,0.,1.)) ;
#124803=DIRECTION('center_axis',(-1.,0.,0.)) ;
#124804=DIRECTION('ref_axis',(0.,0.,1.)) ;
#124805=DIRECTION('',(-1.,0.,0.)) ;
#124806=DIRECTION('center_axis',(-1.,0.,0.)) ;
#124807=DIRECTION('ref_axis',(0.,0.,-1.)) ;
#124808=DIRECTION('',(1.,0.,0.)) ;
#124809=DIRECTION('center_axis',(1.,0.,0.)) ;
#124810=DIRECTION('ref_axis',(0.,0.,-1.)) ;
#124811=DIRECTION('center_axis',(1.,0.,0.)) ;
#124812=DIRECTION('ref_axis',(0.,0.,-1.)) ;
#124813=DIRECTION('',(0.,0.,-1.)) ;
#124814=DIRECTION('center_axis',(-1.,0.,0.)) ;
#124815=DIRECTION('ref_axis',(0.,9.87742904470778E-16,-1.)) ;
#124816=DIRECTION('',(0.,0.,-1.)) ;
#124817=DIRECTION('',(0.,1.,-8.9727076343628E-17)) ;
#124818=DIRECTION('',(0.,0.,1.)) ;
#124819=DIRECTION('',(0.,-1.,-8.9727076343628E-17)) ;
#124820=DIRECTION('center_axis',(0.,1.,0.)) ;
#124821=DIRECTION('ref_axis',(0.,0.,1.)) ;
#124822=DIRECTION('',(-1.,0.,0.)) ;
#124823=DIRECTION('',(0.,0.,-1.)) ;
#124824=DIRECTION('',(1.,0.,7.01133629567814E-33)) ;
#124825=DIRECTION('',(0.,0.,1.)) ;
#124826=DIRECTION('center_axis',(0.,1.,0.)) ;
#124827=DIRECTION('ref_axis',(0.,0.,1.)) ;
#124828=DIRECTION('',(-1.,0.,7.01133629567814E-33)) ;
#124829=DIRECTION('',(0.,0.,-1.)) ;
#124830=DIRECTION('',(1.,0.,0.)) ;
#124831=DIRECTION('',(0.,0.,1.)) ;
#124832=DIRECTION('center_axis',(-1.,0.,0.)) ;
#124833=DIRECTION('ref_axis',(0.,0.,1.)) ;
#124834=DIRECTION('',(-1.,0.,0.)) ;
#124835=DIRECTION('center_axis',(-1.,0.,0.)) ;
#124836=DIRECTION('ref_axis',(0.,0.,-1.)) ;
#124837=DIRECTION('',(1.,0.,0.)) ;
#124838=DIRECTION('center_axis',(1.,0.,0.)) ;
#124839=DIRECTION('ref_axis',(0.,0.,-1.)) ;
#124840=DIRECTION('center_axis',(1.,0.,0.)) ;
#124841=DIRECTION('ref_axis',(0.,0.,-1.)) ;
#124842=DIRECTION('',(0.,0.,-1.)) ;
#124843=DIRECTION('center_axis',(-1.,0.,0.)) ;
#124844=DIRECTION('ref_axis',(0.,3.45710016564773E-15,-1.)) ;
#124845=DIRECTION('',(0.,0.,-1.)) ;
#124846=DIRECTION('',(0.,1.,-8.9727076343628E-17)) ;
#124847=DIRECTION('',(0.,0.,1.)) ;
#124848=DIRECTION('',(0.,-1.,-8.9727076343628E-17)) ;
#124849=DIRECTION('center_axis',(0.,1.,0.)) ;
#124850=DIRECTION('ref_axis',(0.,0.,1.)) ;
#124851=DIRECTION('',(-1.,0.,0.)) ;
#124852=DIRECTION('',(0.,0.,-1.)) ;
#124853=DIRECTION('',(1.,0.,7.01133629567814E-33)) ;
#124854=DIRECTION('',(0.,0.,1.)) ;
#124855=DIRECTION('center_axis',(0.,1.,0.)) ;
#124856=DIRECTION('ref_axis',(0.,0.,1.)) ;
#124857=DIRECTION('',(-1.,0.,7.01133629567814E-33)) ;
#124858=DIRECTION('',(0.,0.,-1.)) ;
#124859=DIRECTION('',(1.,0.,0.)) ;
#124860=DIRECTION('',(0.,0.,1.)) ;
#124861=DIRECTION('center_axis',(-1.,0.,0.)) ;
#124862=DIRECTION('ref_axis',(0.,0.,1.)) ;
#124863=DIRECTION('',(-1.,0.,0.)) ;
#124864=DIRECTION('center_axis',(-1.,0.,0.)) ;
#124865=DIRECTION('ref_axis',(0.,7.85535158932893E-16,-1.)) ;
#124866=DIRECTION('',(1.,0.,0.)) ;
#124867=DIRECTION('center_axis',(1.,0.,0.)) ;
#124868=DIRECTION('ref_axis',(0.,0.,-1.)) ;
#124869=DIRECTION('center_axis',(1.,0.,0.)) ;
#124870=DIRECTION('ref_axis',(0.,0.,-1.)) ;
#124871=DIRECTION('',(0.,0.,-1.)) ;
#124872=DIRECTION('center_axis',(-1.,0.,0.)) ;
#124873=DIRECTION('ref_axis',(0.,0.,-1.)) ;
#124874=DIRECTION('',(0.,0.,-1.)) ;
#124875=DIRECTION('',(0.,1.,-8.9727076343628E-17)) ;
#124876=DIRECTION('',(0.,0.,1.)) ;
#124877=DIRECTION('',(0.,-1.,-8.9727076343628E-17)) ;
#124878=DIRECTION('center_axis',(0.,1.,0.)) ;
#124879=DIRECTION('ref_axis',(0.,0.,1.)) ;
#124880=DIRECTION('',(-1.,0.,0.)) ;
#124881=DIRECTION('',(0.,0.,-1.)) ;
#124882=DIRECTION('',(1.,0.,7.01133629567814E-33)) ;
#124883=DIRECTION('',(0.,0.,1.)) ;
#124884=DIRECTION('center_axis',(0.,1.,0.)) ;
#124885=DIRECTION('ref_axis',(0.,0.,1.)) ;
#124886=DIRECTION('',(-1.,0.,7.01133629567814E-33)) ;
#124887=DIRECTION('',(0.,0.,-1.)) ;
#124888=DIRECTION('',(1.,0.,0.)) ;
#124889=DIRECTION('',(0.,0.,1.)) ;
#124890=DIRECTION('center_axis',(-1.,0.,0.)) ;
#124891=DIRECTION('ref_axis',(0.,0.,1.)) ;
#124892=DIRECTION('',(-1.,0.,0.)) ;
#124893=DIRECTION('center_axis',(-1.,0.,0.)) ;
#124894=DIRECTION('ref_axis',(0.,3.66583074168683E-15,-1.)) ;
#124895=DIRECTION('',(1.,0.,0.)) ;
#124896=DIRECTION('center_axis',(1.,0.,0.)) ;
#124897=DIRECTION('ref_axis',(0.,0.,-1.)) ;
#124898=DIRECTION('center_axis',(1.,0.,0.)) ;
#124899=DIRECTION('ref_axis',(0.,0.,-1.)) ;
#124900=DIRECTION('',(0.,0.,-1.)) ;
#124901=DIRECTION('center_axis',(-1.,0.,0.)) ;
#124902=DIRECTION('ref_axis',(0.,-5.43258597458929E-15,-1.)) ;
#124903=DIRECTION('',(0.,0.,-1.)) ;
#124904=DIRECTION('',(0.,1.,-8.9727076343628E-17)) ;
#124905=DIRECTION('',(0.,0.,1.)) ;
#124906=DIRECTION('',(0.,-1.,-8.9727076343628E-17)) ;
#124907=DIRECTION('center_axis',(0.,1.,0.)) ;
#124908=DIRECTION('ref_axis',(0.,0.,1.)) ;
#124909=DIRECTION('',(-1.,0.,0.)) ;
#124910=DIRECTION('',(0.,0.,-1.)) ;
#124911=DIRECTION('',(1.,0.,7.01133629567814E-33)) ;
#124912=DIRECTION('',(0.,0.,1.)) ;
#124913=DIRECTION('center_axis',(0.,1.,0.)) ;
#124914=DIRECTION('ref_axis',(0.,0.,1.)) ;
#124915=DIRECTION('',(-1.,0.,7.01133629567814E-33)) ;
#124916=DIRECTION('',(0.,0.,-1.)) ;
#124917=DIRECTION('',(1.,0.,0.)) ;
#124918=DIRECTION('',(0.,0.,1.)) ;
#124919=DIRECTION('center_axis',(-1.,0.,0.)) ;
#124920=DIRECTION('ref_axis',(0.,0.,1.)) ;
#124921=DIRECTION('',(-1.,0.,0.)) ;
#124922=DIRECTION('center_axis',(-1.,0.,0.)) ;
#124923=DIRECTION('ref_axis',(0.,3.66583074168683E-15,-1.)) ;
#124924=DIRECTION('',(1.,0.,0.)) ;
#124925=DIRECTION('center_axis',(1.,0.,0.)) ;
#124926=DIRECTION('ref_axis',(0.,0.,-1.)) ;
#124927=DIRECTION('center_axis',(1.,0.,0.)) ;
#124928=DIRECTION('ref_axis',(0.,0.,-1.)) ;
#124929=DIRECTION('',(0.,0.,-1.)) ;
#124930=DIRECTION('center_axis',(-1.,0.,0.)) ;
#124931=DIRECTION('ref_axis',(0.,-5.43258597458929E-15,-1.)) ;
#124932=DIRECTION('',(0.,0.,-1.)) ;
#124933=DIRECTION('',(0.,1.,-8.9727076343628E-17)) ;
#124934=DIRECTION('',(0.,0.,1.)) ;
#124935=DIRECTION('',(0.,-1.,-8.9727076343628E-17)) ;
#124936=DIRECTION('center_axis',(0.,1.,0.)) ;
#124937=DIRECTION('ref_axis',(0.,0.,1.)) ;
#124938=DIRECTION('',(-1.,0.,0.)) ;
#124939=DIRECTION('',(0.,0.,-1.)) ;
#124940=DIRECTION('',(1.,0.,7.01133629567814E-33)) ;
#124941=DIRECTION('',(0.,0.,1.)) ;
#124942=DIRECTION('center_axis',(0.,1.,0.)) ;
#124943=DIRECTION('ref_axis',(0.,0.,1.)) ;
#124944=DIRECTION('',(-1.,0.,7.01133629567814E-33)) ;
#124945=DIRECTION('',(0.,0.,-1.)) ;
#124946=DIRECTION('',(1.,0.,0.)) ;
#124947=DIRECTION('',(0.,0.,1.)) ;
#124948=DIRECTION('center_axis',(-1.,0.,0.)) ;
#124949=DIRECTION('ref_axis',(0.,0.,1.)) ;
#124950=DIRECTION('',(-1.,0.,0.)) ;
#124951=DIRECTION('center_axis',(-1.,0.,0.)) ;
#124952=DIRECTION('ref_axis',(0.,3.66583074168683E-15,-1.)) ;
#124953=DIRECTION('',(1.,0.,0.)) ;
#124954=DIRECTION('center_axis',(1.,0.,0.)) ;
#124955=DIRECTION('ref_axis',(0.,0.,-1.)) ;
#124956=DIRECTION('center_axis',(1.,0.,0.)) ;
#124957=DIRECTION('ref_axis',(0.,0.,-1.)) ;
#124958=DIRECTION('',(0.,0.,-1.)) ;
#124959=DIRECTION('center_axis',(-1.,0.,0.)) ;
#124960=DIRECTION('ref_axis',(0.,-5.43258597458929E-15,-1.)) ;
#124961=DIRECTION('',(0.,0.,-1.)) ;
#124962=DIRECTION('',(0.,1.,-8.9727076343628E-17)) ;
#124963=DIRECTION('',(0.,0.,1.)) ;
#124964=DIRECTION('',(0.,-1.,-8.9727076343628E-17)) ;
#124965=DIRECTION('center_axis',(0.,1.,0.)) ;
#124966=DIRECTION('ref_axis',(0.,0.,1.)) ;
#124967=DIRECTION('',(-1.,0.,0.)) ;
#124968=DIRECTION('',(0.,0.,-1.)) ;
#124969=DIRECTION('',(1.,0.,7.01133629567814E-33)) ;
#124970=DIRECTION('',(0.,0.,1.)) ;
#124971=DIRECTION('center_axis',(0.,1.,0.)) ;
#124972=DIRECTION('ref_axis',(0.,0.,1.)) ;
#124973=DIRECTION('',(-1.,0.,7.01133629567814E-33)) ;
#124974=DIRECTION('',(0.,0.,-1.)) ;
#124975=DIRECTION('',(1.,0.,0.)) ;
#124976=DIRECTION('',(0.,0.,1.)) ;
#124977=DIRECTION('center_axis',(-1.,0.,0.)) ;
#124978=DIRECTION('ref_axis',(0.,0.,1.)) ;
#124979=DIRECTION('',(-1.,0.,0.)) ;
#124980=DIRECTION('center_axis',(-1.,0.,0.)) ;
#124981=DIRECTION('ref_axis',(0.,1.83291537084341E-15,-1.)) ;
#124982=DIRECTION('',(1.,0.,0.)) ;
#124983=DIRECTION('center_axis',(1.,0.,0.)) ;
#124984=DIRECTION('ref_axis',(0.,0.,-1.)) ;
#124985=DIRECTION('center_axis',(1.,0.,0.)) ;
#124986=DIRECTION('ref_axis',(0.,0.,-1.)) ;
#124987=DIRECTION('',(0.,0.,-1.)) ;
#124988=DIRECTION('center_axis',(-1.,0.,0.)) ;
#124989=DIRECTION('ref_axis',(0.,-5.43258597458929E-15,-1.)) ;
#124990=DIRECTION('',(0.,0.,-1.)) ;
#124991=DIRECTION('',(0.,1.,-8.9727076343628E-17)) ;
#124992=DIRECTION('',(0.,0.,1.)) ;
#124993=DIRECTION('',(0.,-1.,-8.9727076343628E-17)) ;
#124994=DIRECTION('center_axis',(0.,1.,0.)) ;
#124995=DIRECTION('ref_axis',(0.,0.,1.)) ;
#124996=DIRECTION('',(-1.,0.,0.)) ;
#124997=DIRECTION('',(0.,0.,-1.)) ;
#124998=DIRECTION('',(1.,0.,7.01133629567814E-33)) ;
#124999=DIRECTION('',(0.,0.,1.)) ;
#125000=DIRECTION('center_axis',(0.,1.,0.)) ;
#125001=DIRECTION('ref_axis',(0.,0.,1.)) ;
#125002=DIRECTION('',(-1.,0.,7.01133629567814E-33)) ;
#125003=DIRECTION('',(0.,0.,-1.)) ;
#125004=DIRECTION('',(1.,0.,0.)) ;
#125005=DIRECTION('',(0.,0.,1.)) ;
#125006=DIRECTION('center_axis',(-1.,0.,0.)) ;
#125007=DIRECTION('ref_axis',(0.,0.,1.)) ;
#125008=DIRECTION('',(-1.,0.,0.)) ;
#125009=DIRECTION('center_axis',(-1.,0.,0.)) ;
#125010=DIRECTION('ref_axis',(0.,0.,-1.)) ;
#125011=DIRECTION('',(1.,0.,0.)) ;
#125012=DIRECTION('center_axis',(1.,0.,0.)) ;
#125013=DIRECTION('ref_axis',(0.,0.,-1.)) ;
#125014=DIRECTION('center_axis',(1.,0.,0.)) ;
#125015=DIRECTION('ref_axis',(0.,0.,-1.)) ;
#125016=DIRECTION('',(0.,0.,-1.)) ;
#125017=DIRECTION('center_axis',(-1.,0.,0.)) ;
#125018=DIRECTION('ref_axis',(0.,-5.43258597458929E-15,-1.)) ;
#125019=DIRECTION('',(0.,0.,-1.)) ;
#125020=DIRECTION('',(0.,1.,-8.9727076343628E-17)) ;
#125021=DIRECTION('',(0.,0.,1.)) ;
#125022=DIRECTION('',(0.,-1.,-8.9727076343628E-17)) ;
#125023=DIRECTION('center_axis',(1.,0.,0.)) ;
#125024=DIRECTION('ref_axis',(0.,0.,-1.)) ;
#125025=DIRECTION('center_axis',(1.,0.,0.)) ;
#125026=DIRECTION('ref_axis',(0.,0.,-1.)) ;
#125027=DIRECTION('center_axis',(1.,0.,0.)) ;
#125028=DIRECTION('ref_axis',(0.,0.,-1.)) ;
#125029=DIRECTION('center_axis',(1.,0.,0.)) ;
#125030=DIRECTION('ref_axis',(0.,0.,-1.)) ;
#125031=DIRECTION('center_axis',(1.,0.,0.)) ;
#125032=DIRECTION('ref_axis',(0.,0.,-1.)) ;
#125033=DIRECTION('center_axis',(1.,0.,0.)) ;
#125034=DIRECTION('ref_axis',(0.,0.,-1.)) ;
#125035=DIRECTION('center_axis',(1.,0.,0.)) ;
#125036=DIRECTION('ref_axis',(0.,0.,-1.)) ;
#125037=DIRECTION('center_axis',(1.,0.,0.)) ;
#125038=DIRECTION('ref_axis',(0.,0.,-1.)) ;
#125039=DIRECTION('center_axis',(1.,0.,0.)) ;
#125040=DIRECTION('ref_axis',(0.,0.,-1.)) ;
#125041=DIRECTION('center_axis',(1.,-1.31418445149758E-16,-2.16840434497101E-16)) ;
#125042=DIRECTION('ref_axis',(-2.16840434497101E-16,0.,-1.)) ;
#125043=DIRECTION('',(2.16840434497101E-16,0.,1.)) ;
#125044=DIRECTION('',(1.31418445149758E-16,1.,0.)) ;
#125045=DIRECTION('',(-2.16840434497101E-16,-2.8496832747207E-32,-1.)) ;
#125046=DIRECTION('',(-1.31418445149758E-16,-1.,0.)) ;
#125047=DIRECTION('center_axis',(-2.16840434497101E-16,2.8496832747207E-32,
1.)) ;
#125048=DIRECTION('ref_axis',(1.,4.92915281362991E-64,2.16840434497101E-16)) ;
#125049=DIRECTION('',(1.,1.31418445149758E-16,2.16840434497101E-16)) ;
#125050=DIRECTION('',(-1.31418445149758E-16,-1.,0.)) ;
#125051=DIRECTION('',(-1.,0.,-2.16840434497101E-16)) ;
#125052=DIRECTION('',(1.31418445149758E-16,1.,0.)) ;
#125053=DIRECTION('center_axis',(-1.,1.31418445149758E-16,4.33680868994202E-16)) ;
#125054=DIRECTION('ref_axis',(4.33680868994202E-16,0.,1.)) ;
#125055=DIRECTION('',(-1.31418445149758E-16,-1.,0.)) ;
#125056=DIRECTION('',(-4.33680868994202E-16,0.,-1.)) ;
#125057=DIRECTION('',(1.31418445149758E-16,1.,0.)) ;
#125058=DIRECTION('',(4.33680868994202E-16,5.69936654944139E-32,1.)) ;
#125059=DIRECTION('center_axis',(-2.16840434497101E-16,2.8496832747207E-32,
-1.)) ;
#125060=DIRECTION('ref_axis',(-1.,-4.92915281362991E-64,2.16840434497101E-16)) ;
#125061=DIRECTION('',(1.,0.,-2.16840434497101E-16)) ;
#125062=DIRECTION('',(1.31418445149758E-16,1.,0.)) ;
#125063=DIRECTION('',(-1.,-1.31418445149758E-16,2.16840434497101E-16)) ;
#125064=DIRECTION('',(-1.31418445149758E-16,-1.,0.)) ;
#125065=DIRECTION('center_axis',(1.,-1.31418445149758E-16,-2.16840434497101E-16)) ;
#125066=DIRECTION('ref_axis',(-2.16840434497101E-16,0.,-1.)) ;
#125067=DIRECTION('',(2.16840434497101E-16,0.,1.)) ;
#125068=DIRECTION('',(1.31418445149758E-16,1.,0.)) ;
#125069=DIRECTION('',(-2.16840434497101E-16,-2.8496832747207E-32,-1.)) ;
#125070=DIRECTION('',(-1.31418445149758E-16,-1.,0.)) ;
#125071=DIRECTION('center_axis',(-2.16840434497101E-16,2.8496832747207E-32,
1.)) ;
#125072=DIRECTION('ref_axis',(1.,4.92915281362991E-64,2.16840434497101E-16)) ;
#125073=DIRECTION('',(1.,1.31418445149758E-16,2.16840434497101E-16)) ;
#125074=DIRECTION('',(-1.31418445149758E-16,-1.,0.)) ;
#125075=DIRECTION('',(-1.,0.,-2.16840434497101E-16)) ;
#125076=DIRECTION('',(1.31418445149758E-16,1.,0.)) ;
#125077=DIRECTION('center_axis',(-1.,1.31418445149758E-16,4.33680868994202E-16)) ;
#125078=DIRECTION('ref_axis',(4.33680868994202E-16,0.,1.)) ;
#125079=DIRECTION('',(-1.31418445149758E-16,-1.,0.)) ;
#125080=DIRECTION('',(-4.33680868994202E-16,0.,-1.)) ;
#125081=DIRECTION('',(1.31418445149758E-16,1.,0.)) ;
#125082=DIRECTION('',(4.33680868994202E-16,5.69936654944139E-32,1.)) ;
#125083=DIRECTION('center_axis',(-2.16840434497101E-16,2.8496832747207E-32,
-1.)) ;
#125084=DIRECTION('ref_axis',(-1.,-4.92915281362991E-64,2.16840434497101E-16)) ;
#125085=DIRECTION('',(1.,0.,-2.16840434497101E-16)) ;
#125086=DIRECTION('',(1.31418445149758E-16,1.,0.)) ;
#125087=DIRECTION('',(-1.,-1.31418445149758E-16,2.16840434497101E-16)) ;
#125088=DIRECTION('',(-1.31418445149758E-16,-1.,0.)) ;
#125089=DIRECTION('center_axis',(1.,-1.31418445149758E-16,-2.16840434497101E-16)) ;
#125090=DIRECTION('ref_axis',(-2.16840434497101E-16,0.,-1.)) ;
#125091=DIRECTION('',(2.16840434497101E-16,0.,1.)) ;
#125092=DIRECTION('',(1.31418445149758E-16,1.,0.)) ;
#125093=DIRECTION('',(-2.16840434497101E-16,-2.8496832747207E-32,-1.)) ;
#125094=DIRECTION('',(-1.31418445149758E-16,-1.,0.)) ;
#125095=DIRECTION('center_axis',(-2.16840434497101E-16,2.8496832747207E-32,
1.)) ;
#125096=DIRECTION('ref_axis',(1.,4.92915281362991E-64,2.16840434497101E-16)) ;
#125097=DIRECTION('',(1.,1.31418445149758E-16,2.16840434497101E-16)) ;
#125098=DIRECTION('',(-1.31418445149758E-16,-1.,0.)) ;
#125099=DIRECTION('',(-1.,0.,-2.16840434497101E-16)) ;
#125100=DIRECTION('',(1.31418445149758E-16,1.,0.)) ;
#125101=DIRECTION('center_axis',(-1.,1.31418445149758E-16,4.33680868994202E-16)) ;
#125102=DIRECTION('ref_axis',(4.33680868994202E-16,0.,1.)) ;
#125103=DIRECTION('',(-1.31418445149758E-16,-1.,0.)) ;
#125104=DIRECTION('',(-4.33680868994202E-16,0.,-1.)) ;
#125105=DIRECTION('',(1.31418445149758E-16,1.,0.)) ;
#125106=DIRECTION('',(4.33680868994202E-16,5.69936654944139E-32,1.)) ;
#125107=DIRECTION('center_axis',(-2.16840434497101E-16,2.8496832747207E-32,
-1.)) ;
#125108=DIRECTION('ref_axis',(-1.,-4.92915281362991E-64,2.16840434497101E-16)) ;
#125109=DIRECTION('',(1.,0.,-2.16840434497101E-16)) ;
#125110=DIRECTION('',(1.31418445149758E-16,1.,0.)) ;
#125111=DIRECTION('',(-1.,-1.31418445149758E-16,2.16840434497101E-16)) ;
#125112=DIRECTION('',(-1.31418445149758E-16,-1.,0.)) ;
#125113=DIRECTION('center_axis',(1.,-1.31418445149758E-16,-2.16840434497101E-16)) ;
#125114=DIRECTION('ref_axis',(-2.16840434497101E-16,0.,-1.)) ;
#125115=DIRECTION('',(2.16840434497101E-16,0.,1.)) ;
#125116=DIRECTION('',(1.31418445149758E-16,1.,0.)) ;
#125117=DIRECTION('',(-2.16840434497101E-16,-2.8496832747207E-32,-1.)) ;
#125118=DIRECTION('',(-1.31418445149758E-16,-1.,0.)) ;
#125119=DIRECTION('center_axis',(-2.16840434497101E-16,2.8496832747207E-32,
1.)) ;
#125120=DIRECTION('ref_axis',(1.,4.92915281362991E-64,2.16840434497101E-16)) ;
#125121=DIRECTION('',(1.,1.31418445149758E-16,2.16840434497101E-16)) ;
#125122=DIRECTION('',(-1.31418445149758E-16,-1.,0.)) ;
#125123=DIRECTION('',(-1.,0.,-2.16840434497101E-16)) ;
#125124=DIRECTION('',(1.31418445149758E-16,1.,0.)) ;
#125125=DIRECTION('center_axis',(-1.,1.31418445149758E-16,4.33680868994202E-16)) ;
#125126=DIRECTION('ref_axis',(4.33680868994202E-16,0.,1.)) ;
#125127=DIRECTION('',(-1.31418445149758E-16,-1.,0.)) ;
#125128=DIRECTION('',(-4.33680868994202E-16,0.,-1.)) ;
#125129=DIRECTION('',(1.31418445149758E-16,1.,0.)) ;
#125130=DIRECTION('',(4.33680868994202E-16,5.69936654944139E-32,1.)) ;
#125131=DIRECTION('center_axis',(-2.16840434497101E-16,2.8496832747207E-32,
-1.)) ;
#125132=DIRECTION('ref_axis',(-1.,-4.92915281362991E-64,2.16840434497101E-16)) ;
#125133=DIRECTION('',(1.,0.,-2.16840434497101E-16)) ;
#125134=DIRECTION('',(1.31418445149758E-16,1.,0.)) ;
#125135=DIRECTION('',(-1.,-1.31418445149758E-16,2.16840434497101E-16)) ;
#125136=DIRECTION('',(-1.31418445149758E-16,-1.,0.)) ;
#125137=DIRECTION('center_axis',(1.,-1.31418445149758E-16,-2.16840434497101E-16)) ;
#125138=DIRECTION('ref_axis',(-2.16840434497101E-16,0.,-1.)) ;
#125139=DIRECTION('',(2.16840434497101E-16,0.,1.)) ;
#125140=DIRECTION('',(1.31418445149758E-16,1.,0.)) ;
#125141=DIRECTION('',(-2.16840434497101E-16,-2.8496832747207E-32,-1.)) ;
#125142=DIRECTION('',(-1.31418445149758E-16,-1.,0.)) ;
#125143=DIRECTION('center_axis',(-2.16840434497101E-16,2.8496832747207E-32,
1.)) ;
#125144=DIRECTION('ref_axis',(1.,4.92915281362991E-64,2.16840434497101E-16)) ;
#125145=DIRECTION('',(1.,1.31418445149758E-16,2.16840434497101E-16)) ;
#125146=DIRECTION('',(-1.31418445149758E-16,-1.,0.)) ;
#125147=DIRECTION('',(-1.,0.,-2.16840434497101E-16)) ;
#125148=DIRECTION('',(1.31418445149758E-16,1.,0.)) ;
#125149=DIRECTION('center_axis',(-1.,1.31418445149758E-16,4.33680868994202E-16)) ;
#125150=DIRECTION('ref_axis',(4.33680868994202E-16,0.,1.)) ;
#125151=DIRECTION('',(-1.31418445149758E-16,-1.,0.)) ;
#125152=DIRECTION('',(-4.33680868994202E-16,0.,-1.)) ;
#125153=DIRECTION('',(1.31418445149758E-16,1.,0.)) ;
#125154=DIRECTION('',(4.33680868994202E-16,5.69936654944139E-32,1.)) ;
#125155=DIRECTION('center_axis',(-2.16840434497101E-16,2.8496832747207E-32,
-1.)) ;
#125156=DIRECTION('ref_axis',(-1.,-4.92915281362991E-64,2.16840434497101E-16)) ;
#125157=DIRECTION('',(1.,0.,-2.16840434497101E-16)) ;
#125158=DIRECTION('',(1.31418445149758E-16,1.,0.)) ;
#125159=DIRECTION('',(-1.,-1.31418445149758E-16,2.16840434497101E-16)) ;
#125160=DIRECTION('',(-1.31418445149758E-16,-1.,0.)) ;
#125161=DIRECTION('center_axis',(1.,-1.31418445149758E-16,-2.16840434497101E-16)) ;
#125162=DIRECTION('ref_axis',(-2.16840434497101E-16,0.,-1.)) ;
#125163=DIRECTION('',(2.16840434497101E-16,0.,1.)) ;
#125164=DIRECTION('',(1.31418445149758E-16,1.,0.)) ;
#125165=DIRECTION('',(-2.16840434497101E-16,-2.8496832747207E-32,-1.)) ;
#125166=DIRECTION('',(-1.31418445149758E-16,-1.,0.)) ;
#125167=DIRECTION('center_axis',(-2.16840434497101E-16,2.8496832747207E-32,
1.)) ;
#125168=DIRECTION('ref_axis',(1.,4.92915281362991E-64,2.16840434497101E-16)) ;
#125169=DIRECTION('',(1.,1.31418445149758E-16,2.16840434497101E-16)) ;
#125170=DIRECTION('',(-1.31418445149758E-16,-1.,0.)) ;
#125171=DIRECTION('',(-1.,0.,-2.16840434497101E-16)) ;
#125172=DIRECTION('',(1.31418445149758E-16,1.,0.)) ;
#125173=DIRECTION('center_axis',(-1.,1.31418445149758E-16,4.33680868994202E-16)) ;
#125174=DIRECTION('ref_axis',(4.33680868994202E-16,0.,1.)) ;
#125175=DIRECTION('',(-1.31418445149758E-16,-1.,0.)) ;
#125176=DIRECTION('',(-4.33680868994202E-16,0.,-1.)) ;
#125177=DIRECTION('',(1.31418445149758E-16,1.,0.)) ;
#125178=DIRECTION('',(4.33680868994202E-16,5.69936654944139E-32,1.)) ;
#125179=DIRECTION('center_axis',(-2.16840434497101E-16,2.8496832747207E-32,
-1.)) ;
#125180=DIRECTION('ref_axis',(-1.,-4.92915281362991E-64,2.16840434497101E-16)) ;
#125181=DIRECTION('',(1.,0.,-2.16840434497101E-16)) ;
#125182=DIRECTION('',(1.31418445149758E-16,1.,0.)) ;
#125183=DIRECTION('',(-1.,-1.31418445149758E-16,2.16840434497101E-16)) ;
#125184=DIRECTION('',(-1.31418445149758E-16,-1.,0.)) ;
#125185=DIRECTION('center_axis',(1.,-1.31418445149758E-16,-2.16840434497101E-16)) ;
#125186=DIRECTION('ref_axis',(-2.16840434497101E-16,0.,-1.)) ;
#125187=DIRECTION('',(2.16840434497101E-16,0.,1.)) ;
#125188=DIRECTION('',(1.31418445149758E-16,1.,0.)) ;
#125189=DIRECTION('',(-2.16840434497101E-16,-2.8496832747207E-32,-1.)) ;
#125190=DIRECTION('',(-1.31418445149758E-16,-1.,0.)) ;
#125191=DIRECTION('center_axis',(-2.16840434497101E-16,2.8496832747207E-32,
1.)) ;
#125192=DIRECTION('ref_axis',(1.,4.92915281362991E-64,2.16840434497101E-16)) ;
#125193=DIRECTION('',(1.,1.31418445149758E-16,2.16840434497101E-16)) ;
#125194=DIRECTION('',(-1.31418445149758E-16,-1.,0.)) ;
#125195=DIRECTION('',(-1.,0.,-2.16840434497101E-16)) ;
#125196=DIRECTION('',(1.31418445149758E-16,1.,0.)) ;
#125197=DIRECTION('center_axis',(-1.,1.31418445149758E-16,4.33680868994202E-16)) ;
#125198=DIRECTION('ref_axis',(4.33680868994202E-16,0.,1.)) ;
#125199=DIRECTION('',(-1.31418445149758E-16,-1.,0.)) ;
#125200=DIRECTION('',(-4.33680868994202E-16,0.,-1.)) ;
#125201=DIRECTION('',(1.31418445149758E-16,1.,0.)) ;
#125202=DIRECTION('',(4.33680868994202E-16,5.69936654944139E-32,1.)) ;
#125203=DIRECTION('center_axis',(-2.16840434497101E-16,2.8496832747207E-32,
-1.)) ;
#125204=DIRECTION('ref_axis',(-1.,-4.92915281362991E-64,2.16840434497101E-16)) ;
#125205=DIRECTION('',(1.,0.,-2.16840434497101E-16)) ;
#125206=DIRECTION('',(1.31418445149758E-16,1.,0.)) ;
#125207=DIRECTION('',(-1.,-1.31418445149758E-16,2.16840434497101E-16)) ;
#125208=DIRECTION('',(-1.31418445149758E-16,-1.,0.)) ;
#125209=DIRECTION('center_axis',(1.,-1.31418445149758E-16,-2.16840434497101E-16)) ;
#125210=DIRECTION('ref_axis',(-2.16840434497101E-16,0.,-1.)) ;
#125211=DIRECTION('',(2.16840434497101E-16,0.,1.)) ;
#125212=DIRECTION('',(1.31418445149758E-16,1.,0.)) ;
#125213=DIRECTION('',(-2.16840434497101E-16,-2.8496832747207E-32,-1.)) ;
#125214=DIRECTION('',(-1.31418445149758E-16,-1.,0.)) ;
#125215=DIRECTION('center_axis',(-2.16840434497101E-16,2.8496832747207E-32,
1.)) ;
#125216=DIRECTION('ref_axis',(1.,4.92915281362991E-64,2.16840434497101E-16)) ;
#125217=DIRECTION('',(1.,1.31418445149758E-16,2.16840434497101E-16)) ;
#125218=DIRECTION('',(-1.31418445149758E-16,-1.,0.)) ;
#125219=DIRECTION('',(-1.,0.,-2.16840434497101E-16)) ;
#125220=DIRECTION('',(1.31418445149758E-16,1.,0.)) ;
#125221=DIRECTION('center_axis',(-1.,1.31418445149758E-16,4.33680868994202E-16)) ;
#125222=DIRECTION('ref_axis',(4.33680868994202E-16,0.,1.)) ;
#125223=DIRECTION('',(-1.31418445149758E-16,-1.,0.)) ;
#125224=DIRECTION('',(-4.33680868994202E-16,0.,-1.)) ;
#125225=DIRECTION('',(1.31418445149758E-16,1.,0.)) ;
#125226=DIRECTION('',(4.33680868994202E-16,5.69936654944139E-32,1.)) ;
#125227=DIRECTION('center_axis',(-2.16840434497101E-16,2.8496832747207E-32,
-1.)) ;
#125228=DIRECTION('ref_axis',(-1.,-4.92915281362991E-64,2.16840434497101E-16)) ;
#125229=DIRECTION('',(1.,0.,-2.16840434497101E-16)) ;
#125230=DIRECTION('',(1.31418445149758E-16,1.,0.)) ;
#125231=DIRECTION('',(-1.,-1.31418445149758E-16,2.16840434497101E-16)) ;
#125232=DIRECTION('',(-1.31418445149758E-16,-1.,0.)) ;
#125233=DIRECTION('center_axis',(1.,-1.31418445149758E-16,-2.16840434497101E-16)) ;
#125234=DIRECTION('ref_axis',(-2.16840434497101E-16,0.,-1.)) ;
#125235=DIRECTION('',(2.16840434497101E-16,0.,1.)) ;
#125236=DIRECTION('',(1.31418445149758E-16,1.,0.)) ;
#125237=DIRECTION('',(-2.16840434497101E-16,-2.8496832747207E-32,-1.)) ;
#125238=DIRECTION('',(-1.31418445149758E-16,-1.,0.)) ;
#125239=DIRECTION('center_axis',(-2.16840434497101E-16,2.8496832747207E-32,
1.)) ;
#125240=DIRECTION('ref_axis',(1.,4.92915281362991E-64,2.16840434497101E-16)) ;
#125241=DIRECTION('',(1.,1.31418445149758E-16,2.16840434497101E-16)) ;
#125242=DIRECTION('',(-1.31418445149758E-16,-1.,0.)) ;
#125243=DIRECTION('',(-1.,0.,-2.16840434497101E-16)) ;
#125244=DIRECTION('',(1.31418445149758E-16,1.,0.)) ;
#125245=DIRECTION('center_axis',(-1.,1.31418445149758E-16,4.33680868994202E-16)) ;
#125246=DIRECTION('ref_axis',(4.33680868994202E-16,0.,1.)) ;
#125247=DIRECTION('',(-1.31418445149758E-16,-1.,0.)) ;
#125248=DIRECTION('',(-4.33680868994202E-16,0.,-1.)) ;
#125249=DIRECTION('',(1.31418445149758E-16,1.,0.)) ;
#125250=DIRECTION('',(4.33680868994202E-16,5.69936654944139E-32,1.)) ;
#125251=DIRECTION('center_axis',(-2.16840434497101E-16,2.8496832747207E-32,
-1.)) ;
#125252=DIRECTION('ref_axis',(-1.,-4.92915281362991E-64,2.16840434497101E-16)) ;
#125253=DIRECTION('',(1.,0.,-2.16840434497101E-16)) ;
#125254=DIRECTION('',(1.31418445149758E-16,1.,0.)) ;
#125255=DIRECTION('',(-1.,-1.31418445149758E-16,2.16840434497101E-16)) ;
#125256=DIRECTION('',(-1.31418445149758E-16,-1.,0.)) ;
#125257=DIRECTION('center_axis',(0.,1.,0.)) ;
#125258=DIRECTION('ref_axis',(0.,0.,1.)) ;
#125259=DIRECTION('',(4.33680868994202E-16,0.,1.)) ;
#125260=DIRECTION('',(1.,0.,2.16840434497101E-16)) ;
#125261=DIRECTION('',(-2.16840434497101E-16,0.,-1.)) ;
#125262=DIRECTION('',(-1.,0.,2.16840434497101E-16)) ;
#125263=DIRECTION('',(1.,0.,0.)) ;
#125264=DIRECTION('center_axis',(0.,-1.,0.)) ;
#125265=DIRECTION('ref_axis',(0.,0.,1.)) ;
#125266=DIRECTION('',(0.,0.,1.)) ;
#125267=DIRECTION('center_axis',(0.,-1.,0.)) ;
#125268=DIRECTION('ref_axis',(0.,0.,1.)) ;
#125269=DIRECTION('',(-1.,0.,0.)) ;
#125270=DIRECTION('center_axis',(0.,-1.,0.)) ;
#125271=DIRECTION('ref_axis',(0.,0.,1.)) ;
#125272=DIRECTION('',(0.,0.,-1.)) ;
#125273=DIRECTION('center_axis',(0.,-1.,0.)) ;
#125274=DIRECTION('ref_axis',(0.,0.,1.)) ;
#125275=DIRECTION('center_axis',(1.,0.,0.)) ;
#125276=DIRECTION('ref_axis',(0.,0.,-1.)) ;
#125277=DIRECTION('',(0.,0.,1.)) ;
#125278=DIRECTION('',(0.,-1.,0.)) ;
#125279=DIRECTION('',(0.,1.,0.)) ;
#125280=DIRECTION('center_axis',(0.,0.,1.)) ;
#125281=DIRECTION('ref_axis',(1.,0.,0.)) ;
#125282=DIRECTION('',(-1.,0.,0.)) ;
#125283=DIRECTION('',(0.,-1.,0.)) ;
#125284=DIRECTION('',(0.,1.,0.)) ;
#125285=DIRECTION('center_axis',(-1.,0.,0.)) ;
#125286=DIRECTION('ref_axis',(0.,0.,1.)) ;
#125287=DIRECTION('',(0.,1.,0.)) ;
#125288=DIRECTION('',(0.,0.,-1.)) ;
#125289=DIRECTION('',(0.,-1.,0.)) ;
#125290=DIRECTION('center_axis',(0.,0.,-1.)) ;
#125291=DIRECTION('ref_axis',(-1.,0.,0.)) ;
#125292=DIRECTION('',(1.,0.,0.)) ;
#125293=DIRECTION('',(0.,-1.,0.)) ;
#125294=DIRECTION('',(0.,1.,0.)) ;
#125295=DIRECTION('center_axis',(0.,1.,0.)) ;
#125296=DIRECTION('ref_axis',(0.,0.,1.)) ;
#125297=DIRECTION('',(4.33680868994202E-16,0.,1.)) ;
#125298=DIRECTION('',(1.,0.,2.16840434497101E-16)) ;
#125299=DIRECTION('',(-2.16840434497101E-16,0.,-1.)) ;
#125300=DIRECTION('',(-1.,0.,2.16840434497101E-16)) ;
#125301=DIRECTION('',(1.,0.,0.)) ;
#125302=DIRECTION('center_axis',(0.,-1.,0.)) ;
#125303=DIRECTION('ref_axis',(0.,0.,1.)) ;
#125304=DIRECTION('',(0.,0.,1.)) ;
#125305=DIRECTION('center_axis',(0.,-1.,0.)) ;
#125306=DIRECTION('ref_axis',(0.,0.,1.)) ;
#125307=DIRECTION('',(-1.,0.,0.)) ;
#125308=DIRECTION('center_axis',(0.,-1.,0.)) ;
#125309=DIRECTION('ref_axis',(0.,0.,1.)) ;
#125310=DIRECTION('',(0.,0.,-1.)) ;
#125311=DIRECTION('center_axis',(0.,-1.,0.)) ;
#125312=DIRECTION('ref_axis',(0.,0.,1.)) ;
#125313=DIRECTION('center_axis',(1.,0.,0.)) ;
#125314=DIRECTION('ref_axis',(0.,0.,-1.)) ;
#125315=DIRECTION('',(0.,0.,1.)) ;
#125316=DIRECTION('',(0.,-1.,0.)) ;
#125317=DIRECTION('',(0.,1.,0.)) ;
#125318=DIRECTION('center_axis',(0.,0.,1.)) ;
#125319=DIRECTION('ref_axis',(1.,0.,0.)) ;
#125320=DIRECTION('',(-1.,0.,0.)) ;
#125321=DIRECTION('',(0.,-1.,0.)) ;
#125322=DIRECTION('',(0.,1.,0.)) ;
#125323=DIRECTION('center_axis',(-1.,0.,0.)) ;
#125324=DIRECTION('ref_axis',(0.,0.,1.)) ;
#125325=DIRECTION('',(0.,1.,0.)) ;
#125326=DIRECTION('',(0.,0.,-1.)) ;
#125327=DIRECTION('',(0.,-1.,0.)) ;
#125328=DIRECTION('center_axis',(0.,0.,-1.)) ;
#125329=DIRECTION('ref_axis',(-1.,0.,0.)) ;
#125330=DIRECTION('',(1.,0.,0.)) ;
#125331=DIRECTION('',(0.,-1.,0.)) ;
#125332=DIRECTION('',(0.,1.,0.)) ;
#125333=DIRECTION('center_axis',(0.,1.,0.)) ;
#125334=DIRECTION('ref_axis',(0.,0.,1.)) ;
#125335=DIRECTION('',(4.33680868994202E-16,0.,1.)) ;
#125336=DIRECTION('',(1.,0.,2.16840434497101E-16)) ;
#125337=DIRECTION('',(-2.16840434497101E-16,0.,-1.)) ;
#125338=DIRECTION('',(-1.,0.,2.16840434497101E-16)) ;
#125339=DIRECTION('',(1.,0.,0.)) ;
#125340=DIRECTION('center_axis',(0.,-1.,0.)) ;
#125341=DIRECTION('ref_axis',(0.,0.,1.)) ;
#125342=DIRECTION('',(0.,0.,1.)) ;
#125343=DIRECTION('center_axis',(0.,-1.,0.)) ;
#125344=DIRECTION('ref_axis',(0.,0.,1.)) ;
#125345=DIRECTION('',(-1.,0.,0.)) ;
#125346=DIRECTION('center_axis',(0.,-1.,0.)) ;
#125347=DIRECTION('ref_axis',(0.,0.,1.)) ;
#125348=DIRECTION('',(0.,0.,-1.)) ;
#125349=DIRECTION('center_axis',(0.,-1.,0.)) ;
#125350=DIRECTION('ref_axis',(0.,0.,1.)) ;
#125351=DIRECTION('center_axis',(1.,0.,0.)) ;
#125352=DIRECTION('ref_axis',(0.,0.,-1.)) ;
#125353=DIRECTION('',(0.,0.,1.)) ;
#125354=DIRECTION('',(0.,-1.,0.)) ;
#125355=DIRECTION('',(0.,1.,0.)) ;
#125356=DIRECTION('center_axis',(0.,0.,1.)) ;
#125357=DIRECTION('ref_axis',(1.,0.,0.)) ;
#125358=DIRECTION('',(-1.,0.,0.)) ;
#125359=DIRECTION('',(0.,-1.,0.)) ;
#125360=DIRECTION('',(0.,1.,0.)) ;
#125361=DIRECTION('center_axis',(-1.,0.,0.)) ;
#125362=DIRECTION('ref_axis',(0.,0.,1.)) ;
#125363=DIRECTION('',(0.,1.,0.)) ;
#125364=DIRECTION('',(0.,0.,-1.)) ;
#125365=DIRECTION('',(0.,-1.,0.)) ;
#125366=DIRECTION('center_axis',(0.,0.,-1.)) ;
#125367=DIRECTION('ref_axis',(-1.,0.,0.)) ;
#125368=DIRECTION('',(1.,0.,0.)) ;
#125369=DIRECTION('',(0.,-1.,0.)) ;
#125370=DIRECTION('',(0.,1.,0.)) ;
#125371=DIRECTION('center_axis',(0.,1.,0.)) ;
#125372=DIRECTION('ref_axis',(0.,0.,1.)) ;
#125373=DIRECTION('',(4.33680868994202E-16,0.,1.)) ;
#125374=DIRECTION('',(1.,0.,2.16840434497101E-16)) ;
#125375=DIRECTION('',(-2.16840434497101E-16,0.,-1.)) ;
#125376=DIRECTION('',(-1.,0.,2.16840434497101E-16)) ;
#125377=DIRECTION('',(1.,0.,0.)) ;
#125378=DIRECTION('center_axis',(0.,-1.,0.)) ;
#125379=DIRECTION('ref_axis',(0.,0.,1.)) ;
#125380=DIRECTION('',(0.,0.,1.)) ;
#125381=DIRECTION('center_axis',(0.,-1.,0.)) ;
#125382=DIRECTION('ref_axis',(0.,0.,1.)) ;
#125383=DIRECTION('',(-1.,0.,0.)) ;
#125384=DIRECTION('center_axis',(0.,-1.,0.)) ;
#125385=DIRECTION('ref_axis',(0.,0.,1.)) ;
#125386=DIRECTION('',(0.,0.,-1.)) ;
#125387=DIRECTION('center_axis',(0.,-1.,0.)) ;
#125388=DIRECTION('ref_axis',(0.,0.,1.)) ;
#125389=DIRECTION('center_axis',(1.,0.,0.)) ;
#125390=DIRECTION('ref_axis',(0.,0.,-1.)) ;
#125391=DIRECTION('',(0.,0.,1.)) ;
#125392=DIRECTION('',(0.,-1.,0.)) ;
#125393=DIRECTION('',(0.,1.,0.)) ;
#125394=DIRECTION('center_axis',(0.,0.,1.)) ;
#125395=DIRECTION('ref_axis',(1.,0.,0.)) ;
#125396=DIRECTION('',(-1.,0.,0.)) ;
#125397=DIRECTION('',(0.,-1.,0.)) ;
#125398=DIRECTION('',(0.,1.,0.)) ;
#125399=DIRECTION('center_axis',(-1.,0.,0.)) ;
#125400=DIRECTION('ref_axis',(0.,0.,1.)) ;
#125401=DIRECTION('',(0.,1.,0.)) ;
#125402=DIRECTION('',(0.,0.,-1.)) ;
#125403=DIRECTION('',(0.,-1.,0.)) ;
#125404=DIRECTION('center_axis',(0.,0.,-1.)) ;
#125405=DIRECTION('ref_axis',(-1.,0.,0.)) ;
#125406=DIRECTION('',(1.,0.,0.)) ;
#125407=DIRECTION('',(0.,-1.,0.)) ;
#125408=DIRECTION('',(0.,1.,0.)) ;
#125409=DIRECTION('center_axis',(0.,1.,0.)) ;
#125410=DIRECTION('ref_axis',(0.,0.,1.)) ;
#125411=DIRECTION('',(4.33680868994202E-16,0.,1.)) ;
#125412=DIRECTION('',(1.,0.,2.16840434497101E-16)) ;
#125413=DIRECTION('',(-2.16840434497101E-16,0.,-1.)) ;
#125414=DIRECTION('',(-1.,0.,2.16840434497101E-16)) ;
#125415=DIRECTION('',(1.,0.,0.)) ;
#125416=DIRECTION('center_axis',(0.,-1.,0.)) ;
#125417=DIRECTION('ref_axis',(0.,0.,1.)) ;
#125418=DIRECTION('',(0.,0.,1.)) ;
#125419=DIRECTION('center_axis',(0.,-1.,0.)) ;
#125420=DIRECTION('ref_axis',(0.,0.,1.)) ;
#125421=DIRECTION('',(-1.,0.,0.)) ;
#125422=DIRECTION('center_axis',(0.,-1.,0.)) ;
#125423=DIRECTION('ref_axis',(0.,0.,1.)) ;
#125424=DIRECTION('',(0.,0.,-1.)) ;
#125425=DIRECTION('center_axis',(0.,-1.,0.)) ;
#125426=DIRECTION('ref_axis',(0.,0.,1.)) ;
#125427=DIRECTION('center_axis',(1.,0.,0.)) ;
#125428=DIRECTION('ref_axis',(0.,0.,-1.)) ;
#125429=DIRECTION('',(0.,0.,1.)) ;
#125430=DIRECTION('',(0.,-1.,0.)) ;
#125431=DIRECTION('',(0.,1.,0.)) ;
#125432=DIRECTION('center_axis',(0.,0.,1.)) ;
#125433=DIRECTION('ref_axis',(1.,0.,0.)) ;
#125434=DIRECTION('',(-1.,0.,0.)) ;
#125435=DIRECTION('',(0.,-1.,0.)) ;
#125436=DIRECTION('',(0.,1.,0.)) ;
#125437=DIRECTION('center_axis',(-1.,0.,0.)) ;
#125438=DIRECTION('ref_axis',(0.,0.,1.)) ;
#125439=DIRECTION('',(0.,1.,0.)) ;
#125440=DIRECTION('',(0.,0.,-1.)) ;
#125441=DIRECTION('',(0.,-1.,0.)) ;
#125442=DIRECTION('center_axis',(0.,0.,-1.)) ;
#125443=DIRECTION('ref_axis',(-1.,0.,0.)) ;
#125444=DIRECTION('',(1.,0.,0.)) ;
#125445=DIRECTION('',(0.,-1.,0.)) ;
#125446=DIRECTION('',(0.,1.,0.)) ;
#125447=DIRECTION('center_axis',(0.,1.,0.)) ;
#125448=DIRECTION('ref_axis',(0.,0.,1.)) ;
#125449=DIRECTION('',(4.33680868994202E-16,0.,1.)) ;
#125450=DIRECTION('',(1.,0.,2.16840434497101E-16)) ;
#125451=DIRECTION('',(-2.16840434497101E-16,0.,-1.)) ;
#125452=DIRECTION('',(-1.,0.,2.16840434497101E-16)) ;
#125453=DIRECTION('',(1.,0.,0.)) ;
#125454=DIRECTION('center_axis',(0.,-1.,0.)) ;
#125455=DIRECTION('ref_axis',(0.,0.,1.)) ;
#125456=DIRECTION('',(0.,0.,1.)) ;
#125457=DIRECTION('center_axis',(0.,-1.,0.)) ;
#125458=DIRECTION('ref_axis',(0.,0.,1.)) ;
#125459=DIRECTION('',(-1.,0.,0.)) ;
#125460=DIRECTION('center_axis',(0.,-1.,0.)) ;
#125461=DIRECTION('ref_axis',(0.,0.,1.)) ;
#125462=DIRECTION('',(0.,0.,-1.)) ;
#125463=DIRECTION('center_axis',(0.,-1.,0.)) ;
#125464=DIRECTION('ref_axis',(0.,0.,1.)) ;
#125465=DIRECTION('center_axis',(1.,0.,0.)) ;
#125466=DIRECTION('ref_axis',(0.,0.,-1.)) ;
#125467=DIRECTION('',(0.,0.,1.)) ;
#125468=DIRECTION('',(0.,-1.,0.)) ;
#125469=DIRECTION('',(0.,1.,0.)) ;
#125470=DIRECTION('center_axis',(0.,0.,1.)) ;
#125471=DIRECTION('ref_axis',(1.,0.,0.)) ;
#125472=DIRECTION('',(-1.,0.,0.)) ;
#125473=DIRECTION('',(0.,-1.,0.)) ;
#125474=DIRECTION('',(0.,1.,0.)) ;
#125475=DIRECTION('center_axis',(-1.,0.,0.)) ;
#125476=DIRECTION('ref_axis',(0.,0.,1.)) ;
#125477=DIRECTION('',(0.,1.,0.)) ;
#125478=DIRECTION('',(0.,0.,-1.)) ;
#125479=DIRECTION('',(0.,-1.,0.)) ;
#125480=DIRECTION('center_axis',(0.,0.,-1.)) ;
#125481=DIRECTION('ref_axis',(-1.,0.,0.)) ;
#125482=DIRECTION('',(1.,0.,0.)) ;
#125483=DIRECTION('',(0.,-1.,0.)) ;
#125484=DIRECTION('',(0.,1.,0.)) ;
#125485=DIRECTION('center_axis',(0.,1.,0.)) ;
#125486=DIRECTION('ref_axis',(0.,0.,1.)) ;
#125487=DIRECTION('',(4.33680868994202E-16,0.,1.)) ;
#125488=DIRECTION('',(1.,0.,2.16840434497101E-16)) ;
#125489=DIRECTION('',(-2.16840434497101E-16,0.,-1.)) ;
#125490=DIRECTION('',(-1.,0.,2.16840434497101E-16)) ;
#125491=DIRECTION('',(1.,0.,0.)) ;
#125492=DIRECTION('center_axis',(0.,-1.,0.)) ;
#125493=DIRECTION('ref_axis',(0.,0.,1.)) ;
#125494=DIRECTION('',(0.,0.,1.)) ;
#125495=DIRECTION('center_axis',(0.,-1.,0.)) ;
#125496=DIRECTION('ref_axis',(0.,0.,1.)) ;
#125497=DIRECTION('',(-1.,0.,0.)) ;
#125498=DIRECTION('center_axis',(0.,-1.,0.)) ;
#125499=DIRECTION('ref_axis',(0.,0.,1.)) ;
#125500=DIRECTION('',(0.,0.,-1.)) ;
#125501=DIRECTION('center_axis',(0.,-1.,0.)) ;
#125502=DIRECTION('ref_axis',(0.,0.,1.)) ;
#125503=DIRECTION('center_axis',(1.,0.,0.)) ;
#125504=DIRECTION('ref_axis',(0.,0.,-1.)) ;
#125505=DIRECTION('',(0.,0.,1.)) ;
#125506=DIRECTION('',(0.,-1.,0.)) ;
#125507=DIRECTION('',(0.,1.,0.)) ;
#125508=DIRECTION('center_axis',(0.,0.,1.)) ;
#125509=DIRECTION('ref_axis',(1.,0.,0.)) ;
#125510=DIRECTION('',(-1.,0.,0.)) ;
#125511=DIRECTION('',(0.,-1.,0.)) ;
#125512=DIRECTION('',(0.,1.,0.)) ;
#125513=DIRECTION('center_axis',(-1.,0.,0.)) ;
#125514=DIRECTION('ref_axis',(0.,0.,1.)) ;
#125515=DIRECTION('',(0.,1.,0.)) ;
#125516=DIRECTION('',(0.,0.,-1.)) ;
#125517=DIRECTION('',(0.,-1.,0.)) ;
#125518=DIRECTION('center_axis',(0.,0.,-1.)) ;
#125519=DIRECTION('ref_axis',(-1.,0.,0.)) ;
#125520=DIRECTION('',(1.,0.,0.)) ;
#125521=DIRECTION('',(0.,-1.,0.)) ;
#125522=DIRECTION('',(0.,1.,0.)) ;
#125523=DIRECTION('center_axis',(0.,1.,0.)) ;
#125524=DIRECTION('ref_axis',(0.,0.,1.)) ;
#125525=DIRECTION('',(4.33680868994202E-16,0.,1.)) ;
#125526=DIRECTION('',(1.,0.,2.16840434497101E-16)) ;
#125527=DIRECTION('',(-2.16840434497101E-16,0.,-1.)) ;
#125528=DIRECTION('',(-1.,0.,2.16840434497101E-16)) ;
#125529=DIRECTION('',(1.,0.,0.)) ;
#125530=DIRECTION('center_axis',(0.,-1.,0.)) ;
#125531=DIRECTION('ref_axis',(0.,0.,1.)) ;
#125532=DIRECTION('',(0.,0.,1.)) ;
#125533=DIRECTION('center_axis',(0.,-1.,0.)) ;
#125534=DIRECTION('ref_axis',(0.,0.,1.)) ;
#125535=DIRECTION('',(-1.,0.,0.)) ;
#125536=DIRECTION('center_axis',(0.,-1.,0.)) ;
#125537=DIRECTION('ref_axis',(0.,0.,1.)) ;
#125538=DIRECTION('',(0.,0.,-1.)) ;
#125539=DIRECTION('center_axis',(0.,-1.,0.)) ;
#125540=DIRECTION('ref_axis',(0.,0.,1.)) ;
#125541=DIRECTION('center_axis',(1.,0.,0.)) ;
#125542=DIRECTION('ref_axis',(0.,0.,-1.)) ;
#125543=DIRECTION('',(0.,0.,1.)) ;
#125544=DIRECTION('',(0.,-1.,0.)) ;
#125545=DIRECTION('',(0.,1.,0.)) ;
#125546=DIRECTION('center_axis',(0.,0.,1.)) ;
#125547=DIRECTION('ref_axis',(1.,0.,0.)) ;
#125548=DIRECTION('',(-1.,0.,0.)) ;
#125549=DIRECTION('',(0.,-1.,0.)) ;
#125550=DIRECTION('',(0.,1.,0.)) ;
#125551=DIRECTION('center_axis',(-1.,0.,0.)) ;
#125552=DIRECTION('ref_axis',(0.,0.,1.)) ;
#125553=DIRECTION('',(0.,1.,0.)) ;
#125554=DIRECTION('',(0.,0.,-1.)) ;
#125555=DIRECTION('',(0.,-1.,0.)) ;
#125556=DIRECTION('center_axis',(0.,0.,-1.)) ;
#125557=DIRECTION('ref_axis',(-1.,0.,0.)) ;
#125558=DIRECTION('',(1.,0.,0.)) ;
#125559=DIRECTION('',(0.,-1.,0.)) ;
#125560=DIRECTION('',(0.,1.,0.)) ;
#125561=DIRECTION('center_axis',(0.,1.,0.)) ;
#125562=DIRECTION('ref_axis',(0.,0.,1.)) ;
#125563=DIRECTION('',(4.33680868994202E-16,0.,1.)) ;
#125564=DIRECTION('',(1.,0.,2.16840434497101E-16)) ;
#125565=DIRECTION('',(-2.16840434497101E-16,0.,-1.)) ;
#125566=DIRECTION('',(-1.,0.,2.16840434497101E-16)) ;
#125567=DIRECTION('',(1.,0.,0.)) ;
#125568=DIRECTION('center_axis',(0.,-1.,0.)) ;
#125569=DIRECTION('ref_axis',(0.,0.,1.)) ;
#125570=DIRECTION('',(0.,0.,1.)) ;
#125571=DIRECTION('center_axis',(0.,-1.,0.)) ;
#125572=DIRECTION('ref_axis',(0.,0.,1.)) ;
#125573=DIRECTION('',(-1.,0.,0.)) ;
#125574=DIRECTION('center_axis',(0.,-1.,0.)) ;
#125575=DIRECTION('ref_axis',(0.,0.,1.)) ;
#125576=DIRECTION('',(0.,0.,-1.)) ;
#125577=DIRECTION('center_axis',(0.,-1.,0.)) ;
#125578=DIRECTION('ref_axis',(0.,0.,1.)) ;
#125579=DIRECTION('center_axis',(1.,0.,0.)) ;
#125580=DIRECTION('ref_axis',(0.,0.,-1.)) ;
#125581=DIRECTION('',(0.,0.,1.)) ;
#125582=DIRECTION('',(0.,-1.,0.)) ;
#125583=DIRECTION('',(0.,1.,0.)) ;
#125584=DIRECTION('center_axis',(0.,0.,1.)) ;
#125585=DIRECTION('ref_axis',(1.,0.,0.)) ;
#125586=DIRECTION('',(-1.,0.,0.)) ;
#125587=DIRECTION('',(0.,-1.,0.)) ;
#125588=DIRECTION('',(0.,1.,0.)) ;
#125589=DIRECTION('center_axis',(-1.,0.,0.)) ;
#125590=DIRECTION('ref_axis',(0.,0.,1.)) ;
#125591=DIRECTION('',(0.,1.,0.)) ;
#125592=DIRECTION('',(0.,0.,-1.)) ;
#125593=DIRECTION('',(0.,-1.,0.)) ;
#125594=DIRECTION('center_axis',(0.,0.,-1.)) ;
#125595=DIRECTION('ref_axis',(-1.,0.,0.)) ;
#125596=DIRECTION('',(1.,0.,0.)) ;
#125597=DIRECTION('',(0.,-1.,0.)) ;
#125598=DIRECTION('',(0.,1.,0.)) ;
#125599=DIRECTION('center_axis',(0.,1.,0.)) ;
#125600=DIRECTION('ref_axis',(0.,0.,1.)) ;
#125601=DIRECTION('',(-1.,0.,0.)) ;
#125602=DIRECTION('',(0.,0.,1.)) ;
#125603=DIRECTION('',(1.,0.,0.)) ;
#125604=DIRECTION('',(0.,0.,-1.)) ;
#125605=DIRECTION('center_axis',(0.,1.,0.)) ;
#125606=DIRECTION('ref_axis',(0.,0.,1.)) ;
#125607=DIRECTION('',(-1.,0.,0.)) ;
#125608=DIRECTION('',(0.,0.,1.)) ;
#125609=DIRECTION('',(1.,0.,0.)) ;
#125610=DIRECTION('',(0.,0.,-1.)) ;
#125611=DIRECTION('center_axis',(0.,1.,0.)) ;
#125612=DIRECTION('ref_axis',(0.,0.,1.)) ;
#125613=DIRECTION('',(-1.,0.,0.)) ;
#125614=DIRECTION('',(0.,0.,1.)) ;
#125615=DIRECTION('',(1.,0.,0.)) ;
#125616=DIRECTION('',(0.,0.,-1.)) ;
#125617=DIRECTION('center_axis',(0.,1.,0.)) ;
#125618=DIRECTION('ref_axis',(0.,0.,1.)) ;
#125619=DIRECTION('',(-1.,0.,0.)) ;
#125620=DIRECTION('',(0.,0.,1.)) ;
#125621=DIRECTION('',(1.,0.,0.)) ;
#125622=DIRECTION('',(0.,0.,-1.)) ;
#125623=DIRECTION('center_axis',(0.,1.,0.)) ;
#125624=DIRECTION('ref_axis',(0.,0.,1.)) ;
#125625=DIRECTION('',(-1.,0.,0.)) ;
#125626=DIRECTION('',(0.,0.,1.)) ;
#125627=DIRECTION('',(1.,0.,0.)) ;
#125628=DIRECTION('',(0.,0.,-1.)) ;
#125629=DIRECTION('center_axis',(0.,1.,0.)) ;
#125630=DIRECTION('ref_axis',(0.,0.,1.)) ;
#125631=DIRECTION('',(-1.,0.,0.)) ;
#125632=DIRECTION('',(0.,0.,1.)) ;
#125633=DIRECTION('',(1.,0.,0.)) ;
#125634=DIRECTION('',(0.,0.,-1.)) ;
#125635=DIRECTION('center_axis',(0.,1.,0.)) ;
#125636=DIRECTION('ref_axis',(0.,0.,1.)) ;
#125637=DIRECTION('',(-1.,0.,0.)) ;
#125638=DIRECTION('',(0.,0.,1.)) ;
#125639=DIRECTION('',(1.,0.,0.)) ;
#125640=DIRECTION('',(0.,0.,-1.)) ;
#125641=DIRECTION('center_axis',(0.,1.,0.)) ;
#125642=DIRECTION('ref_axis',(0.,0.,1.)) ;
#125643=DIRECTION('',(-1.,0.,0.)) ;
#125644=DIRECTION('',(0.,0.,1.)) ;
#125645=DIRECTION('',(1.,0.,0.)) ;
#125646=DIRECTION('',(0.,0.,-1.)) ;
#125647=DIRECTION('center_axis',(0.,1.,0.)) ;
#125648=DIRECTION('ref_axis',(0.,0.,1.)) ;
#125649=DIRECTION('',(-1.,0.,0.)) ;
#125650=DIRECTION('',(0.,0.,1.)) ;
#125651=DIRECTION('',(1.,0.,0.)) ;
#125652=DIRECTION('',(0.,0.,-1.)) ;
#125653=DIRECTION('center_axis',(1.31418445149758E-16,1.,0.)) ;
#125654=DIRECTION('ref_axis',(-1.,1.31418445149758E-16,0.)) ;
#125655=DIRECTION('',(-0.422618261740697,5.55398348498559E-17,0.906307787036651)) ;
#125656=DIRECTION('center_axis',(1.31418445149758E-16,1.,0.)) ;
#125657=DIRECTION('ref_axis',(-1.,1.31418445149758E-16,0.)) ;
#125658=DIRECTION('',(-0.422618261740697,5.55398348498559E-17,0.906307787036651)) ;
#125659=DIRECTION('center_axis',(1.31418445149758E-16,1.,0.)) ;
#125660=DIRECTION('ref_axis',(-1.,1.31418445149758E-16,0.)) ;
#125661=DIRECTION('',(-0.422618261740697,5.55398348498559E-17,0.906307787036651)) ;
#125662=DIRECTION('center_axis',(1.31418445149758E-16,1.,0.)) ;
#125663=DIRECTION('ref_axis',(-1.,1.31418445149758E-16,0.)) ;
#125664=DIRECTION('',(-0.422618261740697,5.55398348498559E-17,0.906307787036651)) ;
#125665=DIRECTION('center_axis',(1.31418445149758E-16,1.,0.)) ;
#125666=DIRECTION('ref_axis',(-1.,1.31418445149758E-16,0.)) ;
#125667=DIRECTION('',(-0.422618261740697,5.55398348498559E-17,0.906307787036651)) ;
#125668=DIRECTION('center_axis',(1.31418445149758E-16,1.,0.)) ;
#125669=DIRECTION('ref_axis',(-1.,1.31418445149758E-16,0.)) ;
#125670=DIRECTION('',(-0.422618261740697,5.55398348498559E-17,0.906307787036651)) ;
#125671=DIRECTION('center_axis',(1.31418445149758E-16,1.,0.)) ;
#125672=DIRECTION('ref_axis',(-1.,1.31418445149758E-16,0.)) ;
#125673=DIRECTION('',(-0.422618261740697,5.55398348498559E-17,0.906307787036651)) ;
#125674=DIRECTION('center_axis',(1.31418445149758E-16,1.,0.)) ;
#125675=DIRECTION('ref_axis',(-1.,1.31418445149758E-16,0.)) ;
#125676=DIRECTION('',(-0.422618261740697,5.55398348498559E-17,0.906307787036651)) ;
#125677=DIRECTION('center_axis',(1.31418445149758E-16,1.,0.)) ;
#125678=DIRECTION('ref_axis',(-1.,1.31418445149758E-16,0.)) ;
#125679=DIRECTION('',(-0.422618261740697,5.55398348498559E-17,0.906307787036651)) ;
#125680=DIRECTION('center_axis',(0.906307787036651,-1.19105560199475E-16,
0.422618261740697)) ;
#125681=DIRECTION('ref_axis',(0.422618261740697,-9.57222084411175E-33,-0.906307787036651)) ;
#125682=DIRECTION('',(0.422618261740697,-5.55398348498559E-17,-0.906307787036651)) ;
#125683=DIRECTION('',(-0.422618261740697,5.55398348498559E-17,0.906307787036651)) ;
#125684=DIRECTION('center_axis',(-0.906307787036651,1.19105560199475E-16,
-0.422618261740697)) ;
#125685=DIRECTION('ref_axis',(-0.422618261740697,9.57222084411175E-33,0.906307787036651)) ;
#125686=DIRECTION('',(0.422618261740697,-5.55398348498559E-17,-0.906307787036651)) ;
#125687=DIRECTION('',(-0.422618261740697,5.55398348498559E-17,0.906307787036651)) ;
#125688=DIRECTION('center_axis',(1.31418445149758E-16,1.,0.)) ;
#125689=DIRECTION('ref_axis',(-1.,1.31418445149758E-16,0.)) ;
#125690=DIRECTION('',(0.422618261740697,-5.55398348498559E-17,-0.906307787036651)) ;
#125691=DIRECTION('',(-0.422618261740697,5.55398348498559E-17,0.906307787036651)) ;
#125692=DIRECTION('center_axis',(0.906307787036651,-1.19105560199475E-16,
0.422618261740697)) ;
#125693=DIRECTION('ref_axis',(0.422618261740697,-9.57222084411175E-33,-0.906307787036651)) ;
#125694=DIRECTION('',(0.422618261740697,-5.55398348498559E-17,-0.906307787036651)) ;
#125695=DIRECTION('',(-0.422618261740697,5.55398348498559E-17,0.906307787036651)) ;
#125696=DIRECTION('center_axis',(-0.906307787036651,1.19105560199475E-16,
-0.422618261740697)) ;
#125697=DIRECTION('ref_axis',(-0.422618261740697,9.57222084411175E-33,0.906307787036651)) ;
#125698=DIRECTION('',(0.422618261740697,-5.55398348498559E-17,-0.906307787036651)) ;
#125699=DIRECTION('',(-0.422618261740697,5.55398348498559E-17,0.906307787036651)) ;
#125700=DIRECTION('center_axis',(1.31418445149758E-16,1.,0.)) ;
#125701=DIRECTION('ref_axis',(-1.,1.31418445149758E-16,0.)) ;
#125702=DIRECTION('',(0.422618261740697,-5.55398348498559E-17,-0.906307787036651)) ;
#125703=DIRECTION('',(-0.422618261740697,5.55398348498559E-17,0.906307787036651)) ;
#125704=DIRECTION('center_axis',(0.906307787036651,-1.19105560199475E-16,
0.422618261740697)) ;
#125705=DIRECTION('ref_axis',(0.422618261740697,-9.57222084411175E-33,-0.906307787036651)) ;
#125706=DIRECTION('',(0.422618261740697,-5.55398348498559E-17,-0.906307787036651)) ;
#125707=DIRECTION('',(-0.422618261740697,5.55398348498559E-17,0.906307787036651)) ;
#125708=DIRECTION('center_axis',(-0.906307787036651,1.19105560199475E-16,
-0.422618261740697)) ;
#125709=DIRECTION('ref_axis',(-0.422618261740697,9.57222084411175E-33,0.906307787036651)) ;
#125710=DIRECTION('',(0.422618261740697,-5.55398348498559E-17,-0.906307787036651)) ;
#125711=DIRECTION('',(-0.422618261740697,5.55398348498559E-17,0.906307787036651)) ;
#125712=DIRECTION('center_axis',(1.31418445149758E-16,1.,0.)) ;
#125713=DIRECTION('ref_axis',(-1.,1.31418445149758E-16,0.)) ;
#125714=DIRECTION('',(0.422618261740697,-5.55398348498559E-17,-0.906307787036651)) ;
#125715=DIRECTION('',(-0.422618261740697,5.55398348498559E-17,0.906307787036651)) ;
#125716=DIRECTION('center_axis',(0.906307787036651,-1.19105560199475E-16,
0.422618261740697)) ;
#125717=DIRECTION('ref_axis',(0.422618261740697,-9.57222084411175E-33,-0.906307787036651)) ;
#125718=DIRECTION('',(0.422618261740697,-5.55398348498559E-17,-0.906307787036651)) ;
#125719=DIRECTION('',(-0.422618261740697,5.55398348498559E-17,0.906307787036651)) ;
#125720=DIRECTION('center_axis',(-0.906307787036651,1.19105560199475E-16,
-0.422618261740697)) ;
#125721=DIRECTION('ref_axis',(-0.422618261740697,9.57222084411175E-33,0.906307787036651)) ;
#125722=DIRECTION('',(0.422618261740697,-5.55398348498559E-17,-0.906307787036651)) ;
#125723=DIRECTION('',(-0.422618261740697,5.55398348498559E-17,0.906307787036651)) ;
#125724=DIRECTION('center_axis',(1.31418445149758E-16,1.,0.)) ;
#125725=DIRECTION('ref_axis',(-1.,1.31418445149758E-16,0.)) ;
#125726=DIRECTION('',(0.422618261740697,-5.55398348498559E-17,-0.906307787036651)) ;
#125727=DIRECTION('',(-0.422618261740697,5.55398348498559E-17,0.906307787036651)) ;
#125728=DIRECTION('center_axis',(0.906307787036651,-1.19105560199475E-16,
0.422618261740697)) ;
#125729=DIRECTION('ref_axis',(0.422618261740697,-9.57222084411175E-33,-0.906307787036651)) ;
#125730=DIRECTION('',(0.422618261740697,-5.55398348498559E-17,-0.906307787036651)) ;
#125731=DIRECTION('',(-0.422618261740697,5.55398348498559E-17,0.906307787036651)) ;
#125732=DIRECTION('center_axis',(-0.906307787036651,1.19105560199475E-16,
-0.422618261740697)) ;
#125733=DIRECTION('ref_axis',(-0.422618261740697,9.57222084411175E-33,0.906307787036651)) ;
#125734=DIRECTION('',(0.422618261740697,-5.55398348498559E-17,-0.906307787036651)) ;
#125735=DIRECTION('',(-0.422618261740697,5.55398348498559E-17,0.906307787036651)) ;
#125736=DIRECTION('center_axis',(1.31418445149758E-16,1.,0.)) ;
#125737=DIRECTION('ref_axis',(-1.,1.31418445149758E-16,0.)) ;
#125738=DIRECTION('',(0.422618261740697,-5.55398348498559E-17,-0.906307787036651)) ;
#125739=DIRECTION('',(-0.422618261740697,5.55398348498559E-17,0.906307787036651)) ;
#125740=DIRECTION('center_axis',(0.906307787036651,-1.19105560199475E-16,
0.422618261740697)) ;
#125741=DIRECTION('ref_axis',(0.422618261740697,-9.57222084411175E-33,-0.906307787036651)) ;
#125742=DIRECTION('',(0.422618261740697,-5.55398348498559E-17,-0.906307787036651)) ;
#125743=DIRECTION('',(-0.422618261740697,5.55398348498559E-17,0.906307787036651)) ;
#125744=DIRECTION('center_axis',(-0.906307787036651,1.19105560199475E-16,
-0.422618261740697)) ;
#125745=DIRECTION('ref_axis',(-0.422618261740697,9.57222084411175E-33,0.906307787036651)) ;
#125746=DIRECTION('',(0.422618261740697,-5.55398348498559E-17,-0.906307787036651)) ;
#125747=DIRECTION('',(-0.422618261740697,5.55398348498559E-17,0.906307787036651)) ;
#125748=DIRECTION('center_axis',(1.31418445149758E-16,1.,0.)) ;
#125749=DIRECTION('ref_axis',(-1.,1.31418445149758E-16,0.)) ;
#125750=DIRECTION('',(0.422618261740697,-5.55398348498559E-17,-0.906307787036651)) ;
#125751=DIRECTION('',(-0.422618261740697,5.55398348498559E-17,0.906307787036651)) ;
#125752=DIRECTION('center_axis',(0.906307787036651,-1.19105560199475E-16,
0.422618261740697)) ;
#125753=DIRECTION('ref_axis',(0.422618261740697,-9.57222084411175E-33,-0.906307787036651)) ;
#125754=DIRECTION('',(0.422618261740697,-5.55398348498559E-17,-0.906307787036651)) ;
#125755=DIRECTION('',(-0.422618261740697,5.55398348498559E-17,0.906307787036651)) ;
#125756=DIRECTION('center_axis',(-0.906307787036651,1.19105560199475E-16,
-0.422618261740697)) ;
#125757=DIRECTION('ref_axis',(-0.422618261740697,9.57222084411175E-33,0.906307787036651)) ;
#125758=DIRECTION('',(0.422618261740697,-5.55398348498559E-17,-0.906307787036651)) ;
#125759=DIRECTION('',(-0.422618261740697,5.55398348498559E-17,0.906307787036651)) ;
#125760=DIRECTION('center_axis',(1.31418445149758E-16,1.,0.)) ;
#125761=DIRECTION('ref_axis',(-1.,1.31418445149758E-16,0.)) ;
#125762=DIRECTION('',(0.422618261740697,-5.55398348498559E-17,-0.906307787036651)) ;
#125763=DIRECTION('',(-0.422618261740697,5.55398348498559E-17,0.906307787036651)) ;
#125764=DIRECTION('center_axis',(0.906307787036651,-1.19105560199475E-16,
0.422618261740697)) ;
#125765=DIRECTION('ref_axis',(0.422618261740697,-9.57222084411175E-33,-0.906307787036651)) ;
#125766=DIRECTION('',(0.422618261740697,-5.55398348498559E-17,-0.906307787036651)) ;
#125767=DIRECTION('',(-0.422618261740697,5.55398348498559E-17,0.906307787036651)) ;
#125768=DIRECTION('center_axis',(-0.906307787036651,1.19105560199475E-16,
-0.422618261740697)) ;
#125769=DIRECTION('ref_axis',(-0.422618261740697,9.57222084411175E-33,0.906307787036651)) ;
#125770=DIRECTION('',(0.422618261740697,-5.55398348498559E-17,-0.906307787036651)) ;
#125771=DIRECTION('',(-0.422618261740697,5.55398348498559E-17,0.906307787036651)) ;
#125772=DIRECTION('center_axis',(1.31418445149758E-16,1.,0.)) ;
#125773=DIRECTION('ref_axis',(-1.,1.31418445149758E-16,0.)) ;
#125774=DIRECTION('',(0.422618261740697,-5.55398348498559E-17,-0.906307787036651)) ;
#125775=DIRECTION('',(-0.422618261740697,5.55398348498559E-17,0.906307787036651)) ;
#125776=DIRECTION('center_axis',(0.906307787036651,-1.19105560199475E-16,
0.422618261740697)) ;
#125777=DIRECTION('ref_axis',(0.422618261740697,-9.57222084411175E-33,-0.906307787036651)) ;
#125778=DIRECTION('',(0.422618261740697,-5.55398348498559E-17,-0.906307787036651)) ;
#125779=DIRECTION('',(-0.422618261740697,5.55398348498559E-17,0.906307787036651)) ;
#125780=DIRECTION('center_axis',(-0.906307787036651,1.19105560199475E-16,
-0.422618261740697)) ;
#125781=DIRECTION('ref_axis',(-0.422618261740697,9.57222084411175E-33,0.906307787036651)) ;
#125782=DIRECTION('',(0.422618261740697,-5.55398348498559E-17,-0.906307787036651)) ;
#125783=DIRECTION('',(-0.422618261740697,5.55398348498559E-17,0.906307787036651)) ;
#125784=DIRECTION('center_axis',(1.31418445149758E-16,1.,0.)) ;
#125785=DIRECTION('ref_axis',(-1.,1.31418445149758E-16,0.)) ;
#125786=DIRECTION('',(0.422618261740697,-5.55398348498559E-17,-0.906307787036651)) ;
#125787=DIRECTION('',(-0.422618261740697,5.55398348498559E-17,0.906307787036651)) ;
#125788=DIRECTION('center_axis',(0.,-1.,0.)) ;
#125789=DIRECTION('ref_axis',(0.,0.,-1.)) ;
#125790=DIRECTION('',(0.,-1.,0.)) ;
#125791=DIRECTION('center_axis',(0.,1.,0.)) ;
#125792=DIRECTION('ref_axis',(5.20417042793045E-14,0.,-1.)) ;
#125793=DIRECTION('',(0.,-1.,0.)) ;
#125794=DIRECTION('center_axis',(0.,-1.,0.)) ;
#125795=DIRECTION('ref_axis',(0.,0.,-1.)) ;
#125796=DIRECTION('center_axis',(0.,0.,1.)) ;
#125797=DIRECTION('ref_axis',(1.,0.,0.)) ;
#125798=DIRECTION('',(-1.,0.,0.)) ;
#125799=DIRECTION('',(0.,-1.,0.)) ;
#125800=DIRECTION('',(1.,0.,0.)) ;
#125801=DIRECTION('center_axis',(0.,-1.,0.)) ;
#125802=DIRECTION('ref_axis',(0.,0.,-1.)) ;
#125803=DIRECTION('center_axis',(0.,1.,0.)) ;
#125804=DIRECTION('ref_axis',(0.,0.,-1.)) ;
#125805=DIRECTION('',(0.,-1.,0.)) ;
#125806=DIRECTION('center_axis',(0.,-1.,0.)) ;
#125807=DIRECTION('ref_axis',(0.,0.,-1.)) ;
#125808=DIRECTION('center_axis',(1.,0.,0.)) ;
#125809=DIRECTION('ref_axis',(0.,0.,-1.)) ;
#125810=DIRECTION('',(0.,0.,1.)) ;
#125811=DIRECTION('',(0.,-1.,0.)) ;
#125812=DIRECTION('',(0.,0.,-1.)) ;
#125813=DIRECTION('center_axis',(0.,-1.,0.)) ;
#125814=DIRECTION('ref_axis',(0.,0.,-1.)) ;
#125815=DIRECTION('center_axis',(0.,1.,0.)) ;
#125816=DIRECTION('ref_axis',(0.,0.,-1.)) ;
#125817=DIRECTION('',(0.,-1.,0.)) ;
#125818=DIRECTION('center_axis',(0.,-1.,0.)) ;
#125819=DIRECTION('ref_axis',(0.,0.,-1.)) ;
#125820=DIRECTION('center_axis',(0.,0.,-1.)) ;
#125821=DIRECTION('ref_axis',(-1.,0.,0.)) ;
#125822=DIRECTION('',(1.,0.,0.)) ;
#125823=DIRECTION('',(0.,-1.,0.)) ;
#125824=DIRECTION('',(-1.,0.,0.)) ;
#125825=DIRECTION('center_axis',(0.,-1.,0.)) ;
#125826=DIRECTION('ref_axis',(0.,0.,-1.)) ;
#125827=DIRECTION('center_axis',(0.,1.,0.)) ;
#125828=DIRECTION('ref_axis',(0.,0.,-1.)) ;
#125829=DIRECTION('',(0.,-1.,0.)) ;
#125830=DIRECTION('center_axis',(0.,-1.,0.)) ;
#125831=DIRECTION('ref_axis',(0.,0.,-1.)) ;
#125832=DIRECTION('center_axis',(-1.,0.,0.)) ;
#125833=DIRECTION('ref_axis',(0.,0.,1.)) ;
#125834=DIRECTION('',(0.,0.,1.)) ;
#125835=DIRECTION('',(0.,0.,-1.)) ;
#125836=DIRECTION('center_axis',(0.,-1.,0.)) ;
#125837=DIRECTION('ref_axis',(0.,0.,-1.)) ;
#125838=DIRECTION('',(1.,0.,0.)) ;
#125839=DIRECTION('',(0.,0.,-1.)) ;
#125840=DIRECTION('',(-1.,0.,0.)) ;
#125841=DIRECTION('',(0.,0.,1.)) ;
#125842=DIRECTION('center_axis',(0.,-1.,0.)) ;
#125843=DIRECTION('ref_axis',(0.,0.,-1.)) ;
#125844=DIRECTION('',(0.,-1.,0.)) ;
#125845=DIRECTION('center_axis',(0.,1.,0.)) ;
#125846=DIRECTION('ref_axis',(5.20417042793045E-14,0.,-1.)) ;
#125847=DIRECTION('',(0.,-1.,0.)) ;
#125848=DIRECTION('center_axis',(0.,-1.,0.)) ;
#125849=DIRECTION('ref_axis',(0.,0.,-1.)) ;
#125850=DIRECTION('center_axis',(0.,0.,1.)) ;
#125851=DIRECTION('ref_axis',(1.,0.,0.)) ;
#125852=DIRECTION('',(-1.,0.,0.)) ;
#125853=DIRECTION('',(0.,-1.,0.)) ;
#125854=DIRECTION('',(1.,0.,0.)) ;
#125855=DIRECTION('center_axis',(0.,-1.,0.)) ;
#125856=DIRECTION('ref_axis',(0.,0.,-1.)) ;
#125857=DIRECTION('center_axis',(0.,1.,0.)) ;
#125858=DIRECTION('ref_axis',(0.,0.,-1.)) ;
#125859=DIRECTION('',(0.,-1.,0.)) ;
#125860=DIRECTION('center_axis',(0.,-1.,0.)) ;
#125861=DIRECTION('ref_axis',(0.,0.,-1.)) ;
#125862=DIRECTION('center_axis',(1.,0.,0.)) ;
#125863=DIRECTION('ref_axis',(0.,0.,-1.)) ;
#125864=DIRECTION('',(0.,0.,1.)) ;
#125865=DIRECTION('',(0.,-1.,0.)) ;
#125866=DIRECTION('',(0.,0.,-1.)) ;
#125867=DIRECTION('center_axis',(0.,-1.,0.)) ;
#125868=DIRECTION('ref_axis',(0.,0.,-1.)) ;
#125869=DIRECTION('center_axis',(0.,1.,0.)) ;
#125870=DIRECTION('ref_axis',(0.,0.,-1.)) ;
#125871=DIRECTION('',(0.,-1.,0.)) ;
#125872=DIRECTION('center_axis',(0.,-1.,0.)) ;
#125873=DIRECTION('ref_axis',(0.,0.,-1.)) ;
#125874=DIRECTION('center_axis',(0.,0.,-1.)) ;
#125875=DIRECTION('ref_axis',(-1.,0.,0.)) ;
#125876=DIRECTION('',(1.,0.,0.)) ;
#125877=DIRECTION('',(0.,-1.,0.)) ;
#125878=DIRECTION('',(-1.,0.,0.)) ;
#125879=DIRECTION('center_axis',(0.,-1.,0.)) ;
#125880=DIRECTION('ref_axis',(0.,0.,-1.)) ;
#125881=DIRECTION('center_axis',(0.,1.,0.)) ;
#125882=DIRECTION('ref_axis',(0.,0.,-1.)) ;
#125883=DIRECTION('',(0.,-1.,0.)) ;
#125884=DIRECTION('center_axis',(0.,-1.,0.)) ;
#125885=DIRECTION('ref_axis',(0.,0.,-1.)) ;
#125886=DIRECTION('center_axis',(-1.,0.,0.)) ;
#125887=DIRECTION('ref_axis',(0.,0.,1.)) ;
#125888=DIRECTION('',(0.,0.,1.)) ;
#125889=DIRECTION('',(0.,0.,-1.)) ;
#125890=DIRECTION('center_axis',(0.,-1.,0.)) ;
#125891=DIRECTION('ref_axis',(0.,0.,-1.)) ;
#125892=DIRECTION('',(1.,0.,0.)) ;
#125893=DIRECTION('',(0.,0.,-1.)) ;
#125894=DIRECTION('',(-1.,0.,0.)) ;
#125895=DIRECTION('',(0.,0.,1.)) ;
#125896=DIRECTION('center_axis',(0.,-1.,0.)) ;
#125897=DIRECTION('ref_axis',(0.,0.,-1.)) ;
#125898=DIRECTION('',(0.,-1.,0.)) ;
#125899=DIRECTION('center_axis',(0.,1.,0.)) ;
#125900=DIRECTION('ref_axis',(5.20417042793045E-14,0.,-1.)) ;
#125901=DIRECTION('',(0.,-1.,0.)) ;
#125902=DIRECTION('center_axis',(0.,-1.,0.)) ;
#125903=DIRECTION('ref_axis',(0.,0.,-1.)) ;
#125904=DIRECTION('center_axis',(0.,0.,1.)) ;
#125905=DIRECTION('ref_axis',(1.,0.,0.)) ;
#125906=DIRECTION('',(-1.,0.,0.)) ;
#125907=DIRECTION('',(0.,-1.,0.)) ;
#125908=DIRECTION('',(1.,0.,0.)) ;
#125909=DIRECTION('center_axis',(0.,-1.,0.)) ;
#125910=DIRECTION('ref_axis',(0.,0.,-1.)) ;
#125911=DIRECTION('center_axis',(0.,1.,0.)) ;
#125912=DIRECTION('ref_axis',(0.,0.,-1.)) ;
#125913=DIRECTION('',(0.,-1.,0.)) ;
#125914=DIRECTION('center_axis',(0.,-1.,0.)) ;
#125915=DIRECTION('ref_axis',(0.,0.,-1.)) ;
#125916=DIRECTION('center_axis',(1.,0.,0.)) ;
#125917=DIRECTION('ref_axis',(0.,0.,-1.)) ;
#125918=DIRECTION('',(0.,0.,1.)) ;
#125919=DIRECTION('',(0.,-1.,0.)) ;
#125920=DIRECTION('',(0.,0.,-1.)) ;
#125921=DIRECTION('center_axis',(0.,-1.,0.)) ;
#125922=DIRECTION('ref_axis',(0.,0.,-1.)) ;
#125923=DIRECTION('center_axis',(0.,1.,0.)) ;
#125924=DIRECTION('ref_axis',(0.,0.,-1.)) ;
#125925=DIRECTION('',(0.,-1.,0.)) ;
#125926=DIRECTION('center_axis',(0.,-1.,0.)) ;
#125927=DIRECTION('ref_axis',(0.,0.,-1.)) ;
#125928=DIRECTION('center_axis',(0.,0.,-1.)) ;
#125929=DIRECTION('ref_axis',(-1.,0.,0.)) ;
#125930=DIRECTION('',(1.,0.,0.)) ;
#125931=DIRECTION('',(0.,-1.,0.)) ;
#125932=DIRECTION('',(-1.,0.,0.)) ;
#125933=DIRECTION('center_axis',(0.,-1.,0.)) ;
#125934=DIRECTION('ref_axis',(0.,0.,-1.)) ;
#125935=DIRECTION('center_axis',(0.,1.,0.)) ;
#125936=DIRECTION('ref_axis',(0.,0.,-1.)) ;
#125937=DIRECTION('',(0.,-1.,0.)) ;
#125938=DIRECTION('center_axis',(0.,-1.,0.)) ;
#125939=DIRECTION('ref_axis',(0.,0.,-1.)) ;
#125940=DIRECTION('center_axis',(-1.,0.,0.)) ;
#125941=DIRECTION('ref_axis',(0.,0.,1.)) ;
#125942=DIRECTION('',(0.,0.,1.)) ;
#125943=DIRECTION('',(0.,0.,-1.)) ;
#125944=DIRECTION('center_axis',(0.,-1.,0.)) ;
#125945=DIRECTION('ref_axis',(0.,0.,-1.)) ;
#125946=DIRECTION('',(1.,0.,0.)) ;
#125947=DIRECTION('',(0.,0.,-1.)) ;
#125948=DIRECTION('',(-1.,0.,0.)) ;
#125949=DIRECTION('',(0.,0.,1.)) ;
#125950=DIRECTION('center_axis',(0.,-1.,0.)) ;
#125951=DIRECTION('ref_axis',(0.,0.,-1.)) ;
#125952=DIRECTION('',(0.,-1.,0.)) ;
#125953=DIRECTION('center_axis',(0.,1.,0.)) ;
#125954=DIRECTION('ref_axis',(5.20417042793045E-14,0.,-1.)) ;
#125955=DIRECTION('',(0.,-1.,0.)) ;
#125956=DIRECTION('center_axis',(0.,-1.,0.)) ;
#125957=DIRECTION('ref_axis',(0.,0.,-1.)) ;
#125958=DIRECTION('center_axis',(0.,0.,1.)) ;
#125959=DIRECTION('ref_axis',(1.,0.,0.)) ;
#125960=DIRECTION('',(-1.,0.,0.)) ;
#125961=DIRECTION('',(0.,-1.,0.)) ;
#125962=DIRECTION('',(1.,0.,0.)) ;
#125963=DIRECTION('center_axis',(0.,-1.,0.)) ;
#125964=DIRECTION('ref_axis',(0.,0.,-1.)) ;
#125965=DIRECTION('center_axis',(0.,1.,0.)) ;
#125966=DIRECTION('ref_axis',(0.,0.,-1.)) ;
#125967=DIRECTION('',(0.,-1.,0.)) ;
#125968=DIRECTION('center_axis',(0.,-1.,0.)) ;
#125969=DIRECTION('ref_axis',(0.,0.,-1.)) ;
#125970=DIRECTION('center_axis',(1.,0.,0.)) ;
#125971=DIRECTION('ref_axis',(0.,0.,-1.)) ;
#125972=DIRECTION('',(0.,0.,1.)) ;
#125973=DIRECTION('',(0.,-1.,0.)) ;
#125974=DIRECTION('',(0.,0.,-1.)) ;
#125975=DIRECTION('center_axis',(0.,-1.,0.)) ;
#125976=DIRECTION('ref_axis',(0.,0.,-1.)) ;
#125977=DIRECTION('center_axis',(0.,1.,0.)) ;
#125978=DIRECTION('ref_axis',(0.,0.,-1.)) ;
#125979=DIRECTION('',(0.,-1.,0.)) ;
#125980=DIRECTION('center_axis',(0.,-1.,0.)) ;
#125981=DIRECTION('ref_axis',(0.,0.,-1.)) ;
#125982=DIRECTION('center_axis',(0.,0.,-1.)) ;
#125983=DIRECTION('ref_axis',(-1.,0.,0.)) ;
#125984=DIRECTION('',(1.,0.,0.)) ;
#125985=DIRECTION('',(0.,-1.,0.)) ;
#125986=DIRECTION('',(-1.,0.,0.)) ;
#125987=DIRECTION('center_axis',(0.,-1.,0.)) ;
#125988=DIRECTION('ref_axis',(0.,0.,-1.)) ;
#125989=DIRECTION('center_axis',(0.,1.,0.)) ;
#125990=DIRECTION('ref_axis',(0.,0.,-1.)) ;
#125991=DIRECTION('',(0.,-1.,0.)) ;
#125992=DIRECTION('center_axis',(0.,-1.,0.)) ;
#125993=DIRECTION('ref_axis',(0.,0.,-1.)) ;
#125994=DIRECTION('center_axis',(-1.,0.,0.)) ;
#125995=DIRECTION('ref_axis',(0.,0.,1.)) ;
#125996=DIRECTION('',(0.,0.,1.)) ;
#125997=DIRECTION('',(0.,0.,-1.)) ;
#125998=DIRECTION('center_axis',(0.,-1.,0.)) ;
#125999=DIRECTION('ref_axis',(0.,0.,-1.)) ;
#126000=DIRECTION('',(1.,0.,0.)) ;
#126001=DIRECTION('',(0.,0.,-1.)) ;
#126002=DIRECTION('',(-1.,0.,0.)) ;
#126003=DIRECTION('',(0.,0.,1.)) ;
#126004=DIRECTION('center_axis',(0.,-1.,0.)) ;
#126005=DIRECTION('ref_axis',(0.,0.,-1.)) ;
#126006=DIRECTION('',(0.,-1.,0.)) ;
#126007=DIRECTION('center_axis',(0.,1.,0.)) ;
#126008=DIRECTION('ref_axis',(5.20417042793045E-14,0.,-1.)) ;
#126009=DIRECTION('',(0.,-1.,0.)) ;
#126010=DIRECTION('center_axis',(0.,-1.,0.)) ;
#126011=DIRECTION('ref_axis',(0.,0.,-1.)) ;
#126012=DIRECTION('center_axis',(0.,0.,1.)) ;
#126013=DIRECTION('ref_axis',(1.,0.,0.)) ;
#126014=DIRECTION('',(-1.,0.,0.)) ;
#126015=DIRECTION('',(0.,-1.,0.)) ;
#126016=DIRECTION('',(1.,0.,0.)) ;
#126017=DIRECTION('center_axis',(0.,-1.,0.)) ;
#126018=DIRECTION('ref_axis',(0.,0.,-1.)) ;
#126019=DIRECTION('center_axis',(0.,1.,0.)) ;
#126020=DIRECTION('ref_axis',(0.,0.,-1.)) ;
#126021=DIRECTION('',(0.,-1.,0.)) ;
#126022=DIRECTION('center_axis',(0.,-1.,0.)) ;
#126023=DIRECTION('ref_axis',(0.,0.,-1.)) ;
#126024=DIRECTION('center_axis',(1.,0.,0.)) ;
#126025=DIRECTION('ref_axis',(0.,0.,-1.)) ;
#126026=DIRECTION('',(0.,0.,1.)) ;
#126027=DIRECTION('',(0.,-1.,0.)) ;
#126028=DIRECTION('',(0.,0.,-1.)) ;
#126029=DIRECTION('center_axis',(0.,-1.,0.)) ;
#126030=DIRECTION('ref_axis',(0.,0.,-1.)) ;
#126031=DIRECTION('center_axis',(0.,1.,0.)) ;
#126032=DIRECTION('ref_axis',(0.,0.,-1.)) ;
#126033=DIRECTION('',(0.,-1.,0.)) ;
#126034=DIRECTION('center_axis',(0.,-1.,0.)) ;
#126035=DIRECTION('ref_axis',(0.,0.,-1.)) ;
#126036=DIRECTION('center_axis',(0.,0.,-1.)) ;
#126037=DIRECTION('ref_axis',(-1.,0.,0.)) ;
#126038=DIRECTION('',(1.,0.,0.)) ;
#126039=DIRECTION('',(0.,-1.,0.)) ;
#126040=DIRECTION('',(-1.,0.,0.)) ;
#126041=DIRECTION('center_axis',(0.,-1.,0.)) ;
#126042=DIRECTION('ref_axis',(0.,0.,-1.)) ;
#126043=DIRECTION('center_axis',(0.,1.,0.)) ;
#126044=DIRECTION('ref_axis',(0.,0.,-1.)) ;
#126045=DIRECTION('',(0.,-1.,0.)) ;
#126046=DIRECTION('center_axis',(0.,-1.,0.)) ;
#126047=DIRECTION('ref_axis',(0.,0.,-1.)) ;
#126048=DIRECTION('center_axis',(-1.,0.,0.)) ;
#126049=DIRECTION('ref_axis',(0.,0.,1.)) ;
#126050=DIRECTION('',(0.,0.,1.)) ;
#126051=DIRECTION('',(0.,0.,-1.)) ;
#126052=DIRECTION('center_axis',(0.,-1.,0.)) ;
#126053=DIRECTION('ref_axis',(0.,0.,-1.)) ;
#126054=DIRECTION('',(1.,0.,0.)) ;
#126055=DIRECTION('',(0.,0.,-1.)) ;
#126056=DIRECTION('',(-1.,0.,0.)) ;
#126057=DIRECTION('',(0.,0.,1.)) ;
#126058=DIRECTION('center_axis',(0.,-1.,0.)) ;
#126059=DIRECTION('ref_axis',(0.,0.,-1.)) ;
#126060=DIRECTION('',(0.,-1.,0.)) ;
#126061=DIRECTION('center_axis',(0.,1.,0.)) ;
#126062=DIRECTION('ref_axis',(5.20417042793045E-14,0.,-1.)) ;
#126063=DIRECTION('',(0.,-1.,0.)) ;
#126064=DIRECTION('center_axis',(0.,-1.,0.)) ;
#126065=DIRECTION('ref_axis',(0.,0.,-1.)) ;
#126066=DIRECTION('center_axis',(0.,0.,1.)) ;
#126067=DIRECTION('ref_axis',(1.,0.,0.)) ;
#126068=DIRECTION('',(-1.,0.,0.)) ;
#126069=DIRECTION('',(0.,-1.,0.)) ;
#126070=DIRECTION('',(1.,0.,0.)) ;
#126071=DIRECTION('center_axis',(0.,-1.,0.)) ;
#126072=DIRECTION('ref_axis',(0.,0.,-1.)) ;
#126073=DIRECTION('center_axis',(0.,1.,0.)) ;
#126074=DIRECTION('ref_axis',(0.,0.,-1.)) ;
#126075=DIRECTION('',(0.,-1.,0.)) ;
#126076=DIRECTION('center_axis',(0.,-1.,0.)) ;
#126077=DIRECTION('ref_axis',(0.,0.,-1.)) ;
#126078=DIRECTION('center_axis',(1.,0.,0.)) ;
#126079=DIRECTION('ref_axis',(0.,0.,-1.)) ;
#126080=DIRECTION('',(0.,0.,1.)) ;
#126081=DIRECTION('',(0.,-1.,0.)) ;
#126082=DIRECTION('',(0.,0.,-1.)) ;
#126083=DIRECTION('center_axis',(0.,-1.,0.)) ;
#126084=DIRECTION('ref_axis',(0.,0.,-1.)) ;
#126085=DIRECTION('center_axis',(0.,1.,0.)) ;
#126086=DIRECTION('ref_axis',(0.,0.,-1.)) ;
#126087=DIRECTION('',(0.,-1.,0.)) ;
#126088=DIRECTION('center_axis',(0.,-1.,0.)) ;
#126089=DIRECTION('ref_axis',(0.,0.,-1.)) ;
#126090=DIRECTION('center_axis',(0.,0.,-1.)) ;
#126091=DIRECTION('ref_axis',(-1.,0.,0.)) ;
#126092=DIRECTION('',(1.,0.,0.)) ;
#126093=DIRECTION('',(0.,-1.,0.)) ;
#126094=DIRECTION('',(-1.,0.,0.)) ;
#126095=DIRECTION('center_axis',(0.,-1.,0.)) ;
#126096=DIRECTION('ref_axis',(0.,0.,-1.)) ;
#126097=DIRECTION('center_axis',(0.,1.,0.)) ;
#126098=DIRECTION('ref_axis',(0.,0.,-1.)) ;
#126099=DIRECTION('',(0.,-1.,0.)) ;
#126100=DIRECTION('center_axis',(0.,-1.,0.)) ;
#126101=DIRECTION('ref_axis',(0.,0.,-1.)) ;
#126102=DIRECTION('center_axis',(-1.,0.,0.)) ;
#126103=DIRECTION('ref_axis',(0.,0.,1.)) ;
#126104=DIRECTION('',(0.,0.,1.)) ;
#126105=DIRECTION('',(0.,0.,-1.)) ;
#126106=DIRECTION('center_axis',(0.,-1.,0.)) ;
#126107=DIRECTION('ref_axis',(0.,0.,-1.)) ;
#126108=DIRECTION('',(1.,0.,0.)) ;
#126109=DIRECTION('',(0.,0.,-1.)) ;
#126110=DIRECTION('',(-1.,0.,0.)) ;
#126111=DIRECTION('',(0.,0.,1.)) ;
#126112=DIRECTION('center_axis',(0.,-1.,0.)) ;
#126113=DIRECTION('ref_axis',(0.,0.,-1.)) ;
#126114=DIRECTION('',(0.,-1.,0.)) ;
#126115=DIRECTION('center_axis',(0.,1.,0.)) ;
#126116=DIRECTION('ref_axis',(5.20417042793045E-14,0.,-1.)) ;
#126117=DIRECTION('',(0.,-1.,0.)) ;
#126118=DIRECTION('center_axis',(0.,-1.,0.)) ;
#126119=DIRECTION('ref_axis',(0.,0.,-1.)) ;
#126120=DIRECTION('center_axis',(0.,0.,1.)) ;
#126121=DIRECTION('ref_axis',(1.,0.,0.)) ;
#126122=DIRECTION('',(-1.,0.,0.)) ;
#126123=DIRECTION('',(0.,-1.,0.)) ;
#126124=DIRECTION('',(1.,0.,0.)) ;
#126125=DIRECTION('center_axis',(0.,-1.,0.)) ;
#126126=DIRECTION('ref_axis',(0.,0.,-1.)) ;
#126127=DIRECTION('center_axis',(0.,1.,0.)) ;
#126128=DIRECTION('ref_axis',(0.,0.,-1.)) ;
#126129=DIRECTION('',(0.,-1.,0.)) ;
#126130=DIRECTION('center_axis',(0.,-1.,0.)) ;
#126131=DIRECTION('ref_axis',(0.,0.,-1.)) ;
#126132=DIRECTION('center_axis',(1.,0.,0.)) ;
#126133=DIRECTION('ref_axis',(0.,0.,-1.)) ;
#126134=DIRECTION('',(0.,0.,1.)) ;
#126135=DIRECTION('',(0.,-1.,0.)) ;
#126136=DIRECTION('',(0.,0.,-1.)) ;
#126137=DIRECTION('center_axis',(0.,-1.,0.)) ;
#126138=DIRECTION('ref_axis',(0.,0.,-1.)) ;
#126139=DIRECTION('center_axis',(0.,1.,0.)) ;
#126140=DIRECTION('ref_axis',(0.,0.,-1.)) ;
#126141=DIRECTION('',(0.,-1.,0.)) ;
#126142=DIRECTION('center_axis',(0.,-1.,0.)) ;
#126143=DIRECTION('ref_axis',(0.,0.,-1.)) ;
#126144=DIRECTION('center_axis',(0.,0.,-1.)) ;
#126145=DIRECTION('ref_axis',(-1.,0.,0.)) ;
#126146=DIRECTION('',(1.,0.,0.)) ;
#126147=DIRECTION('',(0.,-1.,0.)) ;
#126148=DIRECTION('',(-1.,0.,0.)) ;
#126149=DIRECTION('center_axis',(0.,-1.,0.)) ;
#126150=DIRECTION('ref_axis',(0.,0.,-1.)) ;
#126151=DIRECTION('center_axis',(0.,1.,0.)) ;
#126152=DIRECTION('ref_axis',(0.,0.,-1.)) ;
#126153=DIRECTION('',(0.,-1.,0.)) ;
#126154=DIRECTION('center_axis',(0.,-1.,0.)) ;
#126155=DIRECTION('ref_axis',(0.,0.,-1.)) ;
#126156=DIRECTION('center_axis',(-1.,0.,0.)) ;
#126157=DIRECTION('ref_axis',(0.,0.,1.)) ;
#126158=DIRECTION('',(0.,0.,1.)) ;
#126159=DIRECTION('',(0.,0.,-1.)) ;
#126160=DIRECTION('center_axis',(0.,-1.,0.)) ;
#126161=DIRECTION('ref_axis',(0.,0.,-1.)) ;
#126162=DIRECTION('',(1.,0.,0.)) ;
#126163=DIRECTION('',(0.,0.,-1.)) ;
#126164=DIRECTION('',(-1.,0.,0.)) ;
#126165=DIRECTION('',(0.,0.,1.)) ;
#126166=DIRECTION('center_axis',(0.,-1.,0.)) ;
#126167=DIRECTION('ref_axis',(0.,0.,-1.)) ;
#126168=DIRECTION('',(0.,-1.,0.)) ;
#126169=DIRECTION('center_axis',(0.,1.,0.)) ;
#126170=DIRECTION('ref_axis',(5.20417042793045E-14,0.,-1.)) ;
#126171=DIRECTION('',(0.,-1.,0.)) ;
#126172=DIRECTION('center_axis',(0.,-1.,0.)) ;
#126173=DIRECTION('ref_axis',(0.,0.,-1.)) ;
#126174=DIRECTION('center_axis',(0.,0.,1.)) ;
#126175=DIRECTION('ref_axis',(1.,0.,0.)) ;
#126176=DIRECTION('',(-1.,0.,0.)) ;
#126177=DIRECTION('',(0.,-1.,0.)) ;
#126178=DIRECTION('',(1.,0.,0.)) ;
#126179=DIRECTION('center_axis',(0.,-1.,0.)) ;
#126180=DIRECTION('ref_axis',(0.,0.,-1.)) ;
#126181=DIRECTION('center_axis',(0.,1.,0.)) ;
#126182=DIRECTION('ref_axis',(0.,0.,-1.)) ;
#126183=DIRECTION('',(0.,-1.,0.)) ;
#126184=DIRECTION('center_axis',(0.,-1.,0.)) ;
#126185=DIRECTION('ref_axis',(0.,0.,-1.)) ;
#126186=DIRECTION('center_axis',(1.,0.,0.)) ;
#126187=DIRECTION('ref_axis',(0.,0.,-1.)) ;
#126188=DIRECTION('',(0.,0.,1.)) ;
#126189=DIRECTION('',(0.,-1.,0.)) ;
#126190=DIRECTION('',(0.,0.,-1.)) ;
#126191=DIRECTION('center_axis',(0.,-1.,0.)) ;
#126192=DIRECTION('ref_axis',(0.,0.,-1.)) ;
#126193=DIRECTION('center_axis',(0.,1.,0.)) ;
#126194=DIRECTION('ref_axis',(0.,0.,-1.)) ;
#126195=DIRECTION('',(0.,-1.,0.)) ;
#126196=DIRECTION('center_axis',(0.,-1.,0.)) ;
#126197=DIRECTION('ref_axis',(0.,0.,-1.)) ;
#126198=DIRECTION('center_axis',(0.,0.,-1.)) ;
#126199=DIRECTION('ref_axis',(-1.,0.,0.)) ;
#126200=DIRECTION('',(1.,0.,0.)) ;
#126201=DIRECTION('',(0.,-1.,0.)) ;
#126202=DIRECTION('',(-1.,0.,0.)) ;
#126203=DIRECTION('center_axis',(0.,-1.,0.)) ;
#126204=DIRECTION('ref_axis',(0.,0.,-1.)) ;
#126205=DIRECTION('center_axis',(0.,1.,0.)) ;
#126206=DIRECTION('ref_axis',(0.,0.,-1.)) ;
#126207=DIRECTION('',(0.,-1.,0.)) ;
#126208=DIRECTION('center_axis',(0.,-1.,0.)) ;
#126209=DIRECTION('ref_axis',(0.,0.,-1.)) ;
#126210=DIRECTION('center_axis',(-1.,0.,0.)) ;
#126211=DIRECTION('ref_axis',(0.,0.,1.)) ;
#126212=DIRECTION('',(0.,0.,1.)) ;
#126213=DIRECTION('',(0.,0.,-1.)) ;
#126214=DIRECTION('center_axis',(0.,-1.,0.)) ;
#126215=DIRECTION('ref_axis',(0.,0.,-1.)) ;
#126216=DIRECTION('',(1.,0.,0.)) ;
#126217=DIRECTION('',(0.,0.,-1.)) ;
#126218=DIRECTION('',(-1.,0.,0.)) ;
#126219=DIRECTION('',(0.,0.,1.)) ;
#126220=DIRECTION('center_axis',(0.,-1.,0.)) ;
#126221=DIRECTION('ref_axis',(0.,0.,-1.)) ;
#126222=DIRECTION('',(0.,-1.,0.)) ;
#126223=DIRECTION('center_axis',(0.,1.,0.)) ;
#126224=DIRECTION('ref_axis',(5.20417042793027E-14,0.,-1.)) ;
#126225=DIRECTION('',(0.,-1.,0.)) ;
#126226=DIRECTION('center_axis',(0.,-1.,0.)) ;
#126227=DIRECTION('ref_axis',(0.,0.,-1.)) ;
#126228=DIRECTION('center_axis',(0.,0.,1.)) ;
#126229=DIRECTION('ref_axis',(1.,0.,0.)) ;
#126230=DIRECTION('',(-1.,0.,0.)) ;
#126231=DIRECTION('',(0.,-1.,0.)) ;
#126232=DIRECTION('',(1.,0.,0.)) ;
#126233=DIRECTION('center_axis',(0.,-1.,0.)) ;
#126234=DIRECTION('ref_axis',(0.,0.,-1.)) ;
#126235=DIRECTION('center_axis',(0.,1.,0.)) ;
#126236=DIRECTION('ref_axis',(0.,0.,-1.)) ;
#126237=DIRECTION('',(0.,-1.,0.)) ;
#126238=DIRECTION('center_axis',(0.,-1.,0.)) ;
#126239=DIRECTION('ref_axis',(0.,0.,-1.)) ;
#126240=DIRECTION('center_axis',(1.,0.,0.)) ;
#126241=DIRECTION('ref_axis',(0.,0.,-1.)) ;
#126242=DIRECTION('',(0.,0.,1.)) ;
#126243=DIRECTION('',(0.,-1.,0.)) ;
#126244=DIRECTION('',(0.,0.,-1.)) ;
#126245=DIRECTION('center_axis',(0.,-1.,0.)) ;
#126246=DIRECTION('ref_axis',(0.,0.,-1.)) ;
#126247=DIRECTION('center_axis',(0.,1.,0.)) ;
#126248=DIRECTION('ref_axis',(0.,0.,-1.)) ;
#126249=DIRECTION('',(0.,-1.,0.)) ;
#126250=DIRECTION('center_axis',(0.,-1.,0.)) ;
#126251=DIRECTION('ref_axis',(0.,0.,-1.)) ;
#126252=DIRECTION('center_axis',(0.,0.,-1.)) ;
#126253=DIRECTION('ref_axis',(-1.,0.,0.)) ;
#126254=DIRECTION('',(1.,0.,0.)) ;
#126255=DIRECTION('',(0.,-1.,0.)) ;
#126256=DIRECTION('',(-1.,0.,0.)) ;
#126257=DIRECTION('center_axis',(0.,-1.,0.)) ;
#126258=DIRECTION('ref_axis',(0.,0.,-1.)) ;
#126259=DIRECTION('center_axis',(0.,1.,0.)) ;
#126260=DIRECTION('ref_axis',(0.,0.,-1.)) ;
#126261=DIRECTION('',(0.,-1.,0.)) ;
#126262=DIRECTION('center_axis',(0.,-1.,0.)) ;
#126263=DIRECTION('ref_axis',(0.,0.,-1.)) ;
#126264=DIRECTION('center_axis',(-1.,0.,0.)) ;
#126265=DIRECTION('ref_axis',(0.,0.,1.)) ;
#126266=DIRECTION('',(0.,0.,1.)) ;
#126267=DIRECTION('',(0.,0.,-1.)) ;
#126268=DIRECTION('center_axis',(0.,-1.,0.)) ;
#126269=DIRECTION('ref_axis',(0.,0.,-1.)) ;
#126270=DIRECTION('',(1.,0.,0.)) ;
#126271=DIRECTION('',(0.,0.,-1.)) ;
#126272=DIRECTION('',(-1.,0.,0.)) ;
#126273=DIRECTION('',(0.,0.,1.)) ;
#126274=DIRECTION('center_axis',(0.,1.,0.)) ;
#126275=DIRECTION('ref_axis',(1.,0.,0.)) ;
#126276=DIRECTION('center_axis',(-1.73472347597682E-14,0.,-1.)) ;
#126277=DIRECTION('ref_axis',(1.,0.,-1.73472347597682E-14)) ;
#126278=DIRECTION('center_axis',(0.,0.514231796959119,0.857651245551591)) ;
#126279=DIRECTION('ref_axis',(0.,0.857651245551591,-0.514231796959119)) ;
#126280=DIRECTION('center_axis',(-1.,0.,0.)) ;
#126281=DIRECTION('ref_axis',(0.,0.,-1.)) ;
#126282=DIRECTION('center_axis',(1.,0.,0.)) ;
#126283=DIRECTION('ref_axis',(0.,0.,-1.)) ;
#126284=DIRECTION('center_axis',(-2.15682522756814E-14,-0.514231796959101,
0.857651245551602)) ;
#126285=DIRECTION('ref_axis',(-4.48628358333197E-30,-0.857651245551602,
-0.514231796959101)) ;
#126286=DIRECTION('center_axis',(-1.,0.,0.)) ;
#126287=DIRECTION('ref_axis',(0.,0.,1.)) ;
#126288=DIRECTION('center_axis',(-1.,0.,0.)) ;
#126289=DIRECTION('ref_axis',(0.,0.,-1.)) ;
#126290=DIRECTION('center_axis',(0.,0.,1.)) ;
#126291=DIRECTION('ref_axis',(1.,0.,0.)) ;
#126292=DIRECTION('center_axis',(0.,-8.67361737988405E-15,-1.)) ;
#126293=DIRECTION('ref_axis',(0.,1.,-8.67361737988405E-15)) ;
#126294=DIRECTION('center_axis',(0.,-1.,8.97270763436279E-17)) ;
#126295=DIRECTION('ref_axis',(0.,-8.97270763436279E-17,-1.)) ;
#126296=DIRECTION('center_axis',(0.,-1.,8.97270763436279E-17)) ;
#126297=DIRECTION('ref_axis',(0.,-8.97270763436279E-17,-1.)) ;
#126298=DIRECTION('center_axis',(0.,-1.,0.)) ;
#126299=DIRECTION('ref_axis',(0.,0.,-1.)) ;
#126300=DIRECTION('center_axis',(0.,0.,-1.)) ;
#126301=DIRECTION('ref_axis',(-1.,0.,0.)) ;
#126302=DIRECTION('center_axis',(0.,0.,1.)) ;
#126303=DIRECTION('ref_axis',(-1.,0.,0.)) ;
#126304=DIRECTION('center_axis',(0.,0.,-1.)) ;
#126305=DIRECTION('ref_axis',(-1.,0.,0.)) ;
#126306=DIRECTION('center_axis',(0.,1.,0.)) ;
#126307=DIRECTION('ref_axis',(1.,0.,0.)) ;
#126308=DIRECTION('center_axis',(-1.,0.,0.)) ;
#126309=DIRECTION('ref_axis',(0.,0.,-1.)) ;
#126310=DIRECTION('center_axis',(0.,-1.73472347597681E-14,1.)) ;
#126311=DIRECTION('ref_axis',(0.,1.,1.73472347597681E-14)) ;
#126312=DIRECTION('center_axis',(1.,0.,0.)) ;
#126313=DIRECTION('ref_axis',(0.,0.,-1.)) ;
#126314=DIRECTION('center_axis',(0.,0.,1.)) ;
#126315=DIRECTION('ref_axis',(-1.,0.,0.)) ;
#126316=DIRECTION('center_axis',(0.,-0.514231796959101,-0.857651245551602)) ;
#126317=DIRECTION('ref_axis',(0.,-0.857651245551602,0.514231796959101)) ;
#126318=DIRECTION('center_axis',(0.,1.,0.)) ;
#126319=DIRECTION('ref_axis',(1.,0.,0.)) ;
#126320=DIRECTION('center_axis',(-1.,0.,0.)) ;
#126321=DIRECTION('ref_axis',(0.,0.,-1.)) ;
#126322=DIRECTION('center_axis',(0.,1.,8.97270763436279E-17)) ;
#126323=DIRECTION('ref_axis',(0.,-8.97270763436279E-17,1.)) ;
#126324=DIRECTION('center_axis',(0.,-1.,-8.97270763436279E-17)) ;
#126325=DIRECTION('ref_axis',(0.,-8.97270763436279E-17,1.)) ;
#126326=DIRECTION('center_axis',(0.,-1.,0.)) ;
#126327=DIRECTION('ref_axis',(0.,0.,-1.)) ;
#126328=DIRECTION('center_axis',(0.,0.,1.)) ;
#126329=DIRECTION('ref_axis',(1.,0.,0.)) ;
#126330=DIRECTION('center_axis',(0.,0.,1.)) ;
#126331=DIRECTION('ref_axis',(1.,0.,0.)) ;
#126332=DIRECTION('center_axis',(-1.,0.,0.)) ;
#126333=DIRECTION('ref_axis',(0.,0.,1.)) ;
#126334=DIRECTION('center_axis',(-1.,0.,0.)) ;
#126335=DIRECTION('ref_axis',(0.,0.,-1.)) ;
#126336=DIRECTION('center_axis',(1.,0.,0.)) ;
#126337=DIRECTION('ref_axis',(0.,0.,-1.)) ;
#126338=DIRECTION('center_axis',(0.,0.514231796959101,-0.857651245551602)) ;
#126339=DIRECTION('ref_axis',(0.,0.857651245551602,0.514231796959101)) ;
#126340=DIRECTION('center_axis',(0.,0.,-1.)) ;
#126341=DIRECTION('ref_axis',(-1.,0.,0.)) ;
#126342=DIRECTION('center_axis',(-7.01133629567814E-33,8.97270763436279E-17,
1.)) ;
#126343=DIRECTION('ref_axis',(-6.29106707073161E-49,-1.,8.97270763436279E-17)) ;
#126344=DIRECTION('center_axis',(-1.,0.,-7.01133629567814E-33)) ;
#126345=DIRECTION('ref_axis',(-7.01133629567814E-33,0.,1.)) ;
#126346=DIRECTION('center_axis',(-1.,0.,0.)) ;
#126347=DIRECTION('ref_axis',(0.,0.,1.)) ;
#126348=DIRECTION('center_axis',(0.,1.,0.)) ;
#126349=DIRECTION('ref_axis',(1.,0.,0.)) ;
#126350=DIRECTION('center_axis',(-1.,0.,0.)) ;
#126351=DIRECTION('ref_axis',(0.,0.,-1.)) ;
#126352=DIRECTION('center_axis',(1.,0.,0.)) ;
#126353=DIRECTION('ref_axis',(0.,0.,-1.)) ;
#126354=DIRECTION('center_axis',(0.,0.,-1.)) ;
#126355=DIRECTION('ref_axis',(1.,0.,0.)) ;
#126356=DIRECTION('center_axis',(-7.01133629567814E-33,8.97270763436279E-17,
1.)) ;
#126357=DIRECTION('ref_axis',(0.,-1.,0.)) ;
#126358=DIRECTION('center_axis',(0.,-1.,0.)) ;
#126359=DIRECTION('ref_axis',(0.,0.,1.)) ;
#126360=DIRECTION('center_axis',(-1.,0.,7.01133629567814E-33)) ;
#126361=DIRECTION('ref_axis',(7.01133629567814E-33,0.,1.)) ;
#126362=DIRECTION('center_axis',(-1.,0.,0.)) ;
#126363=DIRECTION('ref_axis',(0.,0.,1.)) ;
#126364=DIRECTION('center_axis',(0.,0.,-1.)) ;
#126365=DIRECTION('ref_axis',(-1.,0.,0.)) ;
#126366=DIRECTION('center_axis',(-7.01133629567814E-33,8.97270763436279E-17,
-1.)) ;
#126367=DIRECTION('ref_axis',(6.29106707073161E-49,1.,8.97270763436279E-17)) ;
#126368=DIRECTION('center_axis',(0.,-1.,8.97270763436279E-17)) ;
#126369=DIRECTION('ref_axis',(0.,-8.97270763436279E-17,-1.)) ;
#126370=DIRECTION('center_axis',(0.,-1.,0.)) ;
#126371=DIRECTION('ref_axis',(0.,0.,-1.)) ;
#126372=DIRECTION('center_axis',(1.,7.81406971160724E-17,0.)) ;
#126373=DIRECTION('ref_axis',(-7.81406971160724E-17,1.,0.)) ;
#126374=DIRECTION('center_axis',(1.,0.,0.)) ;
#126375=DIRECTION('ref_axis',(0.,0.,-1.)) ;
#126376=DIRECTION('center_axis',(1.,0.,0.)) ;
#126377=DIRECTION('ref_axis',(0.,0.,-1.)) ;
#126378=DIRECTION('center_axis',(3.78638272950961E-32,-4.8455963016112E-16,
-1.)) ;
#126379=DIRECTION('ref_axis',(1.83472821505963E-47,1.,-4.8455963016112E-16)) ;
#126380=DIRECTION('center_axis',(3.78638272950961E-32,-4.8455963016112E-16,
-1.)) ;
#126381=DIRECTION('ref_axis',(1.83472821505963E-47,1.,-4.8455963016112E-16)) ;
#126382=DIRECTION('center_axis',(0.,0.,-1.)) ;
#126383=DIRECTION('ref_axis',(-1.,0.,0.)) ;
#126384=DIRECTION('center_axis',(-7.01133629567814E-33,8.97270763436279E-17,
-1.)) ;
#126385=DIRECTION('ref_axis',(0.,1.,0.)) ;
#126386=DIRECTION('center_axis',(0.,-1.,0.)) ;
#126387=DIRECTION('ref_axis',(0.,0.,1.)) ;
#126388=DIRECTION('center_axis',(0.,1.,0.)) ;
#126389=DIRECTION('ref_axis',(1.,0.,0.)) ;
#126390=DIRECTION('center_axis',(-1.,0.,0.)) ;
#126391=DIRECTION('ref_axis',(0.,0.,-1.)) ;
#126392=DIRECTION('center_axis',(0.,8.67361737988401E-15,1.)) ;
#126393=DIRECTION('ref_axis',(0.,1.,-8.67361737988401E-15)) ;
#126394=DIRECTION('center_axis',(0.,1.,0.)) ;
#126395=DIRECTION('ref_axis',(1.,0.,0.)) ;
#126396=DIRECTION('center_axis',(0.,1.,0.)) ;
#126397=DIRECTION('ref_axis',(0.,0.,-1.)) ;
#126398=DIRECTION('center_axis',(0.,1.,8.97270763436279E-17)) ;
#126399=DIRECTION('ref_axis',(0.,-8.97270763436279E-17,1.)) ;
#126400=DIRECTION('center_axis',(0.,-1.,0.)) ;
#126401=DIRECTION('ref_axis',(0.,0.,-1.)) ;
#126402=DIRECTION('center_axis',(0.,0.,1.)) ;
#126403=DIRECTION('ref_axis',(1.,0.,0.)) ;
#126404=DIRECTION('center_axis',(0.,0.,1.)) ;
#126405=DIRECTION('ref_axis',(1.,0.,0.)) ;
#126406=DIRECTION('center_axis',(-1.,-7.81406971160724E-17,0.)) ;
#126407=DIRECTION('ref_axis',(7.81406971160724E-17,-1.,0.)) ;
#126408=DIRECTION('center_axis',(-1.,-7.81406971160724E-17,0.)) ;
#126409=DIRECTION('ref_axis',(-7.81406971160724E-17,1.,0.)) ;
#126410=DIRECTION('center_axis',(-7.81406971160724E-17,1.,-8.97270763436279E-17)) ;
#126411=DIRECTION('ref_axis',(-7.01133629567814E-33,8.97270763436279E-17,
1.)) ;
#126412=DIRECTION('center_axis',(0.,1.,0.)) ;
#126413=DIRECTION('ref_axis',(0.,0.,1.)) ;
#126414=DIRECTION('center_axis',(0.,1.,0.)) ;
#126415=DIRECTION('ref_axis',(1.,0.,0.)) ;
#126416=DIRECTION('center_axis',(-1.,0.,0.)) ;
#126417=DIRECTION('ref_axis',(0.,0.,-1.)) ;
#126418=DIRECTION('center_axis',(1.,7.81406971160724E-17,0.)) ;
#126419=DIRECTION('ref_axis',(0.,1.,0.)) ;
#126420=DIRECTION('center_axis',(0.,0.,-1.)) ;
#126421=DIRECTION('ref_axis',(1.,0.,0.)) ;
#126422=DIRECTION('center_axis',(1.,7.81406971160724E-17,0.)) ;
#126423=DIRECTION('ref_axis',(-7.81406971160724E-17,1.,0.)) ;
#126424=DIRECTION('center_axis',(1.,0.,0.)) ;
#126425=DIRECTION('ref_axis',(0.,0.,-1.)) ;
#126426=DIRECTION('center_axis',(1.,0.,0.)) ;
#126427=DIRECTION('ref_axis',(0.,0.,-1.)) ;
#126428=DIRECTION('center_axis',(-1.,-7.81406971160724E-17,0.)) ;
#126429=DIRECTION('ref_axis',(7.81406971160724E-17,-1.,0.)) ;
#126430=DIRECTION('center_axis',(-1.,-7.81406971160724E-17,0.)) ;
#126431=DIRECTION('ref_axis',(-7.81406971160724E-17,1.,0.)) ;
#126432=DIRECTION('center_axis',(0.,0.,-1.)) ;
#126433=DIRECTION('ref_axis',(-1.,0.,0.)) ;
#126434=DIRECTION('center_axis',(0.,0.,-1.)) ;
#126435=DIRECTION('ref_axis',(-1.,0.,0.)) ;
#126436=DIRECTION('center_axis',(0.,1.,0.)) ;
#126437=DIRECTION('ref_axis',(1.,0.,0.)) ;
#126438=DIRECTION('center_axis',(0.,1.,0.)) ;
#126439=DIRECTION('ref_axis',(0.,0.,-1.)) ;
#126440=DIRECTION('center_axis',(1.,7.81406971160724E-17,0.)) ;
#126441=DIRECTION('ref_axis',(0.,1.,0.)) ;
#126442=DIRECTION('center_axis',(0.,-1.,0.)) ;
#126443=DIRECTION('ref_axis',(0.,0.,1.)) ;
#126444=DIRECTION('center_axis',(7.81406971160724E-17,-1.,-8.97270763436279E-17)) ;
#126445=DIRECTION('ref_axis',(-7.01133629567814E-33,8.97270763436279E-17,
-1.)) ;
#126446=DIRECTION('center_axis',(0.,-1.,0.)) ;
#126447=DIRECTION('ref_axis',(0.,0.,-1.)) ;
#126448=DIRECTION('center_axis',(-1.,0.,-8.67361737988401E-15)) ;
#126449=DIRECTION('ref_axis',(-8.67361737988401E-15,0.,1.)) ;
#126450=DIRECTION('center_axis',(-8.67361737988401E-15,8.67361737988405E-15,
-1.)) ;
#126451=DIRECTION('ref_axis',(0.,1.,8.67361737988405E-15)) ;
#126452=DIRECTION('center_axis',(0.,0.,-1.)) ;
#126453=DIRECTION('ref_axis',(-1.,0.,0.)) ;
#126454=DIRECTION('center_axis',(0.,8.67361737988405E-15,-1.)) ;
#126455=DIRECTION('ref_axis',(0.,1.,8.67361737988405E-15)) ;
#126456=DIRECTION('center_axis',(1.,0.,0.)) ;
#126457=DIRECTION('ref_axis',(0.,0.,-1.)) ;
#126458=DIRECTION('center_axis',(-1.,0.,0.)) ;
#126459=DIRECTION('ref_axis',(0.,0.,1.)) ;
#126460=DIRECTION('center_axis',(0.,-1.,0.)) ;
#126461=DIRECTION('ref_axis',(0.,0.,-1.)) ;
#126462=DIRECTION('center_axis',(-1.,0.,0.)) ;
#126463=DIRECTION('ref_axis',(0.,0.,1.)) ;
#126464=DIRECTION('center_axis',(0.,-1.,0.)) ;
#126465=DIRECTION('ref_axis',(0.,0.,-1.)) ;
#126466=DIRECTION('center_axis',(8.67361737988394E-15,0.,-1.)) ;
#126467=DIRECTION('ref_axis',(-1.,0.,-8.67361737988394E-15)) ;
#126468=DIRECTION('center_axis',(-1.,0.,0.)) ;
#126469=DIRECTION('ref_axis',(0.,0.,1.)) ;
#126470=DIRECTION('center_axis',(-1.,1.73472347597681E-14,0.)) ;
#126471=DIRECTION('ref_axis',(-1.73472347597681E-14,-1.,0.)) ;
#126472=DIRECTION('center_axis',(0.,0.,1.)) ;
#126473=DIRECTION('ref_axis',(1.,0.,0.)) ;
#126474=DIRECTION('center_axis',(-8.67361737988409E-15,0.,-1.)) ;
#126475=DIRECTION('ref_axis',(-1.,0.,8.67361737988409E-15)) ;
#126476=DIRECTION('center_axis',(0.,-1.,0.)) ;
#126477=DIRECTION('ref_axis',(0.,0.,-1.)) ;
#126478=DIRECTION('center_axis',(-1.,0.,-2.16840434497101E-16)) ;
#126479=DIRECTION('ref_axis',(-2.16840434497101E-16,0.,1.)) ;
#126480=DIRECTION('center_axis',(0.447219005481266,-5.60223447638367E-6,
-0.894424485971266)) ;
#126481=DIRECTION('ref_axis',(0.894327914919435,-0.0146917039424838,0.447170811246801)) ;
#126482=DIRECTION('center_axis',(-0.447220452186733,-7.1003629231252E-6,
-0.894423762595493)) ;
#126483=DIRECTION('ref_axis',(0.894325663271496,0.0148067719247234,-0.447171519127916)) ;
#126484=DIRECTION('center_axis',(2.16840434497101E-16,0.,-1.)) ;
#126485=DIRECTION('ref_axis',(-1.,0.,-2.16840434497101E-16)) ;
#126486=DIRECTION('center_axis',(0.894423762593898,-7.10036023719333E-6,
-0.447220452189923)) ;
#126487=DIRECTION('ref_axis',(0.447171519131178,0.014806771908337,0.894325663270136)) ;
#126488=DIRECTION('center_axis',(0.894424485971477,-5.6022343618357E-6,
0.447219005480843)) ;
#126489=DIRECTION('ref_axis',(0.447170811246647,0.0146917039013095,-0.894327914920188)) ;
#126490=DIRECTION('center_axis',(0.,0.,1.)) ;
#126491=DIRECTION('ref_axis',(1.,0.,0.)) ;
#126492=DIRECTION('center_axis',(-0.894423762593899,-7.10036026306032E-6,
0.447220452189921)) ;
#126493=DIRECTION('ref_axis',(0.447171519131236,-0.0148067718993793,0.894325663270256)) ;
#126494=DIRECTION('center_axis',(-0.894424485971371,-5.60223466451923E-6,
-0.447219005481054)) ;
#126495=DIRECTION('ref_axis',(0.447170811246984,-0.0146917038828087,-0.894327914920324)) ;
#126496=DIRECTION('center_axis',(1.,0.,-2.16840434497101E-16)) ;
#126497=DIRECTION('ref_axis',(-2.16840434497101E-16,0.,-1.)) ;
#126498=DIRECTION('center_axis',(0.447220452189006,-7.10035961013466E-6,
0.894423762594357)) ;
#126499=DIRECTION('ref_axis',(0.894325663270134,-0.0148067719434002,-0.447171519130021)) ;
#126500=DIRECTION('center_axis',(-0.447219005476855,-5.60223624898873E-6,
0.894424485973471)) ;
#126501=DIRECTION('ref_axis',(0.894327914921509,0.0146917039515858,0.447170811242355)) ;
#126502=DIRECTION('center_axis',(-1.,0.,-2.16840434497101E-16)) ;
#126503=DIRECTION('ref_axis',(-2.16840434497101E-16,0.,1.)) ;
#126504=DIRECTION('center_axis',(0.447219005481374,-5.60223458892711E-6,
-0.894424485971211)) ;
#126505=DIRECTION('ref_axis',(0.894327914919542,-0.0146917039301271,0.447170811246992)) ;
#126506=DIRECTION('center_axis',(-0.447220452186661,-7.10036284809686E-6,
-0.894423762595529)) ;
#126507=DIRECTION('ref_axis',(0.894325663271462,0.0148067719300271,-0.447171519127808)) ;
#126508=DIRECTION('center_axis',(2.16840434497101E-16,0.,-1.)) ;
#126509=DIRECTION('ref_axis',(-1.,0.,-2.16840434497101E-16)) ;
#126510=DIRECTION('center_axis',(0.8944237625938,-7.10036041135031E-6,-0.447220452190118)) ;
#126511=DIRECTION('ref_axis',(0.447171519131424,0.0148067719010635,0.894325663270134)) ;
#126512=DIRECTION('center_axis',(0.894424485971393,-5.60223456270103E-6,
0.44721900548101)) ;
#126513=DIRECTION('ref_axis',(0.44717081124683,0.0146917038993221,-0.89432791492013)) ;
#126514=DIRECTION('center_axis',(0.,0.,1.)) ;
#126515=DIRECTION('ref_axis',(1.,0.,0.)) ;
#126516=DIRECTION('center_axis',(-0.894423762593985,-7.10036011396666E-6,
0.44722045218975)) ;
#126517=DIRECTION('ref_axis',(0.447171519131028,-0.0148067719045682,0.894325663270274)) ;
#126518=DIRECTION('center_axis',(-0.894424485971438,-5.60223469492586E-6,
-0.447219005480921)) ;
#126519=DIRECTION('ref_axis',(0.447170811246701,-0.0146917039057028,-0.894327914920089)) ;
#126520=DIRECTION('center_axis',(1.,0.,-2.16840434497101E-16)) ;
#126521=DIRECTION('ref_axis',(-2.16840434497101E-16,0.,-1.)) ;
#126522=DIRECTION('center_axis',(0.447220452189581,-7.10036082007094E-6,
0.894423762594069)) ;
#126523=DIRECTION('ref_axis',(0.894325663270147,-0.014806771920165,-0.447171519130766)) ;
#126524=DIRECTION('center_axis',(-0.447219005480049,-5.60223383386894E-6,
0.894424485971874)) ;
#126525=DIRECTION('ref_axis',(0.89432791492014,0.0146917039354466,0.447170811245622)) ;
#126526=DIRECTION('center_axis',(-1.,0.,-2.16840434497101E-16)) ;
#126527=DIRECTION('ref_axis',(-2.16840434497101E-16,0.,1.)) ;
#126528=DIRECTION('center_axis',(0.447219005480065,-5.60223452105138E-6,
-0.894424485971866)) ;
#126529=DIRECTION('ref_axis',(0.894327914920316,-0.0146917039210787,0.447170811245742)) ;
#126530=DIRECTION('center_axis',(-0.447220452189082,-7.10035963327167E-6,
-0.894423762594318)) ;
#126531=DIRECTION('ref_axis',(0.894325663270257,0.0148067719312621,-0.447171519130178)) ;
#126532=DIRECTION('center_axis',(2.16840434497101E-16,0.,-1.)) ;
#126533=DIRECTION('ref_axis',(-1.,0.,-2.16840434497101E-16)) ;
#126534=DIRECTION('center_axis',(0.8944237625938,-7.10036041135031E-6,-0.447220452190118)) ;
#126535=DIRECTION('ref_axis',(0.447171519131363,0.014806771910293,0.894325663270012)) ;
#126536=DIRECTION('center_axis',(0.894424485971369,-5.60223461266618E-6,
0.447219005481058)) ;
#126537=DIRECTION('ref_axis',(0.447170811246847,0.0146917039042423,-0.89432791492004)) ;
#126538=DIRECTION('center_axis',(0.,0.,1.)) ;
#126539=DIRECTION('ref_axis',(1.,0.,0.)) ;
#126540=DIRECTION('center_axis',(-0.894423762593847,-7.10036059498734E-6,
0.447220452190025)) ;
#126541=DIRECTION('ref_axis',(0.447171519131148,-0.0148067719290856,0.894325663269808)) ;
#126542=DIRECTION('center_axis',(-0.894424485971523,-5.60223451992655E-6,
-0.447219005480752)) ;
#126543=DIRECTION('ref_axis',(0.447170811246541,-0.0146917039039939,-0.894327914920198)) ;
#126544=DIRECTION('center_axis',(1.,0.,-2.16840434497101E-16)) ;
#126545=DIRECTION('ref_axis',(-2.16840434497101E-16,0.,-1.)) ;
#126546=DIRECTION('center_axis',(0.447220452189557,-7.10036079532928E-6,
0.894423762594081)) ;
#126547=DIRECTION('ref_axis',(0.894325663270269,-0.0148067719118157,-0.447171519130797)) ;
#126548=DIRECTION('center_axis',(-0.447219005480149,-5.60223388206588E-6,
0.894424485971824)) ;
#126549=DIRECTION('ref_axis',(0.894327914920146,0.0146917039311632,0.447170811245751)) ;
#126550=DIRECTION('center_axis',(-1.,0.,-2.16840434497101E-16)) ;
#126551=DIRECTION('ref_axis',(-2.16840434497101E-16,0.,1.)) ;
#126552=DIRECTION('center_axis',(0.447219005480246,-5.60223470853928E-6,
-0.894424485971776)) ;
#126553=DIRECTION('ref_axis',(0.894327914920193,-0.0146917039234679,0.447170811245909)) ;
#126554=DIRECTION('center_axis',(-0.447220452189106,-7.10035965817415E-6,
-0.894423762594306)) ;
#126555=DIRECTION('ref_axis',(0.894325663270211,0.014806771933774,-0.447171519130185)) ;
#126556=DIRECTION('center_axis',(2.16840434497101E-16,0.,-1.)) ;
#126557=DIRECTION('ref_axis',(-1.,0.,-2.16840434497101E-16)) ;
#126558=DIRECTION('center_axis',(0.894423762593813,-7.10036038628687E-6,
-0.447220452190094)) ;
#126559=DIRECTION('ref_axis',(0.447171519131279,0.0148067719193131,0.894325663269904)) ;
#126560=DIRECTION('center_axis',(0.894424485972067,-5.60223311109745E-6,
0.447219005479663)) ;
#126561=DIRECTION('ref_axis',(0.447170811245097,0.0146917039552028,-0.894327914920078)) ;
#126562=DIRECTION('center_axis',(0.,0.,1.)) ;
#126563=DIRECTION('ref_axis',(1.,0.,0.)) ;
#126564=DIRECTION('center_axis',(-0.894423762593869,-7.10036049345021E-6,
0.447220452189981)) ;
#126565=DIRECTION('ref_axis',(0.44717151913113,-0.0148067719249295,0.894325663269886)) ;
#126566=DIRECTION('center_axis',(-0.89442448597151,-5.60223454494956E-6,
-0.447219005480776)) ;
#126567=DIRECTION('ref_axis',(0.447170811246508,-0.0146917039126806,-0.894327914920071)) ;
#126568=DIRECTION('center_axis',(1.,0.,-2.16840434497101E-16)) ;
#126569=DIRECTION('ref_axis',(-2.16840434497101E-16,0.,-1.)) ;
#126570=DIRECTION('center_axis',(0.447220452189376,-7.1003606078408E-6,
0.894423762594172)) ;
#126571=DIRECTION('ref_axis',(0.894325663270274,-0.0148067719183669,-0.44717151913057)) ;
#126572=DIRECTION('center_axis',(-0.447219005480174,-5.60223390704821E-6,
0.894424485971812)) ;
#126573=DIRECTION('ref_axis',(0.894327914920086,0.0146917039347775,0.447170811245753)) ;
#126574=DIRECTION('center_axis',(-1.,0.,-2.16840434497101E-16)) ;
#126575=DIRECTION('ref_axis',(-2.16840434497101E-16,0.,1.)) ;
#126576=DIRECTION('center_axis',(0.447219005480053,-5.60223450851907E-6,
-0.894424485971872)) ;
#126577=DIRECTION('ref_axis',(0.894327914920194,-0.0146917039308781,0.447170811245665)) ;
#126578=DIRECTION('center_axis',(-0.447220452189219,-7.10035971890228E-6,
-0.89442376259425)) ;
#126579=DIRECTION('ref_axis',(0.894325663270168,0.0148067719327317,-0.447171519130306)) ;
#126580=DIRECTION('center_axis',(2.16840434497101E-16,0.,-1.)) ;
#126581=DIRECTION('ref_axis',(-1.,0.,-2.16840434497101E-16)) ;
#126582=DIRECTION('center_axis',(0.894423762593776,-7.10036044814174E-6,
-0.447220452190168)) ;
#126583=DIRECTION('ref_axis',(0.447171519131389,0.0148067719138353,0.894325663269939)) ;
#126584=DIRECTION('center_axis',(0.894424485971344,-5.60223463676545E-6,
0.447219005481109)) ;
#126585=DIRECTION('ref_axis',(0.447170811246964,0.0146917038941729,-0.894327914920147)) ;
#126586=DIRECTION('center_axis',(0.,0.,1.)) ;
#126587=DIRECTION('ref_axis',(1.,0.,0.)) ;
#126588=DIRECTION('center_axis',(-0.89442376259387,-7.10036051931658E-6,
0.447220452189979)) ;
#126589=DIRECTION('ref_axis',(0.447171519131125,-0.0148067719254494,0.89432566326988)) ;
#126590=DIRECTION('center_axis',(-0.894424485971498,-5.60223455703937E-6,
-0.447219005480801)) ;
#126591=DIRECTION('ref_axis',(0.447170811246509,-0.0146917039163654,-0.89432791492001)) ;
#126592=DIRECTION('center_axis',(1.,0.,-2.16840434497101E-16)) ;
#126593=DIRECTION('ref_axis',(-2.16840434497101E-16,0.,-1.)) ;
#126594=DIRECTION('center_axis',(0.447220452189472,-7.10036070777138E-6,
0.894423762594123)) ;
#126595=DIRECTION('ref_axis',(0.894325663270285,-0.0148067719138536,-0.447171519130697)) ;
#126596=DIRECTION('center_axis',(-0.447219005479954,-5.60223370799162E-6,
0.894424485971921)) ;
#126597=DIRECTION('ref_axis',(0.894327914920089,0.0146917039429744,0.447170811245477)) ;
#126598=DIRECTION('center_axis',(-1.,0.,-2.16840434497101E-16)) ;
#126599=DIRECTION('ref_axis',(-2.16840434497101E-16,0.,1.)) ;
#126600=DIRECTION('center_axis',(0.44721900547998,-5.60223443353162E-6,
-0.894424485971908)) ;
#126601=DIRECTION('ref_axis',(0.894327914920239,-0.0146917039302217,0.447170811245596)) ;
#126602=DIRECTION('center_axis',(-0.44722045218906,-7.10035958218204E-6,
-0.894423762594329)) ;
#126603=DIRECTION('ref_axis',(0.894325663270273,0.0148067719309328,-0.447171519130157)) ;
#126604=DIRECTION('center_axis',(2.16840434497101E-16,0.,-1.)) ;
#126605=DIRECTION('ref_axis',(-1.,0.,-2.16840434497101E-16)) ;
#126606=DIRECTION('center_axis',(0.894423762593771,-7.10036080288375E-6,
-0.447220452190178)) ;
#126607=DIRECTION('ref_axis',(0.447171519131049,0.0148067719675465,0.894325663269221)) ;
#126608=DIRECTION('center_axis',(0.894424485971344,-5.60223464973865E-6,
0.447219005481108)) ;
#126609=DIRECTION('ref_axis',(0.447170811246911,0.0146917039020779,-0.894327914920044)) ;
#126610=DIRECTION('center_axis',(0.,0.,1.)) ;
#126611=DIRECTION('ref_axis',(1.,0.,0.)) ;
#126612=DIRECTION('center_axis',(-0.894423762593835,-7.10036060735852E-6,
0.44722045219005)) ;
#126613=DIRECTION('ref_axis',(0.447171519131198,-0.0148067719252183,0.894325663269847)) ;
#126614=DIRECTION('center_axis',(-0.894424485971953,-5.602234646445E-6,
-0.447219005479891)) ;
#126615=DIRECTION('ref_axis',(0.447170811245515,-0.0146917039293451,-0.894327914920294)) ;
#126616=DIRECTION('center_axis',(1.,0.,-2.16840434497101E-16)) ;
#126617=DIRECTION('ref_axis',(-2.16840434497101E-16,0.,-1.)) ;
#126618=DIRECTION('center_axis',(0.447220452189611,-7.10036020924201E-6,
0.894423762594054)) ;
#126619=DIRECTION('ref_axis',(0.894325663270291,-0.0148067719084231,-0.447171519130865)) ;
#126620=DIRECTION('center_axis',(-0.447219005479986,-5.60223428805301E-6,
0.894424485971906)) ;
#126621=DIRECTION('ref_axis',(0.894327914919888,0.0146917039567803,0.447170811245425)) ;
#126622=DIRECTION('center_axis',(-1.,0.,-2.16840434497101E-16)) ;
#126623=DIRECTION('ref_axis',(-2.16840434497101E-16,0.,1.)) ;
#126624=DIRECTION('center_axis',(0.447219005479986,-5.60223379723993E-6,
-0.894424485971905)) ;
#126625=DIRECTION('ref_axis',(0.894327914920294,-0.0146917039261431,0.44717081124562)) ;
#126626=DIRECTION('center_axis',(-0.447220452189224,-7.10036029985229E-6,
-0.894423762594247)) ;
#126627=DIRECTION('ref_axis',(0.894325663270126,0.0148067719354631,-0.447171519130301)) ;
#126628=DIRECTION('center_axis',(2.16840434497101E-16,0.,-1.)) ;
#126629=DIRECTION('ref_axis',(-1.,0.,-2.16840434497101E-16)) ;
#126630=DIRECTION('center_axis',(0.894423762593695,-7.10036088835547E-6,
-0.447220452190328)) ;
#126631=DIRECTION('ref_axis',(0.447171519131228,0.0148067719634075,0.8943256632692)) ;
#126632=DIRECTION('center_axis',(0.894424485971236,-5.60223487474278E-6,
0.447219005481325)) ;
#126633=DIRECTION('ref_axis',(0.447170811247132,0.0146917039018784,-0.894327914919936)) ;
#126634=DIRECTION('center_axis',(0.,0.,1.)) ;
#126635=DIRECTION('ref_axis',(1.,0.,0.)) ;
#126636=DIRECTION('center_axis',(-0.894423762594132,-7.10036099567427E-6,
0.447220452189455)) ;
#126637=DIRECTION('ref_axis',(0.447171519130486,-0.0148067719437975,0.894325663269895)) ;
#126638=DIRECTION('center_axis',(-0.894424485972025,-5.60223448349518E-6,
-0.447219005479747)) ;
#126639=DIRECTION('ref_axis',(0.447170811245346,-0.0146917039328969,-0.89432791492032)) ;
#126640=DIRECTION('center_axis',(1.,0.,-2.16840434497101E-16)) ;
#126641=DIRECTION('ref_axis',(-2.16840434497101E-16,0.,-1.)) ;
#126642=DIRECTION('center_axis',(0.447220452189153,-7.10035973416595E-6,
0.894423762594283)) ;
#126643=DIRECTION('ref_axis',(0.894325663270205,-0.014806771932442,-0.447171519130242)) ;
#126644=DIRECTION('center_axis',(-0.447219005479711,-5.60223412313625E-6,
0.894424485972043)) ;
#126645=DIRECTION('ref_axis',(0.894327914920089,0.0146917039520517,0.447170811245179)) ;
#126646=DIRECTION('center_axis',(-1.,0.,-2.16840434497101E-16)) ;
#126647=DIRECTION('ref_axis',(-2.16840434497101E-16,0.,1.)) ;
#126648=DIRECTION('center_axis',(0.447219005480528,-5.60223404983417E-6,
-0.894424485971634)) ;
#126649=DIRECTION('ref_axis',(0.894327914919937,-0.0146917039325427,0.447170811246124)) ;
#126650=DIRECTION('center_axis',(-0.447220452189473,-7.10036045906616E-6,
-0.894423762594123)) ;
#126651=DIRECTION('ref_axis',(0.894325663270072,0.0148067719300326,-0.447171519130588)) ;
#126652=DIRECTION('center_axis',(2.16840434497101E-16,0.,-1.)) ;
#126653=DIRECTION('ref_axis',(-1.,0.,-2.16840434497101E-16)) ;
#126654=DIRECTION('center_axis',(0.894423762593943,-7.10036005950268E-6,
-0.447220452189833)) ;
#126655=DIRECTION('ref_axis',(0.44717151913091,0.0148067719349505,0.89432566326983)) ;
#126656=DIRECTION('center_axis',(0.894424485971607,-5.60223403505354E-6,
0.447219005480582)) ;
#126657=DIRECTION('ref_axis',(0.447170811245978,0.0146917039629369,-0.894327914919511)) ;
#126658=DIRECTION('center_axis',(0.,0.,1.)) ;
#126659=DIRECTION('ref_axis',(1.,0.,0.)) ;
#126660=DIRECTION('center_axis',(-0.894423762594202,-7.10036078087079E-6,
0.447220452189316)) ;
#126661=DIRECTION('ref_axis',(0.447171519130283,-0.0148067719529112,0.894325663269846)) ;
#126662=DIRECTION('center_axis',(-0.894424485971881,-5.60223416366214E-6,
-0.447219005480035)) ;
#126663=DIRECTION('ref_axis',(0.447170811245601,-0.014691703937177,-0.894327914920122)) ;
#126664=DIRECTION('center_axis',(1.,0.,-2.16840434497101E-16)) ;
#126665=DIRECTION('ref_axis',(-2.16840434497101E-16,0.,-1.)) ;
#126666=DIRECTION('center_axis',(0.4472204521899,-7.10036019911746E-6,0.89442376259391)) ;
#126667=DIRECTION('ref_axis',(0.89432566326982,-0.0148067719330621,-0.447171519130991)) ;
#126668=DIRECTION('center_axis',(-0.447219005479637,-5.60223439043371E-6,
0.89442448597208)) ;
#126669=DIRECTION('ref_axis',(0.894327914920201,0.0146917039462084,0.447170811245147)) ;
#126670=DIRECTION('center_axis',(1.,0.,-2.16840434497101E-16)) ;
#126671=DIRECTION('ref_axis',(-2.16840434497101E-16,0.,-1.)) ;
#126672=DIRECTION('center_axis',(1.,0.,0.)) ;
#126673=DIRECTION('ref_axis',(0.,0.,-1.)) ;
#126674=DIRECTION('center_axis',(-1.,0.,0.)) ;
#126675=DIRECTION('ref_axis',(0.,0.,1.)) ;
#126676=DIRECTION('center_axis',(0.,-1.,0.)) ;
#126677=DIRECTION('ref_axis',(0.,0.,-1.)) ;
#126678=DIRECTION('center_axis',(0.,0.,-1.)) ;
#126679=DIRECTION('ref_axis',(1.,0.,0.)) ;
#126680=DIRECTION('center_axis',(0.,-1.,0.)) ;
#126681=DIRECTION('ref_axis',(0.,0.,-1.)) ;
#126682=DIRECTION('center_axis',(0.,-1.,0.)) ;
#126683=DIRECTION('ref_axis',(0.,0.,-1.)) ;
#126684=DIRECTION('center_axis',(0.,-1.,0.)) ;
#126685=DIRECTION('ref_axis',(0.,0.,-1.)) ;
#126686=DIRECTION('center_axis',(0.,0.,-1.)) ;
#126687=DIRECTION('ref_axis',(1.,0.,0.)) ;
#126688=DIRECTION('center_axis',(0.,0.,1.)) ;
#126689=DIRECTION('ref_axis',(1.,0.,0.)) ;
#126690=DIRECTION('center_axis',(0.,0.,-1.)) ;
#126691=DIRECTION('ref_axis',(-1.,0.,0.)) ;
#126692=DIRECTION('center_axis',(0.,1.,0.)) ;
#126693=DIRECTION('ref_axis',(0.,0.,1.)) ;
#126694=DIRECTION('center_axis',(0.,-1.,0.)) ;
#126695=DIRECTION('ref_axis',(0.,0.,-1.)) ;
#126696=DIRECTION('center_axis',(-1.,0.,2.16840434497101E-16)) ;
#126697=DIRECTION('ref_axis',(2.16840434497101E-16,0.,1.)) ;
#126698=DIRECTION('center_axis',(-1.,0.,0.)) ;
#126699=DIRECTION('ref_axis',(0.,0.,1.)) ;
#126700=DIRECTION('center_axis',(1.,0.,0.)) ;
#126701=DIRECTION('ref_axis',(0.,0.,-1.)) ;
#126702=DIRECTION('center_axis',(0.,1.,0.)) ;
#126703=DIRECTION('ref_axis',(0.,0.,1.)) ;
#126704=DIRECTION('center_axis',(0.,-1.,0.)) ;
#126705=DIRECTION('ref_axis',(0.,0.,-1.)) ;
#126706=DIRECTION('center_axis',(2.16840434497101E-16,0.,-1.)) ;
#126707=DIRECTION('ref_axis',(-1.,0.,-2.16840434497101E-16)) ;
#126708=DIRECTION('center_axis',(0.,0.,-1.)) ;
#126709=DIRECTION('ref_axis',(-1.,0.,0.)) ;
#126710=DIRECTION('center_axis',(-1.,0.,-2.16840434497101E-16)) ;
#126711=DIRECTION('ref_axis',(-2.16840434497101E-16,0.,1.)) ;
#126712=DIRECTION('center_axis',(-1.,0.,0.)) ;
#126713=DIRECTION('ref_axis',(0.,0.,1.)) ;
#126714=DIRECTION('center_axis',(1.,0.,0.)) ;
#126715=DIRECTION('ref_axis',(0.,0.,-1.)) ;
#126716=DIRECTION('center_axis',(0.,-1.,0.)) ;
#126717=DIRECTION('ref_axis',(0.,0.,-1.)) ;
#126718=DIRECTION('center_axis',(0.,-1.,0.)) ;
#126719=DIRECTION('ref_axis',(0.,0.,-1.)) ;
#126720=DIRECTION('center_axis',(0.,1.,0.)) ;
#126721=DIRECTION('ref_axis',(1.,0.,0.)) ;
#126722=DIRECTION('center_axis',(0.,0.,1.)) ;
#126723=DIRECTION('ref_axis',(-1.,0.,0.)) ;
#126724=DIRECTION('center_axis',(0.,1.,0.)) ;
#126725=DIRECTION('ref_axis',(1.,0.,0.)) ;
#126726=DIRECTION('center_axis',(0.,0.,1.)) ;
#126727=DIRECTION('ref_axis',(-1.,0.,0.)) ;
#126728=DIRECTION('center_axis',(0.,-1.,0.)) ;
#126729=DIRECTION('ref_axis',(0.,0.,-1.)) ;
#126730=DIRECTION('center_axis',(0.,-1.,0.)) ;
#126731=DIRECTION('ref_axis',(0.,0.,-1.)) ;
#126732=DIRECTION('center_axis',(0.,1.,0.)) ;
#126733=DIRECTION('ref_axis',(0.,0.,1.)) ;
#126734=DIRECTION('center_axis',(0.,-1.,0.)) ;
#126735=DIRECTION('ref_axis',(0.,0.,-1.)) ;
#126736=DIRECTION('center_axis',(0.,0.,-1.)) ;
#126737=DIRECTION('ref_axis',(-1.,0.,0.)) ;
#126738=DIRECTION('center_axis',(0.,0.,1.)) ;
#126739=DIRECTION('ref_axis',(1.,0.,0.)) ;
#126740=DIRECTION('center_axis',(-2.16840434497101E-16,0.,1.)) ;
#126741=DIRECTION('ref_axis',(1.,0.,2.16840434497101E-16)) ;
#126742=DIRECTION('center_axis',(0.,0.,1.)) ;
#126743=DIRECTION('ref_axis',(1.,0.,0.)) ;
#126744=DIRECTION('center_axis',(0.,1.,0.)) ;
#126745=DIRECTION('ref_axis',(0.,0.,1.)) ;
#126746=DIRECTION('center_axis',(0.,-1.,0.)) ;
#126747=DIRECTION('ref_axis',(0.,0.,-1.)) ;
#126748=DIRECTION('center_axis',(0.,1.,0.)) ;
#126749=DIRECTION('ref_axis',(1.,0.,0.)) ;
#126750=DIRECTION('center_axis',(-1.,0.,0.)) ;
#126751=DIRECTION('ref_axis',(0.,0.,-1.)) ;
#126752=DIRECTION('center_axis',(0.,1.,0.)) ;
#126753=DIRECTION('ref_axis',(1.,0.,0.)) ;
#126754=DIRECTION('center_axis',(1.,0.,0.)) ;
#126755=DIRECTION('ref_axis',(0.,0.,1.)) ;
#126756=DIRECTION('center_axis',(1.,0.,2.16840434497101E-16)) ;
#126757=DIRECTION('ref_axis',(2.16840434497101E-16,0.,-1.)) ;
#126758=DIRECTION('center_axis',(0.,-1.,0.)) ;
#126759=DIRECTION('ref_axis',(0.,0.,-1.)) ;
#126760=DIRECTION('center_axis',(0.,-1.,0.)) ;
#126761=DIRECTION('ref_axis',(0.,0.,-1.)) ;
#126762=DIRECTION('center_axis',(0.,0.,1.)) ;
#126763=DIRECTION('ref_axis',(1.,0.,0.)) ;
#126764=DIRECTION('center_axis',(0.,0.,-1.)) ;
#126765=DIRECTION('ref_axis',(-1.,0.,0.)) ;
#126766=DIRECTION('center_axis',(0.,0.,1.)) ;
#126767=DIRECTION('ref_axis',(1.,0.,0.)) ;
#126768=DIRECTION('center_axis',(0.,-1.,0.)) ;
#126769=DIRECTION('ref_axis',(0.,0.,-1.)) ;
#126770=DIRECTION('center_axis',(0.,-1.,0.)) ;
#126771=DIRECTION('ref_axis',(0.,0.,-1.)) ;
#126772=DIRECTION('center_axis',(0.,1.,0.)) ;
#126773=DIRECTION('ref_axis',(1.,0.,0.)) ;
#126774=DIRECTION('center_axis',(-1.,0.,0.)) ;
#126775=DIRECTION('ref_axis',(0.,0.,-1.)) ;
#126776=DIRECTION('center_axis',(0.,1.,0.)) ;
#126777=DIRECTION('ref_axis',(1.,0.,0.)) ;
#126778=DIRECTION('center_axis',(-1.,0.,0.)) ;
#126779=DIRECTION('ref_axis',(0.,0.,-1.)) ;
#126780=DIRECTION('center_axis',(0.,-1.,0.)) ;
#126781=DIRECTION('ref_axis',(0.,0.,-1.)) ;
#126782=DIRECTION('center_axis',(0.,-1.,0.)) ;
#126783=DIRECTION('ref_axis',(0.,0.,-1.)) ;
#126784=DIRECTION('center_axis',(-1.,0.,0.)) ;
#126785=DIRECTION('ref_axis',(0.,0.,1.)) ;
#126786=DIRECTION('center_axis',(-1.,0.,0.)) ;
#126787=DIRECTION('ref_axis',(0.,0.,1.)) ;
#126788=DIRECTION('center_axis',(1.,0.,0.)) ;
#126789=DIRECTION('ref_axis',(0.,0.,-1.)) ;
#126790=DIRECTION('center_axis',(-1.,0.,0.)) ;
#126791=DIRECTION('ref_axis',(0.,0.,1.)) ;
#126792=DIRECTION('center_axis',(0.,-1.,0.)) ;
#126793=DIRECTION('ref_axis',(0.,0.,-1.)) ;
#126794=DIRECTION('center_axis',(0.,-1.,0.)) ;
#126795=DIRECTION('ref_axis',(0.,0.,-1.)) ;
#126796=DIRECTION('center_axis',(0.,1.,0.)) ;
#126797=DIRECTION('ref_axis',(1.,0.,0.)) ;
#126798=DIRECTION('center_axis',(0.,0.,-1.)) ;
#126799=DIRECTION('ref_axis',(1.,0.,0.)) ;
#126800=DIRECTION('center_axis',(0.,1.,0.)) ;
#126801=DIRECTION('ref_axis',(1.,0.,0.)) ;
#126802=DIRECTION('center_axis',(0.,0.,1.)) ;
#126803=DIRECTION('ref_axis',(-1.,0.,0.)) ;
#126804=DIRECTION('center_axis',(0.,0.,-1.)) ;
#126805=DIRECTION('ref_axis',(-1.,0.,0.)) ;
#126806=DIRECTION('center_axis',(-0.669589480006976,0.669589480006974,-0.321402950403349)) ;
#126807=DIRECTION('ref_axis',(-0.707106781186547,-0.707106781186548,5.45170614306381E-16)) ;
#126808=DIRECTION('center_axis',(0.669589480006969,-0.669589480006984,0.321402950403343)) ;
#126809=DIRECTION('ref_axis',(0.707106781186555,0.70710678118654,-2.64684135297117E-16)) ;
#126810=DIRECTION('center_axis',(0.,1.,0.)) ;
#126811=DIRECTION('ref_axis',(1.,0.,0.)) ;
#126812=DIRECTION('center_axis',(0.,1.,0.)) ;
#126813=DIRECTION('ref_axis',(0.,0.,-1.)) ;
#126814=DIRECTION('center_axis',(0.707106781186548,-0.707106781186548,-1.07330539167836E-14)) ;
#126815=DIRECTION('ref_axis',(-0.707106781186548,-0.707106781186548,3.64780758836058E-31)) ;
#126816=DIRECTION('center_axis',(-0.707106781186549,0.707106781186546,0.)) ;
#126817=DIRECTION('ref_axis',(-0.707106781186546,-0.707106781186549,0.)) ;
#126818=DIRECTION('center_axis',(0.,-1.,0.)) ;
#126819=DIRECTION('ref_axis',(0.,0.,-1.)) ;
#126820=DIRECTION('center_axis',(0.,1.,0.)) ;
#126821=DIRECTION('ref_axis',(0.,0.,1.)) ;
#126822=DIRECTION('center_axis',(-0.879462917689188,-0.219865729422294,
-0.42214220049081)) ;
#126823=DIRECTION('ref_axis',(-0.432731067584771,-5.39224131925863E-16,
0.901523057468274)) ;
#126824=DIRECTION('center_axis',(0.879462917689189,0.219865729422295,0.422142200490806)) ;
#126825=DIRECTION('ref_axis',(0.432731067584767,-3.28412466813249E-16,-0.901523057468275)) ;
#126826=DIRECTION('center_axis',(0.,-1.,0.)) ;
#126827=DIRECTION('ref_axis',(0.,0.,1.)) ;
#126828=DIRECTION('center_axis',(0.,0.,1.)) ;
#126829=DIRECTION('ref_axis',(-1.,0.,0.)) ;
#126830=DIRECTION('center_axis',(0.,1.,0.)) ;
#126831=DIRECTION('ref_axis',(1.,0.,0.)) ;
#126832=DIRECTION('center_axis',(0.970142500145332,0.242535625036333,0.)) ;
#126833=DIRECTION('ref_axis',(0.242535625036333,-0.970142500145332,0.)) ;
#126834=DIRECTION('center_axis',(0.669589480006976,-0.669589480006974,-0.321402950403349)) ;
#126835=DIRECTION('ref_axis',(0.707106781186547,0.707106781186548,5.45170614306381E-16)) ;
#126836=DIRECTION('center_axis',(0.669589480006974,-0.669589480006974,-0.321402950403353)) ;
#126837=DIRECTION('ref_axis',(0.707106781186548,0.707106781186548,1.13338310925322E-17)) ;
#126838=DIRECTION('center_axis',(0.707106781186549,-0.707106781186546,0.)) ;
#126839=DIRECTION('ref_axis',(0.707106781186546,0.707106781186549,0.)) ;
#126840=DIRECTION('center_axis',(-0.70710678118655,0.707106781186545,0.)) ;
#126841=DIRECTION('ref_axis',(-0.707106781186545,-0.70710678118655,0.)) ;
#126842=DIRECTION('center_axis',(0.,0.,1.)) ;
#126843=DIRECTION('ref_axis',(1.,0.,0.)) ;
#126844=DIRECTION('center_axis',(0.,0.,1.)) ;
#126845=DIRECTION('ref_axis',(1.,0.,0.)) ;
#126846=DIRECTION('center_axis',(2.47817639425258E-16,-1.,0.)) ;
#126847=DIRECTION('ref_axis',(1.,2.47817639425258E-16,0.)) ;
#126848=DIRECTION('center_axis',(0.,-1.,0.)) ;
#126849=DIRECTION('ref_axis',(0.,0.,-1.)) ;
#126850=DIRECTION('center_axis',(-0.970142500145333,-0.24253562503633,0.)) ;
#126851=DIRECTION('ref_axis',(0.24253562503633,-0.970142500145333,0.)) ;
#126852=DIRECTION('center_axis',(0.976187060183959,-0.216930457818629,3.32210494350337E-14)) ;
#126853=DIRECTION('ref_axis',(0.216930457818629,0.976187060183959,-2.98116453088841E-12)) ;
#126854=DIRECTION('center_axis',(0.,1.,0.)) ;
#126855=DIRECTION('ref_axis',(1.,0.,0.)) ;
#126856=DIRECTION('center_axis',(9.0350181040459E-15,1.,-4.33680868994203E-15)) ;
#126857=DIRECTION('ref_axis',(1.,-9.03501810404588E-15,4.33680868994201E-15)) ;
#126858=DIRECTION('center_axis',(0.,-1.,0.)) ;
#126859=DIRECTION('ref_axis',(0.,0.,1.)) ;
#126860=DIRECTION('center_axis',(0.,0.,1.)) ;
#126861=DIRECTION('ref_axis',(-1.,8.67361737988401E-15,0.)) ;
#126862=DIRECTION('center_axis',(0.879462917689188,0.219865729422294,-0.42214220049081)) ;
#126863=DIRECTION('ref_axis',(-0.432731067584771,-2.0299798629437E-16,-0.901523057468274)) ;
#126864=DIRECTION('center_axis',(0.879462917689188,0.219865729422297,-0.422142200490809)) ;
#126865=DIRECTION('ref_axis',(-0.43273106758477,8.71332159501362E-17,-0.901523057468274)) ;
#126866=DIRECTION('center_axis',(0.,-1.,0.)) ;
#126867=DIRECTION('ref_axis',(0.,0.,-1.)) ;
#126868=DIRECTION('center_axis',(2.00438979995004E-14,1.,0.)) ;
#126869=DIRECTION('ref_axis',(-1.,2.00438979995004E-14,0.)) ;
#126870=DIRECTION('center_axis',(2.47817639425258E-16,-1.,0.)) ;
#126871=DIRECTION('ref_axis',(1.,2.47817639425258E-16,0.)) ;
#126872=DIRECTION('center_axis',(0.,-1.,0.)) ;
#126873=DIRECTION('ref_axis',(0.,0.,-1.)) ;
#126874=DIRECTION('center_axis',(0.,0.,1.)) ;
#126875=DIRECTION('ref_axis',(1.,0.,0.)) ;
#126876=DIRECTION('center_axis',(0.,0.,1.)) ;
#126877=DIRECTION('ref_axis',(1.,0.,0.)) ;
#126878=DIRECTION('center_axis',(0.,1.,0.)) ;
#126879=DIRECTION('ref_axis',(1.,0.,0.)) ;
#126880=DIRECTION('center_axis',(0.970142500145332,0.242535625036331,0.)) ;
#126881=DIRECTION('ref_axis',(0.242535625036331,-0.970142500145332,0.)) ;
#126882=DIRECTION('center_axis',(-0.97618706018396,0.216930457818626,3.48715666902615E-14)) ;
#126883=DIRECTION('ref_axis',(0.216930457818626,0.976187060183959,-9.11731595942476E-13)) ;
#126884=DIRECTION('center_axis',(0.970142500145333,0.24253562503633,0.)) ;
#126885=DIRECTION('ref_axis',(-0.24253562503633,0.970142500145333,0.)) ;
#126886=DIRECTION('center_axis',(2.47817639425258E-16,-1.,0.)) ;
#126887=DIRECTION('ref_axis',(1.,2.47817639425258E-16,0.)) ;
#126888=DIRECTION('center_axis',(-1.29658294628968E-8,-0.447213597648204,
0.894427189925793)) ;
#126889=DIRECTION('ref_axis',(0.0446435808064758,-0.893535426885365,-0.446767715478149)) ;
#126890=DIRECTION('center_axis',(-0.894427191461922,-0.447213594575946,
-5.57691505343739E-9)) ;
#126891=DIRECTION('ref_axis',(0.446767713219253,-0.89353542818951,-0.0446435773099389)) ;
#126892=DIRECTION('center_axis',(-0.447213595499893,0.894427190999948,6.57429044123456E-13)) ;
#126893=DIRECTION('ref_axis',(0.894427190999948,0.447213595499893,6.87710394375266E-12)) ;
#126894=DIRECTION('center_axis',(-2.76847490273994E-6,0.447215298958337,
0.894426339264414)) ;
#126895=DIRECTION('ref_axis',(0.0170110523159659,-0.894296896128943,0.447150629735935)) ;
#126896=DIRECTION('center_axis',(-0.00225743160624427,0.447523187701884,
0.894269478664953)) ;
#126897=DIRECTION('ref_axis',(-0.0025523933809264,-0.894271422866288,0.44751771756293)) ;
#126898=DIRECTION('center_axis',(0.,0.,1.)) ;
#126899=DIRECTION('ref_axis',(1.,0.,0.)) ;
#126900=DIRECTION('center_axis',(-0.00226103819060068,-0.894269222962555,
-0.44752368045529)) ;
#126901=DIRECTION('ref_axis',(0.00257816448348457,0.447518124036693,-0.894271145529461)) ;
#126902=DIRECTION('center_axis',(-4.29726983982175E-6,-0.894425868918636,
-0.447216239632101)) ;
#126903=DIRECTION('ref_axis',(-0.016983449338369,0.447151803283565,-0.894296833981216)) ;
#126904=DIRECTION('center_axis',(-2.76847487689518E-6,-0.894426339264826,
0.447215298957514)) ;
#126905=DIRECTION('ref_axis',(0.0170110522878384,-0.447150629735325,-0.894296896129782)) ;
#126906=DIRECTION('center_axis',(-0.00225743161331263,-0.894269478664216,
0.447523187703322)) ;
#126907=DIRECTION('ref_axis',(-0.00255239338234728,-0.447517717564354,-0.894271422865571)) ;
#126908=DIRECTION('center_axis',(0.,0.,1.)) ;
#126909=DIRECTION('ref_axis',(1.,0.,0.)) ;
#126910=DIRECTION('center_axis',(-1.29625486687073E-8,0.894427189926062,
-0.447213597647665)) ;
#126911=DIRECTION('ref_axis',(-0.044643580803928,0.446767715477792,0.893535426885671)) ;
#126912=DIRECTION('center_axis',(-1.2961187983127E-8,0.89442718992615,0.447213597647489)) ;
#126913=DIRECTION('ref_axis',(0.0446435808019586,-0.44676771547771,0.89353542688581)) ;
#126914=DIRECTION('center_axis',(2.47817639425258E-16,-1.,0.)) ;
#126915=DIRECTION('ref_axis',(1.,2.47817639425258E-16,0.)) ;
#126916=DIRECTION('center_axis',(-0.00226103817862702,0.447523680453237,
-0.894269222963613)) ;
#126917=DIRECTION('ref_axis',(0.00257816447018989,0.894271145530498,0.447518124034698)) ;
#126918=DIRECTION('center_axis',(-4.29727001441892E-6,0.447216239632936,
-0.894425868918218)) ;
#126919=DIRECTION('ref_axis',(-0.0169834493203687,0.894296833981071,0.447151803284539)) ;
#126920=DIRECTION('center_axis',(-0.447213595499861,0.894427190999964,-6.53094347128148E-13)) ;
#126921=DIRECTION('ref_axis',(0.894427190999964,0.447213595499861,-1.04079071344172E-9)) ;
#126922=DIRECTION('center_axis',(-0.894427191461906,-0.447213594575977,
5.57669377296248E-9)) ;
#126923=DIRECTION('ref_axis',(0.446767713219282,-0.893535428189512,0.0446435773096007)) ;
#126924=DIRECTION('center_axis',(-1.29699385710222E-8,-0.447213597648892,
-0.894427189925449)) ;
#126925=DIRECTION('ref_axis',(-0.044643580804857,0.893535426885168,-0.446767715478704)) ;
#126926=DIRECTION('center_axis',(2.47817639425258E-16,-1.,0.)) ;
#126927=DIRECTION('ref_axis',(1.,2.47817639425258E-16,0.)) ;
#126928=DIRECTION('center_axis',(-1.29715887066227E-8,-0.447213597649164,
0.894427189925313)) ;
#126929=DIRECTION('ref_axis',(0.0446435808063265,-0.893535426885007,-0.446767715478881)) ;
#126930=DIRECTION('center_axis',(-0.894427191462079,-0.447213594575632,
-5.57881081575365E-9)) ;
#126931=DIRECTION('ref_axis',(0.446767713218975,-0.89353542818955,-0.0446435773119127)) ;
#126932=DIRECTION('center_axis',(-0.447213595499893,0.894427190999948,6.57429044122489E-13)) ;
#126933=DIRECTION('ref_axis',(0.894427190999948,0.447213595499893,-2.76140188029019E-10)) ;
#126934=DIRECTION('center_axis',(-2.76847492423738E-6,0.447215298957762,
0.894426339264702)) ;
#126935=DIRECTION('ref_axis',(0.0170110523543263,-0.894296896128646,0.447150629735068)) ;
#126936=DIRECTION('center_axis',(-0.00225743161003937,0.447523187702742,
0.894269478664515)) ;
#126937=DIRECTION('ref_axis',(-0.00255239339121028,-0.894271422865848,0.44751771756375)) ;
#126938=DIRECTION('center_axis',(0.,0.,1.)) ;
#126939=DIRECTION('ref_axis',(1.,0.,0.)) ;
#126940=DIRECTION('center_axis',(-0.00226103819378627,-0.894269222962206,
-0.447523680455971)) ;
#126941=DIRECTION('ref_axis',(0.00257816448755917,0.447518124037357,-0.894271145529117)) ;
#126942=DIRECTION('center_axis',(-4.29727059150273E-6,-0.894425868918584,
-0.447216239632205)) ;
#126943=DIRECTION('ref_axis',(-0.01698344924275,0.447151803284406,-0.894296833982612)) ;
#126944=DIRECTION('center_axis',(-2.76847490340117E-6,-0.894426339264985,
0.447215298957195)) ;
#126945=DIRECTION('ref_axis',(0.0170110522723741,-0.447150629735124,-0.894296896130177)) ;
#126946=DIRECTION('center_axis',(-0.00225743161207314,-0.894269478664265,
0.447523187703229)) ;
#126947=DIRECTION('ref_axis',(-0.00255239338700126,-0.447517717564248,-0.894271422865611)) ;
#126948=DIRECTION('center_axis',(0.,0.,1.)) ;
#126949=DIRECTION('ref_axis',(1.,0.,0.)) ;
#126950=DIRECTION('center_axis',(-1.29671068301384E-8,0.894427189925688,
-0.447213597648414)) ;
#126951=DIRECTION('ref_axis',(-0.0446435808024942,0.446767715478387,0.893535426885445)) ;
#126952=DIRECTION('center_axis',(-1.29614141328542E-8,0.89442718992613,
0.447213597647529)) ;
#126953=DIRECTION('ref_axis',(0.0446435808017462,-0.446767715477745,0.893535426885803)) ;
#126954=DIRECTION('center_axis',(2.47817639425258E-16,-1.,0.)) ;
#126955=DIRECTION('ref_axis',(1.,2.47817639425258E-16,0.)) ;
#126956=DIRECTION('center_axis',(-0.00226103817312033,0.447523680452633,
-0.894269222963929)) ;
#126957=DIRECTION('ref_axis',(0.00257816447255943,0.894271145530794,0.447518124034094)) ;
#126958=DIRECTION('center_axis',(-4.2972691245385E-6,0.447216239632108,
-0.894425868918632)) ;
#126959=DIRECTION('ref_axis',(-0.0169834493350175,0.894296833981269,0.447151803283587)) ;
#126960=DIRECTION('center_axis',(-0.447213595499861,0.894427190999964,-6.53094347126708E-13)) ;
#126961=DIRECTION('ref_axis',(0.894427190999964,0.447213595499861,-1.07153737410966E-9)) ;
#126962=DIRECTION('center_axis',(-0.894427191461917,-0.447213594575955,
5.57686257371582E-9)) ;
#126963=DIRECTION('ref_axis',(0.446767713219204,-0.893535428189395,0.0446435773127371)) ;
#126964=DIRECTION('center_axis',(-1.2970065171587E-8,-0.447213597648908,
-0.894427189925441)) ;
#126965=DIRECTION('ref_axis',(-0.0446435808026991,0.893535426885249,-0.446767715478758)) ;
#126966=DIRECTION('center_axis',(2.47817639425258E-16,-1.,0.)) ;
#126967=DIRECTION('ref_axis',(1.,2.47817639425258E-16,0.)) ;
#126968=DIRECTION('center_axis',(-1.29716114298014E-8,-0.447213597649167,
0.894427189925311)) ;
#126969=DIRECTION('ref_axis',(0.0446435808059489,-0.893535426885021,-0.446767715478891)) ;
#126970=DIRECTION('center_axis',(-0.894427191462087,-0.447213594575616,
-5.57886600061672E-9)) ;
#126971=DIRECTION('ref_axis',(0.446767713218963,-0.893535428189561,-0.0446435773118126)) ;
#126972=DIRECTION('center_axis',(-0.447213595499893,0.894427190999948,6.57429044123457E-13)) ;
#126973=DIRECTION('ref_axis',(0.894427190999948,0.447213595499893,2.28090461718898E-10)) ;
#126974=DIRECTION('center_axis',(-2.76847537946315E-6,0.447215298958076,
0.894426339264545)) ;
#126975=DIRECTION('ref_axis',(0.0170110523834622,-0.894296896128042,0.447150629735167)) ;
#126976=DIRECTION('center_axis',(-0.0022574316137697,0.447523187703219,
0.894269478664266)) ;
#126977=DIRECTION('ref_axis',(-0.00255239337889119,-0.894271422865627,0.447517717564262)) ;
#126978=DIRECTION('center_axis',(0.,0.,1.)) ;
#126979=DIRECTION('ref_axis',(1.,0.,0.)) ;
#126980=DIRECTION('center_axis',(-0.00226103819029805,-0.894269222962415,
-0.447523680455572)) ;
#126981=DIRECTION('ref_axis',(0.00257816448048495,0.447518124036985,-0.894271145529324)) ;
#126982=DIRECTION('center_axis',(-4.29727144208701E-6,-0.894425868918501,
-0.44721623963237)) ;
#126983=DIRECTION('ref_axis',(-0.0169834492064025,0.44715180328486,-0.894296833983075)) ;
#126984=DIRECTION('center_axis',(-2.76847432632209E-6,-0.894426339264659,
0.447215298957848)) ;
#126985=DIRECTION('ref_axis',(0.0170110525173505,-0.447150629733905,-0.894296896126127)) ;
#126986=DIRECTION('center_axis',(-0.0022574316056552,-0.894269478665014,
0.447523187701765)) ;
#126987=DIRECTION('ref_axis',(-0.00255239336525724,-0.447517717562861,-0.894271422866367)) ;
#126988=DIRECTION('center_axis',(0.,0.,1.)) ;
#126989=DIRECTION('ref_axis',(1.,0.,0.)) ;
#126990=DIRECTION('center_axis',(-1.29670895172406E-8,0.894427189925688,
-0.447213597648414)) ;
#126991=DIRECTION('ref_axis',(-0.0446435808044585,0.446767715478348,0.893535426885366)) ;
#126992=DIRECTION('center_axis',(-1.29656779750599E-8,0.894427189925773,
0.447213597648244)) ;
#126993=DIRECTION('ref_axis',(0.0446435808077213,-0.44676771547817,0.893535426885292)) ;
#126994=DIRECTION('center_axis',(2.47817639425258E-16,-1.,0.)) ;
#126995=DIRECTION('ref_axis',(1.,2.47817639425258E-16,0.)) ;
#126996=DIRECTION('center_axis',(-0.00226103819750544,0.447523680456259,
-0.894269222962053)) ;
#126997=DIRECTION('ref_axis',(0.00257816449032981,0.894271145528972,0.447518124037631)) ;
#126998=DIRECTION('center_axis',(-4.29726910766065E-6,0.447216239631639,
-0.894425868918867)) ;
#126999=DIRECTION('ref_axis',(-0.0169834493967404,0.894296833980566,0.447151803282649)) ;
#127000=DIRECTION('center_axis',(-0.447213595499861,0.894427190999964,-6.5309434712767E-13)) ;
#127001=DIRECTION('ref_axis',(0.894427190999964,0.447213595499861,-2.6192932457417E-9)) ;
#127002=DIRECTION('center_axis',(-0.894427191462423,-0.447213594574943,
5.58297186255583E-9)) ;
#127003=DIRECTION('ref_axis',(0.446767713218366,-0.893535428189637,0.0446435773162759)) ;
#127004=DIRECTION('center_axis',(-1.29684675156914E-8,-0.447213597648659,
-0.894427189925565)) ;
#127005=DIRECTION('ref_axis',(-0.0446435808033256,0.893535426885316,-0.446767715478561)) ;
#127006=DIRECTION('center_axis',(2.47817639425258E-16,-1.,0.)) ;
#127007=DIRECTION('ref_axis',(1.,2.47817639425258E-16,0.)) ;
#127008=DIRECTION('center_axis',(-1.29625973612226E-8,-0.447213597647665,
0.894427189926062)) ;
#127009=DIRECTION('ref_axis',(0.044643580802507,-0.893535426885728,-0.446767715477819)) ;
#127010=DIRECTION('center_axis',(-0.894427191461881,-0.447213594576028,
-5.57641568453782E-9)) ;
#127011=DIRECTION('ref_axis',(0.446767713219317,-0.893535428189484,-0.0446435773098233)) ;
#127012=DIRECTION('center_axis',(-0.447213595499893,0.894427190999948,6.57429044120555E-13)) ;
#127013=DIRECTION('ref_axis',(0.894427190999948,0.447213595499893,1.48077938673105E-9)) ;
#127014=DIRECTION('center_axis',(-2.76847531827434E-6,0.447215298957909,
0.894426339264628)) ;
#127015=DIRECTION('ref_axis',(0.0170110523648983,-0.894296896128409,0.447150629735141)) ;
#127016=DIRECTION('center_axis',(-0.00225743160712761,0.447523187702386,
0.8942694786647)) ;
#127017=DIRECTION('ref_axis',(-0.00255239337382405,-0.894271422866046,0.447517717563453)) ;
#127018=DIRECTION('center_axis',(0.,0.,1.)) ;
#127019=DIRECTION('ref_axis',(1.,0.,0.)) ;
#127020=DIRECTION('center_axis',(-0.00226103819018861,-0.894269222962714,
-0.447523680454975)) ;
#127021=DIRECTION('ref_axis',(0.00257816448743253,0.447518124036366,-0.894271145529614)) ;
#127022=DIRECTION('center_axis',(-4.29726974249564E-6,-0.894425868918509,
-0.447216239632354)) ;
#127023=DIRECTION('ref_axis',(-0.0169834493529471,0.447151803283706,-0.894296833980869)) ;
#127024=DIRECTION('center_axis',(-2.76847442575453E-6,-0.894426339264628,
0.447215298957909)) ;
#127025=DIRECTION('ref_axis',(0.0170110523617927,-0.447150629735151,-0.894296896128463)) ;
#127026=DIRECTION('center_axis',(-0.0022574316083322,-0.894269478664822,
0.447523187702137)) ;
#127027=DIRECTION('ref_axis',(-0.00255239338262315,-0.447517717563174,-0.89427142286616)) ;
#127028=DIRECTION('center_axis',(0.,0.,1.)) ;
#127029=DIRECTION('ref_axis',(1.,0.,0.)) ;
#127030=DIRECTION('center_axis',(-1.29666123305221E-8,0.894427189925724,
-0.447213597648341)) ;
#127031=DIRECTION('ref_axis',(-0.0446435808071081,0.446767715478242,0.893535426885287)) ;
#127032=DIRECTION('center_axis',(-1.29660772537652E-8,0.894427189925737,
0.447213597648315)) ;
#127033=DIRECTION('ref_axis',(0.0446435808082692,-0.446767715478214,0.893535426885243)) ;
#127034=DIRECTION('center_axis',(2.47817639425258E-16,-1.,0.)) ;
#127035=DIRECTION('ref_axis',(1.,2.47817639425258E-16,0.)) ;
#127036=DIRECTION('center_axis',(-0.00226103819164361,0.447523680455419,
-0.894269222962488)) ;
#127037=DIRECTION('ref_axis',(0.00257816448196719,0.894271145529399,0.447518124036826)) ;
#127038=DIRECTION('center_axis',(-4.29726920049817E-6,0.447216239631741,
-0.894425868918816)) ;
#127039=DIRECTION('ref_axis',(-0.0169834493771275,0.894296833980812,0.447151803282901)) ;
#127040=DIRECTION('center_axis',(-0.447213595499861,0.894427190999964,-6.5309434712767E-13)) ;
#127041=DIRECTION('ref_axis',(0.894427190999964,0.447213595499861,-5.78704355583638E-9)) ;
#127042=DIRECTION('center_axis',(-0.894427191462433,-0.447213594574924,
5.58308656049955E-9)) ;
#127043=DIRECTION('ref_axis',(0.446767713218432,-0.893535428189805,0.0446435773122526)) ;
#127044=DIRECTION('center_axis',(-1.29685286518626E-8,-0.447213597648669,
-0.89442718992556)) ;
#127045=DIRECTION('ref_axis',(-0.0446435808020355,0.893535426885364,-0.446767715478595)) ;
#127046=DIRECTION('center_axis',(2.47817639425258E-16,-1.,0.)) ;
#127047=DIRECTION('ref_axis',(1.,2.47817639425258E-16,0.)) ;
#127048=DIRECTION('center_axis',(-1.29626249536512E-8,-0.447213597647691,
0.894427189926049)) ;
#127049=DIRECTION('ref_axis',(0.0446435808039496,-0.893535426885658,-0.446767715477815)) ;
#127050=DIRECTION('center_axis',(-0.894427191461901,-0.447213594575988,
-5.57661424183581E-9)) ;
#127051=DIRECTION('ref_axis',(0.446767713219243,-0.893535428189416,-0.044643577311908)) ;
#127052=DIRECTION('center_axis',(-0.447213595499893,0.894427190999948,6.57429044121523E-13)) ;
#127053=DIRECTION('ref_axis',(0.894427190999948,0.447213595499893,4.15610219187823E-9)) ;
#127054=DIRECTION('center_axis',(-2.7684747923646E-6,0.447215298957608,
0.894426339264779)) ;
#127055=DIRECTION('ref_axis',(0.0170110524133555,-0.894296896127826,0.447150629734463)) ;
#127056=DIRECTION('center_axis',(-0.00225743160937446,0.447523187702693,
0.894269478664541)) ;
#127057=DIRECTION('ref_axis',(-0.00255239335690116,-0.894271422865916,0.44751771756381)) ;
#127058=DIRECTION('center_axis',(0.,0.,1.)) ;
#127059=DIRECTION('ref_axis',(1.,0.,0.)) ;
#127060=DIRECTION('center_axis',(-0.00226103818966992,-0.894269222962751,
-0.447523680454904)) ;
#127061=DIRECTION('ref_axis',(0.00257816448730185,0.447518124036296,-0.894271145529649)) ;
#127062=DIRECTION('center_axis',(-4.29727242902498E-6,-0.894425868917683,
-0.447216239634007)) ;
#127063=DIRECTION('ref_axis',(-0.0169834491710572,0.44715180328678,-0.894296833982786)) ;
#127064=DIRECTION('center_axis',(-2.76847671454323E-6,-0.894426339263924,
0.447215298959317)) ;
#127065=DIRECTION('ref_axis',(0.0170110522880356,-0.447150629737154,-0.894296896128864)) ;
#127066=DIRECTION('center_axis',(-0.00225743160349176,-0.894269478665165,
0.447523187701476)) ;
#127067=DIRECTION('ref_axis',(-0.0025523933684872,-0.447517717562564,-0.894271422866506)) ;
#127068=DIRECTION('center_axis',(0.,0.,1.)) ;
#127069=DIRECTION('ref_axis',(1.,0.,0.)) ;
#127070=DIRECTION('center_axis',(-1.29665203557497E-8,0.89442718992574,
-0.447213597648309)) ;
#127071=DIRECTION('ref_axis',(-0.0446435808065546,0.446767715478225,0.893535426885323)) ;
#127072=DIRECTION('center_axis',(-1.29657120598193E-8,0.894427189925768,
0.447213597648254)) ;
#127073=DIRECTION('ref_axis',(0.0446435808049235,-0.446767715478234,0.8935354268854)) ;
#127074=DIRECTION('center_axis',(2.47817639425258E-16,-1.,0.)) ;
#127075=DIRECTION('ref_axis',(1.,2.47817639425258E-16,0.)) ;
#127076=DIRECTION('center_axis',(-0.00226103819699234,0.447523680456176,
-0.894269222962096)) ;
#127077=DIRECTION('ref_axis',(0.00257816450066049,0.894271145529,0.447518124037516)) ;
#127078=DIRECTION('center_axis',(-4.29727019561894E-6,0.447216239632353,
-0.89442586891851)) ;
#127079=DIRECTION('ref_axis',(-0.01698344932343,0.894296833981315,0.447151803283936)) ;
#127080=DIRECTION('center_axis',(-0.447213595499861,0.894427190999964,-6.53094347129588E-13)) ;
#127081=DIRECTION('ref_axis',(0.894427190999964,0.447213595499861,-3.92952546747532E-9)) ;
#127082=DIRECTION('center_axis',(-0.89442719146245,-0.447213594574889,5.58329918452941E-9)) ;
#127083=DIRECTION('ref_axis',(0.446767713218494,-0.893535428189995,0.0446435773078344)) ;
#127084=DIRECTION('center_axis',(-1.29683685075575E-8,-0.447213597648643,
-0.894427189925573)) ;
#127085=DIRECTION('ref_axis',(-0.0446435808018708,0.89353542688538,-0.446767715478578)) ;
#127086=DIRECTION('center_axis',(2.47817639425258E-16,-1.,0.)) ;
#127087=DIRECTION('ref_axis',(1.,2.47817639425258E-16,0.)) ;
#127088=DIRECTION('center_axis',(-1.29627337002934E-8,-0.447213597647736,
0.894427189926027)) ;
#127089=DIRECTION('ref_axis',(0.0446435808020259,-0.893535426885715,-0.446767715477894)) ;
#127090=DIRECTION('center_axis',(-0.894427191461892,-0.447213594576006,
-5.57650928239589E-9)) ;
#127091=DIRECTION('ref_axis',(0.446767713219069,-0.893535428189034,-0.0446435773213116)) ;
#127092=DIRECTION('center_axis',(-0.447213595499893,0.894427190999948,6.57429044123454E-13)) ;
#127093=DIRECTION('ref_axis',(0.894427190999948,0.447213595499893,-1.55677214764901E-10)) ;
#127094=DIRECTION('center_axis',(-2.76847529691129E-6,0.447215298957874,
0.894426339264646)) ;
#127095=DIRECTION('ref_axis',(0.0170110523595498,-0.894296896128508,0.447150629735146)) ;
#127096=DIRECTION('center_axis',(-0.00225743160737611,0.447523187702446,
0.894269478664669)) ;
#127097=DIRECTION('ref_axis',(-0.00255239334383529,-0.894271422866054,0.447517717563608)) ;
#127098=DIRECTION('center_axis',(0.,0.,1.)) ;
#127099=DIRECTION('ref_axis',(1.,0.,0.)) ;
#127100=DIRECTION('center_axis',(-0.0022610381865632,-0.894269222962977,
-0.447523680454467)) ;
#127101=DIRECTION('ref_axis',(0.00257816448573324,0.447518124035868,-0.894271145529868)) ;
#127102=DIRECTION('center_axis',(-4.29727033961916E-6,-0.894425868918326,
-0.447216239632722)) ;
#127103=DIRECTION('ref_axis',(-0.0169834492560518,0.447151803284818,-0.894296833982153)) ;
#127104=DIRECTION('center_axis',(-2.7684756198651E-6,-0.894426339264261,
0.447215298958644)) ;
#127105=DIRECTION('ref_axis',(0.0170110523558667,-0.447150629735949,-0.894296896128176)) ;
#127106=DIRECTION('center_axis',(-0.00225743160937456,-0.894269478664754,
0.447523187702266)) ;
#127107=DIRECTION('ref_axis',(-0.0025523933836389,-0.447517717563299,-0.894271422866095)) ;
#127108=DIRECTION('center_axis',(0.,0.,1.)) ;
#127109=DIRECTION('ref_axis',(1.,0.,0.)) ;
#127110=DIRECTION('center_axis',(-1.29663126009737E-8,0.894427189925752,
-0.447213597648286)) ;
#127111=DIRECTION('ref_axis',(-0.0446435808089956,0.446767715478161,0.893535426885233)) ;
#127112=DIRECTION('center_axis',(-1.29659598506744E-8,0.894427189925758,
0.447213597648273)) ;
#127113=DIRECTION('ref_axis',(0.044643580808027,-0.446767715478182,0.893535426885271)) ;
#127114=DIRECTION('center_axis',(2.47817639425258E-16,-1.,0.)) ;
#127115=DIRECTION('ref_axis',(1.,2.47817639425258E-16,0.)) ;
#127116=DIRECTION('center_axis',(-0.00226103819759674,0.447523680456259,
-0.894269222962053)) ;
#127117=DIRECTION('ref_axis',(0.00257816448891836,0.894271145528974,0.447518124037636)) ;
#127118=DIRECTION('center_axis',(-4.29726939936379E-6,0.447216239631863,
-0.894425868918755)) ;
#127119=DIRECTION('ref_axis',(-0.0169834493845944,0.894296833980636,0.447151803282969)) ;
#127120=DIRECTION('center_axis',(-0.447213595499861,0.894427190999964,-6.53094347125746E-13)) ;
#127121=DIRECTION('ref_axis',(0.894427190999964,0.447213595499861,-1.24562590126493E-8)) ;
#127122=DIRECTION('center_axis',(-0.894427191462441,-0.447213594574908,
5.58318556863866E-9)) ;
#127123=DIRECTION('ref_axis',(0.446767713218345,-0.893535428189663,0.0446435773159677)) ;
#127124=DIRECTION('center_axis',(-1.29684220693358E-8,-0.447213597648652,
-0.894427189925569)) ;
#127125=DIRECTION('ref_axis',(-0.0446435808038521,0.893535426885298,-0.446767715478545)) ;
#127126=DIRECTION('center_axis',(2.47817639425258E-16,-1.,0.)) ;
#127127=DIRECTION('ref_axis',(1.,2.47817639425258E-16,0.)) ;
#127128=DIRECTION('center_axis',(-1.2962669858985E-8,-0.447213597647703,
0.894427189926043)) ;
#127129=DIRECTION('ref_axis',(0.0446435808048981,-0.893535426885615,-0.446767715477806)) ;
#127130=DIRECTION('center_axis',(-0.894427191461877,-0.447213594576036,
-5.57636158173298E-9)) ;
#127131=DIRECTION('ref_axis',(0.446767713219308,-0.893535428189452,-0.0446435773105443)) ;
#127132=DIRECTION('center_axis',(-0.447213595499893,0.894427190999948,6.57429044121523E-13)) ;
#127133=DIRECTION('ref_axis',(0.894427190999948,0.447213595499893,-2.24965278736678E-9)) ;
#127134=DIRECTION('center_axis',(-2.76847551793095E-6,0.44721529895811,
0.894426339264528)) ;
#127135=DIRECTION('ref_axis',(0.0170110523555864,-0.894296896128449,0.447150629735415)) ;
#127136=DIRECTION('center_axis',(-0.00225743160765807,0.447523187702426,
0.894269478664679)) ;
#127137=DIRECTION('ref_axis',(-0.00255239335397715,-0.894271422866052,0.447517717563555)) ;
#127138=DIRECTION('center_axis',(0.,0.,1.)) ;
#127139=DIRECTION('ref_axis',(1.,0.,0.)) ;
#127140=DIRECTION('center_axis',(-0.00226103818742701,-0.894269222962916,
-0.447523680454585)) ;
#127141=DIRECTION('ref_axis',(0.00257816448798919,0.447518124035978,-0.894271145529806)) ;
#127142=DIRECTION('center_axis',(-4.29727014022669E-6,-0.894425868918387,
-0.447216239632599)) ;
#127143=DIRECTION('ref_axis',(-0.0169834493651296,0.447151803283864,-0.894296833980558)) ;
#127144=DIRECTION('center_axis',(-2.76847587648927E-6,-0.894426339264126,
0.447215298958913)) ;
#127145=DIRECTION('ref_axis',(0.0170110521010361,-0.44715062973816,-0.894296896131918)) ;
#127146=DIRECTION('center_axis',(-0.002257431604729,-0.894269478665109,
0.44752318770158)) ;
#127147=DIRECTION('ref_axis',(-0.00255239336633799,-0.447517717562674,-0.894271422866457)) ;
#127148=DIRECTION('center_axis',(0.,0.,1.)) ;
#127149=DIRECTION('ref_axis',(1.,0.,0.)) ;
#127150=DIRECTION('center_axis',(-1.29667389310869E-8,0.894427189925717,
-0.447213597648356)) ;
#127151=DIRECTION('ref_axis',(-0.0446435808059711,0.446767715478274,0.893535426885327)) ;
#127152=DIRECTION('center_axis',(-1.29552366744308E-8,0.89442718992664,
0.447213597646509)) ;
#127153=DIRECTION('ref_axis',(0.044643580802271,-0.446767715476963,0.893535426886168)) ;
#127154=DIRECTION('center_axis',(2.47817639425258E-16,-1.,0.)) ;
#127155=DIRECTION('ref_axis',(1.,2.47817639425258E-16,0.)) ;
#127156=DIRECTION('center_axis',(-0.00226103816569658,0.447523680451593,
-0.894269222964468)) ;
#127157=DIRECTION('ref_axis',(0.00257816445059052,0.894271145531338,0.447518124033133)) ;
#127158=DIRECTION('center_axis',(-4.297269498005E-6,0.447216239632456,-0.894425868918458)) ;
#127159=DIRECTION('ref_axis',(-0.0169834493446286,0.894296833980946,0.447151803283867)) ;
#127160=DIRECTION('center_axis',(-0.447213595499893,0.894427190999948,-6.57429044115844E-13)) ;
#127161=DIRECTION('ref_axis',(0.894427190999948,0.447213595499893,-4.57322843461801E-9)) ;
#127162=DIRECTION('center_axis',(-0.894427191462495,-0.4472135945748,5.5837520250107E-9)) ;
#127163=DIRECTION('ref_axis',(0.446767713218335,-0.893535428189855,0.0446435773122149)) ;
#127164=DIRECTION('center_axis',(-1.30106076504876E-8,-0.447213597655605,
-0.894427189922092)) ;
#127165=DIRECTION('ref_axis',(-0.0446435808103084,0.893535426882409,-0.446767715483678)) ;
#127166=DIRECTION('center_axis',(2.47817639425258E-16,-1.,0.)) ;
#127167=DIRECTION('ref_axis',(1.,2.47817639425258E-16,0.)) ;
#127168=DIRECTION('center_axis',(-1.29988256823834E-8,-0.447213597653671,
0.894427189923059)) ;
#127169=DIRECTION('ref_axis',(0.0446435808102343,-0.893535426883143,-0.446767715482218)) ;
#127170=DIRECTION('center_axis',(-0.894427191462464,-0.447213594574861,
-5.58340955425016E-9)) ;
#127171=DIRECTION('ref_axis',(0.446767713218182,-0.89353542818943,-0.0446435773222543)) ;
#127172=DIRECTION('center_axis',(-0.447213595500006,0.894427190999892,-3.26547173564688E-13)) ;
#127173=DIRECTION('ref_axis',(0.894427190999892,0.447213595500006,-2.22301428109033E-9)) ;
#127174=DIRECTION('center_axis',(-2.76847765482255E-6,0.447215298952696,
0.894426339267235)) ;
#127175=DIRECTION('ref_axis',(0.0170110523220356,-0.894296896131649,0.44715062973029)) ;
#127176=DIRECTION('center_axis',(-0.00225743165439838,0.447523187712696,
0.894269478659421)) ;
#127177=DIRECTION('ref_axis',(-0.00255239347714828,-0.894271422860785,0.447517717573376)) ;
#127178=DIRECTION('center_axis',(0.,0.,1.)) ;
#127179=DIRECTION('ref_axis',(1.,0.,0.)) ;
#127180=DIRECTION('center_axis',(-0.00226103818036704,-0.894269222963449,
-0.447523680453556)) ;
#127181=DIRECTION('ref_axis',(0.00257816445525296,0.447518124035062,-0.894271145530359)) ;
#127182=DIRECTION('center_axis',(-4.29726820748583E-6,-0.894425868918926,
-0.447216239631522)) ;
#127183=DIRECTION('ref_axis',(-0.0169834493497015,0.447151803282875,-0.894296833981346)) ;
#127184=DIRECTION('center_axis',(-2.7684764734789E-6,-0.894426339263942,
0.447215298959281)) ;
#127185=DIRECTION('ref_axis',(0.0170110521812587,-0.447150629737927,-0.894296896130509)) ;
#127186=DIRECTION('center_axis',(-0.0022574316061112,-0.894269478665011,
0.447523187701769)) ;
#127187=DIRECTION('ref_axis',(-0.00255239340400457,-0.447517717562742,-0.894271422866316)) ;
#127188=DIRECTION('center_axis',(0.,0.,1.)) ;
#127189=DIRECTION('ref_axis',(1.,0.,0.)) ;
#127190=DIRECTION('center_axis',(-1.29525055647508E-8,0.894427189926893,
-0.447213597646003)) ;
#127191=DIRECTION('ref_axis',(-0.0446435807975522,0.44676771547666,0.893535426886555)) ;
#127192=DIRECTION('center_axis',(-1.29551603894678E-8,0.894427189926646,
0.447213597646497)) ;
#127193=DIRECTION('ref_axis',(0.0446435808026582,-0.446767715476946,0.893535426886157)) ;
#127194=DIRECTION('center_axis',(2.47817639425258E-16,-1.,0.)) ;
#127195=DIRECTION('ref_axis',(1.,2.47817639425258E-16,0.)) ;
#127196=DIRECTION('center_axis',(-0.00226103816215286,0.447523680451109,
-0.894269222964719)) ;
#127197=DIRECTION('ref_axis',(0.00257816445691698,0.89427114553157,0.447518124032634)) ;
#127198=DIRECTION('center_axis',(-4.29726929913918E-6,0.447216239632333,
-0.89442586891852)) ;
#127199=DIRECTION('ref_axis',(-0.0169834493712717,0.894296833980605,0.447151803283539)) ;
#127200=DIRECTION('center_axis',(-0.447213595499893,0.894427190999948,-6.57429044119711E-13)) ;
#127201=DIRECTION('ref_axis',(0.894427190999948,0.447213595499893,3.44653255660982E-9)) ;
#127202=DIRECTION('center_axis',(-0.894427191462507,-0.447213594574776,
5.58399386455402E-9)) ;
#127203=DIRECTION('ref_axis',(0.446767713218351,-0.893535428189922,0.0446435773107162)) ;
#127204=DIRECTION('center_axis',(-1.30104853781452E-8,-0.447213597655585,
-0.894427189922102)) ;
#127205=DIRECTION('ref_axis',(-0.0446435808113665,0.893535426882374,-0.446767715483642)) ;
#127206=DIRECTION('center_axis',(1.,1.31418445149758E-16,-2.16840434497101E-16)) ;
#127207=DIRECTION('ref_axis',(-2.16840434497101E-16,-2.8496832747207E-32,
-1.)) ;
#127208=DIRECTION('center_axis',(1.,0.,0.)) ;
#127209=DIRECTION('ref_axis',(0.,0.,-1.)) ;
#127210=DIRECTION('center_axis',(-1.,0.,0.)) ;
#127211=DIRECTION('ref_axis',(0.,0.,1.)) ;
#127212=DIRECTION('center_axis',(-1.31418445149758E-16,1.,0.)) ;
#127213=DIRECTION('ref_axis',(-1.,0.,0.)) ;
#127214=DIRECTION('center_axis',(0.,0.,1.)) ;
#127215=DIRECTION('ref_axis',(-1.,0.,0.)) ;
#127216=DIRECTION('center_axis',(-1.31418445149758E-16,1.,0.)) ;
#127217=DIRECTION('ref_axis',(-1.,-1.31418445149758E-16,0.)) ;
#127218=DIRECTION('center_axis',(-1.31418445149758E-16,1.,0.)) ;
#127219=DIRECTION('ref_axis',(-1.,0.,0.)) ;
#127220=DIRECTION('center_axis',(-1.31418445149758E-16,1.,0.)) ;
#127221=DIRECTION('ref_axis',(-1.,-1.31418445149758E-16,0.)) ;
#127222=DIRECTION('center_axis',(0.,0.,1.)) ;
#127223=DIRECTION('ref_axis',(-1.,0.,0.)) ;
#127224=DIRECTION('center_axis',(-4.33680868994202E-16,-5.69936654944139E-32,
-1.)) ;
#127225=DIRECTION('ref_axis',(-1.,2.47170623787823E-47,4.33680868994202E-16)) ;
#127226=DIRECTION('center_axis',(0.,0.,1.)) ;
#127227=DIRECTION('ref_axis',(1.,0.,0.)) ;
#127228=DIRECTION('center_axis',(-1.31418445149758E-16,-1.,0.)) ;
#127229=DIRECTION('ref_axis',(1.,-1.31418445149758E-16,0.)) ;
#127230=DIRECTION('center_axis',(0.,1.,0.)) ;
#127231=DIRECTION('ref_axis',(0.,0.,1.)) ;
#127232=DIRECTION('center_axis',(-1.,0.,2.16840434497101E-16)) ;
#127233=DIRECTION('ref_axis',(2.16840434497101E-16,0.,1.)) ;
#127234=DIRECTION('center_axis',(-1.,4.33680868994201E-15,0.)) ;
#127235=DIRECTION('ref_axis',(-4.33680868994201E-15,-1.,0.)) ;
#127236=DIRECTION('center_axis',(1.,0.,0.)) ;
#127237=DIRECTION('ref_axis',(0.,0.,-1.)) ;
#127238=DIRECTION('center_axis',(-1.31418445149758E-16,-1.,0.)) ;
#127239=DIRECTION('ref_axis',(1.,-1.31418445149758E-16,0.)) ;
#127240=DIRECTION('center_axis',(0.,1.,0.)) ;
#127241=DIRECTION('ref_axis',(0.,0.,1.)) ;
#127242=DIRECTION('center_axis',(2.16840434497101E-16,2.8496832747207E-32,
1.)) ;
#127243=DIRECTION('ref_axis',(1.,-6.17926559469557E-48,-2.16840434497101E-16)) ;
#127244=DIRECTION('center_axis',(0.,0.,1.)) ;
#127245=DIRECTION('ref_axis',(1.,0.,0.)) ;
#127246=DIRECTION('center_axis',(-1.,-1.31418445149758E-16,-2.16840434497101E-16)) ;
#127247=DIRECTION('ref_axis',(-2.16840434497101E-16,-2.8496832747207E-32,
1.)) ;
#127248=DIRECTION('center_axis',(-1.,0.,0.)) ;
#127249=DIRECTION('ref_axis',(0.,0.,1.)) ;
#127250=DIRECTION('center_axis',(1.,0.,0.)) ;
#127251=DIRECTION('ref_axis',(0.,0.,-1.)) ;
#127252=DIRECTION('center_axis',(-1.31418445149758E-16,1.,0.)) ;
#127253=DIRECTION('ref_axis',(-1.,0.,0.)) ;
#127254=DIRECTION('center_axis',(-1.31418445149758E-16,1.,0.)) ;
#127255=DIRECTION('ref_axis',(-1.,-1.31418445149758E-16,0.)) ;
#127256=DIRECTION('center_axis',(0.,1.,0.)) ;
#127257=DIRECTION('ref_axis',(1.,0.,0.)) ;
#127258=DIRECTION('center_axis',(0.,0.,-1.)) ;
#127259=DIRECTION('ref_axis',(1.,0.,0.)) ;
#127260=DIRECTION('center_axis',(0.,1.,0.)) ;
#127261=DIRECTION('ref_axis',(1.,0.,0.)) ;
#127262=DIRECTION('center_axis',(0.,0.,-1.)) ;
#127263=DIRECTION('ref_axis',(1.,0.,0.)) ;
#127264=DIRECTION('center_axis',(-1.31418445149758E-16,1.,0.)) ;
#127265=DIRECTION('ref_axis',(-1.,0.,0.)) ;
#127266=DIRECTION('center_axis',(-1.31418445149758E-16,1.,0.)) ;
#127267=DIRECTION('ref_axis',(-1.,-1.31418445149758E-16,0.)) ;
#127268=DIRECTION('center_axis',(-1.31418445149758E-16,-1.,0.)) ;
#127269=DIRECTION('ref_axis',(1.,-1.31418445149758E-16,0.)) ;
#127270=DIRECTION('center_axis',(0.,1.,0.)) ;
#127271=DIRECTION('ref_axis',(0.,0.,1.)) ;
#127272=DIRECTION('center_axis',(4.33680868994202E-16,0.,1.)) ;
#127273=DIRECTION('ref_axis',(1.,0.,-4.33680868994202E-16)) ;
#127274=DIRECTION('center_axis',(0.,0.,-1.)) ;
#127275=DIRECTION('ref_axis',(-1.,0.,0.)) ;
#127276=DIRECTION('center_axis',(-2.16840434497101E-16,0.,-1.)) ;
#127277=DIRECTION('ref_axis',(-1.,0.,2.16840434497101E-16)) ;
#127278=DIRECTION('center_axis',(0.,4.33680868994201E-15,-1.)) ;
#127279=DIRECTION('ref_axis',(0.,1.,4.33680868994201E-15)) ;
#127280=DIRECTION('center_axis',(-1.31418445149758E-16,-1.,0.)) ;
#127281=DIRECTION('ref_axis',(1.,-1.31418445149758E-16,0.)) ;
#127282=DIRECTION('center_axis',(0.,1.,0.)) ;
#127283=DIRECTION('ref_axis',(0.,0.,1.)) ;
#127284=DIRECTION('center_axis',(0.,1.,0.)) ;
#127285=DIRECTION('ref_axis',(1.,0.,0.)) ;
#127286=DIRECTION('center_axis',(-1.,0.,0.)) ;
#127287=DIRECTION('ref_axis',(0.,0.,-1.)) ;
#127288=DIRECTION('center_axis',(0.,1.,0.)) ;
#127289=DIRECTION('ref_axis',(1.,0.,0.)) ;
#127290=DIRECTION('center_axis',(1.,0.,-4.33680868994203E-15)) ;
#127291=DIRECTION('ref_axis',(4.33680868994203E-15,0.,1.)) ;
#127292=DIRECTION('center_axis',(1.,0.,2.16840434497101E-16)) ;
#127293=DIRECTION('ref_axis',(2.16840434497101E-16,0.,-1.)) ;
#127294=DIRECTION('center_axis',(0.,1.,0.)) ;
#127295=DIRECTION('ref_axis',(0.,0.,1.)) ;
#127296=DIRECTION('center_axis',(0.,1.,0.)) ;
#127297=DIRECTION('ref_axis',(0.,0.,1.)) ;
#127298=DIRECTION('center_axis',(0.,0.,-1.)) ;
#127299=DIRECTION('ref_axis',(-1.,0.,0.)) ;
#127300=DIRECTION('center_axis',(0.,0.,1.)) ;
#127301=DIRECTION('ref_axis',(1.,0.,0.)) ;
#127302=DIRECTION('center_axis',(0.,0.,-1.)) ;
#127303=DIRECTION('ref_axis',(-1.,0.,0.)) ;
#127304=DIRECTION('center_axis',(0.,1.,0.)) ;
#127305=DIRECTION('ref_axis',(0.,0.,1.)) ;
#127306=DIRECTION('center_axis',(0.,1.,0.)) ;
#127307=DIRECTION('ref_axis',(0.,0.,1.)) ;
#127308=DIRECTION('center_axis',(0.,1.,0.)) ;
#127309=DIRECTION('ref_axis',(1.,0.,0.)) ;
#127310=DIRECTION('center_axis',(-1.,0.,0.)) ;
#127311=DIRECTION('ref_axis',(0.,0.,-1.)) ;
#127312=DIRECTION('center_axis',(0.,1.,0.)) ;
#127313=DIRECTION('ref_axis',(1.,0.,0.)) ;
#127314=DIRECTION('center_axis',(-1.,0.,0.)) ;
#127315=DIRECTION('ref_axis',(0.,0.,-1.)) ;
#127316=DIRECTION('center_axis',(0.,1.,0.)) ;
#127317=DIRECTION('ref_axis',(0.,0.,1.)) ;
#127318=DIRECTION('center_axis',(0.,1.,0.)) ;
#127319=DIRECTION('ref_axis',(0.,0.,1.)) ;
#127320=DIRECTION('center_axis',(-1.,0.,0.)) ;
#127321=DIRECTION('ref_axis',(0.,0.,1.)) ;
#127322=DIRECTION('center_axis',(-1.,0.,0.)) ;
#127323=DIRECTION('ref_axis',(0.,0.,1.)) ;
#127324=DIRECTION('center_axis',(1.,0.,0.)) ;
#127325=DIRECTION('ref_axis',(0.,0.,-1.)) ;
#127326=DIRECTION('center_axis',(-1.,0.,0.)) ;
#127327=DIRECTION('ref_axis',(0.,0.,1.)) ;
#127328=DIRECTION('center_axis',(0.,1.,0.)) ;
#127329=DIRECTION('ref_axis',(0.,0.,1.)) ;
#127330=DIRECTION('center_axis',(0.,1.,0.)) ;
#127331=DIRECTION('ref_axis',(0.,0.,1.)) ;
#127332=DIRECTION('center_axis',(0.,1.,0.)) ;
#127333=DIRECTION('ref_axis',(1.,0.,0.)) ;
#127334=DIRECTION('center_axis',(0.,0.,1.)) ;
#127335=DIRECTION('ref_axis',(-1.,0.,0.)) ;
#127336=DIRECTION('center_axis',(0.,1.,0.)) ;
#127337=DIRECTION('ref_axis',(1.,0.,0.)) ;
#127338=DIRECTION('center_axis',(0.,0.,-1.)) ;
#127339=DIRECTION('ref_axis',(1.,0.,0.)) ;
#127340=DIRECTION('center_axis',(0.,0.,1.)) ;
#127341=DIRECTION('ref_axis',(1.,0.,0.)) ;
#127342=DIRECTION('center_axis',(0.,0.,1.)) ;
#127343=DIRECTION('ref_axis',(1.,0.,0.)) ;
#127344=DIRECTION('center_axis',(0.,0.,-1.)) ;
#127345=DIRECTION('ref_axis',(-1.,0.,0.)) ;
#127346=DIRECTION('center_axis',(-8.67361737988401E-15,0.,1.)) ;
#127347=DIRECTION('ref_axis',(1.,0.,8.67361737988401E-15)) ;
#127348=DIRECTION('center_axis',(1.,0.,0.)) ;
#127349=DIRECTION('ref_axis',(0.,0.,-1.)) ;
#127350=DIRECTION('center_axis',(1.,0.,0.)) ;
#127351=DIRECTION('ref_axis',(0.,0.,-1.)) ;
#127352=DIRECTION('center_axis',(1.,0.,0.)) ;
#127353=DIRECTION('ref_axis',(0.,0.,-1.)) ;
#127354=DIRECTION('center_axis',(1.,0.,8.67361737988401E-15)) ;
#127355=DIRECTION('ref_axis',(8.67361737988401E-15,0.,-1.)) ;
#127356=DIRECTION('center_axis',(1.,0.,0.)) ;
#127357=DIRECTION('ref_axis',(0.,0.,-1.)) ;
#127358=DIRECTION('center_axis',(1.,0.,1.73472347597681E-14)) ;
#127359=DIRECTION('ref_axis',(1.73472347597681E-14,0.,-1.)) ;
#127360=DIRECTION('center_axis',(-1.,0.,0.)) ;
#127361=DIRECTION('ref_axis',(0.,0.,1.)) ;
#127362=DIRECTION('center_axis',(1.,0.,0.)) ;
#127363=DIRECTION('ref_axis',(0.,0.,-1.)) ;
#127364=DIRECTION('center_axis',(1.,0.,0.)) ;
#127365=DIRECTION('ref_axis',(0.,0.,-1.)) ;
#127366=DIRECTION('center_axis',(-8.67361737988409E-15,0.,-1.)) ;
#127367=DIRECTION('ref_axis',(-1.,0.,8.67361737988409E-15)) ;
#127368=DIRECTION('center_axis',(1.,0.,0.)) ;
#127369=DIRECTION('ref_axis',(0.,0.,-1.)) ;
#127370=DIRECTION('center_axis',(-8.67361737988409E-15,0.,1.)) ;
#127371=DIRECTION('ref_axis',(1.,0.,8.67361737988409E-15)) ;
#127372=DIRECTION('center_axis',(0.,0.,-1.)) ;
#127373=DIRECTION('ref_axis',(-1.,0.,0.)) ;
#127374=DIRECTION('center_axis',(-0.422618261740697,5.55398348498559E-17,
0.906307787036651)) ;
#127375=DIRECTION('ref_axis',(0.906307787036651,-7.29829988871486E-33,0.422618261740697)) ;
#127376=DIRECTION('center_axis',(0.422618261740697,-5.55398348498559E-17,
-0.906307787036651)) ;
#127377=DIRECTION('ref_axis',(-0.906307787036651,1.03797877997344E-32,-0.422618261740697)) ;
#127378=DIRECTION('center_axis',(-0.422618261740697,5.55398348498559E-17,
0.906307787036651)) ;
#127379=DIRECTION('ref_axis',(0.906307787036651,-1.03797877997344E-32,0.422618261740697)) ;
#127380=DIRECTION('center_axis',(0.422618261740697,-5.55398348498559E-17,
-0.906307787036651)) ;
#127381=DIRECTION('ref_axis',(-0.906307787036651,1.03797877997344E-32,-0.422618261740697)) ;
#127382=DIRECTION('center_axis',(0.,1.,0.)) ;
#127383=DIRECTION('ref_axis',(1.,0.,0.)) ;
#127384=DIRECTION('center_axis',(2.15682522756814E-14,0.514231796959101,
-0.857651245551602)) ;
#127385=DIRECTION('ref_axis',(-4.48628358333197E-30,-0.857651245551602,
-0.514231796959101)) ;
#127386=DIRECTION('center_axis',(0.,-1.73472347597681E-14,1.)) ;
#127387=DIRECTION('ref_axis',(0.,1.,1.73472347597681E-14)) ;
#127388=DIRECTION('center_axis',(-1.,0.,0.)) ;
#127389=DIRECTION('ref_axis',(0.,0.,-1.)) ;
#127390=DIRECTION('center_axis',(0.,0.,1.)) ;
#127391=DIRECTION('ref_axis',(1.,0.,0.)) ;
#127392=DIRECTION('center_axis',(0.,0.,1.)) ;
#127393=DIRECTION('ref_axis',(1.,0.,0.)) ;
#127394=DIRECTION('center_axis',(-1.,0.,0.)) ;
#127395=DIRECTION('ref_axis',(0.,0.,1.)) ;
#127396=DIRECTION('center_axis',(-1.,0.,0.)) ;
#127397=DIRECTION('ref_axis',(0.,0.,-1.)) ;
#127398=DIRECTION('center_axis',(1.,0.,0.)) ;
#127399=DIRECTION('ref_axis',(0.,0.,-1.)) ;
#127400=DIRECTION('center_axis',(0.,-0.514231796959126,-0.857651245551587)) ;
#127401=DIRECTION('ref_axis',(0.,0.857651245551587,-0.514231796959126)) ;
#127402=DIRECTION('center_axis',(0.,1.,8.97270763436279E-17)) ;
#127403=DIRECTION('ref_axis',(0.,-8.97270763436279E-17,1.)) ;
#127404=DIRECTION('center_axis',(0.,-1.,-8.97270763436279E-17)) ;
#127405=DIRECTION('ref_axis',(0.,-8.97270763436279E-17,1.)) ;
#127406=DIRECTION('center_axis',(0.,-1.,0.)) ;
#127407=DIRECTION('ref_axis',(0.,0.,-1.)) ;
#127408=DIRECTION('center_axis',(0.,1.,0.)) ;
#127409=DIRECTION('ref_axis',(1.,0.,0.)) ;
#127410=DIRECTION('center_axis',(-1.,0.,0.)) ;
#127411=DIRECTION('ref_axis',(0.,0.,-1.)) ;
#127412=DIRECTION('center_axis',(1.,0.,0.)) ;
#127413=DIRECTION('ref_axis',(0.,0.,-1.)) ;
#127414=DIRECTION('center_axis',(0.,-0.514231796959101,0.857651245551602)) ;
#127415=DIRECTION('ref_axis',(0.,0.857651245551602,0.514231796959101)) ;
#127416=DIRECTION('center_axis',(0.,0.,-1.)) ;
#127417=DIRECTION('ref_axis',(1.,0.,0.)) ;
#127418=DIRECTION('center_axis',(0.,1.,0.)) ;
#127419=DIRECTION('ref_axis',(1.,0.,0.)) ;
#127420=DIRECTION('center_axis',(-1.73472347597682E-14,0.,-1.)) ;
#127421=DIRECTION('ref_axis',(1.,0.,-1.73472347597682E-14)) ;
#127422=DIRECTION('center_axis',(-1.,0.,0.)) ;
#127423=DIRECTION('ref_axis',(0.,8.67361737988409E-15,-1.)) ;
#127424=DIRECTION('center_axis',(0.,0.,-1.)) ;
#127425=DIRECTION('ref_axis',(-1.,0.,0.)) ;
#127426=DIRECTION('center_axis',(0.,0.,1.)) ;
#127427=DIRECTION('ref_axis',(-1.,0.,0.)) ;
#127428=DIRECTION('center_axis',(0.,0.,-1.)) ;
#127429=DIRECTION('ref_axis',(-1.,0.,0.)) ;
#127430=DIRECTION('center_axis',(-1.,0.,7.01133629567814E-33)) ;
#127431=DIRECTION('ref_axis',(7.01133629567814E-33,0.,1.)) ;
#127432=DIRECTION('center_axis',(-1.,0.,0.)) ;
#127433=DIRECTION('ref_axis',(0.,0.,1.)) ;
#127434=DIRECTION('center_axis',(0.,0.,-1.)) ;
#127435=DIRECTION('ref_axis',(-1.,0.,0.)) ;
#127436=DIRECTION('center_axis',(-7.01133629567814E-33,8.97270763436279E-17,
-1.)) ;
#127437=DIRECTION('ref_axis',(6.29106707073161E-49,1.,8.97270763436279E-17)) ;
#127438=DIRECTION('center_axis',(1.,0.,0.)) ;
#127439=DIRECTION('ref_axis',(0.,0.,-1.)) ;
#127440=DIRECTION('center_axis',(0.,0.514231796959095,0.857651245551606)) ;
#127441=DIRECTION('ref_axis',(0.,-0.857651245551606,0.514231796959095)) ;
#127442=DIRECTION('center_axis',(-1.,0.,0.)) ;
#127443=DIRECTION('ref_axis',(0.,0.,1.)) ;
#127444=DIRECTION('center_axis',(-1.,0.,0.)) ;
#127445=DIRECTION('ref_axis',(0.,-4.33680868994204E-15,-1.)) ;
#127446=DIRECTION('center_axis',(0.,0.,1.)) ;
#127447=DIRECTION('ref_axis',(1.,0.,0.)) ;
#127448=DIRECTION('center_axis',(0.,0.,-1.)) ;
#127449=DIRECTION('ref_axis',(-1.,0.,0.)) ;
#127450=DIRECTION('center_axis',(0.,-1.,8.97270763436279E-17)) ;
#127451=DIRECTION('ref_axis',(0.,-8.97270763436279E-17,-1.)) ;
#127452=DIRECTION('center_axis',(0.,-1.,8.97270763436279E-17)) ;
#127453=DIRECTION('ref_axis',(0.,-8.97270763436279E-17,-1.)) ;
#127454=DIRECTION('center_axis',(0.,-1.,0.)) ;
#127455=DIRECTION('ref_axis',(0.,0.,-1.)) ;
#127456=DIRECTION('center_axis',(-7.01133629567814E-33,8.97270763436279E-17,
-1.)) ;
#127457=DIRECTION('ref_axis',(0.,1.,0.)) ;
#127458=DIRECTION('center_axis',(0.,-1.,0.)) ;
#127459=DIRECTION('ref_axis',(0.,0.,1.)) ;
#127460=DIRECTION('center_axis',(1.,0.,0.)) ;
#127461=DIRECTION('ref_axis',(0.,0.,-1.)) ;
#127462=DIRECTION('center_axis',(0.,0.,1.)) ;
#127463=DIRECTION('ref_axis',(-1.,0.,0.)) ;
#127464=DIRECTION('center_axis',(0.,1.,0.)) ;
#127465=DIRECTION('ref_axis',(1.,0.,0.)) ;
#127466=DIRECTION('center_axis',(-1.,0.,0.)) ;
#127467=DIRECTION('ref_axis',(0.,0.,-1.)) ;
#127468=DIRECTION('center_axis',(1.,7.81406971160724E-17,0.)) ;
#127469=DIRECTION('ref_axis',(-7.81406971160724E-17,1.,0.)) ;
#127470=DIRECTION('center_axis',(1.,0.,0.)) ;
#127471=DIRECTION('ref_axis',(0.,0.,-1.)) ;
#127472=DIRECTION('center_axis',(1.,0.,0.)) ;
#127473=DIRECTION('ref_axis',(0.,0.,-1.)) ;
#127474=DIRECTION('center_axis',(0.,1.,8.97270763436279E-17)) ;
#127475=DIRECTION('ref_axis',(0.,-8.97270763436279E-17,1.)) ;
#127476=DIRECTION('center_axis',(0.,-1.,0.)) ;
#127477=DIRECTION('ref_axis',(0.,0.,-1.)) ;
#127478=DIRECTION('center_axis',(0.,0.,-1.)) ;
#127479=DIRECTION('ref_axis',(-1.,0.,0.)) ;
#127480=DIRECTION('center_axis',(-7.01133629567814E-33,8.97270763436279E-17,
1.)) ;
#127481=DIRECTION('ref_axis',(-6.29106707073161E-49,-1.,8.97270763436279E-17)) ;
#127482=DIRECTION('center_axis',(-1.,0.,-7.01133629567814E-33)) ;
#127483=DIRECTION('ref_axis',(-7.01133629567814E-33,0.,1.)) ;
#127484=DIRECTION('center_axis',(-1.,0.,0.)) ;
#127485=DIRECTION('ref_axis',(0.,0.,1.)) ;
#127486=DIRECTION('center_axis',(1.,0.,0.)) ;
#127487=DIRECTION('ref_axis',(0.,1.,0.)) ;
#127488=DIRECTION('center_axis',(2.16840434497101E-15,1.,0.)) ;
#127489=DIRECTION('ref_axis',(-1.,2.16840434497101E-15,0.)) ;
#127490=DIRECTION('center_axis',(0.,1.,0.)) ;
#127491=DIRECTION('ref_axis',(1.,0.,0.)) ;
#127492=DIRECTION('center_axis',(0.,0.,-1.)) ;
#127493=DIRECTION('ref_axis',(1.,0.,0.)) ;
#127494=DIRECTION('center_axis',(-1.,0.,0.)) ;
#127495=DIRECTION('ref_axis',(0.,0.,-1.)) ;
#127496=DIRECTION('center_axis',(-7.01133629567814E-33,8.97270763436279E-17,
1.)) ;
#127497=DIRECTION('ref_axis',(0.,-1.,0.)) ;
#127498=DIRECTION('center_axis',(0.,-1.,0.)) ;
#127499=DIRECTION('ref_axis',(0.,0.,1.)) ;
#127500=DIRECTION('center_axis',(7.81406971160724E-17,-1.,-8.97270763436279E-17)) ;
#127501=DIRECTION('ref_axis',(-7.01133629567814E-33,8.97270763436279E-17,
-1.)) ;
#127502=DIRECTION('center_axis',(0.,1.,0.)) ;
#127503=DIRECTION('ref_axis',(0.,0.,1.)) ;
#127504=DIRECTION('center_axis',(-1.,-7.81406971160724E-17,0.)) ;
#127505=DIRECTION('ref_axis',(7.81406971160724E-17,-1.,0.)) ;
#127506=DIRECTION('center_axis',(-1.,-7.81406971160724E-17,0.)) ;
#127507=DIRECTION('ref_axis',(-7.81406971160724E-17,1.,0.)) ;
#127508=DIRECTION('center_axis',(0.,0.,1.)) ;
#127509=DIRECTION('ref_axis',(1.,0.,0.)) ;
#127510=DIRECTION('center_axis',(0.,0.,-1.)) ;
#127511=DIRECTION('ref_axis',(-1.,0.,0.)) ;
#127512=DIRECTION('center_axis',(0.,-1.,8.97270763436279E-17)) ;
#127513=DIRECTION('ref_axis',(0.,-8.97270763436279E-17,-1.)) ;
#127514=DIRECTION('center_axis',(0.,-1.,0.)) ;
#127515=DIRECTION('ref_axis',(0.,0.,-1.)) ;
#127516=DIRECTION('center_axis',(1.,7.81406971160724E-17,0.)) ;
#127517=DIRECTION('ref_axis',(0.,1.,0.)) ;
#127518=DIRECTION('center_axis',(0.,0.,1.)) ;
#127519=DIRECTION('ref_axis',(-1.,0.,0.)) ;
#127520=DIRECTION('center_axis',(0.,1.,0.)) ;
#127521=DIRECTION('ref_axis',(1.,0.,0.)) ;
#127522=DIRECTION('center_axis',(-1.,0.,0.)) ;
#127523=DIRECTION('ref_axis',(0.,0.,-1.)) ;
#127524=DIRECTION('center_axis',(0.,0.,-1.)) ;
#127525=DIRECTION('ref_axis',(-1.,0.,0.)) ;
#127526=DIRECTION('center_axis',(0.,0.,1.)) ;
#127527=DIRECTION('ref_axis',(1.,0.,0.)) ;
#127528=DIRECTION('center_axis',(-1.,-7.81406971160724E-17,0.)) ;
#127529=DIRECTION('ref_axis',(7.81406971160724E-17,-1.,0.)) ;
#127530=DIRECTION('center_axis',(-1.,-7.81406971160724E-17,0.)) ;
#127531=DIRECTION('ref_axis',(-7.81406971160724E-17,1.,0.)) ;
#127532=DIRECTION('center_axis',(1.,7.81406971160724E-17,0.)) ;
#127533=DIRECTION('ref_axis',(-7.81406971160724E-17,1.,0.)) ;
#127534=DIRECTION('center_axis',(1.,0.,0.)) ;
#127535=DIRECTION('ref_axis',(0.,0.,-1.)) ;
#127536=DIRECTION('center_axis',(1.,0.,0.)) ;
#127537=DIRECTION('ref_axis',(0.,0.,-1.)) ;
#127538=DIRECTION('center_axis',(3.78638272950961E-32,-4.8455963016112E-16,
-1.)) ;
#127539=DIRECTION('ref_axis',(1.83472821505963E-47,1.,-4.8455963016112E-16)) ;
#127540=DIRECTION('center_axis',(3.78638272950961E-32,-4.8455963016112E-16,
-1.)) ;
#127541=DIRECTION('ref_axis',(1.83472821505963E-47,1.,-4.8455963016112E-16)) ;
#127542=DIRECTION('center_axis',(0.,0.,-1.)) ;
#127543=DIRECTION('ref_axis',(-1.,0.,0.)) ;
#127544=DIRECTION('center_axis',(1.,7.81406971160724E-17,0.)) ;
#127545=DIRECTION('ref_axis',(0.,1.,0.)) ;
#127546=DIRECTION('center_axis',(0.,-1.,0.)) ;
#127547=DIRECTION('ref_axis',(0.,0.,1.)) ;
#127548=DIRECTION('center_axis',(0.,1.,0.)) ;
#127549=DIRECTION('ref_axis',(1.,0.,0.)) ;
#127550=DIRECTION('center_axis',(0.,1.,0.)) ;
#127551=DIRECTION('ref_axis',(0.,0.,-1.)) ;
#127552=DIRECTION('center_axis',(-7.81406971160724E-17,1.,-8.97270763436279E-17)) ;
#127553=DIRECTION('ref_axis',(-7.01133629567814E-33,8.97270763436279E-17,
1.)) ;
#127554=DIRECTION('center_axis',(0.,-1.,0.)) ;
#127555=DIRECTION('ref_axis',(0.,0.,-1.)) ;
#127556=DIRECTION('center_axis',(0.,1.,0.)) ;
#127557=DIRECTION('ref_axis',(0.,0.,1.)) ;
#127558=DIRECTION('center_axis',(0.,-1.,0.)) ;
#127559=DIRECTION('ref_axis',(0.,0.,-1.)) ;
#127560=DIRECTION('center_axis',(0.,-1.,0.)) ;
#127561=DIRECTION('ref_axis',(0.,0.,-1.)) ;
#127562=DIRECTION('center_axis',(0.,1.,0.)) ;
#127563=DIRECTION('ref_axis',(1.,0.,0.)) ;
#127564=DIRECTION('center_axis',(0.,0.,1.)) ;
#127565=DIRECTION('ref_axis',(-1.,0.,0.)) ;
#127566=DIRECTION('center_axis',(1.,0.,0.)) ;
#127567=DIRECTION('ref_axis',(0.,0.,1.)) ;
#127568=DIRECTION('center_axis',(0.,-1.,0.)) ;
#127569=DIRECTION('ref_axis',(0.,0.,-1.)) ;
#127570=DIRECTION('center_axis',(0.,1.,0.)) ;
#127571=DIRECTION('ref_axis',(0.,0.,1.)) ;
#127572=DIRECTION('center_axis',(0.,-1.,0.)) ;
#127573=DIRECTION('ref_axis',(0.,0.,-1.)) ;
#127574=DIRECTION('center_axis',(-1.,0.,2.16840434497101E-16)) ;
#127575=DIRECTION('ref_axis',(2.16840434497101E-16,0.,1.)) ;
#127576=DIRECTION('center_axis',(1.,0.,0.)) ;
#127577=DIRECTION('ref_axis',(0.,0.,-1.)) ;
#127578=DIRECTION('center_axis',(-2.16840434497101E-16,0.,1.)) ;
#127579=DIRECTION('ref_axis',(1.,0.,2.16840434497101E-16)) ;
#127580=DIRECTION('center_axis',(0.,-1.7347234759768E-14,1.)) ;
#127581=DIRECTION('ref_axis',(0.,-1.,-1.7347234759768E-14)) ;
#127582=DIRECTION('center_axis',(0.,1.,0.)) ;
#127583=DIRECTION('ref_axis',(0.,0.,1.)) ;
#127584=DIRECTION('center_axis',(0.,-1.,0.)) ;
#127585=DIRECTION('ref_axis',(0.,0.,-1.)) ;
#127586=DIRECTION('center_axis',(0.,1.,0.)) ;
#127587=DIRECTION('ref_axis',(1.,0.,0.)) ;
#127588=DIRECTION('center_axis',(0.,0.,1.)) ;
#127589=DIRECTION('ref_axis',(-1.,0.,0.)) ;
#127590=DIRECTION('center_axis',(0.,1.,0.)) ;
#127591=DIRECTION('ref_axis',(1.,0.,0.)) ;
#127592=DIRECTION('center_axis',(1.,0.,0.)) ;
#127593=DIRECTION('ref_axis',(0.,0.,1.)) ;
#127594=DIRECTION('center_axis',(0.,0.,-1.)) ;
#127595=DIRECTION('ref_axis',(-1.,0.,0.)) ;
#127596=DIRECTION('center_axis',(-1.7347234759768E-14,0.,1.)) ;
#127597=DIRECTION('ref_axis',(1.,0.,1.7347234759768E-14)) ;
#127598=DIRECTION('center_axis',(1.,0.,2.16840434497101E-16)) ;
#127599=DIRECTION('ref_axis',(2.16840434497101E-16,0.,-1.)) ;
#127600=DIRECTION('center_axis',(1.,0.,0.)) ;
#127601=DIRECTION('ref_axis',(0.,0.,-1.)) ;
#127602=DIRECTION('center_axis',(0.,1.,0.)) ;
#127603=DIRECTION('ref_axis',(1.,0.,0.)) ;
#127604=DIRECTION('center_axis',(0.,1.,0.)) ;
#127605=DIRECTION('ref_axis',(0.,0.,-1.)) ;
#127606=DIRECTION('center_axis',(0.,1.,0.)) ;
#127607=DIRECTION('ref_axis',(0.,0.,1.)) ;
#127608=DIRECTION('center_axis',(0.,1.,0.)) ;
#127609=DIRECTION('ref_axis',(0.,0.,1.)) ;
#127610=DIRECTION('center_axis',(-0.942809041582064,-0.235702260395514,
0.235702260395514)) ;
#127611=DIRECTION('ref_axis',(0.242535625036331,-0.970142500145332,4.49011373492972E-16)) ;
#127612=DIRECTION('center_axis',(-0.970142500145332,-0.242535625036331,
-2.10366121255617E-15)) ;
#127613=DIRECTION('ref_axis',(0.242535625036331,-0.970142500145332,-4.47980524894761E-30)) ;
#127614=DIRECTION('center_axis',(0.970142500145333,0.24253562503633,0.)) ;
#127615=DIRECTION('ref_axis',(-0.24253562503633,0.970142500145333,0.)) ;
#127616=DIRECTION('center_axis',(-0.970142500145333,-0.242535625036331,
-8.41464485022468E-15)) ;
#127617=DIRECTION('ref_axis',(0.242535625036331,-0.970142500145332,-4.3372965844578E-30)) ;
#127618=DIRECTION('center_axis',(0.879462917689188,0.219865729422294,-0.42214220049081)) ;
#127619=DIRECTION('ref_axis',(-0.432731067584771,-5.39224131925863E-16,
-0.901523057468274)) ;
#127620=DIRECTION('center_axis',(0.879462917689187,0.219865729422303,-0.422142200490807)) ;
#127621=DIRECTION('ref_axis',(-0.432731067584769,-6.68249977502363E-17,
-0.901523057468275)) ;
#127622=DIRECTION('center_axis',(0.,1.,0.)) ;
#127623=DIRECTION('ref_axis',(1.,0.,0.)) ;
#127624=DIRECTION('center_axis',(0.,-1.,0.)) ;
#127625=DIRECTION('ref_axis',(0.,0.,1.)) ;
#127626=DIRECTION('center_axis',(0.,-1.,0.)) ;
#127627=DIRECTION('ref_axis',(0.,0.,-1.)) ;
#127628=DIRECTION('center_axis',(-4.51750905202295E-15,-1.,2.168404344971E-15)) ;
#127629=DIRECTION('ref_axis',(1.,-4.51750905202295E-15,3.91831450274155E-31)) ;
#127630=DIRECTION('center_axis',(0.669589480006976,-0.669589480006974,-0.321402950403349)) ;
#127631=DIRECTION('ref_axis',(0.707106781186547,0.707106781186548,5.45170614306381E-16)) ;
#127632=DIRECTION('center_axis',(0.669589480006977,-0.669589480006977,-0.321402950403339)) ;
#127633=DIRECTION('ref_axis',(0.707106781186548,0.707106781186548,1.13950759497276E-17)) ;
#127634=DIRECTION('center_axis',(0.,1.,0.)) ;
#127635=DIRECTION('ref_axis',(1.,0.,0.)) ;
#127636=DIRECTION('center_axis',(0.707106781186541,-0.707106781186554,0.)) ;
#127637=DIRECTION('ref_axis',(-0.707106781186554,-0.707106781186541,0.)) ;
#127638=DIRECTION('center_axis',(0.707106781186549,-0.707106781186546,0.)) ;
#127639=DIRECTION('ref_axis',(0.707106781186546,0.707106781186549,0.)) ;
#127640=DIRECTION('center_axis',(0.707106781186548,-0.707106781186548,-1.53329341668337E-15)) ;
#127641=DIRECTION('ref_axis',(0.707106781186548,0.707106781186548,5.40855345051871E-33)) ;
#127642=DIRECTION('center_axis',(0.577350269189623,-0.577350269189623,-0.577350269189631)) ;
#127643=DIRECTION('ref_axis',(-0.707106781186552,4.49290806924424E-16,-0.707106781186543)) ;
#127644=DIRECTION('center_axis',(-0.577350269189344,0.577350269189586,-0.577350269189947)) ;
#127645=DIRECTION('ref_axis',(1.30446081606812E-15,0.707106781186769,0.707106781186326)) ;
#127646=DIRECTION('center_axis',(-0.707106781186548,0.707106781186548,7.66646708341679E-15)) ;
#127647=DIRECTION('ref_axis',(-0.707106781186548,-0.707106781186548,-2.87534730433018E-31)) ;
#127648=DIRECTION('center_axis',(-0.707106781186549,0.707106781186546,0.)) ;
#127649=DIRECTION('ref_axis',(-0.707106781186546,-0.707106781186549,0.)) ;
#127650=DIRECTION('center_axis',(-0.707106781186548,0.707106781186548,9.19976050010028E-15)) ;
#127651=DIRECTION('ref_axis',(-0.707106781186548,-0.707106781186548,6.30681275467002E-31)) ;
#127652=DIRECTION('center_axis',(-0.669589480006976,0.669589480006974,-0.321402950403349)) ;
#127653=DIRECTION('ref_axis',(-0.707106781186547,-0.707106781186548,5.45170614306381E-16)) ;
#127654=DIRECTION('center_axis',(0.669589480006969,-0.669589480006982,0.321402950403346)) ;
#127655=DIRECTION('ref_axis',(0.707106781186554,0.707106781186541,-7.82217332695337E-17)) ;
#127656=DIRECTION('center_axis',(0.,1.,0.)) ;
#127657=DIRECTION('ref_axis',(1.,0.,0.)) ;
#127658=DIRECTION('center_axis',(0.,1.,0.)) ;
#127659=DIRECTION('ref_axis',(0.,0.,-1.)) ;
#127660=DIRECTION('center_axis',(0.,-1.,0.)) ;
#127661=DIRECTION('ref_axis',(0.,0.,-1.)) ;
#127662=DIRECTION('center_axis',(0.,1.,0.)) ;
#127663=DIRECTION('ref_axis',(0.,0.,1.)) ;
#127664=DIRECTION('center_axis',(-0.879462917689188,-0.219865729422294,
-0.42214220049081)) ;
#127665=DIRECTION('ref_axis',(-0.432731067584771,1.71515946658E-16,0.901523057468274)) ;
#127666=DIRECTION('center_axis',(0.879462917689194,0.219865729422297,0.422142200490796)) ;
#127667=DIRECTION('ref_axis',(0.432731067584757,1.37134448890593E-15,-0.901523057468281)) ;
#127668=DIRECTION('center_axis',(0.,1.,0.)) ;
#127669=DIRECTION('ref_axis',(1.,0.,0.)) ;
#127670=DIRECTION('center_axis',(0.970142500145328,0.242535625036349,0.)) ;
#127671=DIRECTION('ref_axis',(0.242535625036349,-0.970142500145328,0.)) ;
#127672=DIRECTION('center_axis',(-0.970142500145333,-0.24253562503633,0.)) ;
#127673=DIRECTION('ref_axis',(0.24253562503633,-0.970142500145333,0.)) ;
#127674=DIRECTION('center_axis',(0.970142500145332,0.242535625036331,-2.10366121255617E-15)) ;
#127675=DIRECTION('ref_axis',(-0.242535625036331,0.970142500145332,-4.47980524894761E-30)) ;
#127676=DIRECTION('center_axis',(0.942809041582064,0.235702260395514,0.235702260395514)) ;
#127677=DIRECTION('ref_axis',(-0.242535625036331,0.970142500145332,4.49011373492972E-16)) ;
#127678=DIRECTION('center_axis',(0.,-1.,0.)) ;
#127679=DIRECTION('ref_axis',(0.,0.,-1.)) ;
#127680=DIRECTION('center_axis',(-1.,0.,-8.67361737988394E-15)) ;
#127681=DIRECTION('ref_axis',(-8.67361737988394E-15,0.,1.)) ;
#127682=DIRECTION('center_axis',(0.,0.,-1.)) ;
#127683=DIRECTION('ref_axis',(-1.,0.,0.)) ;
#127684=DIRECTION('center_axis',(0.,0.,-1.)) ;
#127685=DIRECTION('ref_axis',(-1.,0.,0.)) ;
#127686=DIRECTION('center_axis',(0.,8.67361737988405E-15,-1.)) ;
#127687=DIRECTION('ref_axis',(0.,1.,8.67361737988405E-15)) ;
#127688=DIRECTION('center_axis',(1.,0.,0.)) ;
#127689=DIRECTION('ref_axis',(0.,0.,-1.)) ;
#127690=DIRECTION('center_axis',(-1.,0.,0.)) ;
#127691=DIRECTION('ref_axis',(0.,0.,1.)) ;
#127692=DIRECTION('center_axis',(0.,-1.,0.)) ;
#127693=DIRECTION('ref_axis',(0.,0.,-1.)) ;
#127694=DIRECTION('center_axis',(-1.,0.,0.)) ;
#127695=DIRECTION('ref_axis',(0.,0.,1.)) ;
#127696=DIRECTION('center_axis',(0.,-1.,0.)) ;
#127697=DIRECTION('ref_axis',(0.,0.,-1.)) ;
#127698=DIRECTION('center_axis',(0.,0.,-1.)) ;
#127699=DIRECTION('ref_axis',(-1.,0.,0.)) ;
#127700=DIRECTION('center_axis',(-1.,0.,0.)) ;
#127701=DIRECTION('ref_axis',(0.,0.,1.)) ;
#127702=DIRECTION('center_axis',(-1.,1.73472347597681E-14,0.)) ;
#127703=DIRECTION('ref_axis',(-1.73472347597681E-14,-1.,0.)) ;
#127704=DIRECTION('center_axis',(0.,0.,1.)) ;
#127705=DIRECTION('ref_axis',(1.,0.,0.)) ;
#127706=DIRECTION('center_axis',(-8.67361737988409E-15,0.,-1.)) ;
#127707=DIRECTION('ref_axis',(-1.,0.,8.67361737988409E-15)) ;
#127708=DIRECTION('center_axis',(0.,-1.,0.)) ;
#127709=DIRECTION('ref_axis',(0.,0.,-1.)) ;
#127710=DIRECTION('center_axis',(0.,-1.,0.)) ;
#127711=DIRECTION('ref_axis',(0.,0.,-1.)) ;
#127712=DIRECTION('center_axis',(0.,-1.,0.)) ;
#127713=DIRECTION('ref_axis',(0.,0.,-1.)) ;
#127714=DIRECTION('center_axis',(0.,0.,1.)) ;
#127715=DIRECTION('ref_axis',(1.,0.,0.)) ;
#127716=DIRECTION('center_axis',(0.,0.,-1.)) ;
#127717=DIRECTION('ref_axis',(-1.,0.,0.)) ;
#127718=DIRECTION('center_axis',(0.,0.,1.)) ;
#127719=DIRECTION('ref_axis',(1.,0.,0.)) ;
#127720=DIRECTION('center_axis',(0.,-1.,0.)) ;
#127721=DIRECTION('ref_axis',(0.,0.,-1.)) ;
#127722=DIRECTION('center_axis',(0.,-1.,0.)) ;
#127723=DIRECTION('ref_axis',(0.,0.,-1.)) ;
#127724=DIRECTION('center_axis',(0.,1.,0.)) ;
#127725=DIRECTION('ref_axis',(1.,0.,0.)) ;
#127726=DIRECTION('center_axis',(-1.,0.,0.)) ;
#127727=DIRECTION('ref_axis',(0.,0.,-1.)) ;
#127728=DIRECTION('center_axis',(0.,1.,0.)) ;
#127729=DIRECTION('ref_axis',(1.,0.,0.)) ;
#127730=DIRECTION('center_axis',(-1.,0.,0.)) ;
#127731=DIRECTION('ref_axis',(0.,0.,-1.)) ;
#127732=DIRECTION('center_axis',(0.,-1.,0.)) ;
#127733=DIRECTION('ref_axis',(0.,0.,-1.)) ;
#127734=DIRECTION('center_axis',(0.,-1.,0.)) ;
#127735=DIRECTION('ref_axis',(0.,0.,-1.)) ;
#127736=DIRECTION('center_axis',(-1.,0.,0.)) ;
#127737=DIRECTION('ref_axis',(0.,0.,1.)) ;
#127738=DIRECTION('center_axis',(-1.,0.,0.)) ;
#127739=DIRECTION('ref_axis',(0.,0.,1.)) ;
#127740=DIRECTION('center_axis',(1.,0.,0.)) ;
#127741=DIRECTION('ref_axis',(0.,0.,-1.)) ;
#127742=DIRECTION('center_axis',(-1.,0.,0.)) ;
#127743=DIRECTION('ref_axis',(0.,0.,1.)) ;
#127744=DIRECTION('center_axis',(0.,-1.,0.)) ;
#127745=DIRECTION('ref_axis',(0.,0.,-1.)) ;
#127746=DIRECTION('center_axis',(0.,-1.,0.)) ;
#127747=DIRECTION('ref_axis',(0.,0.,-1.)) ;
#127748=DIRECTION('center_axis',(0.,1.,0.)) ;
#127749=DIRECTION('ref_axis',(1.,0.,0.)) ;
#127750=DIRECTION('center_axis',(0.,0.,-1.)) ;
#127751=DIRECTION('ref_axis',(1.,0.,0.)) ;
#127752=DIRECTION('center_axis',(0.,1.,0.)) ;
#127753=DIRECTION('ref_axis',(1.,0.,0.)) ;
#127754=DIRECTION('center_axis',(0.,0.,1.)) ;
#127755=DIRECTION('ref_axis',(-1.,0.,0.)) ;
#127756=DIRECTION('center_axis',(0.,0.,-1.)) ;
#127757=DIRECTION('ref_axis',(-1.,0.,0.)) ;
#127758=DIRECTION('center_axis',(1.,1.31418445149758E-16,-2.16840434497101E-16)) ;
#127759=DIRECTION('ref_axis',(-2.16840434497101E-16,-2.8496832747207E-32,
-1.)) ;
#127760=DIRECTION('center_axis',(1.,0.,0.)) ;
#127761=DIRECTION('ref_axis',(0.,0.,-1.)) ;
#127762=DIRECTION('center_axis',(-1.,0.,0.)) ;
#127763=DIRECTION('ref_axis',(0.,0.,1.)) ;
#127764=DIRECTION('center_axis',(-1.31418445149758E-16,1.,0.)) ;
#127765=DIRECTION('ref_axis',(-1.,0.,0.)) ;
#127766=DIRECTION('center_axis',(0.,0.,1.)) ;
#127767=DIRECTION('ref_axis',(-1.,0.,0.)) ;
#127768=DIRECTION('center_axis',(-1.31418445149758E-16,1.,0.)) ;
#127769=DIRECTION('ref_axis',(-1.,-1.31418445149758E-16,0.)) ;
#127770=DIRECTION('center_axis',(-1.31418445149758E-16,1.,0.)) ;
#127771=DIRECTION('ref_axis',(-1.,0.,0.)) ;
#127772=DIRECTION('center_axis',(-1.31418445149758E-16,1.,0.)) ;
#127773=DIRECTION('ref_axis',(-1.,-1.31418445149758E-16,0.)) ;
#127774=DIRECTION('center_axis',(0.,0.,1.)) ;
#127775=DIRECTION('ref_axis',(-1.,0.,0.)) ;
#127776=DIRECTION('center_axis',(-4.33680868994202E-16,-5.69936654944139E-32,
-1.)) ;
#127777=DIRECTION('ref_axis',(-1.,2.47170623787823E-47,4.33680868994202E-16)) ;
#127778=DIRECTION('center_axis',(0.,0.,1.)) ;
#127779=DIRECTION('ref_axis',(1.,0.,0.)) ;
#127780=DIRECTION('center_axis',(-1.31418445149758E-16,-1.,0.)) ;
#127781=DIRECTION('ref_axis',(1.,-1.31418445149758E-16,0.)) ;
#127782=DIRECTION('center_axis',(0.,1.,0.)) ;
#127783=DIRECTION('ref_axis',(0.,0.,1.)) ;
#127784=DIRECTION('center_axis',(-1.,0.,2.16840434497101E-16)) ;
#127785=DIRECTION('ref_axis',(2.16840434497101E-16,0.,1.)) ;
#127786=DIRECTION('center_axis',(-1.,0.,0.)) ;
#127787=DIRECTION('ref_axis',(0.,0.,1.)) ;
#127788=DIRECTION('center_axis',(1.,0.,0.)) ;
#127789=DIRECTION('ref_axis',(0.,0.,-1.)) ;
#127790=DIRECTION('center_axis',(-1.31418445149758E-16,-1.,0.)) ;
#127791=DIRECTION('ref_axis',(1.,-1.31418445149758E-16,0.)) ;
#127792=DIRECTION('center_axis',(0.,1.,0.)) ;
#127793=DIRECTION('ref_axis',(0.,0.,1.)) ;
#127794=DIRECTION('center_axis',(2.16840434497101E-16,2.8496832747207E-32,
1.)) ;
#127795=DIRECTION('ref_axis',(1.,-6.17926559469557E-48,-2.16840434497101E-16)) ;
#127796=DIRECTION('center_axis',(0.,0.,1.)) ;
#127797=DIRECTION('ref_axis',(1.,0.,0.)) ;
#127798=DIRECTION('center_axis',(-1.,-1.31418445149758E-16,-2.16840434497101E-16)) ;
#127799=DIRECTION('ref_axis',(-2.16840434497101E-16,-2.8496832747207E-32,
1.)) ;
#127800=DIRECTION('center_axis',(-1.,0.,0.)) ;
#127801=DIRECTION('ref_axis',(0.,0.,1.)) ;
#127802=DIRECTION('center_axis',(1.,0.,0.)) ;
#127803=DIRECTION('ref_axis',(0.,0.,-1.)) ;
#127804=DIRECTION('center_axis',(-1.31418445149758E-16,1.,0.)) ;
#127805=DIRECTION('ref_axis',(-1.,0.,0.)) ;
#127806=DIRECTION('center_axis',(-1.31418445149758E-16,1.,0.)) ;
#127807=DIRECTION('ref_axis',(-1.,-1.31418445149758E-16,0.)) ;
#127808=DIRECTION('center_axis',(0.,1.,0.)) ;
#127809=DIRECTION('ref_axis',(1.,0.,0.)) ;
#127810=DIRECTION('center_axis',(0.,0.,-1.)) ;
#127811=DIRECTION('ref_axis',(1.,0.,0.)) ;
#127812=DIRECTION('center_axis',(0.,1.,0.)) ;
#127813=DIRECTION('ref_axis',(1.,0.,0.)) ;
#127814=DIRECTION('center_axis',(0.,0.,-1.)) ;
#127815=DIRECTION('ref_axis',(1.,0.,0.)) ;
#127816=DIRECTION('center_axis',(-1.31418445149758E-16,1.,0.)) ;
#127817=DIRECTION('ref_axis',(-1.,0.,0.)) ;
#127818=DIRECTION('center_axis',(-1.31418445149758E-16,1.,0.)) ;
#127819=DIRECTION('ref_axis',(-1.,-1.31418445149758E-16,0.)) ;
#127820=DIRECTION('center_axis',(-1.31418445149758E-16,-1.,0.)) ;
#127821=DIRECTION('ref_axis',(1.,-1.31418445149758E-16,0.)) ;
#127822=DIRECTION('center_axis',(0.,1.,0.)) ;
#127823=DIRECTION('ref_axis',(0.,0.,1.)) ;
#127824=DIRECTION('center_axis',(4.33680868994202E-16,0.,1.)) ;
#127825=DIRECTION('ref_axis',(1.,0.,-4.33680868994202E-16)) ;
#127826=DIRECTION('center_axis',(0.,0.,-1.)) ;
#127827=DIRECTION('ref_axis',(-1.,0.,0.)) ;
#127828=DIRECTION('center_axis',(-2.16840434497101E-16,0.,-1.)) ;
#127829=DIRECTION('ref_axis',(-1.,0.,2.16840434497101E-16)) ;
#127830=DIRECTION('center_axis',(0.,0.,-1.)) ;
#127831=DIRECTION('ref_axis',(-1.,0.,0.)) ;
#127832=DIRECTION('center_axis',(-1.31418445149758E-16,-1.,0.)) ;
#127833=DIRECTION('ref_axis',(1.,-1.31418445149758E-16,0.)) ;
#127834=DIRECTION('center_axis',(0.,1.,0.)) ;
#127835=DIRECTION('ref_axis',(0.,0.,1.)) ;
#127836=DIRECTION('center_axis',(0.,1.,0.)) ;
#127837=DIRECTION('ref_axis',(1.,0.,0.)) ;
#127838=DIRECTION('center_axis',(-1.,0.,0.)) ;
#127839=DIRECTION('ref_axis',(0.,0.,-1.)) ;
#127840=DIRECTION('center_axis',(0.,1.,0.)) ;
#127841=DIRECTION('ref_axis',(1.,0.,0.)) ;
#127842=DIRECTION('center_axis',(1.,0.,0.)) ;
#127843=DIRECTION('ref_axis',(0.,0.,1.)) ;
#127844=DIRECTION('center_axis',(1.,0.,2.16840434497101E-16)) ;
#127845=DIRECTION('ref_axis',(2.16840434497101E-16,0.,-1.)) ;
#127846=DIRECTION('center_axis',(0.,1.,0.)) ;
#127847=DIRECTION('ref_axis',(0.,0.,1.)) ;
#127848=DIRECTION('center_axis',(0.,1.,0.)) ;
#127849=DIRECTION('ref_axis',(0.,0.,1.)) ;
#127850=DIRECTION('center_axis',(0.,0.,-1.)) ;
#127851=DIRECTION('ref_axis',(-1.,0.,0.)) ;
#127852=DIRECTION('center_axis',(0.,0.,1.)) ;
#127853=DIRECTION('ref_axis',(1.,0.,0.)) ;
#127854=DIRECTION('center_axis',(0.,0.,-1.)) ;
#127855=DIRECTION('ref_axis',(-1.,0.,0.)) ;
#127856=DIRECTION('center_axis',(0.,1.,0.)) ;
#127857=DIRECTION('ref_axis',(0.,0.,1.)) ;
#127858=DIRECTION('center_axis',(0.,1.,0.)) ;
#127859=DIRECTION('ref_axis',(0.,0.,1.)) ;
#127860=DIRECTION('center_axis',(0.,1.,0.)) ;
#127861=DIRECTION('ref_axis',(1.,0.,0.)) ;
#127862=DIRECTION('center_axis',(-1.,0.,0.)) ;
#127863=DIRECTION('ref_axis',(0.,0.,-1.)) ;
#127864=DIRECTION('center_axis',(0.,1.,0.)) ;
#127865=DIRECTION('ref_axis',(1.,0.,0.)) ;
#127866=DIRECTION('center_axis',(-1.,0.,0.)) ;
#127867=DIRECTION('ref_axis',(0.,0.,-1.)) ;
#127868=DIRECTION('center_axis',(0.,1.,0.)) ;
#127869=DIRECTION('ref_axis',(0.,0.,1.)) ;
#127870=DIRECTION('center_axis',(0.,1.,0.)) ;
#127871=DIRECTION('ref_axis',(0.,0.,1.)) ;
#127872=DIRECTION('center_axis',(-1.,0.,0.)) ;
#127873=DIRECTION('ref_axis',(0.,0.,1.)) ;
#127874=DIRECTION('center_axis',(-1.,0.,0.)) ;
#127875=DIRECTION('ref_axis',(0.,0.,1.)) ;
#127876=DIRECTION('center_axis',(1.,0.,0.)) ;
#127877=DIRECTION('ref_axis',(0.,0.,-1.)) ;
#127878=DIRECTION('center_axis',(-1.,0.,0.)) ;
#127879=DIRECTION('ref_axis',(0.,0.,1.)) ;
#127880=DIRECTION('center_axis',(0.,1.,0.)) ;
#127881=DIRECTION('ref_axis',(0.,0.,1.)) ;
#127882=DIRECTION('center_axis',(0.,1.,0.)) ;
#127883=DIRECTION('ref_axis',(0.,0.,1.)) ;
#127884=DIRECTION('center_axis',(0.,1.,0.)) ;
#127885=DIRECTION('ref_axis',(1.,0.,0.)) ;
#127886=DIRECTION('center_axis',(0.,0.,1.)) ;
#127887=DIRECTION('ref_axis',(-1.,0.,0.)) ;
#127888=DIRECTION('center_axis',(0.,1.,0.)) ;
#127889=DIRECTION('ref_axis',(1.,0.,0.)) ;
#127890=DIRECTION('center_axis',(0.,0.,-1.)) ;
#127891=DIRECTION('ref_axis',(1.,0.,0.)) ;
#127892=DIRECTION('center_axis',(0.,0.,1.)) ;
#127893=DIRECTION('ref_axis',(1.,0.,0.)) ;
#127894=DIRECTION('center_axis',(0.,0.,1.)) ;
#127895=DIRECTION('ref_axis',(1.,0.,0.)) ;
#127896=DIRECTION('center_axis',(0.,0.,-1.)) ;
#127897=DIRECTION('ref_axis',(-1.,0.,0.)) ;
#127898=DIRECTION('center_axis',(-8.67361737988401E-15,0.,1.)) ;
#127899=DIRECTION('ref_axis',(1.,0.,8.67361737988401E-15)) ;
#127900=DIRECTION('center_axis',(1.,0.,0.)) ;
#127901=DIRECTION('ref_axis',(0.,0.,-1.)) ;
#127902=DIRECTION('center_axis',(1.,0.,0.)) ;
#127903=DIRECTION('ref_axis',(0.,0.,-1.)) ;
#127904=DIRECTION('center_axis',(1.,0.,0.)) ;
#127905=DIRECTION('ref_axis',(0.,0.,-1.)) ;
#127906=DIRECTION('center_axis',(1.,0.,8.67361737988409E-15)) ;
#127907=DIRECTION('ref_axis',(8.67361737988409E-15,0.,-1.)) ;
#127908=DIRECTION('center_axis',(1.,0.,0.)) ;
#127909=DIRECTION('ref_axis',(0.,0.,-1.)) ;
#127910=DIRECTION('center_axis',(1.,0.,1.7347234759768E-14)) ;
#127911=DIRECTION('ref_axis',(1.7347234759768E-14,0.,-1.)) ;
#127912=DIRECTION('center_axis',(-1.,0.,0.)) ;
#127913=DIRECTION('ref_axis',(0.,0.,1.)) ;
#127914=DIRECTION('center_axis',(1.,0.,0.)) ;
#127915=DIRECTION('ref_axis',(0.,0.,-1.)) ;
#127916=DIRECTION('center_axis',(1.,0.,0.)) ;
#127917=DIRECTION('ref_axis',(0.,0.,-1.)) ;
#127918=DIRECTION('center_axis',(-8.67361737988409E-15,0.,-1.)) ;
#127919=DIRECTION('ref_axis',(-1.,0.,8.67361737988409E-15)) ;
#127920=DIRECTION('center_axis',(1.,0.,0.)) ;
#127921=DIRECTION('ref_axis',(0.,0.,-1.)) ;
#127922=DIRECTION('center_axis',(0.,0.,1.)) ;
#127923=DIRECTION('ref_axis',(1.,0.,0.)) ;
#127924=DIRECTION('center_axis',(0.,0.,-1.)) ;
#127925=DIRECTION('ref_axis',(-1.,0.,0.)) ;
#127926=DIRECTION('center_axis',(-0.422618261740697,5.55398348498559E-17,
0.906307787036651)) ;
#127927=DIRECTION('ref_axis',(0.906307787036651,2.16182864926402E-31,0.422618261740697)) ;
#127928=DIRECTION('center_axis',(0.422618261740697,-5.55398348498559E-17,
-0.906307787036651)) ;
#127929=DIRECTION('ref_axis',(-0.906307787036651,-2.07415302975303E-31,
-0.422618261740697)) ;
#127930=DIRECTION('center_axis',(-0.422618261740697,5.55398348498559E-17,
0.906307787036651)) ;
#127931=DIRECTION('ref_axis',(0.906307787036651,2.07415302975303E-31,0.422618261740697)) ;
#127932=DIRECTION('center_axis',(0.422618261740697,-5.55398348498559E-17,
-0.906307787036651)) ;
#127933=DIRECTION('ref_axis',(-0.906307787036651,-2.07415302975303E-31,
-0.422618261740697)) ;
#127934=DIRECTION('center_axis',(0.,1.,0.)) ;
#127935=DIRECTION('ref_axis',(1.,0.,0.)) ;
#127936=DIRECTION('center_axis',(3.64461297742727E-14,0.514231796959095,
-0.857651245551606)) ;
#127937=DIRECTION('ref_axis',(3.46944695195362E-14,-0.857651245551606,-0.514231796959095)) ;
#127938=DIRECTION('center_axis',(0.,-1.73472347597681E-14,1.)) ;
#127939=DIRECTION('ref_axis',(0.,1.,1.73472347597681E-14)) ;
#127940=DIRECTION('center_axis',(-1.,0.,0.)) ;
#127941=DIRECTION('ref_axis',(0.,-8.67361737988409E-15,-1.)) ;
#127942=DIRECTION('center_axis',(0.,0.,1.)) ;
#127943=DIRECTION('ref_axis',(1.,0.,0.)) ;
#127944=DIRECTION('center_axis',(0.,0.,1.)) ;
#127945=DIRECTION('ref_axis',(1.,0.,0.)) ;
#127946=DIRECTION('center_axis',(-1.,0.,0.)) ;
#127947=DIRECTION('ref_axis',(0.,0.,1.)) ;
#127948=DIRECTION('center_axis',(-1.,0.,0.)) ;
#127949=DIRECTION('ref_axis',(0.,-8.67361737988409E-15,-1.)) ;
#127950=DIRECTION('center_axis',(1.,0.,0.)) ;
#127951=DIRECTION('ref_axis',(0.,0.,-1.)) ;
#127952=DIRECTION('center_axis',(0.,-0.514231796959126,-0.857651245551587)) ;
#127953=DIRECTION('ref_axis',(0.,0.857651245551587,-0.514231796959126)) ;
#127954=DIRECTION('center_axis',(0.,1.,8.97270763436279E-17)) ;
#127955=DIRECTION('ref_axis',(0.,-8.97270763436279E-17,1.)) ;
#127956=DIRECTION('center_axis',(0.,-1.,-8.97270763436279E-17)) ;
#127957=DIRECTION('ref_axis',(0.,-8.97270763436279E-17,1.)) ;
#127958=DIRECTION('center_axis',(0.,-1.,0.)) ;
#127959=DIRECTION('ref_axis',(0.,0.,-1.)) ;
#127960=DIRECTION('center_axis',(0.,1.,0.)) ;
#127961=DIRECTION('ref_axis',(1.,0.,0.)) ;
#127962=DIRECTION('center_axis',(-1.,0.,0.)) ;
#127963=DIRECTION('ref_axis',(0.,0.,-1.)) ;
#127964=DIRECTION('center_axis',(1.,0.,0.)) ;
#127965=DIRECTION('ref_axis',(0.,0.,-1.)) ;
#127966=DIRECTION('center_axis',(0.,-0.514231796959095,0.857651245551606)) ;
#127967=DIRECTION('ref_axis',(0.,0.857651245551606,0.514231796959095)) ;
#127968=DIRECTION('center_axis',(0.,0.,-1.)) ;
#127969=DIRECTION('ref_axis',(1.,0.,0.)) ;
#127970=DIRECTION('center_axis',(0.,1.,0.)) ;
#127971=DIRECTION('ref_axis',(1.,0.,0.)) ;
#127972=DIRECTION('center_axis',(-1.73472347597682E-14,0.,-1.)) ;
#127973=DIRECTION('ref_axis',(1.,0.,-1.73472347597682E-14)) ;
#127974=DIRECTION('center_axis',(-1.,0.,0.)) ;
#127975=DIRECTION('ref_axis',(0.,8.67361737988409E-15,-1.)) ;
#127976=DIRECTION('center_axis',(0.,0.,-1.)) ;
#127977=DIRECTION('ref_axis',(-1.,0.,0.)) ;
#127978=DIRECTION('center_axis',(0.,0.,1.)) ;
#127979=DIRECTION('ref_axis',(-1.,0.,0.)) ;
#127980=DIRECTION('center_axis',(0.,0.,-1.)) ;
#127981=DIRECTION('ref_axis',(-1.,0.,0.)) ;
#127982=DIRECTION('center_axis',(-1.,0.,7.01133629567814E-33)) ;
#127983=DIRECTION('ref_axis',(7.01133629567814E-33,0.,1.)) ;
#127984=DIRECTION('center_axis',(-1.,0.,0.)) ;
#127985=DIRECTION('ref_axis',(0.,0.,1.)) ;
#127986=DIRECTION('center_axis',(0.,0.,-1.)) ;
#127987=DIRECTION('ref_axis',(-1.,0.,0.)) ;
#127988=DIRECTION('center_axis',(-7.01133629567814E-33,8.97270763436279E-17,
-1.)) ;
#127989=DIRECTION('ref_axis',(6.29106707073161E-49,1.,8.97270763436279E-17)) ;
#127990=DIRECTION('center_axis',(1.,0.,0.)) ;
#127991=DIRECTION('ref_axis',(0.,0.,-1.)) ;
#127992=DIRECTION('center_axis',(0.,0.514231796959095,0.857651245551606)) ;
#127993=DIRECTION('ref_axis',(0.,-0.857651245551606,0.514231796959095)) ;
#127994=DIRECTION('center_axis',(-1.,0.,0.)) ;
#127995=DIRECTION('ref_axis',(0.,0.,1.)) ;
#127996=DIRECTION('center_axis',(-1.,0.,0.)) ;
#127997=DIRECTION('ref_axis',(0.,-4.33680868994204E-15,-1.)) ;
#127998=DIRECTION('center_axis',(0.,0.,1.)) ;
#127999=DIRECTION('ref_axis',(1.,0.,0.)) ;
#128000=DIRECTION('center_axis',(0.,0.,-1.)) ;
#128001=DIRECTION('ref_axis',(-1.,0.,0.)) ;
#128002=DIRECTION('center_axis',(0.,-1.,8.97270763436279E-17)) ;
#128003=DIRECTION('ref_axis',(0.,-8.97270763436279E-17,-1.)) ;
#128004=DIRECTION('center_axis',(0.,-1.,8.97270763436279E-17)) ;
#128005=DIRECTION('ref_axis',(0.,-8.97270763436279E-17,-1.)) ;
#128006=DIRECTION('center_axis',(0.,-1.,0.)) ;
#128007=DIRECTION('ref_axis',(0.,0.,-1.)) ;
#128008=DIRECTION('center_axis',(-7.01133629567814E-33,8.97270763436279E-17,
-1.)) ;
#128009=DIRECTION('ref_axis',(0.,1.,0.)) ;
#128010=DIRECTION('center_axis',(0.,-1.,0.)) ;
#128011=DIRECTION('ref_axis',(0.,0.,1.)) ;
#128012=DIRECTION('center_axis',(1.,0.,0.)) ;
#128013=DIRECTION('ref_axis',(0.,0.,-1.)) ;
#128014=DIRECTION('center_axis',(0.,0.,1.)) ;
#128015=DIRECTION('ref_axis',(-1.,0.,0.)) ;
#128016=DIRECTION('center_axis',(0.,1.,0.)) ;
#128017=DIRECTION('ref_axis',(1.,0.,0.)) ;
#128018=DIRECTION('center_axis',(-1.,0.,0.)) ;
#128019=DIRECTION('ref_axis',(0.,0.,-1.)) ;
#128020=DIRECTION('center_axis',(1.,7.81406971160724E-17,0.)) ;
#128021=DIRECTION('ref_axis',(-7.81406971160724E-17,1.,0.)) ;
#128022=DIRECTION('center_axis',(1.,0.,0.)) ;
#128023=DIRECTION('ref_axis',(0.,0.,-1.)) ;
#128024=DIRECTION('center_axis',(1.,0.,0.)) ;
#128025=DIRECTION('ref_axis',(0.,0.,-1.)) ;
#128026=DIRECTION('center_axis',(0.,1.,8.97270763436279E-17)) ;
#128027=DIRECTION('ref_axis',(0.,-8.97270763436279E-17,1.)) ;
#128028=DIRECTION('center_axis',(0.,-1.,0.)) ;
#128029=DIRECTION('ref_axis',(0.,0.,-1.)) ;
#128030=DIRECTION('center_axis',(0.,0.,-1.)) ;
#128031=DIRECTION('ref_axis',(-1.,0.,0.)) ;
#128032=DIRECTION('center_axis',(-7.01133629567814E-33,8.97270763436279E-17,
1.)) ;
#128033=DIRECTION('ref_axis',(-6.29106707073161E-49,-1.,8.97270763436279E-17)) ;
#128034=DIRECTION('center_axis',(-1.,0.,-7.01133629567814E-33)) ;
#128035=DIRECTION('ref_axis',(-7.01133629567814E-33,0.,1.)) ;
#128036=DIRECTION('center_axis',(-1.,0.,0.)) ;
#128037=DIRECTION('ref_axis',(0.,0.,1.)) ;
#128038=DIRECTION('center_axis',(1.,0.,0.)) ;
#128039=DIRECTION('ref_axis',(0.,1.,0.)) ;
#128040=DIRECTION('center_axis',(2.16840434497101E-15,1.,0.)) ;
#128041=DIRECTION('ref_axis',(-1.,2.16840434497101E-15,0.)) ;
#128042=DIRECTION('center_axis',(0.,1.,0.)) ;
#128043=DIRECTION('ref_axis',(1.,0.,0.)) ;
#128044=DIRECTION('center_axis',(0.,0.,-1.)) ;
#128045=DIRECTION('ref_axis',(1.,0.,0.)) ;
#128046=DIRECTION('center_axis',(-1.,0.,0.)) ;
#128047=DIRECTION('ref_axis',(0.,0.,-1.)) ;
#128048=DIRECTION('center_axis',(-7.01133629567814E-33,8.97270763436279E-17,
1.)) ;
#128049=DIRECTION('ref_axis',(0.,-1.,0.)) ;
#128050=DIRECTION('center_axis',(0.,-1.,0.)) ;
#128051=DIRECTION('ref_axis',(0.,0.,1.)) ;
#128052=DIRECTION('center_axis',(7.81406971160724E-17,-1.,-8.97270763436279E-17)) ;
#128053=DIRECTION('ref_axis',(-7.01133629567814E-33,8.97270763436279E-17,
-1.)) ;
#128054=DIRECTION('center_axis',(0.,1.,0.)) ;
#128055=DIRECTION('ref_axis',(0.,0.,1.)) ;
#128056=DIRECTION('center_axis',(-1.,-7.81406971160724E-17,0.)) ;
#128057=DIRECTION('ref_axis',(7.81406971160724E-17,-1.,0.)) ;
#128058=DIRECTION('center_axis',(-1.,-7.81406971160724E-17,0.)) ;
#128059=DIRECTION('ref_axis',(-7.81406971160724E-17,1.,0.)) ;
#128060=DIRECTION('center_axis',(0.,0.,1.)) ;
#128061=DIRECTION('ref_axis',(1.,0.,0.)) ;
#128062=DIRECTION('center_axis',(0.,0.,-1.)) ;
#128063=DIRECTION('ref_axis',(-1.,0.,0.)) ;
#128064=DIRECTION('center_axis',(0.,-1.,8.97270763436279E-17)) ;
#128065=DIRECTION('ref_axis',(0.,-8.97270763436279E-17,-1.)) ;
#128066=DIRECTION('center_axis',(0.,-1.,0.)) ;
#128067=DIRECTION('ref_axis',(0.,0.,-1.)) ;
#128068=DIRECTION('center_axis',(1.,7.81406971160724E-17,0.)) ;
#128069=DIRECTION('ref_axis',(0.,1.,0.)) ;
#128070=DIRECTION('center_axis',(0.,0.,1.)) ;
#128071=DIRECTION('ref_axis',(-1.,0.,0.)) ;
#128072=DIRECTION('center_axis',(0.,1.,0.)) ;
#128073=DIRECTION('ref_axis',(1.,0.,0.)) ;
#128074=DIRECTION('center_axis',(-1.,0.,0.)) ;
#128075=DIRECTION('ref_axis',(0.,0.,-1.)) ;
#128076=DIRECTION('center_axis',(0.,0.,-1.)) ;
#128077=DIRECTION('ref_axis',(-1.,0.,0.)) ;
#128078=DIRECTION('center_axis',(0.,0.,1.)) ;
#128079=DIRECTION('ref_axis',(1.,0.,0.)) ;
#128080=DIRECTION('center_axis',(-1.,-7.81406971160724E-17,0.)) ;
#128081=DIRECTION('ref_axis',(7.81406971160724E-17,-1.,0.)) ;
#128082=DIRECTION('center_axis',(-1.,-7.81406971160724E-17,0.)) ;
#128083=DIRECTION('ref_axis',(-7.81406971160724E-17,1.,0.)) ;
#128084=DIRECTION('center_axis',(1.,7.81406971160724E-17,0.)) ;
#128085=DIRECTION('ref_axis',(-7.81406971160724E-17,1.,0.)) ;
#128086=DIRECTION('center_axis',(1.,0.,0.)) ;
#128087=DIRECTION('ref_axis',(0.,0.,-1.)) ;
#128088=DIRECTION('center_axis',(1.,0.,0.)) ;
#128089=DIRECTION('ref_axis',(0.,0.,-1.)) ;
#128090=DIRECTION('center_axis',(3.78638272950961E-32,-4.8455963016112E-16,
-1.)) ;
#128091=DIRECTION('ref_axis',(1.83472821505963E-47,1.,-4.8455963016112E-16)) ;
#128092=DIRECTION('center_axis',(3.78638272950961E-32,-4.8455963016112E-16,
-1.)) ;
#128093=DIRECTION('ref_axis',(1.83472821505963E-47,1.,-4.8455963016112E-16)) ;
#128094=DIRECTION('center_axis',(0.,0.,-1.)) ;
#128095=DIRECTION('ref_axis',(-1.,0.,0.)) ;
#128096=DIRECTION('center_axis',(1.,7.81406971160724E-17,0.)) ;
#128097=DIRECTION('ref_axis',(0.,1.,0.)) ;
#128098=DIRECTION('center_axis',(0.,-1.,0.)) ;
#128099=DIRECTION('ref_axis',(0.,0.,1.)) ;
#128100=DIRECTION('center_axis',(0.,1.,0.)) ;
#128101=DIRECTION('ref_axis',(1.,0.,0.)) ;
#128102=DIRECTION('center_axis',(0.,1.,0.)) ;
#128103=DIRECTION('ref_axis',(0.,0.,-1.)) ;
#128104=DIRECTION('center_axis',(-7.81406971160724E-17,1.,-8.97270763436279E-17)) ;
#128105=DIRECTION('ref_axis',(-7.01133629567814E-33,8.97270763436279E-17,
1.)) ;
#128106=DIRECTION('center_axis',(0.,-1.,0.)) ;
#128107=DIRECTION('ref_axis',(0.,0.,-1.)) ;
#128108=DIRECTION('center_axis',(0.,1.,0.)) ;
#128109=DIRECTION('ref_axis',(0.,0.,1.)) ;
#128110=DIRECTION('center_axis',(0.,-1.,0.)) ;
#128111=DIRECTION('ref_axis',(0.,0.,-1.)) ;
#128112=DIRECTION('center_axis',(0.,-1.,0.)) ;
#128113=DIRECTION('ref_axis',(0.,0.,-1.)) ;
#128114=DIRECTION('center_axis',(0.,1.,0.)) ;
#128115=DIRECTION('ref_axis',(1.,0.,0.)) ;
#128116=DIRECTION('center_axis',(0.,0.,1.)) ;
#128117=DIRECTION('ref_axis',(-1.,0.,0.)) ;
#128118=DIRECTION('center_axis',(1.,0.,0.)) ;
#128119=DIRECTION('ref_axis',(0.,0.,1.)) ;
#128120=DIRECTION('center_axis',(0.,-1.,0.)) ;
#128121=DIRECTION('ref_axis',(0.,0.,-1.)) ;
#128122=DIRECTION('center_axis',(0.,1.,0.)) ;
#128123=DIRECTION('ref_axis',(0.,0.,1.)) ;
#128124=DIRECTION('center_axis',(0.,-1.,0.)) ;
#128125=DIRECTION('ref_axis',(0.,0.,-1.)) ;
#128126=DIRECTION('center_axis',(-1.,0.,2.16840434497101E-16)) ;
#128127=DIRECTION('ref_axis',(2.16840434497101E-16,0.,1.)) ;
#128128=DIRECTION('center_axis',(1.,0.,0.)) ;
#128129=DIRECTION('ref_axis',(0.,0.,-1.)) ;
#128130=DIRECTION('center_axis',(-2.16840434497101E-16,0.,1.)) ;
#128131=DIRECTION('ref_axis',(1.,0.,2.16840434497101E-16)) ;
#128132=DIRECTION('center_axis',(0.,-1.7347234759768E-14,1.)) ;
#128133=DIRECTION('ref_axis',(0.,-1.,-1.7347234759768E-14)) ;
#128134=DIRECTION('center_axis',(0.,1.,0.)) ;
#128135=DIRECTION('ref_axis',(0.,0.,1.)) ;
#128136=DIRECTION('center_axis',(0.,-1.,0.)) ;
#128137=DIRECTION('ref_axis',(0.,0.,-1.)) ;
#128138=DIRECTION('center_axis',(0.,1.,0.)) ;
#128139=DIRECTION('ref_axis',(1.,0.,0.)) ;
#128140=DIRECTION('center_axis',(0.,0.,1.)) ;
#128141=DIRECTION('ref_axis',(-1.,0.,0.)) ;
#128142=DIRECTION('center_axis',(0.,1.,0.)) ;
#128143=DIRECTION('ref_axis',(1.,0.,0.)) ;
#128144=DIRECTION('center_axis',(1.,0.,0.)) ;
#128145=DIRECTION('ref_axis',(0.,0.,1.)) ;
#128146=DIRECTION('center_axis',(0.,0.,-1.)) ;
#128147=DIRECTION('ref_axis',(-1.,0.,0.)) ;
#128148=DIRECTION('center_axis',(-1.7347234759768E-14,0.,1.)) ;
#128149=DIRECTION('ref_axis',(1.,0.,1.7347234759768E-14)) ;
#128150=DIRECTION('center_axis',(1.,0.,2.16840434497101E-16)) ;
#128151=DIRECTION('ref_axis',(2.16840434497101E-16,0.,-1.)) ;
#128152=DIRECTION('center_axis',(1.,0.,0.)) ;
#128153=DIRECTION('ref_axis',(0.,0.,-1.)) ;
#128154=DIRECTION('center_axis',(0.,1.,0.)) ;
#128155=DIRECTION('ref_axis',(1.,0.,0.)) ;
#128156=DIRECTION('center_axis',(0.,1.,0.)) ;
#128157=DIRECTION('ref_axis',(0.,0.,-1.)) ;
#128158=DIRECTION('center_axis',(0.,1.,0.)) ;
#128159=DIRECTION('ref_axis',(0.,0.,1.)) ;
#128160=DIRECTION('center_axis',(0.,1.,0.)) ;
#128161=DIRECTION('ref_axis',(0.,0.,1.)) ;
#128162=DIRECTION('center_axis',(-0.942809041582063,-0.235702260395516,
0.235702260395518)) ;
#128163=DIRECTION('ref_axis',(0.242535625036335,4.64743530723282E-16,0.970142500145331)) ;
#128164=DIRECTION('center_axis',(-0.970142500145332,-0.242535625036331,
-2.10366121255613E-15)) ;
#128165=DIRECTION('ref_axis',(0.242535625036331,-0.970142500145332,-4.48415458566342E-30)) ;
#128166=DIRECTION('center_axis',(0.970142500145333,0.24253562503633,0.)) ;
#128167=DIRECTION('ref_axis',(-0.24253562503633,0.970142500145333,0.)) ;
#128168=DIRECTION('center_axis',(-0.970142500145332,-0.242535625036331,
-8.41464485022476E-15)) ;
#128169=DIRECTION('ref_axis',(0.242535625036331,-0.970142500145332,-1.80900724878918E-29)) ;
#128170=DIRECTION('center_axis',(0.879462917689188,0.219865729422294,-0.42214220049081)) ;
#128171=DIRECTION('ref_axis',(-0.432731067584771,1.71515946658E-16,-0.901523057468274)) ;
#128172=DIRECTION('center_axis',(0.879462917689185,0.219865729422304,-0.42214220049081)) ;
#128173=DIRECTION('ref_axis',(-0.432731067584772,-1.04304727837597E-16,
-0.901523057468273)) ;
#128174=DIRECTION('center_axis',(0.,1.,0.)) ;
#128175=DIRECTION('ref_axis',(1.,0.,0.)) ;
#128176=DIRECTION('center_axis',(-2.00438979995004E-14,-1.,0.)) ;
#128177=DIRECTION('ref_axis',(-1.,2.00438979995004E-14,0.)) ;
#128178=DIRECTION('center_axis',(0.,-1.,0.)) ;
#128179=DIRECTION('ref_axis',(0.,0.,-1.)) ;
#128180=DIRECTION('center_axis',(-4.51750905202295E-15,-1.,2.16840434497102E-15)) ;
#128181=DIRECTION('ref_axis',(1.,-4.51750905202295E-15,3.91831450274151E-31)) ;
#128182=DIRECTION('center_axis',(0.669589480006976,-0.669589480006974,-0.321402950403349)) ;
#128183=DIRECTION('ref_axis',(0.707106781186547,0.707106781186548,5.45170614306381E-16)) ;
#128184=DIRECTION('center_axis',(0.669589480006966,-0.669589480006966,-0.321402950403388)) ;
#128185=DIRECTION('ref_axis',(0.707106781186547,0.707106781186547,-1.18959821530046E-17)) ;
#128186=DIRECTION('center_axis',(0.,1.,0.)) ;
#128187=DIRECTION('ref_axis',(1.,0.,0.)) ;
#128188=DIRECTION('center_axis',(0.707106781186576,-0.707106781186519,0.)) ;
#128189=DIRECTION('ref_axis',(-0.707106781186519,-0.707106781186576,0.)) ;
#128190=DIRECTION('center_axis',(0.707106781186549,-0.707106781186546,0.)) ;
#128191=DIRECTION('ref_axis',(0.707106781186546,0.707106781186549,0.)) ;
#128192=DIRECTION('center_axis',(0.707106781186548,-0.707106781186548,-1.53329341668338E-15)) ;
#128193=DIRECTION('ref_axis',(0.707106781186548,0.707106781186548,1.5356898865553E-31)) ;
#128194=DIRECTION('center_axis',(0.577350269189622,-0.577350269189622,-0.577350269189634)) ;
#128195=DIRECTION('ref_axis',(-0.707106781186554,1.85551679542784E-15,-0.707106781186541)) ;
#128196=DIRECTION('center_axis',(-0.57735026918932,0.577350269189576,-0.577350269189982)) ;
#128197=DIRECTION('ref_axis',(-2.21337158357689E-15,0.707106781186795,0.7071067811863)) ;
#128198=DIRECTION('center_axis',(-0.707106781186548,0.707106781186548,7.66646708341679E-15)) ;
#128199=DIRECTION('ref_axis',(-0.707106781186548,-0.707106781186548,-2.87534730433018E-31)) ;
#128200=DIRECTION('center_axis',(-0.707106781186549,0.707106781186546,0.)) ;
#128201=DIRECTION('ref_axis',(-0.707106781186546,-0.707106781186549,0.)) ;
#128202=DIRECTION('center_axis',(-0.707106781186548,0.707106781186548,0.)) ;
#128203=DIRECTION('ref_axis',(-0.707106781186548,-0.707106781186548,0.)) ;
#128204=DIRECTION('center_axis',(-0.669589480006976,0.669589480006974,-0.321402950403349)) ;
#128205=DIRECTION('ref_axis',(-0.707106781186547,-0.707106781186548,5.45170614306381E-16)) ;
#128206=DIRECTION('center_axis',(0.669589480006977,-0.669589480006973,0.32140295040335)) ;
#128207=DIRECTION('ref_axis',(0.707106781186545,0.70710678118655,-2.76381108894423E-16)) ;
#128208=DIRECTION('center_axis',(0.,1.,0.)) ;
#128209=DIRECTION('ref_axis',(1.,0.,0.)) ;
#128210=DIRECTION('center_axis',(1.00219489997502E-14,1.,0.)) ;
#128211=DIRECTION('ref_axis',(1.,-1.00219489997502E-14,0.)) ;
#128212=DIRECTION('center_axis',(0.,-1.,0.)) ;
#128213=DIRECTION('ref_axis',(0.,0.,-1.)) ;
#128214=DIRECTION('center_axis',(0.,1.,0.)) ;
#128215=DIRECTION('ref_axis',(0.,0.,1.)) ;
#128216=DIRECTION('center_axis',(-0.879462917689188,-0.219865729422294,
-0.42214220049081)) ;
#128217=DIRECTION('ref_axis',(-0.432731067584771,1.71515946658E-16,0.901523057468274)) ;
#128218=DIRECTION('center_axis',(0.879462917689181,0.219865729422293,0.422142200490825)) ;
#128219=DIRECTION('ref_axis',(0.432731067584786,8.68207988095619E-17,-0.901523057468266)) ;
#128220=DIRECTION('center_axis',(0.,1.,0.)) ;
#128221=DIRECTION('ref_axis',(1.,0.,0.)) ;
#128222=DIRECTION('center_axis',(0.970142500145337,0.242535625036315,0.)) ;
#128223=DIRECTION('ref_axis',(0.242535625036315,-0.970142500145336,0.)) ;
#128224=DIRECTION('center_axis',(-0.970142500145333,-0.24253562503633,0.)) ;
#128225=DIRECTION('ref_axis',(0.24253562503633,-0.970142500145333,0.)) ;
#128226=DIRECTION('center_axis',(0.970142500145332,0.242535625036331,-2.10366121255617E-15)) ;
#128227=DIRECTION('ref_axis',(-0.242535625036331,0.970142500145332,-4.47980524894761E-30)) ;
#128228=DIRECTION('center_axis',(0.942809041582064,0.235702260395514,0.235702260395514)) ;
#128229=DIRECTION('ref_axis',(-0.242535625036331,0.970142500145332,4.49011373492972E-16)) ;
#128230=DIRECTION('center_axis',(0.,-1.,0.)) ;
#128231=DIRECTION('ref_axis',(0.,0.,-1.)) ;
#128232=DIRECTION('center_axis',(-1.,0.,-8.67361737988394E-15)) ;
#128233=DIRECTION('ref_axis',(-8.67361737988394E-15,0.,1.)) ;
#128234=DIRECTION('center_axis',(0.,0.,-1.)) ;
#128235=DIRECTION('ref_axis',(-1.,0.,0.)) ;
#128236=DIRECTION('center_axis',(0.,0.,-1.)) ;
#128237=DIRECTION('ref_axis',(-1.,0.,0.)) ;
#128238=DIRECTION('center_axis',(0.,0.,-1.)) ;
#128239=DIRECTION('ref_axis',(-1.,0.,0.)) ;
#128240=DIRECTION('center_axis',(1.,0.,0.)) ;
#128241=DIRECTION('ref_axis',(0.,0.,-1.)) ;
#128242=DIRECTION('center_axis',(-1.,0.,0.)) ;
#128243=DIRECTION('ref_axis',(0.,0.,1.)) ;
#128244=DIRECTION('center_axis',(0.,-1.,0.)) ;
#128245=DIRECTION('ref_axis',(0.,0.,-1.)) ;
#128246=DIRECTION('center_axis',(-1.,0.,0.)) ;
#128247=DIRECTION('ref_axis',(0.,0.,1.)) ;
#128248=DIRECTION('center_axis',(0.,-1.,0.)) ;
#128249=DIRECTION('ref_axis',(0.,0.,-1.)) ;
#128250=DIRECTION('center_axis',(0.,0.,-1.)) ;
#128251=DIRECTION('ref_axis',(-1.,0.,0.)) ;
#128252=DIRECTION('center_axis',(-1.,0.,0.)) ;
#128253=DIRECTION('ref_axis',(0.,0.,1.)) ;
#128254=DIRECTION('center_axis',(-1.,1.73472347597681E-14,0.)) ;
#128255=DIRECTION('ref_axis',(-1.73472347597681E-14,-1.,0.)) ;
#128256=DIRECTION('center_axis',(0.,0.,1.)) ;
#128257=DIRECTION('ref_axis',(1.,0.,0.)) ;
#128258=DIRECTION('center_axis',(0.,0.,-1.)) ;
#128259=DIRECTION('ref_axis',(-1.,0.,0.)) ;
#128260=DIRECTION('center_axis',(0.,-1.,0.)) ;
#128261=DIRECTION('ref_axis',(0.,0.,-1.)) ;
#128262=DIRECTION('center_axis',(0.,-1.,0.)) ;
#128263=DIRECTION('ref_axis',(0.,0.,-1.)) ;
#128264=DIRECTION('center_axis',(0.,-1.,0.)) ;
#128265=DIRECTION('ref_axis',(0.,0.,-1.)) ;
#128266=DIRECTION('center_axis',(0.,0.,1.)) ;
#128267=DIRECTION('ref_axis',(1.,0.,0.)) ;
#128268=DIRECTION('center_axis',(0.,0.,-1.)) ;
#128269=DIRECTION('ref_axis',(-1.,0.,0.)) ;
#128270=DIRECTION('center_axis',(0.,0.,1.)) ;
#128271=DIRECTION('ref_axis',(1.,0.,0.)) ;
#128272=DIRECTION('center_axis',(0.,-1.,0.)) ;
#128273=DIRECTION('ref_axis',(0.,0.,-1.)) ;
#128274=DIRECTION('center_axis',(0.,-1.,0.)) ;
#128275=DIRECTION('ref_axis',(0.,0.,-1.)) ;
#128276=DIRECTION('center_axis',(0.,1.,0.)) ;
#128277=DIRECTION('ref_axis',(1.,0.,0.)) ;
#128278=DIRECTION('center_axis',(-1.,0.,0.)) ;
#128279=DIRECTION('ref_axis',(0.,0.,-1.)) ;
#128280=DIRECTION('center_axis',(0.,1.,0.)) ;
#128281=DIRECTION('ref_axis',(1.,0.,0.)) ;
#128282=DIRECTION('center_axis',(-1.,0.,0.)) ;
#128283=DIRECTION('ref_axis',(0.,0.,-1.)) ;
#128284=DIRECTION('center_axis',(0.,-1.,0.)) ;
#128285=DIRECTION('ref_axis',(0.,0.,-1.)) ;
#128286=DIRECTION('center_axis',(0.,-1.,0.)) ;
#128287=DIRECTION('ref_axis',(0.,0.,-1.)) ;
#128288=DIRECTION('center_axis',(-1.,0.,0.)) ;
#128289=DIRECTION('ref_axis',(0.,0.,1.)) ;
#128290=DIRECTION('center_axis',(-1.,0.,0.)) ;
#128291=DIRECTION('ref_axis',(0.,0.,1.)) ;
#128292=DIRECTION('center_axis',(1.,0.,0.)) ;
#128293=DIRECTION('ref_axis',(0.,0.,-1.)) ;
#128294=DIRECTION('center_axis',(-1.,0.,0.)) ;
#128295=DIRECTION('ref_axis',(0.,0.,1.)) ;
#128296=DIRECTION('center_axis',(0.,-1.,0.)) ;
#128297=DIRECTION('ref_axis',(0.,0.,-1.)) ;
#128298=DIRECTION('center_axis',(0.,-1.,0.)) ;
#128299=DIRECTION('ref_axis',(0.,0.,-1.)) ;
#128300=DIRECTION('center_axis',(0.,1.,0.)) ;
#128301=DIRECTION('ref_axis',(1.,0.,0.)) ;
#128302=DIRECTION('center_axis',(0.,0.,-1.)) ;
#128303=DIRECTION('ref_axis',(1.,0.,0.)) ;
#128304=DIRECTION('center_axis',(0.,1.,0.)) ;
#128305=DIRECTION('ref_axis',(1.,0.,0.)) ;
#128306=DIRECTION('center_axis',(0.,0.,1.)) ;
#128307=DIRECTION('ref_axis',(-1.,0.,0.)) ;
#128308=DIRECTION('center_axis',(0.,0.,-1.)) ;
#128309=DIRECTION('ref_axis',(-1.,0.,0.)) ;
#128310=DIRECTION('center_axis',(1.,1.31418445149758E-16,-2.16840434497101E-16)) ;
#128311=DIRECTION('ref_axis',(-2.16840434497101E-16,-2.8496832747207E-32,
-1.)) ;
#128312=DIRECTION('center_axis',(1.,0.,0.)) ;
#128313=DIRECTION('ref_axis',(0.,0.,-1.)) ;
#128314=DIRECTION('center_axis',(-1.,0.,0.)) ;
#128315=DIRECTION('ref_axis',(0.,0.,1.)) ;
#128316=DIRECTION('center_axis',(-1.31418445149758E-16,1.,0.)) ;
#128317=DIRECTION('ref_axis',(-1.,0.,0.)) ;
#128318=DIRECTION('center_axis',(0.,0.,1.)) ;
#128319=DIRECTION('ref_axis',(-1.,0.,0.)) ;
#128320=DIRECTION('center_axis',(-1.31418445149758E-16,1.,0.)) ;
#128321=DIRECTION('ref_axis',(-1.,-1.31418445149758E-16,0.)) ;
#128322=DIRECTION('center_axis',(-1.31418445149758E-16,1.,0.)) ;
#128323=DIRECTION('ref_axis',(-1.,0.,0.)) ;
#128324=DIRECTION('center_axis',(-1.31418445149758E-16,1.,0.)) ;
#128325=DIRECTION('ref_axis',(-1.,-1.31418445149758E-16,0.)) ;
#128326=DIRECTION('center_axis',(0.,0.,1.)) ;
#128327=DIRECTION('ref_axis',(-1.,0.,0.)) ;
#128328=DIRECTION('center_axis',(-4.33680868994202E-16,-5.69936654944139E-32,
-1.)) ;
#128329=DIRECTION('ref_axis',(-1.,2.47170623787823E-47,4.33680868994202E-16)) ;
#128330=DIRECTION('center_axis',(0.,0.,1.)) ;
#128331=DIRECTION('ref_axis',(1.,0.,0.)) ;
#128332=DIRECTION('center_axis',(-1.31418445149758E-16,-1.,0.)) ;
#128333=DIRECTION('ref_axis',(1.,-1.31418445149758E-16,0.)) ;
#128334=DIRECTION('center_axis',(0.,1.,0.)) ;
#128335=DIRECTION('ref_axis',(0.,0.,1.)) ;
#128336=DIRECTION('center_axis',(-1.,0.,2.16840434497101E-16)) ;
#128337=DIRECTION('ref_axis',(2.16840434497101E-16,0.,1.)) ;
#128338=DIRECTION('center_axis',(-1.,0.,0.)) ;
#128339=DIRECTION('ref_axis',(0.,0.,1.)) ;
#128340=DIRECTION('center_axis',(1.,0.,0.)) ;
#128341=DIRECTION('ref_axis',(0.,0.,-1.)) ;
#128342=DIRECTION('center_axis',(-1.31418445149758E-16,-1.,0.)) ;
#128343=DIRECTION('ref_axis',(1.,-1.31418445149758E-16,0.)) ;
#128344=DIRECTION('center_axis',(0.,1.,0.)) ;
#128345=DIRECTION('ref_axis',(0.,0.,1.)) ;
#128346=DIRECTION('center_axis',(2.16840434497101E-16,2.8496832747207E-32,
1.)) ;
#128347=DIRECTION('ref_axis',(1.,-6.17926559469557E-48,-2.16840434497101E-16)) ;
#128348=DIRECTION('center_axis',(0.,0.,1.)) ;
#128349=DIRECTION('ref_axis',(1.,0.,0.)) ;
#128350=DIRECTION('center_axis',(-1.,-1.31418445149758E-16,-2.16840434497101E-16)) ;
#128351=DIRECTION('ref_axis',(-2.16840434497101E-16,-2.8496832747207E-32,
1.)) ;
#128352=DIRECTION('center_axis',(-1.,0.,0.)) ;
#128353=DIRECTION('ref_axis',(0.,0.,1.)) ;
#128354=DIRECTION('center_axis',(1.,0.,0.)) ;
#128355=DIRECTION('ref_axis',(0.,0.,-1.)) ;
#128356=DIRECTION('center_axis',(-1.31418445149758E-16,1.,0.)) ;
#128357=DIRECTION('ref_axis',(-1.,0.,0.)) ;
#128358=DIRECTION('center_axis',(-1.31418445149758E-16,1.,0.)) ;
#128359=DIRECTION('ref_axis',(-1.,-1.31418445149758E-16,0.)) ;
#128360=DIRECTION('center_axis',(0.,1.,0.)) ;
#128361=DIRECTION('ref_axis',(1.,0.,0.)) ;
#128362=DIRECTION('center_axis',(0.,0.,-1.)) ;
#128363=DIRECTION('ref_axis',(1.,0.,0.)) ;
#128364=DIRECTION('center_axis',(0.,1.,0.)) ;
#128365=DIRECTION('ref_axis',(1.,0.,0.)) ;
#128366=DIRECTION('center_axis',(0.,0.,-1.)) ;
#128367=DIRECTION('ref_axis',(1.,0.,0.)) ;
#128368=DIRECTION('center_axis',(-1.31418445149758E-16,1.,0.)) ;
#128369=DIRECTION('ref_axis',(-1.,0.,0.)) ;
#128370=DIRECTION('center_axis',(-1.31418445149758E-16,1.,0.)) ;
#128371=DIRECTION('ref_axis',(-1.,-1.31418445149758E-16,0.)) ;
#128372=DIRECTION('center_axis',(-1.31418445149758E-16,-1.,0.)) ;
#128373=DIRECTION('ref_axis',(1.,-1.31418445149758E-16,0.)) ;
#128374=DIRECTION('center_axis',(0.,1.,0.)) ;
#128375=DIRECTION('ref_axis',(0.,0.,1.)) ;
#128376=DIRECTION('center_axis',(4.33680868994202E-16,0.,1.)) ;
#128377=DIRECTION('ref_axis',(1.,0.,-4.33680868994202E-16)) ;
#128378=DIRECTION('center_axis',(0.,0.,-1.)) ;
#128379=DIRECTION('ref_axis',(-1.,0.,0.)) ;
#128380=DIRECTION('center_axis',(-2.16840434497101E-16,0.,-1.)) ;
#128381=DIRECTION('ref_axis',(-1.,0.,2.16840434497101E-16)) ;
#128382=DIRECTION('center_axis',(0.,0.,-1.)) ;
#128383=DIRECTION('ref_axis',(-1.,0.,0.)) ;
#128384=DIRECTION('center_axis',(-1.31418445149758E-16,-1.,0.)) ;
#128385=DIRECTION('ref_axis',(1.,-1.31418445149758E-16,0.)) ;
#128386=DIRECTION('center_axis',(0.,1.,0.)) ;
#128387=DIRECTION('ref_axis',(0.,0.,1.)) ;
#128388=DIRECTION('center_axis',(0.,1.,0.)) ;
#128389=DIRECTION('ref_axis',(1.,0.,0.)) ;
#128390=DIRECTION('center_axis',(-1.,0.,0.)) ;
#128391=DIRECTION('ref_axis',(0.,0.,-1.)) ;
#128392=DIRECTION('center_axis',(0.,1.,0.)) ;
#128393=DIRECTION('ref_axis',(1.,0.,0.)) ;
#128394=DIRECTION('center_axis',(1.,0.,0.)) ;
#128395=DIRECTION('ref_axis',(0.,0.,1.)) ;
#128396=DIRECTION('center_axis',(1.,0.,2.16840434497101E-16)) ;
#128397=DIRECTION('ref_axis',(2.16840434497101E-16,0.,-1.)) ;
#128398=DIRECTION('center_axis',(0.,1.,0.)) ;
#128399=DIRECTION('ref_axis',(0.,0.,1.)) ;
#128400=DIRECTION('center_axis',(0.,1.,0.)) ;
#128401=DIRECTION('ref_axis',(0.,0.,1.)) ;
#128402=DIRECTION('center_axis',(0.,0.,-1.)) ;
#128403=DIRECTION('ref_axis',(-1.,0.,0.)) ;
#128404=DIRECTION('center_axis',(0.,0.,1.)) ;
#128405=DIRECTION('ref_axis',(1.,0.,0.)) ;
#128406=DIRECTION('center_axis',(0.,0.,-1.)) ;
#128407=DIRECTION('ref_axis',(-1.,0.,0.)) ;
#128408=DIRECTION('center_axis',(0.,1.,0.)) ;
#128409=DIRECTION('ref_axis',(0.,0.,1.)) ;
#128410=DIRECTION('center_axis',(0.,1.,0.)) ;
#128411=DIRECTION('ref_axis',(0.,0.,1.)) ;
#128412=DIRECTION('center_axis',(0.,1.,0.)) ;
#128413=DIRECTION('ref_axis',(1.,0.,0.)) ;
#128414=DIRECTION('center_axis',(-1.,0.,0.)) ;
#128415=DIRECTION('ref_axis',(0.,0.,-1.)) ;
#128416=DIRECTION('center_axis',(0.,1.,0.)) ;
#128417=DIRECTION('ref_axis',(1.,0.,0.)) ;
#128418=DIRECTION('center_axis',(-1.,0.,0.)) ;
#128419=DIRECTION('ref_axis',(0.,0.,-1.)) ;
#128420=DIRECTION('center_axis',(0.,1.,0.)) ;
#128421=DIRECTION('ref_axis',(0.,0.,1.)) ;
#128422=DIRECTION('center_axis',(0.,1.,0.)) ;
#128423=DIRECTION('ref_axis',(0.,0.,1.)) ;
#128424=DIRECTION('center_axis',(-1.,0.,0.)) ;
#128425=DIRECTION('ref_axis',(0.,0.,1.)) ;
#128426=DIRECTION('center_axis',(-1.,0.,0.)) ;
#128427=DIRECTION('ref_axis',(0.,0.,1.)) ;
#128428=DIRECTION('center_axis',(1.,0.,0.)) ;
#128429=DIRECTION('ref_axis',(0.,0.,-1.)) ;
#128430=DIRECTION('center_axis',(-1.,0.,0.)) ;
#128431=DIRECTION('ref_axis',(0.,0.,1.)) ;
#128432=DIRECTION('center_axis',(0.,1.,0.)) ;
#128433=DIRECTION('ref_axis',(0.,0.,1.)) ;
#128434=DIRECTION('center_axis',(0.,1.,0.)) ;
#128435=DIRECTION('ref_axis',(0.,0.,1.)) ;
#128436=DIRECTION('center_axis',(0.,1.,0.)) ;
#128437=DIRECTION('ref_axis',(1.,0.,0.)) ;
#128438=DIRECTION('center_axis',(0.,0.,1.)) ;
#128439=DIRECTION('ref_axis',(-1.,0.,0.)) ;
#128440=DIRECTION('center_axis',(0.,1.,0.)) ;
#128441=DIRECTION('ref_axis',(1.,0.,0.)) ;
#128442=DIRECTION('center_axis',(0.,0.,-1.)) ;
#128443=DIRECTION('ref_axis',(1.,0.,0.)) ;
#128444=DIRECTION('center_axis',(0.,0.,1.)) ;
#128445=DIRECTION('ref_axis',(1.,0.,0.)) ;
#128446=DIRECTION('center_axis',(0.,0.,1.)) ;
#128447=DIRECTION('ref_axis',(1.,0.,0.)) ;
#128448=DIRECTION('center_axis',(0.,0.,-1.)) ;
#128449=DIRECTION('ref_axis',(-1.,0.,0.)) ;
#128450=DIRECTION('center_axis',(0.,0.,1.)) ;
#128451=DIRECTION('ref_axis',(1.,0.,0.)) ;
#128452=DIRECTION('center_axis',(1.,0.,0.)) ;
#128453=DIRECTION('ref_axis',(0.,0.,-1.)) ;
#128454=DIRECTION('center_axis',(1.,0.,0.)) ;
#128455=DIRECTION('ref_axis',(0.,0.,-1.)) ;
#128456=DIRECTION('center_axis',(1.,0.,0.)) ;
#128457=DIRECTION('ref_axis',(0.,0.,-1.)) ;
#128458=DIRECTION('center_axis',(1.,0.,8.67361737988409E-15)) ;
#128459=DIRECTION('ref_axis',(8.67361737988409E-15,0.,-1.)) ;
#128460=DIRECTION('center_axis',(1.,0.,0.)) ;
#128461=DIRECTION('ref_axis',(0.,0.,-1.)) ;
#128462=DIRECTION('center_axis',(1.,0.,1.73472347597682E-14)) ;
#128463=DIRECTION('ref_axis',(1.73472347597682E-14,0.,-1.)) ;
#128464=DIRECTION('center_axis',(-1.,0.,0.)) ;
#128465=DIRECTION('ref_axis',(0.,0.,1.)) ;
#128466=DIRECTION('center_axis',(1.,0.,0.)) ;
#128467=DIRECTION('ref_axis',(0.,0.,-1.)) ;
#128468=DIRECTION('center_axis',(1.,0.,0.)) ;
#128469=DIRECTION('ref_axis',(0.,0.,-1.)) ;
#128470=DIRECTION('center_axis',(0.,0.,-1.)) ;
#128471=DIRECTION('ref_axis',(-1.,0.,0.)) ;
#128472=DIRECTION('center_axis',(1.,0.,0.)) ;
#128473=DIRECTION('ref_axis',(0.,0.,-1.)) ;
#128474=DIRECTION('center_axis',(0.,0.,1.)) ;
#128475=DIRECTION('ref_axis',(1.,0.,0.)) ;
#128476=DIRECTION('center_axis',(0.,0.,-1.)) ;
#128477=DIRECTION('ref_axis',(-1.,0.,0.)) ;
#128478=DIRECTION('center_axis',(-0.422618261740697,5.55398348498559E-17,
0.906307787036651)) ;
#128479=DIRECTION('ref_axis',(0.906307787036651,-2.19407316623673E-31,0.422618261740697)) ;
#128480=DIRECTION('center_axis',(0.422618261740697,-5.55398348498559E-17,
-0.906307787036651)) ;
#128481=DIRECTION('ref_axis',(-0.906307787036651,2.28174878574772E-31,-0.422618261740697)) ;
#128482=DIRECTION('center_axis',(-0.422618261740697,5.55398348498559E-17,
0.906307787036651)) ;
#128483=DIRECTION('ref_axis',(0.906307787036651,-2.28174878574772E-31,0.422618261740697)) ;
#128484=DIRECTION('center_axis',(0.422618261740697,-5.55398348498559E-17,
-0.906307787036651)) ;
#128485=DIRECTION('ref_axis',(-0.906307787036651,2.28174878574772E-31,-0.422618261740697)) ;
#128486=DIRECTION('center_axis',(0.,1.,0.)) ;
#128487=DIRECTION('ref_axis',(1.,0.,0.)) ;
#128488=DIRECTION('center_axis',(3.64461297742727E-14,0.514231796959095,
-0.857651245551606)) ;
#128489=DIRECTION('ref_axis',(3.46944695195362E-14,-0.857651245551606,-0.514231796959095)) ;
#128490=DIRECTION('center_axis',(0.,-1.73472347597681E-14,1.)) ;
#128491=DIRECTION('ref_axis',(0.,1.,1.73472347597681E-14)) ;
#128492=DIRECTION('center_axis',(-1.,0.,0.)) ;
#128493=DIRECTION('ref_axis',(0.,-8.67361737988409E-15,-1.)) ;
#128494=DIRECTION('center_axis',(0.,0.,1.)) ;
#128495=DIRECTION('ref_axis',(1.,0.,0.)) ;
#128496=DIRECTION('center_axis',(0.,0.,1.)) ;
#128497=DIRECTION('ref_axis',(1.,0.,0.)) ;
#128498=DIRECTION('center_axis',(-1.,0.,0.)) ;
#128499=DIRECTION('ref_axis',(0.,0.,1.)) ;
#128500=DIRECTION('center_axis',(-1.,0.,0.)) ;
#128501=DIRECTION('ref_axis',(0.,-8.67361737988409E-15,-1.)) ;
#128502=DIRECTION('center_axis',(1.,0.,0.)) ;
#128503=DIRECTION('ref_axis',(0.,0.,-1.)) ;
#128504=DIRECTION('center_axis',(0.,-0.514231796959124,-0.857651245551588)) ;
#128505=DIRECTION('ref_axis',(0.,0.857651245551588,-0.514231796959124)) ;
#128506=DIRECTION('center_axis',(0.,1.,8.97270763436279E-17)) ;
#128507=DIRECTION('ref_axis',(0.,-8.97270763436279E-17,1.)) ;
#128508=DIRECTION('center_axis',(0.,-1.,-8.97270763436279E-17)) ;
#128509=DIRECTION('ref_axis',(0.,-8.97270763436279E-17,1.)) ;
#128510=DIRECTION('center_axis',(0.,-1.,0.)) ;
#128511=DIRECTION('ref_axis',(0.,0.,-1.)) ;
#128512=DIRECTION('center_axis',(0.,1.,0.)) ;
#128513=DIRECTION('ref_axis',(1.,0.,0.)) ;
#128514=DIRECTION('center_axis',(-1.,0.,0.)) ;
#128515=DIRECTION('ref_axis',(0.,0.,-1.)) ;
#128516=DIRECTION('center_axis',(1.,0.,0.)) ;
#128517=DIRECTION('ref_axis',(0.,0.,-1.)) ;
#128518=DIRECTION('center_axis',(0.,-0.514231796959095,0.857651245551606)) ;
#128519=DIRECTION('ref_axis',(0.,0.857651245551606,0.514231796959095)) ;
#128520=DIRECTION('center_axis',(0.,0.,-1.)) ;
#128521=DIRECTION('ref_axis',(1.,0.,0.)) ;
#128522=DIRECTION('center_axis',(0.,1.,0.)) ;
#128523=DIRECTION('ref_axis',(1.,0.,0.)) ;
#128524=DIRECTION('center_axis',(-3.46944695195364E-14,0.,-1.)) ;
#128525=DIRECTION('ref_axis',(1.,0.,-3.46944695195364E-14)) ;
#128526=DIRECTION('center_axis',(-1.,0.,0.)) ;
#128527=DIRECTION('ref_axis',(0.,4.33680868994204E-15,-1.)) ;
#128528=DIRECTION('center_axis',(0.,0.,-1.)) ;
#128529=DIRECTION('ref_axis',(-1.,0.,0.)) ;
#128530=DIRECTION('center_axis',(0.,0.,1.)) ;
#128531=DIRECTION('ref_axis',(-1.,0.,0.)) ;
#128532=DIRECTION('center_axis',(0.,0.,-1.)) ;
#128533=DIRECTION('ref_axis',(-1.,0.,0.)) ;
#128534=DIRECTION('center_axis',(-1.,0.,7.01133629567814E-33)) ;
#128535=DIRECTION('ref_axis',(7.01133629567814E-33,0.,1.)) ;
#128536=DIRECTION('center_axis',(-1.,0.,0.)) ;
#128537=DIRECTION('ref_axis',(0.,0.,1.)) ;
#128538=DIRECTION('center_axis',(0.,0.,-1.)) ;
#128539=DIRECTION('ref_axis',(-1.,0.,0.)) ;
#128540=DIRECTION('center_axis',(-7.01133629567814E-33,8.97270763436279E-17,
-1.)) ;
#128541=DIRECTION('ref_axis',(6.29106707073161E-49,1.,8.97270763436279E-17)) ;
#128542=DIRECTION('center_axis',(1.,0.,0.)) ;
#128543=DIRECTION('ref_axis',(0.,0.,-1.)) ;
#128544=DIRECTION('center_axis',(-2.2301249256967E-15,0.514231796959095,
0.857651245551606)) ;
#128545=DIRECTION('ref_axis',(-4.79361507851841E-30,-0.857651245551606,
0.514231796959095)) ;
#128546=DIRECTION('center_axis',(-1.,0.,0.)) ;
#128547=DIRECTION('ref_axis',(0.,0.,1.)) ;
#128548=DIRECTION('center_axis',(-1.,0.,0.)) ;
#128549=DIRECTION('ref_axis',(0.,-4.33680868994204E-15,-1.)) ;
#128550=DIRECTION('center_axis',(0.,0.,1.)) ;
#128551=DIRECTION('ref_axis',(1.,0.,0.)) ;
#128552=DIRECTION('center_axis',(0.,0.,-1.)) ;
#128553=DIRECTION('ref_axis',(-1.,0.,0.)) ;
#128554=DIRECTION('center_axis',(0.,-1.,8.97270763436279E-17)) ;
#128555=DIRECTION('ref_axis',(0.,-8.97270763436279E-17,-1.)) ;
#128556=DIRECTION('center_axis',(0.,-1.,8.97270763436279E-17)) ;
#128557=DIRECTION('ref_axis',(0.,-8.97270763436279E-17,-1.)) ;
#128558=DIRECTION('center_axis',(0.,-1.,0.)) ;
#128559=DIRECTION('ref_axis',(0.,0.,-1.)) ;
#128560=DIRECTION('center_axis',(-7.01133629567814E-33,8.97270763436279E-17,
-1.)) ;
#128561=DIRECTION('ref_axis',(0.,1.,0.)) ;
#128562=DIRECTION('center_axis',(0.,-1.,0.)) ;
#128563=DIRECTION('ref_axis',(0.,0.,1.)) ;
#128564=DIRECTION('center_axis',(1.,0.,0.)) ;
#128565=DIRECTION('ref_axis',(0.,0.,-1.)) ;
#128566=DIRECTION('center_axis',(0.,0.,1.)) ;
#128567=DIRECTION('ref_axis',(-1.,0.,0.)) ;
#128568=DIRECTION('center_axis',(0.,1.,0.)) ;
#128569=DIRECTION('ref_axis',(1.,0.,0.)) ;
#128570=DIRECTION('center_axis',(-1.,0.,0.)) ;
#128571=DIRECTION('ref_axis',(0.,0.,-1.)) ;
#128572=DIRECTION('center_axis',(1.,7.81406971160724E-17,0.)) ;
#128573=DIRECTION('ref_axis',(-7.81406971160724E-17,1.,0.)) ;
#128574=DIRECTION('center_axis',(1.,0.,0.)) ;
#128575=DIRECTION('ref_axis',(0.,0.,-1.)) ;
#128576=DIRECTION('center_axis',(1.,0.,0.)) ;
#128577=DIRECTION('ref_axis',(0.,0.,-1.)) ;
#128578=DIRECTION('center_axis',(0.,1.,8.97270763436279E-17)) ;
#128579=DIRECTION('ref_axis',(0.,-8.97270763436279E-17,1.)) ;
#128580=DIRECTION('center_axis',(0.,-1.,0.)) ;
#128581=DIRECTION('ref_axis',(0.,0.,-1.)) ;
#128582=DIRECTION('center_axis',(0.,0.,-1.)) ;
#128583=DIRECTION('ref_axis',(-1.,0.,0.)) ;
#128584=DIRECTION('center_axis',(-7.01133629567814E-33,8.97270763436279E-17,
1.)) ;
#128585=DIRECTION('ref_axis',(-6.29106707073161E-49,-1.,8.97270763436279E-17)) ;
#128586=DIRECTION('center_axis',(-1.,0.,-7.01133629567814E-33)) ;
#128587=DIRECTION('ref_axis',(-7.01133629567814E-33,0.,1.)) ;
#128588=DIRECTION('center_axis',(-1.,0.,0.)) ;
#128589=DIRECTION('ref_axis',(0.,0.,1.)) ;
#128590=DIRECTION('center_axis',(1.,0.,0.)) ;
#128591=DIRECTION('ref_axis',(0.,1.,0.)) ;
#128592=DIRECTION('center_axis',(0.,1.,0.)) ;
#128593=DIRECTION('ref_axis',(0.,0.,1.)) ;
#128594=DIRECTION('center_axis',(0.,1.,0.)) ;
#128595=DIRECTION('ref_axis',(1.,0.,0.)) ;
#128596=DIRECTION('center_axis',(0.,0.,-1.)) ;
#128597=DIRECTION('ref_axis',(1.,0.,0.)) ;
#128598=DIRECTION('center_axis',(-1.,0.,0.)) ;
#128599=DIRECTION('ref_axis',(0.,0.,-1.)) ;
#128600=DIRECTION('center_axis',(-7.01133629567814E-33,8.97270763436279E-17,
1.)) ;
#128601=DIRECTION('ref_axis',(0.,-1.,0.)) ;
#128602=DIRECTION('center_axis',(0.,-1.,0.)) ;
#128603=DIRECTION('ref_axis',(0.,0.,1.)) ;
#128604=DIRECTION('center_axis',(7.81406971160724E-17,-1.,-8.97270763436279E-17)) ;
#128605=DIRECTION('ref_axis',(-7.01133629567814E-33,8.97270763436279E-17,
-1.)) ;
#128606=DIRECTION('center_axis',(0.,1.,0.)) ;
#128607=DIRECTION('ref_axis',(0.,0.,1.)) ;
#128608=DIRECTION('center_axis',(-1.,-7.81406971160724E-17,0.)) ;
#128609=DIRECTION('ref_axis',(7.81406971160724E-17,-1.,0.)) ;
#128610=DIRECTION('center_axis',(-1.,-7.81406971160724E-17,0.)) ;
#128611=DIRECTION('ref_axis',(-7.81406971160724E-17,1.,0.)) ;
#128612=DIRECTION('center_axis',(0.,0.,1.)) ;
#128613=DIRECTION('ref_axis',(1.,0.,0.)) ;
#128614=DIRECTION('center_axis',(0.,0.,-1.)) ;
#128615=DIRECTION('ref_axis',(-1.,0.,0.)) ;
#128616=DIRECTION('center_axis',(0.,-1.,8.97270763436279E-17)) ;
#128617=DIRECTION('ref_axis',(0.,-8.97270763436279E-17,-1.)) ;
#128618=DIRECTION('center_axis',(0.,-1.,0.)) ;
#128619=DIRECTION('ref_axis',(0.,0.,-1.)) ;
#128620=DIRECTION('center_axis',(1.,7.81406971160724E-17,0.)) ;
#128621=DIRECTION('ref_axis',(0.,1.,0.)) ;
#128622=DIRECTION('center_axis',(0.,0.,1.)) ;
#128623=DIRECTION('ref_axis',(-1.,0.,0.)) ;
#128624=DIRECTION('center_axis',(0.,1.,0.)) ;
#128625=DIRECTION('ref_axis',(1.,0.,0.)) ;
#128626=DIRECTION('center_axis',(-1.,0.,0.)) ;
#128627=DIRECTION('ref_axis',(0.,0.,-1.)) ;
#128628=DIRECTION('center_axis',(0.,0.,-1.)) ;
#128629=DIRECTION('ref_axis',(-1.,0.,0.)) ;
#128630=DIRECTION('center_axis',(0.,0.,1.)) ;
#128631=DIRECTION('ref_axis',(1.,0.,0.)) ;
#128632=DIRECTION('center_axis',(-1.,-7.81406971160724E-17,0.)) ;
#128633=DIRECTION('ref_axis',(7.81406971160724E-17,-1.,0.)) ;
#128634=DIRECTION('center_axis',(-1.,-7.81406971160724E-17,0.)) ;
#128635=DIRECTION('ref_axis',(-7.81406971160724E-17,1.,0.)) ;
#128636=DIRECTION('center_axis',(1.,7.81406971160724E-17,0.)) ;
#128637=DIRECTION('ref_axis',(-7.81406971160724E-17,1.,0.)) ;
#128638=DIRECTION('center_axis',(1.,0.,0.)) ;
#128639=DIRECTION('ref_axis',(0.,0.,-1.)) ;
#128640=DIRECTION('center_axis',(1.,0.,0.)) ;
#128641=DIRECTION('ref_axis',(0.,0.,-1.)) ;
#128642=DIRECTION('center_axis',(3.78638272950961E-32,-4.8455963016112E-16,
-1.)) ;
#128643=DIRECTION('ref_axis',(1.83472821505963E-47,1.,-4.8455963016112E-16)) ;
#128644=DIRECTION('center_axis',(3.78638272950961E-32,-4.8455963016112E-16,
-1.)) ;
#128645=DIRECTION('ref_axis',(1.83472821505963E-47,1.,-4.8455963016112E-16)) ;
#128646=DIRECTION('center_axis',(0.,0.,-1.)) ;
#128647=DIRECTION('ref_axis',(-1.,0.,0.)) ;
#128648=DIRECTION('center_axis',(1.,7.81406971160724E-17,0.)) ;
#128649=DIRECTION('ref_axis',(0.,1.,0.)) ;
#128650=DIRECTION('center_axis',(0.,-1.,0.)) ;
#128651=DIRECTION('ref_axis',(0.,0.,1.)) ;
#128652=DIRECTION('center_axis',(0.,1.,0.)) ;
#128653=DIRECTION('ref_axis',(1.,0.,0.)) ;
#128654=DIRECTION('center_axis',(0.,1.,0.)) ;
#128655=DIRECTION('ref_axis',(0.,0.,-1.)) ;
#128656=DIRECTION('center_axis',(-7.81406971160724E-17,1.,-8.97270763436279E-17)) ;
#128657=DIRECTION('ref_axis',(-7.01133629567814E-33,8.97270763436279E-17,
1.)) ;
#128658=DIRECTION('center_axis',(0.,-1.,0.)) ;
#128659=DIRECTION('ref_axis',(0.,0.,-1.)) ;
#128660=DIRECTION('center_axis',(0.,1.,0.)) ;
#128661=DIRECTION('ref_axis',(0.,0.,1.)) ;
#128662=DIRECTION('center_axis',(0.,-1.,0.)) ;
#128663=DIRECTION('ref_axis',(0.,0.,-1.)) ;
#128664=DIRECTION('center_axis',(0.,-1.,0.)) ;
#128665=DIRECTION('ref_axis',(0.,0.,-1.)) ;
#128666=DIRECTION('center_axis',(0.,1.,0.)) ;
#128667=DIRECTION('ref_axis',(1.,0.,0.)) ;
#128668=DIRECTION('center_axis',(0.,0.,1.)) ;
#128669=DIRECTION('ref_axis',(-1.,0.,0.)) ;
#128670=DIRECTION('center_axis',(1.,0.,0.)) ;
#128671=DIRECTION('ref_axis',(0.,0.,1.)) ;
#128672=DIRECTION('center_axis',(0.,-1.,0.)) ;
#128673=DIRECTION('ref_axis',(0.,0.,-1.)) ;
#128674=DIRECTION('center_axis',(0.,1.,0.)) ;
#128675=DIRECTION('ref_axis',(0.,0.,1.)) ;
#128676=DIRECTION('center_axis',(0.,-1.,0.)) ;
#128677=DIRECTION('ref_axis',(0.,0.,-1.)) ;
#128678=DIRECTION('center_axis',(-1.,0.,2.16840434497101E-16)) ;
#128679=DIRECTION('ref_axis',(2.16840434497101E-16,0.,1.)) ;
#128680=DIRECTION('center_axis',(1.,0.,0.)) ;
#128681=DIRECTION('ref_axis',(0.,0.,-1.)) ;
#128682=DIRECTION('center_axis',(-2.16840434497101E-16,0.,1.)) ;
#128683=DIRECTION('ref_axis',(1.,0.,2.16840434497101E-16)) ;
#128684=DIRECTION('center_axis',(0.,0.,1.)) ;
#128685=DIRECTION('ref_axis',(1.,0.,0.)) ;
#128686=DIRECTION('center_axis',(0.,1.,0.)) ;
#128687=DIRECTION('ref_axis',(0.,0.,1.)) ;
#128688=DIRECTION('center_axis',(0.,-1.,0.)) ;
#128689=DIRECTION('ref_axis',(0.,0.,-1.)) ;
#128690=DIRECTION('center_axis',(0.,1.,0.)) ;
#128691=DIRECTION('ref_axis',(1.,0.,0.)) ;
#128692=DIRECTION('center_axis',(0.,0.,1.)) ;
#128693=DIRECTION('ref_axis',(-1.,0.,0.)) ;
#128694=DIRECTION('center_axis',(0.,1.,0.)) ;
#128695=DIRECTION('ref_axis',(1.,0.,0.)) ;
#128696=DIRECTION('center_axis',(1.,0.,0.)) ;
#128697=DIRECTION('ref_axis',(0.,0.,1.)) ;
#128698=DIRECTION('center_axis',(0.,0.,-1.)) ;
#128699=DIRECTION('ref_axis',(-1.,0.,0.)) ;
#128700=DIRECTION('center_axis',(0.,0.,1.)) ;
#128701=DIRECTION('ref_axis',(1.,0.,0.)) ;
#128702=DIRECTION('center_axis',(1.,0.,2.16840434497101E-16)) ;
#128703=DIRECTION('ref_axis',(2.16840434497101E-16,0.,-1.)) ;
#128704=DIRECTION('center_axis',(1.,0.,0.)) ;
#128705=DIRECTION('ref_axis',(0.,0.,-1.)) ;
#128706=DIRECTION('center_axis',(0.,1.,0.)) ;
#128707=DIRECTION('ref_axis',(1.,0.,0.)) ;
#128708=DIRECTION('center_axis',(0.,1.,0.)) ;
#128709=DIRECTION('ref_axis',(0.,0.,-1.)) ;
#128710=DIRECTION('center_axis',(0.,1.,0.)) ;
#128711=DIRECTION('ref_axis',(0.,0.,1.)) ;
#128712=DIRECTION('center_axis',(0.,1.,0.)) ;
#128713=DIRECTION('ref_axis',(0.,0.,1.)) ;
#128714=DIRECTION('center_axis',(-0.942809041582063,-0.235702260395516,
0.235702260395518)) ;
#128715=DIRECTION('ref_axis',(0.242535625036335,4.64743530723282E-16,0.970142500145331)) ;
#128716=DIRECTION('center_axis',(-0.970142500145332,-0.242535625036331,
-2.10366121255613E-15)) ;
#128717=DIRECTION('ref_axis',(0.242535625036331,-0.970142500145332,-4.48415458566342E-30)) ;
#128718=DIRECTION('center_axis',(0.970142500145333,0.24253562503633,0.)) ;
#128719=DIRECTION('ref_axis',(-0.24253562503633,0.970142500145333,0.)) ;
#128720=DIRECTION('center_axis',(-0.970142500145332,-0.242535625036331,
-8.41464485022476E-15)) ;
#128721=DIRECTION('ref_axis',(0.242535625036331,-0.970142500145332,-1.80900724878918E-29)) ;
#128722=DIRECTION('center_axis',(0.879462917689188,0.219865729422294,-0.42214220049081)) ;
#128723=DIRECTION('ref_axis',(-0.432731067584771,1.71515946658E-16,-0.901523057468274)) ;
#128724=DIRECTION('center_axis',(0.879462917689185,0.219865729422304,-0.42214220049081)) ;
#128725=DIRECTION('ref_axis',(-0.432731067584772,-1.04304727837597E-16,
-0.901523057468273)) ;
#128726=DIRECTION('center_axis',(0.,1.,0.)) ;
#128727=DIRECTION('ref_axis',(1.,0.,0.)) ;
#128728=DIRECTION('center_axis',(-2.00438979995004E-14,-1.,0.)) ;
#128729=DIRECTION('ref_axis',(-1.,2.00438979995004E-14,0.)) ;
#128730=DIRECTION('center_axis',(0.,-1.,0.)) ;
#128731=DIRECTION('ref_axis',(0.,0.,-1.)) ;
#128732=DIRECTION('center_axis',(-4.51750905202295E-15,-1.,2.16840434497102E-15)) ;
#128733=DIRECTION('ref_axis',(1.,-4.51750905202295E-15,3.91831450274151E-31)) ;
#128734=DIRECTION('center_axis',(0.669589480006976,-0.669589480006974,-0.321402950403349)) ;
#128735=DIRECTION('ref_axis',(0.707106781186547,0.707106781186548,5.45170614306381E-16)) ;
#128736=DIRECTION('center_axis',(0.669589480006966,-0.669589480006966,-0.321402950403388)) ;
#128737=DIRECTION('ref_axis',(0.707106781186547,0.707106781186547,-1.18959821530046E-17)) ;
#128738=DIRECTION('center_axis',(0.,1.,0.)) ;
#128739=DIRECTION('ref_axis',(1.,0.,0.)) ;
#128740=DIRECTION('center_axis',(0.707106781186576,-0.707106781186519,0.)) ;
#128741=DIRECTION('ref_axis',(-0.707106781186519,-0.707106781186576,0.)) ;
#128742=DIRECTION('center_axis',(0.707106781186549,-0.707106781186546,0.)) ;
#128743=DIRECTION('ref_axis',(0.707106781186546,0.707106781186549,0.)) ;
#128744=DIRECTION('center_axis',(0.707106781186548,-0.707106781186548,-1.53329341668338E-15)) ;
#128745=DIRECTION('ref_axis',(0.707106781186548,0.707106781186548,1.5356898865553E-31)) ;
#128746=DIRECTION('center_axis',(0.577350269189622,-0.577350269189622,-0.577350269189634)) ;
#128747=DIRECTION('ref_axis',(-0.707106781186554,1.85551679542784E-15,-0.707106781186541)) ;
#128748=DIRECTION('center_axis',(-0.577350269189329,0.577350269189586,-0.577350269189963)) ;
#128749=DIRECTION('ref_axis',(-2.5143735500355E-15,0.707106781186777,0.707106781186318)) ;
#128750=DIRECTION('center_axis',(-0.707106781186548,0.707106781186548,7.66646708341692E-15)) ;
#128751=DIRECTION('ref_axis',(-0.707106781186548,-0.707106781186548,-2.68297081166629E-31)) ;
#128752=DIRECTION('center_axis',(-0.707106781186549,0.707106781186546,0.)) ;
#128753=DIRECTION('ref_axis',(-0.707106781186546,-0.707106781186549,0.)) ;
#128754=DIRECTION('center_axis',(-0.707106781186548,0.707106781186548,-1.22663473334671E-14)) ;
#128755=DIRECTION('ref_axis',(-0.707106781186548,-0.707106781186548,2.94725045705944E-31)) ;
#128756=DIRECTION('center_axis',(-0.669589480006976,0.669589480006974,-0.321402950403349)) ;
#128757=DIRECTION('ref_axis',(-0.707106781186547,-0.707106781186548,5.45170614306381E-16)) ;
#128758=DIRECTION('center_axis',(0.669589480006982,-0.669589480006966,0.321402950403353)) ;
#128759=DIRECTION('ref_axis',(0.707106781186539,0.707106781186556,5.77426876420606E-17)) ;
#128760=DIRECTION('center_axis',(0.,1.,0.)) ;
#128761=DIRECTION('ref_axis',(1.,0.,0.)) ;
#128762=DIRECTION('center_axis',(0.,1.,0.)) ;
#128763=DIRECTION('ref_axis',(0.,0.,-1.)) ;
#128764=DIRECTION('center_axis',(0.,-1.,0.)) ;
#128765=DIRECTION('ref_axis',(0.,0.,-1.)) ;
#128766=DIRECTION('center_axis',(0.,1.,0.)) ;
#128767=DIRECTION('ref_axis',(0.,0.,1.)) ;
#128768=DIRECTION('center_axis',(-0.879462917689188,-0.219865729422294,
-0.42214220049081)) ;
#128769=DIRECTION('ref_axis',(-0.432731067584771,1.71515946658E-16,0.901523057468274)) ;
#128770=DIRECTION('center_axis',(0.879462917689201,0.219865729422298,0.42214220049078)) ;
#128771=DIRECTION('ref_axis',(0.432731067584741,5.42470486237819E-16,-0.901523057468288)) ;
#128772=DIRECTION('center_axis',(0.,1.,0.)) ;
#128773=DIRECTION('ref_axis',(1.,0.,0.)) ;
#128774=DIRECTION('center_axis',(0.970142500145323,0.242535625036368,0.)) ;
#128775=DIRECTION('ref_axis',(0.242535625036368,-0.970142500145323,0.)) ;
#128776=DIRECTION('center_axis',(-0.970142500145333,-0.24253562503633,0.)) ;
#128777=DIRECTION('ref_axis',(0.24253562503633,-0.970142500145333,0.)) ;
#128778=DIRECTION('center_axis',(0.970142500145332,0.242535625036331,-2.10366121255617E-15)) ;
#128779=DIRECTION('ref_axis',(-0.242535625036331,0.970142500145332,-4.47980524894761E-30)) ;
#128780=DIRECTION('center_axis',(0.942809041582064,0.235702260395514,0.235702260395514)) ;
#128781=DIRECTION('ref_axis',(-0.242535625036331,0.970142500145332,4.49011373492972E-16)) ;
#128782=DIRECTION('center_axis',(0.,-1.,0.)) ;
#128783=DIRECTION('ref_axis',(0.,0.,-1.)) ;
#128784=DIRECTION('center_axis',(-1.,0.,-8.67361737988409E-15)) ;
#128785=DIRECTION('ref_axis',(-8.67361737988409E-15,0.,1.)) ;
#128786=DIRECTION('center_axis',(0.,0.,-1.)) ;
#128787=DIRECTION('ref_axis',(-1.,0.,0.)) ;
#128788=DIRECTION('center_axis',(0.,0.,-1.)) ;
#128789=DIRECTION('ref_axis',(-1.,0.,0.)) ;
#128790=DIRECTION('center_axis',(0.,0.,-1.)) ;
#128791=DIRECTION('ref_axis',(-1.,0.,0.)) ;
#128792=DIRECTION('center_axis',(1.,0.,0.)) ;
#128793=DIRECTION('ref_axis',(0.,0.,-1.)) ;
#128794=DIRECTION('center_axis',(-1.,0.,0.)) ;
#128795=DIRECTION('ref_axis',(0.,0.,1.)) ;
#128796=DIRECTION('center_axis',(0.,-1.,0.)) ;
#128797=DIRECTION('ref_axis',(0.,0.,-1.)) ;
#128798=DIRECTION('center_axis',(-1.,0.,0.)) ;
#128799=DIRECTION('ref_axis',(0.,0.,1.)) ;
#128800=DIRECTION('center_axis',(0.,-1.,0.)) ;
#128801=DIRECTION('ref_axis',(0.,0.,-1.)) ;
#128802=DIRECTION('center_axis',(0.,0.,-1.)) ;
#128803=DIRECTION('ref_axis',(-1.,0.,0.)) ;
#128804=DIRECTION('center_axis',(-1.,0.,0.)) ;
#128805=DIRECTION('ref_axis',(0.,0.,1.)) ;
#128806=DIRECTION('center_axis',(-1.,1.73472347597681E-14,0.)) ;
#128807=DIRECTION('ref_axis',(-1.73472347597681E-14,-1.,0.)) ;
#128808=DIRECTION('center_axis',(0.,0.,1.)) ;
#128809=DIRECTION('ref_axis',(1.,0.,0.)) ;
#128810=DIRECTION('center_axis',(0.,0.,-1.)) ;
#128811=DIRECTION('ref_axis',(-1.,0.,0.)) ;
#128812=DIRECTION('center_axis',(0.,-1.,0.)) ;
#128813=DIRECTION('ref_axis',(0.,0.,-1.)) ;
#128814=DIRECTION('center_axis',(0.,-1.,0.)) ;
#128815=DIRECTION('ref_axis',(0.,0.,-1.)) ;
#128816=DIRECTION('center_axis',(0.,-1.,0.)) ;
#128817=DIRECTION('ref_axis',(0.,0.,-1.)) ;
#128818=DIRECTION('center_axis',(0.,0.,1.)) ;
#128819=DIRECTION('ref_axis',(1.,0.,0.)) ;
#128820=DIRECTION('center_axis',(0.,0.,-1.)) ;
#128821=DIRECTION('ref_axis',(-1.,0.,0.)) ;
#128822=DIRECTION('center_axis',(0.,0.,1.)) ;
#128823=DIRECTION('ref_axis',(1.,0.,0.)) ;
#128824=DIRECTION('center_axis',(0.,-1.,0.)) ;
#128825=DIRECTION('ref_axis',(0.,0.,-1.)) ;
#128826=DIRECTION('center_axis',(0.,-1.,0.)) ;
#128827=DIRECTION('ref_axis',(0.,0.,-1.)) ;
#128828=DIRECTION('center_axis',(0.,1.,0.)) ;
#128829=DIRECTION('ref_axis',(1.,0.,0.)) ;
#128830=DIRECTION('center_axis',(-1.,0.,0.)) ;
#128831=DIRECTION('ref_axis',(0.,0.,-1.)) ;
#128832=DIRECTION('center_axis',(0.,1.,0.)) ;
#128833=DIRECTION('ref_axis',(1.,0.,0.)) ;
#128834=DIRECTION('center_axis',(-1.,0.,0.)) ;
#128835=DIRECTION('ref_axis',(0.,0.,-1.)) ;
#128836=DIRECTION('center_axis',(0.,-1.,0.)) ;
#128837=DIRECTION('ref_axis',(0.,0.,-1.)) ;
#128838=DIRECTION('center_axis',(0.,-1.,0.)) ;
#128839=DIRECTION('ref_axis',(0.,0.,-1.)) ;
#128840=DIRECTION('center_axis',(-1.,0.,0.)) ;
#128841=DIRECTION('ref_axis',(0.,0.,1.)) ;
#128842=DIRECTION('center_axis',(-1.,0.,0.)) ;
#128843=DIRECTION('ref_axis',(0.,0.,1.)) ;
#128844=DIRECTION('center_axis',(1.,0.,0.)) ;
#128845=DIRECTION('ref_axis',(0.,0.,-1.)) ;
#128846=DIRECTION('center_axis',(-1.,0.,0.)) ;
#128847=DIRECTION('ref_axis',(0.,0.,1.)) ;
#128848=DIRECTION('center_axis',(0.,-1.,0.)) ;
#128849=DIRECTION('ref_axis',(0.,0.,-1.)) ;
#128850=DIRECTION('center_axis',(0.,-1.,0.)) ;
#128851=DIRECTION('ref_axis',(0.,0.,-1.)) ;
#128852=DIRECTION('center_axis',(0.,1.,0.)) ;
#128853=DIRECTION('ref_axis',(1.,0.,0.)) ;
#128854=DIRECTION('center_axis',(0.,0.,-1.)) ;
#128855=DIRECTION('ref_axis',(1.,0.,0.)) ;
#128856=DIRECTION('center_axis',(0.,1.,0.)) ;
#128857=DIRECTION('ref_axis',(1.,0.,0.)) ;
#128858=DIRECTION('center_axis',(0.,0.,1.)) ;
#128859=DIRECTION('ref_axis',(-1.,0.,0.)) ;
#128860=DIRECTION('center_axis',(0.,0.,-1.)) ;
#128861=DIRECTION('ref_axis',(-1.,0.,0.)) ;
#128862=DIRECTION('center_axis',(1.,1.31418445149758E-16,-2.16840434497101E-16)) ;
#128863=DIRECTION('ref_axis',(-2.16840434497101E-16,-2.8496832747207E-32,
-1.)) ;
#128864=DIRECTION('center_axis',(1.,0.,0.)) ;
#128865=DIRECTION('ref_axis',(0.,0.,-1.)) ;
#128866=DIRECTION('center_axis',(-1.,0.,0.)) ;
#128867=DIRECTION('ref_axis',(0.,0.,1.)) ;
#128868=DIRECTION('center_axis',(-1.31418445149758E-16,1.,0.)) ;
#128869=DIRECTION('ref_axis',(-1.,0.,0.)) ;
#128870=DIRECTION('center_axis',(0.,0.,1.)) ;
#128871=DIRECTION('ref_axis',(-1.,0.,0.)) ;
#128872=DIRECTION('center_axis',(-1.31418445149758E-16,1.,0.)) ;
#128873=DIRECTION('ref_axis',(-1.,-1.31418445149758E-16,0.)) ;
#128874=DIRECTION('center_axis',(-1.31418445149758E-16,1.,0.)) ;
#128875=DIRECTION('ref_axis',(-1.,0.,0.)) ;
#128876=DIRECTION('center_axis',(-1.31418445149758E-16,1.,0.)) ;
#128877=DIRECTION('ref_axis',(-1.,-1.31418445149758E-16,0.)) ;
#128878=DIRECTION('center_axis',(0.,0.,1.)) ;
#128879=DIRECTION('ref_axis',(-1.,0.,0.)) ;
#128880=DIRECTION('center_axis',(-4.33680868994202E-16,-5.69936654944139E-32,
-1.)) ;
#128881=DIRECTION('ref_axis',(-1.,2.47170623787823E-47,4.33680868994202E-16)) ;
#128882=DIRECTION('center_axis',(0.,0.,1.)) ;
#128883=DIRECTION('ref_axis',(1.,0.,0.)) ;
#128884=DIRECTION('center_axis',(-1.31418445149758E-16,-1.,0.)) ;
#128885=DIRECTION('ref_axis',(1.,-1.31418445149758E-16,0.)) ;
#128886=DIRECTION('center_axis',(0.,1.,0.)) ;
#128887=DIRECTION('ref_axis',(0.,0.,1.)) ;
#128888=DIRECTION('center_axis',(-1.,0.,2.16840434497101E-16)) ;
#128889=DIRECTION('ref_axis',(2.16840434497101E-16,0.,1.)) ;
#128890=DIRECTION('center_axis',(-1.,0.,0.)) ;
#128891=DIRECTION('ref_axis',(0.,0.,1.)) ;
#128892=DIRECTION('center_axis',(1.,0.,0.)) ;
#128893=DIRECTION('ref_axis',(0.,0.,-1.)) ;
#128894=DIRECTION('center_axis',(-1.31418445149758E-16,-1.,0.)) ;
#128895=DIRECTION('ref_axis',(1.,-1.31418445149758E-16,0.)) ;
#128896=DIRECTION('center_axis',(0.,1.,0.)) ;
#128897=DIRECTION('ref_axis',(0.,0.,1.)) ;
#128898=DIRECTION('center_axis',(2.16840434497101E-16,2.8496832747207E-32,
1.)) ;
#128899=DIRECTION('ref_axis',(1.,-6.17926559469557E-48,-2.16840434497101E-16)) ;
#128900=DIRECTION('center_axis',(0.,0.,1.)) ;
#128901=DIRECTION('ref_axis',(1.,0.,0.)) ;
#128902=DIRECTION('center_axis',(-1.,-1.31418445149758E-16,-2.16840434497101E-16)) ;
#128903=DIRECTION('ref_axis',(-2.16840434497101E-16,-2.8496832747207E-32,
1.)) ;
#128904=DIRECTION('center_axis',(-1.,0.,0.)) ;
#128905=DIRECTION('ref_axis',(0.,0.,1.)) ;
#128906=DIRECTION('center_axis',(1.,0.,0.)) ;
#128907=DIRECTION('ref_axis',(0.,0.,-1.)) ;
#128908=DIRECTION('center_axis',(-1.31418445149758E-16,1.,0.)) ;
#128909=DIRECTION('ref_axis',(-1.,0.,0.)) ;
#128910=DIRECTION('center_axis',(-1.31418445149758E-16,1.,0.)) ;
#128911=DIRECTION('ref_axis',(-1.,-1.31418445149758E-16,0.)) ;
#128912=DIRECTION('center_axis',(0.,1.,0.)) ;
#128913=DIRECTION('ref_axis',(1.,0.,0.)) ;
#128914=DIRECTION('center_axis',(0.,0.,-1.)) ;
#128915=DIRECTION('ref_axis',(1.,0.,0.)) ;
#128916=DIRECTION('center_axis',(0.,1.,0.)) ;
#128917=DIRECTION('ref_axis',(1.,0.,0.)) ;
#128918=DIRECTION('center_axis',(0.,0.,-1.)) ;
#128919=DIRECTION('ref_axis',(1.,0.,0.)) ;
#128920=DIRECTION('center_axis',(-1.31418445149758E-16,1.,0.)) ;
#128921=DIRECTION('ref_axis',(-1.,0.,0.)) ;
#128922=DIRECTION('center_axis',(-1.31418445149758E-16,1.,0.)) ;
#128923=DIRECTION('ref_axis',(-1.,-1.31418445149758E-16,0.)) ;
#128924=DIRECTION('center_axis',(-1.31418445149758E-16,-1.,0.)) ;
#128925=DIRECTION('ref_axis',(1.,-1.31418445149758E-16,0.)) ;
#128926=DIRECTION('center_axis',(0.,1.,0.)) ;
#128927=DIRECTION('ref_axis',(0.,0.,1.)) ;
#128928=DIRECTION('center_axis',(4.33680868994202E-16,0.,1.)) ;
#128929=DIRECTION('ref_axis',(1.,0.,-4.33680868994202E-16)) ;
#128930=DIRECTION('center_axis',(0.,0.,-1.)) ;
#128931=DIRECTION('ref_axis',(-1.,0.,0.)) ;
#128932=DIRECTION('center_axis',(-2.16840434497101E-16,0.,-1.)) ;
#128933=DIRECTION('ref_axis',(-1.,0.,2.16840434497101E-16)) ;
#128934=DIRECTION('center_axis',(0.,0.,-1.)) ;
#128935=DIRECTION('ref_axis',(-1.,0.,0.)) ;
#128936=DIRECTION('center_axis',(-1.31418445149758E-16,-1.,0.)) ;
#128937=DIRECTION('ref_axis',(1.,-1.31418445149758E-16,0.)) ;
#128938=DIRECTION('center_axis',(0.,1.,0.)) ;
#128939=DIRECTION('ref_axis',(0.,0.,1.)) ;
#128940=DIRECTION('center_axis',(0.,1.,0.)) ;
#128941=DIRECTION('ref_axis',(1.,0.,0.)) ;
#128942=DIRECTION('center_axis',(-1.,0.,0.)) ;
#128943=DIRECTION('ref_axis',(0.,0.,-1.)) ;
#128944=DIRECTION('center_axis',(0.,1.,0.)) ;
#128945=DIRECTION('ref_axis',(1.,0.,0.)) ;
#128946=DIRECTION('center_axis',(1.,0.,0.)) ;
#128947=DIRECTION('ref_axis',(0.,0.,1.)) ;
#128948=DIRECTION('center_axis',(1.,0.,2.16840434497101E-16)) ;
#128949=DIRECTION('ref_axis',(2.16840434497101E-16,0.,-1.)) ;
#128950=DIRECTION('center_axis',(0.,1.,0.)) ;
#128951=DIRECTION('ref_axis',(0.,0.,1.)) ;
#128952=DIRECTION('center_axis',(0.,1.,0.)) ;
#128953=DIRECTION('ref_axis',(0.,0.,1.)) ;
#128954=DIRECTION('center_axis',(0.,0.,-1.)) ;
#128955=DIRECTION('ref_axis',(-1.,0.,0.)) ;
#128956=DIRECTION('center_axis',(0.,0.,1.)) ;
#128957=DIRECTION('ref_axis',(1.,0.,0.)) ;
#128958=DIRECTION('center_axis',(0.,0.,-1.)) ;
#128959=DIRECTION('ref_axis',(-1.,0.,0.)) ;
#128960=DIRECTION('center_axis',(0.,1.,0.)) ;
#128961=DIRECTION('ref_axis',(0.,0.,1.)) ;
#128962=DIRECTION('center_axis',(0.,1.,0.)) ;
#128963=DIRECTION('ref_axis',(0.,0.,1.)) ;
#128964=DIRECTION('center_axis',(0.,1.,0.)) ;
#128965=DIRECTION('ref_axis',(1.,0.,0.)) ;
#128966=DIRECTION('center_axis',(-1.,0.,0.)) ;
#128967=DIRECTION('ref_axis',(0.,0.,-1.)) ;
#128968=DIRECTION('center_axis',(0.,1.,0.)) ;
#128969=DIRECTION('ref_axis',(1.,0.,0.)) ;
#128970=DIRECTION('center_axis',(-1.,0.,0.)) ;
#128971=DIRECTION('ref_axis',(0.,0.,-1.)) ;
#128972=DIRECTION('center_axis',(0.,1.,0.)) ;
#128973=DIRECTION('ref_axis',(0.,0.,1.)) ;
#128974=DIRECTION('center_axis',(0.,1.,0.)) ;
#128975=DIRECTION('ref_axis',(0.,0.,1.)) ;
#128976=DIRECTION('center_axis',(-1.,0.,0.)) ;
#128977=DIRECTION('ref_axis',(0.,0.,1.)) ;
#128978=DIRECTION('center_axis',(-1.,0.,0.)) ;
#128979=DIRECTION('ref_axis',(0.,0.,1.)) ;
#128980=DIRECTION('center_axis',(1.,0.,0.)) ;
#128981=DIRECTION('ref_axis',(0.,0.,-1.)) ;
#128982=DIRECTION('center_axis',(-1.,0.,0.)) ;
#128983=DIRECTION('ref_axis',(0.,0.,1.)) ;
#128984=DIRECTION('center_axis',(0.,1.,0.)) ;
#128985=DIRECTION('ref_axis',(0.,0.,1.)) ;
#128986=DIRECTION('center_axis',(0.,1.,0.)) ;
#128987=DIRECTION('ref_axis',(0.,0.,1.)) ;
#128988=DIRECTION('center_axis',(0.,1.,0.)) ;
#128989=DIRECTION('ref_axis',(1.,0.,0.)) ;
#128990=DIRECTION('center_axis',(0.,0.,1.)) ;
#128991=DIRECTION('ref_axis',(-1.,0.,0.)) ;
#128992=DIRECTION('center_axis',(0.,1.,0.)) ;
#128993=DIRECTION('ref_axis',(1.,0.,0.)) ;
#128994=DIRECTION('center_axis',(0.,0.,-1.)) ;
#128995=DIRECTION('ref_axis',(1.,0.,0.)) ;
#128996=DIRECTION('center_axis',(0.,0.,1.)) ;
#128997=DIRECTION('ref_axis',(1.,0.,0.)) ;
#128998=DIRECTION('center_axis',(0.,0.,1.)) ;
#128999=DIRECTION('ref_axis',(1.,0.,0.)) ;
#129000=DIRECTION('center_axis',(0.,0.,-1.)) ;
#129001=DIRECTION('ref_axis',(-1.,0.,0.)) ;
#129002=DIRECTION('center_axis',(0.,0.,1.)) ;
#129003=DIRECTION('ref_axis',(1.,0.,0.)) ;
#129004=DIRECTION('center_axis',(1.,0.,0.)) ;
#129005=DIRECTION('ref_axis',(0.,0.,-1.)) ;
#129006=DIRECTION('center_axis',(1.,0.,0.)) ;
#129007=DIRECTION('ref_axis',(0.,0.,-1.)) ;
#129008=DIRECTION('center_axis',(1.,0.,0.)) ;
#129009=DIRECTION('ref_axis',(0.,0.,-1.)) ;
#129010=DIRECTION('center_axis',(1.,0.,8.67361737988409E-15)) ;
#129011=DIRECTION('ref_axis',(8.67361737988409E-15,0.,-1.)) ;
#129012=DIRECTION('center_axis',(1.,0.,0.)) ;
#129013=DIRECTION('ref_axis',(0.,0.,-1.)) ;
#129014=DIRECTION('center_axis',(1.,0.,1.73472347597682E-14)) ;
#129015=DIRECTION('ref_axis',(1.73472347597682E-14,0.,-1.)) ;
#129016=DIRECTION('center_axis',(-1.,0.,0.)) ;
#129017=DIRECTION('ref_axis',(0.,0.,1.)) ;
#129018=DIRECTION('center_axis',(1.,0.,0.)) ;
#129019=DIRECTION('ref_axis',(0.,0.,-1.)) ;
#129020=DIRECTION('center_axis',(1.,0.,0.)) ;
#129021=DIRECTION('ref_axis',(0.,0.,-1.)) ;
#129022=DIRECTION('center_axis',(0.,0.,-1.)) ;
#129023=DIRECTION('ref_axis',(-1.,0.,0.)) ;
#129024=DIRECTION('center_axis',(1.,0.,0.)) ;
#129025=DIRECTION('ref_axis',(0.,0.,-1.)) ;
#129026=DIRECTION('center_axis',(0.,0.,1.)) ;
#129027=DIRECTION('ref_axis',(1.,0.,0.)) ;
#129028=DIRECTION('center_axis',(0.,0.,-1.)) ;
#129029=DIRECTION('ref_axis',(-1.,0.,0.)) ;
#129030=DIRECTION('center_axis',(-0.422618261740697,5.55398348498559E-17,
0.906307787036651)) ;
#129031=DIRECTION('ref_axis',(0.906307787036651,-2.19407316623673E-31,0.422618261740697)) ;
#129032=DIRECTION('center_axis',(0.422618261740697,-5.55398348498559E-17,
-0.906307787036651)) ;
#129033=DIRECTION('ref_axis',(-0.906307787036651,2.28174878574772E-31,-0.422618261740697)) ;
#129034=DIRECTION('center_axis',(-0.422618261740697,5.55398348498559E-17,
0.906307787036651)) ;
#129035=DIRECTION('ref_axis',(0.906307787036651,-2.28174878574772E-31,0.422618261740697)) ;
#129036=DIRECTION('center_axis',(0.422618261740697,-5.55398348498559E-17,
-0.906307787036651)) ;
#129037=DIRECTION('ref_axis',(-0.906307787036651,2.28174878574772E-31,-0.422618261740697)) ;
#129038=DIRECTION('center_axis',(0.,1.,0.)) ;
#129039=DIRECTION('ref_axis',(1.,0.,0.)) ;
#129040=DIRECTION('center_axis',(3.4216004848576E-14,0.514231796959095,
-0.857651245551606)) ;
#129041=DIRECTION('ref_axis',(3.46944695195362E-14,-0.857651245551606,-0.514231796959095)) ;
#129042=DIRECTION('center_axis',(0.,-3.46944695195362E-14,1.)) ;
#129043=DIRECTION('ref_axis',(0.,1.,3.46944695195362E-14)) ;
#129044=DIRECTION('center_axis',(-1.,0.,0.)) ;
#129045=DIRECTION('ref_axis',(0.,-4.33680868994204E-15,-1.)) ;
#129046=DIRECTION('center_axis',(0.,0.,1.)) ;
#129047=DIRECTION('ref_axis',(1.,0.,0.)) ;
#129048=DIRECTION('center_axis',(0.,0.,1.)) ;
#129049=DIRECTION('ref_axis',(1.,0.,0.)) ;
#129050=DIRECTION('center_axis',(-1.,0.,0.)) ;
#129051=DIRECTION('ref_axis',(0.,0.,1.)) ;
#129052=DIRECTION('center_axis',(-1.,0.,0.)) ;
#129053=DIRECTION('ref_axis',(0.,-4.33680868994204E-15,-1.)) ;
#129054=DIRECTION('center_axis',(1.,0.,0.)) ;
#129055=DIRECTION('ref_axis',(0.,0.,-1.)) ;
#129056=DIRECTION('center_axis',(0.,-0.514231796959124,-0.857651245551588)) ;
#129057=DIRECTION('ref_axis',(0.,0.857651245551588,-0.514231796959124)) ;
#129058=DIRECTION('center_axis',(0.,1.,8.97270763436279E-17)) ;
#129059=DIRECTION('ref_axis',(0.,-8.97270763436279E-17,1.)) ;
#129060=DIRECTION('center_axis',(0.,-1.,-8.97270763436279E-17)) ;
#129061=DIRECTION('ref_axis',(0.,-8.97270763436279E-17,1.)) ;
#129062=DIRECTION('center_axis',(0.,-1.,0.)) ;
#129063=DIRECTION('ref_axis',(0.,0.,-1.)) ;
#129064=DIRECTION('center_axis',(0.,1.,0.)) ;
#129065=DIRECTION('ref_axis',(1.,0.,0.)) ;
#129066=DIRECTION('center_axis',(-1.,0.,0.)) ;
#129067=DIRECTION('ref_axis',(0.,0.,-1.)) ;
#129068=DIRECTION('center_axis',(1.,0.,0.)) ;
#129069=DIRECTION('ref_axis',(0.,0.,-1.)) ;
#129070=DIRECTION('center_axis',(0.,-0.514231796959093,0.857651245551607)) ;
#129071=DIRECTION('ref_axis',(0.,0.857651245551607,0.514231796959093)) ;
#129072=DIRECTION('center_axis',(0.,0.,-1.)) ;
#129073=DIRECTION('ref_axis',(1.,0.,0.)) ;
#129074=DIRECTION('center_axis',(0.,1.,0.)) ;
#129075=DIRECTION('ref_axis',(1.,0.,0.)) ;
#129076=DIRECTION('center_axis',(-3.46944695195364E-14,0.,-1.)) ;
#129077=DIRECTION('ref_axis',(1.,0.,-3.46944695195364E-14)) ;
#129078=DIRECTION('center_axis',(-1.,0.,0.)) ;
#129079=DIRECTION('ref_axis',(0.,4.33680868994204E-15,-1.)) ;
#129080=DIRECTION('center_axis',(0.,0.,-1.)) ;
#129081=DIRECTION('ref_axis',(-1.,0.,0.)) ;
#129082=DIRECTION('center_axis',(0.,0.,1.)) ;
#129083=DIRECTION('ref_axis',(-1.,0.,0.)) ;
#129084=DIRECTION('center_axis',(0.,0.,-1.)) ;
#129085=DIRECTION('ref_axis',(-1.,0.,0.)) ;
#129086=DIRECTION('center_axis',(-1.,0.,7.01133629567814E-33)) ;
#129087=DIRECTION('ref_axis',(7.01133629567814E-33,0.,1.)) ;
#129088=DIRECTION('center_axis',(-1.,0.,0.)) ;
#129089=DIRECTION('ref_axis',(0.,0.,1.)) ;
#129090=DIRECTION('center_axis',(0.,0.,-1.)) ;
#129091=DIRECTION('ref_axis',(-1.,0.,0.)) ;
#129092=DIRECTION('center_axis',(-7.01133629567814E-33,8.97270763436279E-17,
-1.)) ;
#129093=DIRECTION('ref_axis',(6.29106707073161E-49,1.,8.97270763436279E-17)) ;
#129094=DIRECTION('center_axis',(1.,0.,0.)) ;
#129095=DIRECTION('ref_axis',(0.,0.,-1.)) ;
#129096=DIRECTION('center_axis',(-2.2301249256967E-15,0.514231796959095,
0.857651245551606)) ;
#129097=DIRECTION('ref_axis',(-4.79361507851841E-30,-0.857651245551606,
0.514231796959095)) ;
#129098=DIRECTION('center_axis',(-1.,0.,0.)) ;
#129099=DIRECTION('ref_axis',(0.,0.,1.)) ;
#129100=DIRECTION('center_axis',(-1.,0.,0.)) ;
#129101=DIRECTION('ref_axis',(0.,-4.33680868994204E-15,-1.)) ;
#129102=DIRECTION('center_axis',(0.,0.,1.)) ;
#129103=DIRECTION('ref_axis',(1.,0.,0.)) ;
#129104=DIRECTION('center_axis',(0.,0.,-1.)) ;
#129105=DIRECTION('ref_axis',(-1.,0.,0.)) ;
#129106=DIRECTION('center_axis',(0.,-1.,8.97270763436279E-17)) ;
#129107=DIRECTION('ref_axis',(0.,-8.97270763436279E-17,-1.)) ;
#129108=DIRECTION('center_axis',(0.,-1.,8.97270763436279E-17)) ;
#129109=DIRECTION('ref_axis',(0.,-8.97270763436279E-17,-1.)) ;
#129110=DIRECTION('center_axis',(0.,-1.,0.)) ;
#129111=DIRECTION('ref_axis',(0.,0.,-1.)) ;
#129112=DIRECTION('center_axis',(-7.01133629567814E-33,8.97270763436279E-17,
-1.)) ;
#129113=DIRECTION('ref_axis',(0.,1.,0.)) ;
#129114=DIRECTION('center_axis',(0.,-1.,0.)) ;
#129115=DIRECTION('ref_axis',(0.,0.,1.)) ;
#129116=DIRECTION('center_axis',(1.,0.,0.)) ;
#129117=DIRECTION('ref_axis',(0.,0.,-1.)) ;
#129118=DIRECTION('center_axis',(0.,0.,1.)) ;
#129119=DIRECTION('ref_axis',(-1.,0.,0.)) ;
#129120=DIRECTION('center_axis',(0.,1.,0.)) ;
#129121=DIRECTION('ref_axis',(1.,0.,0.)) ;
#129122=DIRECTION('center_axis',(-1.,0.,0.)) ;
#129123=DIRECTION('ref_axis',(0.,0.,-1.)) ;
#129124=DIRECTION('center_axis',(1.,7.81406971160724E-17,0.)) ;
#129125=DIRECTION('ref_axis',(-7.81406971160724E-17,1.,0.)) ;
#129126=DIRECTION('center_axis',(1.,0.,0.)) ;
#129127=DIRECTION('ref_axis',(0.,0.,-1.)) ;
#129128=DIRECTION('center_axis',(1.,0.,0.)) ;
#129129=DIRECTION('ref_axis',(0.,0.,-1.)) ;
#129130=DIRECTION('center_axis',(0.,1.,8.97270763436279E-17)) ;
#129131=DIRECTION('ref_axis',(0.,-8.97270763436279E-17,1.)) ;
#129132=DIRECTION('center_axis',(0.,-1.,0.)) ;
#129133=DIRECTION('ref_axis',(0.,0.,-1.)) ;
#129134=DIRECTION('center_axis',(0.,0.,-1.)) ;
#129135=DIRECTION('ref_axis',(-1.,0.,0.)) ;
#129136=DIRECTION('center_axis',(-7.01133629567814E-33,8.97270763436279E-17,
1.)) ;
#129137=DIRECTION('ref_axis',(-6.29106707073161E-49,-1.,8.97270763436279E-17)) ;
#129138=DIRECTION('center_axis',(-1.,0.,-7.01133629567814E-33)) ;
#129139=DIRECTION('ref_axis',(-7.01133629567814E-33,0.,1.)) ;
#129140=DIRECTION('center_axis',(-1.,0.,0.)) ;
#129141=DIRECTION('ref_axis',(0.,0.,1.)) ;
#129142=DIRECTION('center_axis',(1.,0.,0.)) ;
#129143=DIRECTION('ref_axis',(0.,1.,0.)) ;
#129144=DIRECTION('center_axis',(4.33680868994202E-15,1.,0.)) ;
#129145=DIRECTION('ref_axis',(-1.,4.33680868994202E-15,0.)) ;
#129146=DIRECTION('center_axis',(0.,1.,0.)) ;
#129147=DIRECTION('ref_axis',(1.,0.,0.)) ;
#129148=DIRECTION('center_axis',(0.,0.,-1.)) ;
#129149=DIRECTION('ref_axis',(1.,0.,0.)) ;
#129150=DIRECTION('center_axis',(-1.,0.,0.)) ;
#129151=DIRECTION('ref_axis',(0.,0.,-1.)) ;
#129152=DIRECTION('center_axis',(-7.01133629567814E-33,8.97270763436279E-17,
1.)) ;
#129153=DIRECTION('ref_axis',(0.,-1.,0.)) ;
#129154=DIRECTION('center_axis',(0.,-1.,0.)) ;
#129155=DIRECTION('ref_axis',(0.,0.,1.)) ;
#129156=DIRECTION('center_axis',(7.81406971160724E-17,-1.,-8.97270763436279E-17)) ;
#129157=DIRECTION('ref_axis',(-7.01133629567814E-33,8.97270763436279E-17,
-1.)) ;
#129158=DIRECTION('center_axis',(0.,1.,0.)) ;
#129159=DIRECTION('ref_axis',(0.,0.,1.)) ;
#129160=DIRECTION('center_axis',(-1.,-7.81406971160724E-17,0.)) ;
#129161=DIRECTION('ref_axis',(7.81406971160724E-17,-1.,0.)) ;
#129162=DIRECTION('center_axis',(-1.,-7.81406971160724E-17,0.)) ;
#129163=DIRECTION('ref_axis',(-7.81406971160724E-17,1.,0.)) ;
#129164=DIRECTION('center_axis',(0.,0.,1.)) ;
#129165=DIRECTION('ref_axis',(1.,0.,0.)) ;
#129166=DIRECTION('center_axis',(0.,0.,-1.)) ;
#129167=DIRECTION('ref_axis',(-1.,0.,0.)) ;
#129168=DIRECTION('center_axis',(0.,-1.,8.97270763436279E-17)) ;
#129169=DIRECTION('ref_axis',(0.,-8.97270763436279E-17,-1.)) ;
#129170=DIRECTION('center_axis',(0.,-1.,0.)) ;
#129171=DIRECTION('ref_axis',(0.,0.,-1.)) ;
#129172=DIRECTION('center_axis',(1.,7.81406971160724E-17,0.)) ;
#129173=DIRECTION('ref_axis',(0.,1.,0.)) ;
#129174=DIRECTION('center_axis',(0.,0.,1.)) ;
#129175=DIRECTION('ref_axis',(-1.,0.,0.)) ;
#129176=DIRECTION('center_axis',(0.,1.,0.)) ;
#129177=DIRECTION('ref_axis',(1.,0.,0.)) ;
#129178=DIRECTION('center_axis',(-1.,0.,0.)) ;
#129179=DIRECTION('ref_axis',(0.,0.,-1.)) ;
#129180=DIRECTION('center_axis',(0.,0.,-1.)) ;
#129181=DIRECTION('ref_axis',(-1.,0.,0.)) ;
#129182=DIRECTION('center_axis',(0.,0.,1.)) ;
#129183=DIRECTION('ref_axis',(1.,0.,0.)) ;
#129184=DIRECTION('center_axis',(-1.,-7.81406971160724E-17,0.)) ;
#129185=DIRECTION('ref_axis',(7.81406971160724E-17,-1.,0.)) ;
#129186=DIRECTION('center_axis',(-1.,-7.81406971160724E-17,0.)) ;
#129187=DIRECTION('ref_axis',(-7.81406971160724E-17,1.,0.)) ;
#129188=DIRECTION('center_axis',(1.,7.81406971160724E-17,0.)) ;
#129189=DIRECTION('ref_axis',(-7.81406971160724E-17,1.,0.)) ;
#129190=DIRECTION('center_axis',(1.,0.,0.)) ;
#129191=DIRECTION('ref_axis',(0.,0.,-1.)) ;
#129192=DIRECTION('center_axis',(1.,0.,0.)) ;
#129193=DIRECTION('ref_axis',(0.,0.,-1.)) ;
#129194=DIRECTION('center_axis',(3.78638272950961E-32,-4.8455963016112E-16,
-1.)) ;
#129195=DIRECTION('ref_axis',(1.83472821505963E-47,1.,-4.8455963016112E-16)) ;
#129196=DIRECTION('center_axis',(3.78638272950961E-32,-4.8455963016112E-16,
-1.)) ;
#129197=DIRECTION('ref_axis',(1.83472821505963E-47,1.,-4.8455963016112E-16)) ;
#129198=DIRECTION('center_axis',(0.,0.,-1.)) ;
#129199=DIRECTION('ref_axis',(-1.,0.,0.)) ;
#129200=DIRECTION('center_axis',(1.,7.81406971160724E-17,0.)) ;
#129201=DIRECTION('ref_axis',(0.,1.,0.)) ;
#129202=DIRECTION('center_axis',(0.,-1.,0.)) ;
#129203=DIRECTION('ref_axis',(0.,0.,1.)) ;
#129204=DIRECTION('center_axis',(0.,1.,0.)) ;
#129205=DIRECTION('ref_axis',(1.,0.,0.)) ;
#129206=DIRECTION('center_axis',(0.,1.,0.)) ;
#129207=DIRECTION('ref_axis',(0.,0.,-1.)) ;
#129208=DIRECTION('center_axis',(-7.81406971160724E-17,1.,-8.97270763436279E-17)) ;
#129209=DIRECTION('ref_axis',(-7.01133629567814E-33,8.97270763436279E-17,
1.)) ;
#129210=DIRECTION('center_axis',(0.,-1.,0.)) ;
#129211=DIRECTION('ref_axis',(0.,0.,-1.)) ;
#129212=DIRECTION('center_axis',(0.,1.,0.)) ;
#129213=DIRECTION('ref_axis',(0.,0.,1.)) ;
#129214=DIRECTION('center_axis',(0.,-1.,0.)) ;
#129215=DIRECTION('ref_axis',(0.,0.,-1.)) ;
#129216=DIRECTION('center_axis',(0.,-1.,0.)) ;
#129217=DIRECTION('ref_axis',(0.,0.,-1.)) ;
#129218=DIRECTION('center_axis',(0.,1.,0.)) ;
#129219=DIRECTION('ref_axis',(1.,0.,0.)) ;
#129220=DIRECTION('center_axis',(0.,0.,1.)) ;
#129221=DIRECTION('ref_axis',(-1.,0.,0.)) ;
#129222=DIRECTION('center_axis',(1.,0.,0.)) ;
#129223=DIRECTION('ref_axis',(0.,0.,1.)) ;
#129224=DIRECTION('center_axis',(0.,-1.,0.)) ;
#129225=DIRECTION('ref_axis',(0.,0.,-1.)) ;
#129226=DIRECTION('center_axis',(0.,1.,0.)) ;
#129227=DIRECTION('ref_axis',(0.,0.,1.)) ;
#129228=DIRECTION('center_axis',(0.,-1.,0.)) ;
#129229=DIRECTION('ref_axis',(0.,0.,-1.)) ;
#129230=DIRECTION('center_axis',(-1.,0.,2.16840434497101E-16)) ;
#129231=DIRECTION('ref_axis',(2.16840434497101E-16,0.,1.)) ;
#129232=DIRECTION('center_axis',(1.,0.,0.)) ;
#129233=DIRECTION('ref_axis',(0.,0.,-1.)) ;
#129234=DIRECTION('center_axis',(-2.16840434497101E-16,0.,1.)) ;
#129235=DIRECTION('ref_axis',(1.,0.,2.16840434497101E-16)) ;
#129236=DIRECTION('center_axis',(0.,0.,1.)) ;
#129237=DIRECTION('ref_axis',(1.,0.,0.)) ;
#129238=DIRECTION('center_axis',(0.,1.,0.)) ;
#129239=DIRECTION('ref_axis',(0.,0.,1.)) ;
#129240=DIRECTION('center_axis',(0.,-1.,0.)) ;
#129241=DIRECTION('ref_axis',(0.,0.,-1.)) ;
#129242=DIRECTION('center_axis',(0.,1.,0.)) ;
#129243=DIRECTION('ref_axis',(1.,0.,0.)) ;
#129244=DIRECTION('center_axis',(0.,0.,1.)) ;
#129245=DIRECTION('ref_axis',(-1.,0.,0.)) ;
#129246=DIRECTION('center_axis',(0.,1.,0.)) ;
#129247=DIRECTION('ref_axis',(1.,0.,0.)) ;
#129248=DIRECTION('center_axis',(1.,0.,0.)) ;
#129249=DIRECTION('ref_axis',(0.,0.,1.)) ;
#129250=DIRECTION('center_axis',(0.,0.,-1.)) ;
#129251=DIRECTION('ref_axis',(-1.,0.,0.)) ;
#129252=DIRECTION('center_axis',(0.,0.,1.)) ;
#129253=DIRECTION('ref_axis',(1.,0.,0.)) ;
#129254=DIRECTION('center_axis',(1.,0.,2.16840434497101E-16)) ;
#129255=DIRECTION('ref_axis',(2.16840434497101E-16,0.,-1.)) ;
#129256=DIRECTION('center_axis',(1.,0.,0.)) ;
#129257=DIRECTION('ref_axis',(0.,0.,-1.)) ;
#129258=DIRECTION('center_axis',(0.,1.,0.)) ;
#129259=DIRECTION('ref_axis',(1.,0.,0.)) ;
#129260=DIRECTION('center_axis',(0.,1.,0.)) ;
#129261=DIRECTION('ref_axis',(0.,0.,-1.)) ;
#129262=DIRECTION('center_axis',(0.,1.,0.)) ;
#129263=DIRECTION('ref_axis',(0.,0.,1.)) ;
#129264=DIRECTION('center_axis',(0.,1.,0.)) ;
#129265=DIRECTION('ref_axis',(0.,0.,1.)) ;
#129266=DIRECTION('center_axis',(-0.942809041582063,-0.235702260395516,
0.235702260395518)) ;
#129267=DIRECTION('ref_axis',(0.242535625036335,4.64743530723282E-16,0.970142500145331)) ;
#129268=DIRECTION('center_axis',(-0.970142500145332,-0.242535625036331,
-2.10366121255617E-15)) ;
#129269=DIRECTION('ref_axis',(0.242535625036331,-0.970142500145332,-4.47980524894761E-30)) ;
#129270=DIRECTION('center_axis',(0.970142500145333,0.24253562503633,0.)) ;
#129271=DIRECTION('ref_axis',(-0.24253562503633,0.970142500145333,0.)) ;
#129272=DIRECTION('center_axis',(-0.970142500145332,-0.242535625036331,
2.73475957632304E-14)) ;
#129273=DIRECTION('ref_axis',(0.242535625036331,-0.970142500145332,1.1454669517322E-30)) ;
#129274=DIRECTION('center_axis',(0.879462917689188,0.219865729422294,-0.42214220049081)) ;
#129275=DIRECTION('ref_axis',(-0.432731067584771,1.71515946658E-16,-0.901523057468274)) ;
#129276=DIRECTION('center_axis',(0.879462917689192,0.219865729422271,-0.422142200490814)) ;
#129277=DIRECTION('ref_axis',(-0.432731067584773,-1.62351711522009E-16,
-0.901523057468273)) ;
#129278=DIRECTION('center_axis',(0.,1.,0.)) ;
#129279=DIRECTION('ref_axis',(1.,0.,0.)) ;
#129280=DIRECTION('center_axis',(0.,-1.,0.)) ;
#129281=DIRECTION('ref_axis',(0.,0.,1.)) ;
#129282=DIRECTION('center_axis',(0.,-1.,0.)) ;
#129283=DIRECTION('ref_axis',(0.,0.,-1.)) ;
#129284=DIRECTION('center_axis',(-4.51750905202295E-15,-1.,2.16840434497102E-15)) ;
#129285=DIRECTION('ref_axis',(1.,-4.51750905202295E-15,3.91831450274151E-31)) ;
#129286=DIRECTION('center_axis',(0.669589480006976,-0.669589480006974,-0.321402950403349)) ;
#129287=DIRECTION('ref_axis',(0.707106781186547,0.707106781186548,5.45170614306381E-16)) ;
#129288=DIRECTION('center_axis',(0.669589480006977,-0.669589480006977,-0.321402950403342)) ;
#129289=DIRECTION('ref_axis',(0.707106781186547,0.707106781186548,-1.94221176494188E-16)) ;
#129290=DIRECTION('center_axis',(0.,1.,0.)) ;
#129291=DIRECTION('ref_axis',(1.,0.,0.)) ;
#129292=DIRECTION('center_axis',(0.707106781186541,-0.707106781186554,0.)) ;
#129293=DIRECTION('ref_axis',(-0.707106781186554,-0.707106781186541,0.)) ;
#129294=DIRECTION('center_axis',(0.707106781186549,-0.707106781186546,0.)) ;
#129295=DIRECTION('ref_axis',(0.707106781186546,0.707106781186549,0.)) ;
#129296=DIRECTION('center_axis',(0.707106781186548,-0.707106781186548,-1.53329341668338E-15)) ;
#129297=DIRECTION('ref_axis',(0.707106781186548,0.707106781186548,1.5356898865553E-31)) ;
#129298=DIRECTION('center_axis',(0.577350269189633,-0.577350269189633,-0.577350269189612)) ;
#129299=DIRECTION('ref_axis',(0.707106781186548,0.707106781186548,1.34560831514457E-17)) ;
#129300=DIRECTION('center_axis',(-0.577350269189344,0.577350269189586,-0.577350269189947)) ;
#129301=DIRECTION('ref_axis',(1.30446081606812E-15,0.707106781186769,0.707106781186326)) ;
#129302=DIRECTION('center_axis',(-0.707106781186548,0.707106781186548,7.66646708341692E-15)) ;
#129303=DIRECTION('ref_axis',(-0.707106781186548,-0.707106781186548,-2.68297081166629E-31)) ;
#129304=DIRECTION('center_axis',(-0.707106781186549,0.707106781186546,0.)) ;
#129305=DIRECTION('ref_axis',(-0.707106781186546,-0.707106781186549,0.)) ;
#129306=DIRECTION('center_axis',(-0.707106781186548,0.707106781186548,-1.22663473334671E-14)) ;
#129307=DIRECTION('ref_axis',(-0.707106781186548,-0.707106781186548,2.94725045705944E-31)) ;
#129308=DIRECTION('center_axis',(-0.669589480006976,0.669589480006974,-0.321402950403349)) ;
#129309=DIRECTION('ref_axis',(-0.707106781186547,-0.707106781186548,5.45170614306381E-16)) ;
#129310=DIRECTION('center_axis',(0.669589480006982,-0.669589480006966,0.321402950403353)) ;
#129311=DIRECTION('ref_axis',(0.707106781186539,0.707106781186556,5.77426876420606E-17)) ;
#129312=DIRECTION('center_axis',(0.,1.,0.)) ;
#129313=DIRECTION('ref_axis',(1.,0.,0.)) ;
#129314=DIRECTION('center_axis',(0.,1.,0.)) ;
#129315=DIRECTION('ref_axis',(0.,0.,-1.)) ;
#129316=DIRECTION('center_axis',(0.,-1.,0.)) ;
#129317=DIRECTION('ref_axis',(0.,0.,-1.)) ;
#129318=DIRECTION('center_axis',(0.,1.,0.)) ;
#129319=DIRECTION('ref_axis',(0.,0.,1.)) ;
#129320=DIRECTION('center_axis',(-0.879462917689188,-0.219865729422294,
-0.42214220049081)) ;
#129321=DIRECTION('ref_axis',(-0.432731067584771,1.71515946658E-16,0.901523057468274)) ;
#129322=DIRECTION('center_axis',(0.879462917689201,0.219865729422298,0.42214220049078)) ;
#129323=DIRECTION('ref_axis',(0.432731067584741,5.42470486237819E-16,-0.901523057468288)) ;
#129324=DIRECTION('center_axis',(0.,1.,0.)) ;
#129325=DIRECTION('ref_axis',(1.,0.,0.)) ;
#129326=DIRECTION('center_axis',(0.970142500145323,0.242535625036368,0.)) ;
#129327=DIRECTION('ref_axis',(0.242535625036368,-0.970142500145323,0.)) ;
#129328=DIRECTION('center_axis',(-0.970142500145333,-0.24253562503633,0.)) ;
#129329=DIRECTION('ref_axis',(0.24253562503633,-0.970142500145333,0.)) ;
#129330=DIRECTION('center_axis',(0.970142500145332,0.242535625036331,-2.10366121255617E-15)) ;
#129331=DIRECTION('ref_axis',(-0.242535625036331,0.970142500145332,-4.47980524894761E-30)) ;
#129332=DIRECTION('center_axis',(0.942809041582064,0.235702260395514,0.235702260395514)) ;
#129333=DIRECTION('ref_axis',(-0.242535625036331,0.970142500145332,4.49011373492972E-16)) ;
#129334=DIRECTION('center_axis',(0.,-1.,0.)) ;
#129335=DIRECTION('ref_axis',(0.,0.,-1.)) ;
#129336=DIRECTION('center_axis',(-1.,0.,-8.67361737988409E-15)) ;
#129337=DIRECTION('ref_axis',(-8.67361737988409E-15,0.,1.)) ;
#129338=DIRECTION('center_axis',(0.,0.,-1.)) ;
#129339=DIRECTION('ref_axis',(-1.,0.,0.)) ;
#129340=DIRECTION('center_axis',(0.,0.,-1.)) ;
#129341=DIRECTION('ref_axis',(-1.,0.,0.)) ;
#129342=DIRECTION('center_axis',(0.,0.,-1.)) ;
#129343=DIRECTION('ref_axis',(-1.,0.,0.)) ;
#129344=DIRECTION('center_axis',(1.,0.,0.)) ;
#129345=DIRECTION('ref_axis',(0.,0.,-1.)) ;
#129346=DIRECTION('center_axis',(-1.,0.,0.)) ;
#129347=DIRECTION('ref_axis',(0.,0.,1.)) ;
#129348=DIRECTION('center_axis',(0.,-1.,0.)) ;
#129349=DIRECTION('ref_axis',(0.,0.,-1.)) ;
#129350=DIRECTION('center_axis',(-1.,0.,0.)) ;
#129351=DIRECTION('ref_axis',(0.,0.,1.)) ;
#129352=DIRECTION('center_axis',(0.,-1.,0.)) ;
#129353=DIRECTION('ref_axis',(0.,0.,-1.)) ;
#129354=DIRECTION('center_axis',(0.,0.,-1.)) ;
#129355=DIRECTION('ref_axis',(-1.,0.,0.)) ;
#129356=DIRECTION('center_axis',(-1.,0.,0.)) ;
#129357=DIRECTION('ref_axis',(0.,0.,1.)) ;
#129358=DIRECTION('center_axis',(-1.,1.73472347597681E-14,0.)) ;
#129359=DIRECTION('ref_axis',(-1.73472347597681E-14,-1.,0.)) ;
#129360=DIRECTION('center_axis',(0.,0.,1.)) ;
#129361=DIRECTION('ref_axis',(1.,0.,0.)) ;
#129362=DIRECTION('center_axis',(-3.46944695195364E-14,0.,-1.)) ;
#129363=DIRECTION('ref_axis',(-1.,0.,3.46944695195364E-14)) ;
#129364=DIRECTION('center_axis',(0.,-1.,0.)) ;
#129365=DIRECTION('ref_axis',(0.,0.,-1.)) ;
#129366=DIRECTION('center_axis',(0.,-1.,0.)) ;
#129367=DIRECTION('ref_axis',(0.,0.,-1.)) ;
#129368=DIRECTION('center_axis',(0.,-1.,0.)) ;
#129369=DIRECTION('ref_axis',(0.,0.,-1.)) ;
#129370=DIRECTION('center_axis',(0.,0.,1.)) ;
#129371=DIRECTION('ref_axis',(1.,0.,0.)) ;
#129372=DIRECTION('center_axis',(0.,0.,-1.)) ;
#129373=DIRECTION('ref_axis',(-1.,0.,0.)) ;
#129374=DIRECTION('center_axis',(0.,0.,1.)) ;
#129375=DIRECTION('ref_axis',(1.,0.,0.)) ;
#129376=DIRECTION('center_axis',(0.,-1.,0.)) ;
#129377=DIRECTION('ref_axis',(0.,0.,-1.)) ;
#129378=DIRECTION('center_axis',(0.,-1.,0.)) ;
#129379=DIRECTION('ref_axis',(0.,0.,-1.)) ;
#129380=DIRECTION('center_axis',(0.,1.,0.)) ;
#129381=DIRECTION('ref_axis',(1.,0.,0.)) ;
#129382=DIRECTION('center_axis',(-1.,0.,0.)) ;
#129383=DIRECTION('ref_axis',(0.,0.,-1.)) ;
#129384=DIRECTION('center_axis',(0.,1.,0.)) ;
#129385=DIRECTION('ref_axis',(1.,0.,0.)) ;
#129386=DIRECTION('center_axis',(-1.,0.,0.)) ;
#129387=DIRECTION('ref_axis',(0.,0.,-1.)) ;
#129388=DIRECTION('center_axis',(0.,-1.,0.)) ;
#129389=DIRECTION('ref_axis',(0.,0.,-1.)) ;
#129390=DIRECTION('center_axis',(0.,-1.,0.)) ;
#129391=DIRECTION('ref_axis',(0.,0.,-1.)) ;
#129392=DIRECTION('center_axis',(-1.,0.,0.)) ;
#129393=DIRECTION('ref_axis',(0.,0.,1.)) ;
#129394=DIRECTION('center_axis',(-1.,0.,0.)) ;
#129395=DIRECTION('ref_axis',(0.,0.,1.)) ;
#129396=DIRECTION('center_axis',(1.,0.,0.)) ;
#129397=DIRECTION('ref_axis',(0.,0.,-1.)) ;
#129398=DIRECTION('center_axis',(-1.,0.,0.)) ;
#129399=DIRECTION('ref_axis',(0.,0.,1.)) ;
#129400=DIRECTION('center_axis',(0.,-1.,0.)) ;
#129401=DIRECTION('ref_axis',(0.,0.,-1.)) ;
#129402=DIRECTION('center_axis',(0.,-1.,0.)) ;
#129403=DIRECTION('ref_axis',(0.,0.,-1.)) ;
#129404=DIRECTION('center_axis',(0.,1.,0.)) ;
#129405=DIRECTION('ref_axis',(1.,0.,0.)) ;
#129406=DIRECTION('center_axis',(0.,0.,-1.)) ;
#129407=DIRECTION('ref_axis',(1.,0.,0.)) ;
#129408=DIRECTION('center_axis',(0.,1.,0.)) ;
#129409=DIRECTION('ref_axis',(1.,0.,0.)) ;
#129410=DIRECTION('center_axis',(0.,0.,1.)) ;
#129411=DIRECTION('ref_axis',(-1.,0.,0.)) ;
#129412=DIRECTION('center_axis',(0.,0.,-1.)) ;
#129413=DIRECTION('ref_axis',(-1.,0.,0.)) ;
#129414=DIRECTION('center_axis',(1.,1.31418445149758E-16,-2.16840434497101E-16)) ;
#129415=DIRECTION('ref_axis',(-2.16840434497101E-16,-2.8496832747207E-32,
-1.)) ;
#129416=DIRECTION('center_axis',(1.,0.,0.)) ;
#129417=DIRECTION('ref_axis',(0.,0.,-1.)) ;
#129418=DIRECTION('center_axis',(-1.,0.,0.)) ;
#129419=DIRECTION('ref_axis',(0.,0.,1.)) ;
#129420=DIRECTION('center_axis',(-1.31418445149758E-16,1.,0.)) ;
#129421=DIRECTION('ref_axis',(-1.,0.,0.)) ;
#129422=DIRECTION('center_axis',(0.,0.,1.)) ;
#129423=DIRECTION('ref_axis',(-1.,0.,0.)) ;
#129424=DIRECTION('center_axis',(-1.31418445149758E-16,1.,0.)) ;
#129425=DIRECTION('ref_axis',(-1.,-1.31418445149758E-16,0.)) ;
#129426=DIRECTION('center_axis',(-1.31418445149758E-16,1.,0.)) ;
#129427=DIRECTION('ref_axis',(-1.,0.,0.)) ;
#129428=DIRECTION('center_axis',(-1.31418445149758E-16,1.,0.)) ;
#129429=DIRECTION('ref_axis',(-1.,-1.31418445149758E-16,0.)) ;
#129430=DIRECTION('center_axis',(0.,0.,1.)) ;
#129431=DIRECTION('ref_axis',(-1.,0.,0.)) ;
#129432=DIRECTION('center_axis',(-4.33680868994202E-16,-5.69936654944139E-32,
-1.)) ;
#129433=DIRECTION('ref_axis',(-1.,2.47170623787823E-47,4.33680868994202E-16)) ;
#129434=DIRECTION('center_axis',(0.,0.,1.)) ;
#129435=DIRECTION('ref_axis',(1.,0.,0.)) ;
#129436=DIRECTION('center_axis',(-1.31418445149758E-16,-1.,0.)) ;
#129437=DIRECTION('ref_axis',(1.,-1.31418445149758E-16,0.)) ;
#129438=DIRECTION('center_axis',(0.,1.,0.)) ;
#129439=DIRECTION('ref_axis',(0.,0.,1.)) ;
#129440=DIRECTION('center_axis',(-1.,0.,2.16840434497101E-16)) ;
#129441=DIRECTION('ref_axis',(2.16840434497101E-16,0.,1.)) ;
#129442=DIRECTION('center_axis',(-1.,0.,0.)) ;
#129443=DIRECTION('ref_axis',(0.,0.,1.)) ;
#129444=DIRECTION('center_axis',(1.,0.,0.)) ;
#129445=DIRECTION('ref_axis',(0.,0.,-1.)) ;
#129446=DIRECTION('center_axis',(-1.31418445149758E-16,-1.,0.)) ;
#129447=DIRECTION('ref_axis',(1.,-1.31418445149758E-16,0.)) ;
#129448=DIRECTION('center_axis',(0.,1.,0.)) ;
#129449=DIRECTION('ref_axis',(0.,0.,1.)) ;
#129450=DIRECTION('center_axis',(2.16840434497101E-16,2.8496832747207E-32,
1.)) ;
#129451=DIRECTION('ref_axis',(1.,-6.17926559469557E-48,-2.16840434497101E-16)) ;
#129452=DIRECTION('center_axis',(0.,0.,1.)) ;
#129453=DIRECTION('ref_axis',(1.,0.,0.)) ;
#129454=DIRECTION('center_axis',(-1.,-1.31418445149758E-16,-2.16840434497101E-16)) ;
#129455=DIRECTION('ref_axis',(-2.16840434497101E-16,-2.8496832747207E-32,
1.)) ;
#129456=DIRECTION('center_axis',(-1.,0.,0.)) ;
#129457=DIRECTION('ref_axis',(0.,0.,1.)) ;
#129458=DIRECTION('center_axis',(1.,0.,0.)) ;
#129459=DIRECTION('ref_axis',(0.,0.,-1.)) ;
#129460=DIRECTION('center_axis',(-1.31418445149758E-16,1.,0.)) ;
#129461=DIRECTION('ref_axis',(-1.,0.,0.)) ;
#129462=DIRECTION('center_axis',(-1.31418445149758E-16,1.,0.)) ;
#129463=DIRECTION('ref_axis',(-1.,-1.31418445149758E-16,0.)) ;
#129464=DIRECTION('center_axis',(0.,1.,0.)) ;
#129465=DIRECTION('ref_axis',(1.,0.,0.)) ;
#129466=DIRECTION('center_axis',(0.,0.,-1.)) ;
#129467=DIRECTION('ref_axis',(1.,0.,0.)) ;
#129468=DIRECTION('center_axis',(0.,1.,0.)) ;
#129469=DIRECTION('ref_axis',(1.,0.,0.)) ;
#129470=DIRECTION('center_axis',(0.,0.,-1.)) ;
#129471=DIRECTION('ref_axis',(1.,0.,0.)) ;
#129472=DIRECTION('center_axis',(-1.31418445149758E-16,1.,0.)) ;
#129473=DIRECTION('ref_axis',(-1.,0.,0.)) ;
#129474=DIRECTION('center_axis',(-1.31418445149758E-16,1.,0.)) ;
#129475=DIRECTION('ref_axis',(-1.,-1.31418445149758E-16,0.)) ;
#129476=DIRECTION('center_axis',(-1.31418445149758E-16,-1.,0.)) ;
#129477=DIRECTION('ref_axis',(1.,-1.31418445149758E-16,0.)) ;
#129478=DIRECTION('center_axis',(0.,1.,0.)) ;
#129479=DIRECTION('ref_axis',(0.,0.,1.)) ;
#129480=DIRECTION('center_axis',(4.33680868994202E-16,0.,1.)) ;
#129481=DIRECTION('ref_axis',(1.,0.,-4.33680868994202E-16)) ;
#129482=DIRECTION('center_axis',(0.,0.,-1.)) ;
#129483=DIRECTION('ref_axis',(-1.,0.,0.)) ;
#129484=DIRECTION('center_axis',(-2.16840434497101E-16,0.,-1.)) ;
#129485=DIRECTION('ref_axis',(-1.,0.,2.16840434497101E-16)) ;
#129486=DIRECTION('center_axis',(0.,0.,-1.)) ;
#129487=DIRECTION('ref_axis',(-1.,0.,0.)) ;
#129488=DIRECTION('center_axis',(-1.31418445149758E-16,-1.,0.)) ;
#129489=DIRECTION('ref_axis',(1.,-1.31418445149758E-16,0.)) ;
#129490=DIRECTION('center_axis',(0.,1.,0.)) ;
#129491=DIRECTION('ref_axis',(0.,0.,1.)) ;
#129492=DIRECTION('center_axis',(0.,1.,0.)) ;
#129493=DIRECTION('ref_axis',(1.,0.,0.)) ;
#129494=DIRECTION('center_axis',(-1.,0.,0.)) ;
#129495=DIRECTION('ref_axis',(0.,0.,-1.)) ;
#129496=DIRECTION('center_axis',(0.,1.,0.)) ;
#129497=DIRECTION('ref_axis',(1.,0.,0.)) ;
#129498=DIRECTION('center_axis',(1.,0.,0.)) ;
#129499=DIRECTION('ref_axis',(0.,0.,1.)) ;
#129500=DIRECTION('center_axis',(1.,0.,2.16840434497101E-16)) ;
#129501=DIRECTION('ref_axis',(2.16840434497101E-16,0.,-1.)) ;
#129502=DIRECTION('center_axis',(0.,1.,0.)) ;
#129503=DIRECTION('ref_axis',(0.,0.,1.)) ;
#129504=DIRECTION('center_axis',(0.,1.,0.)) ;
#129505=DIRECTION('ref_axis',(0.,0.,1.)) ;
#129506=DIRECTION('center_axis',(0.,0.,-1.)) ;
#129507=DIRECTION('ref_axis',(-1.,0.,0.)) ;
#129508=DIRECTION('center_axis',(0.,0.,1.)) ;
#129509=DIRECTION('ref_axis',(1.,0.,0.)) ;
#129510=DIRECTION('center_axis',(0.,0.,-1.)) ;
#129511=DIRECTION('ref_axis',(-1.,0.,0.)) ;
#129512=DIRECTION('center_axis',(0.,1.,0.)) ;
#129513=DIRECTION('ref_axis',(0.,0.,1.)) ;
#129514=DIRECTION('center_axis',(0.,1.,0.)) ;
#129515=DIRECTION('ref_axis',(0.,0.,1.)) ;
#129516=DIRECTION('center_axis',(0.,1.,0.)) ;
#129517=DIRECTION('ref_axis',(1.,0.,0.)) ;
#129518=DIRECTION('center_axis',(-1.,0.,0.)) ;
#129519=DIRECTION('ref_axis',(0.,0.,-1.)) ;
#129520=DIRECTION('center_axis',(0.,1.,0.)) ;
#129521=DIRECTION('ref_axis',(1.,0.,0.)) ;
#129522=DIRECTION('center_axis',(-1.,0.,0.)) ;
#129523=DIRECTION('ref_axis',(0.,0.,-1.)) ;
#129524=DIRECTION('center_axis',(0.,1.,0.)) ;
#129525=DIRECTION('ref_axis',(0.,0.,1.)) ;
#129526=DIRECTION('center_axis',(0.,1.,0.)) ;
#129527=DIRECTION('ref_axis',(0.,0.,1.)) ;
#129528=DIRECTION('center_axis',(-1.,0.,0.)) ;
#129529=DIRECTION('ref_axis',(0.,0.,1.)) ;
#129530=DIRECTION('center_axis',(-1.,0.,0.)) ;
#129531=DIRECTION('ref_axis',(0.,0.,1.)) ;
#129532=DIRECTION('center_axis',(1.,0.,0.)) ;
#129533=DIRECTION('ref_axis',(0.,0.,-1.)) ;
#129534=DIRECTION('center_axis',(-1.,0.,0.)) ;
#129535=DIRECTION('ref_axis',(0.,0.,1.)) ;
#129536=DIRECTION('center_axis',(0.,1.,0.)) ;
#129537=DIRECTION('ref_axis',(0.,0.,1.)) ;
#129538=DIRECTION('center_axis',(0.,1.,0.)) ;
#129539=DIRECTION('ref_axis',(0.,0.,1.)) ;
#129540=DIRECTION('center_axis',(0.,1.,0.)) ;
#129541=DIRECTION('ref_axis',(1.,0.,0.)) ;
#129542=DIRECTION('center_axis',(0.,0.,1.)) ;
#129543=DIRECTION('ref_axis',(-1.,0.,0.)) ;
#129544=DIRECTION('center_axis',(0.,1.,0.)) ;
#129545=DIRECTION('ref_axis',(1.,0.,0.)) ;
#129546=DIRECTION('center_axis',(0.,0.,-1.)) ;
#129547=DIRECTION('ref_axis',(1.,0.,0.)) ;
#129548=DIRECTION('center_axis',(0.,0.,1.)) ;
#129549=DIRECTION('ref_axis',(1.,0.,0.)) ;
#129550=DIRECTION('center_axis',(0.,0.,1.)) ;
#129551=DIRECTION('ref_axis',(1.,0.,0.)) ;
#129552=DIRECTION('center_axis',(0.,0.,-1.)) ;
#129553=DIRECTION('ref_axis',(-1.,0.,0.)) ;
#129554=DIRECTION('center_axis',(0.,0.,1.)) ;
#129555=DIRECTION('ref_axis',(1.,0.,0.)) ;
#129556=DIRECTION('center_axis',(1.,0.,0.)) ;
#129557=DIRECTION('ref_axis',(0.,0.,-1.)) ;
#129558=DIRECTION('center_axis',(1.,0.,0.)) ;
#129559=DIRECTION('ref_axis',(0.,0.,-1.)) ;
#129560=DIRECTION('center_axis',(1.,0.,0.)) ;
#129561=DIRECTION('ref_axis',(0.,0.,-1.)) ;
#129562=DIRECTION('center_axis',(1.,0.,8.67361737988409E-15)) ;
#129563=DIRECTION('ref_axis',(8.67361737988409E-15,0.,-1.)) ;
#129564=DIRECTION('center_axis',(1.,0.,0.)) ;
#129565=DIRECTION('ref_axis',(0.,0.,-1.)) ;
#129566=DIRECTION('center_axis',(1.,0.,1.73472347597682E-14)) ;
#129567=DIRECTION('ref_axis',(1.73472347597682E-14,0.,-1.)) ;
#129568=DIRECTION('center_axis',(-1.,0.,0.)) ;
#129569=DIRECTION('ref_axis',(0.,0.,1.)) ;
#129570=DIRECTION('center_axis',(1.,0.,0.)) ;
#129571=DIRECTION('ref_axis',(0.,0.,-1.)) ;
#129572=DIRECTION('center_axis',(1.,0.,0.)) ;
#129573=DIRECTION('ref_axis',(0.,0.,-1.)) ;
#129574=DIRECTION('center_axis',(-3.46944695195364E-14,0.,-1.)) ;
#129575=DIRECTION('ref_axis',(-1.,0.,3.46944695195364E-14)) ;
#129576=DIRECTION('center_axis',(1.,0.,0.)) ;
#129577=DIRECTION('ref_axis',(0.,0.,-1.)) ;
#129578=DIRECTION('center_axis',(0.,0.,1.)) ;
#129579=DIRECTION('ref_axis',(1.,0.,0.)) ;
#129580=DIRECTION('center_axis',(0.,0.,-1.)) ;
#129581=DIRECTION('ref_axis',(-1.,0.,0.)) ;
#129582=DIRECTION('center_axis',(-0.422618261740697,5.55398348498559E-17,
0.906307787036651)) ;
#129583=DIRECTION('ref_axis',(0.906307787036651,6.51773046476477E-31,0.422618261740697)) ;
#129584=DIRECTION('center_axis',(0.422618261740697,-5.55398348498559E-17,
-0.906307787036651)) ;
#129585=DIRECTION('ref_axis',(-0.906307787036651,-6.46086972436398E-31,
-0.422618261740697)) ;
#129586=DIRECTION('center_axis',(-0.422618261740697,5.55398348498559E-17,
0.906307787036651)) ;
#129587=DIRECTION('ref_axis',(0.906307787036651,6.46086972436398E-31,0.422618261740697)) ;
#129588=DIRECTION('center_axis',(0.422618261740697,-5.55398348498559E-17,
-0.906307787036651)) ;
#129589=DIRECTION('ref_axis',(-0.906307787036651,-6.46086972436398E-31,
-0.422618261740697)) ;
#129590=DIRECTION('center_axis',(0.,1.,0.)) ;
#129591=DIRECTION('ref_axis',(1.,0.,0.)) ;
#129592=DIRECTION('center_axis',(3.4216004848576E-14,0.514231796959095,
-0.857651245551606)) ;
#129593=DIRECTION('ref_axis',(3.46944695195362E-14,-0.857651245551606,-0.514231796959095)) ;
#129594=DIRECTION('center_axis',(0.,-3.46944695195362E-14,1.)) ;
#129595=DIRECTION('ref_axis',(0.,1.,3.46944695195362E-14)) ;
#129596=DIRECTION('center_axis',(-1.,0.,0.)) ;
#129597=DIRECTION('ref_axis',(0.,-4.33680868994204E-15,-1.)) ;
#129598=DIRECTION('center_axis',(0.,0.,1.)) ;
#129599=DIRECTION('ref_axis',(1.,0.,0.)) ;
#129600=DIRECTION('center_axis',(0.,0.,1.)) ;
#129601=DIRECTION('ref_axis',(1.,0.,0.)) ;
#129602=DIRECTION('center_axis',(-1.,0.,0.)) ;
#129603=DIRECTION('ref_axis',(0.,0.,1.)) ;
#129604=DIRECTION('center_axis',(-1.,0.,0.)) ;
#129605=DIRECTION('ref_axis',(0.,-4.33680868994204E-15,-1.)) ;
#129606=DIRECTION('center_axis',(1.,0.,0.)) ;
#129607=DIRECTION('ref_axis',(0.,0.,-1.)) ;
#129608=DIRECTION('center_axis',(0.,-0.514231796959124,-0.857651245551588)) ;
#129609=DIRECTION('ref_axis',(0.,0.857651245551588,-0.514231796959124)) ;
#129610=DIRECTION('center_axis',(0.,1.,8.97270763436279E-17)) ;
#129611=DIRECTION('ref_axis',(0.,-8.97270763436279E-17,1.)) ;
#129612=DIRECTION('center_axis',(0.,-1.,-8.97270763436279E-17)) ;
#129613=DIRECTION('ref_axis',(0.,-8.97270763436279E-17,1.)) ;
#129614=DIRECTION('center_axis',(0.,-1.,0.)) ;
#129615=DIRECTION('ref_axis',(0.,0.,-1.)) ;
#129616=DIRECTION('center_axis',(0.,1.,0.)) ;
#129617=DIRECTION('ref_axis',(1.,0.,0.)) ;
#129618=DIRECTION('center_axis',(-1.,0.,0.)) ;
#129619=DIRECTION('ref_axis',(0.,0.,-1.)) ;
#129620=DIRECTION('center_axis',(1.,0.,0.)) ;
#129621=DIRECTION('ref_axis',(0.,0.,-1.)) ;
#129622=DIRECTION('center_axis',(0.,-0.514231796959093,0.857651245551607)) ;
#129623=DIRECTION('ref_axis',(0.,0.857651245551607,0.514231796959093)) ;
#129624=DIRECTION('center_axis',(0.,0.,-1.)) ;
#129625=DIRECTION('ref_axis',(1.,0.,0.)) ;
#129626=DIRECTION('center_axis',(0.,1.,0.)) ;
#129627=DIRECTION('ref_axis',(1.,0.,0.)) ;
#129628=DIRECTION('center_axis',(-3.46944695195364E-14,0.,-1.)) ;
#129629=DIRECTION('ref_axis',(1.,0.,-3.46944695195364E-14)) ;
#129630=DIRECTION('center_axis',(-1.,0.,0.)) ;
#129631=DIRECTION('ref_axis',(0.,4.33680868994204E-15,-1.)) ;
#129632=DIRECTION('center_axis',(0.,0.,-1.)) ;
#129633=DIRECTION('ref_axis',(-1.,0.,0.)) ;
#129634=DIRECTION('center_axis',(0.,0.,1.)) ;
#129635=DIRECTION('ref_axis',(-1.,0.,0.)) ;
#129636=DIRECTION('center_axis',(0.,0.,-1.)) ;
#129637=DIRECTION('ref_axis',(-1.,0.,0.)) ;
#129638=DIRECTION('center_axis',(-1.,0.,7.01133629567814E-33)) ;
#129639=DIRECTION('ref_axis',(7.01133629567814E-33,0.,1.)) ;
#129640=DIRECTION('center_axis',(-1.,0.,0.)) ;
#129641=DIRECTION('ref_axis',(0.,0.,1.)) ;
#129642=DIRECTION('center_axis',(0.,0.,-1.)) ;
#129643=DIRECTION('ref_axis',(-1.,0.,0.)) ;
#129644=DIRECTION('center_axis',(-7.01133629567814E-33,8.97270763436279E-17,
-1.)) ;
#129645=DIRECTION('ref_axis',(6.29106707073161E-49,1.,8.97270763436279E-17)) ;
#129646=DIRECTION('center_axis',(1.,0.,0.)) ;
#129647=DIRECTION('ref_axis',(0.,0.,-1.)) ;
#129648=DIRECTION('center_axis',(-2.2301249256967E-15,0.514231796959095,
0.857651245551606)) ;
#129649=DIRECTION('ref_axis',(-4.79361507851841E-30,-0.857651245551606,
0.514231796959095)) ;
#129650=DIRECTION('center_axis',(-1.,0.,0.)) ;
#129651=DIRECTION('ref_axis',(0.,0.,1.)) ;
#129652=DIRECTION('center_axis',(-1.,0.,0.)) ;
#129653=DIRECTION('ref_axis',(0.,-4.33680868994204E-15,-1.)) ;
#129654=DIRECTION('center_axis',(0.,0.,1.)) ;
#129655=DIRECTION('ref_axis',(1.,0.,0.)) ;
#129656=DIRECTION('center_axis',(0.,0.,-1.)) ;
#129657=DIRECTION('ref_axis',(-1.,0.,0.)) ;
#129658=DIRECTION('center_axis',(0.,-1.,8.97270763436279E-17)) ;
#129659=DIRECTION('ref_axis',(0.,-8.97270763436279E-17,-1.)) ;
#129660=DIRECTION('center_axis',(0.,-1.,8.97270763436279E-17)) ;
#129661=DIRECTION('ref_axis',(0.,-8.97270763436279E-17,-1.)) ;
#129662=DIRECTION('center_axis',(0.,-1.,0.)) ;
#129663=DIRECTION('ref_axis',(0.,0.,-1.)) ;
#129664=DIRECTION('center_axis',(-7.01133629567814E-33,8.97270763436279E-17,
-1.)) ;
#129665=DIRECTION('ref_axis',(0.,1.,0.)) ;
#129666=DIRECTION('center_axis',(0.,-1.,0.)) ;
#129667=DIRECTION('ref_axis',(0.,0.,1.)) ;
#129668=DIRECTION('center_axis',(1.,0.,0.)) ;
#129669=DIRECTION('ref_axis',(0.,0.,-1.)) ;
#129670=DIRECTION('center_axis',(0.,0.,1.)) ;
#129671=DIRECTION('ref_axis',(-1.,0.,0.)) ;
#129672=DIRECTION('center_axis',(0.,1.,0.)) ;
#129673=DIRECTION('ref_axis',(1.,0.,0.)) ;
#129674=DIRECTION('center_axis',(-1.,0.,0.)) ;
#129675=DIRECTION('ref_axis',(0.,0.,-1.)) ;
#129676=DIRECTION('center_axis',(1.,7.81406971160724E-17,0.)) ;
#129677=DIRECTION('ref_axis',(-7.81406971160724E-17,1.,0.)) ;
#129678=DIRECTION('center_axis',(1.,0.,0.)) ;
#129679=DIRECTION('ref_axis',(0.,0.,-1.)) ;
#129680=DIRECTION('center_axis',(1.,0.,0.)) ;
#129681=DIRECTION('ref_axis',(0.,0.,-1.)) ;
#129682=DIRECTION('center_axis',(0.,1.,8.97270763436279E-17)) ;
#129683=DIRECTION('ref_axis',(0.,-8.97270763436279E-17,1.)) ;
#129684=DIRECTION('center_axis',(0.,-1.,0.)) ;
#129685=DIRECTION('ref_axis',(0.,0.,-1.)) ;
#129686=DIRECTION('center_axis',(0.,0.,-1.)) ;
#129687=DIRECTION('ref_axis',(-1.,0.,0.)) ;
#129688=DIRECTION('center_axis',(-7.01133629567814E-33,8.97270763436279E-17,
1.)) ;
#129689=DIRECTION('ref_axis',(-6.29106707073161E-49,-1.,8.97270763436279E-17)) ;
#129690=DIRECTION('center_axis',(-1.,0.,-7.01133629567814E-33)) ;
#129691=DIRECTION('ref_axis',(-7.01133629567814E-33,0.,1.)) ;
#129692=DIRECTION('center_axis',(-1.,0.,0.)) ;
#129693=DIRECTION('ref_axis',(0.,0.,1.)) ;
#129694=DIRECTION('center_axis',(1.,0.,0.)) ;
#129695=DIRECTION('ref_axis',(0.,1.,0.)) ;
#129696=DIRECTION('center_axis',(2.16840434497101E-15,1.,0.)) ;
#129697=DIRECTION('ref_axis',(-1.,2.16840434497101E-15,0.)) ;
#129698=DIRECTION('center_axis',(0.,1.,0.)) ;
#129699=DIRECTION('ref_axis',(1.,0.,0.)) ;
#129700=DIRECTION('center_axis',(0.,0.,-1.)) ;
#129701=DIRECTION('ref_axis',(1.,0.,0.)) ;
#129702=DIRECTION('center_axis',(-1.,0.,0.)) ;
#129703=DIRECTION('ref_axis',(0.,0.,-1.)) ;
#129704=DIRECTION('center_axis',(-7.01133629567814E-33,8.97270763436279E-17,
1.)) ;
#129705=DIRECTION('ref_axis',(0.,-1.,0.)) ;
#129706=DIRECTION('center_axis',(0.,-1.,0.)) ;
#129707=DIRECTION('ref_axis',(0.,0.,1.)) ;
#129708=DIRECTION('center_axis',(7.81406971160724E-17,-1.,-8.97270763436279E-17)) ;
#129709=DIRECTION('ref_axis',(-7.01133629567814E-33,8.97270763436279E-17,
-1.)) ;
#129710=DIRECTION('center_axis',(0.,1.,0.)) ;
#129711=DIRECTION('ref_axis',(0.,0.,1.)) ;
#129712=DIRECTION('center_axis',(-1.,-7.81406971160724E-17,0.)) ;
#129713=DIRECTION('ref_axis',(7.81406971160724E-17,-1.,0.)) ;
#129714=DIRECTION('center_axis',(-1.,-7.81406971160724E-17,0.)) ;
#129715=DIRECTION('ref_axis',(-7.81406971160724E-17,1.,0.)) ;
#129716=DIRECTION('center_axis',(0.,0.,1.)) ;
#129717=DIRECTION('ref_axis',(1.,0.,0.)) ;
#129718=DIRECTION('center_axis',(0.,0.,-1.)) ;
#129719=DIRECTION('ref_axis',(-1.,0.,0.)) ;
#129720=DIRECTION('center_axis',(0.,-1.,8.97270763436279E-17)) ;
#129721=DIRECTION('ref_axis',(0.,-8.97270763436279E-17,-1.)) ;
#129722=DIRECTION('center_axis',(0.,-1.,0.)) ;
#129723=DIRECTION('ref_axis',(0.,0.,-1.)) ;
#129724=DIRECTION('center_axis',(1.,7.81406971160724E-17,0.)) ;
#129725=DIRECTION('ref_axis',(0.,1.,0.)) ;
#129726=DIRECTION('center_axis',(0.,0.,1.)) ;
#129727=DIRECTION('ref_axis',(-1.,0.,0.)) ;
#129728=DIRECTION('center_axis',(0.,1.,0.)) ;
#129729=DIRECTION('ref_axis',(1.,0.,0.)) ;
#129730=DIRECTION('center_axis',(-1.,0.,0.)) ;
#129731=DIRECTION('ref_axis',(0.,0.,-1.)) ;
#129732=DIRECTION('center_axis',(0.,0.,-1.)) ;
#129733=DIRECTION('ref_axis',(-1.,0.,0.)) ;
#129734=DIRECTION('center_axis',(0.,0.,1.)) ;
#129735=DIRECTION('ref_axis',(1.,0.,0.)) ;
#129736=DIRECTION('center_axis',(-1.,-7.81406971160724E-17,0.)) ;
#129737=DIRECTION('ref_axis',(7.81406971160724E-17,-1.,0.)) ;
#129738=DIRECTION('center_axis',(-1.,-7.81406971160724E-17,0.)) ;
#129739=DIRECTION('ref_axis',(-7.81406971160724E-17,1.,0.)) ;
#129740=DIRECTION('center_axis',(1.,7.81406971160724E-17,0.)) ;
#129741=DIRECTION('ref_axis',(-7.81406971160724E-17,1.,0.)) ;
#129742=DIRECTION('center_axis',(1.,0.,0.)) ;
#129743=DIRECTION('ref_axis',(0.,0.,-1.)) ;
#129744=DIRECTION('center_axis',(1.,0.,0.)) ;
#129745=DIRECTION('ref_axis',(0.,0.,-1.)) ;
#129746=DIRECTION('center_axis',(3.78638272950961E-32,-4.8455963016112E-16,
-1.)) ;
#129747=DIRECTION('ref_axis',(1.83472821505963E-47,1.,-4.8455963016112E-16)) ;
#129748=DIRECTION('center_axis',(3.78638272950961E-32,-4.8455963016112E-16,
-1.)) ;
#129749=DIRECTION('ref_axis',(1.83472821505963E-47,1.,-4.8455963016112E-16)) ;
#129750=DIRECTION('center_axis',(0.,0.,-1.)) ;
#129751=DIRECTION('ref_axis',(-1.,0.,0.)) ;
#129752=DIRECTION('center_axis',(1.,7.81406971160724E-17,0.)) ;
#129753=DIRECTION('ref_axis',(0.,1.,0.)) ;
#129754=DIRECTION('center_axis',(0.,-1.,0.)) ;
#129755=DIRECTION('ref_axis',(0.,0.,1.)) ;
#129756=DIRECTION('center_axis',(0.,1.,0.)) ;
#129757=DIRECTION('ref_axis',(1.,0.,0.)) ;
#129758=DIRECTION('center_axis',(0.,1.,0.)) ;
#129759=DIRECTION('ref_axis',(0.,0.,-1.)) ;
#129760=DIRECTION('center_axis',(-7.81406971160724E-17,1.,-8.97270763436279E-17)) ;
#129761=DIRECTION('ref_axis',(-7.01133629567814E-33,8.97270763436279E-17,
1.)) ;
#129762=DIRECTION('center_axis',(0.,-1.,0.)) ;
#129763=DIRECTION('ref_axis',(0.,0.,-1.)) ;
#129764=DIRECTION('center_axis',(0.,1.,0.)) ;
#129765=DIRECTION('ref_axis',(0.,0.,1.)) ;
#129766=DIRECTION('center_axis',(0.,-1.,0.)) ;
#129767=DIRECTION('ref_axis',(0.,0.,-1.)) ;
#129768=DIRECTION('center_axis',(0.,-1.,0.)) ;
#129769=DIRECTION('ref_axis',(0.,0.,-1.)) ;
#129770=DIRECTION('center_axis',(0.,1.,0.)) ;
#129771=DIRECTION('ref_axis',(1.,0.,0.)) ;
#129772=DIRECTION('center_axis',(0.,0.,1.)) ;
#129773=DIRECTION('ref_axis',(-1.,0.,0.)) ;
#129774=DIRECTION('center_axis',(1.,0.,0.)) ;
#129775=DIRECTION('ref_axis',(0.,0.,1.)) ;
#129776=DIRECTION('center_axis',(0.,-1.,0.)) ;
#129777=DIRECTION('ref_axis',(0.,0.,-1.)) ;
#129778=DIRECTION('center_axis',(0.,1.,0.)) ;
#129779=DIRECTION('ref_axis',(0.,0.,1.)) ;
#129780=DIRECTION('center_axis',(0.,-1.,0.)) ;
#129781=DIRECTION('ref_axis',(0.,0.,-1.)) ;
#129782=DIRECTION('center_axis',(-1.,0.,2.16840434497101E-16)) ;
#129783=DIRECTION('ref_axis',(2.16840434497101E-16,0.,1.)) ;
#129784=DIRECTION('center_axis',(1.,0.,0.)) ;
#129785=DIRECTION('ref_axis',(0.,0.,-1.)) ;
#129786=DIRECTION('center_axis',(-2.16840434497101E-16,0.,1.)) ;
#129787=DIRECTION('ref_axis',(1.,0.,2.16840434497101E-16)) ;
#129788=DIRECTION('center_axis',(0.,0.,1.)) ;
#129789=DIRECTION('ref_axis',(1.,0.,0.)) ;
#129790=DIRECTION('center_axis',(0.,1.,0.)) ;
#129791=DIRECTION('ref_axis',(0.,0.,1.)) ;
#129792=DIRECTION('center_axis',(0.,-1.,0.)) ;
#129793=DIRECTION('ref_axis',(0.,0.,-1.)) ;
#129794=DIRECTION('center_axis',(0.,1.,0.)) ;
#129795=DIRECTION('ref_axis',(1.,0.,0.)) ;
#129796=DIRECTION('center_axis',(0.,0.,1.)) ;
#129797=DIRECTION('ref_axis',(-1.,0.,0.)) ;
#129798=DIRECTION('center_axis',(0.,1.,0.)) ;
#129799=DIRECTION('ref_axis',(1.,0.,0.)) ;
#129800=DIRECTION('center_axis',(1.,0.,0.)) ;
#129801=DIRECTION('ref_axis',(0.,0.,1.)) ;
#129802=DIRECTION('center_axis',(0.,0.,-1.)) ;
#129803=DIRECTION('ref_axis',(-1.,0.,0.)) ;
#129804=DIRECTION('center_axis',(0.,0.,1.)) ;
#129805=DIRECTION('ref_axis',(1.,0.,0.)) ;
#129806=DIRECTION('center_axis',(1.,0.,2.16840434497101E-16)) ;
#129807=DIRECTION('ref_axis',(2.16840434497101E-16,0.,-1.)) ;
#129808=DIRECTION('center_axis',(1.,0.,0.)) ;
#129809=DIRECTION('ref_axis',(0.,0.,-1.)) ;
#129810=DIRECTION('center_axis',(0.,1.,0.)) ;
#129811=DIRECTION('ref_axis',(1.,0.,0.)) ;
#129812=DIRECTION('center_axis',(0.,1.,0.)) ;
#129813=DIRECTION('ref_axis',(0.,0.,-1.)) ;
#129814=DIRECTION('center_axis',(0.,1.,0.)) ;
#129815=DIRECTION('ref_axis',(0.,0.,1.)) ;
#129816=DIRECTION('center_axis',(0.,1.,0.)) ;
#129817=DIRECTION('ref_axis',(0.,0.,1.)) ;
#129818=DIRECTION('center_axis',(-0.942809041582063,-0.235702260395516,
0.235702260395518)) ;
#129819=DIRECTION('ref_axis',(0.242535625036335,4.64743530723282E-16,0.970142500145331)) ;
#129820=DIRECTION('center_axis',(-0.970142500145332,-0.242535625036331,
-2.10366121255617E-15)) ;
#129821=DIRECTION('ref_axis',(0.242535625036331,-0.970142500145332,-4.47980524894761E-30)) ;
#129822=DIRECTION('center_axis',(0.970142500145333,0.24253562503633,0.)) ;
#129823=DIRECTION('ref_axis',(-0.24253562503633,0.970142500145333,0.)) ;
#129824=DIRECTION('center_axis',(-0.970142500145332,-0.242535625036331,
2.73475957632304E-14)) ;
#129825=DIRECTION('ref_axis',(0.242535625036331,-0.970142500145332,1.1454669517322E-30)) ;
#129826=DIRECTION('center_axis',(0.879462917689188,0.219865729422294,-0.42214220049081)) ;
#129827=DIRECTION('ref_axis',(-0.432731067584771,1.71515946658E-16,-0.901523057468274)) ;
#129828=DIRECTION('center_axis',(0.879462917689192,0.219865729422271,-0.422142200490814)) ;
#129829=DIRECTION('ref_axis',(-0.432731067584773,-1.62351711522009E-16,
-0.901523057468273)) ;
#129830=DIRECTION('center_axis',(0.,1.,0.)) ;
#129831=DIRECTION('ref_axis',(1.,0.,0.)) ;
#129832=DIRECTION('center_axis',(0.,-1.,0.)) ;
#129833=DIRECTION('ref_axis',(0.,0.,1.)) ;
#129834=DIRECTION('center_axis',(0.,-1.,0.)) ;
#129835=DIRECTION('ref_axis',(0.,0.,-1.)) ;
#129836=DIRECTION('center_axis',(-4.51750905202295E-15,-1.,2.16840434497102E-15)) ;
#129837=DIRECTION('ref_axis',(1.,-4.51750905202295E-15,3.91831450274151E-31)) ;
#129838=DIRECTION('center_axis',(0.669589480006976,-0.669589480006974,-0.321402950403349)) ;
#129839=DIRECTION('ref_axis',(0.707106781186547,0.707106781186548,5.45170614306381E-16)) ;
#129840=DIRECTION('center_axis',(0.669589480006977,-0.669589480006977,-0.321402950403342)) ;
#129841=DIRECTION('ref_axis',(0.707106781186547,0.707106781186548,-1.94221176494188E-16)) ;
#129842=DIRECTION('center_axis',(0.,1.,0.)) ;
#129843=DIRECTION('ref_axis',(1.,0.,0.)) ;
#129844=DIRECTION('center_axis',(0.707106781186541,-0.707106781186554,0.)) ;
#129845=DIRECTION('ref_axis',(-0.707106781186554,-0.707106781186541,0.)) ;
#129846=DIRECTION('center_axis',(0.707106781186549,-0.707106781186546,0.)) ;
#129847=DIRECTION('ref_axis',(0.707106781186546,0.707106781186549,0.)) ;
#129848=DIRECTION('center_axis',(0.707106781186548,-0.707106781186548,-1.53329341668338E-15)) ;
#129849=DIRECTION('ref_axis',(0.707106781186548,0.707106781186548,1.5356898865553E-31)) ;
#129850=DIRECTION('center_axis',(0.577350269189633,-0.577350269189633,-0.577350269189612)) ;
#129851=DIRECTION('ref_axis',(0.707106781186548,0.707106781186548,1.34560831514457E-17)) ;
#129852=DIRECTION('center_axis',(-0.577350269189344,0.577350269189586,-0.577350269189947)) ;
#129853=DIRECTION('ref_axis',(1.30446081606812E-15,0.707106781186769,0.707106781186326)) ;
#129854=DIRECTION('center_axis',(-0.707106781186548,0.707106781186548,7.66646708341692E-15)) ;
#129855=DIRECTION('ref_axis',(-0.707106781186548,-0.707106781186548,-2.68297081166629E-31)) ;
#129856=DIRECTION('center_axis',(-0.707106781186549,0.707106781186546,0.)) ;
#129857=DIRECTION('ref_axis',(-0.707106781186546,-0.707106781186549,0.)) ;
#129858=DIRECTION('center_axis',(-0.707106781186548,0.707106781186548,-1.22663473334671E-14)) ;
#129859=DIRECTION('ref_axis',(-0.707106781186548,-0.707106781186548,2.94725045705944E-31)) ;
#129860=DIRECTION('center_axis',(-0.669589480006976,0.669589480006974,-0.321402950403349)) ;
#129861=DIRECTION('ref_axis',(-0.707106781186547,-0.707106781186548,5.45170614306381E-16)) ;
#129862=DIRECTION('center_axis',(0.669589480006982,-0.669589480006966,0.321402950403353)) ;
#129863=DIRECTION('ref_axis',(0.707106781186539,0.707106781186556,5.77426876420606E-17)) ;
#129864=DIRECTION('center_axis',(0.,1.,0.)) ;
#129865=DIRECTION('ref_axis',(1.,0.,0.)) ;
#129866=DIRECTION('center_axis',(0.,1.,0.)) ;
#129867=DIRECTION('ref_axis',(0.,0.,-1.)) ;
#129868=DIRECTION('center_axis',(0.,-1.,0.)) ;
#129869=DIRECTION('ref_axis',(0.,0.,-1.)) ;
#129870=DIRECTION('center_axis',(0.,1.,0.)) ;
#129871=DIRECTION('ref_axis',(0.,0.,1.)) ;
#129872=DIRECTION('center_axis',(-0.879462917689188,-0.219865729422294,
-0.42214220049081)) ;
#129873=DIRECTION('ref_axis',(-0.432731067584771,1.71515946658E-16,0.901523057468274)) ;
#129874=DIRECTION('center_axis',(0.879462917689201,0.219865729422298,0.42214220049078)) ;
#129875=DIRECTION('ref_axis',(0.432731067584741,5.42470486237819E-16,-0.901523057468288)) ;
#129876=DIRECTION('center_axis',(0.,1.,0.)) ;
#129877=DIRECTION('ref_axis',(1.,0.,0.)) ;
#129878=DIRECTION('center_axis',(0.970142500145323,0.242535625036368,0.)) ;
#129879=DIRECTION('ref_axis',(0.242535625036368,-0.970142500145323,0.)) ;
#129880=DIRECTION('center_axis',(-0.970142500145333,-0.24253562503633,0.)) ;
#129881=DIRECTION('ref_axis',(0.24253562503633,-0.970142500145333,0.)) ;
#129882=DIRECTION('center_axis',(0.970142500145332,0.242535625036331,-2.10366121255617E-15)) ;
#129883=DIRECTION('ref_axis',(-0.242535625036331,0.970142500145332,-4.47980524894761E-30)) ;
#129884=DIRECTION('center_axis',(0.942809041582064,0.235702260395514,0.235702260395514)) ;
#129885=DIRECTION('ref_axis',(-0.242535625036331,0.970142500145332,4.49011373492972E-16)) ;
#129886=DIRECTION('center_axis',(0.,-1.,0.)) ;
#129887=DIRECTION('ref_axis',(0.,0.,-1.)) ;
#129888=DIRECTION('center_axis',(-1.,0.,-8.67361737988409E-15)) ;
#129889=DIRECTION('ref_axis',(-8.67361737988409E-15,0.,1.)) ;
#129890=DIRECTION('center_axis',(0.,0.,-1.)) ;
#129891=DIRECTION('ref_axis',(-1.,0.,0.)) ;
#129892=DIRECTION('center_axis',(0.,0.,-1.)) ;
#129893=DIRECTION('ref_axis',(-1.,0.,0.)) ;
#129894=DIRECTION('center_axis',(0.,3.46944695195362E-14,-1.)) ;
#129895=DIRECTION('ref_axis',(0.,1.,3.46944695195362E-14)) ;
#129896=DIRECTION('center_axis',(1.,0.,0.)) ;
#129897=DIRECTION('ref_axis',(0.,0.,-1.)) ;
#129898=DIRECTION('center_axis',(-1.,0.,0.)) ;
#129899=DIRECTION('ref_axis',(0.,0.,1.)) ;
#129900=DIRECTION('center_axis',(0.,-1.,0.)) ;
#129901=DIRECTION('ref_axis',(0.,0.,-1.)) ;
#129902=DIRECTION('center_axis',(-1.,0.,0.)) ;
#129903=DIRECTION('ref_axis',(0.,0.,1.)) ;
#129904=DIRECTION('center_axis',(0.,-1.,0.)) ;
#129905=DIRECTION('ref_axis',(0.,0.,-1.)) ;
#129906=DIRECTION('center_axis',(3.46944695195358E-14,0.,-1.)) ;
#129907=DIRECTION('ref_axis',(-1.,0.,-3.46944695195358E-14)) ;
#129908=DIRECTION('center_axis',(-1.,0.,0.)) ;
#129909=DIRECTION('ref_axis',(0.,0.,1.)) ;
#129910=DIRECTION('center_axis',(-1.,1.73472347597681E-14,0.)) ;
#129911=DIRECTION('ref_axis',(-1.73472347597681E-14,-1.,0.)) ;
#129912=DIRECTION('center_axis',(0.,0.,1.)) ;
#129913=DIRECTION('ref_axis',(1.,0.,0.)) ;
#129914=DIRECTION('center_axis',(-3.46944695195364E-14,0.,-1.)) ;
#129915=DIRECTION('ref_axis',(-1.,0.,3.46944695195364E-14)) ;
#129916=DIRECTION('center_axis',(0.,-1.,0.)) ;
#129917=DIRECTION('ref_axis',(0.,0.,-1.)) ;
#129918=DIRECTION('center_axis',(0.,-1.,0.)) ;
#129919=DIRECTION('ref_axis',(0.,0.,-1.)) ;
#129920=DIRECTION('center_axis',(0.,-1.,0.)) ;
#129921=DIRECTION('ref_axis',(0.,0.,-1.)) ;
#129922=DIRECTION('center_axis',(0.,0.,1.)) ;
#129923=DIRECTION('ref_axis',(1.,0.,0.)) ;
#129924=DIRECTION('center_axis',(0.,0.,-1.)) ;
#129925=DIRECTION('ref_axis',(-1.,0.,0.)) ;
#129926=DIRECTION('center_axis',(0.,0.,1.)) ;
#129927=DIRECTION('ref_axis',(1.,0.,0.)) ;
#129928=DIRECTION('center_axis',(0.,-1.,0.)) ;
#129929=DIRECTION('ref_axis',(0.,0.,-1.)) ;
#129930=DIRECTION('center_axis',(0.,-1.,0.)) ;
#129931=DIRECTION('ref_axis',(0.,0.,-1.)) ;
#129932=DIRECTION('center_axis',(0.,1.,0.)) ;
#129933=DIRECTION('ref_axis',(1.,0.,0.)) ;
#129934=DIRECTION('center_axis',(-1.,0.,0.)) ;
#129935=DIRECTION('ref_axis',(0.,0.,-1.)) ;
#129936=DIRECTION('center_axis',(0.,1.,0.)) ;
#129937=DIRECTION('ref_axis',(1.,0.,0.)) ;
#129938=DIRECTION('center_axis',(-1.,0.,0.)) ;
#129939=DIRECTION('ref_axis',(0.,0.,-1.)) ;
#129940=DIRECTION('center_axis',(0.,-1.,0.)) ;
#129941=DIRECTION('ref_axis',(0.,0.,-1.)) ;
#129942=DIRECTION('center_axis',(0.,-1.,0.)) ;
#129943=DIRECTION('ref_axis',(0.,0.,-1.)) ;
#129944=DIRECTION('center_axis',(-1.,0.,0.)) ;
#129945=DIRECTION('ref_axis',(0.,0.,1.)) ;
#129946=DIRECTION('center_axis',(-1.,0.,0.)) ;
#129947=DIRECTION('ref_axis',(0.,0.,1.)) ;
#129948=DIRECTION('center_axis',(1.,0.,0.)) ;
#129949=DIRECTION('ref_axis',(0.,0.,-1.)) ;
#129950=DIRECTION('center_axis',(-1.,0.,0.)) ;
#129951=DIRECTION('ref_axis',(0.,0.,1.)) ;
#129952=DIRECTION('center_axis',(0.,-1.,0.)) ;
#129953=DIRECTION('ref_axis',(0.,0.,-1.)) ;
#129954=DIRECTION('center_axis',(0.,-1.,0.)) ;
#129955=DIRECTION('ref_axis',(0.,0.,-1.)) ;
#129956=DIRECTION('center_axis',(0.,1.,0.)) ;
#129957=DIRECTION('ref_axis',(1.,0.,0.)) ;
#129958=DIRECTION('center_axis',(0.,0.,-1.)) ;
#129959=DIRECTION('ref_axis',(1.,0.,0.)) ;
#129960=DIRECTION('center_axis',(0.,1.,0.)) ;
#129961=DIRECTION('ref_axis',(1.,0.,0.)) ;
#129962=DIRECTION('center_axis',(0.,0.,1.)) ;
#129963=DIRECTION('ref_axis',(-1.,0.,0.)) ;
#129964=DIRECTION('center_axis',(0.,0.,-1.)) ;
#129965=DIRECTION('ref_axis',(-1.,0.,0.)) ;
#129966=DIRECTION('center_axis',(1.,1.31418445149758E-16,-2.16840434497101E-16)) ;
#129967=DIRECTION('ref_axis',(-2.16840434497101E-16,-2.8496832747207E-32,
-1.)) ;
#129968=DIRECTION('center_axis',(1.,0.,0.)) ;
#129969=DIRECTION('ref_axis',(0.,0.,-1.)) ;
#129970=DIRECTION('center_axis',(-1.,0.,0.)) ;
#129971=DIRECTION('ref_axis',(0.,0.,1.)) ;
#129972=DIRECTION('center_axis',(-1.31418445149758E-16,1.,0.)) ;
#129973=DIRECTION('ref_axis',(-1.,0.,0.)) ;
#129974=DIRECTION('center_axis',(0.,0.,1.)) ;
#129975=DIRECTION('ref_axis',(-1.,0.,0.)) ;
#129976=DIRECTION('center_axis',(-1.31418445149758E-16,1.,0.)) ;
#129977=DIRECTION('ref_axis',(-1.,-1.31418445149758E-16,0.)) ;
#129978=DIRECTION('center_axis',(-1.31418445149758E-16,1.,0.)) ;
#129979=DIRECTION('ref_axis',(-1.,0.,0.)) ;
#129980=DIRECTION('center_axis',(-1.31418445149758E-16,1.,0.)) ;
#129981=DIRECTION('ref_axis',(-1.,-1.31418445149758E-16,0.)) ;
#129982=DIRECTION('center_axis',(0.,0.,1.)) ;
#129983=DIRECTION('ref_axis',(-1.,0.,0.)) ;
#129984=DIRECTION('center_axis',(-4.33680868994202E-16,-5.69936654944139E-32,
-1.)) ;
#129985=DIRECTION('ref_axis',(-1.,2.47170623787823E-47,4.33680868994202E-16)) ;
#129986=DIRECTION('center_axis',(0.,0.,1.)) ;
#129987=DIRECTION('ref_axis',(1.,0.,0.)) ;
#129988=DIRECTION('center_axis',(-1.31418445149758E-16,-1.,0.)) ;
#129989=DIRECTION('ref_axis',(1.,-1.31418445149758E-16,0.)) ;
#129990=DIRECTION('center_axis',(0.,1.,0.)) ;
#129991=DIRECTION('ref_axis',(0.,0.,1.)) ;
#129992=DIRECTION('center_axis',(-1.,0.,2.16840434497101E-16)) ;
#129993=DIRECTION('ref_axis',(2.16840434497101E-16,0.,1.)) ;
#129994=DIRECTION('center_axis',(-1.,0.,0.)) ;
#129995=DIRECTION('ref_axis',(0.,0.,1.)) ;
#129996=DIRECTION('center_axis',(1.,0.,0.)) ;
#129997=DIRECTION('ref_axis',(0.,0.,-1.)) ;
#129998=DIRECTION('center_axis',(-1.31418445149758E-16,-1.,0.)) ;
#129999=DIRECTION('ref_axis',(1.,-1.31418445149758E-16,0.)) ;
#130000=DIRECTION('center_axis',(0.,1.,0.)) ;
#130001=DIRECTION('ref_axis',(0.,0.,1.)) ;
#130002=DIRECTION('center_axis',(2.16840434497101E-16,2.8496832747207E-32,
1.)) ;
#130003=DIRECTION('ref_axis',(1.,-6.17926559469557E-48,-2.16840434497101E-16)) ;
#130004=DIRECTION('center_axis',(0.,0.,1.)) ;
#130005=DIRECTION('ref_axis',(1.,0.,0.)) ;
#130006=DIRECTION('center_axis',(-1.,-1.31418445149758E-16,-2.16840434497101E-16)) ;
#130007=DIRECTION('ref_axis',(-2.16840434497101E-16,-2.8496832747207E-32,
1.)) ;
#130008=DIRECTION('center_axis',(-1.,0.,0.)) ;
#130009=DIRECTION('ref_axis',(0.,0.,1.)) ;
#130010=DIRECTION('center_axis',(1.,0.,0.)) ;
#130011=DIRECTION('ref_axis',(0.,0.,-1.)) ;
#130012=DIRECTION('center_axis',(-1.31418445149758E-16,1.,0.)) ;
#130013=DIRECTION('ref_axis',(-1.,0.,0.)) ;
#130014=DIRECTION('center_axis',(-1.31418445149758E-16,1.,0.)) ;
#130015=DIRECTION('ref_axis',(-1.,-1.31418445149758E-16,0.)) ;
#130016=DIRECTION('center_axis',(0.,1.,0.)) ;
#130017=DIRECTION('ref_axis',(1.,0.,0.)) ;
#130018=DIRECTION('center_axis',(0.,0.,-1.)) ;
#130019=DIRECTION('ref_axis',(1.,0.,0.)) ;
#130020=DIRECTION('center_axis',(0.,1.,0.)) ;
#130021=DIRECTION('ref_axis',(1.,0.,0.)) ;
#130022=DIRECTION('center_axis',(0.,0.,-1.)) ;
#130023=DIRECTION('ref_axis',(1.,0.,0.)) ;
#130024=DIRECTION('center_axis',(-1.31418445149758E-16,1.,0.)) ;
#130025=DIRECTION('ref_axis',(-1.,0.,0.)) ;
#130026=DIRECTION('center_axis',(-1.31418445149758E-16,1.,0.)) ;
#130027=DIRECTION('ref_axis',(-1.,-1.31418445149758E-16,0.)) ;
#130028=DIRECTION('center_axis',(-1.31418445149758E-16,-1.,0.)) ;
#130029=DIRECTION('ref_axis',(1.,-1.31418445149758E-16,0.)) ;
#130030=DIRECTION('center_axis',(0.,1.,0.)) ;
#130031=DIRECTION('ref_axis',(0.,0.,1.)) ;
#130032=DIRECTION('center_axis',(4.33680868994202E-16,0.,1.)) ;
#130033=DIRECTION('ref_axis',(1.,0.,-4.33680868994202E-16)) ;
#130034=DIRECTION('center_axis',(0.,0.,-1.)) ;
#130035=DIRECTION('ref_axis',(-1.,0.,0.)) ;
#130036=DIRECTION('center_axis',(-2.16840434497101E-16,0.,-1.)) ;
#130037=DIRECTION('ref_axis',(-1.,0.,2.16840434497101E-16)) ;
#130038=DIRECTION('center_axis',(0.,0.,-1.)) ;
#130039=DIRECTION('ref_axis',(-1.,0.,0.)) ;
#130040=DIRECTION('center_axis',(-1.31418445149758E-16,-1.,0.)) ;
#130041=DIRECTION('ref_axis',(1.,-1.31418445149758E-16,0.)) ;
#130042=DIRECTION('center_axis',(0.,1.,0.)) ;
#130043=DIRECTION('ref_axis',(0.,0.,1.)) ;
#130044=DIRECTION('center_axis',(0.,1.,0.)) ;
#130045=DIRECTION('ref_axis',(1.,0.,0.)) ;
#130046=DIRECTION('center_axis',(-1.,0.,0.)) ;
#130047=DIRECTION('ref_axis',(0.,0.,-1.)) ;
#130048=DIRECTION('center_axis',(0.,1.,0.)) ;
#130049=DIRECTION('ref_axis',(1.,0.,0.)) ;
#130050=DIRECTION('center_axis',(1.,0.,0.)) ;
#130051=DIRECTION('ref_axis',(0.,0.,1.)) ;
#130052=DIRECTION('center_axis',(1.,0.,2.16840434497101E-16)) ;
#130053=DIRECTION('ref_axis',(2.16840434497101E-16,0.,-1.)) ;
#130054=DIRECTION('center_axis',(0.,1.,0.)) ;
#130055=DIRECTION('ref_axis',(0.,0.,1.)) ;
#130056=DIRECTION('center_axis',(0.,1.,0.)) ;
#130057=DIRECTION('ref_axis',(0.,0.,1.)) ;
#130058=DIRECTION('center_axis',(0.,0.,-1.)) ;
#130059=DIRECTION('ref_axis',(-1.,0.,0.)) ;
#130060=DIRECTION('center_axis',(0.,0.,1.)) ;
#130061=DIRECTION('ref_axis',(1.,0.,0.)) ;
#130062=DIRECTION('center_axis',(0.,0.,-1.)) ;
#130063=DIRECTION('ref_axis',(-1.,0.,0.)) ;
#130064=DIRECTION('center_axis',(0.,1.,0.)) ;
#130065=DIRECTION('ref_axis',(0.,0.,1.)) ;
#130066=DIRECTION('center_axis',(0.,1.,0.)) ;
#130067=DIRECTION('ref_axis',(0.,0.,1.)) ;
#130068=DIRECTION('center_axis',(0.,1.,0.)) ;
#130069=DIRECTION('ref_axis',(1.,0.,0.)) ;
#130070=DIRECTION('center_axis',(-1.,0.,0.)) ;
#130071=DIRECTION('ref_axis',(0.,0.,-1.)) ;
#130072=DIRECTION('center_axis',(0.,1.,0.)) ;
#130073=DIRECTION('ref_axis',(1.,0.,0.)) ;
#130074=DIRECTION('center_axis',(-1.,0.,0.)) ;
#130075=DIRECTION('ref_axis',(0.,0.,-1.)) ;
#130076=DIRECTION('center_axis',(0.,1.,0.)) ;
#130077=DIRECTION('ref_axis',(0.,0.,1.)) ;
#130078=DIRECTION('center_axis',(0.,1.,0.)) ;
#130079=DIRECTION('ref_axis',(0.,0.,1.)) ;
#130080=DIRECTION('center_axis',(-1.,0.,0.)) ;
#130081=DIRECTION('ref_axis',(0.,0.,1.)) ;
#130082=DIRECTION('center_axis',(-1.,0.,0.)) ;
#130083=DIRECTION('ref_axis',(0.,0.,1.)) ;
#130084=DIRECTION('center_axis',(1.,0.,0.)) ;
#130085=DIRECTION('ref_axis',(0.,0.,-1.)) ;
#130086=DIRECTION('center_axis',(-1.,0.,0.)) ;
#130087=DIRECTION('ref_axis',(0.,0.,1.)) ;
#130088=DIRECTION('center_axis',(0.,1.,0.)) ;
#130089=DIRECTION('ref_axis',(0.,0.,1.)) ;
#130090=DIRECTION('center_axis',(0.,1.,0.)) ;
#130091=DIRECTION('ref_axis',(0.,0.,1.)) ;
#130092=DIRECTION('center_axis',(0.,1.,0.)) ;
#130093=DIRECTION('ref_axis',(1.,0.,0.)) ;
#130094=DIRECTION('center_axis',(0.,0.,1.)) ;
#130095=DIRECTION('ref_axis',(-1.,0.,0.)) ;
#130096=DIRECTION('center_axis',(0.,1.,0.)) ;
#130097=DIRECTION('ref_axis',(1.,0.,0.)) ;
#130098=DIRECTION('center_axis',(0.,0.,-1.)) ;
#130099=DIRECTION('ref_axis',(1.,0.,0.)) ;
#130100=DIRECTION('center_axis',(0.,0.,1.)) ;
#130101=DIRECTION('ref_axis',(1.,0.,0.)) ;
#130102=DIRECTION('center_axis',(0.,0.,1.)) ;
#130103=DIRECTION('ref_axis',(1.,0.,0.)) ;
#130104=DIRECTION('center_axis',(0.,0.,-1.)) ;
#130105=DIRECTION('ref_axis',(-1.,0.,0.)) ;
#130106=DIRECTION('center_axis',(-3.46944695195361E-14,0.,1.)) ;
#130107=DIRECTION('ref_axis',(1.,0.,3.46944695195361E-14)) ;
#130108=DIRECTION('center_axis',(1.,0.,0.)) ;
#130109=DIRECTION('ref_axis',(0.,0.,-1.)) ;
#130110=DIRECTION('center_axis',(1.,0.,0.)) ;
#130111=DIRECTION('ref_axis',(0.,0.,-1.)) ;
#130112=DIRECTION('center_axis',(1.,0.,0.)) ;
#130113=DIRECTION('ref_axis',(0.,0.,-1.)) ;
#130114=DIRECTION('center_axis',(1.,0.,8.67361737988409E-15)) ;
#130115=DIRECTION('ref_axis',(8.67361737988409E-15,0.,-1.)) ;
#130116=DIRECTION('center_axis',(1.,0.,0.)) ;
#130117=DIRECTION('ref_axis',(0.,0.,-1.)) ;
#130118=DIRECTION('center_axis',(1.,0.,1.73472347597682E-14)) ;
#130119=DIRECTION('ref_axis',(1.73472347597682E-14,0.,-1.)) ;
#130120=DIRECTION('center_axis',(-1.,0.,0.)) ;
#130121=DIRECTION('ref_axis',(0.,0.,1.)) ;
#130122=DIRECTION('center_axis',(1.,0.,0.)) ;
#130123=DIRECTION('ref_axis',(0.,0.,-1.)) ;
#130124=DIRECTION('center_axis',(1.,0.,0.)) ;
#130125=DIRECTION('ref_axis',(0.,0.,-1.)) ;
#130126=DIRECTION('center_axis',(-3.46944695195364E-14,0.,-1.)) ;
#130127=DIRECTION('ref_axis',(-1.,0.,3.46944695195364E-14)) ;
#130128=DIRECTION('center_axis',(1.,0.,0.)) ;
#130129=DIRECTION('ref_axis',(0.,0.,-1.)) ;
#130130=DIRECTION('center_axis',(-3.46944695195364E-14,0.,1.)) ;
#130131=DIRECTION('ref_axis',(1.,0.,3.46944695195364E-14)) ;
#130132=DIRECTION('center_axis',(0.,0.,-1.)) ;
#130133=DIRECTION('ref_axis',(-1.,0.,0.)) ;
#130134=DIRECTION('center_axis',(-0.422618261740697,5.55398348498559E-17,
0.906307787036651)) ;
#130135=DIRECTION('ref_axis',(0.906307787036651,6.51773046476477E-31,0.422618261740697)) ;
#130136=DIRECTION('center_axis',(0.422618261740697,-5.55398348498559E-17,
-0.906307787036651)) ;
#130137=DIRECTION('ref_axis',(-0.906307787036651,-6.46086972436398E-31,
-0.422618261740697)) ;
#130138=DIRECTION('center_axis',(-0.422618261740697,5.55398348498559E-17,
0.906307787036651)) ;
#130139=DIRECTION('ref_axis',(0.906307787036651,6.46086972436398E-31,0.422618261740697)) ;
#130140=DIRECTION('center_axis',(0.422618261740697,-5.55398348498559E-17,
-0.906307787036651)) ;
#130141=DIRECTION('ref_axis',(-0.906307787036651,-6.46086972436398E-31,
-0.422618261740697)) ;
#130142=DIRECTION('center_axis',(0.,1.,0.)) ;
#130143=DIRECTION('ref_axis',(1.,0.,0.)) ;
#130144=DIRECTION('center_axis',(3.4216004848576E-14,0.514231796959095,
-0.857651245551606)) ;
#130145=DIRECTION('ref_axis',(3.46944695195362E-14,-0.857651245551606,-0.514231796959095)) ;
#130146=DIRECTION('center_axis',(0.,-3.46944695195362E-14,1.)) ;
#130147=DIRECTION('ref_axis',(0.,1.,3.46944695195362E-14)) ;
#130148=DIRECTION('center_axis',(-1.,0.,0.)) ;
#130149=DIRECTION('ref_axis',(0.,-4.33680868994204E-15,-1.)) ;
#130150=DIRECTION('center_axis',(0.,0.,1.)) ;
#130151=DIRECTION('ref_axis',(1.,0.,0.)) ;
#130152=DIRECTION('center_axis',(0.,0.,1.)) ;
#130153=DIRECTION('ref_axis',(1.,0.,0.)) ;
#130154=DIRECTION('center_axis',(-1.,0.,0.)) ;
#130155=DIRECTION('ref_axis',(0.,0.,1.)) ;
#130156=DIRECTION('center_axis',(-1.,0.,0.)) ;
#130157=DIRECTION('ref_axis',(0.,-4.33680868994204E-15,-1.)) ;
#130158=DIRECTION('center_axis',(1.,0.,0.)) ;
#130159=DIRECTION('ref_axis',(0.,0.,-1.)) ;
#130160=DIRECTION('center_axis',(0.,-0.514231796959124,-0.857651245551588)) ;
#130161=DIRECTION('ref_axis',(0.,0.857651245551588,-0.514231796959124)) ;
#130162=DIRECTION('center_axis',(0.,1.,8.97270763436279E-17)) ;
#130163=DIRECTION('ref_axis',(0.,-8.97270763436279E-17,1.)) ;
#130164=DIRECTION('center_axis',(0.,-1.,-8.97270763436279E-17)) ;
#130165=DIRECTION('ref_axis',(0.,-8.97270763436279E-17,1.)) ;
#130166=DIRECTION('center_axis',(0.,-1.,0.)) ;
#130167=DIRECTION('ref_axis',(0.,0.,-1.)) ;
#130168=DIRECTION('center_axis',(0.,1.,0.)) ;
#130169=DIRECTION('ref_axis',(1.,0.,0.)) ;
#130170=DIRECTION('center_axis',(-1.,0.,0.)) ;
#130171=DIRECTION('ref_axis',(0.,0.,-1.)) ;
#130172=DIRECTION('center_axis',(1.,0.,0.)) ;
#130173=DIRECTION('ref_axis',(0.,0.,-1.)) ;
#130174=DIRECTION('center_axis',(0.,-0.514231796959093,0.857651245551607)) ;
#130175=DIRECTION('ref_axis',(0.,0.857651245551607,0.514231796959093)) ;
#130176=DIRECTION('center_axis',(0.,0.,-1.)) ;
#130177=DIRECTION('ref_axis',(1.,0.,0.)) ;
#130178=DIRECTION('center_axis',(0.,1.,0.)) ;
#130179=DIRECTION('ref_axis',(1.,0.,0.)) ;
#130180=DIRECTION('center_axis',(-3.46944695195364E-14,0.,-1.)) ;
#130181=DIRECTION('ref_axis',(1.,0.,-3.46944695195364E-14)) ;
#130182=DIRECTION('center_axis',(-1.,0.,0.)) ;
#130183=DIRECTION('ref_axis',(0.,4.33680868994204E-15,-1.)) ;
#130184=DIRECTION('center_axis',(0.,0.,-1.)) ;
#130185=DIRECTION('ref_axis',(-1.,0.,0.)) ;
#130186=DIRECTION('center_axis',(0.,0.,1.)) ;
#130187=DIRECTION('ref_axis',(-1.,0.,0.)) ;
#130188=DIRECTION('center_axis',(0.,0.,-1.)) ;
#130189=DIRECTION('ref_axis',(-1.,0.,0.)) ;
#130190=DIRECTION('center_axis',(-1.,0.,7.01133629567814E-33)) ;
#130191=DIRECTION('ref_axis',(7.01133629567814E-33,0.,1.)) ;
#130192=DIRECTION('center_axis',(-1.,0.,0.)) ;
#130193=DIRECTION('ref_axis',(0.,0.,1.)) ;
#130194=DIRECTION('center_axis',(0.,0.,-1.)) ;
#130195=DIRECTION('ref_axis',(-1.,0.,0.)) ;
#130196=DIRECTION('center_axis',(-7.01133629567814E-33,8.97270763436279E-17,
-1.)) ;
#130197=DIRECTION('ref_axis',(6.29106707073161E-49,1.,8.97270763436279E-17)) ;
#130198=DIRECTION('center_axis',(1.,0.,0.)) ;
#130199=DIRECTION('ref_axis',(0.,0.,-1.)) ;
#130200=DIRECTION('center_axis',(-2.2301249256967E-15,0.514231796959095,
0.857651245551606)) ;
#130201=DIRECTION('ref_axis',(-4.79361507851841E-30,-0.857651245551606,
0.514231796959095)) ;
#130202=DIRECTION('center_axis',(-1.,0.,0.)) ;
#130203=DIRECTION('ref_axis',(0.,0.,1.)) ;
#130204=DIRECTION('center_axis',(-1.,0.,0.)) ;
#130205=DIRECTION('ref_axis',(0.,-4.33680868994204E-15,-1.)) ;
#130206=DIRECTION('center_axis',(0.,0.,1.)) ;
#130207=DIRECTION('ref_axis',(1.,0.,0.)) ;
#130208=DIRECTION('center_axis',(0.,0.,-1.)) ;
#130209=DIRECTION('ref_axis',(-1.,0.,0.)) ;
#130210=DIRECTION('center_axis',(0.,-1.,8.97270763436279E-17)) ;
#130211=DIRECTION('ref_axis',(0.,-8.97270763436279E-17,-1.)) ;
#130212=DIRECTION('center_axis',(0.,-1.,8.97270763436279E-17)) ;
#130213=DIRECTION('ref_axis',(0.,-8.97270763436279E-17,-1.)) ;
#130214=DIRECTION('center_axis',(0.,-1.,0.)) ;
#130215=DIRECTION('ref_axis',(0.,0.,-1.)) ;
#130216=DIRECTION('center_axis',(-7.01133629567814E-33,8.97270763436279E-17,
-1.)) ;
#130217=DIRECTION('ref_axis',(0.,1.,0.)) ;
#130218=DIRECTION('center_axis',(0.,-1.,0.)) ;
#130219=DIRECTION('ref_axis',(0.,0.,1.)) ;
#130220=DIRECTION('center_axis',(1.,0.,0.)) ;
#130221=DIRECTION('ref_axis',(0.,0.,-1.)) ;
#130222=DIRECTION('center_axis',(0.,0.,1.)) ;
#130223=DIRECTION('ref_axis',(-1.,0.,0.)) ;
#130224=DIRECTION('center_axis',(0.,1.,0.)) ;
#130225=DIRECTION('ref_axis',(1.,0.,0.)) ;
#130226=DIRECTION('center_axis',(-1.,0.,0.)) ;
#130227=DIRECTION('ref_axis',(0.,0.,-1.)) ;
#130228=DIRECTION('center_axis',(1.,7.81406971160724E-17,0.)) ;
#130229=DIRECTION('ref_axis',(-7.81406971160724E-17,1.,0.)) ;
#130230=DIRECTION('center_axis',(1.,0.,0.)) ;
#130231=DIRECTION('ref_axis',(0.,0.,-1.)) ;
#130232=DIRECTION('center_axis',(1.,0.,0.)) ;
#130233=DIRECTION('ref_axis',(0.,0.,-1.)) ;
#130234=DIRECTION('center_axis',(0.,1.,8.97270763436279E-17)) ;
#130235=DIRECTION('ref_axis',(0.,-8.97270763436279E-17,1.)) ;
#130236=DIRECTION('center_axis',(0.,-1.,0.)) ;
#130237=DIRECTION('ref_axis',(0.,0.,-1.)) ;
#130238=DIRECTION('center_axis',(0.,0.,-1.)) ;
#130239=DIRECTION('ref_axis',(-1.,0.,0.)) ;
#130240=DIRECTION('center_axis',(-7.01133629567814E-33,8.97270763436279E-17,
1.)) ;
#130241=DIRECTION('ref_axis',(-6.29106707073161E-49,-1.,8.97270763436279E-17)) ;
#130242=DIRECTION('center_axis',(-1.,0.,-7.01133629567814E-33)) ;
#130243=DIRECTION('ref_axis',(-7.01133629567814E-33,0.,1.)) ;
#130244=DIRECTION('center_axis',(-1.,0.,0.)) ;
#130245=DIRECTION('ref_axis',(0.,0.,1.)) ;
#130246=DIRECTION('center_axis',(1.,0.,0.)) ;
#130247=DIRECTION('ref_axis',(0.,1.,0.)) ;
#130248=DIRECTION('center_axis',(2.16840434497101E-15,1.,0.)) ;
#130249=DIRECTION('ref_axis',(-1.,2.16840434497101E-15,0.)) ;
#130250=DIRECTION('center_axis',(0.,1.,0.)) ;
#130251=DIRECTION('ref_axis',(1.,0.,0.)) ;
#130252=DIRECTION('center_axis',(0.,0.,-1.)) ;
#130253=DIRECTION('ref_axis',(1.,0.,0.)) ;
#130254=DIRECTION('center_axis',(-1.,0.,0.)) ;
#130255=DIRECTION('ref_axis',(0.,0.,-1.)) ;
#130256=DIRECTION('center_axis',(-7.01133629567814E-33,8.97270763436279E-17,
1.)) ;
#130257=DIRECTION('ref_axis',(0.,-1.,0.)) ;
#130258=DIRECTION('center_axis',(0.,-1.,0.)) ;
#130259=DIRECTION('ref_axis',(0.,0.,1.)) ;
#130260=DIRECTION('center_axis',(7.81406971160724E-17,-1.,-8.97270763436279E-17)) ;
#130261=DIRECTION('ref_axis',(-7.01133629567814E-33,8.97270763436279E-17,
-1.)) ;
#130262=DIRECTION('center_axis',(0.,1.,0.)) ;
#130263=DIRECTION('ref_axis',(0.,0.,1.)) ;
#130264=DIRECTION('center_axis',(-1.,-7.81406971160724E-17,0.)) ;
#130265=DIRECTION('ref_axis',(7.81406971160724E-17,-1.,0.)) ;
#130266=DIRECTION('center_axis',(-1.,-7.81406971160724E-17,0.)) ;
#130267=DIRECTION('ref_axis',(-7.81406971160724E-17,1.,0.)) ;
#130268=DIRECTION('center_axis',(0.,0.,1.)) ;
#130269=DIRECTION('ref_axis',(1.,0.,0.)) ;
#130270=DIRECTION('center_axis',(0.,0.,-1.)) ;
#130271=DIRECTION('ref_axis',(-1.,0.,0.)) ;
#130272=DIRECTION('center_axis',(0.,-1.,8.97270763436279E-17)) ;
#130273=DIRECTION('ref_axis',(0.,-8.97270763436279E-17,-1.)) ;
#130274=DIRECTION('center_axis',(0.,-1.,0.)) ;
#130275=DIRECTION('ref_axis',(0.,0.,-1.)) ;
#130276=DIRECTION('center_axis',(1.,7.81406971160724E-17,0.)) ;
#130277=DIRECTION('ref_axis',(0.,1.,0.)) ;
#130278=DIRECTION('center_axis',(0.,0.,1.)) ;
#130279=DIRECTION('ref_axis',(-1.,0.,0.)) ;
#130280=DIRECTION('center_axis',(0.,1.,0.)) ;
#130281=DIRECTION('ref_axis',(1.,0.,0.)) ;
#130282=DIRECTION('center_axis',(-1.,0.,0.)) ;
#130283=DIRECTION('ref_axis',(0.,0.,-1.)) ;
#130284=DIRECTION('center_axis',(0.,0.,-1.)) ;
#130285=DIRECTION('ref_axis',(-1.,0.,0.)) ;
#130286=DIRECTION('center_axis',(0.,0.,1.)) ;
#130287=DIRECTION('ref_axis',(1.,0.,0.)) ;
#130288=DIRECTION('center_axis',(-1.,-7.81406971160724E-17,0.)) ;
#130289=DIRECTION('ref_axis',(7.81406971160724E-17,-1.,0.)) ;
#130290=DIRECTION('center_axis',(-1.,-7.81406971160724E-17,0.)) ;
#130291=DIRECTION('ref_axis',(-7.81406971160724E-17,1.,0.)) ;
#130292=DIRECTION('center_axis',(1.,7.81406971160724E-17,0.)) ;
#130293=DIRECTION('ref_axis',(-7.81406971160724E-17,1.,0.)) ;
#130294=DIRECTION('center_axis',(1.,0.,0.)) ;
#130295=DIRECTION('ref_axis',(0.,0.,-1.)) ;
#130296=DIRECTION('center_axis',(1.,0.,0.)) ;
#130297=DIRECTION('ref_axis',(0.,0.,-1.)) ;
#130298=DIRECTION('center_axis',(3.78638272950961E-32,-4.8455963016112E-16,
-1.)) ;
#130299=DIRECTION('ref_axis',(1.83472821505963E-47,1.,-4.8455963016112E-16)) ;
#130300=DIRECTION('center_axis',(3.78638272950961E-32,-4.8455963016112E-16,
-1.)) ;
#130301=DIRECTION('ref_axis',(1.83472821505963E-47,1.,-4.8455963016112E-16)) ;
#130302=DIRECTION('center_axis',(0.,0.,-1.)) ;
#130303=DIRECTION('ref_axis',(-1.,0.,0.)) ;
#130304=DIRECTION('center_axis',(1.,7.81406971160724E-17,0.)) ;
#130305=DIRECTION('ref_axis',(0.,1.,0.)) ;
#130306=DIRECTION('center_axis',(0.,-1.,0.)) ;
#130307=DIRECTION('ref_axis',(0.,0.,1.)) ;
#130308=DIRECTION('center_axis',(0.,1.,0.)) ;
#130309=DIRECTION('ref_axis',(1.,0.,0.)) ;
#130310=DIRECTION('center_axis',(0.,1.,0.)) ;
#130311=DIRECTION('ref_axis',(0.,0.,-1.)) ;
#130312=DIRECTION('center_axis',(-7.81406971160724E-17,1.,-8.97270763436279E-17)) ;
#130313=DIRECTION('ref_axis',(-7.01133629567814E-33,8.97270763436279E-17,
1.)) ;
#130314=DIRECTION('center_axis',(0.,-1.,0.)) ;
#130315=DIRECTION('ref_axis',(0.,0.,-1.)) ;
#130316=DIRECTION('center_axis',(0.,1.,0.)) ;
#130317=DIRECTION('ref_axis',(0.,0.,1.)) ;
#130318=DIRECTION('center_axis',(0.,-1.,0.)) ;
#130319=DIRECTION('ref_axis',(0.,0.,-1.)) ;
#130320=DIRECTION('center_axis',(0.,-1.,0.)) ;
#130321=DIRECTION('ref_axis',(0.,0.,-1.)) ;
#130322=DIRECTION('center_axis',(0.,1.,0.)) ;
#130323=DIRECTION('ref_axis',(1.,0.,0.)) ;
#130324=DIRECTION('center_axis',(0.,0.,1.)) ;
#130325=DIRECTION('ref_axis',(-1.,0.,0.)) ;
#130326=DIRECTION('center_axis',(1.,0.,0.)) ;
#130327=DIRECTION('ref_axis',(0.,0.,1.)) ;
#130328=DIRECTION('center_axis',(0.,-1.,0.)) ;
#130329=DIRECTION('ref_axis',(0.,0.,-1.)) ;
#130330=DIRECTION('center_axis',(0.,1.,0.)) ;
#130331=DIRECTION('ref_axis',(0.,0.,1.)) ;
#130332=DIRECTION('center_axis',(0.,-1.,0.)) ;
#130333=DIRECTION('ref_axis',(0.,0.,-1.)) ;
#130334=DIRECTION('center_axis',(-1.,0.,2.16840434497101E-16)) ;
#130335=DIRECTION('ref_axis',(2.16840434497101E-16,0.,1.)) ;
#130336=DIRECTION('center_axis',(1.,0.,0.)) ;
#130337=DIRECTION('ref_axis',(0.,0.,-1.)) ;
#130338=DIRECTION('center_axis',(-2.16840434497101E-16,0.,1.)) ;
#130339=DIRECTION('ref_axis',(1.,0.,2.16840434497101E-16)) ;
#130340=DIRECTION('center_axis',(0.,0.,1.)) ;
#130341=DIRECTION('ref_axis',(1.,0.,0.)) ;
#130342=DIRECTION('center_axis',(0.,1.,0.)) ;
#130343=DIRECTION('ref_axis',(0.,0.,1.)) ;
#130344=DIRECTION('center_axis',(0.,-1.,0.)) ;
#130345=DIRECTION('ref_axis',(0.,0.,-1.)) ;
#130346=DIRECTION('center_axis',(0.,1.,0.)) ;
#130347=DIRECTION('ref_axis',(1.,0.,0.)) ;
#130348=DIRECTION('center_axis',(0.,0.,1.)) ;
#130349=DIRECTION('ref_axis',(-1.,0.,0.)) ;
#130350=DIRECTION('center_axis',(0.,1.,0.)) ;
#130351=DIRECTION('ref_axis',(1.,0.,0.)) ;
#130352=DIRECTION('center_axis',(1.,0.,0.)) ;
#130353=DIRECTION('ref_axis',(0.,0.,1.)) ;
#130354=DIRECTION('center_axis',(0.,0.,-1.)) ;
#130355=DIRECTION('ref_axis',(-1.,0.,0.)) ;
#130356=DIRECTION('center_axis',(0.,0.,1.)) ;
#130357=DIRECTION('ref_axis',(1.,0.,0.)) ;
#130358=DIRECTION('center_axis',(1.,0.,2.16840434497101E-16)) ;
#130359=DIRECTION('ref_axis',(2.16840434497101E-16,0.,-1.)) ;
#130360=DIRECTION('center_axis',(1.,0.,0.)) ;
#130361=DIRECTION('ref_axis',(0.,0.,-1.)) ;
#130362=DIRECTION('center_axis',(0.,1.,0.)) ;
#130363=DIRECTION('ref_axis',(1.,0.,0.)) ;
#130364=DIRECTION('center_axis',(0.,1.,0.)) ;
#130365=DIRECTION('ref_axis',(0.,0.,-1.)) ;
#130366=DIRECTION('center_axis',(0.,1.,0.)) ;
#130367=DIRECTION('ref_axis',(0.,0.,1.)) ;
#130368=DIRECTION('center_axis',(0.,1.,0.)) ;
#130369=DIRECTION('ref_axis',(0.,0.,1.)) ;
#130370=DIRECTION('center_axis',(-0.942809041582063,-0.235702260395516,
0.235702260395518)) ;
#130371=DIRECTION('ref_axis',(0.242535625036335,4.64743530723282E-16,0.970142500145331)) ;
#130372=DIRECTION('center_axis',(-0.970142500145332,-0.242535625036331,
-2.10366121255617E-15)) ;
#130373=DIRECTION('ref_axis',(0.242535625036331,-0.970142500145332,-4.47980524894761E-30)) ;
#130374=DIRECTION('center_axis',(0.970142500145333,0.24253562503633,0.)) ;
#130375=DIRECTION('ref_axis',(-0.24253562503633,0.970142500145333,0.)) ;
#130376=DIRECTION('center_axis',(-0.970142500145332,-0.242535625036331,
2.73475957632304E-14)) ;
#130377=DIRECTION('ref_axis',(0.242535625036331,-0.970142500145332,1.1454669517322E-30)) ;
#130378=DIRECTION('center_axis',(0.879462917689188,0.219865729422294,-0.42214220049081)) ;
#130379=DIRECTION('ref_axis',(-0.432731067584771,1.71515946658E-16,-0.901523057468274)) ;
#130380=DIRECTION('center_axis',(0.879462917689192,0.219865729422271,-0.422142200490814)) ;
#130381=DIRECTION('ref_axis',(-0.432731067584773,-1.62351711522009E-16,
-0.901523057468273)) ;
#130382=DIRECTION('center_axis',(0.,1.,0.)) ;
#130383=DIRECTION('ref_axis',(1.,0.,0.)) ;
#130384=DIRECTION('center_axis',(0.,-1.,0.)) ;
#130385=DIRECTION('ref_axis',(0.,0.,1.)) ;
#130386=DIRECTION('center_axis',(0.,-1.,0.)) ;
#130387=DIRECTION('ref_axis',(0.,0.,-1.)) ;
#130388=DIRECTION('center_axis',(-4.51750905202295E-15,-1.,2.16840434497102E-15)) ;
#130389=DIRECTION('ref_axis',(1.,-4.51750905202295E-15,3.91831450274151E-31)) ;
#130390=DIRECTION('center_axis',(0.669589480006976,-0.669589480006974,-0.321402950403349)) ;
#130391=DIRECTION('ref_axis',(0.707106781186547,0.707106781186548,5.45170614306381E-16)) ;
#130392=DIRECTION('center_axis',(0.669589480006977,-0.669589480006977,-0.321402950403342)) ;
#130393=DIRECTION('ref_axis',(0.707106781186547,0.707106781186548,-1.94221176494188E-16)) ;
#130394=DIRECTION('center_axis',(0.,1.,0.)) ;
#130395=DIRECTION('ref_axis',(1.,0.,0.)) ;
#130396=DIRECTION('center_axis',(0.707106781186541,-0.707106781186554,0.)) ;
#130397=DIRECTION('ref_axis',(-0.707106781186554,-0.707106781186541,0.)) ;
#130398=DIRECTION('center_axis',(0.707106781186549,-0.707106781186546,0.)) ;
#130399=DIRECTION('ref_axis',(0.707106781186546,0.707106781186549,0.)) ;
#130400=DIRECTION('center_axis',(0.707106781186548,-0.707106781186548,-1.53329341668338E-15)) ;
#130401=DIRECTION('ref_axis',(0.707106781186548,0.707106781186548,1.5356898865553E-31)) ;
#130402=DIRECTION('center_axis',(0.577350269189633,-0.577350269189633,-0.577350269189612)) ;
#130403=DIRECTION('ref_axis',(0.707106781186548,0.707106781186548,1.34560831514457E-17)) ;
#130404=DIRECTION('center_axis',(-0.577350269189344,0.577350269189586,-0.577350269189947)) ;
#130405=DIRECTION('ref_axis',(1.30446081606812E-15,0.707106781186769,0.707106781186326)) ;
#130406=DIRECTION('center_axis',(-0.707106781186548,0.707106781186548,7.66646708341692E-15)) ;
#130407=DIRECTION('ref_axis',(-0.707106781186548,-0.707106781186548,-2.68297081166629E-31)) ;
#130408=DIRECTION('center_axis',(-0.707106781186549,0.707106781186546,0.)) ;
#130409=DIRECTION('ref_axis',(-0.707106781186546,-0.707106781186549,0.)) ;
#130410=DIRECTION('center_axis',(-0.707106781186548,0.707106781186548,-1.22663473334671E-14)) ;
#130411=DIRECTION('ref_axis',(-0.707106781186548,-0.707106781186548,2.94725045705944E-31)) ;
#130412=DIRECTION('center_axis',(-0.669589480006976,0.669589480006974,-0.321402950403349)) ;
#130413=DIRECTION('ref_axis',(-0.707106781186547,-0.707106781186548,5.45170614306381E-16)) ;
#130414=DIRECTION('center_axis',(0.669589480006982,-0.669589480006966,0.321402950403353)) ;
#130415=DIRECTION('ref_axis',(0.707106781186539,0.707106781186556,5.77426876420606E-17)) ;
#130416=DIRECTION('center_axis',(0.,1.,0.)) ;
#130417=DIRECTION('ref_axis',(1.,0.,0.)) ;
#130418=DIRECTION('center_axis',(0.,1.,0.)) ;
#130419=DIRECTION('ref_axis',(0.,0.,-1.)) ;
#130420=DIRECTION('center_axis',(0.,-1.,0.)) ;
#130421=DIRECTION('ref_axis',(0.,0.,-1.)) ;
#130422=DIRECTION('center_axis',(0.,1.,0.)) ;
#130423=DIRECTION('ref_axis',(0.,0.,1.)) ;
#130424=DIRECTION('center_axis',(-0.879462917689188,-0.219865729422294,
-0.42214220049081)) ;
#130425=DIRECTION('ref_axis',(-0.432731067584771,1.71515946658E-16,0.901523057468274)) ;
#130426=DIRECTION('center_axis',(0.879462917689201,0.219865729422298,0.42214220049078)) ;
#130427=DIRECTION('ref_axis',(0.432731067584741,5.42470486237819E-16,-0.901523057468288)) ;
#130428=DIRECTION('center_axis',(0.,1.,0.)) ;
#130429=DIRECTION('ref_axis',(1.,0.,0.)) ;
#130430=DIRECTION('center_axis',(0.970142500145323,0.242535625036368,0.)) ;
#130431=DIRECTION('ref_axis',(0.242535625036368,-0.970142500145323,0.)) ;
#130432=DIRECTION('center_axis',(-0.970142500145333,-0.24253562503633,0.)) ;
#130433=DIRECTION('ref_axis',(0.24253562503633,-0.970142500145333,0.)) ;
#130434=DIRECTION('center_axis',(0.970142500145332,0.242535625036331,-2.10366121255617E-15)) ;
#130435=DIRECTION('ref_axis',(-0.242535625036331,0.970142500145332,-4.47980524894761E-30)) ;
#130436=DIRECTION('center_axis',(0.942809041582064,0.235702260395514,0.235702260395514)) ;
#130437=DIRECTION('ref_axis',(-0.242535625036331,0.970142500145332,4.49011373492972E-16)) ;
#130438=DIRECTION('center_axis',(0.,-1.,0.)) ;
#130439=DIRECTION('ref_axis',(0.,0.,-1.)) ;
#130440=DIRECTION('center_axis',(-1.,0.,-8.67361737988409E-15)) ;
#130441=DIRECTION('ref_axis',(-8.67361737988409E-15,0.,1.)) ;
#130442=DIRECTION('center_axis',(0.,0.,-1.)) ;
#130443=DIRECTION('ref_axis',(-1.,0.,0.)) ;
#130444=DIRECTION('center_axis',(0.,0.,-1.)) ;
#130445=DIRECTION('ref_axis',(-1.,0.,0.)) ;
#130446=DIRECTION('center_axis',(0.,3.46944695195362E-14,-1.)) ;
#130447=DIRECTION('ref_axis',(0.,1.,3.46944695195362E-14)) ;
#130448=DIRECTION('center_axis',(1.,0.,0.)) ;
#130449=DIRECTION('ref_axis',(0.,0.,-1.)) ;
#130450=DIRECTION('center_axis',(-1.,0.,0.)) ;
#130451=DIRECTION('ref_axis',(0.,0.,1.)) ;
#130452=DIRECTION('center_axis',(0.,-1.,0.)) ;
#130453=DIRECTION('ref_axis',(0.,0.,-1.)) ;
#130454=DIRECTION('center_axis',(-1.,0.,0.)) ;
#130455=DIRECTION('ref_axis',(0.,0.,1.)) ;
#130456=DIRECTION('center_axis',(0.,-1.,0.)) ;
#130457=DIRECTION('ref_axis',(0.,0.,-1.)) ;
#130458=DIRECTION('center_axis',(3.46944695195358E-14,0.,-1.)) ;
#130459=DIRECTION('ref_axis',(-1.,0.,-3.46944695195358E-14)) ;
#130460=DIRECTION('center_axis',(-1.,0.,0.)) ;
#130461=DIRECTION('ref_axis',(0.,0.,1.)) ;
#130462=DIRECTION('center_axis',(-1.,1.73472347597681E-14,0.)) ;
#130463=DIRECTION('ref_axis',(-1.73472347597681E-14,-1.,0.)) ;
#130464=DIRECTION('center_axis',(0.,0.,1.)) ;
#130465=DIRECTION('ref_axis',(1.,0.,0.)) ;
#130466=DIRECTION('center_axis',(-3.46944695195364E-14,0.,-1.)) ;
#130467=DIRECTION('ref_axis',(-1.,0.,3.46944695195364E-14)) ;
#130468=DIRECTION('center_axis',(0.,-1.,0.)) ;
#130469=DIRECTION('ref_axis',(0.,0.,-1.)) ;
#130470=DIRECTION('center_axis',(0.,-1.,0.)) ;
#130471=DIRECTION('ref_axis',(0.,0.,-1.)) ;
#130472=DIRECTION('center_axis',(0.,-1.,0.)) ;
#130473=DIRECTION('ref_axis',(0.,0.,-1.)) ;
#130474=DIRECTION('center_axis',(0.,0.,1.)) ;
#130475=DIRECTION('ref_axis',(1.,0.,0.)) ;
#130476=DIRECTION('center_axis',(0.,0.,-1.)) ;
#130477=DIRECTION('ref_axis',(-1.,0.,0.)) ;
#130478=DIRECTION('center_axis',(0.,0.,1.)) ;
#130479=DIRECTION('ref_axis',(1.,0.,0.)) ;
#130480=DIRECTION('center_axis',(0.,-1.,0.)) ;
#130481=DIRECTION('ref_axis',(0.,0.,-1.)) ;
#130482=DIRECTION('center_axis',(0.,-1.,0.)) ;
#130483=DIRECTION('ref_axis',(0.,0.,-1.)) ;
#130484=DIRECTION('center_axis',(0.,1.,0.)) ;
#130485=DIRECTION('ref_axis',(1.,0.,0.)) ;
#130486=DIRECTION('center_axis',(-1.,0.,0.)) ;
#130487=DIRECTION('ref_axis',(0.,0.,-1.)) ;
#130488=DIRECTION('center_axis',(0.,1.,0.)) ;
#130489=DIRECTION('ref_axis',(1.,0.,0.)) ;
#130490=DIRECTION('center_axis',(-1.,0.,0.)) ;
#130491=DIRECTION('ref_axis',(0.,0.,-1.)) ;
#130492=DIRECTION('center_axis',(0.,-1.,0.)) ;
#130493=DIRECTION('ref_axis',(0.,0.,-1.)) ;
#130494=DIRECTION('center_axis',(0.,-1.,0.)) ;
#130495=DIRECTION('ref_axis',(0.,0.,-1.)) ;
#130496=DIRECTION('center_axis',(-1.,0.,0.)) ;
#130497=DIRECTION('ref_axis',(0.,0.,1.)) ;
#130498=DIRECTION('center_axis',(-1.,0.,0.)) ;
#130499=DIRECTION('ref_axis',(0.,0.,1.)) ;
#130500=DIRECTION('center_axis',(1.,0.,0.)) ;
#130501=DIRECTION('ref_axis',(0.,0.,-1.)) ;
#130502=DIRECTION('center_axis',(-1.,0.,0.)) ;
#130503=DIRECTION('ref_axis',(0.,0.,1.)) ;
#130504=DIRECTION('center_axis',(0.,-1.,0.)) ;
#130505=DIRECTION('ref_axis',(0.,0.,-1.)) ;
#130506=DIRECTION('center_axis',(0.,-1.,0.)) ;
#130507=DIRECTION('ref_axis',(0.,0.,-1.)) ;
#130508=DIRECTION('center_axis',(0.,1.,0.)) ;
#130509=DIRECTION('ref_axis',(1.,0.,0.)) ;
#130510=DIRECTION('center_axis',(0.,0.,-1.)) ;
#130511=DIRECTION('ref_axis',(1.,0.,0.)) ;
#130512=DIRECTION('center_axis',(0.,1.,0.)) ;
#130513=DIRECTION('ref_axis',(1.,0.,0.)) ;
#130514=DIRECTION('center_axis',(0.,0.,1.)) ;
#130515=DIRECTION('ref_axis',(-1.,0.,0.)) ;
#130516=DIRECTION('center_axis',(0.,0.,-1.)) ;
#130517=DIRECTION('ref_axis',(-1.,0.,0.)) ;
#130518=DIRECTION('center_axis',(1.,1.31418445149758E-16,-2.16840434497101E-16)) ;
#130519=DIRECTION('ref_axis',(-2.16840434497101E-16,-2.8496832747207E-32,
-1.)) ;
#130520=DIRECTION('center_axis',(1.,0.,0.)) ;
#130521=DIRECTION('ref_axis',(0.,0.,-1.)) ;
#130522=DIRECTION('center_axis',(-1.,0.,0.)) ;
#130523=DIRECTION('ref_axis',(0.,0.,1.)) ;
#130524=DIRECTION('center_axis',(-1.31418445149758E-16,1.,0.)) ;
#130525=DIRECTION('ref_axis',(-1.,0.,0.)) ;
#130526=DIRECTION('center_axis',(0.,0.,1.)) ;
#130527=DIRECTION('ref_axis',(-1.,0.,0.)) ;
#130528=DIRECTION('center_axis',(-1.31418445149758E-16,1.,0.)) ;
#130529=DIRECTION('ref_axis',(-1.,-1.31418445149758E-16,0.)) ;
#130530=DIRECTION('center_axis',(-1.31418445149758E-16,1.,0.)) ;
#130531=DIRECTION('ref_axis',(-1.,0.,0.)) ;
#130532=DIRECTION('center_axis',(-1.31418445149758E-16,1.,0.)) ;
#130533=DIRECTION('ref_axis',(-1.,-1.31418445149758E-16,0.)) ;
#130534=DIRECTION('center_axis',(0.,0.,1.)) ;
#130535=DIRECTION('ref_axis',(-1.,0.,0.)) ;
#130536=DIRECTION('center_axis',(-4.33680868994202E-16,-5.69936654944139E-32,
-1.)) ;
#130537=DIRECTION('ref_axis',(-1.,2.47170623787823E-47,4.33680868994202E-16)) ;
#130538=DIRECTION('center_axis',(0.,0.,1.)) ;
#130539=DIRECTION('ref_axis',(1.,0.,0.)) ;
#130540=DIRECTION('center_axis',(-1.31418445149758E-16,-1.,0.)) ;
#130541=DIRECTION('ref_axis',(1.,-1.31418445149758E-16,0.)) ;
#130542=DIRECTION('center_axis',(0.,1.,0.)) ;
#130543=DIRECTION('ref_axis',(0.,0.,1.)) ;
#130544=DIRECTION('center_axis',(-1.,0.,2.16840434497101E-16)) ;
#130545=DIRECTION('ref_axis',(2.16840434497101E-16,0.,1.)) ;
#130546=DIRECTION('center_axis',(-1.,0.,0.)) ;
#130547=DIRECTION('ref_axis',(0.,0.,1.)) ;
#130548=DIRECTION('center_axis',(1.,0.,0.)) ;
#130549=DIRECTION('ref_axis',(0.,0.,-1.)) ;
#130550=DIRECTION('center_axis',(-1.31418445149758E-16,-1.,0.)) ;
#130551=DIRECTION('ref_axis',(1.,-1.31418445149758E-16,0.)) ;
#130552=DIRECTION('center_axis',(0.,1.,0.)) ;
#130553=DIRECTION('ref_axis',(0.,0.,1.)) ;
#130554=DIRECTION('center_axis',(2.16840434497101E-16,2.8496832747207E-32,
1.)) ;
#130555=DIRECTION('ref_axis',(1.,-6.17926559469557E-48,-2.16840434497101E-16)) ;
#130556=DIRECTION('center_axis',(0.,0.,1.)) ;
#130557=DIRECTION('ref_axis',(1.,0.,0.)) ;
#130558=DIRECTION('center_axis',(-1.,-1.31418445149758E-16,-2.16840434497101E-16)) ;
#130559=DIRECTION('ref_axis',(-2.16840434497101E-16,-2.8496832747207E-32,
1.)) ;
#130560=DIRECTION('center_axis',(-1.,0.,0.)) ;
#130561=DIRECTION('ref_axis',(0.,0.,1.)) ;
#130562=DIRECTION('center_axis',(1.,0.,0.)) ;
#130563=DIRECTION('ref_axis',(0.,0.,-1.)) ;
#130564=DIRECTION('center_axis',(-1.31418445149758E-16,1.,0.)) ;
#130565=DIRECTION('ref_axis',(-1.,0.,0.)) ;
#130566=DIRECTION('center_axis',(-1.31418445149758E-16,1.,0.)) ;
#130567=DIRECTION('ref_axis',(-1.,-1.31418445149758E-16,0.)) ;
#130568=DIRECTION('center_axis',(0.,1.,0.)) ;
#130569=DIRECTION('ref_axis',(1.,0.,0.)) ;
#130570=DIRECTION('center_axis',(0.,0.,-1.)) ;
#130571=DIRECTION('ref_axis',(1.,0.,0.)) ;
#130572=DIRECTION('center_axis',(0.,1.,0.)) ;
#130573=DIRECTION('ref_axis',(1.,0.,0.)) ;
#130574=DIRECTION('center_axis',(0.,0.,-1.)) ;
#130575=DIRECTION('ref_axis',(1.,0.,0.)) ;
#130576=DIRECTION('center_axis',(-1.31418445149758E-16,1.,0.)) ;
#130577=DIRECTION('ref_axis',(-1.,0.,0.)) ;
#130578=DIRECTION('center_axis',(-1.31418445149758E-16,1.,0.)) ;
#130579=DIRECTION('ref_axis',(-1.,-1.31418445149758E-16,0.)) ;
#130580=DIRECTION('center_axis',(-1.31418445149758E-16,-1.,0.)) ;
#130581=DIRECTION('ref_axis',(1.,-1.31418445149758E-16,0.)) ;
#130582=DIRECTION('center_axis',(0.,1.,0.)) ;
#130583=DIRECTION('ref_axis',(0.,0.,1.)) ;
#130584=DIRECTION('center_axis',(4.33680868994202E-16,0.,1.)) ;
#130585=DIRECTION('ref_axis',(1.,0.,-4.33680868994202E-16)) ;
#130586=DIRECTION('center_axis',(0.,0.,-1.)) ;
#130587=DIRECTION('ref_axis',(-1.,0.,0.)) ;
#130588=DIRECTION('center_axis',(-2.16840434497101E-16,0.,-1.)) ;
#130589=DIRECTION('ref_axis',(-1.,0.,2.16840434497101E-16)) ;
#130590=DIRECTION('center_axis',(0.,0.,-1.)) ;
#130591=DIRECTION('ref_axis',(-1.,0.,0.)) ;
#130592=DIRECTION('center_axis',(-1.31418445149758E-16,-1.,0.)) ;
#130593=DIRECTION('ref_axis',(1.,-1.31418445149758E-16,0.)) ;
#130594=DIRECTION('center_axis',(0.,1.,0.)) ;
#130595=DIRECTION('ref_axis',(0.,0.,1.)) ;
#130596=DIRECTION('center_axis',(0.,1.,0.)) ;
#130597=DIRECTION('ref_axis',(1.,0.,0.)) ;
#130598=DIRECTION('center_axis',(-1.,0.,0.)) ;
#130599=DIRECTION('ref_axis',(0.,0.,-1.)) ;
#130600=DIRECTION('center_axis',(0.,1.,0.)) ;
#130601=DIRECTION('ref_axis',(1.,0.,0.)) ;
#130602=DIRECTION('center_axis',(1.,0.,0.)) ;
#130603=DIRECTION('ref_axis',(0.,0.,1.)) ;
#130604=DIRECTION('center_axis',(1.,0.,2.16840434497101E-16)) ;
#130605=DIRECTION('ref_axis',(2.16840434497101E-16,0.,-1.)) ;
#130606=DIRECTION('center_axis',(0.,1.,0.)) ;
#130607=DIRECTION('ref_axis',(0.,0.,1.)) ;
#130608=DIRECTION('center_axis',(0.,1.,0.)) ;
#130609=DIRECTION('ref_axis',(0.,0.,1.)) ;
#130610=DIRECTION('center_axis',(0.,0.,-1.)) ;
#130611=DIRECTION('ref_axis',(-1.,0.,0.)) ;
#130612=DIRECTION('center_axis',(0.,0.,1.)) ;
#130613=DIRECTION('ref_axis',(1.,0.,0.)) ;
#130614=DIRECTION('center_axis',(0.,0.,-1.)) ;
#130615=DIRECTION('ref_axis',(-1.,0.,0.)) ;
#130616=DIRECTION('center_axis',(0.,1.,0.)) ;
#130617=DIRECTION('ref_axis',(0.,0.,1.)) ;
#130618=DIRECTION('center_axis',(0.,1.,0.)) ;
#130619=DIRECTION('ref_axis',(0.,0.,1.)) ;
#130620=DIRECTION('center_axis',(0.,1.,0.)) ;
#130621=DIRECTION('ref_axis',(1.,0.,0.)) ;
#130622=DIRECTION('center_axis',(-1.,0.,0.)) ;
#130623=DIRECTION('ref_axis',(0.,0.,-1.)) ;
#130624=DIRECTION('center_axis',(0.,1.,0.)) ;
#130625=DIRECTION('ref_axis',(1.,0.,0.)) ;
#130626=DIRECTION('center_axis',(-1.,0.,0.)) ;
#130627=DIRECTION('ref_axis',(0.,0.,-1.)) ;
#130628=DIRECTION('center_axis',(0.,1.,0.)) ;
#130629=DIRECTION('ref_axis',(0.,0.,1.)) ;
#130630=DIRECTION('center_axis',(0.,1.,0.)) ;
#130631=DIRECTION('ref_axis',(0.,0.,1.)) ;
#130632=DIRECTION('center_axis',(-1.,0.,0.)) ;
#130633=DIRECTION('ref_axis',(0.,0.,1.)) ;
#130634=DIRECTION('center_axis',(-1.,0.,0.)) ;
#130635=DIRECTION('ref_axis',(0.,0.,1.)) ;
#130636=DIRECTION('center_axis',(1.,0.,0.)) ;
#130637=DIRECTION('ref_axis',(0.,0.,-1.)) ;
#130638=DIRECTION('center_axis',(-1.,0.,0.)) ;
#130639=DIRECTION('ref_axis',(0.,0.,1.)) ;
#130640=DIRECTION('center_axis',(0.,1.,0.)) ;
#130641=DIRECTION('ref_axis',(0.,0.,1.)) ;
#130642=DIRECTION('center_axis',(0.,1.,0.)) ;
#130643=DIRECTION('ref_axis',(0.,0.,1.)) ;
#130644=DIRECTION('center_axis',(0.,1.,0.)) ;
#130645=DIRECTION('ref_axis',(1.,0.,0.)) ;
#130646=DIRECTION('center_axis',(0.,0.,1.)) ;
#130647=DIRECTION('ref_axis',(-1.,0.,0.)) ;
#130648=DIRECTION('center_axis',(0.,1.,0.)) ;
#130649=DIRECTION('ref_axis',(1.,0.,0.)) ;
#130650=DIRECTION('center_axis',(0.,0.,-1.)) ;
#130651=DIRECTION('ref_axis',(1.,0.,0.)) ;
#130652=DIRECTION('center_axis',(0.,0.,1.)) ;
#130653=DIRECTION('ref_axis',(1.,0.,0.)) ;
#130654=DIRECTION('center_axis',(0.,0.,1.)) ;
#130655=DIRECTION('ref_axis',(1.,0.,0.)) ;
#130656=DIRECTION('center_axis',(0.,0.,-1.)) ;
#130657=DIRECTION('ref_axis',(-1.,0.,0.)) ;
#130658=DIRECTION('center_axis',(-3.46944695195361E-14,0.,1.)) ;
#130659=DIRECTION('ref_axis',(1.,0.,3.46944695195361E-14)) ;
#130660=DIRECTION('center_axis',(1.,0.,0.)) ;
#130661=DIRECTION('ref_axis',(0.,0.,-1.)) ;
#130662=DIRECTION('center_axis',(1.,0.,0.)) ;
#130663=DIRECTION('ref_axis',(0.,0.,-1.)) ;
#130664=DIRECTION('center_axis',(1.,0.,0.)) ;
#130665=DIRECTION('ref_axis',(0.,0.,-1.)) ;
#130666=DIRECTION('center_axis',(1.,0.,8.67361737988409E-15)) ;
#130667=DIRECTION('ref_axis',(8.67361737988409E-15,0.,-1.)) ;
#130668=DIRECTION('center_axis',(1.,0.,0.)) ;
#130669=DIRECTION('ref_axis',(0.,0.,-1.)) ;
#130670=DIRECTION('center_axis',(1.,0.,1.73472347597682E-14)) ;
#130671=DIRECTION('ref_axis',(1.73472347597682E-14,0.,-1.)) ;
#130672=DIRECTION('center_axis',(-1.,0.,0.)) ;
#130673=DIRECTION('ref_axis',(0.,0.,1.)) ;
#130674=DIRECTION('center_axis',(1.,0.,0.)) ;
#130675=DIRECTION('ref_axis',(0.,0.,-1.)) ;
#130676=DIRECTION('center_axis',(1.,0.,0.)) ;
#130677=DIRECTION('ref_axis',(0.,0.,-1.)) ;
#130678=DIRECTION('center_axis',(-3.46944695195364E-14,0.,-1.)) ;
#130679=DIRECTION('ref_axis',(-1.,0.,3.46944695195364E-14)) ;
#130680=DIRECTION('center_axis',(1.,0.,0.)) ;
#130681=DIRECTION('ref_axis',(0.,0.,-1.)) ;
#130682=DIRECTION('center_axis',(-3.46944695195364E-14,0.,1.)) ;
#130683=DIRECTION('ref_axis',(1.,0.,3.46944695195364E-14)) ;
#130684=DIRECTION('center_axis',(0.,0.,-1.)) ;
#130685=DIRECTION('ref_axis',(-1.,0.,0.)) ;
#130686=DIRECTION('center_axis',(-0.422618261740697,5.55398348498559E-17,
0.906307787036651)) ;
#130687=DIRECTION('ref_axis',(0.906307787036651,6.51773046476477E-31,0.422618261740697)) ;
#130688=DIRECTION('center_axis',(0.422618261740697,-5.55398348498559E-17,
-0.906307787036651)) ;
#130689=DIRECTION('ref_axis',(-0.906307787036651,-6.46086972436398E-31,
-0.422618261740697)) ;
#130690=DIRECTION('center_axis',(-0.422618261740697,5.55398348498559E-17,
0.906307787036651)) ;
#130691=DIRECTION('ref_axis',(0.906307787036651,6.46086972436398E-31,0.422618261740697)) ;
#130692=DIRECTION('center_axis',(0.422618261740697,-5.55398348498559E-17,
-0.906307787036651)) ;
#130693=DIRECTION('ref_axis',(-0.906307787036651,-6.46086972436398E-31,
-0.422618261740697)) ;
#130694=DIRECTION('center_axis',(0.,1.,0.)) ;
#130695=DIRECTION('ref_axis',(1.,0.,0.)) ;
#130696=DIRECTION('center_axis',(3.4216004848576E-14,0.514231796959095,
-0.857651245551606)) ;
#130697=DIRECTION('ref_axis',(3.46944695195362E-14,-0.857651245551606,-0.514231796959095)) ;
#130698=DIRECTION('center_axis',(0.,-3.46944695195362E-14,1.)) ;
#130699=DIRECTION('ref_axis',(0.,1.,3.46944695195362E-14)) ;
#130700=DIRECTION('center_axis',(-1.,0.,0.)) ;
#130701=DIRECTION('ref_axis',(0.,-4.33680868994204E-15,-1.)) ;
#130702=DIRECTION('center_axis',(0.,0.,1.)) ;
#130703=DIRECTION('ref_axis',(1.,0.,0.)) ;
#130704=DIRECTION('center_axis',(0.,0.,1.)) ;
#130705=DIRECTION('ref_axis',(1.,0.,0.)) ;
#130706=DIRECTION('center_axis',(-1.,0.,0.)) ;
#130707=DIRECTION('ref_axis',(0.,0.,1.)) ;
#130708=DIRECTION('center_axis',(-1.,0.,0.)) ;
#130709=DIRECTION('ref_axis',(0.,-4.33680868994204E-15,-1.)) ;
#130710=DIRECTION('center_axis',(1.,0.,0.)) ;
#130711=DIRECTION('ref_axis',(0.,0.,-1.)) ;
#130712=DIRECTION('center_axis',(0.,-0.514231796959124,-0.857651245551588)) ;
#130713=DIRECTION('ref_axis',(0.,0.857651245551588,-0.514231796959124)) ;
#130714=DIRECTION('center_axis',(0.,1.,8.97270763436279E-17)) ;
#130715=DIRECTION('ref_axis',(0.,-8.97270763436279E-17,1.)) ;
#130716=DIRECTION('center_axis',(0.,-1.,-8.97270763436279E-17)) ;
#130717=DIRECTION('ref_axis',(0.,-8.97270763436279E-17,1.)) ;
#130718=DIRECTION('center_axis',(0.,-1.,0.)) ;
#130719=DIRECTION('ref_axis',(0.,0.,-1.)) ;
#130720=DIRECTION('center_axis',(0.,1.,0.)) ;
#130721=DIRECTION('ref_axis',(1.,0.,0.)) ;
#130722=DIRECTION('center_axis',(-1.,0.,0.)) ;
#130723=DIRECTION('ref_axis',(0.,0.,-1.)) ;
#130724=DIRECTION('center_axis',(1.,0.,0.)) ;
#130725=DIRECTION('ref_axis',(0.,0.,-1.)) ;
#130726=DIRECTION('center_axis',(0.,-0.514231796959093,0.857651245551607)) ;
#130727=DIRECTION('ref_axis',(0.,0.857651245551607,0.514231796959093)) ;
#130728=DIRECTION('center_axis',(0.,0.,-1.)) ;
#130729=DIRECTION('ref_axis',(1.,0.,0.)) ;
#130730=DIRECTION('center_axis',(0.,1.,0.)) ;
#130731=DIRECTION('ref_axis',(1.,0.,0.)) ;
#130732=DIRECTION('center_axis',(-6.93889390390727E-14,0.,-1.)) ;
#130733=DIRECTION('ref_axis',(1.,0.,-6.93889390390727E-14)) ;
#130734=DIRECTION('center_axis',(-1.,0.,0.)) ;
#130735=DIRECTION('ref_axis',(0.,-3.03576608295933E-14,-1.)) ;
#130736=DIRECTION('center_axis',(0.,0.,-1.)) ;
#130737=DIRECTION('ref_axis',(-1.,0.,0.)) ;
#130738=DIRECTION('center_axis',(0.,0.,1.)) ;
#130739=DIRECTION('ref_axis',(-1.,0.,0.)) ;
#130740=DIRECTION('center_axis',(0.,0.,-1.)) ;
#130741=DIRECTION('ref_axis',(-1.,0.,0.)) ;
#130742=DIRECTION('center_axis',(-1.,0.,7.01133629567814E-33)) ;
#130743=DIRECTION('ref_axis',(7.01133629567814E-33,0.,1.)) ;
#130744=DIRECTION('center_axis',(-1.,0.,0.)) ;
#130745=DIRECTION('ref_axis',(0.,0.,1.)) ;
#130746=DIRECTION('center_axis',(0.,0.,-1.)) ;
#130747=DIRECTION('ref_axis',(-1.,0.,0.)) ;
#130748=DIRECTION('center_axis',(-7.01133629567814E-33,8.97270763436279E-17,
-1.)) ;
#130749=DIRECTION('ref_axis',(6.29106707073161E-49,1.,8.97270763436279E-17)) ;
#130750=DIRECTION('center_axis',(1.,0.,0.)) ;
#130751=DIRECTION('ref_axis',(0.,0.,-1.)) ;
#130752=DIRECTION('center_axis',(6.69037477709045E-15,0.51423179695912,
0.85765124555159)) ;
#130753=DIRECTION('ref_axis',(-4.49049578447409E-29,-0.85765124555159,0.51423179695912)) ;
#130754=DIRECTION('center_axis',(-1.,0.,0.)) ;
#130755=DIRECTION('ref_axis',(0.,0.,1.)) ;
#130756=DIRECTION('center_axis',(-1.,0.,0.)) ;
#130757=DIRECTION('ref_axis',(0.,2.60208521396514E-14,-1.)) ;
#130758=DIRECTION('center_axis',(0.,0.,1.)) ;
#130759=DIRECTION('ref_axis',(1.,0.,0.)) ;
#130760=DIRECTION('center_axis',(0.,0.,-1.)) ;
#130761=DIRECTION('ref_axis',(-1.,0.,0.)) ;
#130762=DIRECTION('center_axis',(0.,-1.,8.97270763436279E-17)) ;
#130763=DIRECTION('ref_axis',(0.,-8.97270763436279E-17,-1.)) ;
#130764=DIRECTION('center_axis',(0.,-1.,8.97270763436279E-17)) ;
#130765=DIRECTION('ref_axis',(0.,-8.97270763436279E-17,-1.)) ;
#130766=DIRECTION('center_axis',(0.,-1.,0.)) ;
#130767=DIRECTION('ref_axis',(0.,0.,-1.)) ;
#130768=DIRECTION('center_axis',(-7.01133629567814E-33,8.97270763436279E-17,
-1.)) ;
#130769=DIRECTION('ref_axis',(0.,1.,0.)) ;
#130770=DIRECTION('center_axis',(0.,-1.,0.)) ;
#130771=DIRECTION('ref_axis',(0.,0.,1.)) ;
#130772=DIRECTION('center_axis',(1.,0.,0.)) ;
#130773=DIRECTION('ref_axis',(0.,0.,-1.)) ;
#130774=DIRECTION('center_axis',(0.,0.,1.)) ;
#130775=DIRECTION('ref_axis',(-1.,0.,0.)) ;
#130776=DIRECTION('center_axis',(0.,1.,0.)) ;
#130777=DIRECTION('ref_axis',(1.,0.,0.)) ;
#130778=DIRECTION('center_axis',(-1.,0.,0.)) ;
#130779=DIRECTION('ref_axis',(0.,0.,-1.)) ;
#130780=DIRECTION('center_axis',(1.,7.81406971160724E-17,0.)) ;
#130781=DIRECTION('ref_axis',(-7.81406971160724E-17,1.,0.)) ;
#130782=DIRECTION('center_axis',(1.,0.,0.)) ;
#130783=DIRECTION('ref_axis',(0.,0.,-1.)) ;
#130784=DIRECTION('center_axis',(1.,0.,0.)) ;
#130785=DIRECTION('ref_axis',(0.,0.,-1.)) ;
#130786=DIRECTION('center_axis',(0.,1.,8.97270763436279E-17)) ;
#130787=DIRECTION('ref_axis',(0.,-8.97270763436279E-17,1.)) ;
#130788=DIRECTION('center_axis',(0.,-1.,0.)) ;
#130789=DIRECTION('ref_axis',(0.,0.,-1.)) ;
#130790=DIRECTION('center_axis',(0.,0.,-1.)) ;
#130791=DIRECTION('ref_axis',(-1.,0.,0.)) ;
#130792=DIRECTION('center_axis',(-7.01133629567814E-33,8.97270763436279E-17,
1.)) ;
#130793=DIRECTION('ref_axis',(-6.29106707073161E-49,-1.,8.97270763436279E-17)) ;
#130794=DIRECTION('center_axis',(-1.,0.,-7.01133629567814E-33)) ;
#130795=DIRECTION('ref_axis',(-7.01133629567814E-33,0.,1.)) ;
#130796=DIRECTION('center_axis',(-1.,0.,0.)) ;
#130797=DIRECTION('ref_axis',(0.,0.,1.)) ;
#130798=DIRECTION('center_axis',(1.,0.,0.)) ;
#130799=DIRECTION('ref_axis',(0.,1.,0.)) ;
#130800=DIRECTION('center_axis',(0.,1.,0.)) ;
#130801=DIRECTION('ref_axis',(0.,0.,1.)) ;
#130802=DIRECTION('center_axis',(0.,1.,0.)) ;
#130803=DIRECTION('ref_axis',(1.,0.,0.)) ;
#130804=DIRECTION('center_axis',(0.,0.,-1.)) ;
#130805=DIRECTION('ref_axis',(1.,0.,0.)) ;
#130806=DIRECTION('center_axis',(-1.,0.,0.)) ;
#130807=DIRECTION('ref_axis',(0.,0.,-1.)) ;
#130808=DIRECTION('center_axis',(-7.01133629567814E-33,8.97270763436279E-17,
1.)) ;
#130809=DIRECTION('ref_axis',(0.,-1.,0.)) ;
#130810=DIRECTION('center_axis',(0.,-1.,0.)) ;
#130811=DIRECTION('ref_axis',(0.,0.,1.)) ;
#130812=DIRECTION('center_axis',(7.81406971160724E-17,-1.,-8.97270763436279E-17)) ;
#130813=DIRECTION('ref_axis',(-7.01133629567814E-33,8.97270763436279E-17,
-1.)) ;
#130814=DIRECTION('center_axis',(0.,1.,0.)) ;
#130815=DIRECTION('ref_axis',(0.,0.,1.)) ;
#130816=DIRECTION('center_axis',(-1.,-7.81406971160724E-17,0.)) ;
#130817=DIRECTION('ref_axis',(7.81406971160724E-17,-1.,0.)) ;
#130818=DIRECTION('center_axis',(-1.,-7.81406971160724E-17,0.)) ;
#130819=DIRECTION('ref_axis',(-7.81406971160724E-17,1.,0.)) ;
#130820=DIRECTION('center_axis',(0.,0.,1.)) ;
#130821=DIRECTION('ref_axis',(1.,0.,0.)) ;
#130822=DIRECTION('center_axis',(0.,0.,-1.)) ;
#130823=DIRECTION('ref_axis',(-1.,0.,0.)) ;
#130824=DIRECTION('center_axis',(0.,-1.,8.97270763436279E-17)) ;
#130825=DIRECTION('ref_axis',(0.,-8.97270763436279E-17,-1.)) ;
#130826=DIRECTION('center_axis',(0.,-1.,0.)) ;
#130827=DIRECTION('ref_axis',(0.,0.,-1.)) ;
#130828=DIRECTION('center_axis',(1.,7.81406971160724E-17,0.)) ;
#130829=DIRECTION('ref_axis',(0.,1.,0.)) ;
#130830=DIRECTION('center_axis',(0.,0.,1.)) ;
#130831=DIRECTION('ref_axis',(-1.,0.,0.)) ;
#130832=DIRECTION('center_axis',(0.,1.,0.)) ;
#130833=DIRECTION('ref_axis',(1.,0.,0.)) ;
#130834=DIRECTION('center_axis',(-1.,0.,0.)) ;
#130835=DIRECTION('ref_axis',(0.,0.,-1.)) ;
#130836=DIRECTION('center_axis',(0.,0.,-1.)) ;
#130837=DIRECTION('ref_axis',(-1.,0.,0.)) ;
#130838=DIRECTION('center_axis',(0.,0.,1.)) ;
#130839=DIRECTION('ref_axis',(1.,0.,0.)) ;
#130840=DIRECTION('center_axis',(-1.,-7.81406971160724E-17,0.)) ;
#130841=DIRECTION('ref_axis',(7.81406971160724E-17,-1.,0.)) ;
#130842=DIRECTION('center_axis',(-1.,-7.81406971160724E-17,0.)) ;
#130843=DIRECTION('ref_axis',(-7.81406971160724E-17,1.,0.)) ;
#130844=DIRECTION('center_axis',(1.,7.81406971160724E-17,0.)) ;
#130845=DIRECTION('ref_axis',(-7.81406971160724E-17,1.,0.)) ;
#130846=DIRECTION('center_axis',(1.,0.,0.)) ;
#130847=DIRECTION('ref_axis',(0.,0.,-1.)) ;
#130848=DIRECTION('center_axis',(1.,0.,0.)) ;
#130849=DIRECTION('ref_axis',(0.,0.,-1.)) ;
#130850=DIRECTION('center_axis',(3.78638272950961E-32,-4.8455963016112E-16,
-1.)) ;
#130851=DIRECTION('ref_axis',(1.83472821505963E-47,1.,-4.8455963016112E-16)) ;
#130852=DIRECTION('center_axis',(3.78638272950961E-32,-4.8455963016112E-16,
-1.)) ;
#130853=DIRECTION('ref_axis',(1.83472821505963E-47,1.,-4.8455963016112E-16)) ;
#130854=DIRECTION('center_axis',(0.,0.,-1.)) ;
#130855=DIRECTION('ref_axis',(-1.,0.,0.)) ;
#130856=DIRECTION('center_axis',(1.,7.81406971160724E-17,0.)) ;
#130857=DIRECTION('ref_axis',(0.,1.,0.)) ;
#130858=DIRECTION('center_axis',(0.,-1.,0.)) ;
#130859=DIRECTION('ref_axis',(0.,0.,1.)) ;
#130860=DIRECTION('center_axis',(0.,1.,0.)) ;
#130861=DIRECTION('ref_axis',(1.,0.,0.)) ;
#130862=DIRECTION('center_axis',(0.,1.,0.)) ;
#130863=DIRECTION('ref_axis',(0.,0.,-1.)) ;
#130864=DIRECTION('center_axis',(-7.81406971160724E-17,1.,-8.97270763436279E-17)) ;
#130865=DIRECTION('ref_axis',(-7.01133629567814E-33,8.97270763436279E-17,
1.)) ;
#130866=DIRECTION('center_axis',(0.,-1.,0.)) ;
#130867=DIRECTION('ref_axis',(0.,0.,-1.)) ;
#130868=DIRECTION('center_axis',(0.,1.,0.)) ;
#130869=DIRECTION('ref_axis',(0.,0.,1.)) ;
#130870=DIRECTION('center_axis',(0.,-1.,0.)) ;
#130871=DIRECTION('ref_axis',(0.,0.,-1.)) ;
#130872=DIRECTION('center_axis',(0.,-1.,0.)) ;
#130873=DIRECTION('ref_axis',(0.,0.,-1.)) ;
#130874=DIRECTION('center_axis',(0.,1.,0.)) ;
#130875=DIRECTION('ref_axis',(1.,0.,0.)) ;
#130876=DIRECTION('center_axis',(0.,0.,1.)) ;
#130877=DIRECTION('ref_axis',(-1.,0.,0.)) ;
#130878=DIRECTION('center_axis',(1.,0.,0.)) ;
#130879=DIRECTION('ref_axis',(0.,0.,1.)) ;
#130880=DIRECTION('center_axis',(0.,-1.,0.)) ;
#130881=DIRECTION('ref_axis',(0.,0.,-1.)) ;
#130882=DIRECTION('center_axis',(0.,1.,0.)) ;
#130883=DIRECTION('ref_axis',(0.,0.,1.)) ;
#130884=DIRECTION('center_axis',(0.,-1.,0.)) ;
#130885=DIRECTION('ref_axis',(0.,0.,-1.)) ;
#130886=DIRECTION('center_axis',(-1.,0.,2.16840434497101E-16)) ;
#130887=DIRECTION('ref_axis',(2.16840434497101E-16,0.,1.)) ;
#130888=DIRECTION('center_axis',(1.,0.,0.)) ;
#130889=DIRECTION('ref_axis',(0.,0.,-1.)) ;
#130890=DIRECTION('center_axis',(-2.16840434497101E-16,0.,1.)) ;
#130891=DIRECTION('ref_axis',(1.,0.,2.16840434497101E-16)) ;
#130892=DIRECTION('center_axis',(0.,0.,1.)) ;
#130893=DIRECTION('ref_axis',(1.,0.,0.)) ;
#130894=DIRECTION('center_axis',(0.,1.,0.)) ;
#130895=DIRECTION('ref_axis',(0.,0.,1.)) ;
#130896=DIRECTION('center_axis',(0.,-1.,0.)) ;
#130897=DIRECTION('ref_axis',(0.,0.,-1.)) ;
#130898=DIRECTION('center_axis',(0.,1.,0.)) ;
#130899=DIRECTION('ref_axis',(1.,0.,0.)) ;
#130900=DIRECTION('center_axis',(0.,0.,1.)) ;
#130901=DIRECTION('ref_axis',(-1.,0.,0.)) ;
#130902=DIRECTION('center_axis',(0.,1.,0.)) ;
#130903=DIRECTION('ref_axis',(1.,0.,0.)) ;
#130904=DIRECTION('center_axis',(1.,0.,0.)) ;
#130905=DIRECTION('ref_axis',(0.,0.,1.)) ;
#130906=DIRECTION('center_axis',(0.,0.,-1.)) ;
#130907=DIRECTION('ref_axis',(-1.,0.,0.)) ;
#130908=DIRECTION('center_axis',(0.,0.,1.)) ;
#130909=DIRECTION('ref_axis',(1.,0.,0.)) ;
#130910=DIRECTION('center_axis',(1.,0.,2.16840434497101E-16)) ;
#130911=DIRECTION('ref_axis',(2.16840434497101E-16,0.,-1.)) ;
#130912=DIRECTION('center_axis',(1.,0.,0.)) ;
#130913=DIRECTION('ref_axis',(0.,0.,-1.)) ;
#130914=DIRECTION('center_axis',(0.,1.,0.)) ;
#130915=DIRECTION('ref_axis',(1.,0.,0.)) ;
#130916=DIRECTION('center_axis',(0.,1.,0.)) ;
#130917=DIRECTION('ref_axis',(0.,0.,-1.)) ;
#130918=DIRECTION('center_axis',(0.,1.,0.)) ;
#130919=DIRECTION('ref_axis',(0.,0.,1.)) ;
#130920=DIRECTION('center_axis',(0.,1.,0.)) ;
#130921=DIRECTION('ref_axis',(0.,0.,1.)) ;
#130922=DIRECTION('center_axis',(-0.942809041582063,-0.235702260395516,
0.235702260395518)) ;
#130923=DIRECTION('ref_axis',(0.242535625036335,4.64743530723282E-16,0.970142500145331)) ;
#130924=DIRECTION('center_axis',(-0.970142500145332,-0.242535625036331,
-2.10366121255617E-15)) ;
#130925=DIRECTION('ref_axis',(0.242535625036331,-0.970142500145332,-4.47980524894761E-30)) ;
#130926=DIRECTION('center_axis',(0.970142500145333,0.24253562503633,0.)) ;
#130927=DIRECTION('ref_axis',(-0.24253562503633,0.970142500145333,0.)) ;
#130928=DIRECTION('center_axis',(-0.970142500145332,-0.242535625036331,
2.73475957632304E-14)) ;
#130929=DIRECTION('ref_axis',(0.242535625036331,-0.970142500145332,1.1454669517322E-30)) ;
#130930=DIRECTION('center_axis',(0.879462917689188,0.219865729422294,-0.42214220049081)) ;
#130931=DIRECTION('ref_axis',(-0.432731067584771,1.71515946658E-16,-0.901523057468274)) ;
#130932=DIRECTION('center_axis',(0.879462917689192,0.219865729422271,-0.422142200490814)) ;
#130933=DIRECTION('ref_axis',(-0.432731067584773,-1.62351711522009E-16,
-0.901523057468273)) ;
#130934=DIRECTION('center_axis',(0.,1.,0.)) ;
#130935=DIRECTION('ref_axis',(1.,0.,0.)) ;
#130936=DIRECTION('center_axis',(0.,-1.,0.)) ;
#130937=DIRECTION('ref_axis',(0.,0.,1.)) ;
#130938=DIRECTION('center_axis',(0.,-1.,0.)) ;
#130939=DIRECTION('ref_axis',(0.,0.,-1.)) ;
#130940=DIRECTION('center_axis',(-4.51750905202295E-15,-1.,2.16840434497102E-15)) ;
#130941=DIRECTION('ref_axis',(1.,-4.51750905202295E-15,3.91831450274151E-31)) ;
#130942=DIRECTION('center_axis',(0.669589480006976,-0.669589480006974,-0.321402950403349)) ;
#130943=DIRECTION('ref_axis',(0.707106781186547,0.707106781186548,5.45170614306381E-16)) ;
#130944=DIRECTION('center_axis',(0.669589480006977,-0.669589480006977,-0.321402950403342)) ;
#130945=DIRECTION('ref_axis',(0.707106781186547,0.707106781186548,-1.94221176494188E-16)) ;
#130946=DIRECTION('center_axis',(0.,1.,0.)) ;
#130947=DIRECTION('ref_axis',(1.,0.,0.)) ;
#130948=DIRECTION('center_axis',(0.707106781186541,-0.707106781186554,0.)) ;
#130949=DIRECTION('ref_axis',(-0.707106781186554,-0.707106781186541,0.)) ;
#130950=DIRECTION('center_axis',(0.707106781186549,-0.707106781186546,0.)) ;
#130951=DIRECTION('ref_axis',(0.707106781186546,0.707106781186549,0.)) ;
#130952=DIRECTION('center_axis',(0.707106781186548,-0.707106781186548,-1.53329341668338E-15)) ;
#130953=DIRECTION('ref_axis',(0.707106781186548,0.707106781186548,1.5356898865553E-31)) ;
#130954=DIRECTION('center_axis',(0.577350269189633,-0.577350269189633,-0.577350269189612)) ;
#130955=DIRECTION('ref_axis',(0.707106781186548,0.707106781186548,1.34560831514457E-17)) ;
#130956=DIRECTION('center_axis',(-0.577350269189328,0.577350269189571,-0.577350269189978)) ;
#130957=DIRECTION('ref_axis',(-7.61554280732519E-15,0.707106781186793,0.707106781186302)) ;
#130958=DIRECTION('center_axis',(-0.707106781186548,0.707106781186548,7.66646708341718E-15)) ;
#130959=DIRECTION('ref_axis',(-0.707106781186548,-0.707106781186548,3.27987112860885E-31)) ;
#130960=DIRECTION('center_axis',(-0.707106781186549,0.707106781186546,0.)) ;
#130961=DIRECTION('ref_axis',(-0.707106781186546,-0.707106781186549,0.)) ;
#130962=DIRECTION('center_axis',(-0.707106781186548,0.707106781186548,-1.13463712834566E-13)) ;
#130963=DIRECTION('ref_axis',(-0.707106781186548,-0.707106781186548,1.81538773348134E-28)) ;
#130964=DIRECTION('center_axis',(-0.669589480006976,0.669589480006974,-0.321402950403349)) ;
#130965=DIRECTION('ref_axis',(-0.707106781186547,-0.707106781186548,5.45170614306381E-16)) ;
#130966=DIRECTION('center_axis',(0.66958948000704,-0.669589480006895,0.32140295040338)) ;
#130967=DIRECTION('ref_axis',(0.707106781186471,0.707106781186624,1.36895061126305E-16)) ;
#130968=DIRECTION('center_axis',(0.,1.,0.)) ;
#130969=DIRECTION('ref_axis',(1.,0.,0.)) ;
#130970=DIRECTION('center_axis',(-1.50329234996253E-14,1.,0.)) ;
#130971=DIRECTION('ref_axis',(1.,1.50329234996253E-14,0.)) ;
#130972=DIRECTION('center_axis',(0.,-1.,0.)) ;
#130973=DIRECTION('ref_axis',(0.,0.,-1.)) ;
#130974=DIRECTION('center_axis',(0.,1.,0.)) ;
#130975=DIRECTION('ref_axis',(0.,0.,1.)) ;
#130976=DIRECTION('center_axis',(-0.879462917689188,-0.219865729422294,
-0.42214220049081)) ;
#130977=DIRECTION('ref_axis',(-0.432731067584771,1.71515946658E-16,0.901523057468274)) ;
#130978=DIRECTION('center_axis',(0.879462917689201,0.219865729422298,0.42214220049078)) ;
#130979=DIRECTION('ref_axis',(0.432731067584741,-2.36820597908546E-15,-0.901523057468288)) ;
#130980=DIRECTION('center_axis',(0.,1.,0.)) ;
#130981=DIRECTION('ref_axis',(1.,0.,0.)) ;
#130982=DIRECTION('center_axis',(0.970142500145323,0.242535625036368,0.)) ;
#130983=DIRECTION('ref_axis',(0.242535625036368,-0.970142500145323,0.)) ;
#130984=DIRECTION('center_axis',(-0.970142500145333,-0.24253562503633,0.)) ;
#130985=DIRECTION('ref_axis',(0.24253562503633,-0.970142500145333,0.)) ;
#130986=DIRECTION('center_axis',(0.970142500145333,0.242535625036331,-2.1036612125561E-15)) ;
#130987=DIRECTION('ref_axis',(-0.242535625036331,0.970142500145332,-1.06801962627779E-30)) ;
#130988=DIRECTION('center_axis',(0.942809041582058,0.235702260395512,0.23570226039554)) ;
#130989=DIRECTION('ref_axis',(0.242535625036358,-1.84667126758454E-15,-0.970142500145326)) ;
#130990=DIRECTION('center_axis',(0.,-1.,0.)) ;
#130991=DIRECTION('ref_axis',(0.,0.,-1.)) ;
#130992=DIRECTION('center_axis',(-1.,0.,-8.67361737988409E-15)) ;
#130993=DIRECTION('ref_axis',(-8.67361737988409E-15,0.,1.)) ;
#130994=DIRECTION('center_axis',(0.,0.,-1.)) ;
#130995=DIRECTION('ref_axis',(-1.,0.,0.)) ;
#130996=DIRECTION('center_axis',(0.,0.,-1.)) ;
#130997=DIRECTION('ref_axis',(-1.,0.,0.)) ;
#130998=DIRECTION('center_axis',(0.,3.46944695195362E-14,-1.)) ;
#130999=DIRECTION('ref_axis',(0.,1.,3.46944695195362E-14)) ;
#131000=DIRECTION('center_axis',(1.,0.,0.)) ;
#131001=DIRECTION('ref_axis',(0.,0.,-1.)) ;
#131002=DIRECTION('center_axis',(-1.,0.,0.)) ;
#131003=DIRECTION('ref_axis',(0.,0.,1.)) ;
#131004=DIRECTION('center_axis',(0.,-1.,0.)) ;
#131005=DIRECTION('ref_axis',(0.,0.,-1.)) ;
#131006=DIRECTION('center_axis',(-1.,0.,0.)) ;
#131007=DIRECTION('ref_axis',(0.,0.,1.)) ;
#131008=DIRECTION('center_axis',(0.,-1.,0.)) ;
#131009=DIRECTION('ref_axis',(0.,0.,-1.)) ;
#131010=DIRECTION('center_axis',(3.46944695195358E-14,0.,-1.)) ;
#131011=DIRECTION('ref_axis',(-1.,0.,-3.46944695195358E-14)) ;
#131012=DIRECTION('center_axis',(-1.,0.,0.)) ;
#131013=DIRECTION('ref_axis',(0.,0.,1.)) ;
#131014=DIRECTION('center_axis',(-1.,1.73472347597681E-14,0.)) ;
#131015=DIRECTION('ref_axis',(-1.73472347597681E-14,-1.,0.)) ;
#131016=DIRECTION('center_axis',(0.,0.,1.)) ;
#131017=DIRECTION('ref_axis',(1.,0.,0.)) ;
#131018=DIRECTION('center_axis',(-3.46944695195364E-14,0.,-1.)) ;
#131019=DIRECTION('ref_axis',(-1.,0.,3.46944695195364E-14)) ;
#131020=DIRECTION('center_axis',(0.,-1.,0.)) ;
#131021=DIRECTION('ref_axis',(0.,0.,-1.)) ;
#131022=DIRECTION('center_axis',(0.,-1.,0.)) ;
#131023=DIRECTION('ref_axis',(0.,0.,-1.)) ;
#131024=DIRECTION('center_axis',(0.,-1.,0.)) ;
#131025=DIRECTION('ref_axis',(0.,0.,-1.)) ;
#131026=DIRECTION('center_axis',(0.,0.,1.)) ;
#131027=DIRECTION('ref_axis',(1.,0.,0.)) ;
#131028=DIRECTION('center_axis',(0.,0.,-1.)) ;
#131029=DIRECTION('ref_axis',(-1.,0.,0.)) ;
#131030=DIRECTION('center_axis',(0.,0.,1.)) ;
#131031=DIRECTION('ref_axis',(1.,0.,0.)) ;
#131032=DIRECTION('center_axis',(0.,-1.,0.)) ;
#131033=DIRECTION('ref_axis',(0.,0.,-1.)) ;
#131034=DIRECTION('center_axis',(0.,-1.,0.)) ;
#131035=DIRECTION('ref_axis',(0.,0.,-1.)) ;
#131036=DIRECTION('center_axis',(0.,1.,0.)) ;
#131037=DIRECTION('ref_axis',(1.,0.,0.)) ;
#131038=DIRECTION('center_axis',(-1.,0.,0.)) ;
#131039=DIRECTION('ref_axis',(0.,0.,-1.)) ;
#131040=DIRECTION('center_axis',(0.,1.,0.)) ;
#131041=DIRECTION('ref_axis',(1.,0.,0.)) ;
#131042=DIRECTION('center_axis',(-1.,0.,0.)) ;
#131043=DIRECTION('ref_axis',(0.,0.,-1.)) ;
#131044=DIRECTION('center_axis',(0.,-1.,0.)) ;
#131045=DIRECTION('ref_axis',(0.,0.,-1.)) ;
#131046=DIRECTION('center_axis',(0.,-1.,0.)) ;
#131047=DIRECTION('ref_axis',(0.,0.,-1.)) ;
#131048=DIRECTION('center_axis',(-1.,0.,0.)) ;
#131049=DIRECTION('ref_axis',(0.,0.,1.)) ;
#131050=DIRECTION('center_axis',(-1.,0.,0.)) ;
#131051=DIRECTION('ref_axis',(0.,0.,1.)) ;
#131052=DIRECTION('center_axis',(1.,0.,0.)) ;
#131053=DIRECTION('ref_axis',(0.,0.,-1.)) ;
#131054=DIRECTION('center_axis',(-1.,0.,0.)) ;
#131055=DIRECTION('ref_axis',(0.,0.,1.)) ;
#131056=DIRECTION('center_axis',(0.,-1.,0.)) ;
#131057=DIRECTION('ref_axis',(0.,0.,-1.)) ;
#131058=DIRECTION('center_axis',(0.,-1.,0.)) ;
#131059=DIRECTION('ref_axis',(0.,0.,-1.)) ;
#131060=DIRECTION('center_axis',(0.,1.,0.)) ;
#131061=DIRECTION('ref_axis',(1.,0.,0.)) ;
#131062=DIRECTION('center_axis',(0.,0.,-1.)) ;
#131063=DIRECTION('ref_axis',(1.,0.,0.)) ;
#131064=DIRECTION('center_axis',(0.,1.,0.)) ;
#131065=DIRECTION('ref_axis',(1.,0.,0.)) ;
#131066=DIRECTION('center_axis',(0.,0.,1.)) ;
#131067=DIRECTION('ref_axis',(-1.,0.,0.)) ;
#131068=DIRECTION('center_axis',(0.,0.,-1.)) ;
#131069=DIRECTION('ref_axis',(-1.,0.,0.)) ;
#131070=DIRECTION('center_axis',(1.,1.31418445149758E-16,-2.16840434497101E-16)) ;
#131071=DIRECTION('ref_axis',(-2.16840434497101E-16,-2.8496832747207E-32,
-1.)) ;
#131072=DIRECTION('center_axis',(1.,0.,0.)) ;
#131073=DIRECTION('ref_axis',(0.,0.,-1.)) ;
#131074=DIRECTION('center_axis',(-1.,0.,0.)) ;
#131075=DIRECTION('ref_axis',(0.,0.,1.)) ;
#131076=DIRECTION('center_axis',(-1.31418445149758E-16,1.,0.)) ;
#131077=DIRECTION('ref_axis',(-1.,0.,0.)) ;
#131078=DIRECTION('center_axis',(0.,0.,1.)) ;
#131079=DIRECTION('ref_axis',(-1.,0.,0.)) ;
#131080=DIRECTION('center_axis',(-1.31418445149758E-16,1.,0.)) ;
#131081=DIRECTION('ref_axis',(-1.,-1.31418445149758E-16,0.)) ;
#131082=DIRECTION('center_axis',(-1.31418445149758E-16,1.,0.)) ;
#131083=DIRECTION('ref_axis',(-1.,0.,0.)) ;
#131084=DIRECTION('center_axis',(-1.31418445149758E-16,1.,0.)) ;
#131085=DIRECTION('ref_axis',(-1.,-1.31418445149758E-16,0.)) ;
#131086=DIRECTION('center_axis',(0.,0.,1.)) ;
#131087=DIRECTION('ref_axis',(-1.,0.,0.)) ;
#131088=DIRECTION('center_axis',(-4.33680868994202E-16,-5.69936654944139E-32,
-1.)) ;
#131089=DIRECTION('ref_axis',(-1.,2.47170623787823E-47,4.33680868994202E-16)) ;
#131090=DIRECTION('center_axis',(0.,0.,1.)) ;
#131091=DIRECTION('ref_axis',(1.,0.,0.)) ;
#131092=DIRECTION('center_axis',(-1.31418445149758E-16,-1.,0.)) ;
#131093=DIRECTION('ref_axis',(1.,-1.31418445149758E-16,0.)) ;
#131094=DIRECTION('center_axis',(0.,1.,0.)) ;
#131095=DIRECTION('ref_axis',(0.,0.,1.)) ;
#131096=DIRECTION('center_axis',(-1.,0.,2.16840434497101E-16)) ;
#131097=DIRECTION('ref_axis',(2.16840434497101E-16,0.,1.)) ;
#131098=DIRECTION('center_axis',(-1.,0.,0.)) ;
#131099=DIRECTION('ref_axis',(0.,0.,1.)) ;
#131100=DIRECTION('center_axis',(1.,0.,0.)) ;
#131101=DIRECTION('ref_axis',(0.,0.,-1.)) ;
#131102=DIRECTION('center_axis',(-1.31418445149758E-16,-1.,0.)) ;
#131103=DIRECTION('ref_axis',(1.,-1.31418445149758E-16,0.)) ;
#131104=DIRECTION('center_axis',(0.,1.,0.)) ;
#131105=DIRECTION('ref_axis',(0.,0.,1.)) ;
#131106=DIRECTION('center_axis',(2.16840434497101E-16,2.8496832747207E-32,
1.)) ;
#131107=DIRECTION('ref_axis',(1.,-6.17926559469557E-48,-2.16840434497101E-16)) ;
#131108=DIRECTION('center_axis',(0.,0.,1.)) ;
#131109=DIRECTION('ref_axis',(1.,0.,0.)) ;
#131110=DIRECTION('center_axis',(-1.,-1.31418445149758E-16,-2.16840434497101E-16)) ;
#131111=DIRECTION('ref_axis',(-2.16840434497101E-16,-2.8496832747207E-32,
1.)) ;
#131112=DIRECTION('center_axis',(-1.,0.,0.)) ;
#131113=DIRECTION('ref_axis',(0.,0.,1.)) ;
#131114=DIRECTION('center_axis',(1.,0.,0.)) ;
#131115=DIRECTION('ref_axis',(0.,0.,-1.)) ;
#131116=DIRECTION('center_axis',(-1.31418445149758E-16,1.,0.)) ;
#131117=DIRECTION('ref_axis',(-1.,0.,0.)) ;
#131118=DIRECTION('center_axis',(-1.31418445149758E-16,1.,0.)) ;
#131119=DIRECTION('ref_axis',(-1.,-1.31418445149758E-16,0.)) ;
#131120=DIRECTION('center_axis',(0.,1.,0.)) ;
#131121=DIRECTION('ref_axis',(1.,0.,0.)) ;
#131122=DIRECTION('center_axis',(0.,0.,-1.)) ;
#131123=DIRECTION('ref_axis',(1.,0.,0.)) ;
#131124=DIRECTION('center_axis',(0.,1.,0.)) ;
#131125=DIRECTION('ref_axis',(1.,0.,0.)) ;
#131126=DIRECTION('center_axis',(0.,0.,-1.)) ;
#131127=DIRECTION('ref_axis',(1.,0.,0.)) ;
#131128=DIRECTION('center_axis',(-1.31418445149758E-16,1.,0.)) ;
#131129=DIRECTION('ref_axis',(-1.,0.,0.)) ;
#131130=DIRECTION('center_axis',(-1.31418445149758E-16,1.,0.)) ;
#131131=DIRECTION('ref_axis',(-1.,-1.31418445149758E-16,0.)) ;
#131132=DIRECTION('center_axis',(-1.31418445149758E-16,-1.,0.)) ;
#131133=DIRECTION('ref_axis',(1.,-1.31418445149758E-16,0.)) ;
#131134=DIRECTION('center_axis',(0.,1.,0.)) ;
#131135=DIRECTION('ref_axis',(0.,0.,1.)) ;
#131136=DIRECTION('center_axis',(4.33680868994202E-16,0.,1.)) ;
#131137=DIRECTION('ref_axis',(1.,0.,-4.33680868994202E-16)) ;
#131138=DIRECTION('center_axis',(0.,0.,-1.)) ;
#131139=DIRECTION('ref_axis',(-1.,0.,0.)) ;
#131140=DIRECTION('center_axis',(-2.16840434497101E-16,0.,-1.)) ;
#131141=DIRECTION('ref_axis',(-1.,0.,2.16840434497101E-16)) ;
#131142=DIRECTION('center_axis',(0.,0.,-1.)) ;
#131143=DIRECTION('ref_axis',(-1.,0.,0.)) ;
#131144=DIRECTION('center_axis',(-1.31418445149758E-16,-1.,0.)) ;
#131145=DIRECTION('ref_axis',(1.,-1.31418445149758E-16,0.)) ;
#131146=DIRECTION('center_axis',(0.,1.,0.)) ;
#131147=DIRECTION('ref_axis',(0.,0.,1.)) ;
#131148=DIRECTION('center_axis',(0.,1.,0.)) ;
#131149=DIRECTION('ref_axis',(1.,0.,0.)) ;
#131150=DIRECTION('center_axis',(-1.,0.,0.)) ;
#131151=DIRECTION('ref_axis',(0.,0.,-1.)) ;
#131152=DIRECTION('center_axis',(0.,1.,0.)) ;
#131153=DIRECTION('ref_axis',(1.,0.,0.)) ;
#131154=DIRECTION('center_axis',(1.,0.,0.)) ;
#131155=DIRECTION('ref_axis',(0.,0.,1.)) ;
#131156=DIRECTION('center_axis',(1.,0.,2.16840434497101E-16)) ;
#131157=DIRECTION('ref_axis',(2.16840434497101E-16,0.,-1.)) ;
#131158=DIRECTION('center_axis',(0.,1.,0.)) ;
#131159=DIRECTION('ref_axis',(0.,0.,1.)) ;
#131160=DIRECTION('center_axis',(0.,1.,0.)) ;
#131161=DIRECTION('ref_axis',(0.,0.,1.)) ;
#131162=DIRECTION('center_axis',(0.,0.,-1.)) ;
#131163=DIRECTION('ref_axis',(-1.,0.,0.)) ;
#131164=DIRECTION('center_axis',(0.,0.,1.)) ;
#131165=DIRECTION('ref_axis',(1.,0.,0.)) ;
#131166=DIRECTION('center_axis',(0.,0.,-1.)) ;
#131167=DIRECTION('ref_axis',(-1.,0.,0.)) ;
#131168=DIRECTION('center_axis',(0.,1.,0.)) ;
#131169=DIRECTION('ref_axis',(0.,0.,1.)) ;
#131170=DIRECTION('center_axis',(0.,1.,0.)) ;
#131171=DIRECTION('ref_axis',(0.,0.,1.)) ;
#131172=DIRECTION('center_axis',(0.,1.,0.)) ;
#131173=DIRECTION('ref_axis',(1.,0.,0.)) ;
#131174=DIRECTION('center_axis',(-1.,0.,0.)) ;
#131175=DIRECTION('ref_axis',(0.,0.,-1.)) ;
#131176=DIRECTION('center_axis',(0.,1.,0.)) ;
#131177=DIRECTION('ref_axis',(1.,0.,0.)) ;
#131178=DIRECTION('center_axis',(-1.,0.,0.)) ;
#131179=DIRECTION('ref_axis',(0.,0.,-1.)) ;
#131180=DIRECTION('center_axis',(0.,1.,0.)) ;
#131181=DIRECTION('ref_axis',(0.,0.,1.)) ;
#131182=DIRECTION('center_axis',(0.,1.,0.)) ;
#131183=DIRECTION('ref_axis',(0.,0.,1.)) ;
#131184=DIRECTION('center_axis',(-1.,0.,0.)) ;
#131185=DIRECTION('ref_axis',(0.,0.,1.)) ;
#131186=DIRECTION('center_axis',(-1.,0.,0.)) ;
#131187=DIRECTION('ref_axis',(0.,0.,1.)) ;
#131188=DIRECTION('center_axis',(1.,0.,0.)) ;
#131189=DIRECTION('ref_axis',(0.,0.,-1.)) ;
#131190=DIRECTION('center_axis',(-1.,0.,0.)) ;
#131191=DIRECTION('ref_axis',(0.,0.,1.)) ;
#131192=DIRECTION('center_axis',(0.,1.,0.)) ;
#131193=DIRECTION('ref_axis',(0.,0.,1.)) ;
#131194=DIRECTION('center_axis',(0.,1.,0.)) ;
#131195=DIRECTION('ref_axis',(0.,0.,1.)) ;
#131196=DIRECTION('center_axis',(0.,1.,0.)) ;
#131197=DIRECTION('ref_axis',(1.,0.,0.)) ;
#131198=DIRECTION('center_axis',(0.,0.,1.)) ;
#131199=DIRECTION('ref_axis',(-1.,0.,0.)) ;
#131200=DIRECTION('center_axis',(0.,1.,0.)) ;
#131201=DIRECTION('ref_axis',(1.,0.,0.)) ;
#131202=DIRECTION('center_axis',(0.,0.,-1.)) ;
#131203=DIRECTION('ref_axis',(1.,0.,0.)) ;
#131204=DIRECTION('center_axis',(0.,0.,1.)) ;
#131205=DIRECTION('ref_axis',(1.,0.,0.)) ;
#131206=DIRECTION('center_axis',(0.,0.,1.)) ;
#131207=DIRECTION('ref_axis',(1.,0.,0.)) ;
#131208=DIRECTION('center_axis',(0.,0.,-1.)) ;
#131209=DIRECTION('ref_axis',(-1.,0.,0.)) ;
#131210=DIRECTION('center_axis',(-3.46944695195361E-14,0.,1.)) ;
#131211=DIRECTION('ref_axis',(1.,0.,3.46944695195361E-14)) ;
#131212=DIRECTION('center_axis',(1.,0.,0.)) ;
#131213=DIRECTION('ref_axis',(0.,0.,-1.)) ;
#131214=DIRECTION('center_axis',(1.,0.,0.)) ;
#131215=DIRECTION('ref_axis',(0.,0.,-1.)) ;
#131216=DIRECTION('center_axis',(1.,0.,0.)) ;
#131217=DIRECTION('ref_axis',(0.,0.,-1.)) ;
#131218=DIRECTION('center_axis',(1.,0.,8.67361737988409E-15)) ;
#131219=DIRECTION('ref_axis',(8.67361737988409E-15,0.,-1.)) ;
#131220=DIRECTION('center_axis',(1.,0.,0.)) ;
#131221=DIRECTION('ref_axis',(0.,0.,-1.)) ;
#131222=DIRECTION('center_axis',(1.,0.,1.73472347597682E-14)) ;
#131223=DIRECTION('ref_axis',(1.73472347597682E-14,0.,-1.)) ;
#131224=DIRECTION('center_axis',(-1.,0.,0.)) ;
#131225=DIRECTION('ref_axis',(0.,0.,1.)) ;
#131226=DIRECTION('center_axis',(1.,0.,0.)) ;
#131227=DIRECTION('ref_axis',(0.,0.,-1.)) ;
#131228=DIRECTION('center_axis',(1.,0.,0.)) ;
#131229=DIRECTION('ref_axis',(0.,0.,-1.)) ;
#131230=DIRECTION('center_axis',(-3.46944695195364E-14,0.,-1.)) ;
#131231=DIRECTION('ref_axis',(-1.,0.,3.46944695195364E-14)) ;
#131232=DIRECTION('center_axis',(1.,0.,0.)) ;
#131233=DIRECTION('ref_axis',(0.,0.,-1.)) ;
#131234=DIRECTION('center_axis',(-3.46944695195364E-14,0.,1.)) ;
#131235=DIRECTION('ref_axis',(1.,0.,3.46944695195364E-14)) ;
#131236=DIRECTION('center_axis',(0.,0.,-1.)) ;
#131237=DIRECTION('ref_axis',(-1.,0.,0.)) ;
#131238=DIRECTION('center_axis',(-0.422618261740697,5.55398348498559E-17,
0.906307787036651)) ;
#131239=DIRECTION('ref_axis',(0.906307787036651,6.51773046476477E-31,0.422618261740697)) ;
#131240=DIRECTION('center_axis',(0.422618261740697,-5.55398348498559E-17,
-0.906307787036651)) ;
#131241=DIRECTION('ref_axis',(-0.906307787036651,-6.46086972436398E-31,
-0.422618261740697)) ;
#131242=DIRECTION('center_axis',(-0.422618261740697,5.55398348498559E-17,
0.906307787036651)) ;
#131243=DIRECTION('ref_axis',(0.906307787036651,6.46086972436398E-31,0.422618261740697)) ;
#131244=DIRECTION('center_axis',(0.422618261740697,-5.55398348498559E-17,
-0.906307787036651)) ;
#131245=DIRECTION('ref_axis',(-0.906307787036651,-6.46086972436398E-31,
-0.422618261740697)) ;
#131246=DIRECTION('center_axis',(0.,1.,0.)) ;
#131247=DIRECTION('ref_axis',(1.,0.,0.)) ;
#131248=DIRECTION('center_axis',(8.40428841770292E-14,0.51423179695912,
-0.85765124555159)) ;
#131249=DIRECTION('ref_axis',(3.46944695195355E-14,-0.85765124555159,-0.51423179695912)) ;
#131250=DIRECTION('center_axis',(0.,-6.93889390390724E-14,1.)) ;
#131251=DIRECTION('ref_axis',(0.,1.,6.93889390390724E-14)) ;
#131252=DIRECTION('center_axis',(-1.,0.,0.)) ;
#131253=DIRECTION('ref_axis',(0.,2.16840434497095E-14,-1.)) ;
#131254=DIRECTION('center_axis',(0.,0.,1.)) ;
#131255=DIRECTION('ref_axis',(1.,0.,0.)) ;
#131256=DIRECTION('center_axis',(0.,0.,1.)) ;
#131257=DIRECTION('ref_axis',(1.,0.,0.)) ;
#131258=DIRECTION('center_axis',(-1.,0.,0.)) ;
#131259=DIRECTION('ref_axis',(0.,0.,1.)) ;
#131260=DIRECTION('center_axis',(-1.,0.,0.)) ;
#131261=DIRECTION('ref_axis',(0.,1.30104260698257E-14,-1.)) ;
#131262=DIRECTION('center_axis',(1.,0.,0.)) ;
#131263=DIRECTION('ref_axis',(0.,0.,-1.)) ;
#131264=DIRECTION('center_axis',(0.,-0.514231796959192,-0.857651245551547)) ;
#131265=DIRECTION('ref_axis',(0.,0.857651245551547,-0.514231796959192)) ;
#131266=DIRECTION('center_axis',(0.,1.,8.97270763436279E-17)) ;
#131267=DIRECTION('ref_axis',(0.,-8.97270763436279E-17,1.)) ;
#131268=DIRECTION('center_axis',(0.,-1.,-8.97270763436279E-17)) ;
#131269=DIRECTION('ref_axis',(0.,-8.97270763436279E-17,1.)) ;
#131270=DIRECTION('center_axis',(0.,-1.,0.)) ;
#131271=DIRECTION('ref_axis',(0.,0.,-1.)) ;
#131272=DIRECTION('center_axis',(0.,1.,0.)) ;
#131273=DIRECTION('ref_axis',(1.,0.,0.)) ;
#131274=DIRECTION('center_axis',(-1.,0.,0.)) ;
#131275=DIRECTION('ref_axis',(0.,0.,-1.)) ;
#131276=DIRECTION('center_axis',(1.,0.,0.)) ;
#131277=DIRECTION('ref_axis',(0.,0.,-1.)) ;
#131278=DIRECTION('center_axis',(0.,-0.514231796959126,0.857651245551587)) ;
#131279=DIRECTION('ref_axis',(0.,0.857651245551587,0.514231796959126)) ;
#131280=DIRECTION('center_axis',(0.,0.,-1.)) ;
#131281=DIRECTION('ref_axis',(1.,0.,0.)) ;
#131282=DIRECTION('center_axis',(0.,1.,0.)) ;
#131283=DIRECTION('ref_axis',(1.,0.,0.)) ;
#131284=DIRECTION('center_axis',(-6.93889390390727E-14,0.,-1.)) ;
#131285=DIRECTION('ref_axis',(1.,0.,-6.93889390390727E-14)) ;
#131286=DIRECTION('center_axis',(-1.,0.,0.)) ;
#131287=DIRECTION('ref_axis',(0.,-2.16840434497095E-14,-1.)) ;
#131288=DIRECTION('center_axis',(0.,0.,-1.)) ;
#131289=DIRECTION('ref_axis',(-1.,0.,0.)) ;
#131290=DIRECTION('center_axis',(0.,0.,1.)) ;
#131291=DIRECTION('ref_axis',(-1.,0.,0.)) ;
#131292=DIRECTION('center_axis',(0.,0.,-1.)) ;
#131293=DIRECTION('ref_axis',(-1.,0.,0.)) ;
#131294=DIRECTION('center_axis',(-1.,0.,7.01133629567814E-33)) ;
#131295=DIRECTION('ref_axis',(7.01133629567814E-33,0.,1.)) ;
#131296=DIRECTION('center_axis',(-1.,0.,0.)) ;
#131297=DIRECTION('ref_axis',(0.,0.,1.)) ;
#131298=DIRECTION('center_axis',(0.,0.,-1.)) ;
#131299=DIRECTION('ref_axis',(-1.,0.,0.)) ;
#131300=DIRECTION('center_axis',(-7.01133629567814E-33,8.97270763436279E-17,
-1.)) ;
#131301=DIRECTION('ref_axis',(6.29106707073161E-49,1.,8.97270763436279E-17)) ;
#131302=DIRECTION('center_axis',(1.,0.,0.)) ;
#131303=DIRECTION('ref_axis',(0.,0.,-1.)) ;
#131304=DIRECTION('center_axis',(6.69037477709045E-15,0.51423179695912,
0.85765124555159)) ;
#131305=DIRECTION('ref_axis',(-4.49049578447409E-29,-0.85765124555159,0.51423179695912)) ;
#131306=DIRECTION('center_axis',(-1.,0.,0.)) ;
#131307=DIRECTION('ref_axis',(0.,0.,1.)) ;
#131308=DIRECTION('center_axis',(-1.,0.,0.)) ;
#131309=DIRECTION('ref_axis',(0.,1.30104260698257E-14,-1.)) ;
#131310=DIRECTION('center_axis',(0.,0.,1.)) ;
#131311=DIRECTION('ref_axis',(1.,0.,0.)) ;
#131312=DIRECTION('center_axis',(0.,0.,-1.)) ;
#131313=DIRECTION('ref_axis',(-1.,0.,0.)) ;
#131314=DIRECTION('center_axis',(0.,-1.,8.97270763436279E-17)) ;
#131315=DIRECTION('ref_axis',(0.,-8.97270763436279E-17,-1.)) ;
#131316=DIRECTION('center_axis',(0.,-1.,8.97270763436279E-17)) ;
#131317=DIRECTION('ref_axis',(0.,-8.97270763436279E-17,-1.)) ;
#131318=DIRECTION('center_axis',(0.,-1.,0.)) ;
#131319=DIRECTION('ref_axis',(0.,0.,-1.)) ;
#131320=DIRECTION('center_axis',(-7.01133629567814E-33,8.97270763436279E-17,
-1.)) ;
#131321=DIRECTION('ref_axis',(0.,1.,0.)) ;
#131322=DIRECTION('center_axis',(0.,-1.,0.)) ;
#131323=DIRECTION('ref_axis',(0.,0.,1.)) ;
#131324=DIRECTION('center_axis',(1.,0.,0.)) ;
#131325=DIRECTION('ref_axis',(0.,0.,-1.)) ;
#131326=DIRECTION('center_axis',(0.,0.,1.)) ;
#131327=DIRECTION('ref_axis',(-1.,0.,0.)) ;
#131328=DIRECTION('center_axis',(0.,1.,0.)) ;
#131329=DIRECTION('ref_axis',(1.,0.,0.)) ;
#131330=DIRECTION('center_axis',(-1.,0.,0.)) ;
#131331=DIRECTION('ref_axis',(0.,0.,-1.)) ;
#131332=DIRECTION('center_axis',(1.,7.81406971160724E-17,0.)) ;
#131333=DIRECTION('ref_axis',(-7.81406971160724E-17,1.,0.)) ;
#131334=DIRECTION('center_axis',(1.,0.,0.)) ;
#131335=DIRECTION('ref_axis',(0.,0.,-1.)) ;
#131336=DIRECTION('center_axis',(1.,0.,0.)) ;
#131337=DIRECTION('ref_axis',(0.,0.,-1.)) ;
#131338=DIRECTION('center_axis',(0.,1.,8.97270763436279E-17)) ;
#131339=DIRECTION('ref_axis',(0.,-8.97270763436279E-17,1.)) ;
#131340=DIRECTION('center_axis',(0.,-1.,0.)) ;
#131341=DIRECTION('ref_axis',(0.,0.,-1.)) ;
#131342=DIRECTION('center_axis',(0.,0.,-1.)) ;
#131343=DIRECTION('ref_axis',(-1.,0.,0.)) ;
#131344=DIRECTION('center_axis',(-7.01133629567814E-33,8.97270763436279E-17,
1.)) ;
#131345=DIRECTION('ref_axis',(-6.29106707073161E-49,-1.,8.97270763436279E-17)) ;
#131346=DIRECTION('center_axis',(-1.,0.,-7.01133629567814E-33)) ;
#131347=DIRECTION('ref_axis',(-7.01133629567814E-33,0.,1.)) ;
#131348=DIRECTION('center_axis',(-1.,0.,0.)) ;
#131349=DIRECTION('ref_axis',(0.,0.,1.)) ;
#131350=DIRECTION('center_axis',(1.,0.,0.)) ;
#131351=DIRECTION('ref_axis',(0.,1.,0.)) ;
#131352=DIRECTION('center_axis',(4.33680868994202E-15,1.,0.)) ;
#131353=DIRECTION('ref_axis',(-1.,4.33680868994202E-15,0.)) ;
#131354=DIRECTION('center_axis',(0.,1.,0.)) ;
#131355=DIRECTION('ref_axis',(1.,0.,0.)) ;
#131356=DIRECTION('center_axis',(0.,0.,-1.)) ;
#131357=DIRECTION('ref_axis',(1.,0.,0.)) ;
#131358=DIRECTION('center_axis',(-1.,0.,0.)) ;
#131359=DIRECTION('ref_axis',(0.,0.,-1.)) ;
#131360=DIRECTION('center_axis',(-7.01133629567814E-33,8.97270763436279E-17,
1.)) ;
#131361=DIRECTION('ref_axis',(0.,-1.,0.)) ;
#131362=DIRECTION('center_axis',(0.,-1.,0.)) ;
#131363=DIRECTION('ref_axis',(0.,0.,1.)) ;
#131364=DIRECTION('center_axis',(7.81406971160724E-17,-1.,-8.97270763436279E-17)) ;
#131365=DIRECTION('ref_axis',(-7.01133629567814E-33,8.97270763436279E-17,
-1.)) ;
#131366=DIRECTION('center_axis',(0.,1.,0.)) ;
#131367=DIRECTION('ref_axis',(0.,0.,1.)) ;
#131368=DIRECTION('center_axis',(-1.,-7.81406971160724E-17,0.)) ;
#131369=DIRECTION('ref_axis',(7.81406971160724E-17,-1.,0.)) ;
#131370=DIRECTION('center_axis',(-1.,-7.81406971160724E-17,0.)) ;
#131371=DIRECTION('ref_axis',(-7.81406971160724E-17,1.,0.)) ;
#131372=DIRECTION('center_axis',(0.,0.,1.)) ;
#131373=DIRECTION('ref_axis',(1.,0.,0.)) ;
#131374=DIRECTION('center_axis',(0.,0.,-1.)) ;
#131375=DIRECTION('ref_axis',(-1.,0.,0.)) ;
#131376=DIRECTION('center_axis',(0.,-1.,8.97270763436279E-17)) ;
#131377=DIRECTION('ref_axis',(0.,-8.97270763436279E-17,-1.)) ;
#131378=DIRECTION('center_axis',(0.,-1.,0.)) ;
#131379=DIRECTION('ref_axis',(0.,0.,-1.)) ;
#131380=DIRECTION('center_axis',(1.,7.81406971160724E-17,0.)) ;
#131381=DIRECTION('ref_axis',(0.,1.,0.)) ;
#131382=DIRECTION('center_axis',(0.,0.,1.)) ;
#131383=DIRECTION('ref_axis',(-1.,0.,0.)) ;
#131384=DIRECTION('center_axis',(0.,1.,0.)) ;
#131385=DIRECTION('ref_axis',(1.,0.,0.)) ;
#131386=DIRECTION('center_axis',(-1.,0.,0.)) ;
#131387=DIRECTION('ref_axis',(0.,0.,-1.)) ;
#131388=DIRECTION('center_axis',(0.,0.,-1.)) ;
#131389=DIRECTION('ref_axis',(-1.,0.,0.)) ;
#131390=DIRECTION('center_axis',(0.,0.,1.)) ;
#131391=DIRECTION('ref_axis',(1.,0.,0.)) ;
#131392=DIRECTION('center_axis',(-1.,-7.81406971160724E-17,0.)) ;
#131393=DIRECTION('ref_axis',(7.81406971160724E-17,-1.,0.)) ;
#131394=DIRECTION('center_axis',(-1.,-7.81406971160724E-17,0.)) ;
#131395=DIRECTION('ref_axis',(-7.81406971160724E-17,1.,0.)) ;
#131396=DIRECTION('center_axis',(1.,7.81406971160724E-17,0.)) ;
#131397=DIRECTION('ref_axis',(-7.81406971160724E-17,1.,0.)) ;
#131398=DIRECTION('center_axis',(1.,0.,0.)) ;
#131399=DIRECTION('ref_axis',(0.,0.,-1.)) ;
#131400=DIRECTION('center_axis',(1.,0.,0.)) ;
#131401=DIRECTION('ref_axis',(0.,0.,-1.)) ;
#131402=DIRECTION('center_axis',(3.78638272950961E-32,-4.8455963016112E-16,
-1.)) ;
#131403=DIRECTION('ref_axis',(1.83472821505963E-47,1.,-4.8455963016112E-16)) ;
#131404=DIRECTION('center_axis',(0.,0.,-1.)) ;
#131405=DIRECTION('ref_axis',(-1.,0.,0.)) ;
#131406=DIRECTION('center_axis',(0.,0.,-1.)) ;
#131407=DIRECTION('ref_axis',(-1.,0.,0.)) ;
#131408=DIRECTION('center_axis',(1.,7.81406971160724E-17,0.)) ;
#131409=DIRECTION('ref_axis',(0.,1.,0.)) ;
#131410=DIRECTION('center_axis',(0.,-1.,0.)) ;
#131411=DIRECTION('ref_axis',(0.,0.,1.)) ;
#131412=DIRECTION('center_axis',(0.,1.,0.)) ;
#131413=DIRECTION('ref_axis',(1.,0.,0.)) ;
#131414=DIRECTION('center_axis',(0.,1.,0.)) ;
#131415=DIRECTION('ref_axis',(0.,0.,-1.)) ;
#131416=DIRECTION('center_axis',(-7.81406971160724E-17,1.,-8.97270763436279E-17)) ;
#131417=DIRECTION('ref_axis',(-7.01133629567814E-33,8.97270763436279E-17,
1.)) ;
#131418=DIRECTION('center_axis',(0.,-1.,0.)) ;
#131419=DIRECTION('ref_axis',(0.,0.,-1.)) ;
#131420=DIRECTION('center_axis',(0.,1.,0.)) ;
#131421=DIRECTION('ref_axis',(0.,0.,1.)) ;
#131422=DIRECTION('center_axis',(0.,-1.,0.)) ;
#131423=DIRECTION('ref_axis',(0.,0.,-1.)) ;
#131424=DIRECTION('center_axis',(0.,-1.,0.)) ;
#131425=DIRECTION('ref_axis',(0.,0.,-1.)) ;
#131426=DIRECTION('center_axis',(0.,1.,0.)) ;
#131427=DIRECTION('ref_axis',(1.,0.,0.)) ;
#131428=DIRECTION('center_axis',(0.,0.,1.)) ;
#131429=DIRECTION('ref_axis',(-1.,0.,0.)) ;
#131430=DIRECTION('center_axis',(1.,0.,0.)) ;
#131431=DIRECTION('ref_axis',(0.,0.,1.)) ;
#131432=DIRECTION('center_axis',(0.,-1.,0.)) ;
#131433=DIRECTION('ref_axis',(0.,0.,-1.)) ;
#131434=DIRECTION('center_axis',(0.,1.,0.)) ;
#131435=DIRECTION('ref_axis',(0.,0.,1.)) ;
#131436=DIRECTION('center_axis',(0.,-1.,0.)) ;
#131437=DIRECTION('ref_axis',(0.,0.,-1.)) ;
#131438=DIRECTION('center_axis',(-1.,0.,2.16840434497101E-16)) ;
#131439=DIRECTION('ref_axis',(2.16840434497101E-16,0.,1.)) ;
#131440=DIRECTION('center_axis',(1.,0.,0.)) ;
#131441=DIRECTION('ref_axis',(0.,0.,-1.)) ;
#131442=DIRECTION('center_axis',(-2.16840434497101E-16,0.,1.)) ;
#131443=DIRECTION('ref_axis',(1.,0.,2.16840434497101E-16)) ;
#131444=DIRECTION('center_axis',(0.,0.,1.)) ;
#131445=DIRECTION('ref_axis',(1.,0.,0.)) ;
#131446=DIRECTION('center_axis',(0.,1.,0.)) ;
#131447=DIRECTION('ref_axis',(0.,0.,1.)) ;
#131448=DIRECTION('center_axis',(0.,-1.,0.)) ;
#131449=DIRECTION('ref_axis',(0.,0.,-1.)) ;
#131450=DIRECTION('center_axis',(0.,1.,0.)) ;
#131451=DIRECTION('ref_axis',(1.,0.,0.)) ;
#131452=DIRECTION('center_axis',(0.,0.,1.)) ;
#131453=DIRECTION('ref_axis',(-1.,0.,0.)) ;
#131454=DIRECTION('center_axis',(0.,1.,0.)) ;
#131455=DIRECTION('ref_axis',(1.,0.,0.)) ;
#131456=DIRECTION('center_axis',(1.,0.,0.)) ;
#131457=DIRECTION('ref_axis',(0.,0.,1.)) ;
#131458=DIRECTION('center_axis',(0.,0.,-1.)) ;
#131459=DIRECTION('ref_axis',(-1.,0.,0.)) ;
#131460=DIRECTION('center_axis',(0.,0.,1.)) ;
#131461=DIRECTION('ref_axis',(1.,0.,0.)) ;
#131462=DIRECTION('center_axis',(1.,0.,2.16840434497101E-16)) ;
#131463=DIRECTION('ref_axis',(2.16840434497101E-16,0.,-1.)) ;
#131464=DIRECTION('center_axis',(1.,0.,0.)) ;
#131465=DIRECTION('ref_axis',(0.,0.,-1.)) ;
#131466=DIRECTION('center_axis',(0.,1.,0.)) ;
#131467=DIRECTION('ref_axis',(1.,0.,0.)) ;
#131468=DIRECTION('center_axis',(0.,1.,0.)) ;
#131469=DIRECTION('ref_axis',(0.,0.,-1.)) ;
#131470=DIRECTION('center_axis',(0.,1.,0.)) ;
#131471=DIRECTION('ref_axis',(0.,0.,1.)) ;
#131472=DIRECTION('center_axis',(0.,1.,0.)) ;
#131473=DIRECTION('ref_axis',(0.,0.,1.)) ;
#131474=DIRECTION('center_axis',(-0.942809041582061,-0.235702260395515,
0.235702260395526)) ;
#131475=DIRECTION('ref_axis',(0.242535625036343,2.28772620246771E-15,0.970142500145329)) ;
#131476=DIRECTION('center_axis',(-0.970142500145332,-0.242535625036331,
-2.10366121255624E-15)) ;
#131477=DIRECTION('ref_axis',(0.242535625036331,-0.970142500145332,-4.68743664149877E-30)) ;
#131478=DIRECTION('center_axis',(0.970142500145333,0.24253562503633,0.)) ;
#131479=DIRECTION('ref_axis',(-0.24253562503633,0.970142500145333,0.)) ;
#131480=DIRECTION('center_axis',(-0.970142500145333,-0.242535625036331,
-2.73475957632295E-14)) ;
#131481=DIRECTION('ref_axis',(0.242535625036331,-0.970142500145332,-1.21802906808468E-29)) ;
#131482=DIRECTION('center_axis',(0.879462917689188,0.219865729422294,-0.42214220049081)) ;
#131483=DIRECTION('ref_axis',(-0.432731067584771,1.71515946658E-16,-0.901523057468274)) ;
#131484=DIRECTION('center_axis',(0.879462917689182,0.219865729422321,-0.422142200490809)) ;
#131485=DIRECTION('ref_axis',(-0.432731067584773,-7.60553175829864E-17,
-0.901523057468273)) ;
#131486=DIRECTION('center_axis',(0.,1.,0.)) ;
#131487=DIRECTION('ref_axis',(1.,0.,0.)) ;
#131488=DIRECTION('center_axis',(-2.00438979995004E-14,-1.,0.)) ;
#131489=DIRECTION('ref_axis',(-1.,2.00438979995004E-14,0.)) ;
#131490=DIRECTION('center_axis',(0.,-1.,0.)) ;
#131491=DIRECTION('ref_axis',(0.,0.,-1.)) ;
#131492=DIRECTION('center_axis',(0.,-1.,0.)) ;
#131493=DIRECTION('ref_axis',(0.,0.,-1.)) ;
#131494=DIRECTION('center_axis',(0.669589480006976,-0.669589480006974,-0.321402950403349)) ;
#131495=DIRECTION('ref_axis',(0.707106781186547,0.707106781186548,5.45170614306381E-16)) ;
#131496=DIRECTION('center_axis',(0.669589480006977,-0.669589480006977,-0.321402950403339)) ;
#131497=DIRECTION('ref_axis',(0.707106781186548,0.707106781186548,1.13950759497276E-17)) ;
#131498=DIRECTION('center_axis',(0.,1.,0.)) ;
#131499=DIRECTION('ref_axis',(1.,0.,0.)) ;
#131500=DIRECTION('center_axis',(0.70710678118654,-0.707106781186555,0.)) ;
#131501=DIRECTION('ref_axis',(-0.707106781186555,-0.70710678118654,0.)) ;
#131502=DIRECTION('center_axis',(0.707106781186549,-0.707106781186546,0.)) ;
#131503=DIRECTION('ref_axis',(0.707106781186546,0.707106781186549,0.)) ;
#131504=DIRECTION('center_axis',(0.707106781186548,-0.707106781186548,-1.53329341668333E-15)) ;
#131505=DIRECTION('ref_axis',(0.707106781186548,0.707106781186548,-2.94242918747921E-32)) ;
#131506=DIRECTION('center_axis',(0.57735026918962,-0.57735026918962,-0.577350269189638)) ;
#131507=DIRECTION('ref_axis',(-0.707106781186559,-1.11282436496257E-15,
-0.707106781186536)) ;
#131508=DIRECTION('center_axis',(-0.577350269189328,0.577350269189571,-0.577350269189978)) ;
#131509=DIRECTION('ref_axis',(-7.61554280732519E-15,0.707106781186793,0.707106781186302)) ;
#131510=DIRECTION('center_axis',(-0.707106781186548,0.707106781186548,7.66646708341718E-15)) ;
#131511=DIRECTION('ref_axis',(-0.707106781186548,-0.707106781186548,3.27987112860885E-31)) ;
#131512=DIRECTION('center_axis',(-0.707106781186549,0.707106781186546,0.)) ;
#131513=DIRECTION('ref_axis',(-0.707106781186546,-0.707106781186549,0.)) ;
#131514=DIRECTION('center_axis',(-0.707106781186548,0.707106781186548,-1.13463712834566E-13)) ;
#131515=DIRECTION('ref_axis',(-0.707106781186548,-0.707106781186548,1.81538773348134E-28)) ;
#131516=DIRECTION('center_axis',(-0.669589480006976,0.669589480006974,-0.321402950403349)) ;
#131517=DIRECTION('ref_axis',(-0.707106781186547,-0.707106781186548,5.45170614306381E-16)) ;
#131518=DIRECTION('center_axis',(0.66958948000704,-0.669589480006895,0.32140295040338)) ;
#131519=DIRECTION('ref_axis',(0.707106781186471,0.707106781186624,1.36895061126305E-16)) ;
#131520=DIRECTION('center_axis',(0.,1.,0.)) ;
#131521=DIRECTION('ref_axis',(1.,0.,0.)) ;
#131522=DIRECTION('center_axis',(-1.50329234996253E-14,1.,0.)) ;
#131523=DIRECTION('ref_axis',(1.,1.50329234996253E-14,0.)) ;
#131524=DIRECTION('center_axis',(0.,-1.,0.)) ;
#131525=DIRECTION('ref_axis',(0.,0.,-1.)) ;
#131526=DIRECTION('center_axis',(0.,1.,0.)) ;
#131527=DIRECTION('ref_axis',(0.,0.,1.)) ;
#131528=DIRECTION('center_axis',(-0.879462917689188,-0.219865729422294,
-0.42214220049081)) ;
#131529=DIRECTION('ref_axis',(-0.432731067584771,1.71515946658E-16,0.901523057468274)) ;
#131530=DIRECTION('center_axis',(0.879462917689201,0.219865729422298,0.42214220049078)) ;
#131531=DIRECTION('ref_axis',(0.432731067584741,-2.36820597908546E-15,-0.901523057468288)) ;
#131532=DIRECTION('center_axis',(0.,1.,0.)) ;
#131533=DIRECTION('ref_axis',(1.,0.,0.)) ;
#131534=DIRECTION('center_axis',(0.970142500145323,0.242535625036368,0.)) ;
#131535=DIRECTION('ref_axis',(0.242535625036368,-0.970142500145323,0.)) ;
#131536=DIRECTION('center_axis',(-0.970142500145333,-0.24253562503633,0.)) ;
#131537=DIRECTION('ref_axis',(0.24253562503633,-0.970142500145333,0.)) ;
#131538=DIRECTION('center_axis',(0.970142500145333,0.242535625036331,-2.1036612125561E-15)) ;
#131539=DIRECTION('ref_axis',(-0.242535625036331,0.970142500145332,-1.06801962627779E-30)) ;
#131540=DIRECTION('center_axis',(0.942809041582058,0.235702260395512,0.23570226039554)) ;
#131541=DIRECTION('ref_axis',(0.242535625036358,-1.84667126758454E-15,-0.970142500145326)) ;
#131542=DIRECTION('center_axis',(0.,-1.,0.)) ;
#131543=DIRECTION('ref_axis',(0.,0.,-1.)) ;
#131544=DIRECTION('center_axis',(-1.,0.,-8.67361737988439E-15)) ;
#131545=DIRECTION('ref_axis',(-8.67361737988439E-15,0.,1.)) ;
#131546=DIRECTION('center_axis',(0.,0.,-1.)) ;
#131547=DIRECTION('ref_axis',(-1.,0.,0.)) ;
#131548=DIRECTION('center_axis',(0.,0.,-1.)) ;
#131549=DIRECTION('ref_axis',(-1.,0.,0.)) ;
#131550=DIRECTION('center_axis',(0.,0.,-1.)) ;
#131551=DIRECTION('ref_axis',(-1.,0.,0.)) ;
#131552=DIRECTION('center_axis',(1.,0.,0.)) ;
#131553=DIRECTION('ref_axis',(0.,0.,-1.)) ;
#131554=DIRECTION('center_axis',(-1.,0.,0.)) ;
#131555=DIRECTION('ref_axis',(0.,0.,1.)) ;
#131556=DIRECTION('center_axis',(0.,-1.,0.)) ;
#131557=DIRECTION('ref_axis',(0.,0.,-1.)) ;
#131558=DIRECTION('center_axis',(-1.,0.,0.)) ;
#131559=DIRECTION('ref_axis',(0.,0.,1.)) ;
#131560=DIRECTION('center_axis',(0.,-1.,0.)) ;
#131561=DIRECTION('ref_axis',(0.,0.,-1.)) ;
#131562=DIRECTION('center_axis',(0.,0.,-1.)) ;
#131563=DIRECTION('ref_axis',(-1.,0.,0.)) ;
#131564=DIRECTION('center_axis',(-1.,0.,0.)) ;
#131565=DIRECTION('ref_axis',(0.,0.,1.)) ;
#131566=DIRECTION('center_axis',(-1.,1.73472347597681E-14,0.)) ;
#131567=DIRECTION('ref_axis',(-1.73472347597681E-14,-1.,0.)) ;
#131568=DIRECTION('center_axis',(0.,0.,1.)) ;
#131569=DIRECTION('ref_axis',(1.,0.,0.)) ;
#131570=DIRECTION('center_axis',(0.,0.,-1.)) ;
#131571=DIRECTION('ref_axis',(-1.,0.,0.)) ;
#131572=DIRECTION('center_axis',(0.,-1.,0.)) ;
#131573=DIRECTION('ref_axis',(0.,0.,-1.)) ;
#131574=DIRECTION('center_axis',(0.,-1.,0.)) ;
#131575=DIRECTION('ref_axis',(0.,0.,-1.)) ;
#131576=DIRECTION('center_axis',(0.,-1.,0.)) ;
#131577=DIRECTION('ref_axis',(0.,0.,-1.)) ;
#131578=DIRECTION('center_axis',(0.,0.,1.)) ;
#131579=DIRECTION('ref_axis',(1.,0.,0.)) ;
#131580=DIRECTION('center_axis',(0.,0.,-1.)) ;
#131581=DIRECTION('ref_axis',(-1.,0.,0.)) ;
#131582=DIRECTION('center_axis',(0.,0.,1.)) ;
#131583=DIRECTION('ref_axis',(1.,0.,0.)) ;
#131584=DIRECTION('center_axis',(0.,-1.,0.)) ;
#131585=DIRECTION('ref_axis',(0.,0.,-1.)) ;
#131586=DIRECTION('center_axis',(0.,-1.,0.)) ;
#131587=DIRECTION('ref_axis',(0.,0.,-1.)) ;
#131588=DIRECTION('center_axis',(0.,1.,0.)) ;
#131589=DIRECTION('ref_axis',(1.,0.,0.)) ;
#131590=DIRECTION('center_axis',(-1.,0.,0.)) ;
#131591=DIRECTION('ref_axis',(0.,0.,-1.)) ;
#131592=DIRECTION('center_axis',(0.,1.,0.)) ;
#131593=DIRECTION('ref_axis',(1.,0.,0.)) ;
#131594=DIRECTION('center_axis',(-1.,0.,0.)) ;
#131595=DIRECTION('ref_axis',(0.,0.,-1.)) ;
#131596=DIRECTION('center_axis',(0.,-1.,0.)) ;
#131597=DIRECTION('ref_axis',(0.,0.,-1.)) ;
#131598=DIRECTION('center_axis',(0.,-1.,0.)) ;
#131599=DIRECTION('ref_axis',(0.,0.,-1.)) ;
#131600=DIRECTION('center_axis',(-1.,0.,0.)) ;
#131601=DIRECTION('ref_axis',(0.,0.,1.)) ;
#131602=DIRECTION('center_axis',(-1.,0.,0.)) ;
#131603=DIRECTION('ref_axis',(0.,0.,1.)) ;
#131604=DIRECTION('center_axis',(1.,0.,0.)) ;
#131605=DIRECTION('ref_axis',(0.,0.,-1.)) ;
#131606=DIRECTION('center_axis',(-1.,0.,0.)) ;
#131607=DIRECTION('ref_axis',(0.,0.,1.)) ;
#131608=DIRECTION('center_axis',(0.,-1.,0.)) ;
#131609=DIRECTION('ref_axis',(0.,0.,-1.)) ;
#131610=DIRECTION('center_axis',(0.,-1.,0.)) ;
#131611=DIRECTION('ref_axis',(0.,0.,-1.)) ;
#131612=DIRECTION('center_axis',(0.,1.,0.)) ;
#131613=DIRECTION('ref_axis',(1.,0.,0.)) ;
#131614=DIRECTION('center_axis',(0.,0.,-1.)) ;
#131615=DIRECTION('ref_axis',(1.,0.,0.)) ;
#131616=DIRECTION('center_axis',(0.,1.,0.)) ;
#131617=DIRECTION('ref_axis',(1.,0.,0.)) ;
#131618=DIRECTION('center_axis',(0.,0.,1.)) ;
#131619=DIRECTION('ref_axis',(-1.,0.,0.)) ;
#131620=DIRECTION('center_axis',(0.,0.,-1.)) ;
#131621=DIRECTION('ref_axis',(-1.,0.,0.)) ;
#131622=DIRECTION('center_axis',(1.,1.31418445149758E-16,-2.16840434497101E-16)) ;
#131623=DIRECTION('ref_axis',(-2.16840434497101E-16,-2.8496832747207E-32,
-1.)) ;
#131624=DIRECTION('center_axis',(1.,0.,0.)) ;
#131625=DIRECTION('ref_axis',(0.,0.,-1.)) ;
#131626=DIRECTION('center_axis',(-1.,0.,0.)) ;
#131627=DIRECTION('ref_axis',(0.,0.,1.)) ;
#131628=DIRECTION('center_axis',(-1.31418445149758E-16,1.,0.)) ;
#131629=DIRECTION('ref_axis',(-1.,0.,0.)) ;
#131630=DIRECTION('center_axis',(0.,0.,1.)) ;
#131631=DIRECTION('ref_axis',(-1.,0.,0.)) ;
#131632=DIRECTION('center_axis',(-1.31418445149758E-16,1.,0.)) ;
#131633=DIRECTION('ref_axis',(-1.,-1.31418445149758E-16,0.)) ;
#131634=DIRECTION('center_axis',(-1.31418445149758E-16,1.,0.)) ;
#131635=DIRECTION('ref_axis',(-1.,0.,0.)) ;
#131636=DIRECTION('center_axis',(-1.31418445149758E-16,1.,0.)) ;
#131637=DIRECTION('ref_axis',(-1.,-1.31418445149758E-16,0.)) ;
#131638=DIRECTION('center_axis',(0.,0.,1.)) ;
#131639=DIRECTION('ref_axis',(-1.,0.,0.)) ;
#131640=DIRECTION('center_axis',(-4.33680868994202E-16,-5.69936654944139E-32,
-1.)) ;
#131641=DIRECTION('ref_axis',(-1.,2.47170623787823E-47,4.33680868994202E-16)) ;
#131642=DIRECTION('center_axis',(0.,0.,1.)) ;
#131643=DIRECTION('ref_axis',(1.,0.,0.)) ;
#131644=DIRECTION('center_axis',(-1.31418445149758E-16,-1.,0.)) ;
#131645=DIRECTION('ref_axis',(1.,-1.31418445149758E-16,0.)) ;
#131646=DIRECTION('center_axis',(0.,1.,0.)) ;
#131647=DIRECTION('ref_axis',(0.,0.,1.)) ;
#131648=DIRECTION('center_axis',(-1.,0.,2.16840434497101E-16)) ;
#131649=DIRECTION('ref_axis',(2.16840434497101E-16,0.,1.)) ;
#131650=DIRECTION('center_axis',(-1.,0.,0.)) ;
#131651=DIRECTION('ref_axis',(0.,0.,1.)) ;
#131652=DIRECTION('center_axis',(1.,0.,0.)) ;
#131653=DIRECTION('ref_axis',(0.,0.,-1.)) ;
#131654=DIRECTION('center_axis',(-1.31418445149758E-16,-1.,0.)) ;
#131655=DIRECTION('ref_axis',(1.,-1.31418445149758E-16,0.)) ;
#131656=DIRECTION('center_axis',(0.,1.,0.)) ;
#131657=DIRECTION('ref_axis',(0.,0.,1.)) ;
#131658=DIRECTION('center_axis',(2.16840434497101E-16,2.8496832747207E-32,
1.)) ;
#131659=DIRECTION('ref_axis',(1.,-6.17926559469557E-48,-2.16840434497101E-16)) ;
#131660=DIRECTION('center_axis',(0.,0.,1.)) ;
#131661=DIRECTION('ref_axis',(1.,0.,0.)) ;
#131662=DIRECTION('center_axis',(-1.,-1.31418445149758E-16,-2.16840434497101E-16)) ;
#131663=DIRECTION('ref_axis',(-2.16840434497101E-16,-2.8496832747207E-32,
1.)) ;
#131664=DIRECTION('center_axis',(-1.,0.,0.)) ;
#131665=DIRECTION('ref_axis',(0.,0.,1.)) ;
#131666=DIRECTION('center_axis',(1.,0.,0.)) ;
#131667=DIRECTION('ref_axis',(0.,0.,-1.)) ;
#131668=DIRECTION('center_axis',(-1.31418445149758E-16,1.,0.)) ;
#131669=DIRECTION('ref_axis',(-1.,0.,0.)) ;
#131670=DIRECTION('center_axis',(-1.31418445149758E-16,1.,0.)) ;
#131671=DIRECTION('ref_axis',(-1.,-1.31418445149758E-16,0.)) ;
#131672=DIRECTION('center_axis',(0.,1.,0.)) ;
#131673=DIRECTION('ref_axis',(1.,0.,0.)) ;
#131674=DIRECTION('center_axis',(0.,0.,-1.)) ;
#131675=DIRECTION('ref_axis',(1.,0.,0.)) ;
#131676=DIRECTION('center_axis',(0.,1.,0.)) ;
#131677=DIRECTION('ref_axis',(1.,0.,0.)) ;
#131678=DIRECTION('center_axis',(0.,0.,-1.)) ;
#131679=DIRECTION('ref_axis',(1.,0.,0.)) ;
#131680=DIRECTION('center_axis',(-1.31418445149758E-16,1.,0.)) ;
#131681=DIRECTION('ref_axis',(-1.,0.,0.)) ;
#131682=DIRECTION('center_axis',(-1.31418445149758E-16,1.,0.)) ;
#131683=DIRECTION('ref_axis',(-1.,-1.31418445149758E-16,0.)) ;
#131684=DIRECTION('center_axis',(-1.31418445149758E-16,-1.,0.)) ;
#131685=DIRECTION('ref_axis',(1.,-1.31418445149758E-16,0.)) ;
#131686=DIRECTION('center_axis',(0.,1.,0.)) ;
#131687=DIRECTION('ref_axis',(0.,0.,1.)) ;
#131688=DIRECTION('center_axis',(4.33680868994202E-16,0.,1.)) ;
#131689=DIRECTION('ref_axis',(1.,0.,-4.33680868994202E-16)) ;
#131690=DIRECTION('center_axis',(0.,0.,-1.)) ;
#131691=DIRECTION('ref_axis',(-1.,0.,0.)) ;
#131692=DIRECTION('center_axis',(-2.16840434497101E-16,0.,-1.)) ;
#131693=DIRECTION('ref_axis',(-1.,0.,2.16840434497101E-16)) ;
#131694=DIRECTION('center_axis',(0.,0.,-1.)) ;
#131695=DIRECTION('ref_axis',(-1.,0.,0.)) ;
#131696=DIRECTION('center_axis',(-1.31418445149758E-16,-1.,0.)) ;
#131697=DIRECTION('ref_axis',(1.,-1.31418445149758E-16,0.)) ;
#131698=DIRECTION('center_axis',(0.,1.,0.)) ;
#131699=DIRECTION('ref_axis',(0.,0.,1.)) ;
#131700=DIRECTION('center_axis',(0.,1.,0.)) ;
#131701=DIRECTION('ref_axis',(1.,0.,0.)) ;
#131702=DIRECTION('center_axis',(-1.,0.,0.)) ;
#131703=DIRECTION('ref_axis',(0.,0.,-1.)) ;
#131704=DIRECTION('center_axis',(0.,1.,0.)) ;
#131705=DIRECTION('ref_axis',(1.,0.,0.)) ;
#131706=DIRECTION('center_axis',(1.,0.,0.)) ;
#131707=DIRECTION('ref_axis',(0.,0.,1.)) ;
#131708=DIRECTION('center_axis',(1.,0.,2.16840434497101E-16)) ;
#131709=DIRECTION('ref_axis',(2.16840434497101E-16,0.,-1.)) ;
#131710=DIRECTION('center_axis',(0.,1.,0.)) ;
#131711=DIRECTION('ref_axis',(0.,0.,1.)) ;
#131712=DIRECTION('center_axis',(0.,1.,0.)) ;
#131713=DIRECTION('ref_axis',(0.,0.,1.)) ;
#131714=DIRECTION('center_axis',(0.,0.,-1.)) ;
#131715=DIRECTION('ref_axis',(-1.,0.,0.)) ;
#131716=DIRECTION('center_axis',(0.,0.,1.)) ;
#131717=DIRECTION('ref_axis',(1.,0.,0.)) ;
#131718=DIRECTION('center_axis',(0.,0.,-1.)) ;
#131719=DIRECTION('ref_axis',(-1.,0.,0.)) ;
#131720=DIRECTION('center_axis',(0.,1.,0.)) ;
#131721=DIRECTION('ref_axis',(0.,0.,1.)) ;
#131722=DIRECTION('center_axis',(0.,1.,0.)) ;
#131723=DIRECTION('ref_axis',(0.,0.,1.)) ;
#131724=DIRECTION('center_axis',(0.,1.,0.)) ;
#131725=DIRECTION('ref_axis',(1.,0.,0.)) ;
#131726=DIRECTION('center_axis',(-1.,0.,0.)) ;
#131727=DIRECTION('ref_axis',(0.,0.,-1.)) ;
#131728=DIRECTION('center_axis',(0.,1.,0.)) ;
#131729=DIRECTION('ref_axis',(1.,0.,0.)) ;
#131730=DIRECTION('center_axis',(-1.,0.,0.)) ;
#131731=DIRECTION('ref_axis',(0.,0.,-1.)) ;
#131732=DIRECTION('center_axis',(0.,1.,0.)) ;
#131733=DIRECTION('ref_axis',(0.,0.,1.)) ;
#131734=DIRECTION('center_axis',(0.,1.,0.)) ;
#131735=DIRECTION('ref_axis',(0.,0.,1.)) ;
#131736=DIRECTION('center_axis',(-1.,0.,0.)) ;
#131737=DIRECTION('ref_axis',(0.,0.,1.)) ;
#131738=DIRECTION('center_axis',(-1.,0.,0.)) ;
#131739=DIRECTION('ref_axis',(0.,0.,1.)) ;
#131740=DIRECTION('center_axis',(1.,0.,0.)) ;
#131741=DIRECTION('ref_axis',(0.,0.,-1.)) ;
#131742=DIRECTION('center_axis',(-1.,0.,0.)) ;
#131743=DIRECTION('ref_axis',(0.,0.,1.)) ;
#131744=DIRECTION('center_axis',(0.,1.,0.)) ;
#131745=DIRECTION('ref_axis',(0.,0.,1.)) ;
#131746=DIRECTION('center_axis',(0.,1.,0.)) ;
#131747=DIRECTION('ref_axis',(0.,0.,1.)) ;
#131748=DIRECTION('center_axis',(0.,1.,0.)) ;
#131749=DIRECTION('ref_axis',(1.,0.,0.)) ;
#131750=DIRECTION('center_axis',(0.,0.,1.)) ;
#131751=DIRECTION('ref_axis',(-1.,0.,0.)) ;
#131752=DIRECTION('center_axis',(0.,1.,0.)) ;
#131753=DIRECTION('ref_axis',(1.,0.,0.)) ;
#131754=DIRECTION('center_axis',(0.,0.,-1.)) ;
#131755=DIRECTION('ref_axis',(1.,0.,0.)) ;
#131756=DIRECTION('center_axis',(0.,0.,1.)) ;
#131757=DIRECTION('ref_axis',(1.,0.,0.)) ;
#131758=DIRECTION('center_axis',(0.,0.,1.)) ;
#131759=DIRECTION('ref_axis',(1.,0.,0.)) ;
#131760=DIRECTION('center_axis',(0.,0.,-1.)) ;
#131761=DIRECTION('ref_axis',(-1.,0.,0.)) ;
#131762=DIRECTION('center_axis',(0.,0.,1.)) ;
#131763=DIRECTION('ref_axis',(1.,0.,0.)) ;
#131764=DIRECTION('center_axis',(1.,0.,0.)) ;
#131765=DIRECTION('ref_axis',(0.,0.,-1.)) ;
#131766=DIRECTION('center_axis',(1.,0.,0.)) ;
#131767=DIRECTION('ref_axis',(0.,0.,-1.)) ;
#131768=DIRECTION('center_axis',(1.,0.,0.)) ;
#131769=DIRECTION('ref_axis',(0.,0.,-1.)) ;
#131770=DIRECTION('center_axis',(1.,0.,8.67361737988379E-15)) ;
#131771=DIRECTION('ref_axis',(8.67361737988379E-15,0.,-1.)) ;
#131772=DIRECTION('center_axis',(1.,0.,0.)) ;
#131773=DIRECTION('ref_axis',(0.,0.,-1.)) ;
#131774=DIRECTION('center_axis',(1.,0.,1.73472347597676E-14)) ;
#131775=DIRECTION('ref_axis',(1.73472347597676E-14,0.,-1.)) ;
#131776=DIRECTION('center_axis',(-1.,0.,0.)) ;
#131777=DIRECTION('ref_axis',(0.,0.,1.)) ;
#131778=DIRECTION('center_axis',(1.,0.,0.)) ;
#131779=DIRECTION('ref_axis',(0.,0.,-1.)) ;
#131780=DIRECTION('center_axis',(1.,0.,0.)) ;
#131781=DIRECTION('ref_axis',(0.,0.,-1.)) ;
#131782=DIRECTION('center_axis',(0.,0.,-1.)) ;
#131783=DIRECTION('ref_axis',(-1.,0.,0.)) ;
#131784=DIRECTION('center_axis',(1.,0.,0.)) ;
#131785=DIRECTION('ref_axis',(0.,0.,-1.)) ;
#131786=DIRECTION('center_axis',(0.,0.,1.)) ;
#131787=DIRECTION('ref_axis',(1.,0.,0.)) ;
#131788=DIRECTION('center_axis',(0.,0.,-1.)) ;
#131789=DIRECTION('ref_axis',(-1.,0.,0.)) ;
#131790=DIRECTION('center_axis',(-0.422618261740697,5.55398348498559E-17,
0.906307787036651)) ;
#131791=DIRECTION('ref_axis',(0.906307787036651,6.51773046476477E-31,0.422618261740697)) ;
#131792=DIRECTION('center_axis',(0.422618261740697,-5.55398348498559E-17,
-0.906307787036651)) ;
#131793=DIRECTION('ref_axis',(-0.906307787036651,-6.46086972436398E-31,
-0.422618261740697)) ;
#131794=DIRECTION('center_axis',(-0.422618261740697,5.55398348498559E-17,
0.906307787036651)) ;
#131795=DIRECTION('ref_axis',(0.906307787036651,6.46086972436398E-31,0.422618261740697)) ;
#131796=DIRECTION('center_axis',(0.422618261740697,-5.55398348498559E-17,
-0.906307787036651)) ;
#131797=DIRECTION('ref_axis',(-0.906307787036651,-6.46086972436398E-31,
-0.422618261740697)) ;
#131798=DIRECTION('center_axis',(0.,0.,1.)) ;
#131799=DIRECTION('ref_axis',(1.,0.,0.)) ;
#131800=DIRECTION('center_axis',(7.01133629567814E-33,-8.97270763436279E-17,
-1.)) ;
#131801=DIRECTION('ref_axis',(-6.29106707073161E-49,-1.,8.97270763436279E-17)) ;
#131802=DIRECTION('center_axis',(7.01133629567814E-33,-8.97270763436279E-17,
1.)) ;
#131803=DIRECTION('ref_axis',(6.29106707073161E-49,1.,8.97270763436279E-17)) ;
#131804=DIRECTION('center_axis',(0.,0.,1.)) ;
#131805=DIRECTION('ref_axis',(1.,0.,0.)) ;
#131806=DIRECTION('center_axis',(7.01133629567814E-33,-8.97270763436279E-17,
-1.)) ;
#131807=DIRECTION('ref_axis',(-6.29106707073161E-49,-1.,8.97270763436279E-17)) ;
#131808=DIRECTION('center_axis',(7.01133629567814E-33,-8.97270763436279E-17,
1.)) ;
#131809=DIRECTION('ref_axis',(6.29106707073161E-49,1.,8.97270763436279E-17)) ;
#131810=DIRECTION('center_axis',(0.,0.,1.)) ;
#131811=DIRECTION('ref_axis',(1.,0.,0.)) ;
#131812=DIRECTION('center_axis',(7.01133629567814E-33,-8.97270763436279E-17,
-1.)) ;
#131813=DIRECTION('ref_axis',(-6.29106707073161E-49,-1.,8.97270763436279E-17)) ;
#131814=DIRECTION('center_axis',(7.01133629567814E-33,-8.97270763436279E-17,
1.)) ;
#131815=DIRECTION('ref_axis',(6.29106707073161E-49,1.,8.97270763436279E-17)) ;
#131816=DIRECTION('center_axis',(0.,0.,1.)) ;
#131817=DIRECTION('ref_axis',(1.,0.,0.)) ;
#131818=DIRECTION('center_axis',(7.01133629567814E-33,-8.97270763436279E-17,
-1.)) ;
#131819=DIRECTION('ref_axis',(-6.29106707073161E-49,-1.,8.97270763436279E-17)) ;
#131820=DIRECTION('center_axis',(7.01133629567814E-33,-8.97270763436279E-17,
1.)) ;
#131821=DIRECTION('ref_axis',(6.29106707073161E-49,1.,8.97270763436279E-17)) ;
#131822=DIRECTION('center_axis',(0.,0.,1.)) ;
#131823=DIRECTION('ref_axis',(1.,0.,0.)) ;
#131824=DIRECTION('center_axis',(7.01133629567814E-33,-8.97270763436279E-17,
-1.)) ;
#131825=DIRECTION('ref_axis',(-6.29106707073161E-49,-1.,8.97270763436279E-17)) ;
#131826=DIRECTION('center_axis',(7.01133629567814E-33,-8.97270763436279E-17,
1.)) ;
#131827=DIRECTION('ref_axis',(6.29106707073161E-49,1.,8.97270763436279E-17)) ;
#131828=DIRECTION('center_axis',(0.,0.,1.)) ;
#131829=DIRECTION('ref_axis',(1.,0.,0.)) ;
#131830=DIRECTION('center_axis',(7.01133629567814E-33,-8.97270763436279E-17,
-1.)) ;
#131831=DIRECTION('ref_axis',(-6.29106707073161E-49,-1.,8.97270763436279E-17)) ;
#131832=DIRECTION('center_axis',(7.01133629567814E-33,-8.97270763436279E-17,
1.)) ;
#131833=DIRECTION('ref_axis',(6.29106707073161E-49,1.,8.97270763436279E-17)) ;
#131834=DIRECTION('center_axis',(0.,0.,1.)) ;
#131835=DIRECTION('ref_axis',(1.,0.,0.)) ;
#131836=DIRECTION('center_axis',(7.01133629567814E-33,-8.97270763436279E-17,
-1.)) ;
#131837=DIRECTION('ref_axis',(-6.29106707073161E-49,-1.,8.97270763436279E-17)) ;
#131838=DIRECTION('center_axis',(7.01133629567814E-33,-8.97270763436279E-17,
1.)) ;
#131839=DIRECTION('ref_axis',(6.29106707073161E-49,1.,8.97270763436279E-17)) ;
#131840=DIRECTION('center_axis',(0.,0.,1.)) ;
#131841=DIRECTION('ref_axis',(1.,0.,0.)) ;
#131842=DIRECTION('center_axis',(7.01133629567814E-33,-8.97270763436279E-17,
-1.)) ;
#131843=DIRECTION('ref_axis',(-6.29106707073161E-49,-1.,8.97270763436279E-17)) ;
#131844=DIRECTION('center_axis',(7.01133629567814E-33,-8.97270763436279E-17,
1.)) ;
#131845=DIRECTION('ref_axis',(6.29106707073161E-49,1.,8.97270763436279E-17)) ;
#131846=DIRECTION('center_axis',(0.,0.,1.)) ;
#131847=DIRECTION('ref_axis',(1.,0.,0.)) ;
#131848=DIRECTION('center_axis',(7.01133629567814E-33,-8.97270763436279E-17,
-1.)) ;
#131849=DIRECTION('ref_axis',(-6.29106707073161E-49,-1.,8.97270763436279E-17)) ;
#131850=DIRECTION('center_axis',(7.01133629567814E-33,-8.97270763436279E-17,
1.)) ;
#131851=DIRECTION('ref_axis',(6.29106707073161E-49,1.,8.97270763436279E-17)) ;
#131852=DIRECTION('center_axis',(1.,0.,0.)) ;
#131853=DIRECTION('ref_axis',(0.,0.,-1.)) ;
#131854=DIRECTION('center_axis',(0.,0.,1.)) ;
#131855=DIRECTION('ref_axis',(1.,0.,0.)) ;
#131856=DIRECTION('center_axis',(0.,4.8455963016112E-16,1.)) ;
#131857=DIRECTION('ref_axis',(0.,-1.,4.8455963016112E-16)) ;
#131858=DIRECTION('center_axis',(0.,0.,1.)) ;
#131859=DIRECTION('ref_axis',(1.,0.,0.)) ;
#131860=DIRECTION('center_axis',(0.,0.,1.)) ;
#131861=DIRECTION('ref_axis',(1.,0.,0.)) ;
#131862=DIRECTION('center_axis',(0.,0.,1.)) ;
#131863=DIRECTION('ref_axis',(1.,0.,0.)) ;
#131864=DIRECTION('center_axis',(1.,0.,0.)) ;
#131865=DIRECTION('ref_axis',(0.,0.,-1.)) ;
#131866=DIRECTION('center_axis',(1.,0.,0.)) ;
#131867=DIRECTION('ref_axis',(0.,0.,-1.)) ;
#131868=DIRECTION('center_axis',(1.,0.,0.)) ;
#131869=DIRECTION('ref_axis',(0.,0.,-1.)) ;
#131870=DIRECTION('center_axis',(0.,0.,1.)) ;
#131871=DIRECTION('ref_axis',(1.,0.,0.)) ;
#131872=DIRECTION('center_axis',(0.,4.8455963016112E-16,1.)) ;
#131873=DIRECTION('ref_axis',(0.,-1.,4.8455963016112E-16)) ;
#131874=DIRECTION('center_axis',(0.,0.,1.)) ;
#131875=DIRECTION('ref_axis',(1.,0.,0.)) ;
#131876=DIRECTION('center_axis',(0.,0.,1.)) ;
#131877=DIRECTION('ref_axis',(1.,0.,0.)) ;
#131878=DIRECTION('center_axis',(0.,0.,1.)) ;
#131879=DIRECTION('ref_axis',(1.,0.,0.)) ;
#131880=DIRECTION('center_axis',(1.,0.,0.)) ;
#131881=DIRECTION('ref_axis',(0.,0.,-1.)) ;
#131882=DIRECTION('center_axis',(1.,0.,0.)) ;
#131883=DIRECTION('ref_axis',(0.,0.,-1.)) ;
#131884=DIRECTION('center_axis',(0.,0.,1.)) ;
#131885=DIRECTION('ref_axis',(1.,0.,0.)) ;
#131886=DIRECTION('center_axis',(0.,4.8455963016112E-16,1.)) ;
#131887=DIRECTION('ref_axis',(0.,-1.,4.8455963016112E-16)) ;
#131888=DIRECTION('center_axis',(0.,0.,1.)) ;
#131889=DIRECTION('ref_axis',(1.,0.,0.)) ;
#131890=DIRECTION('center_axis',(0.,0.,1.)) ;
#131891=DIRECTION('ref_axis',(1.,0.,0.)) ;
#131892=DIRECTION('center_axis',(0.,0.,1.)) ;
#131893=DIRECTION('ref_axis',(1.,0.,0.)) ;
#131894=DIRECTION('center_axis',(1.,0.,0.)) ;
#131895=DIRECTION('ref_axis',(0.,0.,-1.)) ;
#131896=DIRECTION('center_axis',(1.,0.,0.)) ;
#131897=DIRECTION('ref_axis',(0.,0.,-1.)) ;
#131898=DIRECTION('center_axis',(0.,0.,1.)) ;
#131899=DIRECTION('ref_axis',(1.,0.,0.)) ;
#131900=DIRECTION('center_axis',(0.,4.8455963016112E-16,1.)) ;
#131901=DIRECTION('ref_axis',(0.,-1.,4.8455963016112E-16)) ;
#131902=DIRECTION('center_axis',(0.,0.,1.)) ;
#131903=DIRECTION('ref_axis',(1.,0.,0.)) ;
#131904=DIRECTION('center_axis',(0.,0.,1.)) ;
#131905=DIRECTION('ref_axis',(1.,0.,0.)) ;
#131906=DIRECTION('center_axis',(0.,0.,1.)) ;
#131907=DIRECTION('ref_axis',(1.,0.,0.)) ;
#131908=DIRECTION('center_axis',(1.,0.,0.)) ;
#131909=DIRECTION('ref_axis',(0.,0.,-1.)) ;
#131910=DIRECTION('center_axis',(1.,0.,0.)) ;
#131911=DIRECTION('ref_axis',(0.,0.,-1.)) ;
#131912=DIRECTION('center_axis',(0.,0.,1.)) ;
#131913=DIRECTION('ref_axis',(1.,0.,0.)) ;
#131914=DIRECTION('center_axis',(0.,4.8455963016112E-16,1.)) ;
#131915=DIRECTION('ref_axis',(0.,-1.,4.8455963016112E-16)) ;
#131916=DIRECTION('center_axis',(0.,0.,1.)) ;
#131917=DIRECTION('ref_axis',(1.,0.,0.)) ;
#131918=DIRECTION('center_axis',(0.,0.,1.)) ;
#131919=DIRECTION('ref_axis',(1.,0.,0.)) ;
#131920=DIRECTION('center_axis',(0.,0.,1.)) ;
#131921=DIRECTION('ref_axis',(1.,0.,0.)) ;
#131922=DIRECTION('center_axis',(1.,0.,0.)) ;
#131923=DIRECTION('ref_axis',(0.,0.,-1.)) ;
#131924=DIRECTION('center_axis',(1.,0.,0.)) ;
#131925=DIRECTION('ref_axis',(0.,0.,-1.)) ;
#131926=DIRECTION('center_axis',(0.,0.,1.)) ;
#131927=DIRECTION('ref_axis',(1.,0.,0.)) ;
#131928=DIRECTION('center_axis',(0.,4.8455963016112E-16,1.)) ;
#131929=DIRECTION('ref_axis',(0.,-1.,4.8455963016112E-16)) ;
#131930=DIRECTION('center_axis',(0.,0.,1.)) ;
#131931=DIRECTION('ref_axis',(1.,0.,0.)) ;
#131932=DIRECTION('center_axis',(0.,0.,1.)) ;
#131933=DIRECTION('ref_axis',(1.,0.,0.)) ;
#131934=DIRECTION('center_axis',(0.,0.,1.)) ;
#131935=DIRECTION('ref_axis',(1.,0.,0.)) ;
#131936=DIRECTION('center_axis',(1.,0.,0.)) ;
#131937=DIRECTION('ref_axis',(0.,0.,-1.)) ;
#131938=DIRECTION('center_axis',(1.,0.,0.)) ;
#131939=DIRECTION('ref_axis',(0.,0.,-1.)) ;
#131940=DIRECTION('center_axis',(0.,0.,1.)) ;
#131941=DIRECTION('ref_axis',(1.,0.,0.)) ;
#131942=DIRECTION('center_axis',(0.,4.8455963016112E-16,1.)) ;
#131943=DIRECTION('ref_axis',(0.,-1.,4.8455963016112E-16)) ;
#131944=DIRECTION('center_axis',(0.,0.,1.)) ;
#131945=DIRECTION('ref_axis',(1.,0.,0.)) ;
#131946=DIRECTION('center_axis',(0.,0.,1.)) ;
#131947=DIRECTION('ref_axis',(1.,0.,0.)) ;
#131948=DIRECTION('center_axis',(0.,0.,1.)) ;
#131949=DIRECTION('ref_axis',(1.,0.,0.)) ;
#131950=DIRECTION('center_axis',(1.,0.,0.)) ;
#131951=DIRECTION('ref_axis',(0.,0.,-1.)) ;
#131952=DIRECTION('center_axis',(1.,0.,0.)) ;
#131953=DIRECTION('ref_axis',(0.,0.,-1.)) ;
#131954=DIRECTION('center_axis',(0.,0.,1.)) ;
#131955=DIRECTION('ref_axis',(1.,0.,0.)) ;
#131956=DIRECTION('center_axis',(0.,4.8455963016112E-16,1.)) ;
#131957=DIRECTION('ref_axis',(0.,-1.,4.8455963016112E-16)) ;
#131958=DIRECTION('center_axis',(0.,0.,1.)) ;
#131959=DIRECTION('ref_axis',(1.,0.,0.)) ;
#131960=DIRECTION('center_axis',(0.,0.,1.)) ;
#131961=DIRECTION('ref_axis',(1.,0.,0.)) ;
#131962=DIRECTION('center_axis',(0.,0.,1.)) ;
#131963=DIRECTION('ref_axis',(1.,0.,0.)) ;
#131964=DIRECTION('center_axis',(1.,0.,0.)) ;
#131965=DIRECTION('ref_axis',(0.,0.,-1.)) ;
#131966=DIRECTION('center_axis',(0.,4.8455963016112E-16,1.)) ;
#131967=DIRECTION('ref_axis',(0.,-1.,4.8455963016112E-16)) ;
#131968=DIRECTION('center_axis',(0.,4.8455963016112E-16,1.)) ;
#131969=DIRECTION('ref_axis',(0.,-1.,4.8455963016112E-16)) ;
#131970=DIRECTION('center_axis',(0.,0.,1.)) ;
#131971=DIRECTION('ref_axis',(1.,0.,0.)) ;
#131972=DIRECTION('center_axis',(0.,0.,1.)) ;
#131973=DIRECTION('ref_axis',(1.,0.,0.)) ;
#131974=DIRECTION('center_axis',(1.,0.,0.)) ;
#131975=DIRECTION('ref_axis',(0.,0.,-1.)) ;
#131976=DIRECTION('center_axis',(-7.01133629567814E-33,8.97270763436279E-17,
1.)) ;
#131977=DIRECTION('ref_axis',(0.,-1.,0.)) ;
#131978=DIRECTION('center_axis',(1.,0.,0.)) ;
#131979=DIRECTION('ref_axis',(0.,0.,-1.)) ;
#131980=DIRECTION('center_axis',(-1.,0.,-7.01133629567814E-33)) ;
#131981=DIRECTION('ref_axis',(-7.01133629567814E-33,0.,1.)) ;
#131982=DIRECTION('center_axis',(1.,0.,0.)) ;
#131983=DIRECTION('ref_axis',(0.,0.,-1.)) ;
#131984=DIRECTION('center_axis',(1.,0.,0.)) ;
#131985=DIRECTION('ref_axis',(0.,0.,-1.)) ;
#131986=DIRECTION('center_axis',(0.,1.,0.)) ;
#131987=DIRECTION('ref_axis',(1.,0.,0.)) ;
#131988=DIRECTION('center_axis',(-7.01133629567814E-33,8.97270763436279E-17,
-1.)) ;
#131989=DIRECTION('ref_axis',(0.,1.,0.)) ;
#131990=DIRECTION('center_axis',(1.,0.,0.)) ;
#131991=DIRECTION('ref_axis',(0.,0.,-1.)) ;
#131992=DIRECTION('center_axis',(-1.,0.,7.01133629567814E-33)) ;
#131993=DIRECTION('ref_axis',(7.01133629567814E-33,0.,1.)) ;
#131994=DIRECTION('center_axis',(1.,0.,0.)) ;
#131995=DIRECTION('ref_axis',(0.,0.,-1.)) ;
#131996=DIRECTION('center_axis',(1.,0.,0.)) ;
#131997=DIRECTION('ref_axis',(0.,0.,-1.)) ;
#131998=DIRECTION('center_axis',(0.,1.,0.)) ;
#131999=DIRECTION('ref_axis',(1.,0.,0.)) ;
#132000=DIRECTION('center_axis',(-7.01133629567814E-33,8.97270763436279E-17,
1.)) ;
#132001=DIRECTION('ref_axis',(0.,-1.,0.)) ;
#132002=DIRECTION('center_axis',(1.,0.,0.)) ;
#132003=DIRECTION('ref_axis',(0.,0.,-1.)) ;
#132004=DIRECTION('center_axis',(-1.,0.,-7.01133629567814E-33)) ;
#132005=DIRECTION('ref_axis',(-7.01133629567814E-33,0.,1.)) ;
#132006=DIRECTION('center_axis',(1.,0.,0.)) ;
#132007=DIRECTION('ref_axis',(0.,0.,-1.)) ;
#132008=DIRECTION('center_axis',(1.,0.,0.)) ;
#132009=DIRECTION('ref_axis',(0.,0.,-1.)) ;
#132010=DIRECTION('center_axis',(0.,1.,0.)) ;
#132011=DIRECTION('ref_axis',(1.,0.,0.)) ;
#132012=DIRECTION('center_axis',(-7.01133629567814E-33,8.97270763436279E-17,
-1.)) ;
#132013=DIRECTION('ref_axis',(0.,1.,0.)) ;
#132014=DIRECTION('center_axis',(1.,0.,0.)) ;
#132015=DIRECTION('ref_axis',(0.,0.,-1.)) ;
#132016=DIRECTION('center_axis',(-1.,0.,7.01133629567814E-33)) ;
#132017=DIRECTION('ref_axis',(7.01133629567814E-33,0.,1.)) ;
#132018=DIRECTION('center_axis',(1.,0.,0.)) ;
#132019=DIRECTION('ref_axis',(0.,0.,-1.)) ;
#132020=DIRECTION('center_axis',(1.,0.,0.)) ;
#132021=DIRECTION('ref_axis',(0.,0.,-1.)) ;
#132022=DIRECTION('center_axis',(0.,1.,0.)) ;
#132023=DIRECTION('ref_axis',(1.,0.,0.)) ;
#132024=DIRECTION('center_axis',(-7.01133629567814E-33,8.97270763436279E-17,
1.)) ;
#132025=DIRECTION('ref_axis',(0.,-1.,0.)) ;
#132026=DIRECTION('center_axis',(1.,0.,0.)) ;
#132027=DIRECTION('ref_axis',(0.,0.,-1.)) ;
#132028=DIRECTION('center_axis',(-1.,0.,-7.01133629567814E-33)) ;
#132029=DIRECTION('ref_axis',(-7.01133629567814E-33,0.,1.)) ;
#132030=DIRECTION('center_axis',(1.,0.,0.)) ;
#132031=DIRECTION('ref_axis',(0.,0.,-1.)) ;
#132032=DIRECTION('center_axis',(1.,0.,0.)) ;
#132033=DIRECTION('ref_axis',(0.,0.,-1.)) ;
#132034=DIRECTION('center_axis',(0.,1.,0.)) ;
#132035=DIRECTION('ref_axis',(1.,0.,0.)) ;
#132036=DIRECTION('center_axis',(-7.01133629567814E-33,8.97270763436279E-17,
-1.)) ;
#132037=DIRECTION('ref_axis',(0.,1.,0.)) ;
#132038=DIRECTION('center_axis',(1.,0.,0.)) ;
#132039=DIRECTION('ref_axis',(0.,0.,-1.)) ;
#132040=DIRECTION('center_axis',(-1.,0.,7.01133629567814E-33)) ;
#132041=DIRECTION('ref_axis',(7.01133629567814E-33,0.,1.)) ;
#132042=DIRECTION('center_axis',(1.,0.,0.)) ;
#132043=DIRECTION('ref_axis',(0.,0.,-1.)) ;
#132044=DIRECTION('center_axis',(1.,0.,0.)) ;
#132045=DIRECTION('ref_axis',(0.,0.,-1.)) ;
#132046=DIRECTION('center_axis',(0.,1.,0.)) ;
#132047=DIRECTION('ref_axis',(1.,0.,0.)) ;
#132048=DIRECTION('center_axis',(-7.01133629567814E-33,8.97270763436279E-17,
1.)) ;
#132049=DIRECTION('ref_axis',(0.,-1.,0.)) ;
#132050=DIRECTION('center_axis',(1.,0.,0.)) ;
#132051=DIRECTION('ref_axis',(0.,0.,-1.)) ;
#132052=DIRECTION('center_axis',(-1.,0.,-7.01133629567814E-33)) ;
#132053=DIRECTION('ref_axis',(-7.01133629567814E-33,0.,1.)) ;
#132054=DIRECTION('center_axis',(1.,0.,0.)) ;
#132055=DIRECTION('ref_axis',(0.,0.,-1.)) ;
#132056=DIRECTION('center_axis',(1.,0.,0.)) ;
#132057=DIRECTION('ref_axis',(0.,0.,-1.)) ;
#132058=DIRECTION('center_axis',(0.,1.,0.)) ;
#132059=DIRECTION('ref_axis',(1.,0.,0.)) ;
#132060=DIRECTION('center_axis',(-7.01133629567814E-33,8.97270763436279E-17,
-1.)) ;
#132061=DIRECTION('ref_axis',(0.,1.,0.)) ;
#132062=DIRECTION('center_axis',(1.,0.,0.)) ;
#132063=DIRECTION('ref_axis',(0.,0.,-1.)) ;
#132064=DIRECTION('center_axis',(-1.,0.,7.01133629567814E-33)) ;
#132065=DIRECTION('ref_axis',(7.01133629567814E-33,0.,1.)) ;
#132066=DIRECTION('center_axis',(1.,0.,0.)) ;
#132067=DIRECTION('ref_axis',(0.,0.,-1.)) ;
#132068=DIRECTION('center_axis',(1.,0.,0.)) ;
#132069=DIRECTION('ref_axis',(0.,0.,-1.)) ;
#132070=DIRECTION('center_axis',(0.,1.,0.)) ;
#132071=DIRECTION('ref_axis',(1.,0.,0.)) ;
#132072=DIRECTION('center_axis',(-7.01133629567814E-33,8.97270763436279E-17,
1.)) ;
#132073=DIRECTION('ref_axis',(0.,-1.,0.)) ;
#132074=DIRECTION('center_axis',(1.,0.,0.)) ;
#132075=DIRECTION('ref_axis',(0.,0.,-1.)) ;
#132076=DIRECTION('center_axis',(-1.,0.,-7.01133629567814E-33)) ;
#132077=DIRECTION('ref_axis',(-7.01133629567814E-33,0.,1.)) ;
#132078=DIRECTION('center_axis',(1.,0.,0.)) ;
#132079=DIRECTION('ref_axis',(0.,0.,-1.)) ;
#132080=DIRECTION('center_axis',(1.,0.,0.)) ;
#132081=DIRECTION('ref_axis',(0.,0.,-1.)) ;
#132082=DIRECTION('center_axis',(0.,1.,0.)) ;
#132083=DIRECTION('ref_axis',(1.,0.,0.)) ;
#132084=DIRECTION('center_axis',(-7.01133629567814E-33,8.97270763436279E-17,
-1.)) ;
#132085=DIRECTION('ref_axis',(0.,1.,0.)) ;
#132086=DIRECTION('center_axis',(1.,0.,0.)) ;
#132087=DIRECTION('ref_axis',(0.,0.,-1.)) ;
#132088=DIRECTION('center_axis',(-1.,0.,7.01133629567814E-33)) ;
#132089=DIRECTION('ref_axis',(7.01133629567814E-33,0.,1.)) ;
#132090=DIRECTION('center_axis',(1.,0.,0.)) ;
#132091=DIRECTION('ref_axis',(0.,0.,-1.)) ;
#132092=DIRECTION('center_axis',(1.,0.,0.)) ;
#132093=DIRECTION('ref_axis',(0.,0.,-1.)) ;
#132094=DIRECTION('center_axis',(0.,1.,0.)) ;
#132095=DIRECTION('ref_axis',(1.,0.,0.)) ;
#132096=DIRECTION('center_axis',(-7.01133629567814E-33,8.97270763436279E-17,
1.)) ;
#132097=DIRECTION('ref_axis',(0.,-1.,0.)) ;
#132098=DIRECTION('center_axis',(1.,0.,0.)) ;
#132099=DIRECTION('ref_axis',(0.,0.,-1.)) ;
#132100=DIRECTION('center_axis',(-1.,0.,-7.01133629567814E-33)) ;
#132101=DIRECTION('ref_axis',(-7.01133629567814E-33,0.,1.)) ;
#132102=DIRECTION('center_axis',(1.,0.,0.)) ;
#132103=DIRECTION('ref_axis',(0.,0.,-1.)) ;
#132104=DIRECTION('center_axis',(1.,0.,0.)) ;
#132105=DIRECTION('ref_axis',(0.,0.,-1.)) ;
#132106=DIRECTION('center_axis',(0.,1.,0.)) ;
#132107=DIRECTION('ref_axis',(1.,0.,0.)) ;
#132108=DIRECTION('center_axis',(-7.01133629567814E-33,8.97270763436279E-17,
-1.)) ;
#132109=DIRECTION('ref_axis',(0.,1.,0.)) ;
#132110=DIRECTION('center_axis',(1.,0.,0.)) ;
#132111=DIRECTION('ref_axis',(0.,0.,-1.)) ;
#132112=DIRECTION('center_axis',(-1.,0.,7.01133629567814E-33)) ;
#132113=DIRECTION('ref_axis',(7.01133629567814E-33,0.,1.)) ;
#132114=DIRECTION('center_axis',(1.,0.,0.)) ;
#132115=DIRECTION('ref_axis',(0.,0.,-1.)) ;
#132116=DIRECTION('center_axis',(1.,0.,0.)) ;
#132117=DIRECTION('ref_axis',(0.,0.,-1.)) ;
#132118=DIRECTION('center_axis',(0.,1.,0.)) ;
#132119=DIRECTION('ref_axis',(1.,0.,0.)) ;
#132120=DIRECTION('center_axis',(-7.01133629567814E-33,8.97270763436279E-17,
1.)) ;
#132121=DIRECTION('ref_axis',(0.,-1.,0.)) ;
#132122=DIRECTION('center_axis',(1.,0.,0.)) ;
#132123=DIRECTION('ref_axis',(0.,0.,-1.)) ;
#132124=DIRECTION('center_axis',(-1.,0.,-7.01133629567814E-33)) ;
#132125=DIRECTION('ref_axis',(-7.01133629567814E-33,0.,1.)) ;
#132126=DIRECTION('center_axis',(1.,0.,0.)) ;
#132127=DIRECTION('ref_axis',(0.,0.,-1.)) ;
#132128=DIRECTION('center_axis',(1.,0.,0.)) ;
#132129=DIRECTION('ref_axis',(0.,0.,-1.)) ;
#132130=DIRECTION('center_axis',(0.,1.,0.)) ;
#132131=DIRECTION('ref_axis',(1.,0.,0.)) ;
#132132=DIRECTION('center_axis',(-7.01133629567814E-33,8.97270763436279E-17,
-1.)) ;
#132133=DIRECTION('ref_axis',(0.,1.,0.)) ;
#132134=DIRECTION('center_axis',(1.,0.,0.)) ;
#132135=DIRECTION('ref_axis',(0.,0.,-1.)) ;
#132136=DIRECTION('center_axis',(-1.,0.,7.01133629567814E-33)) ;
#132137=DIRECTION('ref_axis',(7.01133629567814E-33,0.,1.)) ;
#132138=DIRECTION('center_axis',(1.,0.,0.)) ;
#132139=DIRECTION('ref_axis',(0.,0.,-1.)) ;
#132140=DIRECTION('center_axis',(1.,0.,0.)) ;
#132141=DIRECTION('ref_axis',(0.,0.,-1.)) ;
#132142=DIRECTION('center_axis',(0.,1.,0.)) ;
#132143=DIRECTION('ref_axis',(1.,0.,0.)) ;
#132144=DIRECTION('center_axis',(-7.01133629567814E-33,8.97270763436279E-17,
1.)) ;
#132145=DIRECTION('ref_axis',(0.,-1.,0.)) ;
#132146=DIRECTION('center_axis',(1.,0.,0.)) ;
#132147=DIRECTION('ref_axis',(0.,0.,-1.)) ;
#132148=DIRECTION('center_axis',(-1.,0.,-7.01133629567814E-33)) ;
#132149=DIRECTION('ref_axis',(-7.01133629567814E-33,0.,1.)) ;
#132150=DIRECTION('center_axis',(1.,0.,0.)) ;
#132151=DIRECTION('ref_axis',(0.,0.,-1.)) ;
#132152=DIRECTION('center_axis',(1.,0.,0.)) ;
#132153=DIRECTION('ref_axis',(0.,0.,-1.)) ;
#132154=DIRECTION('center_axis',(0.,1.,0.)) ;
#132155=DIRECTION('ref_axis',(1.,0.,0.)) ;
#132156=DIRECTION('center_axis',(-7.01133629567814E-33,8.97270763436279E-17,
-1.)) ;
#132157=DIRECTION('ref_axis',(0.,1.,0.)) ;
#132158=DIRECTION('center_axis',(1.,0.,0.)) ;
#132159=DIRECTION('ref_axis',(0.,0.,-1.)) ;
#132160=DIRECTION('center_axis',(-1.,0.,7.01133629567814E-33)) ;
#132161=DIRECTION('ref_axis',(7.01133629567814E-33,0.,1.)) ;
#132162=DIRECTION('center_axis',(1.,0.,0.)) ;
#132163=DIRECTION('ref_axis',(0.,0.,-1.)) ;
#132164=DIRECTION('center_axis',(1.,0.,0.)) ;
#132165=DIRECTION('ref_axis',(0.,0.,-1.)) ;
#132166=DIRECTION('center_axis',(0.,1.,0.)) ;
#132167=DIRECTION('ref_axis',(1.,0.,0.)) ;
#132168=DIRECTION('center_axis',(-7.01133629567814E-33,8.97270763436279E-17,
1.)) ;
#132169=DIRECTION('ref_axis',(0.,-1.,0.)) ;
#132170=DIRECTION('center_axis',(1.,0.,0.)) ;
#132171=DIRECTION('ref_axis',(0.,0.,-1.)) ;
#132172=DIRECTION('center_axis',(-1.,0.,-7.01133629567814E-33)) ;
#132173=DIRECTION('ref_axis',(-7.01133629567814E-33,0.,1.)) ;
#132174=DIRECTION('center_axis',(1.,0.,0.)) ;
#132175=DIRECTION('ref_axis',(0.,0.,-1.)) ;
#132176=DIRECTION('center_axis',(1.,0.,0.)) ;
#132177=DIRECTION('ref_axis',(0.,0.,-1.)) ;
#132178=DIRECTION('center_axis',(0.,1.,0.)) ;
#132179=DIRECTION('ref_axis',(1.,0.,0.)) ;
#132180=DIRECTION('center_axis',(-7.01133629567814E-33,8.97270763436279E-17,
-1.)) ;
#132181=DIRECTION('ref_axis',(0.,1.,0.)) ;
#132182=DIRECTION('center_axis',(1.,0.,0.)) ;
#132183=DIRECTION('ref_axis',(0.,0.,-1.)) ;
#132184=DIRECTION('center_axis',(-1.,0.,7.01133629567814E-33)) ;
#132185=DIRECTION('ref_axis',(7.01133629567814E-33,0.,1.)) ;
#132186=DIRECTION('center_axis',(1.,0.,0.)) ;
#132187=DIRECTION('ref_axis',(0.,0.,-1.)) ;
#132188=DIRECTION('center_axis',(1.,0.,0.)) ;
#132189=DIRECTION('ref_axis',(0.,0.,-1.)) ;
#132190=DIRECTION('center_axis',(0.,1.,0.)) ;
#132191=DIRECTION('ref_axis',(1.,0.,0.)) ;
#132192=DIRECTION('center_axis',(1.,0.,0.)) ;
#132193=DIRECTION('ref_axis',(0.,0.,-1.)) ;
#132194=DIRECTION('center_axis',(0.,0.500000000000005,0.866025403784436)) ;
#132195=DIRECTION('ref_axis',(0.,-0.866025403784436,0.500000000000005)) ;
#132196=DIRECTION('center_axis',(0.866025403784441,0.499999999999997,-2.16840434497101E-15)) ;
#132197=DIRECTION('ref_axis',(-0.499999999999997,0.866025403784441,-1.29696145180732E-31)) ;
#132198=DIRECTION('center_axis',(-7.01133629567814E-33,8.97270763436279E-17,
1.)) ;
#132199=DIRECTION('ref_axis',(0.,-1.,0.)) ;
#132200=DIRECTION('center_axis',(1.,0.,0.)) ;
#132201=DIRECTION('ref_axis',(0.,0.,-1.)) ;
#132202=DIRECTION('center_axis',(2.16840434497102E-15,0.500000000000002,
-0.866025403784438)) ;
#132203=DIRECTION('ref_axis',(8.79920118707553E-32,0.866025403784438,0.500000000000002)) ;
#132204=DIRECTION('center_axis',(0.866025403784438,0.500000000000001,0.)) ;
#132205=DIRECTION('ref_axis',(-0.500000000000001,0.866025403784438,0.)) ;
#132206=DIRECTION('center_axis',(-7.01133629567814E-33,8.97270763436279E-17,
-1.)) ;
#132207=DIRECTION('ref_axis',(0.,1.,0.)) ;
#132208=DIRECTION('center_axis',(1.,0.,0.)) ;
#132209=DIRECTION('ref_axis',(0.,0.,-1.)) ;
#132210=DIRECTION('center_axis',(0.,0.49999999999998,0.86602540378445)) ;
#132211=DIRECTION('ref_axis',(0.,-0.86602540378445,0.49999999999998)) ;
#132212=DIRECTION('center_axis',(0.866025403784441,0.499999999999997,-2.16840434497097E-15)) ;
#132213=DIRECTION('ref_axis',(-0.499999999999997,0.866025403784441,2.64734307429885E-31)) ;
#132214=DIRECTION('center_axis',(-7.01133629567814E-33,8.97270763436279E-17,
1.)) ;
#132215=DIRECTION('ref_axis',(0.,-1.,0.)) ;
#132216=DIRECTION('center_axis',(1.,0.,0.)) ;
#132217=DIRECTION('ref_axis',(0.,0.,-1.)) ;
#132218=DIRECTION('center_axis',(7.51157299368579E-15,0.500000000000005,
-0.866025403784436)) ;
#132219=DIRECTION('ref_axis',(8.84230252037551E-31,0.866025403784436,0.500000000000005)) ;
#132220=DIRECTION('center_axis',(0.866025403784438,0.500000000000001,0.)) ;
#132221=DIRECTION('ref_axis',(-0.500000000000001,0.866025403784438,0.)) ;
#132222=DIRECTION('center_axis',(-7.01133629567814E-33,8.97270763436279E-17,
-1.)) ;
#132223=DIRECTION('ref_axis',(0.,1.,0.)) ;
#132224=DIRECTION('center_axis',(1.,0.,0.)) ;
#132225=DIRECTION('ref_axis',(0.,0.,-1.)) ;
#132226=DIRECTION('center_axis',(0.,0.499999999999997,0.866025403784441)) ;
#132227=DIRECTION('ref_axis',(0.,-0.866025403784441,0.499999999999997)) ;
#132228=DIRECTION('center_axis',(0.866025403784441,0.499999999999997,-2.16840434497097E-15)) ;
#132229=DIRECTION('ref_axis',(-0.499999999999997,0.866025403784441,2.64734307429885E-31)) ;
#132230=DIRECTION('center_axis',(-7.01133629567814E-33,8.97270763436279E-17,
1.)) ;
#132231=DIRECTION('ref_axis',(0.,-1.,0.)) ;
#132232=DIRECTION('center_axis',(1.,0.,0.)) ;
#132233=DIRECTION('ref_axis',(0.,0.,-1.)) ;
#132234=DIRECTION('center_axis',(0.,0.499999999999997,-0.866025403784441)) ;
#132235=DIRECTION('ref_axis',(0.,0.866025403784441,0.499999999999997)) ;
#132236=DIRECTION('center_axis',(0.866025403784438,0.500000000000001,0.)) ;
#132237=DIRECTION('ref_axis',(-0.500000000000001,0.866025403784438,0.)) ;
#132238=DIRECTION('center_axis',(-7.01133629567814E-33,8.97270763436279E-17,
-1.)) ;
#132239=DIRECTION('ref_axis',(0.,1.,0.)) ;
#132240=DIRECTION('center_axis',(1.,0.,0.)) ;
#132241=DIRECTION('ref_axis',(0.,0.,-1.)) ;
#132242=DIRECTION('center_axis',(0.,0.500000000000014,0.866025403784431)) ;
#132243=DIRECTION('ref_axis',(0.,-0.866025403784431,0.500000000000014)) ;
#132244=DIRECTION('center_axis',(0.866025403784441,0.499999999999997,-2.16840434497101E-15)) ;
#132245=DIRECTION('ref_axis',(-0.499999999999997,0.866025403784441,-1.29696145180732E-31)) ;
#132246=DIRECTION('center_axis',(-7.01133629567814E-33,8.97270763436279E-17,
1.)) ;
#132247=DIRECTION('ref_axis',(0.,-1.,0.)) ;
#132248=DIRECTION('center_axis',(1.,0.,0.)) ;
#132249=DIRECTION('ref_axis',(0.,0.,-1.)) ;
#132250=DIRECTION('center_axis',(0.,0.499999999999997,-0.866025403784441)) ;
#132251=DIRECTION('ref_axis',(0.,0.866025403784441,0.499999999999997)) ;
#132252=DIRECTION('center_axis',(0.866025403784438,0.500000000000001,0.)) ;
#132253=DIRECTION('ref_axis',(-0.500000000000001,0.866025403784438,0.)) ;
#132254=DIRECTION('center_axis',(-7.01133629567814E-33,8.97270763436279E-17,
-1.)) ;
#132255=DIRECTION('ref_axis',(0.,1.,0.)) ;
#132256=DIRECTION('center_axis',(1.,0.,0.)) ;
#132257=DIRECTION('ref_axis',(0.,0.,-1.)) ;
#132258=DIRECTION('center_axis',(0.,0.500000000000014,0.866025403784431)) ;
#132259=DIRECTION('ref_axis',(0.,-0.866025403784431,0.500000000000014)) ;
#132260=DIRECTION('center_axis',(0.866025403784441,0.499999999999997,-2.16840434497101E-15)) ;
#132261=DIRECTION('ref_axis',(-0.499999999999997,0.866025403784441,-1.29696145180732E-31)) ;
#132262=DIRECTION('center_axis',(-7.01133629567814E-33,8.97270763436279E-17,
1.)) ;
#132263=DIRECTION('ref_axis',(0.,-1.,0.)) ;
#132264=DIRECTION('center_axis',(1.,0.,0.)) ;
#132265=DIRECTION('ref_axis',(0.,0.,-1.)) ;
#132266=DIRECTION('center_axis',(3.87199093546273E-14,0.500000000000014,
-0.866025403784431)) ;
#132267=DIRECTION('ref_axis',(-3.42439963206942E-29,0.866025403784431,0.500000000000014)) ;
#132268=DIRECTION('center_axis',(0.866025403784438,0.500000000000001,0.)) ;
#132269=DIRECTION('ref_axis',(-0.500000000000001,0.866025403784438,0.)) ;
#132270=DIRECTION('center_axis',(-7.01133629567814E-33,8.97270763436279E-17,
-1.)) ;
#132271=DIRECTION('ref_axis',(0.,1.,0.)) ;
#132272=DIRECTION('center_axis',(1.,0.,0.)) ;
#132273=DIRECTION('ref_axis',(0.,0.,-1.)) ;
#132274=DIRECTION('center_axis',(0.,0.500000000000014,0.866025403784431)) ;
#132275=DIRECTION('ref_axis',(0.,-0.866025403784431,0.500000000000014)) ;
#132276=DIRECTION('center_axis',(0.866025403784441,0.499999999999997,-2.16840434497101E-15)) ;
#132277=DIRECTION('ref_axis',(-0.499999999999997,0.866025403784441,-1.29696145180732E-31)) ;
#132278=DIRECTION('center_axis',(-7.01133629567814E-33,8.97270763436279E-17,
1.)) ;
#132279=DIRECTION('ref_axis',(0.,-1.,0.)) ;
#132280=DIRECTION('center_axis',(1.,0.,0.)) ;
#132281=DIRECTION('ref_axis',(0.,0.,-1.)) ;
#132282=DIRECTION('center_axis',(3.87199093546273E-14,0.500000000000014,
-0.866025403784431)) ;
#132283=DIRECTION('ref_axis',(-3.42439963206942E-29,0.866025403784431,0.500000000000014)) ;
#132284=DIRECTION('center_axis',(0.866025403784438,0.500000000000001,0.)) ;
#132285=DIRECTION('ref_axis',(-0.500000000000001,0.866025403784438,0.)) ;
#132286=DIRECTION('center_axis',(-7.01133629567814E-33,8.97270763436279E-17,
-1.)) ;
#132287=DIRECTION('ref_axis',(0.,1.,0.)) ;
#132288=DIRECTION('center_axis',(1.,0.,0.)) ;
#132289=DIRECTION('ref_axis',(0.,0.,-1.)) ;
#132290=DIRECTION('center_axis',(0.,0.500000000000014,0.866025403784431)) ;
#132291=DIRECTION('ref_axis',(0.,-0.866025403784431,0.500000000000014)) ;
#132292=DIRECTION('center_axis',(0.866025403784441,0.499999999999997,-2.16840434497101E-15)) ;
#132293=DIRECTION('ref_axis',(-0.499999999999997,0.866025403784441,-1.29696145180732E-31)) ;
#132294=DIRECTION('center_axis',(-7.01133629567814E-33,8.97270763436279E-17,
1.)) ;
#132295=DIRECTION('ref_axis',(0.,-1.,0.)) ;
#132296=DIRECTION('center_axis',(1.,0.,0.)) ;
#132297=DIRECTION('ref_axis',(0.,0.,-1.)) ;
#132298=DIRECTION('center_axis',(3.87199093546273E-14,0.500000000000014,
-0.866025403784431)) ;
#132299=DIRECTION('ref_axis',(-3.42439963206942E-29,0.866025403784431,0.500000000000014)) ;
#132300=DIRECTION('center_axis',(0.866025403784438,0.500000000000001,0.)) ;
#132301=DIRECTION('ref_axis',(-0.500000000000001,0.866025403784438,0.)) ;
#132302=DIRECTION('center_axis',(-7.01133629567814E-33,8.97270763436279E-17,
-1.)) ;
#132303=DIRECTION('ref_axis',(0.,1.,0.)) ;
#132304=DIRECTION('center_axis',(1.,0.,0.)) ;
#132305=DIRECTION('ref_axis',(0.,0.,-1.)) ;
#132306=DIRECTION('center_axis',(0.,0.500000000000015,0.86602540378443)) ;
#132307=DIRECTION('ref_axis',(0.,-0.86602540378443,0.500000000000015)) ;
#132308=DIRECTION('center_axis',(0.866025403784441,0.499999999999997,-2.16840434497108E-15)) ;
#132309=DIRECTION('ref_axis',(-0.499999999999997,0.866025403784441,-1.29696145180926E-31)) ;
#132310=DIRECTION('center_axis',(-7.01133629567814E-33,8.97270763436279E-17,
1.)) ;
#132311=DIRECTION('ref_axis',(0.,-1.,0.)) ;
#132312=DIRECTION('center_axis',(1.,0.,0.)) ;
#132313=DIRECTION('ref_axis',(0.,0.,-1.)) ;
#132314=DIRECTION('center_axis',(3.87199093546273E-14,0.500000000000014,
-0.866025403784431)) ;
#132315=DIRECTION('ref_axis',(-3.42439963206942E-29,0.866025403784431,0.500000000000014)) ;
#132316=DIRECTION('center_axis',(0.866025403784438,0.500000000000001,0.)) ;
#132317=DIRECTION('ref_axis',(-0.500000000000001,0.866025403784438,0.)) ;
#132318=DIRECTION('center_axis',(-7.01133629567814E-33,8.97270763436279E-17,
-1.)) ;
#132319=DIRECTION('ref_axis',(0.,1.,0.)) ;
#132320=DIRECTION('center_axis',(1.,0.,0.)) ;
#132321=DIRECTION('ref_axis',(0.,0.,-1.)) ;
#132322=DIRECTION('center_axis',(0.,0.500000000000015,0.86602540378443)) ;
#132323=DIRECTION('ref_axis',(0.,-0.86602540378443,0.500000000000015)) ;
#132324=DIRECTION('center_axis',(0.866025403784441,0.499999999999997,-2.16840434497108E-15)) ;
#132325=DIRECTION('ref_axis',(-0.499999999999997,0.866025403784441,-1.29696145180926E-31)) ;
#132326=DIRECTION('center_axis',(-7.01133629567814E-33,8.97270763436279E-17,
1.)) ;
#132327=DIRECTION('ref_axis',(0.,-1.,0.)) ;
#132328=DIRECTION('center_axis',(1.,0.,0.)) ;
#132329=DIRECTION('ref_axis',(0.,0.,-1.)) ;
#132330=DIRECTION('center_axis',(-2.16840434497107E-15,0.500000000000014,
-0.866025403784431)) ;
#132331=DIRECTION('ref_axis',(1.87347069118046E-30,0.866025403784431,0.500000000000014)) ;
#132332=DIRECTION('center_axis',(0.866025403784438,0.500000000000001,0.)) ;
#132333=DIRECTION('ref_axis',(-0.500000000000001,0.866025403784438,0.)) ;
#132334=DIRECTION('center_axis',(-7.01133629567814E-33,8.97270763436279E-17,
-1.)) ;
#132335=DIRECTION('ref_axis',(0.,1.,0.)) ;
#132336=DIRECTION('center_axis',(1.31418445149758E-16,1.,0.)) ;
#132337=DIRECTION('ref_axis',(1.,-1.31418445149758E-16,-1.22464679914735E-16)) ;
#132338=DIRECTION('center_axis',(1.31418445149758E-16,-1.,0.)) ;
#132339=DIRECTION('ref_axis',(-1.,-1.31418445149758E-16,0.)) ;
#132340=DIRECTION('center_axis',(1.31418445149758E-16,1.,0.)) ;
#132341=DIRECTION('ref_axis',(1.,-1.31418445149758E-16,-1.22464679914735E-16)) ;
#132342=DIRECTION('center_axis',(1.31418445149758E-16,-1.,0.)) ;
#132343=DIRECTION('ref_axis',(-1.,-1.31418445149758E-16,0.)) ;
#132344=DIRECTION('center_axis',(1.31418445149758E-16,1.,0.)) ;
#132345=DIRECTION('ref_axis',(1.,-1.31418445149758E-16,-1.22464679914735E-16)) ;
#132346=DIRECTION('center_axis',(1.31418445149758E-16,-1.,0.)) ;
#132347=DIRECTION('ref_axis',(-1.,-1.31418445149758E-16,0.)) ;
#132348=DIRECTION('center_axis',(1.31418445149758E-16,1.,0.)) ;
#132349=DIRECTION('ref_axis',(1.,-1.31418445149758E-16,-1.22464679914735E-16)) ;
#132350=DIRECTION('center_axis',(1.31418445149758E-16,-1.,0.)) ;
#132351=DIRECTION('ref_axis',(-1.,-1.31418445149758E-16,0.)) ;
#132352=DIRECTION('center_axis',(1.31418445149758E-16,1.,0.)) ;
#132353=DIRECTION('ref_axis',(1.,-1.31418445149758E-16,7.6571373978539E-16)) ;
#132354=DIRECTION('center_axis',(1.31418445149758E-16,-1.,0.)) ;
#132355=DIRECTION('ref_axis',(-1.,-1.31418445149758E-16,1.5419764230905E-15)) ;
#132356=DIRECTION('center_axis',(1.31418445149758E-16,1.,0.)) ;
#132357=DIRECTION('ref_axis',(1.,-1.31418445149758E-16,-1.22464679914735E-16)) ;
#132358=DIRECTION('center_axis',(1.31418445149758E-16,-1.,0.)) ;
#132359=DIRECTION('ref_axis',(-1.,-1.31418445149758E-16,0.)) ;
#132360=DIRECTION('center_axis',(0.,1.,0.)) ;
#132361=DIRECTION('ref_axis',(1.,0.,0.)) ;
#132362=DIRECTION('center_axis',(-8.67361737988405E-15,1.,0.)) ;
#132363=DIRECTION('ref_axis',(-1.,-8.67361737988405E-15,0.)) ;
#132364=DIRECTION('center_axis',(-7.81406971160724E-17,1.,0.)) ;
#132365=DIRECTION('ref_axis',(-1.,-7.81406971160724E-17,0.)) ;
#132366=DIRECTION('center_axis',(0.,1.,0.)) ;
#132367=DIRECTION('ref_axis',(0.,0.,1.)) ;
#132368=DIRECTION('center_axis',(0.,0.,-1.)) ;
#132369=DIRECTION('ref_axis',(-1.,0.,0.)) ;
#132370=DIRECTION('center_axis',(1.,0.,0.)) ;
#132371=DIRECTION('ref_axis',(0.,0.,-1.)) ;
#132372=DIRECTION('center_axis',(1.,7.81406971160724E-17,0.)) ;
#132373=DIRECTION('ref_axis',(-7.81406971160724E-17,1.,0.)) ;
#132374=DIRECTION('center_axis',(1.,0.,0.)) ;
#132375=DIRECTION('ref_axis',(0.,0.,-1.)) ;
#132376=DIRECTION('center_axis',(0.,1.,0.)) ;
#132377=DIRECTION('ref_axis',(-1.,0.,0.)) ;
#132378=DIRECTION('center_axis',(0.,1.,0.)) ;
#132379=DIRECTION('ref_axis',(0.,0.,1.)) ;
#132380=DIRECTION('center_axis',(0.,1.,0.)) ;
#132381=DIRECTION('ref_axis',(0.,0.,1.)) ;
#132382=DIRECTION('center_axis',(0.,1.,0.)) ;
#132383=DIRECTION('ref_axis',(0.,0.,1.)) ;
#132384=DIRECTION('center_axis',(0.,1.,0.)) ;
#132385=DIRECTION('ref_axis',(-1.,0.,0.)) ;
#132386=DIRECTION('center_axis',(-1.,0.,0.)) ;
#132387=DIRECTION('ref_axis',(0.,0.,1.)) ;
#132388=DIRECTION('center_axis',(1.,7.81406971160724E-17,0.)) ;
#132389=DIRECTION('ref_axis',(-7.81406971160724E-17,1.,0.)) ;
#132390=DIRECTION('center_axis',(-1.,0.,0.)) ;
#132391=DIRECTION('ref_axis',(0.,0.,1.)) ;
#132392=DIRECTION('center_axis',(0.,1.,0.)) ;
#132393=DIRECTION('ref_axis',(1.,0.,0.)) ;
#132394=DIRECTION('center_axis',(1.,0.,0.)) ;
#132395=DIRECTION('ref_axis',(0.,0.,-1.)) ;
#132396=DIRECTION('center_axis',(0.,0.,-1.)) ;
#132397=DIRECTION('ref_axis',(-1.,0.,0.)) ;
#132398=DIRECTION('center_axis',(0.,1.,0.)) ;
#132399=DIRECTION('ref_axis',(0.,0.,-1.)) ;
#132400=DIRECTION('center_axis',(0.,0.,-1.)) ;
#132401=DIRECTION('ref_axis',(-1.,0.,0.)) ;
#132402=DIRECTION('center_axis',(-1.,-1.31418445149758E-16,0.)) ;
#132403=DIRECTION('ref_axis',(1.31418445149758E-16,-1.,0.)) ;
#132404=DIRECTION('center_axis',(1.,0.,0.)) ;
#132405=DIRECTION('ref_axis',(0.,0.,-1.)) ;
#132406=DIRECTION('center_axis',(-7.81406971160724E-17,1.,0.)) ;
#132407=DIRECTION('ref_axis',(-1.,-7.81406971160724E-17,0.)) ;
#132408=DIRECTION('center_axis',(0.,1.,0.)) ;
#132409=DIRECTION('ref_axis',(0.,0.,1.)) ;
#132410=DIRECTION('center_axis',(0.,0.,1.)) ;
#132411=DIRECTION('ref_axis',(1.,0.,0.)) ;
#132412=DIRECTION('center_axis',(0.,0.,-1.)) ;
#132413=DIRECTION('ref_axis',(-1.,0.,0.)) ;
#132414=DIRECTION('center_axis',(0.,1.,0.)) ;
#132415=DIRECTION('ref_axis',(1.,0.,0.)) ;
#132416=DIRECTION('center_axis',(0.,0.,1.)) ;
#132417=DIRECTION('ref_axis',(-1.,0.,0.)) ;
#132418=DIRECTION('center_axis',(7.81406971160724E-17,-1.,0.)) ;
#132419=DIRECTION('ref_axis',(1.,0.,0.)) ;
#132420=DIRECTION('center_axis',(-7.81406971160724E-17,1.,0.)) ;
#132421=DIRECTION('ref_axis',(1.,7.81406971160724E-17,0.)) ;
#132422=DIRECTION('center_axis',(1.,0.,0.)) ;
#132423=DIRECTION('ref_axis',(0.,0.,1.)) ;
#132424=DIRECTION('center_axis',(0.,0.,1.)) ;
#132425=DIRECTION('ref_axis',(1.,0.,0.)) ;
#132426=DIRECTION('center_axis',(0.,0.,1.)) ;
#132427=DIRECTION('ref_axis',(1.,0.,0.)) ;
#132428=DIRECTION('center_axis',(7.81406971160724E-17,-1.,0.)) ;
#132429=DIRECTION('ref_axis',(1.,7.81406971160724E-17,0.)) ;
#132430=DIRECTION('center_axis',(0.,1.,0.)) ;
#132431=DIRECTION('ref_axis',(0.,0.,1.)) ;
#132432=DIRECTION('center_axis',(1.,7.81406971160724E-17,0.)) ;
#132433=DIRECTION('ref_axis',(-7.81406971160724E-17,1.,0.)) ;
#132434=DIRECTION('center_axis',(0.,1.,0.)) ;
#132435=DIRECTION('ref_axis',(1.,0.,0.)) ;
#132436=DIRECTION('center_axis',(-1.,0.,0.)) ;
#132437=DIRECTION('ref_axis',(0.,0.,-1.)) ;
#132438=DIRECTION('center_axis',(1.,1.31418445149758E-16,0.)) ;
#132439=DIRECTION('ref_axis',(-1.31418445149758E-16,1.,0.)) ;
#132440=DIRECTION('center_axis',(-1.31418445149758E-16,1.,0.)) ;
#132441=DIRECTION('ref_axis',(0.990906098224775,0.,0.134555209861797)) ;
#132442=DIRECTION('center_axis',(-1.31418445149758E-16,1.,0.)) ;
#132443=DIRECTION('ref_axis',(1.,0.,0.)) ;
#132444=DIRECTION('center_axis',(-1.31418445149758E-16,1.,0.)) ;
#132445=DIRECTION('ref_axis',(1.,0.,-1.57898385724467E-15)) ;
#132446=DIRECTION('center_axis',(-1.31418445149758E-16,1.,0.)) ;
#132447=DIRECTION('ref_axis',(1.,0.,0.)) ;
#132448=DIRECTION('center_axis',(-1.31418445149758E-16,1.,0.)) ;
#132449=DIRECTION('ref_axis',(1.,0.,0.)) ;
#132450=DIRECTION('center_axis',(-1.31418445149758E-16,1.,0.)) ;
#132451=DIRECTION('ref_axis',(1.,0.,0.)) ;
#132452=DIRECTION('center_axis',(-1.31418445149758E-16,1.,0.)) ;
#132453=DIRECTION('ref_axis',(1.,0.,0.)) ;
#132454=DIRECTION('center_axis',(0.,1.,0.)) ;
#132455=DIRECTION('ref_axis',(1.,0.,0.)) ;
#132456=DIRECTION('center_axis',(-8.67361737988405E-15,1.,0.)) ;
#132457=DIRECTION('ref_axis',(-1.,-8.67361737988405E-15,0.)) ;
#132458=DIRECTION('center_axis',(-1.31418445149758E-16,1.,0.)) ;
#132459=DIRECTION('ref_axis',(1.,0.,0.)) ;
#132460=DIRECTION('center_axis',(7.81406971160724E-17,-1.,0.)) ;
#132461=DIRECTION('ref_axis',(1.,7.81406971160724E-17,0.)) ;
#132462=DIRECTION('center_axis',(0.,1.,0.)) ;
#132463=DIRECTION('ref_axis',(0.,0.,1.)) ;
#132464=DIRECTION('center_axis',(0.,0.,-1.)) ;
#132465=DIRECTION('ref_axis',(-1.,0.,0.)) ;
#132466=DIRECTION('center_axis',(1.,0.,0.)) ;
#132467=DIRECTION('ref_axis',(0.,0.,-1.)) ;
#132468=DIRECTION('center_axis',(-1.31418445149758E-16,1.,0.)) ;
#132469=DIRECTION('ref_axis',(1.,0.,-1.97372982155583E-16)) ;
#132470=DIRECTION('center_axis',(-1.,-7.81406971160724E-17,0.)) ;
#132471=DIRECTION('ref_axis',(7.81406971160724E-17,-1.,0.)) ;
#132472=DIRECTION('center_axis',(1.,0.,0.)) ;
#132473=DIRECTION('ref_axis',(0.,0.,-1.)) ;
#132474=DIRECTION('center_axis',(0.,1.,0.)) ;
#132475=DIRECTION('ref_axis',(-1.,0.,0.)) ;
#132476=DIRECTION('center_axis',(4.33680868994202E-15,1.,0.)) ;
#132477=DIRECTION('ref_axis',(-1.,4.33680868994202E-15,0.)) ;
#132478=DIRECTION('center_axis',(-1.31418445149758E-16,1.,0.)) ;
#132479=DIRECTION('ref_axis',(0.990906098224775,0.,-0.134555209861799)) ;
#132480=DIRECTION('center_axis',(-1.,-7.81406971160724E-17,-5.25614554872951E-16)) ;
#132481=DIRECTION('ref_axis',(-5.25614554872951E-16,-4.10718877321264E-32,
1.)) ;
#132482=DIRECTION('center_axis',(-1.,0.,0.)) ;
#132483=DIRECTION('ref_axis',(0.,0.,1.)) ;
#132484=DIRECTION('center_axis',(0.,1.,0.)) ;
#132485=DIRECTION('ref_axis',(0.,0.,1.)) ;
#132486=DIRECTION('center_axis',(0.,1.,0.)) ;
#132487=DIRECTION('ref_axis',(0.,0.,1.)) ;
#132488=DIRECTION('center_axis',(7.81406971160724E-17,-1.,0.)) ;
#132489=DIRECTION('ref_axis',(1.,0.,0.)) ;
#132490=DIRECTION('center_axis',(-7.81406971160724E-17,1.,0.)) ;
#132491=DIRECTION('ref_axis',(1.,7.81406971160724E-17,0.)) ;
#132492=DIRECTION('center_axis',(0.,0.,-1.)) ;
#132493=DIRECTION('ref_axis',(1.,0.,0.)) ;
#132494=DIRECTION('center_axis',(0.,1.,0.)) ;
#132495=DIRECTION('ref_axis',(-1.,0.,0.)) ;
#132496=DIRECTION('center_axis',(-1.,0.,0.)) ;
#132497=DIRECTION('ref_axis',(0.,0.,1.)) ;
#132498=DIRECTION('center_axis',(-1.,-1.31418445149758E-16,-5.25614554872951E-16)) ;
#132499=DIRECTION('ref_axis',(-5.25614554872951E-16,-6.90754475494854E-32,
1.)) ;
#132500=DIRECTION('center_axis',(1.,0.,0.)) ;
#132501=DIRECTION('ref_axis',(0.,0.,-1.)) ;
#132502=DIRECTION('center_axis',(7.81406971160724E-17,-1.,1.10147335281612E-31)) ;
#132503=DIRECTION('ref_axis',(1.,7.81406971160724E-17,-8.6069895643829E-48)) ;
#132504=DIRECTION('center_axis',(0.,1.,0.)) ;
#132505=DIRECTION('ref_axis',(0.,0.,1.)) ;
#132506=DIRECTION('center_axis',(0.,0.,1.)) ;
#132507=DIRECTION('ref_axis',(1.,0.,0.)) ;
#132508=DIRECTION('center_axis',(0.,0.,-1.)) ;
#132509=DIRECTION('ref_axis',(-1.,0.,0.)) ;
#132510=DIRECTION('center_axis',(-1.,-7.81406971160724E-17,0.)) ;
#132511=DIRECTION('ref_axis',(7.81406971160724E-17,-1.,0.)) ;
#132512=DIRECTION('center_axis',(-1.,0.,0.)) ;
#132513=DIRECTION('ref_axis',(0.,0.,1.)) ;
#132514=DIRECTION('center_axis',(0.,1.,0.)) ;
#132515=DIRECTION('ref_axis',(1.,0.,0.)) ;
#132516=DIRECTION('center_axis',(1.51788304147971E-14,0.,1.)) ;
#132517=DIRECTION('ref_axis',(-1.,0.,1.51788304147971E-14)) ;
#132518=DIRECTION('center_axis',(0.,0.,-1.)) ;
#132519=DIRECTION('ref_axis',(-1.,0.,0.)) ;
#132520=DIRECTION('center_axis',(0.,1.,0.)) ;
#132521=DIRECTION('ref_axis',(0.,0.,-1.)) ;
#132522=DIRECTION('center_axis',(0.,0.,1.)) ;
#132523=DIRECTION('ref_axis',(1.,0.,0.)) ;
#132524=DIRECTION('center_axis',(0.,0.,1.)) ;
#132525=DIRECTION('ref_axis',(1.,0.,0.)) ;
#132526=DIRECTION('center_axis',(7.81406971160724E-17,-1.,0.)) ;
#132527=DIRECTION('ref_axis',(1.,7.81406971160724E-17,0.)) ;
#132528=DIRECTION('center_axis',(0.,1.,0.)) ;
#132529=DIRECTION('ref_axis',(0.,0.,1.)) ;
#132530=DIRECTION('center_axis',(0.,1.,0.)) ;
#132531=DIRECTION('ref_axis',(1.,0.,0.)) ;
#132532=DIRECTION('center_axis',(-1.,0.,0.)) ;
#132533=DIRECTION('ref_axis',(0.,0.,-1.)) ;
#132534=DIRECTION('center_axis',(1.,1.31418445149758E-16,0.)) ;
#132535=DIRECTION('ref_axis',(-1.31418445149758E-16,1.,0.)) ;
#132536=DIRECTION('center_axis',(-1.,0.,0.)) ;
#132537=DIRECTION('ref_axis',(0.,0.,1.)) ;
#132538=DIRECTION('center_axis',(0.,1.,0.)) ;
#132539=DIRECTION('ref_axis',(1.,0.,0.)) ;
#132540=DIRECTION('center_axis',(0.380709651665466,0.236869643538635,0.893841671158063)) ;
#132541=DIRECTION('ref_axis',(0.920024234945248,1.04575356953145E-17,-0.391861464185253)) ;
#132542=DIRECTION('center_axis',(0.380709651731648,0.236869643589572,-0.893841671116377)) ;
#132543=DIRECTION('ref_axis',(-0.9200242349141,-4.58748474863685E-15,-0.391861464258384)) ;
#152009=CARTESIAN_POINT('',(0.,0.,0.)) ;
#152010=CARTESIAN_POINT('Origin',(-3.91058726874632,3.70028042224035,-36.59)) ;
#152011=CARTESIAN_POINT('',(-3.8208783653803,3.65609543998544,-36.49)) ;
#152012=CARTESIAN_POINT('',(-3.90529363437316,3.80014021112017,-36.49)) ;
#152013=CARTESIAN_POINT('Origin',(-3.91058726874632,3.70028042224035,-36.49)) ;
#152014=CARTESIAN_POINT('',(-3.8208783653803,3.65609543998544,2.2)) ;
#152015=CARTESIAN_POINT('',(-3.8208783653803,3.65609543998544,-36.49)) ;
#152016=CARTESIAN_POINT('',(-3.90529363437316,3.80014021112017,2.2)) ;
#152017=CARTESIAN_POINT('Origin',(-3.91058726874632,3.70028042224035,2.2)) ;
#152018=CARTESIAN_POINT('',(-3.90529363437316,3.80014021112017,-36.59)) ;
#152019=CARTESIAN_POINT('Origin',(1.77490703981927,4.45,1.4854875)) ;
#152020=CARTESIAN_POINT('',(1.77490703981927,4.55,1.65)) ;
#152021=CARTESIAN_POINT('',(1.6487489852016,4.55,1.37990100507126)) ;
#152022=CARTESIAN_POINT('Origin',(1.77490703981927,4.55,1.4854875)) ;
#152023=CARTESIAN_POINT('',(1.77490703981927,4.45,1.55)) ;
#152024=CARTESIAN_POINT('Origin',(1.77490703981927,4.45,1.65)) ;
#152025=CARTESIAN_POINT('',(1.72543498451331,4.45,1.4440824471676)) ;
#152026=CARTESIAN_POINT('Origin',(1.77490703981927,4.45,1.4854875)) ;
#152027=CARTESIAN_POINT('Origin',(1.6487489852016,4.45,1.37990100507126)) ;
#152028=CARTESIAN_POINT('Origin',(1.3145125,4.45,-1.905)) ;
#152029=CARTESIAN_POINT('',(1.22107868287598,4.55,-1.76959510912125)) ;
#152030=CARTESIAN_POINT('',(1.22107868287598,4.55,-2.04040489087875)) ;
#152031=CARTESIAN_POINT('Origin',(1.3145125,4.55,-1.905)) ;
#152032=CARTESIAN_POINT('',(1.27787304021905,4.45,-1.85190185838271)) ;
#152033=CARTESIAN_POINT('Origin',(1.22107868287598,4.45,-1.76959510912125)) ;
#152034=CARTESIAN_POINT('',(1.27787304021905,4.45,-1.9580981416173)) ;
#152035=CARTESIAN_POINT('Origin',(1.3145125,4.45,-1.905)) ;
#152036=CARTESIAN_POINT('Origin',(1.22107868287598,4.45,-2.04040489087875)) ;
#152037=CARTESIAN_POINT('Origin',(-8.21365282185989E-16,2.85,0.)) ;
#152038=CARTESIAN_POINT('',(1.37603597336697,2.75,-1.905)) ;
#152039=CARTESIAN_POINT('',(1.84932420089069,2.75,1.45)) ;
#152040=CARTESIAN_POINT('Origin',(-8.13551212474381E-16,2.75,0.)) ;
#152041=CARTESIAN_POINT('',(1.27787304021905,2.85,-1.85190185838271)) ;
#152042=CARTESIAN_POINT('Ctrl Pts',(1.37603597336697,2.75,-1.905)) ;
#152043=CARTESIAN_POINT('Ctrl Pts',(1.37543428354306,2.75,-1.90468005811351)) ;
#152044=CARTESIAN_POINT('Ctrl Pts',(1.37483253111456,2.75000531372589,-1.90436018434118)) ;
#152045=CARTESIAN_POINT('Ctrl Pts',(1.37388722675069,2.75002207412045,-1.903857355793)) ;
#152046=CARTESIAN_POINT('Ctrl Pts',(1.37354350385561,2.75002991650282,-1.90367448583784)) ;
#152047=CARTESIAN_POINT('Ctrl Pts',(1.37285611423782,2.75004911307826,-1.9033087011159)) ;
#152048=CARTESIAN_POINT('Ctrl Pts',(1.37251244753524,2.75006046723047,-1.90312578638849)) ;
#152049=CARTESIAN_POINT('Ctrl Pts',(1.3714815944481,2.75009981984526,-1.90257700530504)) ;
#152050=CARTESIAN_POINT('Ctrl Pts',(1.37079455494331,2.75013310886333,-1.90221110179681)) ;
#152051=CARTESIAN_POINT('Ctrl Pts',(1.36873453110893,2.75025430438115,-1.90111349441338)) ;
#152052=CARTESIAN_POINT('Ctrl Pts',(1.36736263966052,2.75036354665963,-1.90038189075796)) ;
#152053=CARTESIAN_POINT('Ctrl Pts',(1.36413470836879,2.75068903914081,-1.8986589310622)) ;
#152054=CARTESIAN_POINT('Ctrl Pts',(1.36227932197148,2.75092980851021,-1.89766736227896)) ;
#152055=CARTESIAN_POINT('Ctrl Pts',(1.35746012444743,2.75169859670379,-1.89508881807843)) ;
#152056=CARTESIAN_POINT('Ctrl Pts',(1.35450425835489,2.7523133271765,-1.89350423745892)) ;
#152057=CARTESIAN_POINT('Ctrl Pts',(1.34886973918565,2.75377034241463,-1.89047916949336)) ;
#152058=CARTESIAN_POINT('Ctrl Pts',(1.34617831568151,2.75459534478003,-1.88903214074158)) ;
#152059=CARTESIAN_POINT('Ctrl Pts',(1.34314242260183,2.75567798707048,-1.88739846987703)) ;
#152060=CARTESIAN_POINT('Ctrl Pts',(1.34256163823226,2.75588931242806,-1.887085898215)) ;
#152061=CARTESIAN_POINT('Ctrl Pts',(1.34198261999809,2.75610647364238,-1.8867742184185)) ;
#152062=CARTESIAN_POINT('Ctrl Pts',(1.3413216052292,2.75635697290856,-1.88641837801666)) ;
#152063=CARTESIAN_POINT('Ctrl Pts',(1.3408629143507,2.75653491456656,-1.88617141746806)) ;
#152064=CARTESIAN_POINT('Ctrl Pts',(1.33918548989956,2.7572007950357,-1.88526816249943)) ;
#152065=CARTESIAN_POINT('Ctrl Pts',(1.33797416370948,2.75771112313095,-1.88461565173485)) ;
#152066=CARTESIAN_POINT('Ctrl Pts',(1.33648532079705,2.75837521508442,-1.88381336705108)) ;
#152067=CARTESIAN_POINT('Ctrl Pts',(1.33619776328718,2.75850521488808,-1.88365840269789)) ;
#152068=CARTESIAN_POINT('Ctrl Pts',(1.33107968015626,2.76084915994917,-1.88089996028831)) ;
#152069=CARTESIAN_POINT('Ctrl Pts',(1.32635908659477,2.7635069333901,-1.8783519804515)) ;
#152070=CARTESIAN_POINT('Ctrl Pts',(1.32109760626031,2.76707470328413,-1.87550528308814)) ;
#152071=CARTESIAN_POINT('Ctrl Pts',(1.32035743991824,2.76759128788297,-1.87510464755506)) ;
#152072=CARTESIAN_POINT('Ctrl Pts',(1.3182480554607,2.7691058422748,-1.87396233738911)) ;
#152073=CARTESIAN_POINT('Ctrl Pts',(1.31689309423376,2.77013099976528,-1.87322773664117)) ;
#152074=CARTESIAN_POINT('Ctrl Pts',(1.31545882361435,2.77127278201747,-1.87244887805927)) ;
#152075=CARTESIAN_POINT('Ctrl Pts',(1.31535582310958,2.77135510350022,-1.87239293834655)) ;
#152076=CARTESIAN_POINT('Ctrl Pts',(1.3150485309221,2.77160168095797,-1.87222602655303)) ;
#152077=CARTESIAN_POINT('Ctrl Pts',(1.31461168315426,2.77195498754742,-1.87198869314584)) ;
#152078=CARTESIAN_POINT('Ctrl Pts',(1.31417742224138,2.77231219724368,-1.87175266294293)) ;
#152079=CARTESIAN_POINT('Ctrl Pts',(1.31333096026315,2.77301480846571,-1.87129249386306)) ;
#152080=CARTESIAN_POINT('Ctrl Pts',(1.31272070342856,2.77353368974768,-1.87096054315942)) ;
#152081=CARTESIAN_POINT('Ctrl Pts',(1.30969774837134,2.77616736630455,-1.86931544276183)) ;
#152082=CARTESIAN_POINT('Ctrl Pts',(1.30737022788701,2.77840054644572,-1.86804652010492)) ;
#152083=CARTESIAN_POINT('Ctrl Pts',(1.30464757270885,2.78128817542222,-1.86656129665113)) ;
#152084=CARTESIAN_POINT('Ctrl Pts',(1.3041484598108,2.78182967606622,-1.86628898736925)) ;
#152085=CARTESIAN_POINT('Ctrl Pts',(1.30260826844056,2.78353926416388,-1.86544857136307)) ;
#152086=CARTESIAN_POINT('Ctrl Pts',(1.30158324720849,2.78473373830865,-1.86488876707862)) ;
#152087=CARTESIAN_POINT('Ctrl Pts',(1.30024935135332,2.78636738852738,-1.86416018728324)) ;
#152088=CARTESIAN_POINT('Ctrl Pts',(1.29991860867237,2.78677921519271,-1.86397952491896)) ;
#152089=CARTESIAN_POINT('Ctrl Pts',(1.29915346420735,2.78774794465154,-1.8635615807717)) ;
#152090=CARTESIAN_POINT('Ctrl Pts',(1.29872125904468,2.78830744810472,-1.86332550011269)) ;
#152091=CARTESIAN_POINT('Ctrl Pts',(1.29658637826222,2.79113377451591,-1.8621594679259)) ;
#152092=CARTESIAN_POINT('Ctrl Pts',(1.29496240940488,2.79348720429746,-1.86127301363021)) ;
#152093=CARTESIAN_POINT('Ctrl Pts',(1.29231665668156,2.79769679694546,-1.85982835199505)) ;
#152094=CARTESIAN_POINT('Ctrl Pts',(1.29125115601061,2.79951540543443,-1.8592459513193)) ;
#152095=CARTESIAN_POINT('Ctrl Pts',(1.28927619853496,2.80313430045115,-1.85816512101871)) ;
#152096=CARTESIAN_POINT('Ctrl Pts',(1.2883624199782,2.80493500363977,-1.85766462065405)) ;
#152097=CARTESIAN_POINT('Ctrl Pts',(1.28732027925586,2.80715235940913,-1.8570931587537)) ;
#152098=CARTESIAN_POINT('Ctrl Pts',(1.28695835013166,2.80793550920675,-1.85689461743542)) ;
#152099=CARTESIAN_POINT('Ctrl Pts',(1.28660568774191,2.80872522382218,-1.85670104370722)) ;
#152100=CARTESIAN_POINT('Ctrl Pts',(1.28608376699196,2.80991454434775,-1.85641450210149)) ;
#152101=CARTESIAN_POINT('Ctrl Pts',(1.28574525149601,2.81071375754612,-1.85622856810943)) ;
#152102=CARTESIAN_POINT('Ctrl Pts',(1.28475894023896,2.81312894312824,-1.85568673335099)) ;
#152103=CARTESIAN_POINT('Ctrl Pts',(1.28414040309303,2.81476247656143,-1.85534683370203)) ;
#152104=CARTESIAN_POINT('Ctrl Pts',(1.28339818260913,2.8168875602015,-1.854939111358)) ;
#152105=CARTESIAN_POINT('Ctrl Pts',(1.28323661013043,2.81736137575529,-1.85485036282194)) ;
#152106=CARTESIAN_POINT('Ctrl Pts',(1.2826566889388,2.81910411140435,-1.85453185264633)) ;
#152107=CARTESIAN_POINT('Ctrl Pts',(1.28225920250333,2.82038205281187,-1.85431360767476)) ;
#152108=CARTESIAN_POINT('Ctrl Pts',(1.28170385606936,2.82230051526768,-1.85400866501641)) ;
#152109=CARTESIAN_POINT('Ctrl Pts',(1.28152700208472,2.82293438010912,-1.85391155822972)) ;
#152110=CARTESIAN_POINT('Ctrl Pts',(1.28107448868731,2.82461913389174,-1.85366309085072)) ;
#152111=CARTESIAN_POINT('Ctrl Pts',(1.28081016954773,2.82567198476339,-1.85351801104593)) ;
#152112=CARTESIAN_POINT('Ctrl Pts',(1.28009910353321,2.82871092361135,-1.85312783198231)) ;
#152113=CARTESIAN_POINT('Ctrl Pts',(1.27969380338795,2.83071459002995,-1.85290512911995)) ;
#152114=CARTESIAN_POINT('Ctrl Pts',(1.27923282767964,2.83340629334539,-1.85265154626654)) ;
#152115=CARTESIAN_POINT('Ctrl Pts',(1.27912420342282,2.83408089926113,-1.85259176478417)) ;
#152116=CARTESIAN_POINT('Ctrl Pts',(1.27861441353188,2.83746106027949,-1.85231109118167)) ;
#152117=CARTESIAN_POINT('Ctrl Pts',(1.2783132428757,2.84018799487022,-1.85214490175664)) ;
#152118=CARTESIAN_POINT('Ctrl Pts',(1.27795656969993,2.84527977141542,-1.85194801334391)) ;
#152119=CARTESIAN_POINT('Ctrl Pts',(1.27787304021905,2.8476428621108,-1.8519018583827)) ;
#152120=CARTESIAN_POINT('Ctrl Pts',(1.27787304021905,2.85,-1.8519018583827)) ;
#152121=CARTESIAN_POINT('',(1.72543498451331,2.85,1.4440824471676)) ;
#152122=CARTESIAN_POINT('Origin',(-8.21365282185989E-16,2.85,0.)) ;
#152123=CARTESIAN_POINT('Ctrl Pts',(1.84932420089069,2.75,1.45)) ;
#152124=CARTESIAN_POINT('Ctrl Pts',(1.84863058979364,2.75,1.44997563735877)) ;
#152125=CARTESIAN_POINT('Ctrl Pts',(1.84793752344315,2.75000415508919,1.44995131206652)) ;
#152126=CARTESIAN_POINT('Ctrl Pts',(1.8466682790665,2.75001949937859,1.44990654329321)) ;
#152127=CARTESIAN_POINT('Ctrl Pts',(1.84609162157503,2.75002939777795,1.44988606034608)) ;
#152128=CARTESIAN_POINT('Ctrl Pts',(1.84477120566863,2.75005887738453,1.44983884278185)) ;
#152129=CARTESIAN_POINT('Ctrl Pts',(1.84402746838178,2.7500804333137,1.44981204894611)) ;
#152130=CARTESIAN_POINT('Ctrl Pts',(1.84209973630459,2.75014939605369,1.44974205847089)) ;
#152131=CARTESIAN_POINT('Ctrl Pts',(1.84091590068203,2.75020455995514,1.44969854506027)) ;
#152132=CARTESIAN_POINT('Ctrl Pts',(1.83783446245764,2.75038253459787,1.44958383066685)) ;
#152133=CARTESIAN_POINT('Ctrl Pts',(1.83593755875625,2.75052613609568,1.4495117702051)) ;
#152134=CARTESIAN_POINT('Ctrl Pts',(1.8309456297289,2.75099782379543,1.44931834596177)) ;
#152135=CARTESIAN_POINT('Ctrl Pts',(1.82785402838571,2.7513859024504,1.44919458503464)) ;
#152136=CARTESIAN_POINT('Ctrl Pts',(1.81948035994712,2.7527115862255,1.4488527720359)) ;
#152137=CARTESIAN_POINT('Ctrl Pts',(1.81421215989036,2.75385085634789,1.44862821117908)) ;
#152138=CARTESIAN_POINT('Ctrl Pts',(1.8031061499061,2.75695526843004,1.44814117174278)) ;
#152139=CARTESIAN_POINT('Ctrl Pts',(1.79730846849538,2.75900870786305,1.44788414257244)) ;
#152140=CARTESIAN_POINT('Ctrl Pts',(1.78961597328954,2.76232847656554,1.44753373419531)) ;
#152141=CARTESIAN_POINT('Ctrl Pts',(1.7875531568042,2.76328057020225,1.44743866638175)) ;
#152142=CARTESIAN_POINT('Ctrl Pts',(1.78290815273718,2.76556355836601,1.44722066393822)) ;
#152143=CARTESIAN_POINT('Ctrl Pts',(1.78033073359788,2.76693246555895,1.44709649577908)) ;
#152144=CARTESIAN_POINT('Ctrl Pts',(1.77699233515397,2.76883988197513,1.44693042742489)) ;
#152145=CARTESIAN_POINT('Ctrl Pts',(1.77620130341379,2.76930169056972,1.4468906872056)) ;
#152146=CARTESIAN_POINT('Ctrl Pts',(1.7700212686611,2.77299328866811,1.44657696433726)) ;
#152147=CARTESIAN_POINT('Ctrl Pts',(1.76495428804002,2.77651771769392,1.44630647059977)) ;
#152148=CARTESIAN_POINT('Ctrl Pts',(1.75938438664977,2.78118533571325,1.4460042033466)) ;
#152149=CARTESIAN_POINT('Ctrl Pts',(1.75866155314252,2.78180749701142,1.44596487872825)) ;
#152150=CARTESIAN_POINT('Ctrl Pts',(1.75440101126574,2.7855766156533,1.44573272620675)) ;
#152151=CARTESIAN_POINT('Ctrl Pts',(1.75110534239503,2.78891118859354,1.44556220259829)) ;
#152152=CARTESIAN_POINT('Ctrl Pts',(1.74704475763671,2.79358254909136,1.44534353205998)) ;
#152153=CARTESIAN_POINT('Ctrl Pts',(1.74604050383924,2.79479094319554,1.44528857933487)) ;
#152154=CARTESIAN_POINT('Ctrl Pts',(1.74487333929765,2.79625803001555,1.44522266035845)) ;
#152155=CARTESIAN_POINT('Ctrl Pts',(1.74467927949937,2.79650417922903,1.44521163325506)) ;
#152156=CARTESIAN_POINT('Ctrl Pts',(1.74115657836476,2.80101412428662,1.44501009724943)) ;
#152157=CARTESIAN_POINT('Ctrl Pts',(1.73808736282551,2.80561663574426,1.44483055636364)) ;
#152158=CARTESIAN_POINT('Ctrl Pts',(1.73411503311364,2.81315073291951,1.44459732117177)) ;
#152159=CARTESIAN_POINT('Ctrl Pts',(1.73300100590538,2.81551882664672,1.444535439772)) ;
#152160=CARTESIAN_POINT('Ctrl Pts',(1.73189652742022,2.8181493620667,1.44447069895227)) ;
#152161=CARTESIAN_POINT('Ctrl Pts',(1.73180208385959,2.81837683840677,1.44446516169542)) ;
#152162=CARTESIAN_POINT('Ctrl Pts',(1.73016675860464,2.82236036724297,1.44436925395154)) ;
#152163=CARTESIAN_POINT('Ctrl Pts',(1.72888947962583,2.82624394235942,1.44429466669055)) ;
#152164=CARTESIAN_POINT('Ctrl Pts',(1.72770663337626,2.83096681005806,1.4442247776102)) ;
#152165=CARTESIAN_POINT('Ctrl Pts',(1.72752382530083,2.83174344980706,1.44421394009748)) ;
#152166=CARTESIAN_POINT('Ctrl Pts',(1.7271933356899,2.83324353771473,1.44419425207312)) ;
#152167=CARTESIAN_POINT('Ctrl Pts',(1.72704413780188,2.83396640281164,1.44418527971536)) ;
#152168=CARTESIAN_POINT('Ctrl Pts',(1.7260250143745,2.83926193720951,1.44412308045111)) ;
#152169=CARTESIAN_POINT('Ctrl Pts',(1.72552996843222,2.84393088107443,1.44408905620284)) ;
#152170=CARTESIAN_POINT('Ctrl Pts',(1.72543914472539,2.84906100604569,1.44408273999325)) ;
#152171=CARTESIAN_POINT('Ctrl Pts',(1.72543498451331,2.84953057829521,1.4440824471676)) ;
#152172=CARTESIAN_POINT('Ctrl Pts',(1.72543498451331,2.85,1.4440824471676)) ;
#152173=CARTESIAN_POINT('Origin',(1.3145125,4.45,-5.715)) ;
#152174=CARTESIAN_POINT('',(1.22107868287598,4.55,-5.57959510912125)) ;
#152175=CARTESIAN_POINT('',(1.22107868287598,4.55,-5.85040489087875)) ;
#152176=CARTESIAN_POINT('Origin',(1.3145125,4.55,-5.715)) ;
#152177=CARTESIAN_POINT('',(1.27787304021905,4.45,-5.66190185838271)) ;
#152178=CARTESIAN_POINT('Origin',(1.22107868287598,4.45,-5.57959510912125)) ;
#152179=CARTESIAN_POINT('',(1.27787304021905,4.45,-5.76809814161729)) ;
#152180=CARTESIAN_POINT('Origin',(1.3145125,4.45,-5.715)) ;
#152181=CARTESIAN_POINT('Origin',(1.22107868287598,4.45,-5.85040489087875)) ;
#152182=CARTESIAN_POINT('Origin',(-8.21365282185989E-16,2.85,-3.81)) ;
#152183=CARTESIAN_POINT('',(1.37603597336697,2.75,-5.715)) ;
#152184=CARTESIAN_POINT('Origin',(-8.13551212474381E-16,2.75,-3.81)) ;
#152185=CARTESIAN_POINT('',(1.27787304021905,2.85,-5.66190185838271)) ;
#152186=CARTESIAN_POINT('Ctrl Pts',(1.37603597336697,2.75,-5.715)) ;
#152187=CARTESIAN_POINT('Ctrl Pts',(1.37543428354307,2.75,-5.71468005811352)) ;
#152188=CARTESIAN_POINT('Ctrl Pts',(1.37483253111456,2.7500053137259,-5.71436018434118)) ;
#152189=CARTESIAN_POINT('Ctrl Pts',(1.37388722675069,2.75002207412044,-5.713857355793)) ;
#152190=CARTESIAN_POINT('Ctrl Pts',(1.37354350385561,2.75002991650282,-5.71367448583784)) ;
#152191=CARTESIAN_POINT('Ctrl Pts',(1.37285611423782,2.75004911307826,-5.71330870111591)) ;
#152192=CARTESIAN_POINT('Ctrl Pts',(1.37251244753524,2.75006046723047,-5.71312578638849)) ;
#152193=CARTESIAN_POINT('Ctrl Pts',(1.3714815944481,2.75009981984526,-5.71257700530505)) ;
#152194=CARTESIAN_POINT('Ctrl Pts',(1.37079455494331,2.75013310886333,-5.71221110179682)) ;
#152195=CARTESIAN_POINT('Ctrl Pts',(1.36873453110892,2.75025430438116,-5.71111349441339)) ;
#152196=CARTESIAN_POINT('Ctrl Pts',(1.36736263966051,2.75036354665963,-5.71038189075797)) ;
#152197=CARTESIAN_POINT('Ctrl Pts',(1.36413470836879,2.75068903914081,-5.7086589310622)) ;
#152198=CARTESIAN_POINT('Ctrl Pts',(1.36227932197148,2.75092980851022,-5.70766736227896)) ;
#152199=CARTESIAN_POINT('Ctrl Pts',(1.35746012444743,2.7516985967038,-5.70508881807843)) ;
#152200=CARTESIAN_POINT('Ctrl Pts',(1.35450425835489,2.75231332717651,-5.70350423745893)) ;
#152201=CARTESIAN_POINT('Ctrl Pts',(1.34886973918565,2.75377034241464,-5.70047916949337)) ;
#152202=CARTESIAN_POINT('Ctrl Pts',(1.34617831568151,2.75459534478003,-5.69903214074159)) ;
#152203=CARTESIAN_POINT('Ctrl Pts',(1.34314242260183,2.75567798707049,-5.69739846987704)) ;
#152204=CARTESIAN_POINT('Ctrl Pts',(1.34256163823226,2.75588931242806,-5.697085898215)) ;
#152205=CARTESIAN_POINT('Ctrl Pts',(1.34198261999809,2.75610647364238,-5.69677421841851)) ;
#152206=CARTESIAN_POINT('Ctrl Pts',(1.3413216052292,2.75635697290857,-5.69641837801666)) ;
#152207=CARTESIAN_POINT('Ctrl Pts',(1.3408629143507,2.75653491456656,-5.69617141746806)) ;
#152208=CARTESIAN_POINT('Ctrl Pts',(1.33918548989956,2.7572007950357,-5.69526816249943)) ;
#152209=CARTESIAN_POINT('Ctrl Pts',(1.33797416370948,2.75771112313095,-5.69461565173486)) ;
#152210=CARTESIAN_POINT('Ctrl Pts',(1.33648532079705,2.75837521508442,-5.69381336705109)) ;
#152211=CARTESIAN_POINT('Ctrl Pts',(1.33619776328718,2.75850521488809,-5.69365840269788)) ;
#152212=CARTESIAN_POINT('Ctrl Pts',(1.33107968015654,2.76084915994904,-5.69089996028846)) ;
#152213=CARTESIAN_POINT('Ctrl Pts',(1.32635908659532,2.76350693338979,-5.68835198045179)) ;
#152214=CARTESIAN_POINT('Ctrl Pts',(1.32109760626083,2.76707470328377,-5.68550528308842)) ;
#152215=CARTESIAN_POINT('Ctrl Pts',(1.32035743991849,2.76759128788279,-5.68510464755519)) ;
#152216=CARTESIAN_POINT('Ctrl Pts',(1.31824805546069,2.7691058422748,-5.6839623373891)) ;
#152217=CARTESIAN_POINT('Ctrl Pts',(1.31689309423376,2.77013099976529,-5.68322773664116)) ;
#152218=CARTESIAN_POINT('Ctrl Pts',(1.31545882361434,2.77127278201747,-5.68244887805927)) ;
#152219=CARTESIAN_POINT('Ctrl Pts',(1.31535582310956,2.77135510350023,-5.68239293834654)) ;
#152220=CARTESIAN_POINT('Ctrl Pts',(1.31504853092208,2.77160168095798,-5.68222602655302)) ;
#152221=CARTESIAN_POINT('Ctrl Pts',(1.31461168315424,2.77195498754745,-5.68198869314584)) ;
#152222=CARTESIAN_POINT('Ctrl Pts',(1.31417742224136,2.77231219724369,-5.68175266294292)) ;
#152223=CARTESIAN_POINT('Ctrl Pts',(1.31333096026313,2.77301480846573,-5.68129249386305)) ;
#152224=CARTESIAN_POINT('Ctrl Pts',(1.31272070342853,2.7735336897477,-5.68096054315941)) ;
#152225=CARTESIAN_POINT('Ctrl Pts',(1.30969774837131,2.77616736630457,-5.67931544276182)) ;
#152226=CARTESIAN_POINT('Ctrl Pts',(1.30737022788698,2.77840054644575,-5.67804652010491)) ;
#152227=CARTESIAN_POINT('Ctrl Pts',(1.30464757270883,2.78128817542224,-5.67656129665112)) ;
#152228=CARTESIAN_POINT('Ctrl Pts',(1.30414845981079,2.78182967606623,-5.67628898736924)) ;
#152229=CARTESIAN_POINT('Ctrl Pts',(1.30260826844056,2.78353926416388,-5.67544857136307)) ;
#152230=CARTESIAN_POINT('Ctrl Pts',(1.30158324720849,2.78473373830865,-5.67488876707862)) ;
#152231=CARTESIAN_POINT('Ctrl Pts',(1.30024935135332,2.78636738852738,-5.67416018728324)) ;
#152232=CARTESIAN_POINT('Ctrl Pts',(1.29991860867237,2.78677921519272,-5.67397952491896)) ;
#152233=CARTESIAN_POINT('Ctrl Pts',(1.29915346420734,2.78774794465155,-5.67356158077169)) ;
#152234=CARTESIAN_POINT('Ctrl Pts',(1.29872125904468,2.78830744810472,-5.67332550011269)) ;
#152235=CARTESIAN_POINT('Ctrl Pts',(1.29658637826221,2.79113377451592,-5.6721594679259)) ;
#152236=CARTESIAN_POINT('Ctrl Pts',(1.29496240940487,2.79348720429747,-5.67127301363021)) ;
#152237=CARTESIAN_POINT('Ctrl Pts',(1.29231665668155,2.79769679694548,-5.66982835199504)) ;
#152238=CARTESIAN_POINT('Ctrl Pts',(1.29125115601061,2.79951540543445,-5.6692459513193)) ;
#152239=CARTESIAN_POINT('Ctrl Pts',(1.28927619853496,2.80313430045116,-5.66816512101871)) ;
#152240=CARTESIAN_POINT('Ctrl Pts',(1.2883624199782,2.80493500363978,-5.66766462065405)) ;
#152241=CARTESIAN_POINT('Ctrl Pts',(1.28732027925586,2.80715235940914,-5.6670931587537)) ;
#152242=CARTESIAN_POINT('Ctrl Pts',(1.28695835013166,2.80793550920674,-5.66689461743542)) ;
#152243=CARTESIAN_POINT('Ctrl Pts',(1.28660568774191,2.80872522382218,-5.66670104370723)) ;
#152244=CARTESIAN_POINT('Ctrl Pts',(1.28608376699196,2.80991454434776,-5.6664145021015)) ;
#152245=CARTESIAN_POINT('Ctrl Pts',(1.28574525149601,2.81071375754612,-5.66622856810943)) ;
#152246=CARTESIAN_POINT('Ctrl Pts',(1.28475894023895,2.81312894312825,-5.66568673335099)) ;
#152247=CARTESIAN_POINT('Ctrl Pts',(1.28414040309303,2.81476247656144,-5.66534683370204)) ;
#152248=CARTESIAN_POINT('Ctrl Pts',(1.28339818260912,2.81688756020151,-5.664939111358)) ;
#152249=CARTESIAN_POINT('Ctrl Pts',(1.28323661013043,2.8173613757553,-5.66485036282194)) ;
#152250=CARTESIAN_POINT('Ctrl Pts',(1.28265668893879,2.81910411140437,-5.66453185264632)) ;
#152251=CARTESIAN_POINT('Ctrl Pts',(1.28225920250332,2.82038205281189,-5.66431360767476)) ;
#152252=CARTESIAN_POINT('Ctrl Pts',(1.28170385606936,2.8223005152677,-5.66400866501641)) ;
#152253=CARTESIAN_POINT('Ctrl Pts',(1.28152700208472,2.82293438010912,-5.66391155822972)) ;
#152254=CARTESIAN_POINT('Ctrl Pts',(1.28107448868731,2.82461913389174,-5.66366309085072)) ;
#152255=CARTESIAN_POINT('Ctrl Pts',(1.28081016954773,2.82567198476339,-5.66351801104592)) ;
#152256=CARTESIAN_POINT('Ctrl Pts',(1.28009910353321,2.82871092361135,-5.6631278319823)) ;
#152257=CARTESIAN_POINT('Ctrl Pts',(1.27969380338794,2.83071459002995,-5.66290512911995)) ;
#152258=CARTESIAN_POINT('Ctrl Pts',(1.27923282767964,2.83340629334539,-5.66265154626654)) ;
#152259=CARTESIAN_POINT('Ctrl Pts',(1.27912420342282,2.83408089926113,-5.66259176478417)) ;
#152260=CARTESIAN_POINT('Ctrl Pts',(1.27861441353188,2.8374610602795,-5.66231109118167)) ;
#152261=CARTESIAN_POINT('Ctrl Pts',(1.2783132428757,2.84018799487024,-5.66214490175664)) ;
#152262=CARTESIAN_POINT('Ctrl Pts',(1.27795656969993,2.84527977141544,-5.66194801334391)) ;
#152263=CARTESIAN_POINT('Ctrl Pts',(1.27787304021905,2.8476428621108,-5.6619018583827)) ;
#152264=CARTESIAN_POINT('Ctrl Pts',(1.27787304021905,2.85,-5.6619018583827)) ;
#152265=CARTESIAN_POINT('',(1.27787304021905,2.85,-1.9580981416173)) ;
#152266=CARTESIAN_POINT('Origin',(-8.21365282185989E-16,2.85,-3.81)) ;
#152267=CARTESIAN_POINT('Ctrl Pts',(1.37603597336697,2.75,-1.905)) ;
#152268=CARTESIAN_POINT('Ctrl Pts',(1.37573512845501,2.75,-1.90515997094324)) ;
#152269=CARTESIAN_POINT('Ctrl Pts',(1.37543426791745,2.75000132857104,-1.90531992480456)) ;
#152270=CARTESIAN_POINT('Ctrl Pts',(1.37483257571475,2.75000665190009,-1.90563984485733)) ;
#152271=CARTESIAN_POINT('Ctrl Pts',(1.37453174406034,2.75001064672751,-1.90579981102493)) ;
#152272=CARTESIAN_POINT('Ctrl Pts',(1.37388722675069,2.75002207412045,-1.90614264420702)) ;
#152273=CARTESIAN_POINT('Ctrl Pts',(1.37354350385561,2.75002991650282,-1.90632551416212)) ;
#152274=CARTESIAN_POINT('Ctrl Pts',(1.37285611423782,2.75004911307826,-1.9066912988841)) ;
#152275=CARTESIAN_POINT('Ctrl Pts',(1.37251244753524,2.75006046723047,-1.90687421361152)) ;
#152276=CARTESIAN_POINT('Ctrl Pts',(1.3714815944481,2.75009981984526,-1.90742299469496)) ;
#152277=CARTESIAN_POINT('Ctrl Pts',(1.37079455494331,2.75013310886333,-1.90778889820319)) ;
#152278=CARTESIAN_POINT('Ctrl Pts',(1.36873453110892,2.75025430438115,-1.90888650558662)) ;
#152279=CARTESIAN_POINT('Ctrl Pts',(1.36736263966051,2.75036354665963,-1.90961810924204)) ;
#152280=CARTESIAN_POINT('Ctrl Pts',(1.36413470836879,2.75068903914081,-1.91134106893781)) ;
#152281=CARTESIAN_POINT('Ctrl Pts',(1.36227932197148,2.75092980851022,-1.91233263772104)) ;
#152282=CARTESIAN_POINT('Ctrl Pts',(1.35746012444743,2.7516985967038,-1.91491118192158)) ;
#152283=CARTESIAN_POINT('Ctrl Pts',(1.35450425835489,2.75231332717651,-1.91649576254108)) ;
#152284=CARTESIAN_POINT('Ctrl Pts',(1.34886973918565,2.75377034241464,-1.91952083050664)) ;
#152285=CARTESIAN_POINT('Ctrl Pts',(1.34617831568151,2.75459534478003,-1.92096785925842)) ;
#152286=CARTESIAN_POINT('Ctrl Pts',(1.34314242260183,2.75567798707048,-1.92260153012297)) ;
#152287=CARTESIAN_POINT('Ctrl Pts',(1.34256163823226,2.75588931242806,-1.922914101785)) ;
#152288=CARTESIAN_POINT('Ctrl Pts',(1.34198261999809,2.75610647364238,-1.9232257815815)) ;
#152289=CARTESIAN_POINT('Ctrl Pts',(1.3413216052292,2.75635697290856,-1.92358162198335)) ;
#152290=CARTESIAN_POINT('Ctrl Pts',(1.3408629143507,2.75653491456656,-1.92382858253194)) ;
#152291=CARTESIAN_POINT('Ctrl Pts',(1.33918548989955,2.7572007950357,-1.92473183750057)) ;
#152292=CARTESIAN_POINT('Ctrl Pts',(1.33797416370948,2.75771112313095,-1.92538434826515)) ;
#152293=CARTESIAN_POINT('Ctrl Pts',(1.33648532079705,2.75837521508442,-1.92618663294892)) ;
#152294=CARTESIAN_POINT('Ctrl Pts',(1.33619776328718,2.75850521488809,-1.92634159730212)) ;
#152295=CARTESIAN_POINT('Ctrl Pts',(1.3310796801563,2.76084915994915,-1.92910003971167)) ;
#152296=CARTESIAN_POINT('Ctrl Pts',(1.32635908659486,2.76350693339004,-1.93164801954846)) ;
#152297=CARTESIAN_POINT('Ctrl Pts',(1.32109760626039,2.76707470328407,-1.93449471691182)) ;
#152298=CARTESIAN_POINT('Ctrl Pts',(1.32035743991827,2.76759128788294,-1.93489535244492)) ;
#152299=CARTESIAN_POINT('Ctrl Pts',(1.3182480554607,2.76910584227479,-1.93603766261089)) ;
#152300=CARTESIAN_POINT('Ctrl Pts',(1.31689309423376,2.77013099976528,-1.93677226335883)) ;
#152301=CARTESIAN_POINT('Ctrl Pts',(1.31545882361434,2.77127278201747,-1.93755112194073)) ;
#152302=CARTESIAN_POINT('Ctrl Pts',(1.31535582310957,2.77135510350021,-1.93760706165345)) ;
#152303=CARTESIAN_POINT('Ctrl Pts',(1.31504853092209,2.77160168095797,-1.93777397344698)) ;
#152304=CARTESIAN_POINT('Ctrl Pts',(1.31461168315425,2.77195498754744,-1.93801130685414)) ;
#152305=CARTESIAN_POINT('Ctrl Pts',(1.31417742224137,2.77231219724368,-1.93824733705707)) ;
#152306=CARTESIAN_POINT('Ctrl Pts',(1.31333096026314,2.77301480846571,-1.93870750613694)) ;
#152307=CARTESIAN_POINT('Ctrl Pts',(1.31272070342855,2.77353368974768,-1.93903945684058)) ;
#152308=CARTESIAN_POINT('Ctrl Pts',(1.30969774837133,2.77616736630456,-1.94068455723817)) ;
#152309=CARTESIAN_POINT('Ctrl Pts',(1.307370227887,2.77840054644573,-1.94195347989508)) ;
#152310=CARTESIAN_POINT('Ctrl Pts',(1.30464757270885,2.78128817542222,-1.94343870334887)) ;
#152311=CARTESIAN_POINT('Ctrl Pts',(1.30414845981079,2.78182967606621,-1.94371101263075)) ;
#152312=CARTESIAN_POINT('Ctrl Pts',(1.30260826844056,2.78353926416388,-1.94455142863693)) ;
#152313=CARTESIAN_POINT('Ctrl Pts',(1.30158324720849,2.78473373830865,-1.94511123292138)) ;
#152314=CARTESIAN_POINT('Ctrl Pts',(1.30024935135332,2.78636738852738,-1.94583981271676)) ;
#152315=CARTESIAN_POINT('Ctrl Pts',(1.29991860867237,2.78677921519272,-1.94602047508104)) ;
#152316=CARTESIAN_POINT('Ctrl Pts',(1.29915346420735,2.78774794465154,-1.94643841922831)) ;
#152317=CARTESIAN_POINT('Ctrl Pts',(1.29872125904468,2.78830744810472,-1.94667449988731)) ;
#152318=CARTESIAN_POINT('Ctrl Pts',(1.29658637826222,2.79113377451592,-1.9478405320741)) ;
#152319=CARTESIAN_POINT('Ctrl Pts',(1.29496240940488,2.79348720429747,-1.94872698636979)) ;
#152320=CARTESIAN_POINT('Ctrl Pts',(1.29231665668155,2.79769679694547,-1.95017164800495)) ;
#152321=CARTESIAN_POINT('Ctrl Pts',(1.29125115601061,2.79951540543444,-1.95075404868069)) ;
#152322=CARTESIAN_POINT('Ctrl Pts',(1.28927619853496,2.80313430045115,-1.95183487898129)) ;
#152323=CARTESIAN_POINT('Ctrl Pts',(1.2883624199782,2.80493500363977,-1.95233537934595)) ;
#152324=CARTESIAN_POINT('Ctrl Pts',(1.28732027925586,2.80715235940913,-1.9529068412463)) ;
#152325=CARTESIAN_POINT('Ctrl Pts',(1.28695835013166,2.80793550920675,-1.95310538256458)) ;
#152326=CARTESIAN_POINT('Ctrl Pts',(1.28660568774191,2.80872522382218,-1.95329895629277)) ;
#152327=CARTESIAN_POINT('Ctrl Pts',(1.28608376699196,2.80991454434775,-1.95358549789851)) ;
#152328=CARTESIAN_POINT('Ctrl Pts',(1.28574525149601,2.81071375754612,-1.95377143189057)) ;
#152329=CARTESIAN_POINT('Ctrl Pts',(1.28475894023896,2.81312894312824,-1.95431326664901)) ;
#152330=CARTESIAN_POINT('Ctrl Pts',(1.28414040309303,2.81476247656143,-1.95465316629796)) ;
#152331=CARTESIAN_POINT('Ctrl Pts',(1.28339818260913,2.8168875602015,-1.955060888642)) ;
#152332=CARTESIAN_POINT('Ctrl Pts',(1.28323661013043,2.81736137575529,-1.95514963717806)) ;
#152333=CARTESIAN_POINT('Ctrl Pts',(1.2826566889388,2.81910411140435,-1.95546814735368)) ;
#152334=CARTESIAN_POINT('Ctrl Pts',(1.28225920250333,2.82038205281187,-1.95568639232524)) ;
#152335=CARTESIAN_POINT('Ctrl Pts',(1.28170385606936,2.82230051526768,-1.95599133498359)) ;
#152336=CARTESIAN_POINT('Ctrl Pts',(1.28152700208472,2.82293438010912,-1.95608844177028)) ;
#152337=CARTESIAN_POINT('Ctrl Pts',(1.28107448868731,2.82461913389174,-1.95633690914928)) ;
#152338=CARTESIAN_POINT('Ctrl Pts',(1.28081016954773,2.82567198476339,-1.95648198895408)) ;
#152339=CARTESIAN_POINT('Ctrl Pts',(1.28009910353321,2.82871092361134,-1.95687216801769)) ;
#152340=CARTESIAN_POINT('Ctrl Pts',(1.27969380338795,2.83071459002995,-1.95709487088005)) ;
#152341=CARTESIAN_POINT('Ctrl Pts',(1.27923282767965,2.83340629334537,-1.95734845373346)) ;
#152342=CARTESIAN_POINT('Ctrl Pts',(1.27912420342282,2.83408089926112,-1.95740823521583)) ;
#152343=CARTESIAN_POINT('Ctrl Pts',(1.27861441353188,2.83746106027947,-1.95768890881833)) ;
#152344=CARTESIAN_POINT('Ctrl Pts',(1.2783132428757,2.8401879948702,-1.95785509824336)) ;
#152345=CARTESIAN_POINT('Ctrl Pts',(1.27795656969993,2.8452797714154,-1.95805198665609)) ;
#152346=CARTESIAN_POINT('Ctrl Pts',(1.27787304021905,2.84764286211078,-1.9580981416173)) ;
#152347=CARTESIAN_POINT('Ctrl Pts',(1.27787304021905,2.85,-1.9580981416173)) ;
#152348=CARTESIAN_POINT('Origin',(1.3145125,4.45,-9.525)) ;
#152349=CARTESIAN_POINT('',(1.22107868287598,4.55,-9.38959510912125)) ;
#152350=CARTESIAN_POINT('',(1.22107868287598,4.55,-9.66040489087875)) ;
#152351=CARTESIAN_POINT('Origin',(1.3145125,4.55,-9.525)) ;
#152352=CARTESIAN_POINT('',(1.27787304021905,4.45,-9.4719018583827)) ;
#152353=CARTESIAN_POINT('Origin',(1.22107868287598,4.45,-9.38959510912125)) ;
#152354=CARTESIAN_POINT('',(1.27787304021905,4.45,-9.57809814161729)) ;
#152355=CARTESIAN_POINT('Origin',(1.3145125,4.45,-9.525)) ;
#152356=CARTESIAN_POINT('Origin',(1.22107868287598,4.45,-9.66040489087875)) ;
#152357=CARTESIAN_POINT('Origin',(-8.21365282185989E-16,2.85,-7.62)) ;
#152358=CARTESIAN_POINT('',(1.37603597336697,2.75,-9.525)) ;
#152359=CARTESIAN_POINT('Origin',(-8.13551212474381E-16,2.75,-7.62)) ;
#152360=CARTESIAN_POINT('',(1.27787304021905,2.85,-9.4719018583827)) ;
#152361=CARTESIAN_POINT('Ctrl Pts',(1.37603597336697,2.75,-9.525)) ;
#152362=CARTESIAN_POINT('Ctrl Pts',(1.37599182636237,2.75000002234121,-9.52497652572716)) ;
#152363=CARTESIAN_POINT('Ctrl Pts',(1.37594767935777,2.75000004468243,-9.52495305145431)) ;
#152364=CARTESIAN_POINT('Ctrl Pts',(1.3756975209442,2.75000017127862,-9.52482003479991)) ;
#152365=CARTESIAN_POINT('Ctrl Pts',(1.37511460540165,2.75000290680017,-9.52451012344317)) ;
#152366=CARTESIAN_POINT('Ctrl Pts',(1.37453174406036,2.75001064672751,-9.52420018897501)) ;
#152367=CARTESIAN_POINT('Ctrl Pts',(1.3738872267507,2.75002207412045,-9.52385735579295)) ;
#152368=CARTESIAN_POINT('Ctrl Pts',(1.37354350385558,2.75002991650282,-9.52367448583783)) ;
#152369=CARTESIAN_POINT('Ctrl Pts',(1.37285611423782,2.75004911307825,-9.52330870111588)) ;
#152370=CARTESIAN_POINT('Ctrl Pts',(1.37251244753524,2.75006046723047,-9.52312578638847)) ;
#152371=CARTESIAN_POINT('Ctrl Pts',(1.37148159444809,2.75009981984525,-9.52257700530504)) ;
#152372=CARTESIAN_POINT('Ctrl Pts',(1.37079455494331,2.75013310886332,-9.52221110179681)) ;
#152373=CARTESIAN_POINT('Ctrl Pts',(1.36873453110892,2.75025430438115,-9.52111349441339)) ;
#152374=CARTESIAN_POINT('Ctrl Pts',(1.36736263966052,2.75036354665962,-9.52038189075796)) ;
#152375=CARTESIAN_POINT('Ctrl Pts',(1.36413470836879,2.7506890391408,-9.51865893106218)) ;
#152376=CARTESIAN_POINT('Ctrl Pts',(1.36227932197148,2.7509298085102,-9.51766736227895)) ;
#152377=CARTESIAN_POINT('Ctrl Pts',(1.35746012444742,2.75169859670377,-9.51508881807842)) ;
#152378=CARTESIAN_POINT('Ctrl Pts',(1.35450425835489,2.75231332717647,-9.51350423745891)) ;
#152379=CARTESIAN_POINT('Ctrl Pts',(1.34886973918564,2.7537703424146,-9.51047916949335)) ;
#152380=CARTESIAN_POINT('Ctrl Pts',(1.3461783156815,2.75459534477999,-9.50903214074156)) ;
#152381=CARTESIAN_POINT('Ctrl Pts',(1.34314242260182,2.75567798707045,-9.50739846987701)) ;
#152382=CARTESIAN_POINT('Ctrl Pts',(1.34256163823225,2.75588931242802,-9.50708589821498)) ;
#152383=CARTESIAN_POINT('Ctrl Pts',(1.34198261999809,2.75610647364234,-9.50677421841848)) ;
#152384=CARTESIAN_POINT('Ctrl Pts',(1.34132160522919,2.75635697290853,-9.50641837801664)) ;
#152385=CARTESIAN_POINT('Ctrl Pts',(1.34086291435069,2.75653491456652,-9.50617141746804)) ;
#152386=CARTESIAN_POINT('Ctrl Pts',(1.33918548989955,2.75720079503567,-9.50526816249941)) ;
#152387=CARTESIAN_POINT('Ctrl Pts',(1.33797416370947,2.75771112313092,-9.50461565173483)) ;
#152388=CARTESIAN_POINT('Ctrl Pts',(1.33648532079704,2.75837521508439,-9.50381336705106)) ;
#152389=CARTESIAN_POINT('Ctrl Pts',(1.33619776328717,2.75850521488806,-9.50365840269787)) ;
#152390=CARTESIAN_POINT('Ctrl Pts',(1.33107968015649,2.76084915994903,-9.50089996028843)) ;
#152391=CARTESIAN_POINT('Ctrl Pts',(1.32635908659524,2.76350693338982,-9.49835198045175)) ;
#152392=CARTESIAN_POINT('Ctrl Pts',(1.32109760626075,2.76707470328381,-9.49550528308838)) ;
#152393=CARTESIAN_POINT('Ctrl Pts',(1.32035743991845,2.76759128788282,-9.49510464755518)) ;
#152394=CARTESIAN_POINT('Ctrl Pts',(1.31824805546069,2.7691058422748,-9.49396233738911)) ;
#152395=CARTESIAN_POINT('Ctrl Pts',(1.31689309423376,2.77013099976528,-9.49322773664117)) ;
#152396=CARTESIAN_POINT('Ctrl Pts',(1.31545882361434,2.77127278201747,-9.49244887805927)) ;
#152397=CARTESIAN_POINT('Ctrl Pts',(1.31535582310956,2.77135510350022,-9.49239293834655)) ;
#152398=CARTESIAN_POINT('Ctrl Pts',(1.31504853092208,2.77160168095798,-9.49222602655302)) ;
#152399=CARTESIAN_POINT('Ctrl Pts',(1.31461168315426,2.77195498754743,-9.49198869314583)) ;
#152400=CARTESIAN_POINT('Ctrl Pts',(1.31417742224137,2.77231219724369,-9.49175266294293)) ;
#152401=CARTESIAN_POINT('Ctrl Pts',(1.31333096026314,2.77301480846572,-9.49129249386305)) ;
#152402=CARTESIAN_POINT('Ctrl Pts',(1.31272070342854,2.77353368974769,-9.49096054315942)) ;
#152403=CARTESIAN_POINT('Ctrl Pts',(1.30969774837133,2.77616736630456,-9.48931544276183)) ;
#152404=CARTESIAN_POINT('Ctrl Pts',(1.307370227887,2.77840054644573,-9.48804652010492)) ;
#152405=CARTESIAN_POINT('Ctrl Pts',(1.30464757270884,2.78128817542223,-9.48656129665113)) ;
#152406=CARTESIAN_POINT('Ctrl Pts',(1.30414845981079,2.78182967606623,-9.48628898736924)) ;
#152407=CARTESIAN_POINT('Ctrl Pts',(1.30260826844056,2.78353926416389,-9.48544857136307)) ;
#152408=CARTESIAN_POINT('Ctrl Pts',(1.30158324720849,2.78473373830866,-9.48488876707862)) ;
#152409=CARTESIAN_POINT('Ctrl Pts',(1.30024935135332,2.78636738852739,-9.48416018728324)) ;
#152410=CARTESIAN_POINT('Ctrl Pts',(1.29991860867237,2.78677921519272,-9.48397952491896)) ;
#152411=CARTESIAN_POINT('Ctrl Pts',(1.29915346420735,2.78774794465155,-9.48356158077169)) ;
#152412=CARTESIAN_POINT('Ctrl Pts',(1.29872125904468,2.78830744810473,-9.48332550011269)) ;
#152413=CARTESIAN_POINT('Ctrl Pts',(1.29658637826222,2.79113377451592,-9.4821594679259)) ;
#152414=CARTESIAN_POINT('Ctrl Pts',(1.29496240940488,2.79348720429747,-9.48127301363021)) ;
#152415=CARTESIAN_POINT('Ctrl Pts',(1.29231665668155,2.79769679694548,-9.47982835199505)) ;
#152416=CARTESIAN_POINT('Ctrl Pts',(1.29125115601061,2.79951540543445,-9.4792459513193)) ;
#152417=CARTESIAN_POINT('Ctrl Pts',(1.28927619853496,2.80313430045116,-9.47816512101871)) ;
#152418=CARTESIAN_POINT('Ctrl Pts',(1.2883624199782,2.80493500363978,-9.47766462065405)) ;
#152419=CARTESIAN_POINT('Ctrl Pts',(1.28732027925585,2.80715235940914,-9.4770931587537)) ;
#152420=CARTESIAN_POINT('Ctrl Pts',(1.28695835013167,2.80793550920674,-9.47689461743542)) ;
#152421=CARTESIAN_POINT('Ctrl Pts',(1.28660568774191,2.80872522382218,-9.47670104370723)) ;
#152422=CARTESIAN_POINT('Ctrl Pts',(1.28608376699196,2.80991454434776,-9.47641450210149)) ;
#152423=CARTESIAN_POINT('Ctrl Pts',(1.28574525149601,2.81071375754613,-9.47622856810943)) ;
#152424=CARTESIAN_POINT('Ctrl Pts',(1.28475894023896,2.81312894312825,-9.47568673335099)) ;
#152425=CARTESIAN_POINT('Ctrl Pts',(1.28414040309303,2.81476247656144,-9.47534683370204)) ;
#152426=CARTESIAN_POINT('Ctrl Pts',(1.28339818260913,2.81688756020151,-9.474939111358)) ;
#152427=CARTESIAN_POINT('Ctrl Pts',(1.28323661013043,2.8173613757553,-9.47485036282194)) ;
#152428=CARTESIAN_POINT('Ctrl Pts',(1.28265668893879,2.81910411140437,-9.47453185264632)) ;
#152429=CARTESIAN_POINT('Ctrl Pts',(1.28225920250332,2.82038205281189,-9.47431360767476)) ;
#152430=CARTESIAN_POINT('Ctrl Pts',(1.28170385606936,2.8223005152677,-9.47400866501641)) ;
#152431=CARTESIAN_POINT('Ctrl Pts',(1.28152700208472,2.82293438010913,-9.47391155822972)) ;
#152432=CARTESIAN_POINT('Ctrl Pts',(1.28107448868731,2.82461913389175,-9.47366309085072)) ;
#152433=CARTESIAN_POINT('Ctrl Pts',(1.28081016954773,2.82567198476339,-9.47351801104593)) ;
#152434=CARTESIAN_POINT('Ctrl Pts',(1.28009910353322,2.82871092361134,-9.47312783198231)) ;
#152435=CARTESIAN_POINT('Ctrl Pts',(1.27969380338795,2.83071459002995,-9.47290512911995)) ;
#152436=CARTESIAN_POINT('Ctrl Pts',(1.27923282767965,2.83340629334537,-9.47265154626654)) ;
#152437=CARTESIAN_POINT('Ctrl Pts',(1.27912420342282,2.83408089926112,-9.47259176478417)) ;
#152438=CARTESIAN_POINT('Ctrl Pts',(1.27861441353188,2.83746106027947,-9.47231109118166)) ;
#152439=CARTESIAN_POINT('Ctrl Pts',(1.2783132428757,2.8401879948702,-9.47214490175664)) ;
#152440=CARTESIAN_POINT('Ctrl Pts',(1.27795656969993,2.8452797714154,-9.4719480133439)) ;
#152441=CARTESIAN_POINT('Ctrl Pts',(1.27787304021905,2.84764286211078,-9.4719018583827)) ;
#152442=CARTESIAN_POINT('Ctrl Pts',(1.27787304021905,2.85,-9.4719018583827)) ;
#152443=CARTESIAN_POINT('',(1.27787304021905,2.85,-5.76809814161729)) ;
#152444=CARTESIAN_POINT('Origin',(-8.21365282185989E-16,2.85,-7.62)) ;
#152445=CARTESIAN_POINT('Ctrl Pts',(1.37603597336697,2.75,-5.715)) ;
#152446=CARTESIAN_POINT('Ctrl Pts',(1.37543428354306,2.75,-5.71531994188649)) ;
#152447=CARTESIAN_POINT('Ctrl Pts',(1.37483253111456,2.7500053137259,-5.71563981565882)) ;
#152448=CARTESIAN_POINT('Ctrl Pts',(1.37388722675069,2.75002207412044,-5.71614264420701)) ;
#152449=CARTESIAN_POINT('Ctrl Pts',(1.37354350385561,2.75002991650282,-5.71632551416217)) ;
#152450=CARTESIAN_POINT('Ctrl Pts',(1.37285611423782,2.75004911307826,-5.7166912988841)) ;
#152451=CARTESIAN_POINT('Ctrl Pts',(1.37251244753524,2.75006046723047,-5.71687421361152)) ;
#152452=CARTESIAN_POINT('Ctrl Pts',(1.3714815944481,2.75009981984526,-5.71742299469496)) ;
#152453=CARTESIAN_POINT('Ctrl Pts',(1.37079455494331,2.75013310886333,-5.71778889820319)) ;
#152454=CARTESIAN_POINT('Ctrl Pts',(1.36873453110892,2.75025430438115,-5.71888650558662)) ;
#152455=CARTESIAN_POINT('Ctrl Pts',(1.36736263966051,2.75036354665963,-5.71961810924204)) ;
#152456=CARTESIAN_POINT('Ctrl Pts',(1.36413470836879,2.75068903914081,-5.72134106893781)) ;
#152457=CARTESIAN_POINT('Ctrl Pts',(1.36227932197148,2.75092980851021,-5.72233263772104)) ;
#152458=CARTESIAN_POINT('Ctrl Pts',(1.35746012444743,2.7516985967038,-5.72491118192158)) ;
#152459=CARTESIAN_POINT('Ctrl Pts',(1.35450425835489,2.7523133271765,-5.72649576254108)) ;
#152460=CARTESIAN_POINT('Ctrl Pts',(1.34886973918565,2.75377034241463,-5.72952083050664)) ;
#152461=CARTESIAN_POINT('Ctrl Pts',(1.3461783156815,2.75459534478002,-5.73096785925842)) ;
#152462=CARTESIAN_POINT('Ctrl Pts',(1.34314242260183,2.75567798707048,-5.73260153012297)) ;
#152463=CARTESIAN_POINT('Ctrl Pts',(1.34256163823226,2.75588931242805,-5.73291410178501)) ;
#152464=CARTESIAN_POINT('Ctrl Pts',(1.34198261999809,2.75610647364238,-5.7332257815815)) ;
#152465=CARTESIAN_POINT('Ctrl Pts',(1.3413216052292,2.75635697290856,-5.73358162198335)) ;
#152466=CARTESIAN_POINT('Ctrl Pts',(1.3408629143507,2.75653491456656,-5.73382858253195)) ;
#152467=CARTESIAN_POINT('Ctrl Pts',(1.33918548989955,2.7572007950357,-5.73473183750058)) ;
#152468=CARTESIAN_POINT('Ctrl Pts',(1.33797416370948,2.75771112313095,-5.73538434826515)) ;
#152469=CARTESIAN_POINT('Ctrl Pts',(1.33648532079705,2.75837521508442,-5.73618663294892)) ;
#152470=CARTESIAN_POINT('Ctrl Pts',(1.33619776328717,2.75850521488808,-5.73634159730212)) ;
#152471=CARTESIAN_POINT('Ctrl Pts',(1.33107968015659,2.76084915994901,-5.73910003971151)) ;
#152472=CARTESIAN_POINT('Ctrl Pts',(1.32635908659541,2.76350693338973,-5.74164801954816)) ;
#152473=CARTESIAN_POINT('Ctrl Pts',(1.3210976062609,2.76707470328371,-5.74449471691154)) ;
#152474=CARTESIAN_POINT('Ctrl Pts',(1.32035743991852,2.76759128788277,-5.74489535244479)) ;
#152475=CARTESIAN_POINT('Ctrl Pts',(1.31824805546068,2.76910584227481,-5.7460376626109)) ;
#152476=CARTESIAN_POINT('Ctrl Pts',(1.31689309423375,2.77013099976529,-5.74677226335884)) ;
#152477=CARTESIAN_POINT('Ctrl Pts',(1.31545882361434,2.77127278201747,-5.74755112194074)) ;
#152478=CARTESIAN_POINT('Ctrl Pts',(1.31535582310955,2.77135510350023,-5.74760706165346)) ;
#152479=CARTESIAN_POINT('Ctrl Pts',(1.31504853092206,2.77160168095799,-5.74777397344699)) ;
#152480=CARTESIAN_POINT('Ctrl Pts',(1.31461168315424,2.77195498754746,-5.74801130685418)) ;
#152481=CARTESIAN_POINT('Ctrl Pts',(1.31417742224134,2.77231219724371,-5.74824733705709)) ;
#152482=CARTESIAN_POINT('Ctrl Pts',(1.31333096026311,2.77301480846574,-5.74870750613696)) ;
#152483=CARTESIAN_POINT('Ctrl Pts',(1.31272070342852,2.77353368974771,-5.7490394568406)) ;
#152484=CARTESIAN_POINT('Ctrl Pts',(1.3096977483713,2.77616736630459,-5.75068455723819)) ;
#152485=CARTESIAN_POINT('Ctrl Pts',(1.30737022788696,2.77840054644576,-5.7519534798951)) ;
#152486=CARTESIAN_POINT('Ctrl Pts',(1.30464757270882,2.78128817542225,-5.75343870334889)) ;
#152487=CARTESIAN_POINT('Ctrl Pts',(1.30414845981078,2.78182967606623,-5.75371101263076)) ;
#152488=CARTESIAN_POINT('Ctrl Pts',(1.30260826844056,2.78353926416388,-5.75455142863693)) ;
#152489=CARTESIAN_POINT('Ctrl Pts',(1.30158324720849,2.78473373830865,-5.75511123292138)) ;
#152490=CARTESIAN_POINT('Ctrl Pts',(1.30024935135332,2.78636738852737,-5.75583981271676)) ;
#152491=CARTESIAN_POINT('Ctrl Pts',(1.29991860867237,2.78677921519271,-5.75602047508104)) ;
#152492=CARTESIAN_POINT('Ctrl Pts',(1.29915346420734,2.78774794465154,-5.75643841922831)) ;
#152493=CARTESIAN_POINT('Ctrl Pts',(1.29872125904468,2.78830744810472,-5.75667449988731)) ;
#152494=CARTESIAN_POINT('Ctrl Pts',(1.29658637826222,2.79113377451591,-5.7578405320741)) ;
#152495=CARTESIAN_POINT('Ctrl Pts',(1.29496240940487,2.79348720429746,-5.75872698636979)) ;
#152496=CARTESIAN_POINT('Ctrl Pts',(1.29231665668155,2.79769679694547,-5.76017164800495)) ;
#152497=CARTESIAN_POINT('Ctrl Pts',(1.29125115601061,2.79951540543444,-5.7607540486807)) ;
#152498=CARTESIAN_POINT('Ctrl Pts',(1.28927619853496,2.80313430045115,-5.76183487898129)) ;
#152499=CARTESIAN_POINT('Ctrl Pts',(1.2883624199782,2.80493500363977,-5.76233537934595)) ;
#152500=CARTESIAN_POINT('Ctrl Pts',(1.28732027925585,2.80715235940913,-5.7629068412463)) ;
#152501=CARTESIAN_POINT('Ctrl Pts',(1.28695835013167,2.80793550920675,-5.76310538256458)) ;
#152502=CARTESIAN_POINT('Ctrl Pts',(1.28660568774191,2.80872522382218,-5.76329895629278)) ;
#152503=CARTESIAN_POINT('Ctrl Pts',(1.28608376699196,2.80991454434776,-5.76358549789851)) ;
#152504=CARTESIAN_POINT('Ctrl Pts',(1.28574525149601,2.81071375754613,-5.76377143189058)) ;
#152505=CARTESIAN_POINT('Ctrl Pts',(1.28475894023895,2.81312894312825,-5.76431326664902)) ;
#152506=CARTESIAN_POINT('Ctrl Pts',(1.28414040309303,2.81476247656144,-5.76465316629797)) ;
#152507=CARTESIAN_POINT('Ctrl Pts',(1.28339818260913,2.81688756020152,-5.765060888642)) ;
#152508=CARTESIAN_POINT('Ctrl Pts',(1.28323661013043,2.81736137575531,-5.76514963717807)) ;
#152509=CARTESIAN_POINT('Ctrl Pts',(1.28265668893879,2.81910411140438,-5.76546814735368)) ;
#152510=CARTESIAN_POINT('Ctrl Pts',(1.28225920250332,2.8203820528119,-5.76568639232524)) ;
#152511=CARTESIAN_POINT('Ctrl Pts',(1.28170385606936,2.8223005152677,-5.76599133498359)) ;
#152512=CARTESIAN_POINT('Ctrl Pts',(1.28152700208472,2.82293438010913,-5.76608844177028)) ;
#152513=CARTESIAN_POINT('Ctrl Pts',(1.28107448868731,2.82461913389174,-5.76633690914928)) ;
#152514=CARTESIAN_POINT('Ctrl Pts',(1.28081016954773,2.82567198476339,-5.76648198895407)) ;
#152515=CARTESIAN_POINT('Ctrl Pts',(1.28009910353322,2.82871092361134,-5.76687216801769)) ;
#152516=CARTESIAN_POINT('Ctrl Pts',(1.27969380338795,2.83071459002994,-5.76709487088005)) ;
#152517=CARTESIAN_POINT('Ctrl Pts',(1.27923282767965,2.83340629334537,-5.76734845373346)) ;
#152518=CARTESIAN_POINT('Ctrl Pts',(1.27912420342282,2.83408089926112,-5.76740823521583)) ;
#152519=CARTESIAN_POINT('Ctrl Pts',(1.27861441353188,2.83746106027947,-5.76768890881833)) ;
#152520=CARTESIAN_POINT('Ctrl Pts',(1.2783132428757,2.8401879948702,-5.76785509824336)) ;
#152521=CARTESIAN_POINT('Ctrl Pts',(1.27795656969993,2.8452797714154,-5.76805198665609)) ;
#152522=CARTESIAN_POINT('Ctrl Pts',(1.27787304021905,2.84764286211079,-5.7680981416173)) ;
#152523=CARTESIAN_POINT('Ctrl Pts',(1.27787304021905,2.85,-5.7680981416173)) ;
#152524=CARTESIAN_POINT('Origin',(1.3145125,4.45,-13.335)) ;
#152525=CARTESIAN_POINT('',(1.22107868287598,4.55,-13.1995951091212)) ;
#152526=CARTESIAN_POINT('',(1.22107868287598,4.55,-13.4704048908787)) ;
#152527=CARTESIAN_POINT('Origin',(1.3145125,4.55,-13.335)) ;
#152528=CARTESIAN_POINT('',(1.27787304021905,4.45,-13.2819018583827)) ;
#152529=CARTESIAN_POINT('Origin',(1.22107868287598,4.45,-13.1995951091212)) ;
#152530=CARTESIAN_POINT('',(1.27787304021905,4.45,-13.3880981416173)) ;
#152531=CARTESIAN_POINT('Origin',(1.3145125,4.45,-13.335)) ;
#152532=CARTESIAN_POINT('Origin',(1.22107868287598,4.45,-13.4704048908787)) ;
#152533=CARTESIAN_POINT('Origin',(-8.21365282185989E-16,2.85,-11.43)) ;
#152534=CARTESIAN_POINT('',(1.37603597336697,2.75,-13.335)) ;
#152535=CARTESIAN_POINT('Origin',(-8.13551212474381E-16,2.75,-11.43)) ;
#152536=CARTESIAN_POINT('',(1.27787304021905,2.85,-13.2819018583827)) ;
#152537=CARTESIAN_POINT('Ctrl Pts',(1.37603597336697,2.75,-13.335)) ;
#152538=CARTESIAN_POINT('Ctrl Pts',(1.37573512845501,2.75,-13.3348400290568)) ;
#152539=CARTESIAN_POINT('Ctrl Pts',(1.37513340737757,2.7500026571284,-13.3345201213288)) ;
#152540=CARTESIAN_POINT('Ctrl Pts',(1.37453174406033,2.75001064672752,-13.3342001889751)) ;
#152541=CARTESIAN_POINT('Ctrl Pts',(1.37388722675068,2.75002207412044,-13.333857355793)) ;
#152542=CARTESIAN_POINT('Ctrl Pts',(1.3735435038556,2.75002991650282,-13.3336744858378)) ;
#152543=CARTESIAN_POINT('Ctrl Pts',(1.37285611423781,2.75004911307826,-13.3333087011159)) ;
#152544=CARTESIAN_POINT('Ctrl Pts',(1.37251244753524,2.75006046723047,-13.3331257863885)) ;
#152545=CARTESIAN_POINT('Ctrl Pts',(1.3714815944481,2.75009981984526,-13.332577005305)) ;
#152546=CARTESIAN_POINT('Ctrl Pts',(1.37079455494331,2.75013310886333,-13.3322111017968)) ;
#152547=CARTESIAN_POINT('Ctrl Pts',(1.36873453110892,2.75025430438116,-13.3311134944134)) ;
#152548=CARTESIAN_POINT('Ctrl Pts',(1.36736263966051,2.75036354665964,-13.3303818907579)) ;
#152549=CARTESIAN_POINT('Ctrl Pts',(1.36413470836878,2.75068903914083,-13.3286589310622)) ;
#152550=CARTESIAN_POINT('Ctrl Pts',(1.36227932197147,2.75092980851023,-13.327667362279)) ;
#152551=CARTESIAN_POINT('Ctrl Pts',(1.35746012444742,2.75169859670383,-13.3250888180784)) ;
#152552=CARTESIAN_POINT('Ctrl Pts',(1.3545042583549,2.75231332717655,-13.3235042374589)) ;
#152553=CARTESIAN_POINT('Ctrl Pts',(1.34886973918565,2.75377034241467,-13.3204791694934)) ;
#152554=CARTESIAN_POINT('Ctrl Pts',(1.34617831568151,2.75459534478006,-13.3190321407416)) ;
#152555=CARTESIAN_POINT('Ctrl Pts',(1.34314242260183,2.75567798707052,-13.3173984698771)) ;
#152556=CARTESIAN_POINT('Ctrl Pts',(1.34256163823227,2.75588931242809,-13.317085898215)) ;
#152557=CARTESIAN_POINT('Ctrl Pts',(1.3419826199981,2.75610647364241,-13.3167742184185)) ;
#152558=CARTESIAN_POINT('Ctrl Pts',(1.34132160522921,2.7563569729086,-13.3164183780167)) ;
#152559=CARTESIAN_POINT('Ctrl Pts',(1.34086291435071,2.75653491456659,-13.3161714174681)) ;
#152560=CARTESIAN_POINT('Ctrl Pts',(1.33918548989956,2.75720079503573,-13.3152681624994)) ;
#152561=CARTESIAN_POINT('Ctrl Pts',(1.33797416370949,2.75771112313098,-13.3146156517349)) ;
#152562=CARTESIAN_POINT('Ctrl Pts',(1.33648532079706,2.75837521508446,-13.3138133670511)) ;
#152563=CARTESIAN_POINT('Ctrl Pts',(1.33619776328718,2.75850521488813,-13.3136584026979)) ;
#152564=CARTESIAN_POINT('Ctrl Pts',(1.33107968015567,2.76084915994947,-13.310899960288)) ;
#152565=CARTESIAN_POINT('Ctrl Pts',(1.32635908659362,2.76350693339075,-13.3083519804509)) ;
#152566=CARTESIAN_POINT('Ctrl Pts',(1.32109760625921,2.76707470328488,-13.3055052830876)) ;
#152567=CARTESIAN_POINT('Ctrl Pts',(1.32035743991769,2.76759128788335,-13.3051046475548)) ;
#152568=CARTESIAN_POINT('Ctrl Pts',(1.31824805546069,2.76910584227479,-13.3039623373891)) ;
#152569=CARTESIAN_POINT('Ctrl Pts',(1.31689309423375,2.77013099976527,-13.3032277366412)) ;
#152570=CARTESIAN_POINT('Ctrl Pts',(1.31545882361434,2.77127278201746,-13.3024488780593)) ;
#152571=CARTESIAN_POINT('Ctrl Pts',(1.31535582310956,2.77135510350021,-13.3023929383466)) ;
#152572=CARTESIAN_POINT('Ctrl Pts',(1.31504853092208,2.77160168095796,-13.302226026553)) ;
#152573=CARTESIAN_POINT('Ctrl Pts',(1.31461168315426,2.77195498754743,-13.3019886931459)) ;
#152574=CARTESIAN_POINT('Ctrl Pts',(1.31417742224136,2.77231219724367,-13.3017526629429)) ;
#152575=CARTESIAN_POINT('Ctrl Pts',(1.31333096026314,2.77301480846571,-13.3012924938631)) ;
#152576=CARTESIAN_POINT('Ctrl Pts',(1.31272070342854,2.77353368974768,-13.3009605431594)) ;
#152577=CARTESIAN_POINT('Ctrl Pts',(1.30969774837133,2.77616736630456,-13.2993154427618)) ;
#152578=CARTESIAN_POINT('Ctrl Pts',(1.30737022788699,2.77840054644573,-13.2980465201049)) ;
#152579=CARTESIAN_POINT('Ctrl Pts',(1.30464757270884,2.78128817542222,-13.2965612966511)) ;
#152580=CARTESIAN_POINT('Ctrl Pts',(1.30414845981078,2.7818296760662,-13.2962889873693)) ;
#152581=CARTESIAN_POINT('Ctrl Pts',(1.30260826844055,2.78353926416386,-13.2954485713631)) ;
#152582=CARTESIAN_POINT('Ctrl Pts',(1.30158324720848,2.78473373830863,-13.2948887670786)) ;
#152583=CARTESIAN_POINT('Ctrl Pts',(1.30024935135331,2.78636738852735,-13.2941601872833)) ;
#152584=CARTESIAN_POINT('Ctrl Pts',(1.29991860867236,2.78677921519269,-13.293979524919)) ;
#152585=CARTESIAN_POINT('Ctrl Pts',(1.29915346420733,2.78774794465152,-13.2935615807717)) ;
#152586=CARTESIAN_POINT('Ctrl Pts',(1.29872125904467,2.78830744810469,-13.2933255001127)) ;
#152587=CARTESIAN_POINT('Ctrl Pts',(1.29658637826221,2.79113377451589,-13.2921594679259)) ;
#152588=CARTESIAN_POINT('Ctrl Pts',(1.29496240940488,2.79348720429744,-13.2912730136302)) ;
#152589=CARTESIAN_POINT('Ctrl Pts',(1.29231665668155,2.79769679694545,-13.2898283519951)) ;
#152590=CARTESIAN_POINT('Ctrl Pts',(1.29125115601061,2.79951540543443,-13.2892459513193)) ;
#152591=CARTESIAN_POINT('Ctrl Pts',(1.28927619853495,2.80313430045115,-13.2881651210187)) ;
#152592=CARTESIAN_POINT('Ctrl Pts',(1.28836241997819,2.80493500363977,-13.2876646206541)) ;
#152593=CARTESIAN_POINT('Ctrl Pts',(1.28732027925585,2.80715235940913,-13.2870931587537)) ;
#152594=CARTESIAN_POINT('Ctrl Pts',(1.28695835013165,2.80793550920675,-13.2868946174355)) ;
#152595=CARTESIAN_POINT('Ctrl Pts',(1.2866056877419,2.80872522382218,-13.2867010437072)) ;
#152596=CARTESIAN_POINT('Ctrl Pts',(1.28608376699196,2.80991454434775,-13.2864145021015)) ;
#152597=CARTESIAN_POINT('Ctrl Pts',(1.285745251496,2.81071375754612,-13.2862285681094)) ;
#152598=CARTESIAN_POINT('Ctrl Pts',(1.28475894023895,2.81312894312824,-13.285686733351)) ;
#152599=CARTESIAN_POINT('Ctrl Pts',(1.28414040309303,2.81476247656143,-13.285346833702)) ;
#152600=CARTESIAN_POINT('Ctrl Pts',(1.28339818260913,2.8168875602015,-13.284939111358)) ;
#152601=CARTESIAN_POINT('Ctrl Pts',(1.28323661013044,2.81736137575529,-13.2848503628219)) ;
#152602=CARTESIAN_POINT('Ctrl Pts',(1.2826566889388,2.81910411140436,-13.2845318526463)) ;
#152603=CARTESIAN_POINT('Ctrl Pts',(1.28225920250333,2.82038205281188,-13.2843136076747)) ;
#152604=CARTESIAN_POINT('Ctrl Pts',(1.28170385606937,2.82230051526769,-13.2840086650164)) ;
#152605=CARTESIAN_POINT('Ctrl Pts',(1.28152700208473,2.82293438010912,-13.2839115582297)) ;
#152606=CARTESIAN_POINT('Ctrl Pts',(1.28107448868732,2.82461913389175,-13.2836630908507)) ;
#152607=CARTESIAN_POINT('Ctrl Pts',(1.28081016954773,2.82567198476339,-13.2835180110459)) ;
#152608=CARTESIAN_POINT('Ctrl Pts',(1.28009910353321,2.82871092361135,-13.2831278319823)) ;
#152609=CARTESIAN_POINT('Ctrl Pts',(1.27969380338794,2.83071459002995,-13.28290512912)) ;
#152610=CARTESIAN_POINT('Ctrl Pts',(1.27923282767964,2.83340629334539,-13.2826515462665)) ;
#152611=CARTESIAN_POINT('Ctrl Pts',(1.27912420342281,2.83408089926113,-13.2825917647842)) ;
#152612=CARTESIAN_POINT('Ctrl Pts',(1.27861441353187,2.83746106027949,-13.2823110911817)) ;
#152613=CARTESIAN_POINT('Ctrl Pts',(1.2783132428757,2.84018799487023,-13.2821449017566)) ;
#152614=CARTESIAN_POINT('Ctrl Pts',(1.27795656969994,2.84527977141544,-13.2819480133439)) ;
#152615=CARTESIAN_POINT('Ctrl Pts',(1.27787304021904,2.8476428621108,-13.2819018583827)) ;
#152616=CARTESIAN_POINT('Ctrl Pts',(1.27787304021905,2.85,-13.2819018583827)) ;
#152617=CARTESIAN_POINT('',(1.27787304021905,2.85,-9.57809814161729)) ;
#152618=CARTESIAN_POINT('Origin',(-8.21365282185989E-16,2.85,-11.43)) ;
#152619=CARTESIAN_POINT('Ctrl Pts',(1.37603597327321,2.75,-9.52500000004986)) ;
#152620=CARTESIAN_POINT('Ctrl Pts',(1.37573512836126,2.75000000000028,-9.52515997099309)) ;
#152621=CARTESIAN_POINT('Ctrl Pts',(1.37543426791168,2.7500013285371,-9.52531992481688)) ;
#152622=CARTESIAN_POINT('Ctrl Pts',(1.37483257571475,2.75000665190009,-9.5256398448573)) ;
#152623=CARTESIAN_POINT('Ctrl Pts',(1.37453174406034,2.75001064672751,-9.5257998110249)) ;
#152624=CARTESIAN_POINT('Ctrl Pts',(1.37388722675069,2.75002207412045,-9.52614264420698)) ;
#152625=CARTESIAN_POINT('Ctrl Pts',(1.37354350385557,2.75002991650282,-9.52632551416214)) ;
#152626=CARTESIAN_POINT('Ctrl Pts',(1.37285611423782,2.75004911307826,-9.52669129888408)) ;
#152627=CARTESIAN_POINT('Ctrl Pts',(1.37251244753524,2.75006046723047,-9.5268742136115)) ;
#152628=CARTESIAN_POINT('Ctrl Pts',(1.3714815944481,2.75009981984526,-9.52742299469495)) ;
#152629=CARTESIAN_POINT('Ctrl Pts',(1.37079455494331,2.75013310886333,-9.52778889820318)) ;
#152630=CARTESIAN_POINT('Ctrl Pts',(1.36873453110892,2.75025430438116,-9.52888650558661)) ;
#152631=CARTESIAN_POINT('Ctrl Pts',(1.36736263966051,2.75036354665964,-9.52961810924203)) ;
#152632=CARTESIAN_POINT('Ctrl Pts',(1.36413470836879,2.75068903914083,-9.5313410689378)) ;
#152633=CARTESIAN_POINT('Ctrl Pts',(1.36227932197147,2.75092980851024,-9.53233263772104)) ;
#152634=CARTESIAN_POINT('Ctrl Pts',(1.35746012444742,2.75169859670383,-9.53491118192157)) ;
#152635=CARTESIAN_POINT('Ctrl Pts',(1.35450425835489,2.75231332717654,-9.53649576254107)) ;
#152636=CARTESIAN_POINT('Ctrl Pts',(1.34886973918565,2.75377034241467,-9.53952083050663)) ;
#152637=CARTESIAN_POINT('Ctrl Pts',(1.34617831568151,2.75459534478006,-9.54096785925841)) ;
#152638=CARTESIAN_POINT('Ctrl Pts',(1.34314242260183,2.75567798707052,-9.54260153012296)) ;
#152639=CARTESIAN_POINT('Ctrl Pts',(1.34256163823227,2.75588931242809,-9.54291410178499)) ;
#152640=CARTESIAN_POINT('Ctrl Pts',(1.3419826199981,2.75610647364241,-9.54322578158149)) ;
#152641=CARTESIAN_POINT('Ctrl Pts',(1.34132160522921,2.7563569729086,-9.54358162198333)) ;
#152642=CARTESIAN_POINT('Ctrl Pts',(1.34086291435071,2.75653491456659,-9.54382858253193)) ;
#152643=CARTESIAN_POINT('Ctrl Pts',(1.33918548989956,2.75720079503573,-9.54473183750056)) ;
#152644=CARTESIAN_POINT('Ctrl Pts',(1.33797416370949,2.75771112313098,-9.54538434826513)) ;
#152645=CARTESIAN_POINT('Ctrl Pts',(1.33648532079706,2.75837521508445,-9.5461866329489)) ;
#152646=CARTESIAN_POINT('Ctrl Pts',(1.33619776328718,2.75850521488811,-9.5463415973021)) ;
#152647=CARTESIAN_POINT('Ctrl Pts',(1.33107968015623,2.7608491599492,-9.54910003971169)) ;
#152648=CARTESIAN_POINT('Ctrl Pts',(1.32635908659471,2.76350693339014,-9.55164801954852)) ;
#152649=CARTESIAN_POINT('Ctrl Pts',(1.32109760626024,2.76707470328417,-9.55449471691189)) ;
#152650=CARTESIAN_POINT('Ctrl Pts',(1.3203574399182,2.767591287883,-9.55489535244495)) ;
#152651=CARTESIAN_POINT('Ctrl Pts',(1.31824805546069,2.7691058422748,-9.55603766261088)) ;
#152652=CARTESIAN_POINT('Ctrl Pts',(1.31689309423376,2.77013099976528,-9.55677226335883)) ;
#152653=CARTESIAN_POINT('Ctrl Pts',(1.31545882361435,2.77127278201747,-9.55755112194072)) ;
#152654=CARTESIAN_POINT('Ctrl Pts',(1.31535582310957,2.77135510350022,-9.55760706165345)) ;
#152655=CARTESIAN_POINT('Ctrl Pts',(1.31504853092209,2.77160168095797,-9.55777397344697)) ;
#152656=CARTESIAN_POINT('Ctrl Pts',(1.31461168315425,2.77195498754744,-9.55801130685416)) ;
#152657=CARTESIAN_POINT('Ctrl Pts',(1.31417742224137,2.77231219724368,-9.55824733705706)) ;
#152658=CARTESIAN_POINT('Ctrl Pts',(1.31333096026314,2.77301480846571,-9.55870750613694)) ;
#152659=CARTESIAN_POINT('Ctrl Pts',(1.31272070342855,2.77353368974768,-9.55903945684058)) ;
#152660=CARTESIAN_POINT('Ctrl Pts',(1.30969774837134,2.77616736630456,-9.56068455723817)) ;
#152661=CARTESIAN_POINT('Ctrl Pts',(1.30737022788701,2.77840054644572,-9.56195347989507)) ;
#152662=CARTESIAN_POINT('Ctrl Pts',(1.30464757270885,2.78128817542222,-9.56343870334886)) ;
#152663=CARTESIAN_POINT('Ctrl Pts',(1.3041484598108,2.78182967606622,-9.56371101263075)) ;
#152664=CARTESIAN_POINT('Ctrl Pts',(1.30260826844056,2.78353926416388,-9.56455142863692)) ;
#152665=CARTESIAN_POINT('Ctrl Pts',(1.30158324720849,2.78473373830865,-9.56511123292138)) ;
#152666=CARTESIAN_POINT('Ctrl Pts',(1.30024935135332,2.78636738852738,-9.56583981271676)) ;
#152667=CARTESIAN_POINT('Ctrl Pts',(1.29991860867237,2.78677921519272,-9.56602047508104)) ;
#152668=CARTESIAN_POINT('Ctrl Pts',(1.29915346420735,2.78774794465155,-9.5664384192283)) ;
#152669=CARTESIAN_POINT('Ctrl Pts',(1.29872125904468,2.78830744810473,-9.56667449988731)) ;
#152670=CARTESIAN_POINT('Ctrl Pts',(1.29658637826222,2.79113377451592,-9.5678405320741)) ;
#152671=CARTESIAN_POINT('Ctrl Pts',(1.29496240940488,2.79348720429747,-9.56872698636979)) ;
#152672=CARTESIAN_POINT('Ctrl Pts',(1.29231665668155,2.79769679694547,-9.57017164800495)) ;
#152673=CARTESIAN_POINT('Ctrl Pts',(1.29125115601061,2.79951540543444,-9.5707540486807)) ;
#152674=CARTESIAN_POINT('Ctrl Pts',(1.28927619853496,2.80313430045115,-9.57183487898129)) ;
#152675=CARTESIAN_POINT('Ctrl Pts',(1.2883624199782,2.80493500363977,-9.57233537934596)) ;
#152676=CARTESIAN_POINT('Ctrl Pts',(1.28732027925585,2.80715235940913,-9.5729068412463)) ;
#152677=CARTESIAN_POINT('Ctrl Pts',(1.28695835013167,2.80793550920673,-9.57310538256458)) ;
#152678=CARTESIAN_POINT('Ctrl Pts',(1.28660568774191,2.80872522382218,-9.57329895629278)) ;
#152679=CARTESIAN_POINT('Ctrl Pts',(1.28608376699196,2.80991454434775,-9.57358549789851)) ;
#152680=CARTESIAN_POINT('Ctrl Pts',(1.28574525149602,2.81071375754612,-9.57377143189058)) ;
#152681=CARTESIAN_POINT('Ctrl Pts',(1.28475894023896,2.81312894312824,-9.57431326664902)) ;
#152682=CARTESIAN_POINT('Ctrl Pts',(1.28414040309303,2.81476247656142,-9.57465316629797)) ;
#152683=CARTESIAN_POINT('Ctrl Pts',(1.28339818260913,2.8168875602015,-9.575060888642)) ;
#152684=CARTESIAN_POINT('Ctrl Pts',(1.28323661013044,2.81736137575528,-9.57514963717806)) ;
#152685=CARTESIAN_POINT('Ctrl Pts',(1.2826566889388,2.81910411140435,-9.57546814735368)) ;
#152686=CARTESIAN_POINT('Ctrl Pts',(1.28225920250333,2.82038205281187,-9.57568639232524)) ;
#152687=CARTESIAN_POINT('Ctrl Pts',(1.28170385606936,2.82230051526768,-9.57599133498359)) ;
#152688=CARTESIAN_POINT('Ctrl Pts',(1.28152700208472,2.82293438010912,-9.57608844177028)) ;
#152689=CARTESIAN_POINT('Ctrl Pts',(1.28107448868731,2.82461913389174,-9.57633690914928)) ;
#152690=CARTESIAN_POINT('Ctrl Pts',(1.28081016954773,2.82567198476339,-9.57648198895408)) ;
#152691=CARTESIAN_POINT('Ctrl Pts',(1.28009910353322,2.82871092361134,-9.57687216801769)) ;
#152692=CARTESIAN_POINT('Ctrl Pts',(1.27969380338795,2.83071459002995,-9.57709487088005)) ;
#152693=CARTESIAN_POINT('Ctrl Pts',(1.27923282767965,2.83340629334538,-9.57734845373346)) ;
#152694=CARTESIAN_POINT('Ctrl Pts',(1.27912420342282,2.83408089926112,-9.57740823521583)) ;
#152695=CARTESIAN_POINT('Ctrl Pts',(1.27861441353188,2.83746106027948,-9.57768890881833)) ;
#152696=CARTESIAN_POINT('Ctrl Pts',(1.2783132428757,2.84018799487021,-9.57785509824336)) ;
#152697=CARTESIAN_POINT('Ctrl Pts',(1.27795656969993,2.84527977141542,-9.57805198665609)) ;
#152698=CARTESIAN_POINT('Ctrl Pts',(1.27787304021905,2.84764286211079,-9.57809814161729)) ;
#152699=CARTESIAN_POINT('Ctrl Pts',(1.27787304021905,2.85,-9.57809814161729)) ;
#152700=CARTESIAN_POINT('Origin',(1.3145125,4.45,-17.145)) ;
#152701=CARTESIAN_POINT('',(1.22107868287598,4.55,-17.0095951091213)) ;
#152702=CARTESIAN_POINT('',(1.22107868287598,4.55,-17.2804048908787)) ;
#152703=CARTESIAN_POINT('Origin',(1.3145125,4.55,-17.145)) ;
#152704=CARTESIAN_POINT('',(1.27787304021905,4.45,-17.0919018583827)) ;
#152705=CARTESIAN_POINT('Origin',(1.22107868287598,4.45,-17.0095951091213)) ;
#152706=CARTESIAN_POINT('',(1.27787304021905,4.45,-17.1980981416173)) ;
#152707=CARTESIAN_POINT('Origin',(1.3145125,4.45,-17.145)) ;
#152708=CARTESIAN_POINT('Origin',(1.22107868287598,4.45,-17.2804048908787)) ;
#152709=CARTESIAN_POINT('Origin',(-8.21365282185989E-16,2.85,-15.24)) ;
#152710=CARTESIAN_POINT('',(1.37603597336697,2.75,-17.145)) ;
#152711=CARTESIAN_POINT('Origin',(-8.13551212474381E-16,2.75,-15.24)) ;
#152712=CARTESIAN_POINT('',(1.27787304021905,2.85,-17.0919018583827)) ;
#152713=CARTESIAN_POINT('Ctrl Pts',(1.37603597336697,2.75,-17.145)) ;
#152714=CARTESIAN_POINT('Ctrl Pts',(1.37543428354306,2.75,-17.1446800581135)) ;
#152715=CARTESIAN_POINT('Ctrl Pts',(1.37483253111456,2.75000531372589,-17.1443601843412)) ;
#152716=CARTESIAN_POINT('Ctrl Pts',(1.37388722675069,2.75002207412045,-17.143857355793)) ;
#152717=CARTESIAN_POINT('Ctrl Pts',(1.37354350385561,2.75002991650282,-17.1436744858378)) ;
#152718=CARTESIAN_POINT('Ctrl Pts',(1.37285611423782,2.75004911307826,-17.1433087011159)) ;
#152719=CARTESIAN_POINT('Ctrl Pts',(1.37251244753524,2.75006046723047,-17.1431257863885)) ;
#152720=CARTESIAN_POINT('Ctrl Pts',(1.3714815944481,2.75009981984526,-17.142577005305)) ;
#152721=CARTESIAN_POINT('Ctrl Pts',(1.37079455494331,2.75013310886333,-17.1422111017968)) ;
#152722=CARTESIAN_POINT('Ctrl Pts',(1.36873453110892,2.75025430438115,-17.1411134944134)) ;
#152723=CARTESIAN_POINT('Ctrl Pts',(1.36736263966051,2.75036354665963,-17.1403818907579)) ;
#152724=CARTESIAN_POINT('Ctrl Pts',(1.36413470836879,2.75068903914081,-17.1386589310622)) ;
#152725=CARTESIAN_POINT('Ctrl Pts',(1.36227932197147,2.75092980851021,-17.137667362279)) ;
#152726=CARTESIAN_POINT('Ctrl Pts',(1.35746012444742,2.7516985967038,-17.1350888180784)) ;
#152727=CARTESIAN_POINT('Ctrl Pts',(1.35450425835489,2.75231332717651,-17.1335042374589)) ;
#152728=CARTESIAN_POINT('Ctrl Pts',(1.34886973918565,2.75377034241464,-17.1304791694934)) ;
#152729=CARTESIAN_POINT('Ctrl Pts',(1.3461783156815,2.75459534478002,-17.1290321407416)) ;
#152730=CARTESIAN_POINT('Ctrl Pts',(1.34314242260183,2.75567798707048,-17.1273984698771)) ;
#152731=CARTESIAN_POINT('Ctrl Pts',(1.34256163823226,2.75588931242806,-17.127085898215)) ;
#152732=CARTESIAN_POINT('Ctrl Pts',(1.34198261999809,2.75610647364238,-17.1267742184185)) ;
#152733=CARTESIAN_POINT('Ctrl Pts',(1.3413216052292,2.75635697290856,-17.1264183780167)) ;
#152734=CARTESIAN_POINT('Ctrl Pts',(1.3408629143507,2.75653491456656,-17.1261714174681)) ;
#152735=CARTESIAN_POINT('Ctrl Pts',(1.33918548989955,2.7572007950357,-17.1252681624994)) ;
#152736=CARTESIAN_POINT('Ctrl Pts',(1.33797416370948,2.75771112313095,-17.1246156517348)) ;
#152737=CARTESIAN_POINT('Ctrl Pts',(1.33648532079705,2.75837521508443,-17.1238133670511)) ;
#152738=CARTESIAN_POINT('Ctrl Pts',(1.33619776328717,2.7585052148881,-17.1236584026979)) ;
#152739=CARTESIAN_POINT('Ctrl Pts',(1.33107968015588,2.76084915994935,-17.1208999602881)) ;
#152740=CARTESIAN_POINT('Ctrl Pts',(1.32635908659402,2.76350693339051,-17.1183519804511)) ;
#152741=CARTESIAN_POINT('Ctrl Pts',(1.32109760625958,2.76707470328462,-17.1155052830878)) ;
#152742=CARTESIAN_POINT('Ctrl Pts',(1.32035743991785,2.76759128788324,-17.1151046475549)) ;
#152743=CARTESIAN_POINT('Ctrl Pts',(1.31824805546066,2.76910584227481,-17.1139623373891)) ;
#152744=CARTESIAN_POINT('Ctrl Pts',(1.31689309423374,2.77013099976528,-17.1132277366412)) ;
#152745=CARTESIAN_POINT('Ctrl Pts',(1.31545882361432,2.77127278201747,-17.1124488780593)) ;
#152746=CARTESIAN_POINT('Ctrl Pts',(1.31535582310953,2.77135510350024,-17.1123929383466)) ;
#152747=CARTESIAN_POINT('Ctrl Pts',(1.31504853092203,2.771601680958,-17.112226026553)) ;
#152748=CARTESIAN_POINT('Ctrl Pts',(1.31461168315421,2.77195498754747,-17.1119886931459)) ;
#152749=CARTESIAN_POINT('Ctrl Pts',(1.31417742224132,2.77231219724372,-17.1117526629429)) ;
#152750=CARTESIAN_POINT('Ctrl Pts',(1.31333096026309,2.77301480846575,-17.1112924938631)) ;
#152751=CARTESIAN_POINT('Ctrl Pts',(1.31272070342849,2.77353368974772,-17.1109605431594)) ;
#152752=CARTESIAN_POINT('Ctrl Pts',(1.30969774837127,2.77616736630461,-17.1093154427618)) ;
#152753=CARTESIAN_POINT('Ctrl Pts',(1.30737022788694,2.77840054644579,-17.1080465201049)) ;
#152754=CARTESIAN_POINT('Ctrl Pts',(1.3046475727088,2.78128817542226,-17.1065612966511)) ;
#152755=CARTESIAN_POINT('Ctrl Pts',(1.30414845981076,2.78182967606623,-17.1062889873693)) ;
#152756=CARTESIAN_POINT('Ctrl Pts',(1.30260826844056,2.78353926416388,-17.1054485713631)) ;
#152757=CARTESIAN_POINT('Ctrl Pts',(1.30158324720849,2.78473373830866,-17.1048887670786)) ;
#152758=CARTESIAN_POINT('Ctrl Pts',(1.30024935135332,2.78636738852739,-17.1041601872832)) ;
#152759=CARTESIAN_POINT('Ctrl Pts',(1.29991860867237,2.78677921519272,-17.103979524919)) ;
#152760=CARTESIAN_POINT('Ctrl Pts',(1.29915346420734,2.78774794465155,-17.1035615807717)) ;
#152761=CARTESIAN_POINT('Ctrl Pts',(1.29872125904467,2.78830744810473,-17.1033255001127)) ;
#152762=CARTESIAN_POINT('Ctrl Pts',(1.2965863782622,2.79113377451592,-17.1021594679259)) ;
#152763=CARTESIAN_POINT('Ctrl Pts',(1.29496240940485,2.79348720429746,-17.1012730136302)) ;
#152764=CARTESIAN_POINT('Ctrl Pts',(1.29231665668153,2.79769679694546,-17.099828351995)) ;
#152765=CARTESIAN_POINT('Ctrl Pts',(1.29125115601059,2.79951540543443,-17.0992459513193)) ;
#152766=CARTESIAN_POINT('Ctrl Pts',(1.28927619853494,2.80313430045113,-17.0981651210187)) ;
#152767=CARTESIAN_POINT('Ctrl Pts',(1.28836241997818,2.80493500363976,-17.097664620654)) ;
#152768=CARTESIAN_POINT('Ctrl Pts',(1.28732027925584,2.80715235940912,-17.0970931587537)) ;
#152769=CARTESIAN_POINT('Ctrl Pts',(1.28695835013164,2.80793550920672,-17.0968946174353)) ;
#152770=CARTESIAN_POINT('Ctrl Pts',(1.28660568774189,2.80872522382217,-17.0967010437072)) ;
#152771=CARTESIAN_POINT('Ctrl Pts',(1.28608376699194,2.80991454434775,-17.0964145021015)) ;
#152772=CARTESIAN_POINT('Ctrl Pts',(1.28574525149599,2.81071375754612,-17.0962285681094)) ;
#152773=CARTESIAN_POINT('Ctrl Pts',(1.28475894023894,2.81312894312825,-17.095686733351)) ;
#152774=CARTESIAN_POINT('Ctrl Pts',(1.28414040309302,2.81476247656145,-17.095346833702)) ;
#152775=CARTESIAN_POINT('Ctrl Pts',(1.28339818260912,2.81688756020153,-17.094939111358)) ;
#152776=CARTESIAN_POINT('Ctrl Pts',(1.28323661013042,2.81736137575532,-17.0948503628219)) ;
#152777=CARTESIAN_POINT('Ctrl Pts',(1.28265668893879,2.8191041114044,-17.0945318526463)) ;
#152778=CARTESIAN_POINT('Ctrl Pts',(1.28225920250332,2.82038205281193,-17.0943136076747)) ;
#152779=CARTESIAN_POINT('Ctrl Pts',(1.28170385606936,2.82230051526773,-17.0940086650164)) ;
#152780=CARTESIAN_POINT('Ctrl Pts',(1.28152700208472,2.82293438010914,-17.0939115582297)) ;
#152781=CARTESIAN_POINT('Ctrl Pts',(1.28107448868731,2.82461913389175,-17.0936630908507)) ;
#152782=CARTESIAN_POINT('Ctrl Pts',(1.28081016954772,2.82567198476339,-17.0935180110459)) ;
#152783=CARTESIAN_POINT('Ctrl Pts',(1.2800991035332,2.82871092361134,-17.0931278319823)) ;
#152784=CARTESIAN_POINT('Ctrl Pts',(1.27969380338793,2.83071459002993,-17.0929051291199)) ;
#152785=CARTESIAN_POINT('Ctrl Pts',(1.27923282767964,2.83340629334536,-17.0926515462665)) ;
#152786=CARTESIAN_POINT('Ctrl Pts',(1.27912420342281,2.8340808992611,-17.0925917647842)) ;
#152787=CARTESIAN_POINT('Ctrl Pts',(1.27861441353188,2.83746106027945,-17.0923110911817)) ;
#152788=CARTESIAN_POINT('Ctrl Pts',(1.27831324287571,2.84018799487017,-17.0921449017566)) ;
#152789=CARTESIAN_POINT('Ctrl Pts',(1.27795656969996,2.84527977141539,-17.0919480133439)) ;
#152790=CARTESIAN_POINT('Ctrl Pts',(1.27787304021907,2.84764286211077,-17.0919018583827)) ;
#152791=CARTESIAN_POINT('Ctrl Pts',(1.27787304021907,2.85,-17.0919018583827)) ;
#152792=CARTESIAN_POINT('',(1.27787304021905,2.85,-13.3880981416173)) ;
#152793=CARTESIAN_POINT('Origin',(-8.21365282185989E-16,2.85,-15.24)) ;
#152794=CARTESIAN_POINT('Ctrl Pts',(1.37603597336697,2.75,-13.335)) ;
#152795=CARTESIAN_POINT('Ctrl Pts',(1.37573512845505,2.75,-13.3351599709432)) ;
#152796=CARTESIAN_POINT('Ctrl Pts',(1.37543426791753,2.75000132857281,-13.3353199248048)) ;
#152797=CARTESIAN_POINT('Ctrl Pts',(1.37483257571477,2.75000665190009,-13.3356398448574)) ;
#152798=CARTESIAN_POINT('Ctrl Pts',(1.37453174406036,2.75001064672752,-13.335799811025)) ;
#152799=CARTESIAN_POINT('Ctrl Pts',(1.3738872267507,2.75002207412044,-13.3361426442071)) ;
#152800=CARTESIAN_POINT('Ctrl Pts',(1.37354350385558,2.75002991650282,-13.3363255141619)) ;
#152801=CARTESIAN_POINT('Ctrl Pts',(1.37285611423782,2.75004911307826,-13.3366912988841)) ;
#152802=CARTESIAN_POINT('Ctrl Pts',(1.37251244753524,2.75006046723047,-13.3368742136115)) ;
#152803=CARTESIAN_POINT('Ctrl Pts',(1.37148159444809,2.75009981984526,-13.337422994695)) ;
#152804=CARTESIAN_POINT('Ctrl Pts',(1.37079455494331,2.75013310886333,-13.3377888982032)) ;
#152805=CARTESIAN_POINT('Ctrl Pts',(1.36873453110893,2.75025430438115,-13.3388865055866)) ;
#152806=CARTESIAN_POINT('Ctrl Pts',(1.36736263966052,2.75036354665962,-13.3396181092421)) ;
#152807=CARTESIAN_POINT('Ctrl Pts',(1.36413470836879,2.7506890391408,-13.3413410689378)) ;
#152808=CARTESIAN_POINT('Ctrl Pts',(1.36227932197148,2.7509298085102,-13.342332637721)) ;
#152809=CARTESIAN_POINT('Ctrl Pts',(1.35746012444742,2.75169859670378,-13.3449111819216)) ;
#152810=CARTESIAN_POINT('Ctrl Pts',(1.35450425835489,2.75231332717648,-13.3464957625411)) ;
#152811=CARTESIAN_POINT('Ctrl Pts',(1.34886973918563,2.7537703424146,-13.3495208305066)) ;
#152812=CARTESIAN_POINT('Ctrl Pts',(1.34617831568149,2.75459534477999,-13.3509678592584)) ;
#152813=CARTESIAN_POINT('Ctrl Pts',(1.34314242260182,2.75567798707045,-13.352601530123)) ;
#152814=CARTESIAN_POINT('Ctrl Pts',(1.34256163823225,2.75588931242803,-13.352914101785)) ;
#152815=CARTESIAN_POINT('Ctrl Pts',(1.34198261999808,2.75610647364235,-13.3532257815815)) ;
#152816=CARTESIAN_POINT('Ctrl Pts',(1.34132160522919,2.75635697290854,-13.3535816219834)) ;
#152817=CARTESIAN_POINT('Ctrl Pts',(1.34086291435069,2.75653491456653,-13.3538285825319)) ;
#152818=CARTESIAN_POINT('Ctrl Pts',(1.33918548989955,2.75720079503567,-13.3547318375006)) ;
#152819=CARTESIAN_POINT('Ctrl Pts',(1.33797416370947,2.75771112313093,-13.3553843482652)) ;
#152820=CARTESIAN_POINT('Ctrl Pts',(1.33648532079705,2.75837521508441,-13.3561866329489)) ;
#152821=CARTESIAN_POINT('Ctrl Pts',(1.33619776328717,2.75850521488808,-13.3563415973022)) ;
#152822=CARTESIAN_POINT('Ctrl Pts',(1.33107968015608,2.76084915994924,-13.3591000397118)) ;
#152823=CARTESIAN_POINT('Ctrl Pts',(1.32635908659443,2.76350693339028,-13.3616480195487)) ;
#152824=CARTESIAN_POINT('Ctrl Pts',(1.32109760625997,2.76707470328435,-13.364494716912)) ;
#152825=CARTESIAN_POINT('Ctrl Pts',(1.32035743991805,2.7675912878831,-13.364895352445)) ;
#152826=CARTESIAN_POINT('Ctrl Pts',(1.31824805546067,2.76910584227481,-13.3660376626109)) ;
#152827=CARTESIAN_POINT('Ctrl Pts',(1.31689309423375,2.77013099976529,-13.3667722633588)) ;
#152828=CARTESIAN_POINT('Ctrl Pts',(1.31545882361433,2.77127278201748,-13.3675511219407)) ;
#152829=CARTESIAN_POINT('Ctrl Pts',(1.31535582310954,2.77135510350024,-13.3676070616534)) ;
#152830=CARTESIAN_POINT('Ctrl Pts',(1.31504853092205,2.77160168095801,-13.367773973447)) ;
#152831=CARTESIAN_POINT('Ctrl Pts',(1.31461168315421,2.77195498754746,-13.3680113068541)) ;
#152832=CARTESIAN_POINT('Ctrl Pts',(1.31417742224133,2.77231219724372,-13.3682473370571)) ;
#152833=CARTESIAN_POINT('Ctrl Pts',(1.3133309602631,2.77301480846575,-13.3687075061369)) ;
#152834=CARTESIAN_POINT('Ctrl Pts',(1.31272070342851,2.77353368974773,-13.3690394568406)) ;
#152835=CARTESIAN_POINT('Ctrl Pts',(1.30969774837129,2.77616736630461,-13.3706845572382)) ;
#152836=CARTESIAN_POINT('Ctrl Pts',(1.30737022788695,2.77840054644579,-13.3719534798951)) ;
#152837=CARTESIAN_POINT('Ctrl Pts',(1.30464757270881,2.78128817542227,-13.3734387033489)) ;
#152838=CARTESIAN_POINT('Ctrl Pts',(1.30414845981078,2.78182967606624,-13.3737110126307)) ;
#152839=CARTESIAN_POINT('Ctrl Pts',(1.30260826844057,2.78353926416389,-13.3745514286369)) ;
#152840=CARTESIAN_POINT('Ctrl Pts',(1.30158324720849,2.78473373830867,-13.3751112329214)) ;
#152841=CARTESIAN_POINT('Ctrl Pts',(1.30024935135332,2.7863673885274,-13.3758398127168)) ;
#152842=CARTESIAN_POINT('Ctrl Pts',(1.29991860867237,2.78677921519273,-13.376020475081)) ;
#152843=CARTESIAN_POINT('Ctrl Pts',(1.29915346420734,2.78774794465156,-13.3764384192283)) ;
#152844=CARTESIAN_POINT('Ctrl Pts',(1.29872125904468,2.78830744810474,-13.3766744998873)) ;
#152845=CARTESIAN_POINT('Ctrl Pts',(1.29658637826221,2.79113377451593,-13.3778405320741)) ;
#152846=CARTESIAN_POINT('Ctrl Pts',(1.29496240940486,2.79348720429747,-13.3787269863698)) ;
#152847=CARTESIAN_POINT('Ctrl Pts',(1.29231665668153,2.79769679694547,-13.3801716480049)) ;
#152848=CARTESIAN_POINT('Ctrl Pts',(1.29125115601059,2.79951540543443,-13.3807540486807)) ;
#152849=CARTESIAN_POINT('Ctrl Pts',(1.28927619853494,2.80313430045114,-13.3818348789813)) ;
#152850=CARTESIAN_POINT('Ctrl Pts',(1.28836241997818,2.80493500363976,-13.382335379346)) ;
#152851=CARTESIAN_POINT('Ctrl Pts',(1.28732027925584,2.80715235940912,-13.3829068412463)) ;
#152852=CARTESIAN_POINT('Ctrl Pts',(1.28695835013164,2.80793550920674,-13.3831053825645)) ;
#152853=CARTESIAN_POINT('Ctrl Pts',(1.28660568774189,2.80872522382217,-13.3832989562928)) ;
#152854=CARTESIAN_POINT('Ctrl Pts',(1.28608376699195,2.80991454434774,-13.3835854978985)) ;
#152855=CARTESIAN_POINT('Ctrl Pts',(1.285745251496,2.81071375754611,-13.3837714318906)) ;
#152856=CARTESIAN_POINT('Ctrl Pts',(1.28475894023895,2.81312894312824,-13.384313266649)) ;
#152857=CARTESIAN_POINT('Ctrl Pts',(1.28414040309303,2.81476247656143,-13.384653166298)) ;
#152858=CARTESIAN_POINT('Ctrl Pts',(1.28339818260913,2.81688756020151,-13.385060888642)) ;
#152859=CARTESIAN_POINT('Ctrl Pts',(1.28323661013044,2.8173613757553,-13.3851496371781)) ;
#152860=CARTESIAN_POINT('Ctrl Pts',(1.28265668893881,2.81910411140437,-13.3854681473537)) ;
#152861=CARTESIAN_POINT('Ctrl Pts',(1.28225920250334,2.82038205281189,-13.3856863923252)) ;
#152862=CARTESIAN_POINT('Ctrl Pts',(1.28170385606938,2.8223005152677,-13.3859913349836)) ;
#152863=CARTESIAN_POINT('Ctrl Pts',(1.28152700208474,2.82293438010913,-13.3860884417703)) ;
#152864=CARTESIAN_POINT('Ctrl Pts',(1.28107448868732,2.82461913389175,-13.3863369091493)) ;
#152865=CARTESIAN_POINT('Ctrl Pts',(1.28081016954773,2.8256719847634,-13.3864819889541)) ;
#152866=CARTESIAN_POINT('Ctrl Pts',(1.28009910353321,2.82871092361134,-13.3868721680177)) ;
#152867=CARTESIAN_POINT('Ctrl Pts',(1.27969380338794,2.83071459002995,-13.38709487088)) ;
#152868=CARTESIAN_POINT('Ctrl Pts',(1.27923282767964,2.83340629334538,-13.3873484537334)) ;
#152869=CARTESIAN_POINT('Ctrl Pts',(1.27912420342282,2.83408089926112,-13.3874082352158)) ;
#152870=CARTESIAN_POINT('Ctrl Pts',(1.27861441353188,2.83746106027948,-13.3876889088183)) ;
#152871=CARTESIAN_POINT('Ctrl Pts',(1.2783132428757,2.84018799487021,-13.3878550982434)) ;
#152872=CARTESIAN_POINT('Ctrl Pts',(1.27795656969994,2.84527977141541,-13.3880519866561)) ;
#152873=CARTESIAN_POINT('Ctrl Pts',(1.27787304021904,2.84764286211079,-13.3880981416173)) ;
#152874=CARTESIAN_POINT('Ctrl Pts',(1.27787304021904,2.85,-13.3880981416173)) ;
#152875=CARTESIAN_POINT('Origin',(1.3145125,4.45,-20.955)) ;
#152876=CARTESIAN_POINT('',(1.22107868287598,4.55,-20.8195951091213)) ;
#152877=CARTESIAN_POINT('',(1.22107868287598,4.55,-21.0904048908787)) ;
#152878=CARTESIAN_POINT('Origin',(1.3145125,4.55,-20.955)) ;
#152879=CARTESIAN_POINT('',(1.27787304021905,4.45,-20.9019018583827)) ;
#152880=CARTESIAN_POINT('Origin',(1.22107868287598,4.45,-20.8195951091213)) ;
#152881=CARTESIAN_POINT('',(1.27787304021905,4.45,-21.0080981416173)) ;
#152882=CARTESIAN_POINT('Origin',(1.3145125,4.45,-20.955)) ;
#152883=CARTESIAN_POINT('Origin',(1.22107868287598,4.45,-21.0904048908787)) ;
#152884=CARTESIAN_POINT('Origin',(-8.21365282185989E-16,2.85,-19.05)) ;
#152885=CARTESIAN_POINT('',(1.37603597336697,2.75,-20.955)) ;
#152886=CARTESIAN_POINT('Origin',(-8.13551212474381E-16,2.75,-19.05)) ;
#152887=CARTESIAN_POINT('',(1.27787304021905,2.85,-20.9019018583827)) ;
#152888=CARTESIAN_POINT('Ctrl Pts',(1.37603597336697,2.75,-20.955)) ;
#152889=CARTESIAN_POINT('Ctrl Pts',(1.37543428354306,2.75,-20.9546800581135)) ;
#152890=CARTESIAN_POINT('Ctrl Pts',(1.37483253111456,2.7500053137259,-20.9543601843411)) ;
#152891=CARTESIAN_POINT('Ctrl Pts',(1.37388722675069,2.75002207412044,-20.9538573557929)) ;
#152892=CARTESIAN_POINT('Ctrl Pts',(1.37354350385561,2.75002991650282,-20.9536744858381)) ;
#152893=CARTESIAN_POINT('Ctrl Pts',(1.37285611423782,2.75004911307826,-20.9533087011159)) ;
#152894=CARTESIAN_POINT('Ctrl Pts',(1.37251244753524,2.75006046723047,-20.9531257863885)) ;
#152895=CARTESIAN_POINT('Ctrl Pts',(1.3714815944481,2.75009981984526,-20.952577005305)) ;
#152896=CARTESIAN_POINT('Ctrl Pts',(1.37079455494331,2.75013310886333,-20.9522111017968)) ;
#152897=CARTESIAN_POINT('Ctrl Pts',(1.36873453110892,2.75025430438116,-20.9511134944134)) ;
#152898=CARTESIAN_POINT('Ctrl Pts',(1.36736263966051,2.75036354665963,-20.9503818907579)) ;
#152899=CARTESIAN_POINT('Ctrl Pts',(1.36413470836879,2.75068903914081,-20.9486589310622)) ;
#152900=CARTESIAN_POINT('Ctrl Pts',(1.36227932197147,2.75092980851022,-20.947667362279)) ;
#152901=CARTESIAN_POINT('Ctrl Pts',(1.35746012444742,2.7516985967038,-20.9450888180784)) ;
#152902=CARTESIAN_POINT('Ctrl Pts',(1.35450425835489,2.7523133271765,-20.943504237459)) ;
#152903=CARTESIAN_POINT('Ctrl Pts',(1.34886973918564,2.75377034241463,-20.9404791694934)) ;
#152904=CARTESIAN_POINT('Ctrl Pts',(1.3461783156815,2.75459534478002,-20.9390321407416)) ;
#152905=CARTESIAN_POINT('Ctrl Pts',(1.34314242260183,2.75567798707048,-20.9373984698771)) ;
#152906=CARTESIAN_POINT('Ctrl Pts',(1.34256163823226,2.75588931242806,-20.937085898215)) ;
#152907=CARTESIAN_POINT('Ctrl Pts',(1.34198261999809,2.75610647364238,-20.9367742184185)) ;
#152908=CARTESIAN_POINT('Ctrl Pts',(1.3413216052292,2.75635697290857,-20.9364183780167)) ;
#152909=CARTESIAN_POINT('Ctrl Pts',(1.3408629143507,2.75653491456656,-20.9361714174681)) ;
#152910=CARTESIAN_POINT('Ctrl Pts',(1.33918548989955,2.7572007950357,-20.9352681624994)) ;
#152911=CARTESIAN_POINT('Ctrl Pts',(1.33797416370948,2.75771112313095,-20.9346156517349)) ;
#152912=CARTESIAN_POINT('Ctrl Pts',(1.33648532079705,2.75837521508443,-20.9338133670511)) ;
#152913=CARTESIAN_POINT('Ctrl Pts',(1.33619776328717,2.7585052148881,-20.9336584026979)) ;
#152914=CARTESIAN_POINT('Ctrl Pts',(1.33107968015532,2.76084915994961,-20.9308999602878)) ;
#152915=CARTESIAN_POINT('Ctrl Pts',(1.32635908659293,2.76350693339113,-20.9283519804505)) ;
#152916=CARTESIAN_POINT('Ctrl Pts',(1.32109760625854,2.76707470328536,-20.9255052830872)) ;
#152917=CARTESIAN_POINT('Ctrl Pts',(1.32035743991734,2.76759128788362,-20.9251046475546)) ;
#152918=CARTESIAN_POINT('Ctrl Pts',(1.31824805546067,2.76910584227483,-20.9239623373891)) ;
#152919=CARTESIAN_POINT('Ctrl Pts',(1.31689309423375,2.77013099976531,-20.9232277366411)) ;
#152920=CARTESIAN_POINT('Ctrl Pts',(1.31545882361433,2.7712727820175,-20.9224488780592)) ;
#152921=CARTESIAN_POINT('Ctrl Pts',(1.31535582310954,2.77135510350026,-20.9223929383465)) ;
#152922=CARTESIAN_POINT('Ctrl Pts',(1.31504853092203,2.77160168095803,-20.922226026553)) ;
#152923=CARTESIAN_POINT('Ctrl Pts',(1.31461168315421,2.7719549875475,-20.9219886931459)) ;
#152924=CARTESIAN_POINT('Ctrl Pts',(1.31417742224132,2.77231219724374,-20.9217526629429)) ;
#152925=CARTESIAN_POINT('Ctrl Pts',(1.31333096026308,2.77301480846578,-20.921292493863)) ;
#152926=CARTESIAN_POINT('Ctrl Pts',(1.31272070342849,2.77353368974775,-20.9209605431594)) ;
#152927=CARTESIAN_POINT('Ctrl Pts',(1.30969774837126,2.77616736630462,-20.9193154427618)) ;
#152928=CARTESIAN_POINT('Ctrl Pts',(1.30737022788692,2.7784005464458,-20.9180465201049)) ;
#152929=CARTESIAN_POINT('Ctrl Pts',(1.30464757270879,2.78128817542227,-20.9165612966511)) ;
#152930=CARTESIAN_POINT('Ctrl Pts',(1.30414845981076,2.78182967606623,-20.9162889873692)) ;
#152931=CARTESIAN_POINT('Ctrl Pts',(1.30260826844055,2.78353926416386,-20.9154485713631)) ;
#152932=CARTESIAN_POINT('Ctrl Pts',(1.30158324720848,2.78473373830863,-20.9148887670786)) ;
#152933=CARTESIAN_POINT('Ctrl Pts',(1.30024935135331,2.78636738852735,-20.9141601872833)) ;
#152934=CARTESIAN_POINT('Ctrl Pts',(1.29991860867236,2.78677921519269,-20.913979524919)) ;
#152935=CARTESIAN_POINT('Ctrl Pts',(1.29915346420734,2.78774794465152,-20.9135615807717)) ;
#152936=CARTESIAN_POINT('Ctrl Pts',(1.29872125904468,2.78830744810469,-20.9133255001127)) ;
#152937=CARTESIAN_POINT('Ctrl Pts',(1.29658637826222,2.79113377451588,-20.9121594679259)) ;
#152938=CARTESIAN_POINT('Ctrl Pts',(1.29496240940488,2.79348720429743,-20.9112730136302)) ;
#152939=CARTESIAN_POINT('Ctrl Pts',(1.29231665668155,2.79769679694544,-20.909828351995)) ;
#152940=CARTESIAN_POINT('Ctrl Pts',(1.2912511560106,2.79951540543442,-20.9092459513193)) ;
#152941=CARTESIAN_POINT('Ctrl Pts',(1.28927619853494,2.80313430045114,-20.9081651210187)) ;
#152942=CARTESIAN_POINT('Ctrl Pts',(1.28836241997818,2.80493500363976,-20.907664620654)) ;
#152943=CARTESIAN_POINT('Ctrl Pts',(1.28732027925583,2.80715235940912,-20.9070931587537)) ;
#152944=CARTESIAN_POINT('Ctrl Pts',(1.28695835013165,2.80793550920672,-20.9068946174353)) ;
#152945=CARTESIAN_POINT('Ctrl Pts',(1.28660568774189,2.80872522382216,-20.9067010437072)) ;
#152946=CARTESIAN_POINT('Ctrl Pts',(1.28608376699195,2.80991454434774,-20.9064145021015)) ;
#152947=CARTESIAN_POINT('Ctrl Pts',(1.285745251496,2.8107137575461,-20.9062285681094)) ;
#152948=CARTESIAN_POINT('Ctrl Pts',(1.28475894023895,2.81312894312822,-20.905686733351)) ;
#152949=CARTESIAN_POINT('Ctrl Pts',(1.28414040309303,2.81476247656142,-20.905346833702)) ;
#152950=CARTESIAN_POINT('Ctrl Pts',(1.28339818260913,2.81688756020149,-20.904939111358)) ;
#152951=CARTESIAN_POINT('Ctrl Pts',(1.28323661013043,2.81736137575528,-20.9048503628219)) ;
#152952=CARTESIAN_POINT('Ctrl Pts',(1.2826566889388,2.81910411140435,-20.9045318526463)) ;
#152953=CARTESIAN_POINT('Ctrl Pts',(1.28225920250334,2.82038205281187,-20.9043136076747)) ;
#152954=CARTESIAN_POINT('Ctrl Pts',(1.28170385606937,2.82230051526769,-20.9040086650164)) ;
#152955=CARTESIAN_POINT('Ctrl Pts',(1.28152700208473,2.82293438010912,-20.9039115582297)) ;
#152956=CARTESIAN_POINT('Ctrl Pts',(1.28107448868731,2.82461913389174,-20.9036630908507)) ;
#152957=CARTESIAN_POINT('Ctrl Pts',(1.28081016954772,2.82567198476339,-20.9035180110459)) ;
#152958=CARTESIAN_POINT('Ctrl Pts',(1.2800991035332,2.82871092361133,-20.9031278319823)) ;
#152959=CARTESIAN_POINT('Ctrl Pts',(1.27969380338793,2.83071459002993,-20.9029051291199)) ;
#152960=CARTESIAN_POINT('Ctrl Pts',(1.27923282767964,2.83340629334536,-20.9026515462665)) ;
#152961=CARTESIAN_POINT('Ctrl Pts',(1.27912420342282,2.8340808992611,-20.9025917647842)) ;
#152962=CARTESIAN_POINT('Ctrl Pts',(1.27861441353189,2.83746106027945,-20.9023110911817)) ;
#152963=CARTESIAN_POINT('Ctrl Pts',(1.27831324287571,2.84018799487017,-20.9021449017566)) ;
#152964=CARTESIAN_POINT('Ctrl Pts',(1.27795656969996,2.84527977141539,-20.9019480133439)) ;
#152965=CARTESIAN_POINT('Ctrl Pts',(1.27787304021906,2.84764286211077,-20.9019018583827)) ;
#152966=CARTESIAN_POINT('Ctrl Pts',(1.27787304021907,2.85,-20.9019018583827)) ;
#152967=CARTESIAN_POINT('',(1.27787304021905,2.85,-17.1980981416173)) ;
#152968=CARTESIAN_POINT('Origin',(-8.21365282185989E-16,2.85,-19.05)) ;
#152969=CARTESIAN_POINT('Ctrl Pts',(1.37603597336697,2.75,-17.145)) ;
#152970=CARTESIAN_POINT('Ctrl Pts',(1.37573512845497,2.75,-17.1451599709439)) ;
#152971=CARTESIAN_POINT('Ctrl Pts',(1.37543426791699,2.75000132857849,-17.1453199247894)) ;
#152972=CARTESIAN_POINT('Ctrl Pts',(1.37483257571475,2.75000665190009,-17.1456398448574)) ;
#152973=CARTESIAN_POINT('Ctrl Pts',(1.37453174406034,2.75001064672751,-17.145799811025)) ;
#152974=CARTESIAN_POINT('Ctrl Pts',(1.37388722675069,2.75002207412045,-17.1461426442071)) ;
#152975=CARTESIAN_POINT('Ctrl Pts',(1.37354350385561,2.75002991650282,-17.1463255141619)) ;
#152976=CARTESIAN_POINT('Ctrl Pts',(1.37285611423782,2.75004911307826,-17.1466912988841)) ;
#152977=CARTESIAN_POINT('Ctrl Pts',(1.37251244753524,2.75006046723047,-17.1468742136116)) ;
#152978=CARTESIAN_POINT('Ctrl Pts',(1.3714815944481,2.75009981984526,-17.147422994695)) ;
#152979=CARTESIAN_POINT('Ctrl Pts',(1.37079455494331,2.75013310886333,-17.1477888982032)) ;
#152980=CARTESIAN_POINT('Ctrl Pts',(1.36873453110892,2.75025430438115,-17.1488865055866)) ;
#152981=CARTESIAN_POINT('Ctrl Pts',(1.36736263966051,2.75036354665963,-17.1496181092421)) ;
#152982=CARTESIAN_POINT('Ctrl Pts',(1.36413470836879,2.75068903914081,-17.1513410689378)) ;
#152983=CARTESIAN_POINT('Ctrl Pts',(1.36227932197147,2.75092980851021,-17.152332637721)) ;
#152984=CARTESIAN_POINT('Ctrl Pts',(1.35746012444742,2.7516985967038,-17.1549111819216)) ;
#152985=CARTESIAN_POINT('Ctrl Pts',(1.35450425835489,2.75231332717652,-17.1564957625411)) ;
#152986=CARTESIAN_POINT('Ctrl Pts',(1.34886973918565,2.75377034241464,-17.1595208305066)) ;
#152987=CARTESIAN_POINT('Ctrl Pts',(1.3461783156815,2.75459534478002,-17.1609678592584)) ;
#152988=CARTESIAN_POINT('Ctrl Pts',(1.34314242260183,2.75567798707048,-17.1626015301229)) ;
#152989=CARTESIAN_POINT('Ctrl Pts',(1.34256163823226,2.75588931242806,-17.162914101785)) ;
#152990=CARTESIAN_POINT('Ctrl Pts',(1.34198261999809,2.75610647364238,-17.1632257815815)) ;
#152991=CARTESIAN_POINT('Ctrl Pts',(1.3413216052292,2.75635697290857,-17.1635816219833)) ;
#152992=CARTESIAN_POINT('Ctrl Pts',(1.3408629143507,2.75653491456656,-17.1638285825319)) ;
#152993=CARTESIAN_POINT('Ctrl Pts',(1.33918548989955,2.7572007950357,-17.1647318375006)) ;
#152994=CARTESIAN_POINT('Ctrl Pts',(1.33797416370948,2.75771112313095,-17.1653843482652)) ;
#152995=CARTESIAN_POINT('Ctrl Pts',(1.33648532079705,2.75837521508443,-17.1661866329489)) ;
#152996=CARTESIAN_POINT('Ctrl Pts',(1.33619776328717,2.7585052148881,-17.1663415973021)) ;
#152997=CARTESIAN_POINT('Ctrl Pts',(1.33107968015773,2.7608491599485,-17.1691000397109)) ;
#152998=CARTESIAN_POINT('Ctrl Pts',(1.32635908659765,2.76350693338849,-17.171648019547)) ;
#152999=CARTESIAN_POINT('Ctrl Pts',(1.32109760626303,2.76707470328226,-17.1744947169104)) ;
#153000=CARTESIAN_POINT('Ctrl Pts',(1.32035743991956,2.76759128788205,-17.1748953524443)) ;
#153001=CARTESIAN_POINT('Ctrl Pts',(1.31824805546067,2.76910584227484,-17.1760376626109)) ;
#153002=CARTESIAN_POINT('Ctrl Pts',(1.31689309423375,2.77013099976532,-17.1767722633589)) ;
#153003=CARTESIAN_POINT('Ctrl Pts',(1.31545882361434,2.77127278201751,-17.1775511219408)) ;
#153004=CARTESIAN_POINT('Ctrl Pts',(1.31535582310954,2.77135510350027,-17.1776070616535)) ;
#153005=CARTESIAN_POINT('Ctrl Pts',(1.31504853092204,2.77160168095804,-17.177773973447)) ;
#153006=CARTESIAN_POINT('Ctrl Pts',(1.3146116831542,2.77195498754749,-17.1780113068541)) ;
#153007=CARTESIAN_POINT('Ctrl Pts',(1.31417742224132,2.77231219724375,-17.1782473370571)) ;
#153008=CARTESIAN_POINT('Ctrl Pts',(1.31333096026309,2.77301480846578,-17.178707506137)) ;
#153009=CARTESIAN_POINT('Ctrl Pts',(1.31272070342849,2.77353368974775,-17.1790394568406)) ;
#153010=CARTESIAN_POINT('Ctrl Pts',(1.30969774837126,2.77616736630463,-17.1806845572382)) ;
#153011=CARTESIAN_POINT('Ctrl Pts',(1.30737022788692,2.7784005464458,-17.1819534798951)) ;
#153012=CARTESIAN_POINT('Ctrl Pts',(1.30464757270879,2.78128817542227,-17.1834387033489)) ;
#153013=CARTESIAN_POINT('Ctrl Pts',(1.30414845981076,2.78182967606624,-17.1837110126307)) ;
#153014=CARTESIAN_POINT('Ctrl Pts',(1.30260826844056,2.78353926416388,-17.1845514286369)) ;
#153015=CARTESIAN_POINT('Ctrl Pts',(1.30158324720849,2.78473373830866,-17.1851112329214)) ;
#153016=CARTESIAN_POINT('Ctrl Pts',(1.30024935135332,2.78636738852739,-17.1858398127168)) ;
#153017=CARTESIAN_POINT('Ctrl Pts',(1.29991860867237,2.78677921519272,-17.186020475081)) ;
#153018=CARTESIAN_POINT('Ctrl Pts',(1.29915346420734,2.78774794465155,-17.1864384192283)) ;
#153019=CARTESIAN_POINT('Ctrl Pts',(1.29872125904467,2.78830744810473,-17.1866744998873)) ;
#153020=CARTESIAN_POINT('Ctrl Pts',(1.2965863782622,2.79113377451592,-17.1878405320741)) ;
#153021=CARTESIAN_POINT('Ctrl Pts',(1.29496240940485,2.79348720429746,-17.1887269863698)) ;
#153022=CARTESIAN_POINT('Ctrl Pts',(1.29231665668153,2.79769679694546,-17.190171648005)) ;
#153023=CARTESIAN_POINT('Ctrl Pts',(1.29125115601059,2.79951540543443,-17.1907540486807)) ;
#153024=CARTESIAN_POINT('Ctrl Pts',(1.28927619853494,2.80313430045113,-17.1918348789813)) ;
#153025=CARTESIAN_POINT('Ctrl Pts',(1.28836241997818,2.80493500363976,-17.192335379346)) ;
#153026=CARTESIAN_POINT('Ctrl Pts',(1.28732027925583,2.80715235940912,-17.1929068412463)) ;
#153027=CARTESIAN_POINT('Ctrl Pts',(1.28695835013165,2.80793550920674,-17.1931053825647)) ;
#153028=CARTESIAN_POINT('Ctrl Pts',(1.28660568774189,2.80872522382217,-17.1932989562928)) ;
#153029=CARTESIAN_POINT('Ctrl Pts',(1.28608376699194,2.80991454434774,-17.1935854978985)) ;
#153030=CARTESIAN_POINT('Ctrl Pts',(1.28574525149599,2.81071375754611,-17.1937714318906)) ;
#153031=CARTESIAN_POINT('Ctrl Pts',(1.28475894023894,2.81312894312823,-17.194313266649)) ;
#153032=CARTESIAN_POINT('Ctrl Pts',(1.28414040309303,2.81476247656143,-17.194653166298)) ;
#153033=CARTESIAN_POINT('Ctrl Pts',(1.28339818260913,2.81688756020151,-17.195060888642)) ;
#153034=CARTESIAN_POINT('Ctrl Pts',(1.28323661013044,2.81736137575529,-17.1951496371781)) ;
#153035=CARTESIAN_POINT('Ctrl Pts',(1.2826566889388,2.81910411140436,-17.1954681473537)) ;
#153036=CARTESIAN_POINT('Ctrl Pts',(1.28225920250334,2.82038205281189,-17.1956863923252)) ;
#153037=CARTESIAN_POINT('Ctrl Pts',(1.28170385606938,2.8223005152677,-17.1959913349836)) ;
#153038=CARTESIAN_POINT('Ctrl Pts',(1.28152700208473,2.82293438010913,-17.1960884417703)) ;
#153039=CARTESIAN_POINT('Ctrl Pts',(1.28107448868731,2.82461913389174,-17.1963369091493)) ;
#153040=CARTESIAN_POINT('Ctrl Pts',(1.28081016954773,2.82567198476338,-17.1964819889541)) ;
#153041=CARTESIAN_POINT('Ctrl Pts',(1.2800991035332,2.82871092361133,-17.1968721680177)) ;
#153042=CARTESIAN_POINT('Ctrl Pts',(1.27969380338793,2.83071459002993,-17.1970948708801)) ;
#153043=CARTESIAN_POINT('Ctrl Pts',(1.27923282767964,2.83340629334536,-17.1973484537335)) ;
#153044=CARTESIAN_POINT('Ctrl Pts',(1.27912420342282,2.83408089926111,-17.1974082352158)) ;
#153045=CARTESIAN_POINT('Ctrl Pts',(1.27861441353188,2.83746106027946,-17.1976889088183)) ;
#153046=CARTESIAN_POINT('Ctrl Pts',(1.27831324287571,2.84018799487019,-17.1978550982434)) ;
#153047=CARTESIAN_POINT('Ctrl Pts',(1.27795656969996,2.8452797714154,-17.1980519866561)) ;
#153048=CARTESIAN_POINT('Ctrl Pts',(1.27787304021907,2.84764286211078,-17.1980981416173)) ;
#153049=CARTESIAN_POINT('Ctrl Pts',(1.27787304021907,2.85,-17.1980981416173)) ;
#153050=CARTESIAN_POINT('Origin',(1.3145125,4.45,-24.765)) ;
#153051=CARTESIAN_POINT('',(1.22107868287598,4.55,-24.6295951091213)) ;
#153052=CARTESIAN_POINT('',(1.22107868287598,4.55,-24.9004048908787)) ;
#153053=CARTESIAN_POINT('Origin',(1.3145125,4.55,-24.765)) ;
#153054=CARTESIAN_POINT('',(1.27787304021905,4.45,-24.7119018583827)) ;
#153055=CARTESIAN_POINT('Origin',(1.22107868287598,4.45,-24.6295951091213)) ;
#153056=CARTESIAN_POINT('',(1.27787304021905,4.45,-24.8180981416173)) ;
#153057=CARTESIAN_POINT('Origin',(1.3145125,4.45,-24.765)) ;
#153058=CARTESIAN_POINT('Origin',(1.22107868287598,4.45,-24.9004048908787)) ;
#153059=CARTESIAN_POINT('Origin',(-8.21365282185989E-16,2.85,-22.86)) ;
#153060=CARTESIAN_POINT('',(1.37603597336697,2.75,-24.765)) ;
#153061=CARTESIAN_POINT('Origin',(-8.13551212474381E-16,2.75,-22.86)) ;
#153062=CARTESIAN_POINT('',(1.27787304021905,2.85,-24.7119018583827)) ;
#153063=CARTESIAN_POINT('Ctrl Pts',(1.37603597336697,2.75,-24.765)) ;
#153064=CARTESIAN_POINT('Ctrl Pts',(1.37543428354307,2.75,-24.7646800581135)) ;
#153065=CARTESIAN_POINT('Ctrl Pts',(1.37483253111456,2.7500053137259,-24.7643601843412)) ;
#153066=CARTESIAN_POINT('Ctrl Pts',(1.37388722675069,2.75002207412044,-24.763857355793)) ;
#153067=CARTESIAN_POINT('Ctrl Pts',(1.37354350385561,2.75002991650282,-24.7636744858378)) ;
#153068=CARTESIAN_POINT('Ctrl Pts',(1.37285611423782,2.75004911307826,-24.7633087011159)) ;
#153069=CARTESIAN_POINT('Ctrl Pts',(1.37251244753524,2.75006046723047,-24.7631257863885)) ;
#153070=CARTESIAN_POINT('Ctrl Pts',(1.3714815944481,2.75009981984526,-24.7625770053051)) ;
#153071=CARTESIAN_POINT('Ctrl Pts',(1.37079455494331,2.75013310886333,-24.7622111017968)) ;
#153072=CARTESIAN_POINT('Ctrl Pts',(1.36873453110893,2.75025430438115,-24.7611134944134)) ;
#153073=CARTESIAN_POINT('Ctrl Pts',(1.36736263966052,2.75036354665963,-24.760381890758)) ;
#153074=CARTESIAN_POINT('Ctrl Pts',(1.36413470836879,2.75068903914081,-24.7586589310622)) ;
#153075=CARTESIAN_POINT('Ctrl Pts',(1.36227932197148,2.75092980851021,-24.757667362279)) ;
#153076=CARTESIAN_POINT('Ctrl Pts',(1.35746012444743,2.7516985967038,-24.7550888180784)) ;
#153077=CARTESIAN_POINT('Ctrl Pts',(1.35450425835489,2.75231332717649,-24.753504237459)) ;
#153078=CARTESIAN_POINT('Ctrl Pts',(1.34886973918564,2.75377034241463,-24.7504791694934)) ;
#153079=CARTESIAN_POINT('Ctrl Pts',(1.34617831568151,2.75459534478002,-24.7490321407416)) ;
#153080=CARTESIAN_POINT('Ctrl Pts',(1.34314242260183,2.75567798707047,-24.7473984698771)) ;
#153081=CARTESIAN_POINT('Ctrl Pts',(1.34256163823227,2.75588931242805,-24.747085898215)) ;
#153082=CARTESIAN_POINT('Ctrl Pts',(1.3419826199981,2.75610647364237,-24.7467742184185)) ;
#153083=CARTESIAN_POINT('Ctrl Pts',(1.3413216052292,2.75635697290856,-24.7464183780167)) ;
#153084=CARTESIAN_POINT('Ctrl Pts',(1.34086291435071,2.75653491456655,-24.7461714174681)) ;
#153085=CARTESIAN_POINT('Ctrl Pts',(1.33918548989956,2.7572007950357,-24.7452681624994)) ;
#153086=CARTESIAN_POINT('Ctrl Pts',(1.33797416370948,2.75771112313095,-24.7446156517348)) ;
#153087=CARTESIAN_POINT('Ctrl Pts',(1.33648532079705,2.75837521508443,-24.7438133670511)) ;
#153088=CARTESIAN_POINT('Ctrl Pts',(1.33619776328718,2.7585052148881,-24.7436584026979)) ;
#153089=CARTESIAN_POINT('Ctrl Pts',(1.33107968015587,2.76084915994935,-24.7408999602881)) ;
#153090=CARTESIAN_POINT('Ctrl Pts',(1.326359086594,2.76350693339053,-24.7383519804511)) ;
#153091=CARTESIAN_POINT('Ctrl Pts',(1.32109760625957,2.76707470328464,-24.7355052830878)) ;
#153092=CARTESIAN_POINT('Ctrl Pts',(1.32035743991787,2.76759128788323,-24.7351046475549)) ;
#153093=CARTESIAN_POINT('Ctrl Pts',(1.31824805546069,2.76910584227479,-24.7339623373891)) ;
#153094=CARTESIAN_POINT('Ctrl Pts',(1.31689309423376,2.77013099976528,-24.7332277366412)) ;
#153095=CARTESIAN_POINT('Ctrl Pts',(1.31545882361435,2.77127278201747,-24.7324488780593)) ;
#153096=CARTESIAN_POINT('Ctrl Pts',(1.31535582310957,2.77135510350022,-24.7323929383466)) ;
#153097=CARTESIAN_POINT('Ctrl Pts',(1.31504853092209,2.77160168095797,-24.732226026553)) ;
#153098=CARTESIAN_POINT('Ctrl Pts',(1.31461168315425,2.77195498754744,-24.7319886931459)) ;
#153099=CARTESIAN_POINT('Ctrl Pts',(1.31417742224137,2.77231219724369,-24.7317526629429)) ;
#153100=CARTESIAN_POINT('Ctrl Pts',(1.31333096026314,2.77301480846572,-24.7312924938631)) ;
#153101=CARTESIAN_POINT('Ctrl Pts',(1.31272070342855,2.77353368974769,-24.7309605431594)) ;
#153102=CARTESIAN_POINT('Ctrl Pts',(1.30969774837133,2.77616736630457,-24.7293154427618)) ;
#153103=CARTESIAN_POINT('Ctrl Pts',(1.307370227887,2.77840054644575,-24.7280465201049)) ;
#153104=CARTESIAN_POINT('Ctrl Pts',(1.30464757270885,2.78128817542223,-24.7265612966511)) ;
#153105=CARTESIAN_POINT('Ctrl Pts',(1.30414845981079,2.78182967606622,-24.7262889873693)) ;
#153106=CARTESIAN_POINT('Ctrl Pts',(1.30260826844056,2.78353926416387,-24.7254485713631)) ;
#153107=CARTESIAN_POINT('Ctrl Pts',(1.30158324720849,2.78473373830863,-24.7248887670787)) ;
#153108=CARTESIAN_POINT('Ctrl Pts',(1.30024935135333,2.78636738852735,-24.7241601872833)) ;
#153109=CARTESIAN_POINT('Ctrl Pts',(1.29991860867238,2.78677921519269,-24.723979524919)) ;
#153110=CARTESIAN_POINT('Ctrl Pts',(1.29915346420736,2.78774794465151,-24.7235615807717)) ;
#153111=CARTESIAN_POINT('Ctrl Pts',(1.2987212590447,2.78830744810469,-24.7233255001127)) ;
#153112=CARTESIAN_POINT('Ctrl Pts',(1.29658637826224,2.79113377451587,-24.7221594679259)) ;
#153113=CARTESIAN_POINT('Ctrl Pts',(1.29496240940491,2.79348720429741,-24.7212730136302)) ;
#153114=CARTESIAN_POINT('Ctrl Pts',(1.29231665668157,2.79769679694542,-24.7198283519951)) ;
#153115=CARTESIAN_POINT('Ctrl Pts',(1.29125115601062,2.79951540543441,-24.7192459513193)) ;
#153116=CARTESIAN_POINT('Ctrl Pts',(1.28927619853494,2.80313430045114,-24.7181651210187)) ;
#153117=CARTESIAN_POINT('Ctrl Pts',(1.28836241997818,2.80493500363977,-24.7176646206541)) ;
#153118=CARTESIAN_POINT('Ctrl Pts',(1.28732027925584,2.80715235940912,-24.7170931587537)) ;
#153119=CARTESIAN_POINT('Ctrl Pts',(1.28695835013164,2.80793550920674,-24.7168946174355)) ;
#153120=CARTESIAN_POINT('Ctrl Pts',(1.2866056877419,2.80872522382218,-24.7167010437072)) ;
#153121=CARTESIAN_POINT('Ctrl Pts',(1.28608376699195,2.80991454434775,-24.7164145021015)) ;
#153122=CARTESIAN_POINT('Ctrl Pts',(1.285745251496,2.81071375754612,-24.7162285681094)) ;
#153123=CARTESIAN_POINT('Ctrl Pts',(1.28475894023895,2.81312894312825,-24.715686733351)) ;
#153124=CARTESIAN_POINT('Ctrl Pts',(1.28414040309302,2.81476247656145,-24.715346833702)) ;
#153125=CARTESIAN_POINT('Ctrl Pts',(1.28339818260913,2.81688756020153,-24.714939111358)) ;
#153126=CARTESIAN_POINT('Ctrl Pts',(1.28323661013044,2.81736137575531,-24.7148503628219)) ;
#153127=CARTESIAN_POINT('Ctrl Pts',(1.2826566889388,2.81910411140439,-24.7145318526463)) ;
#153128=CARTESIAN_POINT('Ctrl Pts',(1.28225920250333,2.82038205281191,-24.7143136076748)) ;
#153129=CARTESIAN_POINT('Ctrl Pts',(1.28170385606937,2.82230051526772,-24.7140086650164)) ;
#153130=CARTESIAN_POINT('Ctrl Pts',(1.28152700208474,2.82293438010913,-24.7139115582297)) ;
#153131=CARTESIAN_POINT('Ctrl Pts',(1.28107448868732,2.82461913389174,-24.7136630908507)) ;
#153132=CARTESIAN_POINT('Ctrl Pts',(1.28081016954773,2.82567198476338,-24.7135180110459)) ;
#153133=CARTESIAN_POINT('Ctrl Pts',(1.28009910353321,2.82871092361133,-24.7131278319823)) ;
#153134=CARTESIAN_POINT('Ctrl Pts',(1.27969380338794,2.83071459002993,-24.71290512912)) ;
#153135=CARTESIAN_POINT('Ctrl Pts',(1.27923282767965,2.83340629334535,-24.7126515462666)) ;
#153136=CARTESIAN_POINT('Ctrl Pts',(1.27912420342283,2.83408089926109,-24.7125917647842)) ;
#153137=CARTESIAN_POINT('Ctrl Pts',(1.27861441353189,2.83746106027943,-24.7123110911817)) ;
#153138=CARTESIAN_POINT('Ctrl Pts',(1.27831324287572,2.84018799487015,-24.7121449017567)) ;
#153139=CARTESIAN_POINT('Ctrl Pts',(1.27795656969997,2.84527977141537,-24.7119480133439)) ;
#153140=CARTESIAN_POINT('Ctrl Pts',(1.27787304021907,2.84764286211077,-24.7119018583827)) ;
#153141=CARTESIAN_POINT('Ctrl Pts',(1.27787304021907,2.85,-24.7119018583827)) ;
#153142=CARTESIAN_POINT('',(1.27787304021905,2.85,-21.0080981416173)) ;
#153143=CARTESIAN_POINT('Origin',(-8.21365282185989E-16,2.85,-22.86)) ;
#153144=CARTESIAN_POINT('Ctrl Pts',(1.37603597336697,2.75,-20.955)) ;
#153145=CARTESIAN_POINT('Ctrl Pts',(1.37573512845497,2.75,-20.9551599709441)) ;
#153146=CARTESIAN_POINT('Ctrl Pts',(1.37543426791699,2.75000132857849,-20.9553199247806)) ;
#153147=CARTESIAN_POINT('Ctrl Pts',(1.37483257571475,2.75000665190009,-20.9556398448574)) ;
#153148=CARTESIAN_POINT('Ctrl Pts',(1.37453174406034,2.75001064672752,-20.955799811025)) ;
#153149=CARTESIAN_POINT('Ctrl Pts',(1.37388722675069,2.75002207412044,-20.9561426442071)) ;
#153150=CARTESIAN_POINT('Ctrl Pts',(1.37354350385561,2.75002991650282,-20.9563255141619)) ;
#153151=CARTESIAN_POINT('Ctrl Pts',(1.37285611423782,2.75004911307826,-20.9566912988841)) ;
#153152=CARTESIAN_POINT('Ctrl Pts',(1.37251244753524,2.75006046723047,-20.9568742136115)) ;
#153153=CARTESIAN_POINT('Ctrl Pts',(1.3714815944481,2.75009981984526,-20.957422994695)) ;
#153154=CARTESIAN_POINT('Ctrl Pts',(1.37079455494331,2.75013310886333,-20.9577888982032)) ;
#153155=CARTESIAN_POINT('Ctrl Pts',(1.36873453110892,2.75025430438116,-20.9588865055866)) ;
#153156=CARTESIAN_POINT('Ctrl Pts',(1.36736263966051,2.75036354665963,-20.9596181092421)) ;
#153157=CARTESIAN_POINT('Ctrl Pts',(1.36413470836879,2.75068903914081,-20.9613410689378)) ;
#153158=CARTESIAN_POINT('Ctrl Pts',(1.36227932197147,2.75092980851022,-20.962332637721)) ;
#153159=CARTESIAN_POINT('Ctrl Pts',(1.35746012444742,2.7516985967038,-20.9649111819216)) ;
#153160=CARTESIAN_POINT('Ctrl Pts',(1.35450425835489,2.75231332717652,-20.9664957625411)) ;
#153161=CARTESIAN_POINT('Ctrl Pts',(1.34886973918565,2.75377034241464,-20.9695208305066)) ;
#153162=CARTESIAN_POINT('Ctrl Pts',(1.3461783156815,2.75459534478003,-20.9709678592584)) ;
#153163=CARTESIAN_POINT('Ctrl Pts',(1.34314242260183,2.75567798707048,-20.9726015301229)) ;
#153164=CARTESIAN_POINT('Ctrl Pts',(1.34256163823226,2.75588931242806,-20.972914101785)) ;
#153165=CARTESIAN_POINT('Ctrl Pts',(1.34198261999809,2.75610647364238,-20.9732257815815)) ;
#153166=CARTESIAN_POINT('Ctrl Pts',(1.3413216052292,2.75635697290857,-20.9735816219833)) ;
#153167=CARTESIAN_POINT('Ctrl Pts',(1.3408629143507,2.75653491456656,-20.9738285825319)) ;
#153168=CARTESIAN_POINT('Ctrl Pts',(1.33918548989956,2.7572007950357,-20.9747318375006)) ;
#153169=CARTESIAN_POINT('Ctrl Pts',(1.33797416370948,2.75771112313096,-20.9753843482651)) ;
#153170=CARTESIAN_POINT('Ctrl Pts',(1.33648532079705,2.75837521508444,-20.9761866329489)) ;
#153171=CARTESIAN_POINT('Ctrl Pts',(1.33619776328717,2.7585052148881,-20.9763415973021)) ;
#153172=CARTESIAN_POINT('Ctrl Pts',(1.33107968015759,2.76084915994857,-20.979100039711)) ;
#153173=CARTESIAN_POINT('Ctrl Pts',(1.32635908659737,2.76350693338865,-20.9816480195471)) ;
#153174=CARTESIAN_POINT('Ctrl Pts',(1.32109760626276,2.76707470328244,-20.9844947169106)) ;
#153175=CARTESIAN_POINT('Ctrl Pts',(1.32035743991943,2.76759128788214,-20.9848953524443)) ;
#153176=CARTESIAN_POINT('Ctrl Pts',(1.31824805546067,2.76910584227485,-20.9860376626109)) ;
#153177=CARTESIAN_POINT('Ctrl Pts',(1.31689309423375,2.77013099976532,-20.9867722633589)) ;
#153178=CARTESIAN_POINT('Ctrl Pts',(1.31545882361433,2.77127278201751,-20.9875511219408)) ;
#153179=CARTESIAN_POINT('Ctrl Pts',(1.31535582310953,2.77135510350028,-20.9876070616535)) ;
#153180=CARTESIAN_POINT('Ctrl Pts',(1.31504853092203,2.77160168095805,-20.987773973447)) ;
#153181=CARTESIAN_POINT('Ctrl Pts',(1.31461168315419,2.7719549875475,-20.9880113068541)) ;
#153182=CARTESIAN_POINT('Ctrl Pts',(1.31417742224131,2.77231219724376,-20.9882473370571)) ;
#153183=CARTESIAN_POINT('Ctrl Pts',(1.31333096026308,2.77301480846579,-20.988707506137)) ;
#153184=CARTESIAN_POINT('Ctrl Pts',(1.31272070342848,2.77353368974776,-20.9890394568406)) ;
#153185=CARTESIAN_POINT('Ctrl Pts',(1.30969774837125,2.77616736630464,-20.9906845572382)) ;
#153186=CARTESIAN_POINT('Ctrl Pts',(1.30737022788691,2.77840054644581,-20.9919534798951)) ;
#153187=CARTESIAN_POINT('Ctrl Pts',(1.30464757270878,2.78128817542228,-20.9934387033489)) ;
#153188=CARTESIAN_POINT('Ctrl Pts',(1.30414845981075,2.78182967606624,-20.9937110126307)) ;
#153189=CARTESIAN_POINT('Ctrl Pts',(1.30260826844056,2.78353926416389,-20.9945514286369)) ;
#153190=CARTESIAN_POINT('Ctrl Pts',(1.30158324720848,2.78473373830866,-20.9951112329214)) ;
#153191=CARTESIAN_POINT('Ctrl Pts',(1.30024935135331,2.7863673885274,-20.9958398127168)) ;
#153192=CARTESIAN_POINT('Ctrl Pts',(1.29991860867236,2.78677921519273,-20.996020475081)) ;
#153193=CARTESIAN_POINT('Ctrl Pts',(1.29915346420733,2.78774794465156,-20.9964384192283)) ;
#153194=CARTESIAN_POINT('Ctrl Pts',(1.29872125904466,2.78830744810474,-20.9966744998873)) ;
#153195=CARTESIAN_POINT('Ctrl Pts',(1.29658637826218,2.79113377451594,-20.9978405320741)) ;
#153196=CARTESIAN_POINT('Ctrl Pts',(1.29496240940483,2.79348720429749,-20.9987269863698)) ;
#153197=CARTESIAN_POINT('Ctrl Pts',(1.29231665668151,2.79769679694549,-21.000171648005)) ;
#153198=CARTESIAN_POINT('Ctrl Pts',(1.29125115601058,2.79951540543444,-21.0007540486807)) ;
#153199=CARTESIAN_POINT('Ctrl Pts',(1.28927619853494,2.80313430045113,-21.0018348789813)) ;
#153200=CARTESIAN_POINT('Ctrl Pts',(1.28836241997818,2.80493500363975,-21.002335379346)) ;
#153201=CARTESIAN_POINT('Ctrl Pts',(1.28732027925583,2.80715235940912,-21.0029068412463)) ;
#153202=CARTESIAN_POINT('Ctrl Pts',(1.28695835013163,2.80793550920672,-21.0031053825645)) ;
#153203=CARTESIAN_POINT('Ctrl Pts',(1.28660568774189,2.80872522382217,-21.0032989562928)) ;
#153204=CARTESIAN_POINT('Ctrl Pts',(1.28608376699194,2.80991454434776,-21.0035854978985)) ;
#153205=CARTESIAN_POINT('Ctrl Pts',(1.28574525149598,2.81071375754613,-21.0037714318906)) ;
#153206=CARTESIAN_POINT('Ctrl Pts',(1.28475894023893,2.81312894312826,-21.004313266649)) ;
#153207=CARTESIAN_POINT('Ctrl Pts',(1.284140403093,2.81476247656146,-21.004653166298)) ;
#153208=CARTESIAN_POINT('Ctrl Pts',(1.2833981826091,2.81688756020155,-21.005060888642)) ;
#153209=CARTESIAN_POINT('Ctrl Pts',(1.28323661013042,2.81736137575535,-21.0051496371781)) ;
#153210=CARTESIAN_POINT('Ctrl Pts',(1.28265668893878,2.81910411140443,-21.0054681473537)) ;
#153211=CARTESIAN_POINT('Ctrl Pts',(1.28225920250331,2.82038205281195,-21.0056863923253)) ;
#153212=CARTESIAN_POINT('Ctrl Pts',(1.28170385606935,2.82230051526775,-21.0059913349836)) ;
#153213=CARTESIAN_POINT('Ctrl Pts',(1.28152700208472,2.82293438010915,-21.0060884417703)) ;
#153214=CARTESIAN_POINT('Ctrl Pts',(1.28107448868731,2.82461913389174,-21.0063369091493)) ;
#153215=CARTESIAN_POINT('Ctrl Pts',(1.28081016954772,2.82567198476338,-21.0064819889541)) ;
#153216=CARTESIAN_POINT('Ctrl Pts',(1.2800991035332,2.82871092361133,-21.0068721680177)) ;
#153217=CARTESIAN_POINT('Ctrl Pts',(1.27969380338793,2.83071459002992,-21.00709487088)) ;
#153218=CARTESIAN_POINT('Ctrl Pts',(1.27923282767964,2.83340629334535,-21.0073484537334)) ;
#153219=CARTESIAN_POINT('Ctrl Pts',(1.27912420342281,2.83408089926109,-21.0074082352158)) ;
#153220=CARTESIAN_POINT('Ctrl Pts',(1.27861441353188,2.83746106027943,-21.0076889088183)) ;
#153221=CARTESIAN_POINT('Ctrl Pts',(1.27831324287571,2.84018799487015,-21.0078550982434)) ;
#153222=CARTESIAN_POINT('Ctrl Pts',(1.27795656969996,2.84527977141538,-21.0080519866561)) ;
#153223=CARTESIAN_POINT('Ctrl Pts',(1.27787304021907,2.84764286211077,-21.0080981416173)) ;
#153224=CARTESIAN_POINT('Ctrl Pts',(1.27787304021907,2.85,-21.0080981416173)) ;
#153225=CARTESIAN_POINT('Origin',(1.3145125,4.45,-28.575)) ;
#153226=CARTESIAN_POINT('',(1.22107868287598,4.55,-28.4395951091213)) ;
#153227=CARTESIAN_POINT('',(1.22107868287598,4.55,-28.7104048908787)) ;
#153228=CARTESIAN_POINT('Origin',(1.3145125,4.55,-28.575)) ;
#153229=CARTESIAN_POINT('',(1.27787304021905,4.45,-28.5219018583827)) ;
#153230=CARTESIAN_POINT('Origin',(1.22107868287598,4.45,-28.4395951091213)) ;
#153231=CARTESIAN_POINT('',(1.27787304021905,4.45,-28.6280981416173)) ;
#153232=CARTESIAN_POINT('Origin',(1.3145125,4.45,-28.575)) ;
#153233=CARTESIAN_POINT('Origin',(1.22107868287598,4.45,-28.7104048908787)) ;
#153234=CARTESIAN_POINT('Origin',(-8.21365282185989E-16,2.85,-26.67)) ;
#153235=CARTESIAN_POINT('',(1.37603597336697,2.75,-28.575)) ;
#153236=CARTESIAN_POINT('Origin',(-8.13551212474381E-16,2.75,-26.67)) ;
#153237=CARTESIAN_POINT('',(1.27787304021905,2.85,-28.5219018583827)) ;
#153238=CARTESIAN_POINT('Ctrl Pts',(1.37603597336697,2.75,-28.575)) ;
#153239=CARTESIAN_POINT('Ctrl Pts',(1.37573512845497,2.75,-28.5748400290576)) ;
#153240=CARTESIAN_POINT('Ctrl Pts',(1.37543426791934,2.75000132857352,-28.5746800751649)) ;
#153241=CARTESIAN_POINT('Ctrl Pts',(1.37483257571476,2.75000665190009,-28.5743601551427)) ;
#153242=CARTESIAN_POINT('Ctrl Pts',(1.37453174406035,2.75001064672751,-28.5742001889751)) ;
#153243=CARTESIAN_POINT('Ctrl Pts',(1.37388722675069,2.75002207412045,-28.573857355793)) ;
#153244=CARTESIAN_POINT('Ctrl Pts',(1.37354350385561,2.75002991650282,-28.5736744858378)) ;
#153245=CARTESIAN_POINT('Ctrl Pts',(1.37285611423782,2.75004911307826,-28.5733087011159)) ;
#153246=CARTESIAN_POINT('Ctrl Pts',(1.37251244753524,2.75006046723047,-28.5731257863885)) ;
#153247=CARTESIAN_POINT('Ctrl Pts',(1.3714815944481,2.75009981984526,-28.572577005305)) ;
#153248=CARTESIAN_POINT('Ctrl Pts',(1.37079455494331,2.75013310886333,-28.5722111017968)) ;
#153249=CARTESIAN_POINT('Ctrl Pts',(1.36873453110893,2.75025430438115,-28.5711134944134)) ;
#153250=CARTESIAN_POINT('Ctrl Pts',(1.36736263966052,2.75036354665963,-28.5703818907579)) ;
#153251=CARTESIAN_POINT('Ctrl Pts',(1.36413470836879,2.75068903914081,-28.5686589310622)) ;
#153252=CARTESIAN_POINT('Ctrl Pts',(1.36227932197148,2.75092980851021,-28.567667362279)) ;
#153253=CARTESIAN_POINT('Ctrl Pts',(1.35746012444743,2.7516985967038,-28.5650888180784)) ;
#153254=CARTESIAN_POINT('Ctrl Pts',(1.35450425835489,2.75231332717651,-28.5635042374589)) ;
#153255=CARTESIAN_POINT('Ctrl Pts',(1.34886973918565,2.75377034241464,-28.5604791694934)) ;
#153256=CARTESIAN_POINT('Ctrl Pts',(1.34617831568151,2.75459534478003,-28.5590321407416)) ;
#153257=CARTESIAN_POINT('Ctrl Pts',(1.34314242260183,2.75567798707048,-28.5573984698771)) ;
#153258=CARTESIAN_POINT('Ctrl Pts',(1.34256163823226,2.75588931242806,-28.557085898215)) ;
#153259=CARTESIAN_POINT('Ctrl Pts',(1.34198261999809,2.75610647364238,-28.5567742184185)) ;
#153260=CARTESIAN_POINT('Ctrl Pts',(1.3413216052292,2.75635697290856,-28.5564183780167)) ;
#153261=CARTESIAN_POINT('Ctrl Pts',(1.3408629143507,2.75653491456656,-28.5561714174681)) ;
#153262=CARTESIAN_POINT('Ctrl Pts',(1.33918548989956,2.7572007950357,-28.5552681624994)) ;
#153263=CARTESIAN_POINT('Ctrl Pts',(1.33797416370948,2.75771112313095,-28.5546156517349)) ;
#153264=CARTESIAN_POINT('Ctrl Pts',(1.33648532079705,2.75837521508443,-28.5538133670511)) ;
#153265=CARTESIAN_POINT('Ctrl Pts',(1.33619776328718,2.7585052148881,-28.5536584026979)) ;
#153266=CARTESIAN_POINT('Ctrl Pts',(1.33107968015599,2.7608491599493,-28.5508999602882)) ;
#153267=CARTESIAN_POINT('Ctrl Pts',(1.32635908659425,2.76350693339039,-28.5483519804512)) ;
#153268=CARTESIAN_POINT('Ctrl Pts',(1.32109760625981,2.76707470328447,-28.5455052830879)) ;
#153269=CARTESIAN_POINT('Ctrl Pts',(1.32035743991799,2.76759128788314,-28.545104647555)) ;
#153270=CARTESIAN_POINT('Ctrl Pts',(1.3182480554607,2.76910584227479,-28.5439623373891)) ;
#153271=CARTESIAN_POINT('Ctrl Pts',(1.31689309423377,2.77013099976528,-28.5432277366412)) ;
#153272=CARTESIAN_POINT('Ctrl Pts',(1.31545882361435,2.77127278201747,-28.5424488780593)) ;
#153273=CARTESIAN_POINT('Ctrl Pts',(1.31535582310958,2.77135510350021,-28.5423929383466)) ;
#153274=CARTESIAN_POINT('Ctrl Pts',(1.31504853092211,2.77160168095796,-28.542226026553)) ;
#153275=CARTESIAN_POINT('Ctrl Pts',(1.31461168315429,2.77195498754743,-28.5419886931459)) ;
#153276=CARTESIAN_POINT('Ctrl Pts',(1.31417742224139,2.77231219724367,-28.5417526629429)) ;
#153277=CARTESIAN_POINT('Ctrl Pts',(1.31333096026317,2.77301480846571,-28.5412924938631)) ;
#153278=CARTESIAN_POINT('Ctrl Pts',(1.31272070342857,2.77353368974768,-28.5409605431594)) ;
#153279=CARTESIAN_POINT('Ctrl Pts',(1.30969774837136,2.77616736630455,-28.5393154427618)) ;
#153280=CARTESIAN_POINT('Ctrl Pts',(1.30737022788703,2.77840054644572,-28.5380465201049)) ;
#153281=CARTESIAN_POINT('Ctrl Pts',(1.30464757270886,2.78128817542221,-28.5365612966511)) ;
#153282=CARTESIAN_POINT('Ctrl Pts',(1.3041484598108,2.78182967606621,-28.5362889873693)) ;
#153283=CARTESIAN_POINT('Ctrl Pts',(1.30260826844056,2.78353926416386,-28.5354485713631)) ;
#153284=CARTESIAN_POINT('Ctrl Pts',(1.30158324720849,2.78473373830863,-28.5348887670786)) ;
#153285=CARTESIAN_POINT('Ctrl Pts',(1.30024935135332,2.78636738852735,-28.5341601872833)) ;
#153286=CARTESIAN_POINT('Ctrl Pts',(1.29991860867238,2.78677921519269,-28.533979524919)) ;
#153287=CARTESIAN_POINT('Ctrl Pts',(1.29915346420735,2.78774794465151,-28.5335615807717)) ;
#153288=CARTESIAN_POINT('Ctrl Pts',(1.29872125904469,2.78830744810468,-28.5333255001127)) ;
#153289=CARTESIAN_POINT('Ctrl Pts',(1.29658637826223,2.79113377451586,-28.5321594679259)) ;
#153290=CARTESIAN_POINT('Ctrl Pts',(1.29496240940489,2.79348720429741,-28.5312730136302)) ;
#153291=CARTESIAN_POINT('Ctrl Pts',(1.29231665668156,2.79769679694542,-28.5298283519951)) ;
#153292=CARTESIAN_POINT('Ctrl Pts',(1.2912511560106,2.79951540543441,-28.5292459513193)) ;
#153293=CARTESIAN_POINT('Ctrl Pts',(1.28927619853494,2.80313430045114,-28.5281651210187)) ;
#153294=CARTESIAN_POINT('Ctrl Pts',(1.28836241997818,2.80493500363976,-28.527664620654)) ;
#153295=CARTESIAN_POINT('Ctrl Pts',(1.28732027925583,2.80715235940912,-28.5270931587537)) ;
#153296=CARTESIAN_POINT('Ctrl Pts',(1.28695835013163,2.80793550920674,-28.5268946174353)) ;
#153297=CARTESIAN_POINT('Ctrl Pts',(1.28660568774188,2.80872522382217,-28.5267010437072)) ;
#153298=CARTESIAN_POINT('Ctrl Pts',(1.28608376699193,2.80991454434775,-28.5264145021015)) ;
#153299=CARTESIAN_POINT('Ctrl Pts',(1.28574525149598,2.81071375754612,-28.5262285681094)) ;
#153300=CARTESIAN_POINT('Ctrl Pts',(1.28475894023892,2.81312894312826,-28.525686733351)) ;
#153301=CARTESIAN_POINT('Ctrl Pts',(1.284140403093,2.81476247656147,-28.525346833702)) ;
#153302=CARTESIAN_POINT('Ctrl Pts',(1.2833981826091,2.81688756020156,-28.524939111358)) ;
#153303=CARTESIAN_POINT('Ctrl Pts',(1.28323661013041,2.81736137575535,-28.5248503628219)) ;
#153304=CARTESIAN_POINT('Ctrl Pts',(1.28265668893878,2.81910411140443,-28.5245318526463)) ;
#153305=CARTESIAN_POINT('Ctrl Pts',(1.2822592025033,2.82038205281196,-28.5243136076747)) ;
#153306=CARTESIAN_POINT('Ctrl Pts',(1.28170385606935,2.82230051526775,-28.5240086650164)) ;
#153307=CARTESIAN_POINT('Ctrl Pts',(1.28152700208472,2.82293438010915,-28.5239115582297)) ;
#153308=CARTESIAN_POINT('Ctrl Pts',(1.2810744886873,2.82461913389174,-28.5236630908507)) ;
#153309=CARTESIAN_POINT('Ctrl Pts',(1.28081016954772,2.82567198476338,-28.5235180110459)) ;
#153310=CARTESIAN_POINT('Ctrl Pts',(1.2800991035332,2.82871092361133,-28.5231278319823)) ;
#153311=CARTESIAN_POINT('Ctrl Pts',(1.27969380338793,2.83071459002993,-28.52290512912)) ;
#153312=CARTESIAN_POINT('Ctrl Pts',(1.27923282767963,2.83340629334536,-28.5226515462665)) ;
#153313=CARTESIAN_POINT('Ctrl Pts',(1.27912420342281,2.8340808992611,-28.5225917647842)) ;
#153314=CARTESIAN_POINT('Ctrl Pts',(1.27861441353188,2.83746106027946,-28.5223110911817)) ;
#153315=CARTESIAN_POINT('Ctrl Pts',(1.2783132428757,2.84018799487019,-28.5221449017566)) ;
#153316=CARTESIAN_POINT('Ctrl Pts',(1.27795656969995,2.8452797714154,-28.5219480133439)) ;
#153317=CARTESIAN_POINT('Ctrl Pts',(1.27787304021906,2.84764286211078,-28.5219018583827)) ;
#153318=CARTESIAN_POINT('Ctrl Pts',(1.27787304021907,2.85,-28.5219018583827)) ;
#153319=CARTESIAN_POINT('',(1.27787304021905,2.85,-24.8180981416173)) ;
#153320=CARTESIAN_POINT('Origin',(-8.21365282185989E-16,2.85,-26.67)) ;
#153321=CARTESIAN_POINT('Ctrl Pts',(1.37603597336697,2.75,-24.765)) ;
#153322=CARTESIAN_POINT('Ctrl Pts',(1.37573512845502,2.75,-24.7651599709433)) ;
#153323=CARTESIAN_POINT('Ctrl Pts',(1.37513340736836,2.75000265707422,-24.7654798786905)) ;
#153324=CARTESIAN_POINT('Ctrl Pts',(1.37453174406034,2.75001064672752,-24.7657998110249)) ;
#153325=CARTESIAN_POINT('Ctrl Pts',(1.37388722675069,2.75002207412044,-24.766142644207)) ;
#153326=CARTESIAN_POINT('Ctrl Pts',(1.37354350385561,2.75002991650282,-24.7663255141622)) ;
#153327=CARTESIAN_POINT('Ctrl Pts',(1.37285611423782,2.75004911307826,-24.7666912988841)) ;
#153328=CARTESIAN_POINT('Ctrl Pts',(1.37251244753524,2.75006046723047,-24.7668742136115)) ;
#153329=CARTESIAN_POINT('Ctrl Pts',(1.3714815944481,2.75009981984526,-24.767422994695)) ;
#153330=CARTESIAN_POINT('Ctrl Pts',(1.37079455494331,2.75013310886333,-24.7677888982032)) ;
#153331=CARTESIAN_POINT('Ctrl Pts',(1.36873453110893,2.75025430438116,-24.7688865055866)) ;
#153332=CARTESIAN_POINT('Ctrl Pts',(1.36736263966052,2.75036354665963,-24.7696181092421)) ;
#153333=CARTESIAN_POINT('Ctrl Pts',(1.36413470836879,2.75068903914081,-24.7713410689378)) ;
#153334=CARTESIAN_POINT('Ctrl Pts',(1.36227932197148,2.75092980851021,-24.772332637721)) ;
#153335=CARTESIAN_POINT('Ctrl Pts',(1.35746012444743,2.7516985967038,-24.7749111819216)) ;
#153336=CARTESIAN_POINT('Ctrl Pts',(1.35450425835489,2.75231332717651,-24.7764957625411)) ;
#153337=CARTESIAN_POINT('Ctrl Pts',(1.34886973918564,2.75377034241463,-24.7795208305066)) ;
#153338=CARTESIAN_POINT('Ctrl Pts',(1.3461783156815,2.75459534478002,-24.7809678592584)) ;
#153339=CARTESIAN_POINT('Ctrl Pts',(1.34314242260182,2.75567798707047,-24.7826015301229)) ;
#153340=CARTESIAN_POINT('Ctrl Pts',(1.34256163823226,2.75588931242805,-24.782914101785)) ;
#153341=CARTESIAN_POINT('Ctrl Pts',(1.34198261999809,2.75610647364237,-24.7832257815815)) ;
#153342=CARTESIAN_POINT('Ctrl Pts',(1.3413216052292,2.75635697290856,-24.7835816219833)) ;
#153343=CARTESIAN_POINT('Ctrl Pts',(1.3408629143507,2.75653491456655,-24.7838285825319)) ;
#153344=CARTESIAN_POINT('Ctrl Pts',(1.33918548989955,2.75720079503569,-24.7847318375006)) ;
#153345=CARTESIAN_POINT('Ctrl Pts',(1.33797416370948,2.75771112313095,-24.7853843482652)) ;
#153346=CARTESIAN_POINT('Ctrl Pts',(1.33648532079705,2.75837521508443,-24.7861866329489)) ;
#153347=CARTESIAN_POINT('Ctrl Pts',(1.33619776328718,2.75850521488809,-24.7863415973021)) ;
#153348=CARTESIAN_POINT('Ctrl Pts',(1.33107968015567,2.76084915994944,-24.789100039712)) ;
#153349=CARTESIAN_POINT('Ctrl Pts',(1.32635908659363,2.76350693339074,-24.7916480195491)) ;
#153350=CARTESIAN_POINT('Ctrl Pts',(1.32109760625924,2.76707470328487,-24.7944947169124)) ;
#153351=CARTESIAN_POINT('Ctrl Pts',(1.32035743991773,2.76759128788333,-24.7948953524452)) ;
#153352=CARTESIAN_POINT('Ctrl Pts',(1.31824805546073,2.76910584227477,-24.7960376626109)) ;
#153353=CARTESIAN_POINT('Ctrl Pts',(1.31689309423378,2.77013099976526,-24.7967722633588)) ;
#153354=CARTESIAN_POINT('Ctrl Pts',(1.31545882361437,2.77127278201745,-24.7975511219407)) ;
#153355=CARTESIAN_POINT('Ctrl Pts',(1.31535582310962,2.77135510350017,-24.7976070616534)) ;
#153356=CARTESIAN_POINT('Ctrl Pts',(1.31504853092216,2.77160168095791,-24.7977739734469)) ;
#153357=CARTESIAN_POINT('Ctrl Pts',(1.31461168315434,2.77195498754736,-24.7980113068543)) ;
#153358=CARTESIAN_POINT('Ctrl Pts',(1.31417742224145,2.77231219724361,-24.798247337057)) ;
#153359=CARTESIAN_POINT('Ctrl Pts',(1.31333096026322,2.77301480846564,-24.7987075061369)) ;
#153360=CARTESIAN_POINT('Ctrl Pts',(1.31272070342863,2.77353368974761,-24.7990394568406)) ;
#153361=CARTESIAN_POINT('Ctrl Pts',(1.30969774837141,2.77616736630447,-24.8006845572381)) ;
#153362=CARTESIAN_POINT('Ctrl Pts',(1.30737022788708,2.77840054644563,-24.801953479895)) ;
#153363=CARTESIAN_POINT('Ctrl Pts',(1.30464757270891,2.78128817542216,-24.8034387033489)) ;
#153364=CARTESIAN_POINT('Ctrl Pts',(1.30414845981082,2.78182967606617,-24.8037110126308)) ;
#153365=CARTESIAN_POINT('Ctrl Pts',(1.30260826844055,2.78353926416387,-24.804551428637)) ;
#153366=CARTESIAN_POINT('Ctrl Pts',(1.30158324720848,2.78473373830866,-24.8051112329214)) ;
#153367=CARTESIAN_POINT('Ctrl Pts',(1.3002493513533,2.78636738852739,-24.8058398127168)) ;
#153368=CARTESIAN_POINT('Ctrl Pts',(1.29991860867235,2.78677921519272,-24.8060204750811)) ;
#153369=CARTESIAN_POINT('Ctrl Pts',(1.29915346420732,2.78774794465155,-24.8064384192283)) ;
#153370=CARTESIAN_POINT('Ctrl Pts',(1.29872125904465,2.78830744810474,-24.8066744998873)) ;
#153371=CARTESIAN_POINT('Ctrl Pts',(1.29658637826217,2.79113377451593,-24.8078405320741)) ;
#153372=CARTESIAN_POINT('Ctrl Pts',(1.29496240940481,2.79348720429748,-24.8087269863698)) ;
#153373=CARTESIAN_POINT('Ctrl Pts',(1.2923166566815,2.79769679694548,-24.810171648005)) ;
#153374=CARTESIAN_POINT('Ctrl Pts',(1.29125115601058,2.79951540543444,-24.8107540486807)) ;
#153375=CARTESIAN_POINT('Ctrl Pts',(1.28927619853494,2.80313430045114,-24.8118348789813)) ;
#153376=CARTESIAN_POINT('Ctrl Pts',(1.28836241997819,2.80493500363977,-24.8123353793459)) ;
#153377=CARTESIAN_POINT('Ctrl Pts',(1.28732027925585,2.80715235940913,-24.8129068412463)) ;
#153378=CARTESIAN_POINT('Ctrl Pts',(1.28695835013167,2.80793550920673,-24.8131053825645)) ;
#153379=CARTESIAN_POINT('Ctrl Pts',(1.28660568774192,2.80872522382217,-24.8132989562928)) ;
#153380=CARTESIAN_POINT('Ctrl Pts',(1.28608376699197,2.80991454434774,-24.8135854978985)) ;
#153381=CARTESIAN_POINT('Ctrl Pts',(1.28574525149603,2.8107137575461,-24.8137714318906)) ;
#153382=CARTESIAN_POINT('Ctrl Pts',(1.28475894023898,2.81312894312821,-24.814313266649)) ;
#153383=CARTESIAN_POINT('Ctrl Pts',(1.28414040309306,2.81476247656139,-24.8146531662979)) ;
#153384=CARTESIAN_POINT('Ctrl Pts',(1.28339818260916,2.81688756020145,-24.815060888642)) ;
#153385=CARTESIAN_POINT('Ctrl Pts',(1.28323661013047,2.81736137575524,-24.815149637178)) ;
#153386=CARTESIAN_POINT('Ctrl Pts',(1.28265668893884,2.81910411140429,-24.8154681473537)) ;
#153387=CARTESIAN_POINT('Ctrl Pts',(1.28225920250336,2.8203820528118,-24.8156863923252)) ;
#153388=CARTESIAN_POINT('Ctrl Pts',(1.28170385606938,2.82230051526763,-24.8159913349835)) ;
#153389=CARTESIAN_POINT('Ctrl Pts',(1.28152700208473,2.82293438010909,-24.8160884417702)) ;
#153390=CARTESIAN_POINT('Ctrl Pts',(1.28107448868731,2.82461913389175,-24.8163369091493)) ;
#153391=CARTESIAN_POINT('Ctrl Pts',(1.28081016954774,2.8256719847634,-24.8164819889541)) ;
#153392=CARTESIAN_POINT('Ctrl Pts',(1.28009910353322,2.82871092361135,-24.8168721680177)) ;
#153393=CARTESIAN_POINT('Ctrl Pts',(1.27969380338795,2.83071459002995,-24.81709487088)) ;
#153394=CARTESIAN_POINT('Ctrl Pts',(1.27923282767965,2.83340629334538,-24.8173484537334)) ;
#153395=CARTESIAN_POINT('Ctrl Pts',(1.27912420342283,2.83408089926112,-24.8174082352158)) ;
#153396=CARTESIAN_POINT('Ctrl Pts',(1.27861441353189,2.83746106027947,-24.8176889088183)) ;
#153397=CARTESIAN_POINT('Ctrl Pts',(1.27831324287571,2.8401879948702,-24.8178550982434)) ;
#153398=CARTESIAN_POINT('Ctrl Pts',(1.27795656969995,2.84527977141541,-24.8180519866561)) ;
#153399=CARTESIAN_POINT('Ctrl Pts',(1.27787304021905,2.84764286211078,-24.8180981416173)) ;
#153400=CARTESIAN_POINT('Ctrl Pts',(1.27787304021904,2.85,-24.8180981416173)) ;
#153401=CARTESIAN_POINT('Origin',(1.31451250000001,4.45,-32.385)) ;
#153402=CARTESIAN_POINT('',(1.22107868287598,4.55,-32.2495951091213)) ;
#153403=CARTESIAN_POINT('',(1.22107868287599,4.55,-32.5204048908788)) ;
#153404=CARTESIAN_POINT('Origin',(1.31451250000001,4.55,-32.385)) ;
#153405=CARTESIAN_POINT('',(1.27787304021906,4.45,-32.3319018583827)) ;
#153406=CARTESIAN_POINT('Origin',(1.22107868287598,4.45,-32.2495951091213)) ;
#153407=CARTESIAN_POINT('',(1.27787304021906,4.45,-32.4380981416173)) ;
#153408=CARTESIAN_POINT('Origin',(1.31451250000001,4.45,-32.385)) ;
#153409=CARTESIAN_POINT('Origin',(1.22107868287599,4.45,-32.5204048908788)) ;
#153410=CARTESIAN_POINT('Origin',(-3.7454256867681E-16,2.85,-30.48)) ;
#153411=CARTESIAN_POINT('',(1.37603597336698,2.75,-32.385)) ;
#153412=CARTESIAN_POINT('Origin',(-3.66728498965203E-16,2.75,-30.48)) ;
#153413=CARTESIAN_POINT('',(1.27787304021906,2.85,-32.3319018583827)) ;
#153414=CARTESIAN_POINT('Ctrl Pts',(1.37603597336698,2.75,-32.385)) ;
#153415=CARTESIAN_POINT('Ctrl Pts',(1.37573512845502,2.75,-32.3848400290568)) ;
#153416=CARTESIAN_POINT('Ctrl Pts',(1.37513340736834,2.75000265707422,-32.3845201213094)) ;
#153417=CARTESIAN_POINT('Ctrl Pts',(1.37453174406034,2.75001064672751,-32.3842001889751)) ;
#153418=CARTESIAN_POINT('Ctrl Pts',(1.37388722675068,2.75002207412045,-32.383857355793)) ;
#153419=CARTESIAN_POINT('Ctrl Pts',(1.3735435038556,2.75002991650282,-32.3836744858382)) ;
#153420=CARTESIAN_POINT('Ctrl Pts',(1.37285611423781,2.75004911307826,-32.3833087011159)) ;
#153421=CARTESIAN_POINT('Ctrl Pts',(1.37251244753524,2.75006046723047,-32.3831257863885)) ;
#153422=CARTESIAN_POINT('Ctrl Pts',(1.3714815944481,2.75009981984526,-32.382577005305)) ;
#153423=CARTESIAN_POINT('Ctrl Pts',(1.37079455494331,2.75013310886333,-32.3822111017968)) ;
#153424=CARTESIAN_POINT('Ctrl Pts',(1.36873453110892,2.75025430438116,-32.3811134944134)) ;
#153425=CARTESIAN_POINT('Ctrl Pts',(1.36736263966051,2.75036354665963,-32.380381890758)) ;
#153426=CARTESIAN_POINT('Ctrl Pts',(1.36413470836879,2.75068903914081,-32.3786589310622)) ;
#153427=CARTESIAN_POINT('Ctrl Pts',(1.36227932197147,2.75092980851022,-32.377667362279)) ;
#153428=CARTESIAN_POINT('Ctrl Pts',(1.35746012444743,2.75169859670379,-32.3750888180785)) ;
#153429=CARTESIAN_POINT('Ctrl Pts',(1.35450425835489,2.75231332717652,-32.3735042374589)) ;
#153430=CARTESIAN_POINT('Ctrl Pts',(1.34886973918565,2.75377034241464,-32.3704791694934)) ;
#153431=CARTESIAN_POINT('Ctrl Pts',(1.34617831568151,2.75459534478003,-32.3690321407416)) ;
#153432=CARTESIAN_POINT('Ctrl Pts',(1.34314242260183,2.75567798707049,-32.3673984698771)) ;
#153433=CARTESIAN_POINT('Ctrl Pts',(1.34256163823227,2.75588931242806,-32.367085898215)) ;
#153434=CARTESIAN_POINT('Ctrl Pts',(1.3419826199981,2.75610647364238,-32.3667742184185)) ;
#153435=CARTESIAN_POINT('Ctrl Pts',(1.34132160522921,2.75635697290857,-32.3664183780167)) ;
#153436=CARTESIAN_POINT('Ctrl Pts',(1.34086291435071,2.75653491456656,-32.3661714174681)) ;
#153437=CARTESIAN_POINT('Ctrl Pts',(1.33918548989957,2.7572007950357,-32.3652681624994)) ;
#153438=CARTESIAN_POINT('Ctrl Pts',(1.33797416370949,2.75771112313095,-32.3646156517349)) ;
#153439=CARTESIAN_POINT('Ctrl Pts',(1.33648532079706,2.75837521508443,-32.3638133670511)) ;
#153440=CARTESIAN_POINT('Ctrl Pts',(1.33619776328718,2.7585052148881,-32.3636584026979)) ;
#153441=CARTESIAN_POINT('Ctrl Pts',(1.33107968015827,2.76084915994826,-32.3608999602894)) ;
#153442=CARTESIAN_POINT('Ctrl Pts',(1.3263590865987,2.76350693338791,-32.3583519804536)) ;
#153443=CARTESIAN_POINT('Ctrl Pts',(1.32109760626403,2.76707470328156,-32.3555052830901)) ;
#153444=CARTESIAN_POINT('Ctrl Pts',(1.32035743992007,2.76759128788168,-32.355104647556)) ;
#153445=CARTESIAN_POINT('Ctrl Pts',(1.31824805546069,2.76910584227482,-32.3539623373891)) ;
#153446=CARTESIAN_POINT('Ctrl Pts',(1.31689309423376,2.7701309997653,-32.3532277366412)) ;
#153447=CARTESIAN_POINT('Ctrl Pts',(1.31545882361434,2.77127278201748,-32.3524488780593)) ;
#153448=CARTESIAN_POINT('Ctrl Pts',(1.31535582310956,2.77135510350024,-32.3523929383466)) ;
#153449=CARTESIAN_POINT('Ctrl Pts',(1.31504853092207,2.771601680958,-32.352226026553)) ;
#153450=CARTESIAN_POINT('Ctrl Pts',(1.31461168315425,2.77195498754747,-32.3519886931459)) ;
#153451=CARTESIAN_POINT('Ctrl Pts',(1.31417742224135,2.77231219724371,-32.3517526629429)) ;
#153452=CARTESIAN_POINT('Ctrl Pts',(1.31333096026312,2.77301480846575,-32.351292493863)) ;
#153453=CARTESIAN_POINT('Ctrl Pts',(1.31272070342853,2.77353368974772,-32.3509605431594)) ;
#153454=CARTESIAN_POINT('Ctrl Pts',(1.30969774837131,2.7761673663046,-32.3493154427618)) ;
#153455=CARTESIAN_POINT('Ctrl Pts',(1.30737022788697,2.77840054644578,-32.3480465201049)) ;
#153456=CARTESIAN_POINT('Ctrl Pts',(1.30464757270883,2.78128817542226,-32.3465612966511)) ;
#153457=CARTESIAN_POINT('Ctrl Pts',(1.30414845981079,2.78182967606624,-32.3462889873692)) ;
#153458=CARTESIAN_POINT('Ctrl Pts',(1.30260826844057,2.78353926416389,-32.3454485713631)) ;
#153459=CARTESIAN_POINT('Ctrl Pts',(1.3015832472085,2.78473373830867,-32.3448887670786)) ;
#153460=CARTESIAN_POINT('Ctrl Pts',(1.30024935135333,2.78636738852739,-32.3441601872832)) ;
#153461=CARTESIAN_POINT('Ctrl Pts',(1.29991860867238,2.78677921519273,-32.343979524919)) ;
#153462=CARTESIAN_POINT('Ctrl Pts',(1.29915346420735,2.78774794465156,-32.3435615807717)) ;
#153463=CARTESIAN_POINT('Ctrl Pts',(1.29872125904468,2.78830744810473,-32.3433255001127)) ;
#153464=CARTESIAN_POINT('Ctrl Pts',(1.29658637826221,2.79113377451592,-32.3421594679259)) ;
#153465=CARTESIAN_POINT('Ctrl Pts',(1.29496240940486,2.79348720429747,-32.3412730136302)) ;
#153466=CARTESIAN_POINT('Ctrl Pts',(1.29231665668154,2.79769679694547,-32.339828351995)) ;
#153467=CARTESIAN_POINT('Ctrl Pts',(1.2912511560106,2.79951540543444,-32.3392459513193)) ;
#153468=CARTESIAN_POINT('Ctrl Pts',(1.28927619853495,2.80313430045114,-32.3381651210187)) ;
#153469=CARTESIAN_POINT('Ctrl Pts',(1.28836241997819,2.80493500363976,-32.337664620654)) ;
#153470=CARTESIAN_POINT('Ctrl Pts',(1.28732027925585,2.80715235940912,-32.3370931587537)) ;
#153471=CARTESIAN_POINT('Ctrl Pts',(1.28695835013165,2.80793550920672,-32.3368946174355)) ;
#153472=CARTESIAN_POINT('Ctrl Pts',(1.2866056877419,2.80872522382217,-32.3367010437072)) ;
#153473=CARTESIAN_POINT('Ctrl Pts',(1.28608376699195,2.80991454434775,-32.3364145021015)) ;
#153474=CARTESIAN_POINT('Ctrl Pts',(1.28574525149599,2.81071375754612,-32.3362285681094)) ;
#153475=CARTESIAN_POINT('Ctrl Pts',(1.28475894023894,2.81312894312826,-32.335686733351)) ;
#153476=CARTESIAN_POINT('Ctrl Pts',(1.28414040309302,2.81476247656146,-32.335346833702)) ;
#153477=CARTESIAN_POINT('Ctrl Pts',(1.28339818260913,2.81688756020155,-32.334939111358)) ;
#153478=CARTESIAN_POINT('Ctrl Pts',(1.28323661013043,2.81736137575533,-32.3348503628219)) ;
#153479=CARTESIAN_POINT('Ctrl Pts',(1.2826566889388,2.81910411140441,-32.3345318526463)) ;
#153480=CARTESIAN_POINT('Ctrl Pts',(1.28225920250332,2.82038205281194,-32.3343136076747)) ;
#153481=CARTESIAN_POINT('Ctrl Pts',(1.28170385606937,2.82230051526773,-32.3340086650164)) ;
#153482=CARTESIAN_POINT('Ctrl Pts',(1.28152700208473,2.82293438010914,-32.3339115582297)) ;
#153483=CARTESIAN_POINT('Ctrl Pts',(1.28107448868731,2.82461913389174,-32.3336630908507)) ;
#153484=CARTESIAN_POINT('Ctrl Pts',(1.28081016954773,2.82567198476338,-32.3335180110459)) ;
#153485=CARTESIAN_POINT('Ctrl Pts',(1.28009910353321,2.82871092361133,-32.3331278319823)) ;
#153486=CARTESIAN_POINT('Ctrl Pts',(1.27969380338794,2.83071459002993,-32.33290512912)) ;
#153487=CARTESIAN_POINT('Ctrl Pts',(1.27923282767964,2.83340629334536,-32.3326515462665)) ;
#153488=CARTESIAN_POINT('Ctrl Pts',(1.27912420342282,2.83408089926111,-32.3325917647842)) ;
#153489=CARTESIAN_POINT('Ctrl Pts',(1.27861441353189,2.83746106027946,-32.3323110911817)) ;
#153490=CARTESIAN_POINT('Ctrl Pts',(1.27831324287571,2.84018799487018,-32.3321449017566)) ;
#153491=CARTESIAN_POINT('Ctrl Pts',(1.27795656969997,2.8452797714154,-32.3319480133439)) ;
#153492=CARTESIAN_POINT('Ctrl Pts',(1.27787304021907,2.84764286211078,-32.3319018583827)) ;
#153493=CARTESIAN_POINT('Ctrl Pts',(1.27787304021907,2.85,-32.3319018583827)) ;
#153494=CARTESIAN_POINT('',(1.27787304021905,2.85,-28.6280981416173)) ;
#153495=CARTESIAN_POINT('Origin',(-3.7454256867681E-16,2.85,-30.48)) ;
#153496=CARTESIAN_POINT('Ctrl Pts',(1.37603597336697,2.75,-28.575)) ;
#153497=CARTESIAN_POINT('Ctrl Pts',(1.37543428354306,2.75,-28.5753199418865)) ;
#153498=CARTESIAN_POINT('Ctrl Pts',(1.37483253111456,2.7500053137259,-28.5756398156588)) ;
#153499=CARTESIAN_POINT('Ctrl Pts',(1.37388722675069,2.75002207412044,-28.576142644207)) ;
#153500=CARTESIAN_POINT('Ctrl Pts',(1.37354350385561,2.75002991650282,-28.5763255141622)) ;
#153501=CARTESIAN_POINT('Ctrl Pts',(1.37285611423782,2.75004911307826,-28.5766912988841)) ;
#153502=CARTESIAN_POINT('Ctrl Pts',(1.37251244753524,2.75006046723047,-28.5768742136115)) ;
#153503=CARTESIAN_POINT('Ctrl Pts',(1.3714815944481,2.75009981984526,-28.577422994695)) ;
#153504=CARTESIAN_POINT('Ctrl Pts',(1.37079455494331,2.75013310886333,-28.5777888982032)) ;
#153505=CARTESIAN_POINT('Ctrl Pts',(1.36873453110892,2.75025430438116,-28.5788865055866)) ;
#153506=CARTESIAN_POINT('Ctrl Pts',(1.36736263966051,2.75036354665963,-28.5796181092421)) ;
#153507=CARTESIAN_POINT('Ctrl Pts',(1.36413470836879,2.75068903914081,-28.5813410689378)) ;
#153508=CARTESIAN_POINT('Ctrl Pts',(1.36227932197147,2.75092980851022,-28.582332637721)) ;
#153509=CARTESIAN_POINT('Ctrl Pts',(1.35746012444742,2.75169859670381,-28.5849111819216)) ;
#153510=CARTESIAN_POINT('Ctrl Pts',(1.35450425835489,2.75231332717652,-28.5864957625411)) ;
#153511=CARTESIAN_POINT('Ctrl Pts',(1.34886973918565,2.75377034241464,-28.5895208305066)) ;
#153512=CARTESIAN_POINT('Ctrl Pts',(1.3461783156815,2.75459534478003,-28.5909678592584)) ;
#153513=CARTESIAN_POINT('Ctrl Pts',(1.34314242260182,2.75567798707048,-28.5926015301229)) ;
#153514=CARTESIAN_POINT('Ctrl Pts',(1.34256163823226,2.75588931242806,-28.592914101785)) ;
#153515=CARTESIAN_POINT('Ctrl Pts',(1.34198261999809,2.75610647364238,-28.5932257815815)) ;
#153516=CARTESIAN_POINT('Ctrl Pts',(1.3413216052292,2.75635697290856,-28.5935816219833)) ;
#153517=CARTESIAN_POINT('Ctrl Pts',(1.3408629143507,2.75653491456656,-28.5938285825319)) ;
#153518=CARTESIAN_POINT('Ctrl Pts',(1.33918548989955,2.7572007950357,-28.5947318375006)) ;
#153519=CARTESIAN_POINT('Ctrl Pts',(1.33797416370948,2.75771112313095,-28.5953843482651)) ;
#153520=CARTESIAN_POINT('Ctrl Pts',(1.33648532079705,2.75837521508443,-28.5961866329489)) ;
#153521=CARTESIAN_POINT('Ctrl Pts',(1.33619776328718,2.7585052148881,-28.5963415973021)) ;
#153522=CARTESIAN_POINT('Ctrl Pts',(1.33107968015592,2.76084915994933,-28.5991000397119)) ;
#153523=CARTESIAN_POINT('Ctrl Pts',(1.32635908659411,2.76350693339047,-28.6016480195489)) ;
#153524=CARTESIAN_POINT('Ctrl Pts',(1.32109760625968,2.76707470328456,-28.6044947169122)) ;
#153525=CARTESIAN_POINT('Ctrl Pts',(1.32035743991793,2.76759128788319,-28.6048953524451)) ;
#153526=CARTESIAN_POINT('Ctrl Pts',(1.31824805546071,2.76910584227479,-28.6060376626109)) ;
#153527=CARTESIAN_POINT('Ctrl Pts',(1.31689309423377,2.77013099976528,-28.6067722633588)) ;
#153528=CARTESIAN_POINT('Ctrl Pts',(1.31545882361436,2.77127278201746,-28.6075511219407)) ;
#153529=CARTESIAN_POINT('Ctrl Pts',(1.31535582310959,2.77135510350021,-28.6076070616534)) ;
#153530=CARTESIAN_POINT('Ctrl Pts',(1.31504853092212,2.77160168095795,-28.607773973447)) ;
#153531=CARTESIAN_POINT('Ctrl Pts',(1.31461168315428,2.77195498754742,-28.6080113068541)) ;
#153532=CARTESIAN_POINT('Ctrl Pts',(1.3141774222414,2.77231219724366,-28.6082473370571)) ;
#153533=CARTESIAN_POINT('Ctrl Pts',(1.31333096026317,2.77301480846569,-28.6087075061369)) ;
#153534=CARTESIAN_POINT('Ctrl Pts',(1.31272070342858,2.77353368974767,-28.6090394568406)) ;
#153535=CARTESIAN_POINT('Ctrl Pts',(1.30969774837137,2.77616736630455,-28.6106845572382)) ;
#153536=CARTESIAN_POINT('Ctrl Pts',(1.30737022788704,2.77840054644571,-28.6119534798951)) ;
#153537=CARTESIAN_POINT('Ctrl Pts',(1.30464757270887,2.7812881754222,-28.6134387033489)) ;
#153538=CARTESIAN_POINT('Ctrl Pts',(1.3041484598108,2.7818296760662,-28.6137110126307)) ;
#153539=CARTESIAN_POINT('Ctrl Pts',(1.30260826844057,2.78353926416388,-28.6145514286369)) ;
#153540=CARTESIAN_POINT('Ctrl Pts',(1.3015832472085,2.78473373830865,-28.6151112329214)) ;
#153541=CARTESIAN_POINT('Ctrl Pts',(1.30024935135333,2.78636738852737,-28.6158398127168)) ;
#153542=CARTESIAN_POINT('Ctrl Pts',(1.29991860867239,2.78677921519271,-28.616020475081)) ;
#153543=CARTESIAN_POINT('Ctrl Pts',(1.29915346420736,2.78774794465154,-28.6164384192283)) ;
#153544=CARTESIAN_POINT('Ctrl Pts',(1.29872125904469,2.78830744810471,-28.6166744998873)) ;
#153545=CARTESIAN_POINT('Ctrl Pts',(1.29658637826223,2.79113377451589,-28.6178405320741)) ;
#153546=CARTESIAN_POINT('Ctrl Pts',(1.29496240940489,2.79348720429744,-28.6187269863698)) ;
#153547=CARTESIAN_POINT('Ctrl Pts',(1.29231665668157,2.79769679694545,-28.6201716480049)) ;
#153548=CARTESIAN_POINT('Ctrl Pts',(1.29125115601062,2.79951540543443,-28.6207540486807)) ;
#153549=CARTESIAN_POINT('Ctrl Pts',(1.28927619853496,2.80313430045116,-28.6218348789813)) ;
#153550=CARTESIAN_POINT('Ctrl Pts',(1.2883624199782,2.80493500363978,-28.6223353793459)) ;
#153551=CARTESIAN_POINT('Ctrl Pts',(1.28732027925586,2.80715235940914,-28.6229068412463)) ;
#153552=CARTESIAN_POINT('Ctrl Pts',(1.28695835013168,2.80793550920674,-28.6231053825645)) ;
#153553=CARTESIAN_POINT('Ctrl Pts',(1.28660568774192,2.80872522382218,-28.6232989562928)) ;
#153554=CARTESIAN_POINT('Ctrl Pts',(1.28608376699197,2.80991454434775,-28.6235854978985)) ;
#153555=CARTESIAN_POINT('Ctrl Pts',(1.28574525149602,2.81071375754612,-28.6237714318906)) ;
#153556=CARTESIAN_POINT('Ctrl Pts',(1.28475894023896,2.81312894312823,-28.624313266649)) ;
#153557=CARTESIAN_POINT('Ctrl Pts',(1.28414040309304,2.81476247656142,-28.624653166298)) ;
#153558=CARTESIAN_POINT('Ctrl Pts',(1.28339818260914,2.81688756020149,-28.625060888642)) ;
#153559=CARTESIAN_POINT('Ctrl Pts',(1.28323661013045,2.81736137575528,-28.6251496371781)) ;
#153560=CARTESIAN_POINT('Ctrl Pts',(1.28265668893881,2.81910411140434,-28.6254681473537)) ;
#153561=CARTESIAN_POINT('Ctrl Pts',(1.28225920250334,2.82038205281186,-28.6256863923253)) ;
#153562=CARTESIAN_POINT('Ctrl Pts',(1.28170385606937,2.82230051526767,-28.6259913349836)) ;
#153563=CARTESIAN_POINT('Ctrl Pts',(1.28152700208473,2.82293438010911,-28.6260884417703)) ;
#153564=CARTESIAN_POINT('Ctrl Pts',(1.2810744886873,2.82461913389174,-28.6263369091493)) ;
#153565=CARTESIAN_POINT('Ctrl Pts',(1.28081016954771,2.82567198476339,-28.6264819889541)) ;
#153566=CARTESIAN_POINT('Ctrl Pts',(1.28009910353319,2.82871092361134,-28.6268721680177)) ;
#153567=CARTESIAN_POINT('Ctrl Pts',(1.27969380338793,2.83071459002994,-28.6270948708801)) ;
#153568=CARTESIAN_POINT('Ctrl Pts',(1.27923282767963,2.83340629334537,-28.6273484537335)) ;
#153569=CARTESIAN_POINT('Ctrl Pts',(1.27912420342281,2.83408089926111,-28.6274082352158)) ;
#153570=CARTESIAN_POINT('Ctrl Pts',(1.27861441353187,2.83746106027946,-28.6276889088183)) ;
#153571=CARTESIAN_POINT('Ctrl Pts',(1.27831324287571,2.8401879948702,-28.6278550982434)) ;
#153572=CARTESIAN_POINT('Ctrl Pts',(1.27795656969996,2.84527977141541,-28.6280519866561)) ;
#153573=CARTESIAN_POINT('Ctrl Pts',(1.27787304021906,2.84764286211078,-28.6280981416173)) ;
#153574=CARTESIAN_POINT('Ctrl Pts',(1.27787304021907,2.85,-28.6280981416173)) ;
#153575=CARTESIAN_POINT('Origin',(1.77490703981929,4.45,-35.7754875)) ;
#153576=CARTESIAN_POINT('',(1.64874898520161,4.55,-35.6699010050713)) ;
#153577=CARTESIAN_POINT('',(1.77490703981929,4.55,-35.94)) ;
#153578=CARTESIAN_POINT('Origin',(1.77490703981929,4.55,-35.7754875)) ;
#153579=CARTESIAN_POINT('',(1.72543498451332,4.45,-35.7340824471676)) ;
#153580=CARTESIAN_POINT('Origin',(1.64874898520161,4.45,-35.6699010050713)) ;
#153581=CARTESIAN_POINT('',(1.77490703981929,4.45,-35.84)) ;
#153582=CARTESIAN_POINT('Origin',(1.77490703981929,4.45,-35.7754875)) ;
#153583=CARTESIAN_POINT('Origin',(1.77490703981929,4.45,-35.94)) ;
#153584=CARTESIAN_POINT('Origin',(-3.7454256867681E-16,2.85,-34.29)) ;
#153585=CARTESIAN_POINT('',(1.8493242008907,2.75,-35.74)) ;
#153586=CARTESIAN_POINT('Origin',(-3.66728498965203E-16,2.75,-34.29)) ;
#153587=CARTESIAN_POINT('',(1.72543498451332,2.85,-35.7340824471676)) ;
#153588=CARTESIAN_POINT('Ctrl Pts',(1.8493242008907,2.75,-35.74)) ;
#153589=CARTESIAN_POINT('Ctrl Pts',(1.84863058979382,2.75,-35.7399756373587)) ;
#153590=CARTESIAN_POINT('Ctrl Pts',(1.84793752344333,2.75000415508911,-35.7399513120665)) ;
#153591=CARTESIAN_POINT('Ctrl Pts',(1.84666827906651,2.75001949937824,-35.7399065432933)) ;
#153592=CARTESIAN_POINT('Ctrl Pts',(1.84609162157503,2.75002939777743,-35.7398860603461)) ;
#153593=CARTESIAN_POINT('Ctrl Pts',(1.84477120566862,2.75005887738352,-35.7398388427818)) ;
#153594=CARTESIAN_POINT('Ctrl Pts',(1.84402746838176,2.75008043331235,-35.7398120489461)) ;
#153595=CARTESIAN_POINT('Ctrl Pts',(1.84209973630451,2.75014939605133,-35.7397420584709)) ;
#153596=CARTESIAN_POINT('Ctrl Pts',(1.84091590068189,2.75020455995203,-35.7396985450601)) ;
#153597=CARTESIAN_POINT('Ctrl Pts',(1.83783446245732,2.75038253459259,-35.7395838306667)) ;
#153598=CARTESIAN_POINT('Ctrl Pts',(1.83593755875577,2.75052613608887,-35.7395117702048)) ;
#153599=CARTESIAN_POINT('Ctrl Pts',(1.83094562972781,2.75099782378457,-35.7393183459611)) ;
#153600=CARTESIAN_POINT('Ctrl Pts',(1.82785402838397,2.75138590243717,-35.7391945850334)) ;
#153601=CARTESIAN_POINT('Ctrl Pts',(1.8194803599521,2.75271158620497,-35.7388527720391)) ;
#153602=CARTESIAN_POINT('Ctrl Pts',(1.81421216401677,2.75385084739026,-35.7386282240443)) ;
#153603=CARTESIAN_POINT('Ctrl Pts',(1.80309951666291,2.7569571777553,-35.7381406444328)) ;
#153604=CARTESIAN_POINT('Ctrl Pts',(1.79729559107017,2.75901332923639,-35.7378834222529)) ;
#153605=CARTESIAN_POINT('Ctrl Pts',(1.78960373217334,2.76233413717723,-35.7375331406995)) ;
#153606=CARTESIAN_POINT('Ctrl Pts',(1.78754713318247,2.76328353076603,-35.7374383836782)) ;
#153607=CARTESIAN_POINT('Ctrl Pts',(1.7829081527366,2.76556355836307,-35.7372206639426)) ;
#153608=CARTESIAN_POINT('Ctrl Pts',(1.78033073359812,2.76693246555665,-35.7370964957842)) ;
#153609=CARTESIAN_POINT('Ctrl Pts',(1.7769923351545,2.76883988197349,-35.7369304274279)) ;
#153610=CARTESIAN_POINT('Ctrl Pts',(1.77620130341387,2.7693016905685,-35.7368906872082)) ;
#153611=CARTESIAN_POINT('Ctrl Pts',(1.7700212686897,2.77299328865073,-35.7365769643392)) ;
#153612=CARTESIAN_POINT('Ctrl Pts',(1.76495428809394,2.77651771765647,-35.7363064706027)) ;
#153613=CARTESIAN_POINT('Ctrl Pts',(1.75938438670095,2.78118533566922,-35.7360042033494)) ;
#153614=CARTESIAN_POINT('Ctrl Pts',(1.75866155316797,2.78180749698893,-35.7359648787297)) ;
#153615=CARTESIAN_POINT('Ctrl Pts',(1.75440101126575,2.78557661565333,-35.7357327262068)) ;
#153616=CARTESIAN_POINT('Ctrl Pts',(1.75110534239499,2.7889111885936,-35.7355622025983)) ;
#153617=CARTESIAN_POINT('Ctrl Pts',(1.74704475763666,2.79358254909143,-35.73534353206)) ;
#153618=CARTESIAN_POINT('Ctrl Pts',(1.74604050383922,2.79479094319558,-35.7352885793349)) ;
#153619=CARTESIAN_POINT('Ctrl Pts',(1.74487333929766,2.79625803001554,-35.7352226603584)) ;
#153620=CARTESIAN_POINT('Ctrl Pts',(1.74467927949938,2.79650417922903,-35.7352116332551)) ;
#153621=CARTESIAN_POINT('Ctrl Pts',(1.74115657836479,2.8010141242866,-35.7350100972494)) ;
#153622=CARTESIAN_POINT('Ctrl Pts',(1.73808736282556,2.80561663574421,-35.7348305563636)) ;
#153623=CARTESIAN_POINT('Ctrl Pts',(1.73411503311369,2.81315073291946,-35.7345973211718)) ;
#153624=CARTESIAN_POINT('Ctrl Pts',(1.73300100590541,2.81551882664669,-35.734535439772)) ;
#153625=CARTESIAN_POINT('Ctrl Pts',(1.73189652742024,2.8181493620667,-35.7344706989523)) ;
#153626=CARTESIAN_POINT('Ctrl Pts',(1.73180208385961,2.81837683840677,-35.7344651616954)) ;
#153627=CARTESIAN_POINT('Ctrl Pts',(1.73016675860412,2.82236036724429,-35.7343692539515)) ;
#153628=CARTESIAN_POINT('Ctrl Pts',(1.72888947962493,2.82624394236213,-35.7342946666905)) ;
#153629=CARTESIAN_POINT('Ctrl Pts',(1.7277066333756,2.83096681006087,-35.7342247776101)) ;
#153630=CARTESIAN_POINT('Ctrl Pts',(1.72752382530051,2.83174344980853,-35.7342139400975)) ;
#153631=CARTESIAN_POINT('Ctrl Pts',(1.72719333568989,2.83324353771481,-35.7341942520731)) ;
#153632=CARTESIAN_POINT('Ctrl Pts',(1.72704413780186,2.83396640281167,-35.7341852797154)) ;
#153633=CARTESIAN_POINT('Ctrl Pts',(1.72602501437422,2.83926193721102,-35.7341230804511)) ;
#153634=CARTESIAN_POINT('Ctrl Pts',(1.7255299684319,2.84393088107749,-35.7340890562028)) ;
#153635=CARTESIAN_POINT('Ctrl Pts',(1.72543914472536,2.84906100604876,-35.7340827399932)) ;
#153636=CARTESIAN_POINT('Ctrl Pts',(1.72543498451331,2.84953057829675,-35.7340824471676)) ;
#153637=CARTESIAN_POINT('Ctrl Pts',(1.72543498451331,2.85,-35.7340824471676)) ;
#153638=CARTESIAN_POINT('',(1.27787304021906,2.85,-32.4380981416173)) ;
#153639=CARTESIAN_POINT('Origin',(-3.7454256867681E-16,2.85,-34.29)) ;
#153640=CARTESIAN_POINT('Ctrl Pts',(1.37603597336698,2.75,-32.385)) ;
#153641=CARTESIAN_POINT('Ctrl Pts',(1.37543428354307,2.75,-32.3853199418865)) ;
#153642=CARTESIAN_POINT('Ctrl Pts',(1.37483253111457,2.7500053137259,-32.3856398156589)) ;
#153643=CARTESIAN_POINT('Ctrl Pts',(1.3738872267507,2.75002207412044,-32.3861426442071)) ;
#153644=CARTESIAN_POINT('Ctrl Pts',(1.37354350385558,2.75002991650282,-32.3863255141623)) ;
#153645=CARTESIAN_POINT('Ctrl Pts',(1.37285611423782,2.75004911307826,-32.3866912988841)) ;
#153646=CARTESIAN_POINT('Ctrl Pts',(1.37251244753525,2.75006046723047,-32.3868742136115)) ;
#153647=CARTESIAN_POINT('Ctrl Pts',(1.3714815944481,2.75009981984526,-32.387422994695)) ;
#153648=CARTESIAN_POINT('Ctrl Pts',(1.37079455494331,2.75013310886333,-32.3877888982032)) ;
#153649=CARTESIAN_POINT('Ctrl Pts',(1.36873453110893,2.75025430438115,-32.3888865055866)) ;
#153650=CARTESIAN_POINT('Ctrl Pts',(1.36736263966052,2.75036354665963,-32.3896181092421)) ;
#153651=CARTESIAN_POINT('Ctrl Pts',(1.36413470836879,2.75068903914081,-32.3913410689378)) ;
#153652=CARTESIAN_POINT('Ctrl Pts',(1.36227932197148,2.75092980851021,-32.392332637721)) ;
#153653=CARTESIAN_POINT('Ctrl Pts',(1.35746012444743,2.7516985967038,-32.3949111819216)) ;
#153654=CARTESIAN_POINT('Ctrl Pts',(1.35450425835489,2.75231332717651,-32.3964957625411)) ;
#153655=CARTESIAN_POINT('Ctrl Pts',(1.34886973918565,2.75377034241463,-32.3995208305066)) ;
#153656=CARTESIAN_POINT('Ctrl Pts',(1.34617831568151,2.75459534478001,-32.4009678592584)) ;
#153657=CARTESIAN_POINT('Ctrl Pts',(1.34314242260183,2.75567798707047,-32.4026015301229)) ;
#153658=CARTESIAN_POINT('Ctrl Pts',(1.34256163823227,2.75588931242805,-32.402914101785)) ;
#153659=CARTESIAN_POINT('Ctrl Pts',(1.3419826199981,2.75610647364237,-32.4032257815815)) ;
#153660=CARTESIAN_POINT('Ctrl Pts',(1.34132160522921,2.75635697290855,-32.4035816219833)) ;
#153661=CARTESIAN_POINT('Ctrl Pts',(1.34086291435071,2.75653491456655,-32.4038285825319)) ;
#153662=CARTESIAN_POINT('Ctrl Pts',(1.33918548989956,2.75720079503569,-32.4047318375006)) ;
#153663=CARTESIAN_POINT('Ctrl Pts',(1.33797416370949,2.75771112313094,-32.4053843482652)) ;
#153664=CARTESIAN_POINT('Ctrl Pts',(1.33648532079706,2.75837521508442,-32.4061866329489)) ;
#153665=CARTESIAN_POINT('Ctrl Pts',(1.33619776328718,2.75850521488809,-32.4063415973022)) ;
#153666=CARTESIAN_POINT('Ctrl Pts',(1.33107968015782,2.76084915994844,-32.4091000397109)) ;
#153667=CARTESIAN_POINT('Ctrl Pts',(1.32635908659783,2.76350693338837,-32.4116480195469)) ;
#153668=CARTESIAN_POINT('Ctrl Pts',(1.32109760626318,2.76707470328213,-32.4144947169103)) ;
#153669=CARTESIAN_POINT('Ctrl Pts',(1.32035743991961,2.76759128788199,-32.4148953524442)) ;
#153670=CARTESIAN_POINT('Ctrl Pts',(1.31824805546064,2.76910584227485,-32.4160376626109)) ;
#153671=CARTESIAN_POINT('Ctrl Pts',(1.31689309423374,2.77013099976531,-32.4167722633589)) ;
#153672=CARTESIAN_POINT('Ctrl Pts',(1.31545882361431,2.77127278201751,-32.4175511219408)) ;
#153673=CARTESIAN_POINT('Ctrl Pts',(1.31535582310949,2.77135510350029,-32.4176070616535)) ;
#153674=CARTESIAN_POINT('Ctrl Pts',(1.31504853092197,2.77160168095808,-32.4177739734471)) ;
#153675=CARTESIAN_POINT('Ctrl Pts',(1.31461168315413,2.77195498754755,-32.4180113068542)) ;
#153676=CARTESIAN_POINT('Ctrl Pts',(1.31417742224124,2.77231219724379,-32.4182473370572)) ;
#153677=CARTESIAN_POINT('Ctrl Pts',(1.31333096026301,2.77301480846583,-32.418707506137)) ;
#153678=CARTESIAN_POINT('Ctrl Pts',(1.31272070342842,2.77353368974781,-32.4190394568407)) ;
#153679=CARTESIAN_POINT('Ctrl Pts',(1.30969774837119,2.77616736630471,-32.4206845572383)) ;
#153680=CARTESIAN_POINT('Ctrl Pts',(1.30737022788685,2.7784005464459,-32.4219534798952)) ;
#153681=CARTESIAN_POINT('Ctrl Pts',(1.30464757270875,2.78128817542236,-32.423438703349)) ;
#153682=CARTESIAN_POINT('Ctrl Pts',(1.30414845981073,2.78182967606625,-32.4237110126308)) ;
#153683=CARTESIAN_POINT('Ctrl Pts',(1.30260826844057,2.78353926416386,-32.4245514286369)) ;
#153684=CARTESIAN_POINT('Ctrl Pts',(1.30158324720851,2.78473373830864,-32.4251112329214)) ;
#153685=CARTESIAN_POINT('Ctrl Pts',(1.30024935135334,2.78636738852736,-32.4258398127168)) ;
#153686=CARTESIAN_POINT('Ctrl Pts',(1.29991860867239,2.7867792151927,-32.4260204750811)) ;
#153687=CARTESIAN_POINT('Ctrl Pts',(1.29915346420736,2.78774794465152,-32.4264384192283)) ;
#153688=CARTESIAN_POINT('Ctrl Pts',(1.2987212590447,2.7883074481047,-32.4266744998873)) ;
#153689=CARTESIAN_POINT('Ctrl Pts',(1.29658637826224,2.79113377451588,-32.4278405320741)) ;
#153690=CARTESIAN_POINT('Ctrl Pts',(1.29496240940489,2.79348720429742,-32.4287269863698)) ;
#153691=CARTESIAN_POINT('Ctrl Pts',(1.29231665668157,2.79769679694543,-32.430171648005)) ;
#153692=CARTESIAN_POINT('Ctrl Pts',(1.29125115601062,2.79951540543442,-32.4307540486807)) ;
#153693=CARTESIAN_POINT('Ctrl Pts',(1.28927619853496,2.80313430045114,-32.4318348789813)) ;
#153694=CARTESIAN_POINT('Ctrl Pts',(1.2883624199782,2.80493500363976,-32.4323353793459)) ;
#153695=CARTESIAN_POINT('Ctrl Pts',(1.28732027925586,2.80715235940912,-32.4329068412463)) ;
#153696=CARTESIAN_POINT('Ctrl Pts',(1.28695835013166,2.80793550920672,-32.4331053825645)) ;
#153697=CARTESIAN_POINT('Ctrl Pts',(1.28660568774192,2.80872522382215,-32.4332989562928)) ;
#153698=CARTESIAN_POINT('Ctrl Pts',(1.28608376699198,2.80991454434771,-32.4335854978985)) ;
#153699=CARTESIAN_POINT('Ctrl Pts',(1.28574525149603,2.81071375754607,-32.4337714318906)) ;
#153700=CARTESIAN_POINT('Ctrl Pts',(1.28475894023899,2.81312894312816,-32.434313266649)) ;
#153701=CARTESIAN_POINT('Ctrl Pts',(1.28414040309307,2.81476247656134,-32.434653166298)) ;
#153702=CARTESIAN_POINT('Ctrl Pts',(1.28339818260918,2.81688756020139,-32.435060888642)) ;
#153703=CARTESIAN_POINT('Ctrl Pts',(1.28323661013049,2.81736137575517,-32.4351496371781)) ;
#153704=CARTESIAN_POINT('Ctrl Pts',(1.28265668893886,2.81910411140422,-32.4354681473537)) ;
#153705=CARTESIAN_POINT('Ctrl Pts',(1.2822592025034,2.82038205281173,-32.4356863923252)) ;
#153706=CARTESIAN_POINT('Ctrl Pts',(1.28170385606942,2.82230051526758,-32.4359913349836)) ;
#153707=CARTESIAN_POINT('Ctrl Pts',(1.28152700208476,2.82293438010907,-32.4360884417703)) ;
#153708=CARTESIAN_POINT('Ctrl Pts',(1.28107448868733,2.82461913389174,-32.4363369091493)) ;
#153709=CARTESIAN_POINT('Ctrl Pts',(1.28081016954774,2.82567198476339,-32.4364819889541)) ;
#153710=CARTESIAN_POINT('Ctrl Pts',(1.28009910353322,2.82871092361133,-32.4368721680177)) ;
#153711=CARTESIAN_POINT('Ctrl Pts',(1.27969380338795,2.83071459002993,-32.43709487088)) ;
#153712=CARTESIAN_POINT('Ctrl Pts',(1.27923282767965,2.83340629334535,-32.4373484537334)) ;
#153713=CARTESIAN_POINT('Ctrl Pts',(1.27912420342283,2.83408089926109,-32.4374082352158)) ;
#153714=CARTESIAN_POINT('Ctrl Pts',(1.27861441353189,2.83746106027944,-32.4376889088183)) ;
#153715=CARTESIAN_POINT('Ctrl Pts',(1.27831324287571,2.84018799487016,-32.4378550982434)) ;
#153716=CARTESIAN_POINT('Ctrl Pts',(1.27795656969996,2.84527977141538,-32.4380519866561)) ;
#153717=CARTESIAN_POINT('Ctrl Pts',(1.27787304021906,2.84764286211077,-32.4380981416173)) ;
#153718=CARTESIAN_POINT('Ctrl Pts',(1.27787304021907,2.85,-32.4380981416173)) ;
#153719=CARTESIAN_POINT('Origin',(1.3145125,-1.51907484122731,-28.575)) ;
#153720=CARTESIAN_POINT('Origin',(1.3145125,2.85,-28.575)) ;
#153721=CARTESIAN_POINT('',(1.27787304021905,-1.51907484122731,-28.6280981416173)) ;
#153722=CARTESIAN_POINT('',(1.27787304021905,-1.51907484122731,-28.5219018583827)) ;
#153723=CARTESIAN_POINT('Origin',(1.3145125,-1.51907484122731,-24.765)) ;
#153724=CARTESIAN_POINT('Origin',(1.3145125,2.85,-24.765)) ;
#153725=CARTESIAN_POINT('',(1.27787304021905,-1.51907484122731,-24.8180981416173)) ;
#153726=CARTESIAN_POINT('',(1.27787304021905,-1.51907484122731,-24.7119018583827)) ;
#153727=CARTESIAN_POINT('Origin',(1.3145125,-1.51907484122731,-20.955)) ;
#153728=CARTESIAN_POINT('Origin',(1.3145125,2.85,-20.955)) ;
#153729=CARTESIAN_POINT('',(1.27787304021905,-1.51907484122731,-21.0080981416173)) ;
#153730=CARTESIAN_POINT('',(1.27787304021905,-1.51907484122731,-20.9019018583827)) ;
#153731=CARTESIAN_POINT('Origin',(1.3145125,-1.51907484122731,-17.145)) ;
#153732=CARTESIAN_POINT('Origin',(1.3145125,2.85,-17.145)) ;
#153733=CARTESIAN_POINT('',(1.27787304021905,-1.51907484122731,-17.1980981416173)) ;
#153734=CARTESIAN_POINT('',(1.27787304021905,-1.51907484122731,-17.0919018583827)) ;
#153735=CARTESIAN_POINT('Origin',(1.3145125,-1.51907484122731,-13.335)) ;
#153736=CARTESIAN_POINT('Origin',(1.3145125,2.85,-13.335)) ;
#153737=CARTESIAN_POINT('',(1.27787304021905,-1.51907484122731,-13.3880981416173)) ;
#153738=CARTESIAN_POINT('',(1.27787304021905,-1.51907484122731,-13.2819018583827)) ;
#153739=CARTESIAN_POINT('Origin',(1.3145125,-1.51907484122731,-9.525)) ;
#153740=CARTESIAN_POINT('Origin',(1.3145125,2.85,-9.525)) ;
#153741=CARTESIAN_POINT('',(1.27787304021905,-1.51907484122731,-9.57809814161729)) ;
#153742=CARTESIAN_POINT('',(1.27787304021905,-1.51907484122731,-9.4719018583827)) ;
#153743=CARTESIAN_POINT('Origin',(1.3145125,-1.51907484122731,-5.715)) ;
#153744=CARTESIAN_POINT('Origin',(1.3145125,2.85,-5.715)) ;
#153745=CARTESIAN_POINT('',(1.27787304021905,-1.51907484122731,-5.76809814161729)) ;
#153746=CARTESIAN_POINT('',(1.27787304021905,-1.51907484122731,-5.66190185838271)) ;
#153747=CARTESIAN_POINT('Origin',(9.24142135623731,0.,-34.29)) ;
#153748=CARTESIAN_POINT('',(9.17071067811866,-1.18877772485616E-16,-33.3192893218813)) ;
#153749=CARTESIAN_POINT('Origin',(9.17071067811866,0.,-34.29)) ;
#153750=CARTESIAN_POINT('',(9.24142135623731,-1.22464679914736E-16,-33.29)) ;
#153751=CARTESIAN_POINT('Origin',(9.24142135623731,-1.10218211923262E-16,
-33.39)) ;
#153752=CARTESIAN_POINT('Origin',(9.24142135623731,0.,-34.29)) ;
#153753=CARTESIAN_POINT('Origin',(-6.11095769946375E-16,4.45,-34.29)) ;
#153754=CARTESIAN_POINT('',(1.5,4.45,-34.29)) ;
#153755=CARTESIAN_POINT('Origin',(-6.11095769946375E-16,4.45,-34.29)) ;
#153756=CARTESIAN_POINT('',(1.6,4.55,-34.29)) ;
#153757=CARTESIAN_POINT('Origin',(1.6,4.45,-34.29)) ;
#153758=CARTESIAN_POINT('Origin',(-6.24237614461351E-16,4.55,-34.29)) ;
#153759=CARTESIAN_POINT('Origin',(10.1,0.,-34.29)) ;
#153760=CARTESIAN_POINT('',(10.1,-1.22464679914735E-16,-33.29)) ;
#153761=CARTESIAN_POINT('Origin',(10.1,0.,-34.29)) ;
#153762=CARTESIAN_POINT('',(10.2,-1.34711147906209E-16,-33.19)) ;
#153763=CARTESIAN_POINT('Origin',(10.1,-1.34711147906209E-16,-33.19)) ;
#153764=CARTESIAN_POINT('Origin',(10.2,0.,-34.29)) ;
#153765=CARTESIAN_POINT('Origin',(9.24142135623731,0.,-30.48)) ;
#153766=CARTESIAN_POINT('',(9.17071067811866,-1.18877772485617E-16,-29.5092893218813)) ;
#153767=CARTESIAN_POINT('Origin',(9.17071067811866,0.,-30.48)) ;
#153768=CARTESIAN_POINT('',(9.24142135623731,-1.22464679914735E-16,-29.48)) ;
#153769=CARTESIAN_POINT('Origin',(9.24142135623731,-1.10218211923262E-16,
-29.58)) ;
#153770=CARTESIAN_POINT('Origin',(9.24142135623731,0.,-30.48)) ;
#153771=CARTESIAN_POINT('Origin',(-6.11095769946375E-16,4.45,-30.48)) ;
#153772=CARTESIAN_POINT('',(1.5,4.45,-30.48)) ;
#153773=CARTESIAN_POINT('Origin',(-6.11095769946375E-16,4.45,-30.48)) ;
#153774=CARTESIAN_POINT('',(1.6,4.55,-30.48)) ;
#153775=CARTESIAN_POINT('Origin',(1.6,4.45,-30.48)) ;
#153776=CARTESIAN_POINT('Origin',(-6.24237614461351E-16,4.55,-30.48)) ;
#153777=CARTESIAN_POINT('Origin',(10.1,0.,-30.48)) ;
#153778=CARTESIAN_POINT('',(10.1,-1.22464679914735E-16,-29.48)) ;
#153779=CARTESIAN_POINT('Origin',(10.1,0.,-30.48)) ;
#153780=CARTESIAN_POINT('',(10.2,-1.34711147906209E-16,-29.38)) ;
#153781=CARTESIAN_POINT('Origin',(10.1,-1.34711147906209E-16,-29.38)) ;
#153782=CARTESIAN_POINT('Origin',(10.2,0.,-30.48)) ;
#153783=CARTESIAN_POINT('Origin',(9.24142135623731,0.,-26.67)) ;
#153784=CARTESIAN_POINT('',(9.17071067811866,-1.18877772485617E-16,-25.6992893218813)) ;
#153785=CARTESIAN_POINT('Origin',(9.17071067811866,0.,-26.67)) ;
#153786=CARTESIAN_POINT('',(9.24142135623731,-1.22464679914735E-16,-25.67)) ;
#153787=CARTESIAN_POINT('Origin',(9.24142135623731,-1.10218211923262E-16,
-25.77)) ;
#153788=CARTESIAN_POINT('Origin',(9.24142135623731,0.,-26.67)) ;
#153789=CARTESIAN_POINT('Origin',(-6.11095769946375E-16,4.45,-26.67)) ;
#153790=CARTESIAN_POINT('',(1.5,4.45,-26.67)) ;
#153791=CARTESIAN_POINT('Origin',(-6.11095769946375E-16,4.45,-26.67)) ;
#153792=CARTESIAN_POINT('',(1.6,4.55,-26.67)) ;
#153793=CARTESIAN_POINT('Origin',(1.6,4.45,-26.67)) ;
#153794=CARTESIAN_POINT('Origin',(-6.24237614461351E-16,4.55,-26.67)) ;
#153795=CARTESIAN_POINT('Origin',(10.1,0.,-26.67)) ;
#153796=CARTESIAN_POINT('',(10.1,-1.22464679914735E-16,-25.67)) ;
#153797=CARTESIAN_POINT('Origin',(10.1,0.,-26.67)) ;
#153798=CARTESIAN_POINT('',(10.2,-1.34711147906209E-16,-25.57)) ;
#153799=CARTESIAN_POINT('Origin',(10.1,-1.34711147906209E-16,-25.57)) ;
#153800=CARTESIAN_POINT('Origin',(10.2,0.,-26.67)) ;
#153801=CARTESIAN_POINT('Origin',(9.24142135623731,0.,-22.86)) ;
#153802=CARTESIAN_POINT('',(9.17071067811866,-1.18877772485617E-16,-21.8892893218813)) ;
#153803=CARTESIAN_POINT('Origin',(9.17071067811866,0.,-22.86)) ;
#153804=CARTESIAN_POINT('',(9.24142135623731,-1.22464679914735E-16,-21.86)) ;
#153805=CARTESIAN_POINT('Origin',(9.24142135623731,-1.10218211923262E-16,
-21.96)) ;
#153806=CARTESIAN_POINT('Origin',(9.24142135623731,0.,-22.86)) ;
#153807=CARTESIAN_POINT('Origin',(-6.11095769946375E-16,4.45,-22.86)) ;
#153808=CARTESIAN_POINT('',(1.5,4.45,-22.86)) ;
#153809=CARTESIAN_POINT('Origin',(-6.11095769946375E-16,4.45,-22.86)) ;
#153810=CARTESIAN_POINT('',(1.6,4.55,-22.86)) ;
#153811=CARTESIAN_POINT('Origin',(1.6,4.45,-22.86)) ;
#153812=CARTESIAN_POINT('Origin',(-6.24237614461351E-16,4.55,-22.86)) ;
#153813=CARTESIAN_POINT('Origin',(10.1,0.,-22.86)) ;
#153814=CARTESIAN_POINT('',(10.1,-1.22464679914735E-16,-21.86)) ;
#153815=CARTESIAN_POINT('Origin',(10.1,0.,-22.86)) ;
#153816=CARTESIAN_POINT('',(10.2,-1.34711147906209E-16,-21.76)) ;
#153817=CARTESIAN_POINT('Origin',(10.1,-1.34711147906209E-16,-21.76)) ;
#153818=CARTESIAN_POINT('Origin',(10.2,0.,-22.86)) ;
#153819=CARTESIAN_POINT('Origin',(9.24142135623731,0.,-19.05)) ;
#153820=CARTESIAN_POINT('',(9.17071067811866,-1.18877772485617E-16,-18.0792893218813)) ;
#153821=CARTESIAN_POINT('Origin',(9.17071067811866,0.,-19.05)) ;
#153822=CARTESIAN_POINT('',(9.24142135623731,-1.22464679914736E-16,-18.05)) ;
#153823=CARTESIAN_POINT('Origin',(9.24142135623731,-1.10218211923262E-16,
-18.15)) ;
#153824=CARTESIAN_POINT('Origin',(9.24142135623731,0.,-19.05)) ;
#153825=CARTESIAN_POINT('Origin',(-6.11095769946375E-16,4.45,-19.05)) ;
#153826=CARTESIAN_POINT('',(1.5,4.45,-19.05)) ;
#153827=CARTESIAN_POINT('Origin',(-6.11095769946375E-16,4.45,-19.05)) ;
#153828=CARTESIAN_POINT('',(1.6,4.55,-19.05)) ;
#153829=CARTESIAN_POINT('Origin',(1.6,4.45,-19.05)) ;
#153830=CARTESIAN_POINT('Origin',(-6.24237614461351E-16,4.55,-19.05)) ;
#153831=CARTESIAN_POINT('Origin',(10.1,0.,-19.05)) ;
#153832=CARTESIAN_POINT('',(10.1,-1.22464679914735E-16,-18.05)) ;
#153833=CARTESIAN_POINT('Origin',(10.1,0.,-19.05)) ;
#153834=CARTESIAN_POINT('',(10.2,-1.34711147906209E-16,-17.95)) ;
#153835=CARTESIAN_POINT('Origin',(10.1,-1.34711147906209E-16,-17.95)) ;
#153836=CARTESIAN_POINT('Origin',(10.2,0.,-19.05)) ;
#153837=CARTESIAN_POINT('Origin',(9.24142135623732,0.,-15.24)) ;
#153838=CARTESIAN_POINT('',(9.17071067811866,-1.18877772485617E-16,-14.2692893218813)) ;
#153839=CARTESIAN_POINT('Origin',(9.17071067811866,0.,-15.24)) ;
#153840=CARTESIAN_POINT('',(9.24142135623732,-1.22464679914736E-16,-14.24)) ;
#153841=CARTESIAN_POINT('Origin',(9.24142135623732,-1.10218211923262E-16,
-14.34)) ;
#153842=CARTESIAN_POINT('Origin',(9.24142135623732,0.,-15.24)) ;
#153843=CARTESIAN_POINT('Origin',(-6.11095769946375E-16,4.45,-15.24)) ;
#153844=CARTESIAN_POINT('',(1.5,4.45,-15.24)) ;
#153845=CARTESIAN_POINT('Origin',(-6.11095769946375E-16,4.45,-15.24)) ;
#153846=CARTESIAN_POINT('',(1.6,4.55,-15.24)) ;
#153847=CARTESIAN_POINT('Origin',(1.6,4.45,-15.24)) ;
#153848=CARTESIAN_POINT('Origin',(-6.24237614461351E-16,4.55,-15.24)) ;
#153849=CARTESIAN_POINT('Origin',(10.1,0.,-15.24)) ;
#153850=CARTESIAN_POINT('',(10.1,-1.22464679914735E-16,-14.24)) ;
#153851=CARTESIAN_POINT('Origin',(10.1,0.,-15.24)) ;
#153852=CARTESIAN_POINT('',(10.2,-1.34711147906209E-16,-14.14)) ;
#153853=CARTESIAN_POINT('Origin',(10.1,-1.34711147906209E-16,-14.14)) ;
#153854=CARTESIAN_POINT('Origin',(10.2,0.,-15.24)) ;
#153855=CARTESIAN_POINT('Origin',(9.24142135623732,0.,-11.43)) ;
#153856=CARTESIAN_POINT('',(9.17071067811866,-1.18877772485617E-16,-10.4592893218813)) ;
#153857=CARTESIAN_POINT('Origin',(9.17071067811866,0.,-11.43)) ;
#153858=CARTESIAN_POINT('',(9.24142135623732,-1.22464679914736E-16,-10.43)) ;
#153859=CARTESIAN_POINT('Origin',(9.24142135623732,-1.10218211923262E-16,
-10.53)) ;
#153860=CARTESIAN_POINT('Origin',(9.24142135623732,0.,-11.43)) ;
#153861=CARTESIAN_POINT('Origin',(-6.11095769946375E-16,4.45,-11.43)) ;
#153862=CARTESIAN_POINT('',(1.5,4.45,-11.43)) ;
#153863=CARTESIAN_POINT('Origin',(-6.11095769946375E-16,4.45,-11.43)) ;
#153864=CARTESIAN_POINT('',(1.6,4.55,-11.43)) ;
#153865=CARTESIAN_POINT('Origin',(1.6,4.45,-11.43)) ;
#153866=CARTESIAN_POINT('Origin',(-6.24237614461351E-16,4.55,-11.43)) ;
#153867=CARTESIAN_POINT('Origin',(10.1,0.,-11.43)) ;
#153868=CARTESIAN_POINT('',(10.1,-1.22464679914735E-16,-10.43)) ;
#153869=CARTESIAN_POINT('Origin',(10.1,0.,-11.43)) ;
#153870=CARTESIAN_POINT('',(10.2,-1.34711147906209E-16,-10.33)) ;
#153871=CARTESIAN_POINT('Origin',(10.1,-1.34711147906209E-16,-10.33)) ;
#153872=CARTESIAN_POINT('Origin',(10.2,0.,-11.43)) ;
#153873=CARTESIAN_POINT('Origin',(9.24142135623731,0.,-7.62)) ;
#153874=CARTESIAN_POINT('',(9.17071067811866,-1.18877772485617E-16,-6.64928932188134)) ;
#153875=CARTESIAN_POINT('Origin',(9.17071067811866,0.,-7.62)) ;
#153876=CARTESIAN_POINT('',(9.24142135623731,-1.22464679914735E-16,-6.62)) ;
#153877=CARTESIAN_POINT('Origin',(9.24142135623731,-1.10218211923262E-16,
-6.72)) ;
#153878=CARTESIAN_POINT('Origin',(9.24142135623731,0.,-7.62)) ;
#153879=CARTESIAN_POINT('Origin',(-6.11095769946375E-16,4.45,-7.62)) ;
#153880=CARTESIAN_POINT('',(1.5,4.45,-7.62)) ;
#153881=CARTESIAN_POINT('Origin',(-6.11095769946375E-16,4.45,-7.62)) ;
#153882=CARTESIAN_POINT('',(1.6,4.55,-7.62)) ;
#153883=CARTESIAN_POINT('Origin',(1.6,4.45,-7.62)) ;
#153884=CARTESIAN_POINT('Origin',(-6.24237614461351E-16,4.55,-7.62)) ;
#153885=CARTESIAN_POINT('Origin',(10.1,0.,-7.62)) ;
#153886=CARTESIAN_POINT('',(10.1,-1.22464679914735E-16,-6.62)) ;
#153887=CARTESIAN_POINT('Origin',(10.1,0.,-7.62)) ;
#153888=CARTESIAN_POINT('',(10.2,-1.34711147906209E-16,-6.52)) ;
#153889=CARTESIAN_POINT('Origin',(10.1,-1.34711147906209E-16,-6.52)) ;
#153890=CARTESIAN_POINT('Origin',(10.2,0.,-7.62)) ;
#153891=CARTESIAN_POINT('Origin',(9.24142135623731,0.,-3.81)) ;
#153892=CARTESIAN_POINT('',(9.17071067811866,-1.18877772485617E-16,-2.83928932188134)) ;
#153893=CARTESIAN_POINT('Origin',(9.17071067811866,0.,-3.81)) ;
#153894=CARTESIAN_POINT('',(9.24142135623731,-1.22464679914735E-16,-2.81)) ;
#153895=CARTESIAN_POINT('Origin',(9.24142135623731,-1.10218211923262E-16,
-2.91)) ;
#153896=CARTESIAN_POINT('Origin',(9.24142135623731,0.,-3.81)) ;
#153897=CARTESIAN_POINT('Origin',(-6.11095769946375E-16,4.45,-3.81)) ;
#153898=CARTESIAN_POINT('',(1.5,4.45,-3.81)) ;
#153899=CARTESIAN_POINT('Origin',(-6.11095769946375E-16,4.45,-3.81)) ;
#153900=CARTESIAN_POINT('',(1.6,4.55,-3.81)) ;
#153901=CARTESIAN_POINT('Origin',(1.6,4.45,-3.81)) ;
#153902=CARTESIAN_POINT('Origin',(-6.24237614461351E-16,4.55,-3.81)) ;
#153903=CARTESIAN_POINT('Origin',(10.1,0.,-3.81)) ;
#153904=CARTESIAN_POINT('',(10.1,-1.22464679914735E-16,-2.81)) ;
#153905=CARTESIAN_POINT('Origin',(10.1,0.,-3.81)) ;
#153906=CARTESIAN_POINT('',(10.2,-1.34711147906209E-16,-2.71)) ;
#153907=CARTESIAN_POINT('Origin',(10.1,-1.34711147906209E-16,-2.71)) ;
#153908=CARTESIAN_POINT('Origin',(10.2,0.,-3.81)) ;
#153909=CARTESIAN_POINT('Origin',(-7.29372370581158E-16,3.55,-3.81)) ;
#153910=CARTESIAN_POINT('',(-0.17080731546663,3.55,-2.31975677791071)) ;
#153911=CARTESIAN_POINT('',(1.5,3.55,-3.81)) ;
#153912=CARTESIAN_POINT('Origin',(-7.29372370581158E-16,3.55,-3.81)) ;
#153913=CARTESIAN_POINT('',(-0.273932138433073,3.45,-2.3352250396981)) ;
#153914=CARTESIAN_POINT('Ctrl Pts',(-0.170807315466632,3.55,-2.31975677791071)) ;
#153915=CARTESIAN_POINT('Ctrl Pts',(-0.18388243342709,3.55,-2.32125540965426)) ;
#153916=CARTESIAN_POINT('Ctrl Pts',(-0.197859036177013,3.54752250383109,
-2.32305117609769)) ;
#153917=CARTESIAN_POINT('Ctrl Pts',(-0.223597793566256,3.53719045839678,
-2.32670064673137)) ;
#153918=CARTESIAN_POINT('Ctrl Pts',(-0.235362682979178,3.52934133421403,
-2.32855041868906)) ;
#153919=CARTESIAN_POINT('Ctrl Pts',(-0.253465441530115,3.51138121637726,
-2.33154294802378)) ;
#153920=CARTESIAN_POINT('Ctrl Pts',(-0.261168570620306,3.50026979217228,
-2.3329034821853)) ;
#153921=CARTESIAN_POINT('Ctrl Pts',(-0.271399896344097,3.47583586070553,
-2.33474636459954)) ;
#153922=CARTESIAN_POINT('Ctrl Pts',(-0.273932138433075,3.46251477070021,
-2.3352250396981)) ;
#153923=CARTESIAN_POINT('Ctrl Pts',(-0.273932138433075,3.45,-2.3352250396981)) ;
#153924=CARTESIAN_POINT('',(-0.273932138433073,3.15,-2.3352250396981)) ;
#153925=CARTESIAN_POINT('',(-0.273932138433073,3.05,-2.3352250396981)) ;
#153926=CARTESIAN_POINT('',(-0.373948193368569,3.05,-2.35736007604211)) ;
#153927=CARTESIAN_POINT('Ctrl Pts',(-0.273932138433074,3.15,-2.33522503969809)) ;
#153928=CARTESIAN_POINT('Ctrl Pts',(-0.273932138433074,3.13744372549049,
-2.33522503969809)) ;
#153929=CARTESIAN_POINT('Ctrl Pts',(-0.276486468486165,3.12408297110069,
-2.33569113023559)) ;
#153930=CARTESIAN_POINT('Ctrl Pts',(-0.28674027764043,3.0995678553947,-2.33765377899357)) ;
#153931=CARTESIAN_POINT('Ctrl Pts',(-0.294439768310518,3.08841385970397,
-2.33915484113775)) ;
#153932=CARTESIAN_POINT('Ctrl Pts',(-0.312194128344973,3.07061084469361,
-2.34281939995099)) ;
#153933=CARTESIAN_POINT('Ctrl Pts',(-0.323517908844218,3.0628422827531,
-2.3452474862748)) ;
#153934=CARTESIAN_POINT('Ctrl Pts',(-0.348172117123306,3.05253676672645,
-2.35091383875347)) ;
#153935=CARTESIAN_POINT('Ctrl Pts',(-0.361501722536398,3.05,-2.35415602305916)) ;
#153936=CARTESIAN_POINT('Ctrl Pts',(-0.37394819336857,3.05,-2.35736007604211)) ;
#153937=CARTESIAN_POINT('',(-0.872417476238727,3.05,-2.58980011999949)) ;
#153938=CARTESIAN_POINT('Origin',(-7.95081593156037E-16,3.05,-3.81)) ;
#153939=CARTESIAN_POINT('',(-0.953662978710562,3.15,-2.65218873600362)) ;
#153940=CARTESIAN_POINT('Ctrl Pts',(-0.872417476238727,3.05,-2.58980011999949)) ;
#153941=CARTESIAN_POINT('Ctrl Pts',(-0.882808783297377,3.05,-2.59722968791498)) ;
#153942=CARTESIAN_POINT('Ctrl Pts',(-0.893798224191975,3.05250629897269,
-2.60530936231458)) ;
#153943=CARTESIAN_POINT('Ctrl Pts',(-0.913892243159219,3.06269675232156,
-2.62047776912462)) ;
#153944=CARTESIAN_POINT('Ctrl Pts',(-0.922999225059833,3.07038074042647,
-2.62756342856912)) ;
#153945=CARTESIAN_POINT('Ctrl Pts',(-0.937285134131706,3.08810056349785,
-2.63885587110341)) ;
#153946=CARTESIAN_POINT('Ctrl Pts',(-0.943452174397235,3.09929464195085,
-2.64384309680397)) ;
#153947=CARTESIAN_POINT('Ctrl Pts',(-0.951639309815362,3.12392729225934,
-2.65051099979639)) ;
#153948=CARTESIAN_POINT('Ctrl Pts',(-0.953662978710562,3.13736547222678,
-2.65218873600362)) ;
#153949=CARTESIAN_POINT('Ctrl Pts',(-0.953662978710562,3.15,-2.65218873600362)) ;
#153950=CARTESIAN_POINT('',(-0.953662978710562,3.45,-2.65218873600362)) ;
#153951=CARTESIAN_POINT('',(-0.953662978710562,3.05,-2.65218873600362)) ;
#153952=CARTESIAN_POINT('',(-1.03179971315145,3.55,-2.72124412656437)) ;
#153953=CARTESIAN_POINT('Ctrl Pts',(-0.953662978710565,3.45,-2.65218873600362)) ;
#153954=CARTESIAN_POINT('Ctrl Pts',(-0.953662978710565,3.45580715149871,
-2.65218873600362)) ;
#153955=CARTESIAN_POINT('Ctrl Pts',(-0.954069792639904,3.46165880969181,
-2.65252363156927)) ;
#153956=CARTESIAN_POINT('Ctrl Pts',(-0.954880405808389,3.46741264967889,
-2.65319273207538)) ;
#153957=CARTESIAN_POINT('Ctrl Pts',(-0.955592557016219,3.47246759358526,
-2.65378055960165)) ;
#153958=CARTESIAN_POINT('Ctrl Pts',(-0.956615573654934,3.47744631522377,
-2.65462581144883)) ;
#153959=CARTESIAN_POINT('Ctrl Pts',(-0.957920385817347,3.48225893605767,
-2.65570864404338)) ;
#153960=CARTESIAN_POINT('Ctrl Pts',(-0.959423079246192,3.48780141482277,
-2.65695569359675)) ;
#153961=CARTESIAN_POINT('Ctrl Pts',(-0.961323201468143,3.49320783601914,
-2.65853745938163)) ;
#153962=CARTESIAN_POINT('Ctrl Pts',(-0.963574238618811,3.49834560049868,
-2.66042425789638)) ;
#153963=CARTESIAN_POINT('Ctrl Pts',(-0.965499706648001,3.50274028640776,
-2.66203816738543)) ;
#153964=CARTESIAN_POINT('Ctrl Pts',(-0.967680912999541,3.5069382066956,
-2.66387459445843)) ;
#153965=CARTESIAN_POINT('Ctrl Pts',(-0.970068248378239,3.51087311165944,
-2.66589878354725)) ;
#153966=CARTESIAN_POINT('Ctrl Pts',(-0.972933246979055,3.51559532091263,
-2.66832797676366)) ;
#153967=CARTESIAN_POINT('Ctrl Pts',(-0.976138831290358,3.52000896466723,
-2.67106468556238)) ;
#153968=CARTESIAN_POINT('Ctrl Pts',(-0.979601776802477,3.52400782220665,
-2.67405098434758)) ;
#153969=CARTESIAN_POINT('Ctrl Pts',(-0.982467725203494,3.52731729367563,
-2.67652245789472)) ;
#153970=CARTESIAN_POINT('Ctrl Pts',(-0.985508986896834,3.53034305696182,
-2.67916417360478)) ;
#153971=CARTESIAN_POINT('Ctrl Pts',(-0.988666612105885,3.53304718478134,
-2.68193159333883)) ;
#153972=CARTESIAN_POINT('Ctrl Pts',(-0.992701606803651,3.53650267449006,
-2.68546796108803)) ;
#153973=CARTESIAN_POINT('Ctrl Pts',(-0.996988044734313,3.53948417067186,
-2.68926358811777)) ;
#153974=CARTESIAN_POINT('Ctrl Pts',(-1.00141585135915,3.54192188246042,
-2.69323403520351)) ;
#153975=CARTESIAN_POINT('Ctrl Pts',(-1.00487400994927,3.54382575827888,
-2.69633499169497)) ;
#153976=CARTESIAN_POINT('Ctrl Pts',(-1.00841776012225,3.54539884758397,
-2.69954196087253)) ;
#153977=CARTESIAN_POINT('Ctrl Pts',(-1.01199129263161,3.54662946216441,
-2.70280822634667)) ;
#153978=CARTESIAN_POINT('Ctrl Pts',(-1.016523626954,3.54819025857131,-2.70695085190716)) ;
#153979=CARTESIAN_POINT('Ctrl Pts',(-1.02116533136121,3.54921942038456,
-2.71124536311626)) ;
#153980=CARTESIAN_POINT('Ctrl Pts',(-1.02580209629924,3.54969340754028,
-2.71559145717195)) ;
#153981=CARTESIAN_POINT('Ctrl Pts',(-1.02780524115376,3.54989817637043,
-2.71746902829346)) ;
#153982=CARTESIAN_POINT('Ctrl Pts',(-1.02980744674852,3.55,-2.71935608172969)) ;
#153983=CARTESIAN_POINT('Ctrl Pts',(-1.03179971315145,3.55,-2.72124412656437)) ;
#153984=CARTESIAN_POINT('',(0.170807315466631,3.55,-5.30024322208929)) ;
#153985=CARTESIAN_POINT('Origin',(-7.29372370581158E-16,3.55,-3.81)) ;
#153986=CARTESIAN_POINT('',(0.273932138433074,3.45,-5.2847749603019)) ;
#153987=CARTESIAN_POINT('Ctrl Pts',(0.170807315466627,3.55,-5.30024322208929)) ;
#153988=CARTESIAN_POINT('Ctrl Pts',(0.183882433427085,3.55,-5.29874459034574)) ;
#153989=CARTESIAN_POINT('Ctrl Pts',(0.197859036177008,3.54752250383109,
-5.29694882390231)) ;
#153990=CARTESIAN_POINT('Ctrl Pts',(0.223597793566251,3.53719045839678,
-5.29329935326863)) ;
#153991=CARTESIAN_POINT('Ctrl Pts',(0.235362682979173,3.52934133421403,
-5.29144958131094)) ;
#153992=CARTESIAN_POINT('Ctrl Pts',(0.25346544153011,3.51138121637726,-5.28845705197622)) ;
#153993=CARTESIAN_POINT('Ctrl Pts',(0.261168570620301,3.50026979217228,
-5.2870965178147)) ;
#153994=CARTESIAN_POINT('Ctrl Pts',(0.271399896344092,3.47583586070552,
-5.28525363540046)) ;
#153995=CARTESIAN_POINT('Ctrl Pts',(0.27393213843307,3.46251477070021,-5.28477496030191)) ;
#153996=CARTESIAN_POINT('Ctrl Pts',(0.27393213843307,3.45,-5.28477496030191)) ;
#153997=CARTESIAN_POINT('',(0.273932138433074,3.15,-5.2847749603019)) ;
#153998=CARTESIAN_POINT('',(0.273932138433074,3.05,-5.2847749603019)) ;
#153999=CARTESIAN_POINT('',(0.37394819336857,3.05,-5.26263992395789)) ;
#154000=CARTESIAN_POINT('Ctrl Pts',(0.273932138433074,3.15,-5.2847749603019)) ;
#154001=CARTESIAN_POINT('Ctrl Pts',(0.273932138433074,3.13736547222678,
-5.2847749603019)) ;
#154002=CARTESIAN_POINT('Ctrl Pts',(0.276518148223581,3.12392729225934,
-5.28430316803635)) ;
#154003=CARTESIAN_POINT('Ctrl Pts',(0.28688864746378,3.09929464195085,-5.28231750387035)) ;
#154004=CARTESIAN_POINT('Ctrl Pts',(0.294673181069391,3.08810056349785,
-5.28079900383148)) ;
#154005=CARTESIAN_POINT('Ctrl Pts',(0.312506499266534,3.07038074042647,
-5.27711400471621)) ;
#154006=CARTESIAN_POINT('Ctrl Pts',(0.323788284437181,3.06269675232156,
-5.27469222593504)) ;
#154007=CARTESIAN_POINT('Ctrl Pts',(0.348324144605931,3.05250629897269,
-5.26904937832144)) ;
#154008=CARTESIAN_POINT('Ctrl Pts',(0.36157741072639,3.05,-5.26582449278551)) ;
#154009=CARTESIAN_POINT('Ctrl Pts',(0.37394819336857,3.05,-5.26263992395789)) ;
#154010=CARTESIAN_POINT('',(0.872417476238728,3.05,-5.03019988000051)) ;
#154011=CARTESIAN_POINT('Origin',(-7.95081593156037E-16,3.05,-3.81)) ;
#154012=CARTESIAN_POINT('',(0.953662978710562,3.15,-4.96781126399638)) ;
#154013=CARTESIAN_POINT('Ctrl Pts',(0.872417476238727,3.05,-5.03019988000051)) ;
#154014=CARTESIAN_POINT('Ctrl Pts',(0.882872360457018,3.05,-5.0227248557413)) ;
#154015=CARTESIAN_POINT('Ctrl Pts',(0.893924122929505,3.05253676672645,
-5.01459782148564)) ;
#154016=CARTESIAN_POINT('Ctrl Pts',(0.914112220366976,3.0628422827531,-4.99935386339936)) ;
#154017=CARTESIAN_POINT('Ctrl Pts',(0.923251028202469,3.07061084469361,
-4.99224008807701)) ;
#154018=CARTESIAN_POINT('Ctrl Pts',(0.937470525765898,3.08841385970397,
-4.9809949922316)) ;
#154019=CARTESIAN_POINT('Ctrl Pts',(0.943569543283849,3.0995678553947,-4.97606170433658)) ;
#154020=CARTESIAN_POINT('Ctrl Pts',(0.951664040935142,3.12408297110069,
-4.96946839711695)) ;
#154021=CARTESIAN_POINT('Ctrl Pts',(0.953662978710561,3.13744372549049,
-4.96781126399638)) ;
#154022=CARTESIAN_POINT('Ctrl Pts',(0.953662978710561,3.15,-4.96781126399638)) ;
#154023=CARTESIAN_POINT('',(0.953662978710562,3.45,-4.96781126399638)) ;
#154024=CARTESIAN_POINT('',(0.953662978710562,3.05,-4.96781126399638)) ;
#154025=CARTESIAN_POINT('',(1.03179971315145,3.55,-4.89875587343563)) ;
#154026=CARTESIAN_POINT('Ctrl Pts',(0.95366297871056,3.45,-4.96781126399638)) ;
#154027=CARTESIAN_POINT('Ctrl Pts',(0.95366297871056,3.45580715149871,-4.96781126399638)) ;
#154028=CARTESIAN_POINT('Ctrl Pts',(0.9540697926399,3.46165880969182,-4.96747636843074)) ;
#154029=CARTESIAN_POINT('Ctrl Pts',(0.954880405808386,3.46741264967889,
-4.96680726792462)) ;
#154030=CARTESIAN_POINT('Ctrl Pts',(0.955592557016217,3.47246759358527,
-4.96621944039835)) ;
#154031=CARTESIAN_POINT('Ctrl Pts',(0.95661557365493,3.47744631522378,-4.96537418855118)) ;
#154032=CARTESIAN_POINT('Ctrl Pts',(0.957920385817345,3.48225893605768,
-4.96429135595663)) ;
#154033=CARTESIAN_POINT('Ctrl Pts',(0.959423079246193,3.48780141482279,
-4.96304430640326)) ;
#154034=CARTESIAN_POINT('Ctrl Pts',(0.961323201468142,3.49320783601915,
-4.96146254061837)) ;
#154035=CARTESIAN_POINT('Ctrl Pts',(0.963574238618813,3.49834560049869,
-4.95957574210361)) ;
#154036=CARTESIAN_POINT('Ctrl Pts',(0.965499706648002,3.50274028640777,
-4.95796183261456)) ;
#154037=CARTESIAN_POINT('Ctrl Pts',(0.967680912999539,3.5069382066956,-4.95612540554157)) ;
#154038=CARTESIAN_POINT('Ctrl Pts',(0.970068248378239,3.51087311165944,
-4.95410121645275)) ;
#154039=CARTESIAN_POINT('Ctrl Pts',(0.972933246979058,3.51559532091264,
-4.95167202323633)) ;
#154040=CARTESIAN_POINT('Ctrl Pts',(0.976138831290365,3.52000896466724,
-4.94893531443762)) ;
#154041=CARTESIAN_POINT('Ctrl Pts',(0.979601776802482,3.52400782220666,
-4.94594901565242)) ;
#154042=CARTESIAN_POINT('Ctrl Pts',(0.982467725203495,3.52731729367563,
-4.94347754210529)) ;
#154043=CARTESIAN_POINT('Ctrl Pts',(0.985508986896837,3.53034305696182,
-4.94083582639522)) ;
#154044=CARTESIAN_POINT('Ctrl Pts',(0.988666612105885,3.53304718478134,
-4.93806840666118)) ;
#154045=CARTESIAN_POINT('Ctrl Pts',(0.992701606803651,3.53650267449006,
-4.93453203891197)) ;
#154046=CARTESIAN_POINT('Ctrl Pts',(0.996988044734314,3.53948417067186,
-4.93073641188224)) ;
#154047=CARTESIAN_POINT('Ctrl Pts',(1.00141585135915,3.54192188246042,-4.92676596479649)) ;
#154048=CARTESIAN_POINT('Ctrl Pts',(1.00487400994927,3.54382575827888,-4.92366500830503)) ;
#154049=CARTESIAN_POINT('Ctrl Pts',(1.00841776012226,3.54539884758397,-4.92045803912747)) ;
#154050=CARTESIAN_POINT('Ctrl Pts',(1.01199129263161,3.54662946216441,-4.91719177365334)) ;
#154051=CARTESIAN_POINT('Ctrl Pts',(1.016523626954,3.54819025857131,-4.91304914809286)) ;
#154052=CARTESIAN_POINT('Ctrl Pts',(1.02116533136121,3.54921942038456,-4.90875463688374)) ;
#154053=CARTESIAN_POINT('Ctrl Pts',(1.02580209629923,3.54969340754028,-4.90440854282806)) ;
#154054=CARTESIAN_POINT('Ctrl Pts',(1.02780524115375,3.54989817637043,-4.90253097170654)) ;
#154055=CARTESIAN_POINT('Ctrl Pts',(1.02980744674851,3.55,-4.90064391827031)) ;
#154056=CARTESIAN_POINT('Ctrl Pts',(1.03179971315145,3.55,-4.89875587343563)) ;
#154057=CARTESIAN_POINT('Origin',(-7.29372370581158E-16,3.55,-3.81)) ;
#154058=CARTESIAN_POINT('',(1.5,3.55,-3.81)) ;
#154059=CARTESIAN_POINT('Origin',(-7.29372370581158E-16,3.55,-7.62)) ;
#154060=CARTESIAN_POINT('',(-0.170807315466631,3.55,-6.12975677791071)) ;
#154061=CARTESIAN_POINT('',(1.5,3.55,-7.62)) ;
#154062=CARTESIAN_POINT('Origin',(-7.29372370581158E-16,3.55,-7.62)) ;
#154063=CARTESIAN_POINT('',(-0.273932138433073,3.45,-6.1452250396981)) ;
#154064=CARTESIAN_POINT('Ctrl Pts',(-0.170807315466633,3.55,-6.1297567779107)) ;
#154065=CARTESIAN_POINT('Ctrl Pts',(-0.18388243342709,3.55,-6.13125540965426)) ;
#154066=CARTESIAN_POINT('Ctrl Pts',(-0.197859036177013,3.54752250383109,
-6.13305117609769)) ;
#154067=CARTESIAN_POINT('Ctrl Pts',(-0.223597793566256,3.53719045839678,
-6.13670064673137)) ;
#154068=CARTESIAN_POINT('Ctrl Pts',(-0.235362682979179,3.52934133421403,
-6.13855041868906)) ;
#154069=CARTESIAN_POINT('Ctrl Pts',(-0.253465441530116,3.51138121637726,
-6.14154294802378)) ;
#154070=CARTESIAN_POINT('Ctrl Pts',(-0.261168570620306,3.50026979217228,
-6.1429034821853)) ;
#154071=CARTESIAN_POINT('Ctrl Pts',(-0.271399896344097,3.47583586070553,
-6.14474636459954)) ;
#154072=CARTESIAN_POINT('Ctrl Pts',(-0.273932138433075,3.46251477070021,
-6.1452250396981)) ;
#154073=CARTESIAN_POINT('Ctrl Pts',(-0.273932138433075,3.45,-6.1452250396981)) ;
#154074=CARTESIAN_POINT('',(-0.273932138433073,3.15,-6.1452250396981)) ;
#154075=CARTESIAN_POINT('',(-0.273932138433073,3.05,-6.1452250396981)) ;
#154076=CARTESIAN_POINT('',(-0.373948193368569,3.05,-6.16736007604211)) ;
#154077=CARTESIAN_POINT('Ctrl Pts',(-0.273932138433075,3.15,-6.14522503969809)) ;
#154078=CARTESIAN_POINT('Ctrl Pts',(-0.273932138433075,3.13744372549049,
-6.14522503969809)) ;
#154079=CARTESIAN_POINT('Ctrl Pts',(-0.276486468486165,3.12408297110069,
-6.1456911302356)) ;
#154080=CARTESIAN_POINT('Ctrl Pts',(-0.28674027764043,3.0995678553947,-6.14765377899357)) ;
#154081=CARTESIAN_POINT('Ctrl Pts',(-0.294439768310518,3.08841385970397,
-6.14915484113775)) ;
#154082=CARTESIAN_POINT('Ctrl Pts',(-0.312194128344973,3.07061084469361,
-6.15281939995099)) ;
#154083=CARTESIAN_POINT('Ctrl Pts',(-0.323517908844218,3.0628422827531,
-6.1552474862748)) ;
#154084=CARTESIAN_POINT('Ctrl Pts',(-0.348172117123305,3.05253676672645,
-6.16091383875347)) ;
#154085=CARTESIAN_POINT('Ctrl Pts',(-0.361501722536398,3.05,-6.16415602305916)) ;
#154086=CARTESIAN_POINT('Ctrl Pts',(-0.37394819336857,3.05,-6.16736007604211)) ;
#154087=CARTESIAN_POINT('',(-0.872417476238727,3.05,-6.39980011999949)) ;
#154088=CARTESIAN_POINT('Origin',(-7.95081593156037E-16,3.05,-7.62)) ;
#154089=CARTESIAN_POINT('',(-0.953662978710562,3.15,-6.46218873600362)) ;
#154090=CARTESIAN_POINT('Ctrl Pts',(-0.872417476238727,3.05,-6.39980011999949)) ;
#154091=CARTESIAN_POINT('Ctrl Pts',(-0.882808783297377,3.05,-6.40722968791498)) ;
#154092=CARTESIAN_POINT('Ctrl Pts',(-0.893798224191975,3.05250629897269,
-6.41530936231458)) ;
#154093=CARTESIAN_POINT('Ctrl Pts',(-0.913892243159219,3.06269675232156,
-6.43047776912462)) ;
#154094=CARTESIAN_POINT('Ctrl Pts',(-0.922999225059833,3.07038074042647,
-6.43756342856912)) ;
#154095=CARTESIAN_POINT('Ctrl Pts',(-0.937285134131705,3.08810056349785,
-6.44885587110341)) ;
#154096=CARTESIAN_POINT('Ctrl Pts',(-0.943452174397235,3.09929464195085,
-6.45384309680397)) ;
#154097=CARTESIAN_POINT('Ctrl Pts',(-0.951639309815362,3.12392729225934,
-6.46051099979639)) ;
#154098=CARTESIAN_POINT('Ctrl Pts',(-0.953662978710561,3.13736547222678,
-6.46218873600362)) ;
#154099=CARTESIAN_POINT('Ctrl Pts',(-0.953662978710561,3.15,-6.46218873600362)) ;
#154100=CARTESIAN_POINT('',(-0.953662978710562,3.45,-6.46218873600362)) ;
#154101=CARTESIAN_POINT('',(-0.953662978710562,3.05,-6.46218873600362)) ;
#154102=CARTESIAN_POINT('',(-1.03179971315145,3.55,-6.53124412656437)) ;
#154103=CARTESIAN_POINT('Ctrl Pts',(-0.953662978710565,3.45,-6.46218873600362)) ;
#154104=CARTESIAN_POINT('Ctrl Pts',(-0.953662978710565,3.45580715149871,
-6.46218873600362)) ;
#154105=CARTESIAN_POINT('Ctrl Pts',(-0.954069792639906,3.46165880969183,
-6.46252363156927)) ;
#154106=CARTESIAN_POINT('Ctrl Pts',(-0.954880405808391,3.4674126496789,
-6.46319273207538)) ;
#154107=CARTESIAN_POINT('Ctrl Pts',(-0.955592557016221,3.47246759358527,
-6.46378055960165)) ;
#154108=CARTESIAN_POINT('Ctrl Pts',(-0.956615573654934,3.47744631522377,
-6.46462581144883)) ;
#154109=CARTESIAN_POINT('Ctrl Pts',(-0.957920385817348,3.48225893605767,
-6.46570864404338)) ;
#154110=CARTESIAN_POINT('Ctrl Pts',(-0.959423079246195,3.48780141482278,
-6.46695569359675)) ;
#154111=CARTESIAN_POINT('Ctrl Pts',(-0.961323201468146,3.49320783601915,
-6.46853745938164)) ;
#154112=CARTESIAN_POINT('Ctrl Pts',(-0.963574238618818,3.49834560049869,
-6.47042425789639)) ;
#154113=CARTESIAN_POINT('Ctrl Pts',(-0.965499706648006,3.50274028640777,
-6.47203816738544)) ;
#154114=CARTESIAN_POINT('Ctrl Pts',(-0.967680912999541,3.5069382066956,
-6.47387459445843)) ;
#154115=CARTESIAN_POINT('Ctrl Pts',(-0.97006824837824,3.51087311165944,
-6.47589878354725)) ;
#154116=CARTESIAN_POINT('Ctrl Pts',(-0.97293324697906,3.51559532091263,
-6.47832797676366)) ;
#154117=CARTESIAN_POINT('Ctrl Pts',(-0.976138831290367,3.52000896466724,
-6.48106468556238)) ;
#154118=CARTESIAN_POINT('Ctrl Pts',(-0.979601776802484,3.52400782220665,
-6.48405098434758)) ;
#154119=CARTESIAN_POINT('Ctrl Pts',(-0.982467725203496,3.52731729367563,
-6.48652245789472)) ;
#154120=CARTESIAN_POINT('Ctrl Pts',(-0.985508986896839,3.53034305696182,
-6.48916417360478)) ;
#154121=CARTESIAN_POINT('Ctrl Pts',(-0.988666612105887,3.53304718478134,
-6.49193159333883)) ;
#154122=CARTESIAN_POINT('Ctrl Pts',(-0.992701606803653,3.53650267449006,
-6.49546796108803)) ;
#154123=CARTESIAN_POINT('Ctrl Pts',(-0.996988044734315,3.53948417067186,
-6.49926358811777)) ;
#154124=CARTESIAN_POINT('Ctrl Pts',(-1.00141585135916,3.54192188246042,
-6.50323403520352)) ;
#154125=CARTESIAN_POINT('Ctrl Pts',(-1.00487400994927,3.54382575827888,
-6.50633499169497)) ;
#154126=CARTESIAN_POINT('Ctrl Pts',(-1.00841776012226,3.54539884758397,
-6.50954196087253)) ;
#154127=CARTESIAN_POINT('Ctrl Pts',(-1.01199129263161,3.54662946216441,
-6.51280822634666)) ;
#154128=CARTESIAN_POINT('Ctrl Pts',(-1.016523626954,3.54819025857131,-6.51695085190715)) ;
#154129=CARTESIAN_POINT('Ctrl Pts',(-1.0211653313612,3.54921942038456,-6.52124536311625)) ;
#154130=CARTESIAN_POINT('Ctrl Pts',(-1.02580209629923,3.54969340754027,
-6.52559145717194)) ;
#154131=CARTESIAN_POINT('Ctrl Pts',(-1.02780524115375,3.54989817637043,
-6.52746902829346)) ;
#154132=CARTESIAN_POINT('Ctrl Pts',(-1.02980744674852,3.55,-6.52935608172969)) ;
#154133=CARTESIAN_POINT('Ctrl Pts',(-1.03179971315145,3.55,-6.53124412656437)) ;
#154134=CARTESIAN_POINT('',(0.170807315466631,3.55,-9.11024322208929)) ;
#154135=CARTESIAN_POINT('Origin',(-7.29372370581158E-16,3.55,-7.62)) ;
#154136=CARTESIAN_POINT('',(0.273932138433074,3.45,-9.0947749603019)) ;
#154137=CARTESIAN_POINT('Ctrl Pts',(0.170807315466626,3.55,-9.1102432220893)) ;
#154138=CARTESIAN_POINT('Ctrl Pts',(0.183882433427084,3.55,-9.10874459034575)) ;
#154139=CARTESIAN_POINT('Ctrl Pts',(0.197859036177007,3.54752250383109,
-9.10694882390231)) ;
#154140=CARTESIAN_POINT('Ctrl Pts',(0.223597793566251,3.53719045839678,
-9.10329935326863)) ;
#154141=CARTESIAN_POINT('Ctrl Pts',(0.235362682979173,3.52934133421403,
-9.10144958131094)) ;
#154142=CARTESIAN_POINT('Ctrl Pts',(0.25346544153011,3.51138121637726,-9.09845705197622)) ;
#154143=CARTESIAN_POINT('Ctrl Pts',(0.2611685706203,3.50026979217228,-9.0970965178147)) ;
#154144=CARTESIAN_POINT('Ctrl Pts',(0.271399896344091,3.47583586070553,
-9.09525363540046)) ;
#154145=CARTESIAN_POINT('Ctrl Pts',(0.273932138433069,3.46251477070021,
-9.0947749603019)) ;
#154146=CARTESIAN_POINT('Ctrl Pts',(0.273932138433069,3.45,-9.0947749603019)) ;
#154147=CARTESIAN_POINT('',(0.273932138433074,3.15,-9.0947749603019)) ;
#154148=CARTESIAN_POINT('',(0.273932138433074,3.05,-9.0947749603019)) ;
#154149=CARTESIAN_POINT('',(0.37394819336857,3.05,-9.07263992395789)) ;
#154150=CARTESIAN_POINT('Ctrl Pts',(0.273932138433074,3.15,-9.0947749603019)) ;
#154151=CARTESIAN_POINT('Ctrl Pts',(0.273932138433074,3.13736547222678,
-9.0947749603019)) ;
#154152=CARTESIAN_POINT('Ctrl Pts',(0.276518148223582,3.12392729225934,
-9.09430316803635)) ;
#154153=CARTESIAN_POINT('Ctrl Pts',(0.28688864746378,3.09929464195085,-9.09231750387035)) ;
#154154=CARTESIAN_POINT('Ctrl Pts',(0.294673181069391,3.08810056349785,
-9.09079900383148)) ;
#154155=CARTESIAN_POINT('Ctrl Pts',(0.312506499266534,3.07038074042647,
-9.08711400471621)) ;
#154156=CARTESIAN_POINT('Ctrl Pts',(0.323788284437181,3.06269675232156,
-9.08469222593504)) ;
#154157=CARTESIAN_POINT('Ctrl Pts',(0.348324144605931,3.05250629897269,
-9.07904937832144)) ;
#154158=CARTESIAN_POINT('Ctrl Pts',(0.36157741072639,3.05,-9.07582449278551)) ;
#154159=CARTESIAN_POINT('Ctrl Pts',(0.37394819336857,3.05,-9.07263992395789)) ;
#154160=CARTESIAN_POINT('',(0.872417476238728,3.05,-8.84019988000051)) ;
#154161=CARTESIAN_POINT('Origin',(-7.95081593156037E-16,3.05,-7.62)) ;
#154162=CARTESIAN_POINT('',(0.953662978710562,3.15,-8.77781126399638)) ;
#154163=CARTESIAN_POINT('Ctrl Pts',(0.872417476238727,3.05,-8.84019988000051)) ;
#154164=CARTESIAN_POINT('Ctrl Pts',(0.882872360457018,3.05,-8.8327248557413)) ;
#154165=CARTESIAN_POINT('Ctrl Pts',(0.893924122929505,3.05253676672645,
-8.82459782148564)) ;
#154166=CARTESIAN_POINT('Ctrl Pts',(0.914112220366976,3.0628422827531,-8.80935386339936)) ;
#154167=CARTESIAN_POINT('Ctrl Pts',(0.923251028202469,3.07061084469361,
-8.80224008807701)) ;
#154168=CARTESIAN_POINT('Ctrl Pts',(0.937470525765898,3.08841385970397,
-8.7909949922316)) ;
#154169=CARTESIAN_POINT('Ctrl Pts',(0.943569543283849,3.0995678553947,-8.78606170433658)) ;
#154170=CARTESIAN_POINT('Ctrl Pts',(0.951664040935142,3.12408297110069,
-8.77946839711695)) ;
#154171=CARTESIAN_POINT('Ctrl Pts',(0.953662978710561,3.13744372549049,
-8.77781126399638)) ;
#154172=CARTESIAN_POINT('Ctrl Pts',(0.953662978710561,3.15,-8.77781126399638)) ;
#154173=CARTESIAN_POINT('',(0.953662978710562,3.45,-8.77781126399638)) ;
#154174=CARTESIAN_POINT('',(0.953662978710562,3.05,-8.77781126399638)) ;
#154175=CARTESIAN_POINT('',(1.03179971315145,3.55,-8.70875587343563)) ;
#154176=CARTESIAN_POINT('Ctrl Pts',(0.95366297871056,3.45,-8.77781126399638)) ;
#154177=CARTESIAN_POINT('Ctrl Pts',(0.95366297871056,3.45580715149871,-8.77781126399638)) ;
#154178=CARTESIAN_POINT('Ctrl Pts',(0.9540697926399,3.46165880969182,-8.77747636843074)) ;
#154179=CARTESIAN_POINT('Ctrl Pts',(0.954880405808385,3.46741264967889,
-8.77680726792462)) ;
#154180=CARTESIAN_POINT('Ctrl Pts',(0.955592557016215,3.47246759358526,
-8.77621944039836)) ;
#154181=CARTESIAN_POINT('Ctrl Pts',(0.956615573654929,3.47744631522378,
-8.77537418855117)) ;
#154182=CARTESIAN_POINT('Ctrl Pts',(0.957920385817344,3.48225893605768,
-8.77429135595662)) ;
#154183=CARTESIAN_POINT('Ctrl Pts',(0.959423079246191,3.48780141482278,
-8.77304430640325)) ;
#154184=CARTESIAN_POINT('Ctrl Pts',(0.961323201468144,3.49320783601915,
-8.77146254061837)) ;
#154185=CARTESIAN_POINT('Ctrl Pts',(0.963574238618813,3.49834560049869,
-8.76957574210362)) ;
#154186=CARTESIAN_POINT('Ctrl Pts',(0.965499706648001,3.50274028640777,
-8.76796183261456)) ;
#154187=CARTESIAN_POINT('Ctrl Pts',(0.967680912999538,3.5069382066956,-8.76612540554157)) ;
#154188=CARTESIAN_POINT('Ctrl Pts',(0.970068248378235,3.51087311165944,
-8.76410121645275)) ;
#154189=CARTESIAN_POINT('Ctrl Pts',(0.972933246979052,3.51559532091263,
-8.76167202323634)) ;
#154190=CARTESIAN_POINT('Ctrl Pts',(0.976138831290364,3.52000896466724,
-8.75893531443762)) ;
#154191=CARTESIAN_POINT('Ctrl Pts',(0.97960177680248,3.52400782220665,-8.75594901565243)) ;
#154192=CARTESIAN_POINT('Ctrl Pts',(0.982467725203493,3.52731729367563,
-8.75347754210529)) ;
#154193=CARTESIAN_POINT('Ctrl Pts',(0.985508986896836,3.53034305696182,
-8.75083582639522)) ;
#154194=CARTESIAN_POINT('Ctrl Pts',(0.988666612105887,3.53304718478134,
-8.74806840666118)) ;
#154195=CARTESIAN_POINT('Ctrl Pts',(0.99270160680366,3.53650267449007,-8.74453203891197)) ;
#154196=CARTESIAN_POINT('Ctrl Pts',(0.996988044734325,3.53948417067186,
-8.74073641188223)) ;
#154197=CARTESIAN_POINT('Ctrl Pts',(1.00141585135916,3.54192188246042,-8.73676596479647)) ;
#154198=CARTESIAN_POINT('Ctrl Pts',(1.00487400994927,3.54382575827888,-8.73366500830502)) ;
#154199=CARTESIAN_POINT('Ctrl Pts',(1.00841776012226,3.54539884758398,-8.73045803912746)) ;
#154200=CARTESIAN_POINT('Ctrl Pts',(1.01199129263161,3.54662946216441,-8.72719177365333)) ;
#154201=CARTESIAN_POINT('Ctrl Pts',(1.016523626954,3.54819025857131,-8.72304914809285)) ;
#154202=CARTESIAN_POINT('Ctrl Pts',(1.02116533136121,3.54921942038456,-8.71875463688375)) ;
#154203=CARTESIAN_POINT('Ctrl Pts',(1.02580209629923,3.54969340754028,-8.71440854282806)) ;
#154204=CARTESIAN_POINT('Ctrl Pts',(1.02780524115375,3.54989817637043,-8.71253097170654)) ;
#154205=CARTESIAN_POINT('Ctrl Pts',(1.02980744674851,3.55,-8.71064391827031)) ;
#154206=CARTESIAN_POINT('Ctrl Pts',(1.03179971315145,3.55,-8.70875587343563)) ;
#154207=CARTESIAN_POINT('Origin',(-7.29372370581158E-16,3.55,-7.62)) ;
#154208=CARTESIAN_POINT('',(1.5,3.55,-7.62)) ;
#154209=CARTESIAN_POINT('Origin',(-7.29372370581158E-16,3.55,-11.43)) ;
#154210=CARTESIAN_POINT('',(-0.17080731546663,3.55,-9.9397567779107)) ;
#154211=CARTESIAN_POINT('',(1.5,3.55,-11.43)) ;
#154212=CARTESIAN_POINT('Origin',(-7.29372370581158E-16,3.55,-11.43)) ;
#154213=CARTESIAN_POINT('',(-0.273932138433073,3.45,-9.9552250396981)) ;
#154214=CARTESIAN_POINT('Ctrl Pts',(-0.170807315466628,3.55,-9.9397567779107)) ;
#154215=CARTESIAN_POINT('Ctrl Pts',(-0.183882433427086,3.55,-9.94125540965426)) ;
#154216=CARTESIAN_POINT('Ctrl Pts',(-0.197859036177008,3.54752250383109,
-9.94305117609769)) ;
#154217=CARTESIAN_POINT('Ctrl Pts',(-0.223597793566252,3.53719045839678,
-9.94670064673137)) ;
#154218=CARTESIAN_POINT('Ctrl Pts',(-0.235362682979173,3.52934133421403,
-9.94855041868906)) ;
#154219=CARTESIAN_POINT('Ctrl Pts',(-0.25346544153011,3.51138121637726,
-9.95154294802378)) ;
#154220=CARTESIAN_POINT('Ctrl Pts',(-0.261168570620301,3.50026979217228,
-9.9529034821853)) ;
#154221=CARTESIAN_POINT('Ctrl Pts',(-0.271399896344092,3.47583586070553,
-9.95474636459954)) ;
#154222=CARTESIAN_POINT('Ctrl Pts',(-0.27393213843307,3.46251477070021,
-9.95522503969809)) ;
#154223=CARTESIAN_POINT('Ctrl Pts',(-0.27393213843307,3.45,-9.95522503969809)) ;
#154224=CARTESIAN_POINT('',(-0.273932138433073,3.15,-9.9552250396981)) ;
#154225=CARTESIAN_POINT('',(-0.273932138433073,3.05,-9.9552250396981)) ;
#154226=CARTESIAN_POINT('',(-0.373948193368569,3.05,-9.97736007604211)) ;
#154227=CARTESIAN_POINT('Ctrl Pts',(-0.27393213843307,3.15,-9.95522503969809)) ;
#154228=CARTESIAN_POINT('Ctrl Pts',(-0.27393213843307,3.13744372549049,
-9.95522503969809)) ;
#154229=CARTESIAN_POINT('Ctrl Pts',(-0.276486468486161,3.12408297110069,
-9.9556911302356)) ;
#154230=CARTESIAN_POINT('Ctrl Pts',(-0.286740277640426,3.0995678553947,
-9.95765377899357)) ;
#154231=CARTESIAN_POINT('Ctrl Pts',(-0.294439768310514,3.08841385970397,
-9.95915484113775)) ;
#154232=CARTESIAN_POINT('Ctrl Pts',(-0.312194128344968,3.07061084469361,
-9.96281939995099)) ;
#154233=CARTESIAN_POINT('Ctrl Pts',(-0.323517908844214,3.0628422827531,
-9.9652474862748)) ;
#154234=CARTESIAN_POINT('Ctrl Pts',(-0.348172117123301,3.05253676672645,
-9.97091383875347)) ;
#154235=CARTESIAN_POINT('Ctrl Pts',(-0.361501722536394,3.05,-9.97415602305916)) ;
#154236=CARTESIAN_POINT('Ctrl Pts',(-0.373948193368566,3.05,-9.97736007604211)) ;
#154237=CARTESIAN_POINT('',(-0.872417476238727,3.05,-10.2098001199995)) ;
#154238=CARTESIAN_POINT('Origin',(-7.95081593156037E-16,3.05,-11.43)) ;
#154239=CARTESIAN_POINT('',(-0.953662978710562,3.15,-10.2721887360036)) ;
#154240=CARTESIAN_POINT('Ctrl Pts',(-0.872417476238731,3.05,-10.2098001199995)) ;
#154241=CARTESIAN_POINT('Ctrl Pts',(-0.882808783297381,3.05,-10.217229687915)) ;
#154242=CARTESIAN_POINT('Ctrl Pts',(-0.893798224191977,3.05250629897269,
-10.2253093623146)) ;
#154243=CARTESIAN_POINT('Ctrl Pts',(-0.913892243159222,3.06269675232156,
-10.2404777691246)) ;
#154244=CARTESIAN_POINT('Ctrl Pts',(-0.922999225059836,3.07038074042647,
-10.2475634285691)) ;
#154245=CARTESIAN_POINT('Ctrl Pts',(-0.937285134131709,3.08810056349785,
-10.2588558711034)) ;
#154246=CARTESIAN_POINT('Ctrl Pts',(-0.943452174397238,3.09929464195085,
-10.263843096804)) ;
#154247=CARTESIAN_POINT('Ctrl Pts',(-0.951639309815365,3.12392729225934,
-10.2705109997964)) ;
#154248=CARTESIAN_POINT('Ctrl Pts',(-0.953662978710564,3.13736547222678,
-10.2721887360036)) ;
#154249=CARTESIAN_POINT('Ctrl Pts',(-0.953662978710564,3.15,-10.2721887360036)) ;
#154250=CARTESIAN_POINT('',(-0.953662978710562,3.45,-10.2721887360036)) ;
#154251=CARTESIAN_POINT('',(-0.953662978710562,3.05,-10.2721887360036)) ;
#154252=CARTESIAN_POINT('',(-1.03179971315145,3.55,-10.3412441265644)) ;
#154253=CARTESIAN_POINT('Ctrl Pts',(-0.953662978710575,3.45,-10.2721887360036)) ;
#154254=CARTESIAN_POINT('Ctrl Pts',(-0.953662978710575,3.45580715149871,
-10.2721887360036)) ;
#154255=CARTESIAN_POINT('Ctrl Pts',(-0.954069792639919,3.46165880969182,
-10.2725236315692)) ;
#154256=CARTESIAN_POINT('Ctrl Pts',(-0.95488040580839,3.4674126496789,-10.2731927320754)) ;
#154257=CARTESIAN_POINT('Ctrl Pts',(-0.955592557016208,3.47246759358527,
-10.2737805596017)) ;
#154258=CARTESIAN_POINT('Ctrl Pts',(-0.956615573654938,3.47744631522378,
-10.2746258114488)) ;
#154259=CARTESIAN_POINT('Ctrl Pts',(-0.957920385817356,3.48225893605768,
-10.2757086440434)) ;
#154260=CARTESIAN_POINT('Ctrl Pts',(-0.959423079246207,3.48780141482279,
-10.2769556935967)) ;
#154261=CARTESIAN_POINT('Ctrl Pts',(-0.961323201468137,3.49320783601914,
-10.2785374593817)) ;
#154262=CARTESIAN_POINT('Ctrl Pts',(-0.963574238618807,3.49834560049868,
-10.2804242578964)) ;
#154263=CARTESIAN_POINT('Ctrl Pts',(-0.965499706647995,3.50274028640776,
-10.2820381673855)) ;
#154264=CARTESIAN_POINT('Ctrl Pts',(-0.96768091299954,3.50693820669559,
-10.2838745944584)) ;
#154265=CARTESIAN_POINT('Ctrl Pts',(-0.970068248378245,3.51087311165943,
-10.2858987835472)) ;
#154266=CARTESIAN_POINT('Ctrl Pts',(-0.972933246979072,3.51559532091262,
-10.2883279767636)) ;
#154267=CARTESIAN_POINT('Ctrl Pts',(-0.97613883129036,3.52000896466724,
-10.2910646855624)) ;
#154268=CARTESIAN_POINT('Ctrl Pts',(-0.979601776802481,3.52400782220665,
-10.2940509843476)) ;
#154269=CARTESIAN_POINT('Ctrl Pts',(-0.982467725203496,3.52731729367563,
-10.2965224578947)) ;
#154270=CARTESIAN_POINT('Ctrl Pts',(-0.985508986896836,3.5303430569618,
-10.2991641736047)) ;
#154271=CARTESIAN_POINT('Ctrl Pts',(-0.988666612105891,3.53304718478134,
-10.3019315933388)) ;
#154272=CARTESIAN_POINT('Ctrl Pts',(-0.992701606803668,3.53650267449007,
-10.3054679610881)) ;
#154273=CARTESIAN_POINT('Ctrl Pts',(-0.996988044734306,3.53948417067184,
-10.3092635881177)) ;
#154274=CARTESIAN_POINT('Ctrl Pts',(-1.00141585135915,3.54192188246041,
-10.3132340352035)) ;
#154275=CARTESIAN_POINT('Ctrl Pts',(-1.00487400994927,3.54382575827887,
-10.3163349916949)) ;
#154276=CARTESIAN_POINT('Ctrl Pts',(-1.00841776012226,3.54539884758398,
-10.3195419608726)) ;
#154277=CARTESIAN_POINT('Ctrl Pts',(-1.01199129263162,3.54662946216441,
-10.3228082263467)) ;
#154278=CARTESIAN_POINT('Ctrl Pts',(-1.01652362695402,3.54819025857132,
-10.3269508519072)) ;
#154279=CARTESIAN_POINT('Ctrl Pts',(-1.0211653313612,3.54921942038456,-10.3312453631162)) ;
#154280=CARTESIAN_POINT('Ctrl Pts',(-1.02580209629924,3.54969340754028,
-10.3355914571719)) ;
#154281=CARTESIAN_POINT('Ctrl Pts',(-1.02780524115376,3.54989817637043,
-10.3374690282934)) ;
#154282=CARTESIAN_POINT('Ctrl Pts',(-1.02980744674853,3.55,-10.3393560817297)) ;
#154283=CARTESIAN_POINT('Ctrl Pts',(-1.03179971315146,3.55,-10.3412441265644)) ;
#154284=CARTESIAN_POINT('',(0.170807315466631,3.55,-12.9202432220893)) ;
#154285=CARTESIAN_POINT('Origin',(-7.29372370581158E-16,3.55,-11.43)) ;
#154286=CARTESIAN_POINT('',(0.273932138433074,3.45,-12.9047749603019)) ;
#154287=CARTESIAN_POINT('Ctrl Pts',(0.170807315466622,3.55,-12.9202432220893)) ;
#154288=CARTESIAN_POINT('Ctrl Pts',(0.18388243342708,3.55,-12.9187445903457)) ;
#154289=CARTESIAN_POINT('Ctrl Pts',(0.197859036177003,3.54752250383109,
-12.9169488239023)) ;
#154290=CARTESIAN_POINT('Ctrl Pts',(0.223597793566246,3.53719045839678,
-12.9132993532686)) ;
#154291=CARTESIAN_POINT('Ctrl Pts',(0.235362682979168,3.52934133421403,
-12.9114495813109)) ;
#154292=CARTESIAN_POINT('Ctrl Pts',(0.253465441530105,3.51138121637726,
-12.9084570519762)) ;
#154293=CARTESIAN_POINT('Ctrl Pts',(0.261168570620296,3.50026979217228,
-12.9070965178147)) ;
#154294=CARTESIAN_POINT('Ctrl Pts',(0.271399896344087,3.47583586070553,
-12.9052536354005)) ;
#154295=CARTESIAN_POINT('Ctrl Pts',(0.273932138433065,3.46251477070021,
-12.9047749603019)) ;
#154296=CARTESIAN_POINT('Ctrl Pts',(0.273932138433065,3.45,-12.9047749603019)) ;
#154297=CARTESIAN_POINT('',(0.273932138433074,3.15,-12.9047749603019)) ;
#154298=CARTESIAN_POINT('',(0.273932138433074,3.05,-12.9047749603019)) ;
#154299=CARTESIAN_POINT('',(0.37394819336857,3.05,-12.8826399239579)) ;
#154300=CARTESIAN_POINT('Ctrl Pts',(0.27393213843307,3.15,-12.9047749603019)) ;
#154301=CARTESIAN_POINT('Ctrl Pts',(0.27393213843307,3.13736547222678,-12.9047749603019)) ;
#154302=CARTESIAN_POINT('Ctrl Pts',(0.276518148223577,3.12392729225934,
-12.9043031680364)) ;
#154303=CARTESIAN_POINT('Ctrl Pts',(0.286888647463776,3.09929464195085,
-12.9023175038704)) ;
#154304=CARTESIAN_POINT('Ctrl Pts',(0.294673181069387,3.08810056349785,
-12.9007990038315)) ;
#154305=CARTESIAN_POINT('Ctrl Pts',(0.31250649926653,3.07038074042647,-12.8971140047162)) ;
#154306=CARTESIAN_POINT('Ctrl Pts',(0.323788284437177,3.06269675232156,
-12.894692225935)) ;
#154307=CARTESIAN_POINT('Ctrl Pts',(0.348324144605927,3.05250629897269,
-12.8890493783214)) ;
#154308=CARTESIAN_POINT('Ctrl Pts',(0.361577410726386,3.05,-12.8858244927855)) ;
#154309=CARTESIAN_POINT('Ctrl Pts',(0.373948193368566,3.05,-12.8826399239579)) ;
#154310=CARTESIAN_POINT('',(0.872417476238727,3.05,-12.6501998800005)) ;
#154311=CARTESIAN_POINT('Origin',(-7.95081593156037E-16,3.05,-11.43)) ;
#154312=CARTESIAN_POINT('',(0.953662978710562,3.15,-12.5878112639964)) ;
#154313=CARTESIAN_POINT('Ctrl Pts',(0.87241747623873,3.05,-12.6501998800005)) ;
#154314=CARTESIAN_POINT('Ctrl Pts',(0.882872360457021,3.05,-12.6427248557413)) ;
#154315=CARTESIAN_POINT('Ctrl Pts',(0.893924122929508,3.05253676672645,
-12.6345978214856)) ;
#154316=CARTESIAN_POINT('Ctrl Pts',(0.914112220366979,3.0628422827531,-12.6193538633994)) ;
#154317=CARTESIAN_POINT('Ctrl Pts',(0.923251028202472,3.07061084469361,
-12.612240088077)) ;
#154318=CARTESIAN_POINT('Ctrl Pts',(0.937470525765901,3.08841385970397,
-12.6009949922316)) ;
#154319=CARTESIAN_POINT('Ctrl Pts',(0.943569543283853,3.0995678553947,-12.5960617043366)) ;
#154320=CARTESIAN_POINT('Ctrl Pts',(0.951664040935146,3.12408297110069,
-12.5894683971169)) ;
#154321=CARTESIAN_POINT('Ctrl Pts',(0.953662978710565,3.13744372549049,
-12.5878112639964)) ;
#154322=CARTESIAN_POINT('Ctrl Pts',(0.953662978710565,3.15,-12.5878112639964)) ;
#154323=CARTESIAN_POINT('',(0.953662978710562,3.45,-12.5878112639964)) ;
#154324=CARTESIAN_POINT('',(0.953662978710562,3.05,-12.5878112639964)) ;
#154325=CARTESIAN_POINT('',(1.03179971315145,3.55,-12.5187558734356)) ;
#154326=CARTESIAN_POINT('Ctrl Pts',(0.95366297871057,3.45,-12.5878112639964)) ;
#154327=CARTESIAN_POINT('Ctrl Pts',(0.95366297871057,3.45580715149871,-12.5878112639964)) ;
#154328=CARTESIAN_POINT('Ctrl Pts',(0.954069792639914,3.46165880969181,
-12.5874763684308)) ;
#154329=CARTESIAN_POINT('Ctrl Pts',(0.954880405808384,3.46741264967889,
-12.5868072679246)) ;
#154330=CARTESIAN_POINT('Ctrl Pts',(0.955592557016202,3.47246759358526,
-12.5862194403983)) ;
#154331=CARTESIAN_POINT('Ctrl Pts',(0.956615573654934,3.47744631522378,
-12.5853741885512)) ;
#154332=CARTESIAN_POINT('Ctrl Pts',(0.957920385817353,3.48225893605768,
-12.5842913559566)) ;
#154333=CARTESIAN_POINT('Ctrl Pts',(0.959423079246204,3.48780141482279,
-12.5830443064033)) ;
#154334=CARTESIAN_POINT('Ctrl Pts',(0.961323201468133,3.49320783601914,
-12.5814625406183)) ;
#154335=CARTESIAN_POINT('Ctrl Pts',(0.963574238618804,3.49834560049868,
-12.5795757421036)) ;
#154336=CARTESIAN_POINT('Ctrl Pts',(0.965499706647994,3.50274028640776,
-12.5779618326145)) ;
#154337=CARTESIAN_POINT('Ctrl Pts',(0.967680912999537,3.5069382066956,-12.5761254055416)) ;
#154338=CARTESIAN_POINT('Ctrl Pts',(0.970068248378243,3.51087311165944,
-12.5741012164528)) ;
#154339=CARTESIAN_POINT('Ctrl Pts',(0.972933246979071,3.51559532091263,
-12.5716720232364)) ;
#154340=CARTESIAN_POINT('Ctrl Pts',(0.97613883129036,3.52000896466724,-12.5689353144376)) ;
#154341=CARTESIAN_POINT('Ctrl Pts',(0.979601776802481,3.52400782220666,
-12.5659490156524)) ;
#154342=CARTESIAN_POINT('Ctrl Pts',(0.982467725203496,3.52731729367563,
-12.5634775421053)) ;
#154343=CARTESIAN_POINT('Ctrl Pts',(0.985508986896835,3.5303430569618,-12.5608358263953)) ;
#154344=CARTESIAN_POINT('Ctrl Pts',(0.988666612105891,3.53304718478134,
-12.5580684066612)) ;
#154345=CARTESIAN_POINT('Ctrl Pts',(0.992701606803667,3.53650267449007,
-12.554532038912)) ;
#154346=CARTESIAN_POINT('Ctrl Pts',(0.996988044734304,3.53948417067185,
-12.5507364118823)) ;
#154347=CARTESIAN_POINT('Ctrl Pts',(1.00141585135915,3.54192188246041,-12.5467659647965)) ;
#154348=CARTESIAN_POINT('Ctrl Pts',(1.00487400994927,3.54382575827887,-12.5436650083051)) ;
#154349=CARTESIAN_POINT('Ctrl Pts',(1.00841776012225,3.54539884758398,-12.5404580391274)) ;
#154350=CARTESIAN_POINT('Ctrl Pts',(1.01199129263162,3.54662946216441,-12.5371917736533)) ;
#154351=CARTESIAN_POINT('Ctrl Pts',(1.01652362695402,3.54819025857132,-12.5330491480928)) ;
#154352=CARTESIAN_POINT('Ctrl Pts',(1.02116533136119,3.54921942038456,-12.5287546368838)) ;
#154353=CARTESIAN_POINT('Ctrl Pts',(1.02580209629923,3.54969340754027,-12.5244085428281)) ;
#154354=CARTESIAN_POINT('Ctrl Pts',(1.02780524115376,3.54989817637043,-12.5225309717066)) ;
#154355=CARTESIAN_POINT('Ctrl Pts',(1.02980744674852,3.55,-12.5206439182703)) ;
#154356=CARTESIAN_POINT('Ctrl Pts',(1.03179971315146,3.55,-12.5187558734356)) ;
#154357=CARTESIAN_POINT('Origin',(-7.29372370581158E-16,3.55,-11.43)) ;
#154358=CARTESIAN_POINT('',(1.5,3.55,-11.43)) ;
#154359=CARTESIAN_POINT('Origin',(-7.29372370581158E-16,3.55,-15.24)) ;
#154360=CARTESIAN_POINT('',(-0.17080731546663,3.55,-13.7497567779107)) ;
#154361=CARTESIAN_POINT('',(1.5,3.55,-15.24)) ;
#154362=CARTESIAN_POINT('Origin',(-7.29372370581158E-16,3.55,-15.24)) ;
#154363=CARTESIAN_POINT('',(-0.273932138433073,3.45,-13.7652250396981)) ;
#154364=CARTESIAN_POINT('Ctrl Pts',(-0.17080731546662,3.55,-13.7497567779107)) ;
#154365=CARTESIAN_POINT('Ctrl Pts',(-0.183882433427078,3.55,-13.7512554096543)) ;
#154366=CARTESIAN_POINT('Ctrl Pts',(-0.197859036177,3.54752250383109,-13.7530511760977)) ;
#154367=CARTESIAN_POINT('Ctrl Pts',(-0.223597793566244,3.53719045839678,
-13.7567006467314)) ;
#154368=CARTESIAN_POINT('Ctrl Pts',(-0.235362682979166,3.52934133421403,
-13.7585504186891)) ;
#154369=CARTESIAN_POINT('Ctrl Pts',(-0.253465441530103,3.51138121637726,
-13.7615429480238)) ;
#154370=CARTESIAN_POINT('Ctrl Pts',(-0.261168570620294,3.50026979217228,
-13.7629034821853)) ;
#154371=CARTESIAN_POINT('Ctrl Pts',(-0.271399896344085,3.47583586070553,
-13.7647463645995)) ;
#154372=CARTESIAN_POINT('Ctrl Pts',(-0.273932138433063,3.46251477070021,
-13.7652250396981)) ;
#154373=CARTESIAN_POINT('Ctrl Pts',(-0.273932138433063,3.45,-13.7652250396981)) ;
#154374=CARTESIAN_POINT('',(-0.273932138433073,3.15,-13.7652250396981)) ;
#154375=CARTESIAN_POINT('',(-0.273932138433073,3.05,-13.7652250396981)) ;
#154376=CARTESIAN_POINT('',(-0.373948193368569,3.05,-13.7873600760421)) ;
#154377=CARTESIAN_POINT('Ctrl Pts',(-0.27393213843307,3.15,-13.7652250396981)) ;
#154378=CARTESIAN_POINT('Ctrl Pts',(-0.27393213843307,3.13744372549049,
-13.7652250396981)) ;
#154379=CARTESIAN_POINT('Ctrl Pts',(-0.276486468486161,3.12408297110069,
-13.7656911302356)) ;
#154380=CARTESIAN_POINT('Ctrl Pts',(-0.286740277640426,3.0995678553947,
-13.7676537789936)) ;
#154381=CARTESIAN_POINT('Ctrl Pts',(-0.294439768310514,3.08841385970397,
-13.7691548411377)) ;
#154382=CARTESIAN_POINT('Ctrl Pts',(-0.312194128344968,3.07061084469361,
-13.772819399951)) ;
#154383=CARTESIAN_POINT('Ctrl Pts',(-0.323517908844214,3.0628422827531,
-13.7752474862748)) ;
#154384=CARTESIAN_POINT('Ctrl Pts',(-0.348172117123302,3.05253676672645,
-13.7809138387535)) ;
#154385=CARTESIAN_POINT('Ctrl Pts',(-0.361501722536394,3.05,-13.7841560230592)) ;
#154386=CARTESIAN_POINT('Ctrl Pts',(-0.373948193368566,3.05,-13.7873600760421)) ;
#154387=CARTESIAN_POINT('',(-0.872417476238727,3.05,-14.0198001199995)) ;
#154388=CARTESIAN_POINT('Origin',(-7.95081593156037E-16,3.05,-15.24)) ;
#154389=CARTESIAN_POINT('',(-0.953662978710562,3.15,-14.0821887360036)) ;
#154390=CARTESIAN_POINT('Ctrl Pts',(-0.872417476238731,3.05,-14.0198001199995)) ;
#154391=CARTESIAN_POINT('Ctrl Pts',(-0.882808783297382,3.05,-14.027229687915)) ;
#154392=CARTESIAN_POINT('Ctrl Pts',(-0.893798224191979,3.05250629897269,
-14.0353093623146)) ;
#154393=CARTESIAN_POINT('Ctrl Pts',(-0.913892243159222,3.06269675232156,
-14.0504777691246)) ;
#154394=CARTESIAN_POINT('Ctrl Pts',(-0.922999225059838,3.07038074042647,
-14.0575634285691)) ;
#154395=CARTESIAN_POINT('Ctrl Pts',(-0.93728513413171,3.08810056349785,
-14.0688558711034)) ;
#154396=CARTESIAN_POINT('Ctrl Pts',(-0.943452174397239,3.09929464195085,
-14.073843096804)) ;
#154397=CARTESIAN_POINT('Ctrl Pts',(-0.951639309815366,3.12392729225934,
-14.0805109997964)) ;
#154398=CARTESIAN_POINT('Ctrl Pts',(-0.953662978710566,3.13736547222678,
-14.0821887360036)) ;
#154399=CARTESIAN_POINT('Ctrl Pts',(-0.953662978710566,3.15,-14.0821887360036)) ;
#154400=CARTESIAN_POINT('',(-0.953662978710562,3.45,-14.0821887360036)) ;
#154401=CARTESIAN_POINT('',(-0.953662978710562,3.05,-14.0821887360036)) ;
#154402=CARTESIAN_POINT('',(-1.03179971315145,3.55,-14.1512441265644)) ;
#154403=CARTESIAN_POINT('Ctrl Pts',(-0.953662978710574,3.45,-14.0821887360036)) ;
#154404=CARTESIAN_POINT('Ctrl Pts',(-0.953662978710574,3.45580715149871,
-14.0821887360036)) ;
#154405=CARTESIAN_POINT('Ctrl Pts',(-0.954069792639917,3.46165880969181,
-14.0825236315692)) ;
#154406=CARTESIAN_POINT('Ctrl Pts',(-0.954880405808387,3.46741264967889,
-14.0831927320754)) ;
#154407=CARTESIAN_POINT('Ctrl Pts',(-0.955592557016205,3.47246759358526,
-14.0837805596017)) ;
#154408=CARTESIAN_POINT('Ctrl Pts',(-0.956615573654938,3.47744631522378,
-14.0846258114488)) ;
#154409=CARTESIAN_POINT('Ctrl Pts',(-0.957920385817356,3.48225893605768,
-14.0857086440434)) ;
#154410=CARTESIAN_POINT('Ctrl Pts',(-0.959423079246208,3.48780141482279,
-14.0869556935967)) ;
#154411=CARTESIAN_POINT('Ctrl Pts',(-0.961323201468142,3.49320783601915,
-14.0885374593817)) ;
#154412=CARTESIAN_POINT('Ctrl Pts',(-0.963574238618814,3.4983456004987,
-14.0904242578964)) ;
#154413=CARTESIAN_POINT('Ctrl Pts',(-0.965499706648002,3.50274028640777,
-14.0920381673855)) ;
#154414=CARTESIAN_POINT('Ctrl Pts',(-0.967680912999544,3.5069382066956,
-14.0938745944584)) ;
#154415=CARTESIAN_POINT('Ctrl Pts',(-0.970068248378245,3.51087311165944,
-14.0958987835472)) ;
#154416=CARTESIAN_POINT('Ctrl Pts',(-0.97293324697907,3.51559532091262,
-14.0983279767636)) ;
#154417=CARTESIAN_POINT('Ctrl Pts',(-0.976138831290361,3.52000896466724,
-14.1010646855624)) ;
#154418=CARTESIAN_POINT('Ctrl Pts',(-0.979601776802482,3.52400782220665,
-14.1040509843476)) ;
#154419=CARTESIAN_POINT('Ctrl Pts',(-0.982467725203497,3.52731729367563,
-14.1065224578947)) ;
#154420=CARTESIAN_POINT('Ctrl Pts',(-0.985508986896835,3.5303430569618,
-14.1091641736047)) ;
#154421=CARTESIAN_POINT('Ctrl Pts',(-0.988666612105892,3.53304718478134,
-14.1119315933388)) ;
#154422=CARTESIAN_POINT('Ctrl Pts',(-0.99270160680367,3.53650267449007,
-14.1154679610881)) ;
#154423=CARTESIAN_POINT('Ctrl Pts',(-0.996988044734306,3.53948417067184,
-14.1192635881177)) ;
#154424=CARTESIAN_POINT('Ctrl Pts',(-1.00141585135915,3.54192188246041,
-14.1232340352035)) ;
#154425=CARTESIAN_POINT('Ctrl Pts',(-1.00487400994927,3.54382575827887,
-14.1263349916949)) ;
#154426=CARTESIAN_POINT('Ctrl Pts',(-1.00841776012226,3.54539884758398,
-14.1295419608726)) ;
#154427=CARTESIAN_POINT('Ctrl Pts',(-1.01199129263162,3.54662946216441,
-14.1328082263467)) ;
#154428=CARTESIAN_POINT('Ctrl Pts',(-1.01652362695401,3.54819025857132,
-14.1369508519072)) ;
#154429=CARTESIAN_POINT('Ctrl Pts',(-1.02116533136119,3.54921942038456,
-14.1412453631162)) ;
#154430=CARTESIAN_POINT('Ctrl Pts',(-1.02580209629922,3.54969340754027,
-14.1455914571719)) ;
#154431=CARTESIAN_POINT('Ctrl Pts',(-1.02780524115375,3.54989817637043,
-14.1474690282934)) ;
#154432=CARTESIAN_POINT('Ctrl Pts',(-1.02980744674853,3.55,-14.1493560817297)) ;
#154433=CARTESIAN_POINT('Ctrl Pts',(-1.03179971315146,3.55,-14.1512441265644)) ;
#154434=CARTESIAN_POINT('',(0.170807315466632,3.55,-16.7302432220893)) ;
#154435=CARTESIAN_POINT('Origin',(-7.29372370581158E-16,3.55,-15.24)) ;
#154436=CARTESIAN_POINT('',(0.273932138433074,3.45,-16.7147749603019)) ;
#154437=CARTESIAN_POINT('Ctrl Pts',(0.170807315466623,3.55,-16.7302432220893)) ;
#154438=CARTESIAN_POINT('Ctrl Pts',(0.183882433427081,3.55,-16.7287445903457)) ;
#154439=CARTESIAN_POINT('Ctrl Pts',(0.197859036177004,3.54752250383109,
-16.7269488239023)) ;
#154440=CARTESIAN_POINT('Ctrl Pts',(0.223597793566247,3.53719045839678,
-16.7232993532686)) ;
#154441=CARTESIAN_POINT('Ctrl Pts',(0.235362682979168,3.52934133421403,
-16.7214495813109)) ;
#154442=CARTESIAN_POINT('Ctrl Pts',(0.253465441530106,3.51138121637726,
-16.7184570519762)) ;
#154443=CARTESIAN_POINT('Ctrl Pts',(0.261168570620297,3.50026979217228,
-16.7170965178147)) ;
#154444=CARTESIAN_POINT('Ctrl Pts',(0.271399896344088,3.47583586070553,
-16.7152536354005)) ;
#154445=CARTESIAN_POINT('Ctrl Pts',(0.273932138433066,3.46251477070021,
-16.7147749603019)) ;
#154446=CARTESIAN_POINT('Ctrl Pts',(0.273932138433066,3.45,-16.7147749603019)) ;
#154447=CARTESIAN_POINT('',(0.273932138433074,3.15,-16.7147749603019)) ;
#154448=CARTESIAN_POINT('',(0.273932138433074,3.05,-16.7147749603019)) ;
#154449=CARTESIAN_POINT('',(0.37394819336857,3.05,-16.6926399239579)) ;
#154450=CARTESIAN_POINT('Ctrl Pts',(0.273932138433069,3.15,-16.7147749603019)) ;
#154451=CARTESIAN_POINT('Ctrl Pts',(0.273932138433069,3.13736547222678,
-16.7147749603019)) ;
#154452=CARTESIAN_POINT('Ctrl Pts',(0.276518148223576,3.12392729225934,
-16.7143031680364)) ;
#154453=CARTESIAN_POINT('Ctrl Pts',(0.286888647463775,3.09929464195085,
-16.7123175038704)) ;
#154454=CARTESIAN_POINT('Ctrl Pts',(0.294673181069385,3.08810056349785,
-16.7107990038315)) ;
#154455=CARTESIAN_POINT('Ctrl Pts',(0.312506499266529,3.07038074042647,
-16.7071140047162)) ;
#154456=CARTESIAN_POINT('Ctrl Pts',(0.323788284437176,3.06269675232156,
-16.704692225935)) ;
#154457=CARTESIAN_POINT('Ctrl Pts',(0.348324144605926,3.05250629897269,
-16.6990493783214)) ;
#154458=CARTESIAN_POINT('Ctrl Pts',(0.361577410726385,3.05,-16.6958244927855)) ;
#154459=CARTESIAN_POINT('Ctrl Pts',(0.373948193368565,3.05,-16.6926399239579)) ;
#154460=CARTESIAN_POINT('',(0.872417476238728,3.05,-16.4601998800005)) ;
#154461=CARTESIAN_POINT('Origin',(-7.95081593156037E-16,3.05,-15.24)) ;
#154462=CARTESIAN_POINT('',(0.953662978710562,3.15,-16.3978112639964)) ;
#154463=CARTESIAN_POINT('Ctrl Pts',(0.87241747623873,3.05,-16.4601998800005)) ;
#154464=CARTESIAN_POINT('Ctrl Pts',(0.882872360457022,3.05,-16.4527248557413)) ;
#154465=CARTESIAN_POINT('Ctrl Pts',(0.893924122929508,3.05253676672645,
-16.4445978214856)) ;
#154466=CARTESIAN_POINT('Ctrl Pts',(0.914112220366979,3.0628422827531,-16.4293538633994)) ;
#154467=CARTESIAN_POINT('Ctrl Pts',(0.923251028202472,3.07061084469361,
-16.422240088077)) ;
#154468=CARTESIAN_POINT('Ctrl Pts',(0.937470525765901,3.08841385970397,
-16.4109949922316)) ;
#154469=CARTESIAN_POINT('Ctrl Pts',(0.943569543283853,3.0995678553947,-16.4060617043366)) ;
#154470=CARTESIAN_POINT('Ctrl Pts',(0.951664040935145,3.12408297110069,
-16.3994683971169)) ;
#154471=CARTESIAN_POINT('Ctrl Pts',(0.953662978710565,3.13744372549049,
-16.3978112639964)) ;
#154472=CARTESIAN_POINT('Ctrl Pts',(0.953662978710565,3.15,-16.3978112639964)) ;
#154473=CARTESIAN_POINT('',(0.953662978710562,3.45,-16.3978112639964)) ;
#154474=CARTESIAN_POINT('',(0.953662978710562,3.05,-16.3978112639964)) ;
#154475=CARTESIAN_POINT('',(1.03179971315145,3.55,-16.3287558734356)) ;
#154476=CARTESIAN_POINT('Ctrl Pts',(0.953662978710576,3.45,-16.3978112639964)) ;
#154477=CARTESIAN_POINT('Ctrl Pts',(0.953662978710576,3.45580715149871,
-16.3978112639964)) ;
#154478=CARTESIAN_POINT('Ctrl Pts',(0.95406979263992,3.46165880969181,-16.3974763684308)) ;
#154479=CARTESIAN_POINT('Ctrl Pts',(0.95488040580839,3.46741264967889,-16.3968072679246)) ;
#154480=CARTESIAN_POINT('Ctrl Pts',(0.955592557016207,3.47246759358526,
-16.3962194403983)) ;
#154481=CARTESIAN_POINT('Ctrl Pts',(0.95661557365494,3.47744631522378,-16.3953741885512)) ;
#154482=CARTESIAN_POINT('Ctrl Pts',(0.957920385817358,3.48225893605768,
-16.3942913559566)) ;
#154483=CARTESIAN_POINT('Ctrl Pts',(0.959423079246208,3.48780141482278,
-16.3930443064033)) ;
#154484=CARTESIAN_POINT('Ctrl Pts',(0.961323201468132,3.49320783601912,
-16.3914625406183)) ;
#154485=CARTESIAN_POINT('Ctrl Pts',(0.963574238618799,3.49834560049866,
-16.3895757421036)) ;
#154486=CARTESIAN_POINT('Ctrl Pts',(0.965499706647992,3.50274028640775,
-16.3879618326145)) ;
#154487=CARTESIAN_POINT('Ctrl Pts',(0.967680912999541,3.50693820669559,
-16.3861254055416)) ;
#154488=CARTESIAN_POINT('Ctrl Pts',(0.970068248378248,3.51087311165943,
-16.3841012164528)) ;
#154489=CARTESIAN_POINT('Ctrl Pts',(0.972933246979074,3.51559532091262,
-16.3816720232364)) ;
#154490=CARTESIAN_POINT('Ctrl Pts',(0.976138831290367,3.52000896466725,
-16.3789353144376)) ;
#154491=CARTESIAN_POINT('Ctrl Pts',(0.979601776802491,3.52400782220666,
-16.3759490156524)) ;
#154492=CARTESIAN_POINT('Ctrl Pts',(0.982467725203503,3.52731729367563,
-16.3734775421053)) ;
#154493=CARTESIAN_POINT('Ctrl Pts',(0.985508986896837,3.5303430569618,-16.3708358263953)) ;
#154494=CARTESIAN_POINT('Ctrl Pts',(0.988666612105889,3.53304718478133,
-16.3680684066612)) ;
#154495=CARTESIAN_POINT('Ctrl Pts',(0.992701606803676,3.53650267449008,
-16.3645320389119)) ;
#154496=CARTESIAN_POINT('Ctrl Pts',(0.996988044734359,3.53948417067189,
-16.3607364118822)) ;
#154497=CARTESIAN_POINT('Ctrl Pts',(1.0014158513592,3.54192188246044,-16.3567659647965)) ;
#154498=CARTESIAN_POINT('Ctrl Pts',(1.0048740099493,3.54382575827887,-16.3536650083051)) ;
#154499=CARTESIAN_POINT('Ctrl Pts',(1.00841776012226,3.54539884758398,-16.3504580391274)) ;
#154500=CARTESIAN_POINT('Ctrl Pts',(1.01199129263161,3.54662946216441,-16.3471917736533)) ;
#154501=CARTESIAN_POINT('Ctrl Pts',(1.01652362695402,3.54819025857132,-16.3430491480928)) ;
#154502=CARTESIAN_POINT('Ctrl Pts',(1.0211653313612,3.54921942038456,-16.3387546368838)) ;
#154503=CARTESIAN_POINT('Ctrl Pts',(1.02580209629924,3.54969340754027,-16.3344085428281)) ;
#154504=CARTESIAN_POINT('Ctrl Pts',(1.02780524115376,3.54989817637043,-16.3325309717066)) ;
#154505=CARTESIAN_POINT('Ctrl Pts',(1.02980744674853,3.55,-16.3306439182703)) ;
#154506=CARTESIAN_POINT('Ctrl Pts',(1.03179971315146,3.55,-16.3287558734356)) ;
#154507=CARTESIAN_POINT('Origin',(-7.29372370581158E-16,3.55,-15.24)) ;
#154508=CARTESIAN_POINT('',(1.5,3.55,-15.24)) ;
#154509=CARTESIAN_POINT('Origin',(-7.29372370581158E-16,3.55,-19.05)) ;
#154510=CARTESIAN_POINT('',(-0.170807315466631,3.55,-17.5597567779107)) ;
#154511=CARTESIAN_POINT('',(1.5,3.55,-19.05)) ;
#154512=CARTESIAN_POINT('Origin',(-7.29372370581158E-16,3.55,-19.05)) ;
#154513=CARTESIAN_POINT('',(-0.273932138433073,3.45,-17.5752250396981)) ;
#154514=CARTESIAN_POINT('Ctrl Pts',(-0.170807315466618,3.55,-17.5597567779107)) ;
#154515=CARTESIAN_POINT('Ctrl Pts',(-0.183882433427076,3.55,-17.5612554096543)) ;
#154516=CARTESIAN_POINT('Ctrl Pts',(-0.197859036176998,3.54752250383109,
-17.5630511760977)) ;
#154517=CARTESIAN_POINT('Ctrl Pts',(-0.223597793566241,3.53719045839678,
-17.5667006467314)) ;
#154518=CARTESIAN_POINT('Ctrl Pts',(-0.235362682979163,3.52934133421403,
-17.5685504186891)) ;
#154519=CARTESIAN_POINT('Ctrl Pts',(-0.2534654415301,3.51138121637726,-17.5715429480238)) ;
#154520=CARTESIAN_POINT('Ctrl Pts',(-0.261168570620293,3.50026979217228,
-17.5729034821853)) ;
#154521=CARTESIAN_POINT('Ctrl Pts',(-0.271399896344084,3.47583586070553,
-17.5747463645995)) ;
#154522=CARTESIAN_POINT('Ctrl Pts',(-0.273932138433061,3.46251477070021,
-17.5752250396981)) ;
#154523=CARTESIAN_POINT('Ctrl Pts',(-0.273932138433061,3.45,-17.5752250396981)) ;
#154524=CARTESIAN_POINT('',(-0.273932138433073,3.15,-17.5752250396981)) ;
#154525=CARTESIAN_POINT('',(-0.273932138433073,3.05,-17.5752250396981)) ;
#154526=CARTESIAN_POINT('',(-0.373948193368567,3.05,-17.5973600760421)) ;
#154527=CARTESIAN_POINT('Ctrl Pts',(-0.273932138433067,3.15,-17.5752250396981)) ;
#154528=CARTESIAN_POINT('Ctrl Pts',(-0.273932138433067,3.13744372549049,
-17.5752250396981)) ;
#154529=CARTESIAN_POINT('Ctrl Pts',(-0.276486468486159,3.12408297110069,
-17.5756911302356)) ;
#154530=CARTESIAN_POINT('Ctrl Pts',(-0.286740277640424,3.0995678553947,
-17.5776537789936)) ;
#154531=CARTESIAN_POINT('Ctrl Pts',(-0.294439768310511,3.08841385970397,
-17.5791548411377)) ;
#154532=CARTESIAN_POINT('Ctrl Pts',(-0.312194128344966,3.07061084469361,
-17.582819399951)) ;
#154533=CARTESIAN_POINT('Ctrl Pts',(-0.323517908844211,3.0628422827531,
-17.5852474862748)) ;
#154534=CARTESIAN_POINT('Ctrl Pts',(-0.348172117123299,3.05253676672645,
-17.5909138387535)) ;
#154535=CARTESIAN_POINT('Ctrl Pts',(-0.361501722536391,3.05,-17.5941560230592)) ;
#154536=CARTESIAN_POINT('Ctrl Pts',(-0.373948193368564,3.05,-17.5973600760421)) ;
#154537=CARTESIAN_POINT('',(-0.872417476238727,3.05,-17.8298001199995)) ;
#154538=CARTESIAN_POINT('Origin',(-7.95081593156037E-16,3.05,-19.05)) ;
#154539=CARTESIAN_POINT('',(-0.953662978710562,3.15,-17.8921887360036)) ;
#154540=CARTESIAN_POINT('Ctrl Pts',(-0.87241747623873,3.05,-17.8298001199995)) ;
#154541=CARTESIAN_POINT('Ctrl Pts',(-0.88280878329738,3.05,-17.837229687915)) ;
#154542=CARTESIAN_POINT('Ctrl Pts',(-0.893798224191977,3.05250629897269,
-17.8453093623146)) ;
#154543=CARTESIAN_POINT('Ctrl Pts',(-0.913892243159221,3.06269675232156,
-17.8604777691246)) ;
#154544=CARTESIAN_POINT('Ctrl Pts',(-0.922999225059836,3.07038074042647,
-17.8675634285691)) ;
#154545=CARTESIAN_POINT('Ctrl Pts',(-0.937285134131708,3.08810056349785,
-17.8788558711034)) ;
#154546=CARTESIAN_POINT('Ctrl Pts',(-0.943452174397237,3.09929464195085,
-17.883843096804)) ;
#154547=CARTESIAN_POINT('Ctrl Pts',(-0.951639309815365,3.12392729225934,
-17.8905109997964)) ;
#154548=CARTESIAN_POINT('Ctrl Pts',(-0.953662978710563,3.13736547222678,
-17.8921887360036)) ;
#154549=CARTESIAN_POINT('Ctrl Pts',(-0.953662978710563,3.15,-17.8921887360036)) ;
#154550=CARTESIAN_POINT('',(-0.953662978710562,3.45,-17.8921887360036)) ;
#154551=CARTESIAN_POINT('',(-0.953662978710562,3.05,-17.8921887360036)) ;
#154552=CARTESIAN_POINT('',(-1.03179971315145,3.55,-17.9612441265644)) ;
#154553=CARTESIAN_POINT('Ctrl Pts',(-0.953662978710576,3.45,-17.8921887360036)) ;
#154554=CARTESIAN_POINT('Ctrl Pts',(-0.953662978710576,3.45580715149871,
-17.8921887360036)) ;
#154555=CARTESIAN_POINT('Ctrl Pts',(-0.954069792639918,3.4616588096918,
-17.8925236315692)) ;
#154556=CARTESIAN_POINT('Ctrl Pts',(-0.954880405808387,3.46741264967887,
-17.8931927320754)) ;
#154557=CARTESIAN_POINT('Ctrl Pts',(-0.955592557016204,3.47246759358525,
-17.8937805596017)) ;
#154558=CARTESIAN_POINT('Ctrl Pts',(-0.956615573654935,3.47744631522377,
-17.8946258114488)) ;
#154559=CARTESIAN_POINT('Ctrl Pts',(-0.957920385817355,3.48225893605768,
-17.8957086440434)) ;
#154560=CARTESIAN_POINT('Ctrl Pts',(-0.959423079246204,3.48780141482278,
-17.8969556935967)) ;
#154561=CARTESIAN_POINT('Ctrl Pts',(-0.96132320146813,3.49320783601912,
-17.8985374593817)) ;
#154562=CARTESIAN_POINT('Ctrl Pts',(-0.963574238618794,3.49834560049866,
-17.9004242578964)) ;
#154563=CARTESIAN_POINT('Ctrl Pts',(-0.965499706647985,3.50274028640774,
-17.9020381673855)) ;
#154564=CARTESIAN_POINT('Ctrl Pts',(-0.967680912999533,3.50693820669558,
-17.9038745944584)) ;
#154565=CARTESIAN_POINT('Ctrl Pts',(-0.970068248378242,3.51087311165943,
-17.9058987835472)) ;
#154566=CARTESIAN_POINT('Ctrl Pts',(-0.972933246979071,3.51559532091262,
-17.9083279767636)) ;
#154567=CARTESIAN_POINT('Ctrl Pts',(-0.976138831290368,3.52000896466725,
-17.9110646855624)) ;
#154568=CARTESIAN_POINT('Ctrl Pts',(-0.979601776802492,3.52400782220666,
-17.9140509843476)) ;
#154569=CARTESIAN_POINT('Ctrl Pts',(-0.982467725203504,3.52731729367563,
-17.9165224578947)) ;
#154570=CARTESIAN_POINT('Ctrl Pts',(-0.985508986896838,3.5303430569618,
-17.9191641736047)) ;
#154571=CARTESIAN_POINT('Ctrl Pts',(-0.988666612105874,3.53304718478133,
-17.9219315933388)) ;
#154572=CARTESIAN_POINT('Ctrl Pts',(-0.992701606803626,3.53650267449005,
-17.9254679610881)) ;
#154573=CARTESIAN_POINT('Ctrl Pts',(-0.996988044734298,3.53948417067184,
-17.9292635881177)) ;
#154574=CARTESIAN_POINT('Ctrl Pts',(-1.00141585135914,3.5419218824604,-17.9332340352035)) ;
#154575=CARTESIAN_POINT('Ctrl Pts',(-1.00487400994926,3.54382575827887,
-17.9363349916949)) ;
#154576=CARTESIAN_POINT('Ctrl Pts',(-1.00841776012225,3.54539884758397,
-17.9395419608726)) ;
#154577=CARTESIAN_POINT('Ctrl Pts',(-1.01199129263161,3.54662946216441,
-17.9428082263467)) ;
#154578=CARTESIAN_POINT('Ctrl Pts',(-1.01652362695402,3.54819025857132,
-17.9469508519072)) ;
#154579=CARTESIAN_POINT('Ctrl Pts',(-1.02116533136121,3.54921942038456,
-17.9512453631162)) ;
#154580=CARTESIAN_POINT('Ctrl Pts',(-1.02580209629926,3.54969340754028,
-17.9555914571719)) ;
#154581=CARTESIAN_POINT('Ctrl Pts',(-1.02780524115377,3.54989817637043,
-17.9574690282934)) ;
#154582=CARTESIAN_POINT('Ctrl Pts',(-1.02980744674854,3.55,-17.9593560817297)) ;
#154583=CARTESIAN_POINT('Ctrl Pts',(-1.03179971315146,3.55,-17.9612441265644)) ;
#154584=CARTESIAN_POINT('',(0.170807315466633,3.55,-20.5402432220893)) ;
#154585=CARTESIAN_POINT('Origin',(-7.29372370581158E-16,3.55,-19.05)) ;
#154586=CARTESIAN_POINT('',(0.273932138433074,3.45,-20.5247749603019)) ;
#154587=CARTESIAN_POINT('Ctrl Pts',(0.170807315466623,3.55,-20.5402432220893)) ;
#154588=CARTESIAN_POINT('Ctrl Pts',(0.18388243342708,3.55,-20.5387445903457)) ;
#154589=CARTESIAN_POINT('Ctrl Pts',(0.197859036177002,3.54752250383109,
-20.5369488239023)) ;
#154590=CARTESIAN_POINT('Ctrl Pts',(0.223597793566245,3.53719045839678,
-20.5332993532686)) ;
#154591=CARTESIAN_POINT('Ctrl Pts',(0.235362682979168,3.52934133421403,
-20.531449581311)) ;
#154592=CARTESIAN_POINT('Ctrl Pts',(0.253465441530105,3.51138121637726,
-20.5284570519762)) ;
#154593=CARTESIAN_POINT('Ctrl Pts',(0.261168570620294,3.50026979217228,
-20.5270965178147)) ;
#154594=CARTESIAN_POINT('Ctrl Pts',(0.271399896344085,3.47583586070553,
-20.5252536354005)) ;
#154595=CARTESIAN_POINT('Ctrl Pts',(0.273932138433065,3.46251477070021,
-20.5247749603019)) ;
#154596=CARTESIAN_POINT('Ctrl Pts',(0.273932138433065,3.45,-20.5247749603019)) ;
#154597=CARTESIAN_POINT('',(0.273932138433074,3.15,-20.5247749603019)) ;
#154598=CARTESIAN_POINT('',(0.273932138433074,3.05,-20.5247749603019)) ;
#154599=CARTESIAN_POINT('',(0.373948193368569,3.05,-20.5026399239579)) ;
#154600=CARTESIAN_POINT('Ctrl Pts',(0.273932138433072,3.15,-20.5247749603019)) ;
#154601=CARTESIAN_POINT('Ctrl Pts',(0.273932138433072,3.13736547222678,
-20.5247749603019)) ;
#154602=CARTESIAN_POINT('Ctrl Pts',(0.276518148223578,3.12392729225934,
-20.5243031680364)) ;
#154603=CARTESIAN_POINT('Ctrl Pts',(0.286888647463776,3.09929464195085,
-20.5223175038704)) ;
#154604=CARTESIAN_POINT('Ctrl Pts',(0.294673181069388,3.08810056349785,
-20.5207990038315)) ;
#154605=CARTESIAN_POINT('Ctrl Pts',(0.312506499266531,3.07038074042647,
-20.5171140047162)) ;
#154606=CARTESIAN_POINT('Ctrl Pts',(0.323788284437176,3.06269675232156,
-20.514692225935)) ;
#154607=CARTESIAN_POINT('Ctrl Pts',(0.348324144605927,3.05250629897269,
-20.5090493783214)) ;
#154608=CARTESIAN_POINT('Ctrl Pts',(0.361577410726387,3.05,-20.5058244927855)) ;
#154609=CARTESIAN_POINT('Ctrl Pts',(0.373948193368567,3.05,-20.5026399239579)) ;
#154610=CARTESIAN_POINT('',(0.872417476238729,3.05,-20.2701998800005)) ;
#154611=CARTESIAN_POINT('Origin',(-7.95081593156037E-16,3.05,-19.05)) ;
#154612=CARTESIAN_POINT('',(0.953662978710562,3.15,-20.2078112639964)) ;
#154613=CARTESIAN_POINT('Ctrl Pts',(0.872417476238732,3.05,-20.2701998800005)) ;
#154614=CARTESIAN_POINT('Ctrl Pts',(0.88287236045702,3.05,-20.2627248557413)) ;
#154615=CARTESIAN_POINT('Ctrl Pts',(0.893924122929511,3.05253676672645,
-20.2545978214856)) ;
#154616=CARTESIAN_POINT('Ctrl Pts',(0.914112220366982,3.0628422827531,-20.2393538633994)) ;
#154617=CARTESIAN_POINT('Ctrl Pts',(0.923251028202474,3.07061084469361,
-20.232240088077)) ;
#154618=CARTESIAN_POINT('Ctrl Pts',(0.937470525765903,3.08841385970397,
-20.2209949922316)) ;
#154619=CARTESIAN_POINT('Ctrl Pts',(0.943569543283854,3.0995678553947,-20.2160617043366)) ;
#154620=CARTESIAN_POINT('Ctrl Pts',(0.951664040935147,3.12408297110069,
-20.2094683971169)) ;
#154621=CARTESIAN_POINT('Ctrl Pts',(0.953662978710566,3.13744372549049,
-20.2078112639964)) ;
#154622=CARTESIAN_POINT('Ctrl Pts',(0.953662978710566,3.15,-20.2078112639964)) ;
#154623=CARTESIAN_POINT('',(0.953662978710562,3.45,-20.2078112639964)) ;
#154624=CARTESIAN_POINT('',(0.953662978710562,3.05,-20.2078112639964)) ;
#154625=CARTESIAN_POINT('',(1.03179971315145,3.55,-20.1387558734356)) ;
#154626=CARTESIAN_POINT('Ctrl Pts',(0.953662978710579,3.45,-20.2078112639964)) ;
#154627=CARTESIAN_POINT('Ctrl Pts',(0.953662978710579,3.45580715149871,
-20.2078112639964)) ;
#154628=CARTESIAN_POINT('Ctrl Pts',(0.954069792639924,3.46165880969181,
-20.2074763684308)) ;
#154629=CARTESIAN_POINT('Ctrl Pts',(0.954880405808395,3.46741264967889,
-20.2068072679246)) ;
#154630=CARTESIAN_POINT('Ctrl Pts',(0.955592557016213,3.47246759358527,
-20.2062194403983)) ;
#154631=CARTESIAN_POINT('Ctrl Pts',(0.956615573654944,3.47744631522378,
-20.2053741885512)) ;
#154632=CARTESIAN_POINT('Ctrl Pts',(0.957920385817361,3.48225893605768,
-20.2042913559566)) ;
#154633=CARTESIAN_POINT('Ctrl Pts',(0.959423079246211,3.48780141482278,
-20.2030443064033)) ;
#154634=CARTESIAN_POINT('Ctrl Pts',(0.961323201468137,3.49320783601913,
-20.2014625406183)) ;
#154635=CARTESIAN_POINT('Ctrl Pts',(0.963574238618808,3.49834560049867,
-20.1995757421036)) ;
#154636=CARTESIAN_POINT('Ctrl Pts',(0.965499706647999,3.50274028640776,
-20.1979618326145)) ;
#154637=CARTESIAN_POINT('Ctrl Pts',(0.967680912999541,3.50693820669559,
-20.1961254055416)) ;
#154638=CARTESIAN_POINT('Ctrl Pts',(0.970068248378246,3.51087311165943,
-20.1941012164528)) ;
#154639=CARTESIAN_POINT('Ctrl Pts',(0.972933246979075,3.51559532091262,
-20.1916720232364)) ;
#154640=CARTESIAN_POINT('Ctrl Pts',(0.97613883129037,3.52000896466725,-20.1889353144376)) ;
#154641=CARTESIAN_POINT('Ctrl Pts',(0.979601776802495,3.52400782220666,
-20.1859490156524)) ;
#154642=CARTESIAN_POINT('Ctrl Pts',(0.982467725203507,3.52731729367563,
-20.1834775421053)) ;
#154643=CARTESIAN_POINT('Ctrl Pts',(0.98550898689684,3.5303430569618,-20.1808358263953)) ;
#154644=CARTESIAN_POINT('Ctrl Pts',(0.988666612105893,3.53304718478133,
-20.1780684066612)) ;
#154645=CARTESIAN_POINT('Ctrl Pts',(0.992701606803678,3.53650267449007,
-20.1745320389119)) ;
#154646=CARTESIAN_POINT('Ctrl Pts',(0.996988044734317,3.53948417067185,
-20.1707364118823)) ;
#154647=CARTESIAN_POINT('Ctrl Pts',(1.00141585135917,3.54192188246042,-20.1667659647965)) ;
#154648=CARTESIAN_POINT('Ctrl Pts',(1.00487400994928,3.54382575827887,-20.1636650083051)) ;
#154649=CARTESIAN_POINT('Ctrl Pts',(1.00841776012227,3.54539884758398,-20.1604580391274)) ;
#154650=CARTESIAN_POINT('Ctrl Pts',(1.01199129263161,3.54662946216441,-20.1571917736533)) ;
#154651=CARTESIAN_POINT('Ctrl Pts',(1.01652362695402,3.54819025857132,-20.1530491480928)) ;
#154652=CARTESIAN_POINT('Ctrl Pts',(1.02116533136121,3.54921942038456,-20.1487546368838)) ;
#154653=CARTESIAN_POINT('Ctrl Pts',(1.02580209629926,3.54969340754028,-20.1444085428281)) ;
#154654=CARTESIAN_POINT('Ctrl Pts',(1.02780524115377,3.54989817637043,-20.1425309717066)) ;
#154655=CARTESIAN_POINT('Ctrl Pts',(1.02980744674853,3.55,-20.1406439182703)) ;
#154656=CARTESIAN_POINT('Ctrl Pts',(1.03179971315146,3.55,-20.1387558734356)) ;
#154657=CARTESIAN_POINT('Origin',(-7.29372370581158E-16,3.55,-19.05)) ;
#154658=CARTESIAN_POINT('',(1.5,3.55,-19.05)) ;
#154659=CARTESIAN_POINT('Origin',(-7.29372370581158E-16,3.55,-22.86)) ;
#154660=CARTESIAN_POINT('',(-0.170807315466631,3.55,-21.3697567779107)) ;
#154661=CARTESIAN_POINT('',(1.5,3.55,-22.86)) ;
#154662=CARTESIAN_POINT('Origin',(-7.29372370581158E-16,3.55,-22.86)) ;
#154663=CARTESIAN_POINT('',(-0.273932138433073,3.45,-21.3852250396981)) ;
#154664=CARTESIAN_POINT('Ctrl Pts',(-0.17080731546662,3.55,-21.3697567779107)) ;
#154665=CARTESIAN_POINT('Ctrl Pts',(-0.183882433427077,3.55,-21.3712554096543)) ;
#154666=CARTESIAN_POINT('Ctrl Pts',(-0.197859036177001,3.54752250383109,
-21.3730511760977)) ;
#154667=CARTESIAN_POINT('Ctrl Pts',(-0.223597793566244,3.53719045839678,
-21.3767006467314)) ;
#154668=CARTESIAN_POINT('Ctrl Pts',(-0.235362682979166,3.52934133421403,
-21.3785504186891)) ;
#154669=CARTESIAN_POINT('Ctrl Pts',(-0.253465441530103,3.51138121637726,
-21.3815429480238)) ;
#154670=CARTESIAN_POINT('Ctrl Pts',(-0.261168570620293,3.50026979217228,
-21.3829034821853)) ;
#154671=CARTESIAN_POINT('Ctrl Pts',(-0.271399896344084,3.47583586070552,
-21.3847463645995)) ;
#154672=CARTESIAN_POINT('Ctrl Pts',(-0.273932138433062,3.46251477070021,
-21.3852250396981)) ;
#154673=CARTESIAN_POINT('Ctrl Pts',(-0.273932138433062,3.45,-21.3852250396981)) ;
#154674=CARTESIAN_POINT('',(-0.273932138433073,3.15,-21.3852250396981)) ;
#154675=CARTESIAN_POINT('',(-0.273932138433073,3.05,-21.3852250396981)) ;
#154676=CARTESIAN_POINT('',(-0.373948193368567,3.05,-21.4073600760421)) ;
#154677=CARTESIAN_POINT('Ctrl Pts',(-0.27393213843307,3.15,-21.3852250396981)) ;
#154678=CARTESIAN_POINT('Ctrl Pts',(-0.27393213843307,3.13744372549049,
-21.3852250396981)) ;
#154679=CARTESIAN_POINT('Ctrl Pts',(-0.276486468486162,3.12408297110069,
-21.3856911302356)) ;
#154680=CARTESIAN_POINT('Ctrl Pts',(-0.286740277640426,3.0995678553947,
-21.3876537789936)) ;
#154681=CARTESIAN_POINT('Ctrl Pts',(-0.294439768310513,3.08841385970397,
-21.3891548411377)) ;
#154682=CARTESIAN_POINT('Ctrl Pts',(-0.312194128344967,3.07061084469361,
-21.392819399951)) ;
#154683=CARTESIAN_POINT('Ctrl Pts',(-0.323517908844212,3.0628422827531,
-21.3952474862748)) ;
#154684=CARTESIAN_POINT('Ctrl Pts',(-0.3481721171233,3.05253676672645,-21.4009138387535)) ;
#154685=CARTESIAN_POINT('Ctrl Pts',(-0.361501722536393,3.05,-21.4041560230592)) ;
#154686=CARTESIAN_POINT('Ctrl Pts',(-0.373948193368565,3.05,-21.4073600760421)) ;
#154687=CARTESIAN_POINT('',(-0.872417476238727,3.05,-21.6398001199995)) ;
#154688=CARTESIAN_POINT('Origin',(-7.95081593156037E-16,3.05,-22.86)) ;
#154689=CARTESIAN_POINT('',(-0.953662978710562,3.15,-21.7021887360036)) ;
#154690=CARTESIAN_POINT('Ctrl Pts',(-0.872417476238732,3.05,-21.6398001199995)) ;
#154691=CARTESIAN_POINT('Ctrl Pts',(-0.882808783297382,3.05,-21.647229687915)) ;
#154692=CARTESIAN_POINT('Ctrl Pts',(-0.893798224191979,3.05250629897269,
-21.6553093623146)) ;
#154693=CARTESIAN_POINT('Ctrl Pts',(-0.913892243159223,3.06269675232156,
-21.6704777691246)) ;
#154694=CARTESIAN_POINT('Ctrl Pts',(-0.922999225059838,3.07038074042647,
-21.6775634285691)) ;
#154695=CARTESIAN_POINT('Ctrl Pts',(-0.93728513413171,3.08810056349785,
-21.6888558711034)) ;
#154696=CARTESIAN_POINT('Ctrl Pts',(-0.94345217439724,3.09929464195085,
-21.693843096804)) ;
#154697=CARTESIAN_POINT('Ctrl Pts',(-0.951639309815367,3.12392729225934,
-21.7005109997964)) ;
#154698=CARTESIAN_POINT('Ctrl Pts',(-0.953662978710565,3.13736547222678,
-21.7021887360036)) ;
#154699=CARTESIAN_POINT('Ctrl Pts',(-0.953662978710565,3.15,-21.7021887360036)) ;
#154700=CARTESIAN_POINT('',(-0.953662978710562,3.45,-21.7021887360036)) ;
#154701=CARTESIAN_POINT('',(-0.953662978710562,3.05,-21.7021887360036)) ;
#154702=CARTESIAN_POINT('',(-1.03179971315145,3.55,-21.7712441265644)) ;
#154703=CARTESIAN_POINT('Ctrl Pts',(-0.953662978710576,3.45,-21.7021887360036)) ;
#154704=CARTESIAN_POINT('Ctrl Pts',(-0.953662978710576,3.4558071514987,
-21.7021887360036)) ;
#154705=CARTESIAN_POINT('Ctrl Pts',(-0.954069792639918,3.4616588096918,
-21.7025236315692)) ;
#154706=CARTESIAN_POINT('Ctrl Pts',(-0.954880405808386,3.46741264967887,
-21.7031927320754)) ;
#154707=CARTESIAN_POINT('Ctrl Pts',(-0.955592557016204,3.47246759358525,
-21.7037805596017)) ;
#154708=CARTESIAN_POINT('Ctrl Pts',(-0.956615573654935,3.47744631522377,
-21.7046258114488)) ;
#154709=CARTESIAN_POINT('Ctrl Pts',(-0.957920385817355,3.48225893605768,
-21.7057086440434)) ;
#154710=CARTESIAN_POINT('Ctrl Pts',(-0.959423079246203,3.48780141482278,
-21.7069556935967)) ;
#154711=CARTESIAN_POINT('Ctrl Pts',(-0.961323201468129,3.49320783601912,
-21.7085374593817)) ;
#154712=CARTESIAN_POINT('Ctrl Pts',(-0.963574238618792,3.49834560049865,
-21.7104242578964)) ;
#154713=CARTESIAN_POINT('Ctrl Pts',(-0.965499706647984,3.50274028640774,
-21.7120381673855)) ;
#154714=CARTESIAN_POINT('Ctrl Pts',(-0.967680912999533,3.50693820669559,
-21.7138745944584)) ;
#154715=CARTESIAN_POINT('Ctrl Pts',(-0.970068248378244,3.51087311165943,
-21.7158987835472)) ;
#154716=CARTESIAN_POINT('Ctrl Pts',(-0.972933246979067,3.51559532091262,
-21.7183279767636)) ;
#154717=CARTESIAN_POINT('Ctrl Pts',(-0.976138831290349,3.52000896466723,
-21.7210646855624)) ;
#154718=CARTESIAN_POINT('Ctrl Pts',(-0.979601776802468,3.52400782220664,
-21.7240509843476)) ;
#154719=CARTESIAN_POINT('Ctrl Pts',(-0.982467725203489,3.52731729367562,
-21.7265224578947)) ;
#154720=CARTESIAN_POINT('Ctrl Pts',(-0.98550898689683,3.5303430569618,-21.7291641736047)) ;
#154721=CARTESIAN_POINT('Ctrl Pts',(-0.988666612105892,3.53304718478134,
-21.7319315933388)) ;
#154722=CARTESIAN_POINT('Ctrl Pts',(-0.992701606803676,3.53650267449008,
-21.7354679610881)) ;
#154723=CARTESIAN_POINT('Ctrl Pts',(-0.996988044734315,3.53948417067185,
-21.7392635881177)) ;
#154724=CARTESIAN_POINT('Ctrl Pts',(-1.00141585135917,3.54192188246042,
-21.7432340352035)) ;
#154725=CARTESIAN_POINT('Ctrl Pts',(-1.00487400994928,3.54382575827887,
-21.7463349916949)) ;
#154726=CARTESIAN_POINT('Ctrl Pts',(-1.00841776012226,3.54539884758398,
-21.7495419608726)) ;
#154727=CARTESIAN_POINT('Ctrl Pts',(-1.01199129263161,3.54662946216441,
-21.7528082263467)) ;
#154728=CARTESIAN_POINT('Ctrl Pts',(-1.01652362695403,3.54819025857132,
-21.7569508519072)) ;
#154729=CARTESIAN_POINT('Ctrl Pts',(-1.02116533136127,3.54921942038457,
-21.7612453631163)) ;
#154730=CARTESIAN_POINT('Ctrl Pts',(-1.0258020962993,3.54969340754028,-21.765591457172)) ;
#154731=CARTESIAN_POINT('Ctrl Pts',(-1.02780524115378,3.54989817637043,
-21.7674690282935)) ;
#154732=CARTESIAN_POINT('Ctrl Pts',(-1.02980744674854,3.55,-21.7693560817297)) ;
#154733=CARTESIAN_POINT('Ctrl Pts',(-1.03179971315146,3.55,-21.7712441265644)) ;
#154734=CARTESIAN_POINT('',(0.170807315466633,3.55,-24.3502432220893)) ;
#154735=CARTESIAN_POINT('Origin',(-7.29372370581158E-16,3.55,-22.86)) ;
#154736=CARTESIAN_POINT('',(0.273932138433074,3.45,-24.3347749603019)) ;
#154737=CARTESIAN_POINT('Ctrl Pts',(0.170807315466623,3.55,-24.3502432220893)) ;
#154738=CARTESIAN_POINT('Ctrl Pts',(0.18388243342708,3.55,-24.3487445903457)) ;
#154739=CARTESIAN_POINT('Ctrl Pts',(0.197859036177004,3.54752250383109,
-24.3469488239023)) ;
#154740=CARTESIAN_POINT('Ctrl Pts',(0.223597793566247,3.53719045839678,
-24.3432993532686)) ;
#154741=CARTESIAN_POINT('Ctrl Pts',(0.235362682979169,3.52934133421403,
-24.3414495813109)) ;
#154742=CARTESIAN_POINT('Ctrl Pts',(0.253465441530107,3.51138121637726,
-24.3384570519762)) ;
#154743=CARTESIAN_POINT('Ctrl Pts',(0.261168570620295,3.50026979217228,
-24.3370965178147)) ;
#154744=CARTESIAN_POINT('Ctrl Pts',(0.271399896344086,3.47583586070552,
-24.3352536354005)) ;
#154745=CARTESIAN_POINT('Ctrl Pts',(0.273932138433066,3.46251477070021,
-24.3347749603019)) ;
#154746=CARTESIAN_POINT('Ctrl Pts',(0.273932138433066,3.45,-24.3347749603019)) ;
#154747=CARTESIAN_POINT('',(0.273932138433074,3.15,-24.3347749603019)) ;
#154748=CARTESIAN_POINT('',(0.273932138433074,3.05,-24.3347749603019)) ;
#154749=CARTESIAN_POINT('',(0.373948193368569,3.05,-24.3126399239579)) ;
#154750=CARTESIAN_POINT('Ctrl Pts',(0.273932138433069,3.15,-24.3347749603019)) ;
#154751=CARTESIAN_POINT('Ctrl Pts',(0.273932138433069,3.13736547222678,
-24.3347749603019)) ;
#154752=CARTESIAN_POINT('Ctrl Pts',(0.276518148223577,3.12392729225934,
-24.3343031680364)) ;
#154753=CARTESIAN_POINT('Ctrl Pts',(0.286888647463776,3.09929464195085,
-24.3323175038704)) ;
#154754=CARTESIAN_POINT('Ctrl Pts',(0.294673181069385,3.08810056349785,
-24.3307990038315)) ;
#154755=CARTESIAN_POINT('Ctrl Pts',(0.312506499266529,3.07038074042647,
-24.3271140047162)) ;
#154756=CARTESIAN_POINT('Ctrl Pts',(0.323788284437175,3.06269675232156,
-24.324692225935)) ;
#154757=CARTESIAN_POINT('Ctrl Pts',(0.348324144605926,3.05250629897269,
-24.3190493783214)) ;
#154758=CARTESIAN_POINT('Ctrl Pts',(0.361577410726384,3.05,-24.3158244927855)) ;
#154759=CARTESIAN_POINT('Ctrl Pts',(0.373948193368564,3.05,-24.3126399239579)) ;
#154760=CARTESIAN_POINT('',(0.872417476238729,3.05,-24.0801998800005)) ;
#154761=CARTESIAN_POINT('Origin',(-7.95081593156037E-16,3.05,-22.86)) ;
#154762=CARTESIAN_POINT('',(0.953662978710562,3.15,-24.0178112639964)) ;
#154763=CARTESIAN_POINT('Ctrl Pts',(0.872417476238731,3.05,-24.0801998800005)) ;
#154764=CARTESIAN_POINT('Ctrl Pts',(0.882872360457021,3.05,-24.0727248557413)) ;
#154765=CARTESIAN_POINT('Ctrl Pts',(0.893924122929508,3.05253676672645,
-24.0645978214856)) ;
#154766=CARTESIAN_POINT('Ctrl Pts',(0.914112220366979,3.0628422827531,-24.0493538633994)) ;
#154767=CARTESIAN_POINT('Ctrl Pts',(0.923251028202473,3.07061084469361,
-24.042240088077)) ;
#154768=CARTESIAN_POINT('Ctrl Pts',(0.937470525765902,3.08841385970397,
-24.0309949922316)) ;
#154769=CARTESIAN_POINT('Ctrl Pts',(0.943569543283853,3.0995678553947,-24.0260617043366)) ;
#154770=CARTESIAN_POINT('Ctrl Pts',(0.951664040935146,3.12408297110069,
-24.0194683971169)) ;
#154771=CARTESIAN_POINT('Ctrl Pts',(0.953662978710564,3.13744372549049,
-24.0178112639964)) ;
#154772=CARTESIAN_POINT('Ctrl Pts',(0.953662978710564,3.15,-24.0178112639964)) ;
#154773=CARTESIAN_POINT('',(0.953662978710562,3.45,-24.0178112639964)) ;
#154774=CARTESIAN_POINT('',(0.953662978710562,3.05,-24.0178112639964)) ;
#154775=CARTESIAN_POINT('',(1.03179971315145,3.55,-23.9487558734356)) ;
#154776=CARTESIAN_POINT('Ctrl Pts',(0.953662978710579,3.45,-24.0178112639964)) ;
#154777=CARTESIAN_POINT('Ctrl Pts',(0.953662978710579,3.4558071514987,-24.0178112639964)) ;
#154778=CARTESIAN_POINT('Ctrl Pts',(0.954069792639922,3.4616588096918,-24.0174763684308)) ;
#154779=CARTESIAN_POINT('Ctrl Pts',(0.954880405808391,3.46741264967887,
-24.0168072679246)) ;
#154780=CARTESIAN_POINT('Ctrl Pts',(0.955592557016209,3.47246759358525,
-24.0162194403983)) ;
#154781=CARTESIAN_POINT('Ctrl Pts',(0.956615573654939,3.47744631522377,
-24.0153741885512)) ;
#154782=CARTESIAN_POINT('Ctrl Pts',(0.957920385817358,3.48225893605767,
-24.0142913559566)) ;
#154783=CARTESIAN_POINT('Ctrl Pts',(0.959423079246211,3.48780141482279,
-24.0130443064033)) ;
#154784=CARTESIAN_POINT('Ctrl Pts',(0.96132320146814,3.49320783601914,-24.0114625406183)) ;
#154785=CARTESIAN_POINT('Ctrl Pts',(0.963574238618814,3.49834560049869,
-24.0095757421036)) ;
#154786=CARTESIAN_POINT('Ctrl Pts',(0.965499706648003,3.50274028640777,
-24.0079618326145)) ;
#154787=CARTESIAN_POINT('Ctrl Pts',(0.967680912999543,3.50693820669559,
-24.0061254055416)) ;
#154788=CARTESIAN_POINT('Ctrl Pts',(0.970068248378244,3.51087311165943,
-24.0041012164528)) ;
#154789=CARTESIAN_POINT('Ctrl Pts',(0.972933246979073,3.51559532091262,
-24.0016720232364)) ;
#154790=CARTESIAN_POINT('Ctrl Pts',(0.976138831290369,3.52000896466725,
-23.9989353144376)) ;
#154791=CARTESIAN_POINT('Ctrl Pts',(0.979601776802496,3.52400782220667,
-23.9959490156524)) ;
#154792=CARTESIAN_POINT('Ctrl Pts',(0.982467725203506,3.52731729367563,
-23.9934775421053)) ;
#154793=CARTESIAN_POINT('Ctrl Pts',(0.985508986896841,3.5303430569618,-23.9908358263953)) ;
#154794=CARTESIAN_POINT('Ctrl Pts',(0.988666612105891,3.53304718478133,
-23.9880684066612)) ;
#154795=CARTESIAN_POINT('Ctrl Pts',(0.992701606803682,3.53650267449008,
-23.984532038912)) ;
#154796=CARTESIAN_POINT('Ctrl Pts',(0.996988044734363,3.53948417067189,
-23.9807364118822)) ;
#154797=CARTESIAN_POINT('Ctrl Pts',(1.0014158513592,3.54192188246045,-23.9767659647964)) ;
#154798=CARTESIAN_POINT('Ctrl Pts',(1.00487400994929,3.54382575827889,-23.973665008305)) ;
#154799=CARTESIAN_POINT('Ctrl Pts',(1.00841776012227,3.54539884758398,-23.9704580391274)) ;
#154800=CARTESIAN_POINT('Ctrl Pts',(1.01199129263161,3.54662946216441,-23.9671917736533)) ;
#154801=CARTESIAN_POINT('Ctrl Pts',(1.01652362695402,3.54819025857132,-23.9630491480928)) ;
#154802=CARTESIAN_POINT('Ctrl Pts',(1.0211653313612,3.54921942038456,-23.9587546368838)) ;
#154803=CARTESIAN_POINT('Ctrl Pts',(1.02580209629924,3.54969340754027,-23.9544085428281)) ;
#154804=CARTESIAN_POINT('Ctrl Pts',(1.02780524115376,3.54989817637043,-23.9525309717066)) ;
#154805=CARTESIAN_POINT('Ctrl Pts',(1.02980744674854,3.55,-23.9506439182703)) ;
#154806=CARTESIAN_POINT('Ctrl Pts',(1.03179971315146,3.55,-23.9487558734356)) ;
#154807=CARTESIAN_POINT('Origin',(-7.29372370581158E-16,3.55,-22.86)) ;
#154808=CARTESIAN_POINT('',(1.5,3.55,-22.86)) ;
#154809=CARTESIAN_POINT('Origin',(-7.29372370581158E-16,3.55,-26.67)) ;
#154810=CARTESIAN_POINT('',(-0.170807315466631,3.55,-25.1797567779107)) ;
#154811=CARTESIAN_POINT('',(1.5,3.55,-26.67)) ;
#154812=CARTESIAN_POINT('Origin',(-7.29372370581158E-16,3.55,-26.67)) ;
#154813=CARTESIAN_POINT('',(-0.273932138433073,3.45,-25.1952250396981)) ;
#154814=CARTESIAN_POINT('Ctrl Pts',(-0.170807315466618,3.55,-25.1797567779107)) ;
#154815=CARTESIAN_POINT('Ctrl Pts',(-0.183882433427076,3.55,-25.1812554096543)) ;
#154816=CARTESIAN_POINT('Ctrl Pts',(-0.197859036176999,3.54752250383109,
-25.1830511760977)) ;
#154817=CARTESIAN_POINT('Ctrl Pts',(-0.223597793566242,3.53719045839678,
-25.1867006467314)) ;
#154818=CARTESIAN_POINT('Ctrl Pts',(-0.235362682979164,3.52934133421403,
-25.1885504186891)) ;
#154819=CARTESIAN_POINT('Ctrl Pts',(-0.253465441530101,3.51138121637726,
-25.1915429480238)) ;
#154820=CARTESIAN_POINT('Ctrl Pts',(-0.261168570620291,3.50026979217228,
-25.1929034821853)) ;
#154821=CARTESIAN_POINT('Ctrl Pts',(-0.271399896344082,3.47583586070552,
-25.1947463645995)) ;
#154822=CARTESIAN_POINT('Ctrl Pts',(-0.27393213843306,3.46251477070021,
-25.1952250396981)) ;
#154823=CARTESIAN_POINT('Ctrl Pts',(-0.27393213843306,3.45,-25.1952250396981)) ;
#154824=CARTESIAN_POINT('',(-0.273932138433073,3.15,-25.1952250396981)) ;
#154825=CARTESIAN_POINT('',(-0.273932138433073,3.05,-25.1952250396981)) ;
#154826=CARTESIAN_POINT('',(-0.373948193368567,3.05,-25.2173600760421)) ;
#154827=CARTESIAN_POINT('Ctrl Pts',(-0.27393213843307,3.15,-25.1952250396981)) ;
#154828=CARTESIAN_POINT('Ctrl Pts',(-0.27393213843307,3.13744372549049,
-25.1952250396981)) ;
#154829=CARTESIAN_POINT('Ctrl Pts',(-0.276486468486162,3.12408297110069,
-25.1956911302356)) ;
#154830=CARTESIAN_POINT('Ctrl Pts',(-0.286740277640426,3.0995678553947,
-25.1976537789936)) ;
#154831=CARTESIAN_POINT('Ctrl Pts',(-0.294439768310513,3.08841385970397,
-25.1991548411377)) ;
#154832=CARTESIAN_POINT('Ctrl Pts',(-0.312194128344967,3.07061084469361,
-25.202819399951)) ;
#154833=CARTESIAN_POINT('Ctrl Pts',(-0.323517908844212,3.0628422827531,
-25.2052474862748)) ;
#154834=CARTESIAN_POINT('Ctrl Pts',(-0.3481721171233,3.05253676672645,-25.2109138387535)) ;
#154835=CARTESIAN_POINT('Ctrl Pts',(-0.361501722536393,3.05,-25.2141560230592)) ;
#154836=CARTESIAN_POINT('Ctrl Pts',(-0.373948193368565,3.05,-25.2173600760421)) ;
#154837=CARTESIAN_POINT('',(-0.872417476238727,3.05,-25.4498001199995)) ;
#154838=CARTESIAN_POINT('Origin',(-7.95081593156037E-16,3.05,-26.67)) ;
#154839=CARTESIAN_POINT('',(-0.953662978710562,3.15,-25.5121887360036)) ;
#154840=CARTESIAN_POINT('Ctrl Pts',(-0.872417476238731,3.05,-25.4498001199995)) ;
#154841=CARTESIAN_POINT('Ctrl Pts',(-0.882808783297381,3.05,-25.457229687915)) ;
#154842=CARTESIAN_POINT('Ctrl Pts',(-0.893798224191978,3.05250629897269,
-25.4653093623146)) ;
#154843=CARTESIAN_POINT('Ctrl Pts',(-0.913892243159222,3.06269675232156,
-25.4804777691246)) ;
#154844=CARTESIAN_POINT('Ctrl Pts',(-0.922999225059836,3.07038074042647,
-25.4875634285691)) ;
#154845=CARTESIAN_POINT('Ctrl Pts',(-0.937285134131708,3.08810056349785,
-25.4988558711034)) ;
#154846=CARTESIAN_POINT('Ctrl Pts',(-0.943452174397238,3.09929464195085,
-25.503843096804)) ;
#154847=CARTESIAN_POINT('Ctrl Pts',(-0.951639309815365,3.12392729225934,
-25.5105109997964)) ;
#154848=CARTESIAN_POINT('Ctrl Pts',(-0.953662978710564,3.13736547222678,
-25.5121887360036)) ;
#154849=CARTESIAN_POINT('Ctrl Pts',(-0.953662978710564,3.15,-25.5121887360036)) ;
#154850=CARTESIAN_POINT('',(-0.953662978710562,3.45,-25.5121887360036)) ;
#154851=CARTESIAN_POINT('',(-0.953662978710562,3.05,-25.5121887360036)) ;
#154852=CARTESIAN_POINT('',(-1.03179971315145,3.55,-25.5812441265644)) ;
#154853=CARTESIAN_POINT('Ctrl Pts',(-0.953662978710574,3.45,-25.5121887360036)) ;
#154854=CARTESIAN_POINT('Ctrl Pts',(-0.953662978710574,3.45580715149871,
-25.5121887360036)) ;
#154855=CARTESIAN_POINT('Ctrl Pts',(-0.954069792639918,3.4616588096918,
-25.5125236315693)) ;
#154856=CARTESIAN_POINT('Ctrl Pts',(-0.954880405808386,3.46741264967887,
-25.5131927320754)) ;
#154857=CARTESIAN_POINT('Ctrl Pts',(-0.955592557016204,3.47246759358525,
-25.5137805596017)) ;
#154858=CARTESIAN_POINT('Ctrl Pts',(-0.956615573654937,3.47744631522377,
-25.5146258114488)) ;
#154859=CARTESIAN_POINT('Ctrl Pts',(-0.957920385817356,3.48225893605768,
-25.5157086440434)) ;
#154860=CARTESIAN_POINT('Ctrl Pts',(-0.959423079246205,3.48780141482278,
-25.5169556935967)) ;
#154861=CARTESIAN_POINT('Ctrl Pts',(-0.96132320146813,3.49320783601912,
-25.5185374593817)) ;
#154862=CARTESIAN_POINT('Ctrl Pts',(-0.963574238618798,3.49834560049866,
-25.5204242578964)) ;
#154863=CARTESIAN_POINT('Ctrl Pts',(-0.96549970664799,3.50274028640775,
-25.5220381673855)) ;
#154864=CARTESIAN_POINT('Ctrl Pts',(-0.967680912999533,3.50693820669559,
-25.5238745944585)) ;
#154865=CARTESIAN_POINT('Ctrl Pts',(-0.970068248378241,3.51087311165943,
-25.5258987835472)) ;
#154866=CARTESIAN_POINT('Ctrl Pts',(-0.972933246979067,3.51559532091262,
-25.5283279767636)) ;
#154867=CARTESIAN_POINT('Ctrl Pts',(-0.976138831290359,3.52000896466724,
-25.5310646855624)) ;
#154868=CARTESIAN_POINT('Ctrl Pts',(-0.97960177680248,3.52400782220665,
-25.5340509843476)) ;
#154869=CARTESIAN_POINT('Ctrl Pts',(-0.982467725203495,3.52731729367562,
-25.5365224578947)) ;
#154870=CARTESIAN_POINT('Ctrl Pts',(-0.985508986896829,3.5303430569618,
-25.5391641736047)) ;
#154871=CARTESIAN_POINT('Ctrl Pts',(-0.988666612105887,3.53304718478133,
-25.5419315933388)) ;
#154872=CARTESIAN_POINT('Ctrl Pts',(-0.992701606803673,3.53650267449007,
-25.5454679610881)) ;
#154873=CARTESIAN_POINT('Ctrl Pts',(-0.996988044734313,3.53948417067185,
-25.5492635881177)) ;
#154874=CARTESIAN_POINT('Ctrl Pts',(-1.00141585135917,3.54192188246042,
-25.5532340352035)) ;
#154875=CARTESIAN_POINT('Ctrl Pts',(-1.00487400994928,3.54382575827887,
-25.5563349916949)) ;
#154876=CARTESIAN_POINT('Ctrl Pts',(-1.00841776012226,3.54539884758398,
-25.5595419608726)) ;
#154877=CARTESIAN_POINT('Ctrl Pts',(-1.01199129263161,3.54662946216441,
-25.5628082263467)) ;
#154878=CARTESIAN_POINT('Ctrl Pts',(-1.016523626954,3.54819025857132,-25.5669508519072)) ;
#154879=CARTESIAN_POINT('Ctrl Pts',(-1.0211653313612,3.54921942038456,-25.5712453631162)) ;
#154880=CARTESIAN_POINT('Ctrl Pts',(-1.02580209629924,3.54969340754027,
-25.5755914571719)) ;
#154881=CARTESIAN_POINT('Ctrl Pts',(-1.02780524115376,3.54989817637043,
-25.5774690282934)) ;
#154882=CARTESIAN_POINT('Ctrl Pts',(-1.02980744674854,3.55,-25.5793560817297)) ;
#154883=CARTESIAN_POINT('Ctrl Pts',(-1.03179971315146,3.55,-25.5812441265644)) ;
#154884=CARTESIAN_POINT('',(0.170807315466633,3.55,-28.1602432220893)) ;
#154885=CARTESIAN_POINT('Origin',(-7.29372370581158E-16,3.55,-26.67)) ;
#154886=CARTESIAN_POINT('',(0.273932138433074,3.45,-28.1447749603019)) ;
#154887=CARTESIAN_POINT('Ctrl Pts',(0.170807315466623,3.55,-28.1602432220893)) ;
#154888=CARTESIAN_POINT('Ctrl Pts',(0.18388243342708,3.55,-28.1587445903457)) ;
#154889=CARTESIAN_POINT('Ctrl Pts',(0.197859036177004,3.54752250383109,
-28.1569488239023)) ;
#154890=CARTESIAN_POINT('Ctrl Pts',(0.223597793566247,3.53719045839678,
-28.1532993532686)) ;
#154891=CARTESIAN_POINT('Ctrl Pts',(0.235362682979169,3.52934133421403,
-28.1514495813109)) ;
#154892=CARTESIAN_POINT('Ctrl Pts',(0.253465441530107,3.51138121637726,
-28.1484570519762)) ;
#154893=CARTESIAN_POINT('Ctrl Pts',(0.261168570620295,3.50026979217228,
-28.1470965178147)) ;
#154894=CARTESIAN_POINT('Ctrl Pts',(0.271399896344086,3.47583586070552,
-28.1452536354005)) ;
#154895=CARTESIAN_POINT('Ctrl Pts',(0.273932138433066,3.46251477070021,
-28.1447749603019)) ;
#154896=CARTESIAN_POINT('Ctrl Pts',(0.273932138433066,3.45,-28.1447749603019)) ;
#154897=CARTESIAN_POINT('',(0.273932138433074,3.15,-28.1447749603019)) ;
#154898=CARTESIAN_POINT('',(0.273932138433074,3.05,-28.1447749603019)) ;
#154899=CARTESIAN_POINT('',(0.373948193368569,3.05,-28.1226399239579)) ;
#154900=CARTESIAN_POINT('Ctrl Pts',(0.273932138433071,3.15,-28.1447749603019)) ;
#154901=CARTESIAN_POINT('Ctrl Pts',(0.273932138433071,3.13736547222678,
-28.1447749603019)) ;
#154902=CARTESIAN_POINT('Ctrl Pts',(0.276518148223579,3.12392729225934,
-28.1443031680364)) ;
#154903=CARTESIAN_POINT('Ctrl Pts',(0.286888647463777,3.09929464195085,
-28.1423175038704)) ;
#154904=CARTESIAN_POINT('Ctrl Pts',(0.294673181069387,3.08810056349785,
-28.1407990038315)) ;
#154905=CARTESIAN_POINT('Ctrl Pts',(0.31250649926653,3.07038074042647,-28.1371140047162)) ;
#154906=CARTESIAN_POINT('Ctrl Pts',(0.323788284437176,3.06269675232156,
-28.134692225935)) ;
#154907=CARTESIAN_POINT('Ctrl Pts',(0.348324144605927,3.05250629897269,
-28.1290493783214)) ;
#154908=CARTESIAN_POINT('Ctrl Pts',(0.361577410726386,3.05,-28.1258244927855)) ;
#154909=CARTESIAN_POINT('Ctrl Pts',(0.373948193368566,3.05,-28.1226399239579)) ;
#154910=CARTESIAN_POINT('',(0.872417476238729,3.05,-27.8901998800005)) ;
#154911=CARTESIAN_POINT('Origin',(-7.95081593156037E-16,3.05,-26.67)) ;
#154912=CARTESIAN_POINT('',(0.953662978710562,3.15,-27.8278112639964)) ;
#154913=CARTESIAN_POINT('Ctrl Pts',(0.872417476238731,3.05,-27.8901998800005)) ;
#154914=CARTESIAN_POINT('Ctrl Pts',(0.882872360457021,3.05,-27.8827248557413)) ;
#154915=CARTESIAN_POINT('Ctrl Pts',(0.893924122929508,3.05253676672645,
-27.8745978214856)) ;
#154916=CARTESIAN_POINT('Ctrl Pts',(0.914112220366979,3.0628422827531,-27.8593538633994)) ;
#154917=CARTESIAN_POINT('Ctrl Pts',(0.923251028202473,3.07061084469361,
-27.852240088077)) ;
#154918=CARTESIAN_POINT('Ctrl Pts',(0.937470525765902,3.08841385970397,
-27.8409949922316)) ;
#154919=CARTESIAN_POINT('Ctrl Pts',(0.943569543283853,3.0995678553947,-27.8360617043366)) ;
#154920=CARTESIAN_POINT('Ctrl Pts',(0.951664040935146,3.12408297110069,
-27.8294683971169)) ;
#154921=CARTESIAN_POINT('Ctrl Pts',(0.953662978710564,3.13744372549049,
-27.8278112639964)) ;
#154922=CARTESIAN_POINT('Ctrl Pts',(0.953662978710564,3.15,-27.8278112639964)) ;
#154923=CARTESIAN_POINT('',(0.953662978710562,3.45,-27.8278112639964)) ;
#154924=CARTESIAN_POINT('',(0.953662978710562,3.05,-27.8278112639964)) ;
#154925=CARTESIAN_POINT('',(1.03179971315145,3.55,-27.7587558734356)) ;
#154926=CARTESIAN_POINT('Ctrl Pts',(0.953662978710579,3.45,-27.8278112639964)) ;
#154927=CARTESIAN_POINT('Ctrl Pts',(0.953662978710579,3.45580715149871,
-27.8278112639964)) ;
#154928=CARTESIAN_POINT('Ctrl Pts',(0.954069792639921,3.4616588096918,-27.8274763684308)) ;
#154929=CARTESIAN_POINT('Ctrl Pts',(0.954880405808391,3.46741264967888,
-27.8268072679246)) ;
#154930=CARTESIAN_POINT('Ctrl Pts',(0.95559255701621,3.47246759358526,-27.8262194403983)) ;
#154931=CARTESIAN_POINT('Ctrl Pts',(0.956615573654943,3.47744631522378,
-27.8253741885512)) ;
#154932=CARTESIAN_POINT('Ctrl Pts',(0.957920385817362,3.48225893605768,
-27.8242913559566)) ;
#154933=CARTESIAN_POINT('Ctrl Pts',(0.959423079246214,3.48780141482278,
-27.8230443064033)) ;
#154934=CARTESIAN_POINT('Ctrl Pts',(0.961323201468142,3.49320783601914,
-27.8214625406183)) ;
#154935=CARTESIAN_POINT('Ctrl Pts',(0.963574238618811,3.49834560049868,
-27.8195757421036)) ;
#154936=CARTESIAN_POINT('Ctrl Pts',(0.965499706647999,3.50274028640776,
-27.8179618326145)) ;
#154937=CARTESIAN_POINT('Ctrl Pts',(0.967680912999544,3.50693820669559,
-27.8161254055416)) ;
#154938=CARTESIAN_POINT('Ctrl Pts',(0.970068248378247,3.51087311165943,
-27.8141012164528)) ;
#154939=CARTESIAN_POINT('Ctrl Pts',(0.972933246979075,3.51559532091262,
-27.8116720232364)) ;
#154940=CARTESIAN_POINT('Ctrl Pts',(0.976138831290371,3.52000896466725,
-27.8089353144376)) ;
#154941=CARTESIAN_POINT('Ctrl Pts',(0.979601776802497,3.52400782220666,
-27.8059490156524)) ;
#154942=CARTESIAN_POINT('Ctrl Pts',(0.982467725203508,3.52731729367563,
-27.8034775421053)) ;
#154943=CARTESIAN_POINT('Ctrl Pts',(0.985508986896839,3.5303430569618,-27.8008358263953)) ;
#154944=CARTESIAN_POINT('Ctrl Pts',(0.98866661210589,3.53304718478133,-27.7980684066612)) ;
#154945=CARTESIAN_POINT('Ctrl Pts',(0.99270160680368,3.53650267449008,-27.7945320389119)) ;
#154946=CARTESIAN_POINT('Ctrl Pts',(0.996988044734364,3.53948417067189,
-27.7907364118822)) ;
#154947=CARTESIAN_POINT('Ctrl Pts',(1.0014158513592,3.54192188246044,-27.7867659647965)) ;
#154948=CARTESIAN_POINT('Ctrl Pts',(1.0048740099493,3.54382575827887,-27.7836650083051)) ;
#154949=CARTESIAN_POINT('Ctrl Pts',(1.00841776012228,3.54539884758398,-27.7804580391274)) ;
#154950=CARTESIAN_POINT('Ctrl Pts',(1.0119912926316,3.5466294621644,-27.7771917736534)) ;
#154951=CARTESIAN_POINT('Ctrl Pts',(1.01652362695395,3.54819025857129,-27.7730491480929)) ;
#154952=CARTESIAN_POINT('Ctrl Pts',(1.02116533136117,3.54921942038455,-27.7687546368838)) ;
#154953=CARTESIAN_POINT('Ctrl Pts',(1.02580209629915,3.54969340754027,-27.7644085428281)) ;
#154954=CARTESIAN_POINT('Ctrl Pts',(1.02780524115368,3.54989817637043,-27.7625309717066)) ;
#154955=CARTESIAN_POINT('Ctrl Pts',(1.02980744674847,3.55,-27.7606439182704)) ;
#154956=CARTESIAN_POINT('Ctrl Pts',(1.03179971315146,3.55,-27.7587558734356)) ;
#154957=CARTESIAN_POINT('Origin',(-7.29372370581158E-16,3.55,-26.67)) ;
#154958=CARTESIAN_POINT('',(1.5,3.55,-26.67)) ;
#154959=CARTESIAN_POINT('Origin',(-7.29372370581158E-16,3.55,-30.48)) ;
#154960=CARTESIAN_POINT('',(-0.170807315466631,3.55,-28.9897567779107)) ;
#154961=CARTESIAN_POINT('',(1.5,3.55,-30.48)) ;
#154962=CARTESIAN_POINT('Origin',(-7.29372370581158E-16,3.55,-30.48)) ;
#154963=CARTESIAN_POINT('',(-0.273932138433073,3.45,-29.0052250396981)) ;
#154964=CARTESIAN_POINT('Ctrl Pts',(-0.17080731546662,3.55,-28.9897567779107)) ;
#154965=CARTESIAN_POINT('Ctrl Pts',(-0.183882433427078,3.55,-28.9912554096543)) ;
#154966=CARTESIAN_POINT('Ctrl Pts',(-0.197859036177001,3.54752250383109,
-28.9930511760977)) ;
#154967=CARTESIAN_POINT('Ctrl Pts',(-0.223597793566244,3.53719045839678,
-28.9967006467314)) ;
#154968=CARTESIAN_POINT('Ctrl Pts',(-0.235362682979166,3.52934133421403,
-28.9985504186891)) ;
#154969=CARTESIAN_POINT('Ctrl Pts',(-0.253465441530102,3.51138121637726,
-29.0015429480238)) ;
#154970=CARTESIAN_POINT('Ctrl Pts',(-0.261168570620293,3.50026979217228,
-29.0029034821853)) ;
#154971=CARTESIAN_POINT('Ctrl Pts',(-0.271399896344084,3.47583586070553,
-29.0047463645995)) ;
#154972=CARTESIAN_POINT('Ctrl Pts',(-0.273932138433062,3.46251477070021,
-29.0052250396981)) ;
#154973=CARTESIAN_POINT('Ctrl Pts',(-0.273932138433062,3.45,-29.0052250396981)) ;
#154974=CARTESIAN_POINT('',(-0.273932138433073,3.15,-29.0052250396981)) ;
#154975=CARTESIAN_POINT('',(-0.273932138433073,3.05,-29.0052250396981)) ;
#154976=CARTESIAN_POINT('',(-0.373948193368567,3.05,-29.0273600760421)) ;
#154977=CARTESIAN_POINT('Ctrl Pts',(-0.27393213843307,3.15,-29.0052250396981)) ;
#154978=CARTESIAN_POINT('Ctrl Pts',(-0.27393213843307,3.13744372549049,
-29.0052250396981)) ;
#154979=CARTESIAN_POINT('Ctrl Pts',(-0.276486468486161,3.12408297110069,
-29.0056911302356)) ;
#154980=CARTESIAN_POINT('Ctrl Pts',(-0.286740277640426,3.0995678553947,
-29.0076537789936)) ;
#154981=CARTESIAN_POINT('Ctrl Pts',(-0.294439768310513,3.08841385970397,
-29.0091548411377)) ;
#154982=CARTESIAN_POINT('Ctrl Pts',(-0.312194128344968,3.07061084469361,
-29.012819399951)) ;
#154983=CARTESIAN_POINT('Ctrl Pts',(-0.323517908844213,3.0628422827531,
-29.0152474862748)) ;
#154984=CARTESIAN_POINT('Ctrl Pts',(-0.348172117123301,3.05253676672645,
-29.0209138387535)) ;
#154985=CARTESIAN_POINT('Ctrl Pts',(-0.361501722536393,3.05,-29.0241560230592)) ;
#154986=CARTESIAN_POINT('Ctrl Pts',(-0.373948193368565,3.05,-29.0273600760421)) ;
#154987=CARTESIAN_POINT('',(-0.872417476238727,3.05,-29.2598001199995)) ;
#154988=CARTESIAN_POINT('Origin',(-7.95081593156037E-16,3.05,-30.48)) ;
#154989=CARTESIAN_POINT('',(-0.953662978710562,3.15,-29.3221887360036)) ;
#154990=CARTESIAN_POINT('Ctrl Pts',(-0.87241747623873,3.05,-29.2598001199995)) ;
#154991=CARTESIAN_POINT('Ctrl Pts',(-0.882808783297378,3.05,-29.267229687915)) ;
#154992=CARTESIAN_POINT('Ctrl Pts',(-0.893798224191981,3.05250629897269,
-29.2753093623146)) ;
#154993=CARTESIAN_POINT('Ctrl Pts',(-0.913892243159222,3.06269675232156,
-29.2904777691246)) ;
#154994=CARTESIAN_POINT('Ctrl Pts',(-0.922999225059836,3.07038074042647,
-29.2975634285691)) ;
#154995=CARTESIAN_POINT('Ctrl Pts',(-0.937285134131708,3.08810056349785,
-29.3088558711034)) ;
#154996=CARTESIAN_POINT('Ctrl Pts',(-0.943452174397237,3.09929464195085,
-29.313843096804)) ;
#154997=CARTESIAN_POINT('Ctrl Pts',(-0.951639309815364,3.12392729225934,
-29.3205109997964)) ;
#154998=CARTESIAN_POINT('Ctrl Pts',(-0.953662978710564,3.13736547222678,
-29.3221887360036)) ;
#154999=CARTESIAN_POINT('Ctrl Pts',(-0.953662978710564,3.15,-29.3221887360036)) ;
#155000=CARTESIAN_POINT('',(-0.953662978710562,3.45,-29.3221887360036)) ;
#155001=CARTESIAN_POINT('',(-0.953662978710562,3.05,-29.3221887360036)) ;
#155002=CARTESIAN_POINT('',(-1.03179971315145,3.55,-29.3912441265644)) ;
#155003=CARTESIAN_POINT('Ctrl Pts',(-0.953662978710576,3.45,-29.3221887360036)) ;
#155004=CARTESIAN_POINT('Ctrl Pts',(-0.953662978710576,3.4558071514987,
-29.3221887360036)) ;
#155005=CARTESIAN_POINT('Ctrl Pts',(-0.954069792639918,3.4616588096918,
-29.3225236315693)) ;
#155006=CARTESIAN_POINT('Ctrl Pts',(-0.954880405808387,3.46741264967887,
-29.3231927320754)) ;
#155007=CARTESIAN_POINT('Ctrl Pts',(-0.955592557016205,3.47246759358525,
-29.3237805596017)) ;
#155008=CARTESIAN_POINT('Ctrl Pts',(-0.956615573654937,3.47744631522377,
-29.3246258114488)) ;
#155009=CARTESIAN_POINT('Ctrl Pts',(-0.957920385817357,3.48225893605768,
-29.3257086440434)) ;
#155010=CARTESIAN_POINT('Ctrl Pts',(-0.959423079246206,3.48780141482278,
-29.3269556935967)) ;
#155011=CARTESIAN_POINT('Ctrl Pts',(-0.961323201468129,3.49320783601912,
-29.3285374593817)) ;
#155012=CARTESIAN_POINT('Ctrl Pts',(-0.963574238618794,3.49834560049866,
-29.3304242578964)) ;
#155013=CARTESIAN_POINT('Ctrl Pts',(-0.965499706647985,3.50274028640774,
-29.3320381673855)) ;
#155014=CARTESIAN_POINT('Ctrl Pts',(-0.967680912999537,3.50693820669559,
-29.3338745944584)) ;
#155015=CARTESIAN_POINT('Ctrl Pts',(-0.970068248378244,3.51087311165943,
-29.3358987835472)) ;
#155016=CARTESIAN_POINT('Ctrl Pts',(-0.972933246979068,3.51559532091262,
-29.3383279767636)) ;
#155017=CARTESIAN_POINT('Ctrl Pts',(-0.976138831290358,3.52000896466724,
-29.3410646855624)) ;
#155018=CARTESIAN_POINT('Ctrl Pts',(-0.979601776802481,3.52400782220665,
-29.3440509843476)) ;
#155019=CARTESIAN_POINT('Ctrl Pts',(-0.982467725203497,3.52731729367563,
-29.3465224578947)) ;
#155020=CARTESIAN_POINT('Ctrl Pts',(-0.985508986896832,3.5303430569618,
-29.3491641736047)) ;
#155021=CARTESIAN_POINT('Ctrl Pts',(-0.988666612105887,3.53304718478133,
-29.3519315933388)) ;
#155022=CARTESIAN_POINT('Ctrl Pts',(-0.992701606803678,3.53650267449008,
-29.3554679610881)) ;
#155023=CARTESIAN_POINT('Ctrl Pts',(-0.996988044734361,3.53948417067189,
-29.3592635881178)) ;
#155024=CARTESIAN_POINT('Ctrl Pts',(-1.0014158513592,3.54192188246045,-29.3632340352036)) ;
#155025=CARTESIAN_POINT('Ctrl Pts',(-1.00487400994929,3.54382575827889,
-29.366334991695)) ;
#155026=CARTESIAN_POINT('Ctrl Pts',(-1.00841776012226,3.54539884758397,
-29.3695419608726)) ;
#155027=CARTESIAN_POINT('Ctrl Pts',(-1.01199129263159,3.5466294621644,-29.3728082263467)) ;
#155028=CARTESIAN_POINT('Ctrl Pts',(-1.01652362695395,3.54819025857129,
-29.3769508519071)) ;
#155029=CARTESIAN_POINT('Ctrl Pts',(-1.02116533136117,3.54921942038455,
-29.3812453631162)) ;
#155030=CARTESIAN_POINT('Ctrl Pts',(-1.02580209629915,3.54969340754027,
-29.3855914571719)) ;
#155031=CARTESIAN_POINT('Ctrl Pts',(-1.02780524115368,3.54989817637043,
-29.3874690282934)) ;
#155032=CARTESIAN_POINT('Ctrl Pts',(-1.02980744674846,3.55,-29.3893560817296)) ;
#155033=CARTESIAN_POINT('Ctrl Pts',(-1.03179971315146,3.55,-29.3912441265644)) ;
#155034=CARTESIAN_POINT('',(0.170807315466633,3.55,-31.9702432220893)) ;
#155035=CARTESIAN_POINT('Origin',(-7.29372370581158E-16,3.55,-30.48)) ;
#155036=CARTESIAN_POINT('',(0.273932138433074,3.45,-31.9547749603019)) ;
#155037=CARTESIAN_POINT('Ctrl Pts',(0.17080731546662,3.55,-31.9702432220893)) ;
#155038=CARTESIAN_POINT('Ctrl Pts',(0.183882433427078,3.55,-31.9687445903457)) ;
#155039=CARTESIAN_POINT('Ctrl Pts',(0.197859036177002,3.54752250383109,
-31.9669488239023)) ;
#155040=CARTESIAN_POINT('Ctrl Pts',(0.223597793566245,3.53719045839678,
-31.9632993532686)) ;
#155041=CARTESIAN_POINT('Ctrl Pts',(0.235362682979166,3.52934133421403,
-31.9614495813109)) ;
#155042=CARTESIAN_POINT('Ctrl Pts',(0.253465441530103,3.51138121637726,
-31.9584570519762)) ;
#155043=CARTESIAN_POINT('Ctrl Pts',(0.261168570620294,3.50026979217228,
-31.9570965178147)) ;
#155044=CARTESIAN_POINT('Ctrl Pts',(0.271399896344085,3.47583586070553,
-31.9552536354005)) ;
#155045=CARTESIAN_POINT('Ctrl Pts',(0.273932138433063,3.46251477070021,
-31.9547749603019)) ;
#155046=CARTESIAN_POINT('Ctrl Pts',(0.273932138433063,3.45,-31.9547749603019)) ;
#155047=CARTESIAN_POINT('',(0.273932138433074,3.15,-31.9547749603019)) ;
#155048=CARTESIAN_POINT('',(0.273932138433074,3.05,-31.9547749603019)) ;
#155049=CARTESIAN_POINT('',(0.373948193368569,3.05,-31.9326399239579)) ;
#155050=CARTESIAN_POINT('Ctrl Pts',(0.273932138433071,3.15,-31.9547749603019)) ;
#155051=CARTESIAN_POINT('Ctrl Pts',(0.273932138433071,3.13736547222678,
-31.9547749603019)) ;
#155052=CARTESIAN_POINT('Ctrl Pts',(0.276518148223577,3.12392729225934,
-31.9543031680363)) ;
#155053=CARTESIAN_POINT('Ctrl Pts',(0.286888647463776,3.09929464195085,
-31.9523175038703)) ;
#155054=CARTESIAN_POINT('Ctrl Pts',(0.294673181069387,3.08810056349785,
-31.9507990038315)) ;
#155055=CARTESIAN_POINT('Ctrl Pts',(0.31250649926653,3.07038074042647,-31.9471140047162)) ;
#155056=CARTESIAN_POINT('Ctrl Pts',(0.323788284437177,3.06269675232156,
-31.944692225935)) ;
#155057=CARTESIAN_POINT('Ctrl Pts',(0.348324144605927,3.05250629897269,
-31.9390493783214)) ;
#155058=CARTESIAN_POINT('Ctrl Pts',(0.361577410726386,3.05,-31.9358244927855)) ;
#155059=CARTESIAN_POINT('Ctrl Pts',(0.373948193368566,3.05,-31.9326399239579)) ;
#155060=CARTESIAN_POINT('',(0.87241747623873,3.05,-31.7001998800005)) ;
#155061=CARTESIAN_POINT('Origin',(-7.95081593156037E-16,3.05,-30.48)) ;
#155062=CARTESIAN_POINT('',(0.953662978710562,3.15,-31.6378112639964)) ;
#155063=CARTESIAN_POINT('Ctrl Pts',(0.872417476238731,3.05,-31.7001998800005)) ;
#155064=CARTESIAN_POINT('Ctrl Pts',(0.882872360457021,3.05,-31.6927248557413)) ;
#155065=CARTESIAN_POINT('Ctrl Pts',(0.893924122929511,3.05253676672645,
-31.6845978214856)) ;
#155066=CARTESIAN_POINT('Ctrl Pts',(0.914112220366982,3.0628422827531,-31.6693538633994)) ;
#155067=CARTESIAN_POINT('Ctrl Pts',(0.923251028202473,3.07061084469361,
-31.662240088077)) ;
#155068=CARTESIAN_POINT('Ctrl Pts',(0.937470525765902,3.08841385970397,
-31.6509949922316)) ;
#155069=CARTESIAN_POINT('Ctrl Pts',(0.943569543283852,3.0995678553947,-31.6460617043366)) ;
#155070=CARTESIAN_POINT('Ctrl Pts',(0.951664040935145,3.12408297110069,
-31.6394683971169)) ;
#155071=CARTESIAN_POINT('Ctrl Pts',(0.953662978710564,3.13744372549049,
-31.6378112639964)) ;
#155072=CARTESIAN_POINT('Ctrl Pts',(0.953662978710564,3.15,-31.6378112639964)) ;
#155073=CARTESIAN_POINT('',(0.953662978710562,3.45,-31.6378112639964)) ;
#155074=CARTESIAN_POINT('',(0.953662978710562,3.05,-31.6378112639964)) ;
#155075=CARTESIAN_POINT('',(1.03179971315145,3.55,-31.5687558734356)) ;
#155076=CARTESIAN_POINT('Ctrl Pts',(0.953662978710579,3.45,-31.6378112639964)) ;
#155077=CARTESIAN_POINT('Ctrl Pts',(0.953662978710579,3.4558071514987,-31.6378112639964)) ;
#155078=CARTESIAN_POINT('Ctrl Pts',(0.954069792639918,3.46165880969179,
-31.6374763684308)) ;
#155079=CARTESIAN_POINT('Ctrl Pts',(0.954880405808387,3.46741264967886,
-31.6368072679246)) ;
#155080=CARTESIAN_POINT('Ctrl Pts',(0.955592557016206,3.47246759358525,
-31.6362194403983)) ;
#155081=CARTESIAN_POINT('Ctrl Pts',(0.956615573654938,3.47744631522377,
-31.6353741885512)) ;
#155082=CARTESIAN_POINT('Ctrl Pts',(0.957920385817359,3.48225893605768,
-31.6342913559566)) ;
#155083=CARTESIAN_POINT('Ctrl Pts',(0.959423079246214,3.48780141482279,
-31.6330443064033)) ;
#155084=CARTESIAN_POINT('Ctrl Pts',(0.96132320146816,3.49320783601916,-31.6314625406184)) ;
#155085=CARTESIAN_POINT('Ctrl Pts',(0.963574238618836,3.49834560049872,
-31.6295757421036)) ;
#155086=CARTESIAN_POINT('Ctrl Pts',(0.965499706648023,3.50274028640779,
-31.6279618326145)) ;
#155087=CARTESIAN_POINT('Ctrl Pts',(0.967680912999547,3.5069382066956,-31.6261254055416)) ;
#155088=CARTESIAN_POINT('Ctrl Pts',(0.970068248378247,3.51087311165943,
-31.6241012164528)) ;
#155089=CARTESIAN_POINT('Ctrl Pts',(0.972933246979074,3.51559532091262,
-31.6216720232364)) ;
#155090=CARTESIAN_POINT('Ctrl Pts',(0.976138831290361,3.52000896466724,
-31.6189353144376)) ;
#155091=CARTESIAN_POINT('Ctrl Pts',(0.979601776802483,3.52400782220665,
-31.6159490156524)) ;
#155092=CARTESIAN_POINT('Ctrl Pts',(0.982467725203497,3.52731729367562,
-31.6134775421053)) ;
#155093=CARTESIAN_POINT('Ctrl Pts',(0.985508986896839,3.5303430569618,-31.6108358263953)) ;
#155094=CARTESIAN_POINT('Ctrl Pts',(0.988666612105884,3.53304718478132,
-31.6080684066612)) ;
#155095=CARTESIAN_POINT('Ctrl Pts',(0.992701606803627,3.53650267449002,
-31.604532038912)) ;
#155096=CARTESIAN_POINT('Ctrl Pts',(0.996988044734275,3.53948417067183,
-31.6007364118823)) ;
#155097=CARTESIAN_POINT('Ctrl Pts',(1.0014158513591,3.54192188246038,-31.5967659647965)) ;
#155098=CARTESIAN_POINT('Ctrl Pts',(1.00487400994924,3.54382575827886,-31.5936650083051)) ;
#155099=CARTESIAN_POINT('Ctrl Pts',(1.00841776012224,3.54539884758397,-31.5904580391274)) ;
#155100=CARTESIAN_POINT('Ctrl Pts',(1.01199129263162,3.54662946216441,-31.5871917736533)) ;
#155101=CARTESIAN_POINT('Ctrl Pts',(1.01652362695402,3.54819025857132,-31.5830491480928)) ;
#155102=CARTESIAN_POINT('Ctrl Pts',(1.02116533136121,3.54921942038456,-31.5787546368838)) ;
#155103=CARTESIAN_POINT('Ctrl Pts',(1.02580209629926,3.54969340754028,-31.5744085428281)) ;
#155104=CARTESIAN_POINT('Ctrl Pts',(1.02780524115377,3.54989817637043,-31.5725309717066)) ;
#155105=CARTESIAN_POINT('Ctrl Pts',(1.02980744674854,3.55,-31.5706439182703)) ;
#155106=CARTESIAN_POINT('Ctrl Pts',(1.03179971315146,3.55,-31.5687558734356)) ;
#155107=CARTESIAN_POINT('Origin',(-7.29372370581158E-16,3.55,-30.48)) ;
#155108=CARTESIAN_POINT('',(1.5,3.55,-30.48)) ;
#155109=CARTESIAN_POINT('Origin',(-7.29372370581158E-16,3.55,-34.29)) ;
#155110=CARTESIAN_POINT('',(-0.170807315466631,3.55,-32.7997567779107)) ;
#155111=CARTESIAN_POINT('',(1.5,3.55,-34.29)) ;
#155112=CARTESIAN_POINT('Origin',(-7.29372370581158E-16,3.55,-34.29)) ;
#155113=CARTESIAN_POINT('',(-0.273932138433073,3.45,-32.8152250396981)) ;
#155114=CARTESIAN_POINT('Ctrl Pts',(-0.17080731546662,3.55,-32.7997567779107)) ;
#155115=CARTESIAN_POINT('Ctrl Pts',(-0.183882433427078,3.55,-32.8012554096543)) ;
#155116=CARTESIAN_POINT('Ctrl Pts',(-0.197859036177001,3.54752250383109,
-32.8030511760977)) ;
#155117=CARTESIAN_POINT('Ctrl Pts',(-0.223597793566244,3.53719045839678,
-32.8067006467314)) ;
#155118=CARTESIAN_POINT('Ctrl Pts',(-0.235362682979166,3.52934133421403,
-32.8085504186891)) ;
#155119=CARTESIAN_POINT('Ctrl Pts',(-0.253465441530102,3.51138121637726,
-32.8115429480238)) ;
#155120=CARTESIAN_POINT('Ctrl Pts',(-0.261168570620293,3.50026979217228,
-32.8129034821853)) ;
#155121=CARTESIAN_POINT('Ctrl Pts',(-0.271399896344084,3.47583586070553,
-32.8147463645995)) ;
#155122=CARTESIAN_POINT('Ctrl Pts',(-0.273932138433062,3.46251477070021,
-32.8152250396981)) ;
#155123=CARTESIAN_POINT('Ctrl Pts',(-0.273932138433062,3.45,-32.8152250396981)) ;
#155124=CARTESIAN_POINT('',(-0.273932138433073,3.15,-32.8152250396981)) ;
#155125=CARTESIAN_POINT('',(-0.273932138433073,3.05,-32.8152250396981)) ;
#155126=CARTESIAN_POINT('',(-0.373948193368568,3.05,-32.8373600760421)) ;
#155127=CARTESIAN_POINT('Ctrl Pts',(-0.27393213843307,3.15,-32.8152250396981)) ;
#155128=CARTESIAN_POINT('Ctrl Pts',(-0.27393213843307,3.13744372549049,
-32.8152250396981)) ;
#155129=CARTESIAN_POINT('Ctrl Pts',(-0.276486468486161,3.12408297110069,
-32.8156911302356)) ;
#155130=CARTESIAN_POINT('Ctrl Pts',(-0.286740277640426,3.0995678553947,
-32.8176537789936)) ;
#155131=CARTESIAN_POINT('Ctrl Pts',(-0.294439768310513,3.08841385970397,
-32.8191548411377)) ;
#155132=CARTESIAN_POINT('Ctrl Pts',(-0.312194128344968,3.07061084469361,
-32.822819399951)) ;
#155133=CARTESIAN_POINT('Ctrl Pts',(-0.323517908844213,3.0628422827531,
-32.8252474862748)) ;
#155134=CARTESIAN_POINT('Ctrl Pts',(-0.348172117123301,3.05253676672645,
-32.8309138387535)) ;
#155135=CARTESIAN_POINT('Ctrl Pts',(-0.361501722536393,3.05,-32.8341560230592)) ;
#155136=CARTESIAN_POINT('Ctrl Pts',(-0.373948193368565,3.05,-32.8373600760421)) ;
#155137=CARTESIAN_POINT('',(-0.872417476238727,3.05,-33.0698001199995)) ;
#155138=CARTESIAN_POINT('Origin',(-7.95081593156037E-16,3.05,-34.29)) ;
#155139=CARTESIAN_POINT('',(-0.953662978710562,3.15,-33.1321887360036)) ;
#155140=CARTESIAN_POINT('Ctrl Pts',(-0.872417476238729,3.05,-33.0698001199995)) ;
#155141=CARTESIAN_POINT('Ctrl Pts',(-0.882808783297379,3.05,-33.077229687915)) ;
#155142=CARTESIAN_POINT('Ctrl Pts',(-0.893798224191978,3.05250629897269,
-33.0853093623146)) ;
#155143=CARTESIAN_POINT('Ctrl Pts',(-0.913892243159221,3.06269675232156,
-33.1004777691246)) ;
#155144=CARTESIAN_POINT('Ctrl Pts',(-0.922999225059835,3.07038074042647,
-33.1075634285691)) ;
#155145=CARTESIAN_POINT('Ctrl Pts',(-0.937285134131707,3.08810056349785,
-33.1188558711034)) ;
#155146=CARTESIAN_POINT('Ctrl Pts',(-0.943452174397235,3.09929464195085,
-33.123843096804)) ;
#155147=CARTESIAN_POINT('Ctrl Pts',(-0.951639309815362,3.12392729225934,
-33.1305109997964)) ;
#155148=CARTESIAN_POINT('Ctrl Pts',(-0.953662978710562,3.13736547222678,
-33.1321887360036)) ;
#155149=CARTESIAN_POINT('Ctrl Pts',(-0.953662978710562,3.15,-33.1321887360036)) ;
#155150=CARTESIAN_POINT('',(-0.953662978710562,3.45,-33.1321887360036)) ;
#155151=CARTESIAN_POINT('',(-0.953662978710562,3.05,-33.1321887360036)) ;
#155152=CARTESIAN_POINT('',(-1.03179971315145,3.55,-33.2012441265644)) ;
#155153=CARTESIAN_POINT('Ctrl Pts',(-0.953662978710574,3.45,-33.1321887360036)) ;
#155154=CARTESIAN_POINT('Ctrl Pts',(-0.953662978710574,3.45580715149871,
-33.1321887360036)) ;
#155155=CARTESIAN_POINT('Ctrl Pts',(-0.954069792639916,3.46165880969181,
-33.1325236315692)) ;
#155156=CARTESIAN_POINT('Ctrl Pts',(-0.954880405808388,3.46741264967889,
-33.1331927320754)) ;
#155157=CARTESIAN_POINT('Ctrl Pts',(-0.955592557016207,3.47246759358527,
-33.1337805596017)) ;
#155158=CARTESIAN_POINT('Ctrl Pts',(-0.956615573654936,3.47744631522378,
-33.1346258114488)) ;
#155159=CARTESIAN_POINT('Ctrl Pts',(-0.957920385817355,3.48225893605768,
-33.1357086440434)) ;
#155160=CARTESIAN_POINT('Ctrl Pts',(-0.959423079246211,3.4878014148228,
-33.1369556935967)) ;
#155161=CARTESIAN_POINT('Ctrl Pts',(-0.96132320146816,3.49320783601917,
-33.1385374593816)) ;
#155162=CARTESIAN_POINT('Ctrl Pts',(-0.96357423861884,3.49834560049873,
-33.1404242578964)) ;
#155163=CARTESIAN_POINT('Ctrl Pts',(-0.965499706648026,3.5027402864078,
-33.1420381673855)) ;
#155164=CARTESIAN_POINT('Ctrl Pts',(-0.967680912999544,3.5069382066956,
-33.1438745944585)) ;
#155165=CARTESIAN_POINT('Ctrl Pts',(-0.970068248378232,3.51087311165944,
-33.1458987835473)) ;
#155166=CARTESIAN_POINT('Ctrl Pts',(-0.972933246979047,3.51559532091265,
-33.1483279767637)) ;
#155167=CARTESIAN_POINT('Ctrl Pts',(-0.976138831290362,3.52000896466724,
-33.1510646855624)) ;
#155168=CARTESIAN_POINT('Ctrl Pts',(-0.979601776802488,3.52400782220666,
-33.1540509843476)) ;
#155169=CARTESIAN_POINT('Ctrl Pts',(-0.982467725203504,3.52731729367563,
-33.1565224578947)) ;
#155170=CARTESIAN_POINT('Ctrl Pts',(-0.985508986896833,3.5303430569618,
-33.1591641736047)) ;
#155171=CARTESIAN_POINT('Ctrl Pts',(-0.988666612105891,3.53304718478134,
-33.1619315933388)) ;
#155172=CARTESIAN_POINT('Ctrl Pts',(-0.992701606803667,3.53650267449007,
-33.1654679610881)) ;
#155173=CARTESIAN_POINT('Ctrl Pts',(-0.996988044734294,3.53948417067184,
-33.1692635881177)) ;
#155174=CARTESIAN_POINT('Ctrl Pts',(-1.00141585135913,3.5419218824604,-33.1732340352035)) ;
#155175=CARTESIAN_POINT('Ctrl Pts',(-1.00487400994926,3.54382575827887,
-33.1763349916949)) ;
#155176=CARTESIAN_POINT('Ctrl Pts',(-1.00841776012225,3.54539884758397,
-33.1795419608726)) ;
#155177=CARTESIAN_POINT('Ctrl Pts',(-1.0119912926316,3.54662946216441,-33.1828082263467)) ;
#155178=CARTESIAN_POINT('Ctrl Pts',(-1.01652362695394,3.54819025857129,
-33.1869508519071)) ;
#155179=CARTESIAN_POINT('Ctrl Pts',(-1.0211653313611,3.54921942038454,-33.1912453631161)) ;
#155180=CARTESIAN_POINT('Ctrl Pts',(-1.02580209629909,3.54969340754026,
-33.1955914571718)) ;
#155181=CARTESIAN_POINT('Ctrl Pts',(-1.02780524115366,3.54989817637043,
-33.1974690282933)) ;
#155182=CARTESIAN_POINT('Ctrl Pts',(-1.02980744674846,3.55,-33.1993560817296)) ;
#155183=CARTESIAN_POINT('Ctrl Pts',(-1.03179971315146,3.55,-33.2012441265644)) ;
#155184=CARTESIAN_POINT('',(0.170807315466633,3.55,-35.7802432220893)) ;
#155185=CARTESIAN_POINT('Origin',(-7.29372370581158E-16,3.55,-34.29)) ;
#155186=CARTESIAN_POINT('',(0.273932138433074,3.45,-35.7647749603019)) ;
#155187=CARTESIAN_POINT('Ctrl Pts',(0.170807315466624,3.55,-35.7802432220893)) ;
#155188=CARTESIAN_POINT('Ctrl Pts',(0.183882433427082,3.55,-35.7787445903457)) ;
#155189=CARTESIAN_POINT('Ctrl Pts',(0.197859036177005,3.54752250383108,
-35.7769488239023)) ;
#155190=CARTESIAN_POINT('Ctrl Pts',(0.223597793566249,3.53719045839678,
-35.7732993532686)) ;
#155191=CARTESIAN_POINT('Ctrl Pts',(0.235362682979172,3.52934133421403,
-35.7714495813109)) ;
#155192=CARTESIAN_POINT('Ctrl Pts',(0.253465441530109,3.51138121637726,
-35.7684570519762)) ;
#155193=CARTESIAN_POINT('Ctrl Pts',(0.261168570620297,3.50026979217228,
-35.7670965178147)) ;
#155194=CARTESIAN_POINT('Ctrl Pts',(0.271399896344088,3.47583586070552,
-35.7652536354005)) ;
#155195=CARTESIAN_POINT('Ctrl Pts',(0.273932138433068,3.46251477070021,
-35.7647749603019)) ;
#155196=CARTESIAN_POINT('Ctrl Pts',(0.273932138433068,3.45,-35.7647749603019)) ;
#155197=CARTESIAN_POINT('',(0.273932138433074,3.15,-35.7647749603019)) ;
#155198=CARTESIAN_POINT('',(0.273932138433074,3.05,-35.7647749603019)) ;
#155199=CARTESIAN_POINT('',(0.373948193368569,3.05,-35.7426399239579)) ;
#155200=CARTESIAN_POINT('Ctrl Pts',(0.273932138433073,3.15,-35.7647749603019)) ;
#155201=CARTESIAN_POINT('Ctrl Pts',(0.273932138433073,3.13736547222678,
-35.7647749603019)) ;
#155202=CARTESIAN_POINT('Ctrl Pts',(0.276518148223579,3.12392729225934,
-35.7643031680363)) ;
#155203=CARTESIAN_POINT('Ctrl Pts',(0.286888647463778,3.09929464195085,
-35.7623175038703)) ;
#155204=CARTESIAN_POINT('Ctrl Pts',(0.294673181069389,3.08810056349785,
-35.7607990038315)) ;
#155205=CARTESIAN_POINT('Ctrl Pts',(0.312506499266532,3.07038074042647,
-35.7571140047162)) ;
#155206=CARTESIAN_POINT('Ctrl Pts',(0.323788284437179,3.06269675232156,
-35.754692225935)) ;
#155207=CARTESIAN_POINT('Ctrl Pts',(0.348324144605929,3.05250629897269,
-35.7490493783214)) ;
#155208=CARTESIAN_POINT('Ctrl Pts',(0.361577410726388,3.05,-35.7458244927855)) ;
#155209=CARTESIAN_POINT('Ctrl Pts',(0.373948193368567,3.05,-35.7426399239579)) ;
#155210=CARTESIAN_POINT('',(0.872417476238728,3.05,-35.5101998800005)) ;
#155211=CARTESIAN_POINT('Origin',(-7.95081593156037E-16,3.05,-34.29)) ;
#155212=CARTESIAN_POINT('',(0.953662978710562,3.15,-35.4478112639964)) ;
#155213=CARTESIAN_POINT('Ctrl Pts',(0.872417476238731,3.05,-35.5101998800005)) ;
#155214=CARTESIAN_POINT('Ctrl Pts',(0.882872360457019,3.05,-35.5027248557413)) ;
#155215=CARTESIAN_POINT('Ctrl Pts',(0.893924122929511,3.05253676672645,
-35.4945978214856)) ;
#155216=CARTESIAN_POINT('Ctrl Pts',(0.914112220366982,3.0628422827531,-35.4793538633994)) ;
#155217=CARTESIAN_POINT('Ctrl Pts',(0.923251028202473,3.07061084469361,
-35.472240088077)) ;
#155218=CARTESIAN_POINT('Ctrl Pts',(0.937470525765902,3.08841385970397,
-35.4609949922316)) ;
#155219=CARTESIAN_POINT('Ctrl Pts',(0.943569543283852,3.0995678553947,-35.4560617043366)) ;
#155220=CARTESIAN_POINT('Ctrl Pts',(0.951664040935145,3.12408297110069,
-35.4494683971169)) ;
#155221=CARTESIAN_POINT('Ctrl Pts',(0.953662978710564,3.13744372549049,
-35.4478112639964)) ;
#155222=CARTESIAN_POINT('Ctrl Pts',(0.953662978710564,3.15,-35.4478112639964)) ;
#155223=CARTESIAN_POINT('',(0.953662978710562,3.45,-35.4478112639964)) ;
#155224=CARTESIAN_POINT('',(0.953662978710562,3.05,-35.4478112639964)) ;
#155225=CARTESIAN_POINT('',(1.03179971315145,3.55,-35.3787558734356)) ;
#155226=CARTESIAN_POINT('Ctrl Pts',(0.953662978710577,3.45,-35.4478112639964)) ;
#155227=CARTESIAN_POINT('Ctrl Pts',(0.953662978710577,3.4558071514987,-35.4478112639964)) ;
#155228=CARTESIAN_POINT('Ctrl Pts',(0.95406979263992,3.4616588096918,-35.4474763684308)) ;
#155229=CARTESIAN_POINT('Ctrl Pts',(0.954880405808407,3.46741264967886,
-35.4468072679247)) ;
#155230=CARTESIAN_POINT('Ctrl Pts',(0.955592557016242,3.47246759358524,
-35.4462194403984)) ;
#155231=CARTESIAN_POINT('Ctrl Pts',(0.956615573654938,3.47744631522377,
-35.4453741885512)) ;
#155232=CARTESIAN_POINT('Ctrl Pts',(0.957920385817358,3.48225893605768,
-35.4442913559566)) ;
#155233=CARTESIAN_POINT('Ctrl Pts',(0.95942307924621,3.48780141482279,-35.4430443064033)) ;
#155234=CARTESIAN_POINT('Ctrl Pts',(0.961323201468138,3.49320783601914,
-35.4414625406184)) ;
#155235=CARTESIAN_POINT('Ctrl Pts',(0.96357423861882,3.49834560049869,-35.4395757421036)) ;
#155236=CARTESIAN_POINT('Ctrl Pts',(0.965499706648018,3.50274028640778,
-35.4379618326146)) ;
#155237=CARTESIAN_POINT('Ctrl Pts',(0.96768091299954,3.50693820669559,-35.4361254055416)) ;
#155238=CARTESIAN_POINT('Ctrl Pts',(0.970068248378245,3.51087311165943,
-35.4341012164528)) ;
#155239=CARTESIAN_POINT('Ctrl Pts',(0.972933246979074,3.51559532091262,
-35.4316720232364)) ;
#155240=CARTESIAN_POINT('Ctrl Pts',(0.976138831290363,3.52000896466724,
-35.4289353144376)) ;
#155241=CARTESIAN_POINT('Ctrl Pts',(0.979601776802487,3.52400782220666,
-35.4259490156524)) ;
#155242=CARTESIAN_POINT('Ctrl Pts',(0.982467725203501,3.52731729367563,
-35.4234775421053)) ;
#155243=CARTESIAN_POINT('Ctrl Pts',(0.985508986896839,3.5303430569618,-35.4208358263953)) ;
#155244=CARTESIAN_POINT('Ctrl Pts',(0.988666612105879,3.53304718478133,
-35.4180684066612)) ;
#155245=CARTESIAN_POINT('Ctrl Pts',(0.992701606803641,3.53650267449006,
-35.414532038912)) ;
#155246=CARTESIAN_POINT('Ctrl Pts',(0.996988044734314,3.53948417067185,
-35.4107364118823)) ;
#155247=CARTESIAN_POINT('Ctrl Pts',(1.00141585135917,3.54192188246041,-35.4067659647965)) ;
#155248=CARTESIAN_POINT('Ctrl Pts',(1.00487400994928,3.54382575827887,-35.4036650083051)) ;
#155249=CARTESIAN_POINT('Ctrl Pts',(1.00841776012226,3.54539884758398,-35.4004580391274)) ;
#155250=CARTESIAN_POINT('Ctrl Pts',(1.01199129263161,3.54662946216441,-35.3971917736533)) ;
#155251=CARTESIAN_POINT('Ctrl Pts',(1.01652362695402,3.54819025857132,-35.3930491480928)) ;
#155252=CARTESIAN_POINT('Ctrl Pts',(1.02116533136126,3.54921942038457,-35.3887546368837)) ;
#155253=CARTESIAN_POINT('Ctrl Pts',(1.02580209629929,3.54969340754028,-35.384408542828)) ;
#155254=CARTESIAN_POINT('Ctrl Pts',(1.02780524115378,3.54989817637043,-35.3825309717066)) ;
#155255=CARTESIAN_POINT('Ctrl Pts',(1.02980744674854,3.55,-35.3806439182703)) ;
#155256=CARTESIAN_POINT('Ctrl Pts',(1.03179971315146,3.55,-35.3787558734356)) ;
#155257=CARTESIAN_POINT('Origin',(-7.29372370581158E-16,3.55,-34.29)) ;
#155258=CARTESIAN_POINT('',(1.5,3.55,-34.29)) ;
#155259=CARTESIAN_POINT('Origin',(9.2,0.,-34.29)) ;
#155260=CARTESIAN_POINT('',(8.7,-6.12323399573675E-17,-33.79)) ;
#155261=CARTESIAN_POINT('Origin',(8.7,0.,-34.29)) ;
#155262=CARTESIAN_POINT('',(9.2,-1.22464679914735E-16,-33.29)) ;
#155263=CARTESIAN_POINT('Origin',(9.2,0.,-30.48)) ;
#155264=CARTESIAN_POINT('',(8.7,-6.12323399573674E-17,-29.98)) ;
#155265=CARTESIAN_POINT('Origin',(8.7,0.,-30.48)) ;
#155266=CARTESIAN_POINT('',(9.2,-1.22464679914735E-16,-29.48)) ;
#155267=CARTESIAN_POINT('Origin',(9.2,0.,-26.67)) ;
#155268=CARTESIAN_POINT('',(8.7,-6.12323399573674E-17,-26.17)) ;
#155269=CARTESIAN_POINT('Origin',(8.7,0.,-26.67)) ;
#155270=CARTESIAN_POINT('',(9.2,-1.22464679914735E-16,-25.67)) ;
#155271=CARTESIAN_POINT('Origin',(9.2,0.,-22.86)) ;
#155272=CARTESIAN_POINT('',(8.7,-6.12323399573674E-17,-22.36)) ;
#155273=CARTESIAN_POINT('Origin',(8.7,0.,-22.86)) ;
#155274=CARTESIAN_POINT('',(9.2,-1.22464679914735E-16,-21.86)) ;
#155275=CARTESIAN_POINT('Origin',(9.2,0.,-19.05)) ;
#155276=CARTESIAN_POINT('',(8.7,-6.12323399573673E-17,-18.55)) ;
#155277=CARTESIAN_POINT('Origin',(8.7,0.,-19.05)) ;
#155278=CARTESIAN_POINT('',(9.2,-1.22464679914735E-16,-18.05)) ;
#155279=CARTESIAN_POINT('Origin',(9.2,0.,-15.24)) ;
#155280=CARTESIAN_POINT('',(8.7,-6.12323399573673E-17,-14.74)) ;
#155281=CARTESIAN_POINT('Origin',(8.7,0.,-15.24)) ;
#155282=CARTESIAN_POINT('',(9.2,-1.22464679914735E-16,-14.24)) ;
#155283=CARTESIAN_POINT('Origin',(9.2,0.,-11.43)) ;
#155284=CARTESIAN_POINT('',(8.7,-6.12323399573673E-17,-10.93)) ;
#155285=CARTESIAN_POINT('Origin',(8.7,0.,-11.43)) ;
#155286=CARTESIAN_POINT('',(9.2,-1.22464679914735E-16,-10.43)) ;
#155287=CARTESIAN_POINT('Origin',(9.2,0.,-7.62)) ;
#155288=CARTESIAN_POINT('',(8.7,-6.12323399573673E-17,-7.12)) ;
#155289=CARTESIAN_POINT('Origin',(8.7,0.,-7.62)) ;
#155290=CARTESIAN_POINT('',(9.2,-1.22464679914735E-16,-6.62)) ;
#155291=CARTESIAN_POINT('Origin',(9.2,0.,-3.81)) ;
#155292=CARTESIAN_POINT('',(8.7,-6.12323399573674E-17,-3.31)) ;
#155293=CARTESIAN_POINT('Origin',(8.7,0.,-3.81)) ;
#155294=CARTESIAN_POINT('',(9.2,-1.22464679914735E-16,-2.81)) ;
#155295=CARTESIAN_POINT('Origin',(9.2,0.,-3.81)) ;
#155296=CARTESIAN_POINT('',(9.2,-1.22464679914735E-16,-2.81)) ;
#155297=CARTESIAN_POINT('Origin',(9.2,0.,-7.62)) ;
#155298=CARTESIAN_POINT('',(9.2,-1.22464679914735E-16,-6.62)) ;
#155299=CARTESIAN_POINT('Origin',(9.2,0.,-11.43)) ;
#155300=CARTESIAN_POINT('',(9.2,-1.22464679914735E-16,-10.43)) ;
#155301=CARTESIAN_POINT('Origin',(9.2,0.,-15.24)) ;
#155302=CARTESIAN_POINT('',(9.2,-1.22464679914735E-16,-14.24)) ;
#155303=CARTESIAN_POINT('Origin',(9.2,0.,-19.05)) ;
#155304=CARTESIAN_POINT('',(9.2,-1.22464679914735E-16,-18.05)) ;
#155305=CARTESIAN_POINT('Origin',(9.2,0.,-22.86)) ;
#155306=CARTESIAN_POINT('',(9.2,-1.22464679914735E-16,-21.86)) ;
#155307=CARTESIAN_POINT('Origin',(9.2,0.,-26.67)) ;
#155308=CARTESIAN_POINT('',(9.2,-1.22464679914735E-16,-25.67)) ;
#155309=CARTESIAN_POINT('Origin',(9.2,0.,-30.48)) ;
#155310=CARTESIAN_POINT('',(9.2,-1.22464679914735E-16,-29.48)) ;
#155311=CARTESIAN_POINT('Origin',(9.2,0.,-34.29)) ;
#155312=CARTESIAN_POINT('',(9.2,-1.22464679914735E-16,-33.29)) ;
#155313=CARTESIAN_POINT('Origin',(9.24142135623731,0.,0.)) ;
#155314=CARTESIAN_POINT('',(9.17071067811866,-1.18877772485617E-16,0.970710678118656)) ;
#155315=CARTESIAN_POINT('Origin',(9.17071067811866,0.,0.)) ;
#155316=CARTESIAN_POINT('',(9.24142135623731,-1.22464679914735E-16,1.)) ;
#155317=CARTESIAN_POINT('Origin',(9.24142135623731,-1.10218211923262E-16,
0.9)) ;
#155318=CARTESIAN_POINT('Origin',(9.24142135623731,0.,0.)) ;
#155319=CARTESIAN_POINT('Origin',(-6.11095769946375E-16,4.45,0.)) ;
#155320=CARTESIAN_POINT('',(1.5,4.45,-1.83697019872103E-16)) ;
#155321=CARTESIAN_POINT('Origin',(-6.11095769946375E-16,4.45,0.)) ;
#155322=CARTESIAN_POINT('',(1.6,4.55,-1.95943487863577E-16)) ;
#155323=CARTESIAN_POINT('Origin',(1.6,4.45,-1.95943487863577E-16)) ;
#155324=CARTESIAN_POINT('Origin',(-6.24237614461351E-16,4.55,0.)) ;
#155325=CARTESIAN_POINT('Origin',(10.1,0.,0.)) ;
#155326=CARTESIAN_POINT('',(10.1,-1.22464679914735E-16,1.)) ;
#155327=CARTESIAN_POINT('Origin',(10.1,0.,0.)) ;
#155328=CARTESIAN_POINT('',(10.2,-1.34711147906209E-16,1.1)) ;
#155329=CARTESIAN_POINT('Origin',(10.1,-1.34711147906209E-16,1.1)) ;
#155330=CARTESIAN_POINT('Origin',(10.2,0.,0.)) ;
#155331=CARTESIAN_POINT('Origin',(1.31451250000001,-1.51907484122731,-32.385)) ;
#155332=CARTESIAN_POINT('Origin',(1.31451250000001,2.85,-32.385)) ;
#155333=CARTESIAN_POINT('',(1.27787304021906,-1.51907484122731,-32.4380981416173)) ;
#155334=CARTESIAN_POINT('',(1.27787304021906,-1.51907484122731,-32.3319018583827)) ;
#155335=CARTESIAN_POINT('Origin',(1.77490703981929,-1.51907484122731,-35.7754875)) ;
#155336=CARTESIAN_POINT('',(1.77490703981929,2.85,-35.84)) ;
#155337=CARTESIAN_POINT('Origin',(1.77490703981929,2.85,-35.7754875)) ;
#155338=CARTESIAN_POINT('',(1.77490703981929,-1.51907484122731,-35.84)) ;
#155339=CARTESIAN_POINT('',(1.72543498451332,-1.51907484122731,-35.7340824471676)) ;
#155340=CARTESIAN_POINT('Origin',(1.77490703981927,-1.51907484122731,1.4854875)) ;
#155341=CARTESIAN_POINT('',(1.77490703981927,2.85,1.55)) ;
#155342=CARTESIAN_POINT('Origin',(1.77490703981927,2.85,1.4854875)) ;
#155343=CARTESIAN_POINT('',(1.72543498451331,-1.51907484122731,1.4440824471676)) ;
#155344=CARTESIAN_POINT('',(1.77490703981927,-1.51907484122731,1.55)) ;
#155345=CARTESIAN_POINT('Origin',(1.3145125,-1.51907484122731,-1.905)) ;
#155346=CARTESIAN_POINT('Origin',(1.3145125,2.85,-1.905)) ;
#155347=CARTESIAN_POINT('',(1.27787304021905,-1.51907484122731,-1.9580981416173)) ;
#155348=CARTESIAN_POINT('',(1.27787304021905,-1.51907484122731,-1.85190185838271)) ;
#155349=CARTESIAN_POINT('Origin',(-7.29372370581158E-16,3.55,0.)) ;
#155350=CARTESIAN_POINT('',(-0.17080731546663,3.55,1.49024322208929)) ;
#155351=CARTESIAN_POINT('',(1.5,3.55,-1.83697019872103E-16)) ;
#155352=CARTESIAN_POINT('Origin',(-7.29372370581158E-16,3.55,0.)) ;
#155353=CARTESIAN_POINT('',(-0.273932138433073,3.45,1.4747749603019)) ;
#155354=CARTESIAN_POINT('Ctrl Pts',(-0.170807315466632,3.55,1.49024322208929)) ;
#155355=CARTESIAN_POINT('Ctrl Pts',(-0.18388243342709,3.55,1.48874459034574)) ;
#155356=CARTESIAN_POINT('Ctrl Pts',(-0.197859036177013,3.54752250383109,
1.48694882390231)) ;
#155357=CARTESIAN_POINT('Ctrl Pts',(-0.223597793566256,3.53719045839678,
1.48329935326863)) ;
#155358=CARTESIAN_POINT('Ctrl Pts',(-0.235362682979178,3.52934133421403,
1.48144958131094)) ;
#155359=CARTESIAN_POINT('Ctrl Pts',(-0.253465441530115,3.51138121637726,
1.47845705197622)) ;
#155360=CARTESIAN_POINT('Ctrl Pts',(-0.261168570620306,3.50026979217228,
1.4770965178147)) ;
#155361=CARTESIAN_POINT('Ctrl Pts',(-0.271399896344097,3.47583586070553,
1.47525363540046)) ;
#155362=CARTESIAN_POINT('Ctrl Pts',(-0.273932138433075,3.46251477070021,
1.4747749603019)) ;
#155363=CARTESIAN_POINT('Ctrl Pts',(-0.273932138433075,3.45,1.4747749603019)) ;
#155364=CARTESIAN_POINT('',(-0.273932138433073,3.15,1.4747749603019)) ;
#155365=CARTESIAN_POINT('',(-0.273932138433073,3.05,1.4747749603019)) ;
#155366=CARTESIAN_POINT('',(-0.373948193368569,3.05,1.45263992395789)) ;
#155367=CARTESIAN_POINT('Ctrl Pts',(-0.273932138433073,3.15,1.4747749603019)) ;
#155368=CARTESIAN_POINT('Ctrl Pts',(-0.273932138433073,3.13744372549049,
1.4747749603019)) ;
#155369=CARTESIAN_POINT('Ctrl Pts',(-0.276486468486165,3.12408297110069,
1.47430886976441)) ;
#155370=CARTESIAN_POINT('Ctrl Pts',(-0.28674027764043,3.0995678553947,1.47234622100643)) ;
#155371=CARTESIAN_POINT('Ctrl Pts',(-0.294439768310517,3.08841385970397,
1.47084515886225)) ;
#155372=CARTESIAN_POINT('Ctrl Pts',(-0.312194128344972,3.07061084469361,
1.46718060004901)) ;
#155373=CARTESIAN_POINT('Ctrl Pts',(-0.323517908844217,3.0628422827531,
1.4647525137252)) ;
#155374=CARTESIAN_POINT('Ctrl Pts',(-0.348172117123305,3.05253676672645,
1.45908616124653)) ;
#155375=CARTESIAN_POINT('Ctrl Pts',(-0.361501722536397,3.05,1.45584397694084)) ;
#155376=CARTESIAN_POINT('Ctrl Pts',(-0.37394819336857,3.05,1.45263992395789)) ;
#155377=CARTESIAN_POINT('',(-0.872417476238727,3.05,1.22019988000051)) ;
#155378=CARTESIAN_POINT('Origin',(-7.95081593156037E-16,3.05,0.)) ;
#155379=CARTESIAN_POINT('',(-0.953662978710562,3.15,1.15781126399638)) ;
#155380=CARTESIAN_POINT('Ctrl Pts',(-0.872417476238727,3.05,1.22019988000051)) ;
#155381=CARTESIAN_POINT('Ctrl Pts',(-0.882808783297377,3.05,1.21277031208502)) ;
#155382=CARTESIAN_POINT('Ctrl Pts',(-0.893798224191975,3.05250629897269,
1.20469063768542)) ;
#155383=CARTESIAN_POINT('Ctrl Pts',(-0.913892243159219,3.06269675232156,
1.18952223087538)) ;
#155384=CARTESIAN_POINT('Ctrl Pts',(-0.922999225059834,3.07038074042647,
1.18243657143088)) ;
#155385=CARTESIAN_POINT('Ctrl Pts',(-0.937285134131706,3.08810056349785,
1.17114412889658)) ;
#155386=CARTESIAN_POINT('Ctrl Pts',(-0.943452174397235,3.09929464195085,
1.16615690319603)) ;
#155387=CARTESIAN_POINT('Ctrl Pts',(-0.951639309815362,3.12392729225934,
1.15948900020361)) ;
#155388=CARTESIAN_POINT('Ctrl Pts',(-0.953662978710562,3.13736547222678,
1.15781126399638)) ;
#155389=CARTESIAN_POINT('Ctrl Pts',(-0.953662978710562,3.15,1.15781126399638)) ;
#155390=CARTESIAN_POINT('',(-0.953662978710562,3.45,1.15781126399638)) ;
#155391=CARTESIAN_POINT('',(-0.953662978710562,3.05,1.15781126399638)) ;
#155392=CARTESIAN_POINT('',(-1.03179971315145,3.55,1.08875587343563)) ;
#155393=CARTESIAN_POINT('Ctrl Pts',(-0.953662978710565,3.45,1.15781126399638)) ;
#155394=CARTESIAN_POINT('Ctrl Pts',(-0.953662978710565,3.45580715149871,
1.15781126399638)) ;
#155395=CARTESIAN_POINT('Ctrl Pts',(-0.954069792639904,3.46165880969181,
1.15747636843074)) ;
#155396=CARTESIAN_POINT('Ctrl Pts',(-0.95488040580839,3.46741264967889,
1.15680726792462)) ;
#155397=CARTESIAN_POINT('Ctrl Pts',(-0.955592557016221,3.47246759358527,
1.15621944039835)) ;
#155398=CARTESIAN_POINT('Ctrl Pts',(-0.956615573654933,3.47744631522377,
1.15537418855117)) ;
#155399=CARTESIAN_POINT('Ctrl Pts',(-0.957920385817348,3.48225893605768,
1.15429135595662)) ;
#155400=CARTESIAN_POINT('Ctrl Pts',(-0.959423079246195,3.48780141482278,
1.15304430640325)) ;
#155401=CARTESIAN_POINT('Ctrl Pts',(-0.961323201468143,3.49320783601914,
1.15146254061837)) ;
#155402=CARTESIAN_POINT('Ctrl Pts',(-0.963574238618815,3.49834560049868,
1.14957574210362)) ;
#155403=CARTESIAN_POINT('Ctrl Pts',(-0.965499706648006,3.50274028640777,
1.14796183261456)) ;
#155404=CARTESIAN_POINT('Ctrl Pts',(-0.967680912999541,3.5069382066956,
1.14612540554157)) ;
#155405=CARTESIAN_POINT('Ctrl Pts',(-0.970068248378241,3.51087311165944,
1.14410121645275)) ;
#155406=CARTESIAN_POINT('Ctrl Pts',(-0.97293324697906,3.51559532091263,
1.14167202323634)) ;
#155407=CARTESIAN_POINT('Ctrl Pts',(-0.976138831290367,3.52000896466724,
1.13893531443762)) ;
#155408=CARTESIAN_POINT('Ctrl Pts',(-0.979601776802485,3.52400782220665,
1.13594901565242)) ;
#155409=CARTESIAN_POINT('Ctrl Pts',(-0.982467725203496,3.52731729367563,
1.13347754210528)) ;
#155410=CARTESIAN_POINT('Ctrl Pts',(-0.985508986896839,3.53034305696182,
1.13083582639522)) ;
#155411=CARTESIAN_POINT('Ctrl Pts',(-0.988666612105887,3.53304718478134,
1.12806840666118)) ;
#155412=CARTESIAN_POINT('Ctrl Pts',(-0.992701606803652,3.53650267449006,
1.12453203891198)) ;
#155413=CARTESIAN_POINT('Ctrl Pts',(-0.996988044734313,3.53948417067186,
1.12073641188223)) ;
#155414=CARTESIAN_POINT('Ctrl Pts',(-1.00141585135915,3.54192188246042,
1.11676596479649)) ;
#155415=CARTESIAN_POINT('Ctrl Pts',(-1.00487400994927,3.54382575827888,
1.11366500830503)) ;
#155416=CARTESIAN_POINT('Ctrl Pts',(-1.00841776012225,3.54539884758397,
1.11045803912747)) ;
#155417=CARTESIAN_POINT('Ctrl Pts',(-1.0119912926316,3.54662946216441,1.10719177365334)) ;
#155418=CARTESIAN_POINT('Ctrl Pts',(-1.01652362695399,3.54819025857131,
1.10304914809285)) ;
#155419=CARTESIAN_POINT('Ctrl Pts',(-1.0211653313612,3.54921942038456,1.09875463688375)) ;
#155420=CARTESIAN_POINT('Ctrl Pts',(-1.02580209629923,3.54969340754027,
1.09440854282807)) ;
#155421=CARTESIAN_POINT('Ctrl Pts',(-1.02780524115375,3.54989817637043,
1.09253097170655)) ;
#155422=CARTESIAN_POINT('Ctrl Pts',(-1.02980744674852,3.55,1.09064391827031)) ;
#155423=CARTESIAN_POINT('Ctrl Pts',(-1.03179971315145,3.55,1.08875587343563)) ;
#155424=CARTESIAN_POINT('',(0.170807315466631,3.55,-1.49024322208929)) ;
#155425=CARTESIAN_POINT('Origin',(-7.29372370581158E-16,3.55,0.)) ;
#155426=CARTESIAN_POINT('',(0.273932138433074,3.45,-1.4747749603019)) ;
#155427=CARTESIAN_POINT('Ctrl Pts',(0.170807315466627,3.55,-1.4902432220893)) ;
#155428=CARTESIAN_POINT('Ctrl Pts',(0.183882433427085,3.55,-1.48874459034574)) ;
#155429=CARTESIAN_POINT('Ctrl Pts',(0.197859036177008,3.54752250383109,
-1.48694882390231)) ;
#155430=CARTESIAN_POINT('Ctrl Pts',(0.223597793566251,3.53719045839678,
-1.48329935326863)) ;
#155431=CARTESIAN_POINT('Ctrl Pts',(0.235362682979173,3.52934133421403,
-1.48144958131094)) ;
#155432=CARTESIAN_POINT('Ctrl Pts',(0.25346544153011,3.51138121637726,-1.47845705197622)) ;
#155433=CARTESIAN_POINT('Ctrl Pts',(0.261168570620301,3.50026979217228,
-1.4770965178147)) ;
#155434=CARTESIAN_POINT('Ctrl Pts',(0.271399896344092,3.47583586070553,
-1.47525363540046)) ;
#155435=CARTESIAN_POINT('Ctrl Pts',(0.27393213843307,3.46251477070021,-1.47477496030191)) ;
#155436=CARTESIAN_POINT('Ctrl Pts',(0.27393213843307,3.45,-1.47477496030191)) ;
#155437=CARTESIAN_POINT('',(0.273932138433074,3.15,-1.4747749603019)) ;
#155438=CARTESIAN_POINT('',(0.273932138433074,3.05,-1.4747749603019)) ;
#155439=CARTESIAN_POINT('',(0.37394819336857,3.05,-1.45263992395789)) ;
#155440=CARTESIAN_POINT('Ctrl Pts',(0.273932138433074,3.15,-1.4747749603019)) ;
#155441=CARTESIAN_POINT('Ctrl Pts',(0.273932138433074,3.13736547222678,
-1.4747749603019)) ;
#155442=CARTESIAN_POINT('Ctrl Pts',(0.276518148223581,3.12392729225934,
-1.47430316803635)) ;
#155443=CARTESIAN_POINT('Ctrl Pts',(0.28688864746378,3.09929464195085,-1.47231750387035)) ;
#155444=CARTESIAN_POINT('Ctrl Pts',(0.294673181069391,3.08810056349785,
-1.47079900383148)) ;
#155445=CARTESIAN_POINT('Ctrl Pts',(0.312506499266534,3.07038074042647,
-1.46711400471621)) ;
#155446=CARTESIAN_POINT('Ctrl Pts',(0.32378828443718,3.06269675232156,-1.46469222593504)) ;
#155447=CARTESIAN_POINT('Ctrl Pts',(0.348324144605931,3.05250629897269,
-1.45904937832144)) ;
#155448=CARTESIAN_POINT('Ctrl Pts',(0.36157741072639,3.05,-1.45582449278551)) ;
#155449=CARTESIAN_POINT('Ctrl Pts',(0.37394819336857,3.05,-1.45263992395789)) ;
#155450=CARTESIAN_POINT('',(0.872417476238728,3.05,-1.22019988000051)) ;
#155451=CARTESIAN_POINT('Origin',(-7.95081593156037E-16,3.05,0.)) ;
#155452=CARTESIAN_POINT('',(0.953662978710562,3.15,-1.15781126399638)) ;
#155453=CARTESIAN_POINT('Ctrl Pts',(0.872417476238728,3.05,-1.22019988000051)) ;
#155454=CARTESIAN_POINT('Ctrl Pts',(0.882872360457018,3.05,-1.2127248557413)) ;
#155455=CARTESIAN_POINT('Ctrl Pts',(0.893924122929505,3.05253676672645,
-1.20459782148564)) ;
#155456=CARTESIAN_POINT('Ctrl Pts',(0.914112220366976,3.0628422827531,-1.18935386339936)) ;
#155457=CARTESIAN_POINT('Ctrl Pts',(0.923251028202469,3.07061084469361,
-1.18224008807701)) ;
#155458=CARTESIAN_POINT('Ctrl Pts',(0.937470525765899,3.08841385970397,
-1.1709949922316)) ;
#155459=CARTESIAN_POINT('Ctrl Pts',(0.94356954328385,3.0995678553947,-1.16606170433658)) ;
#155460=CARTESIAN_POINT('Ctrl Pts',(0.951664040935143,3.12408297110069,
-1.15946839711695)) ;
#155461=CARTESIAN_POINT('Ctrl Pts',(0.953662978710562,3.13744372549049,
-1.15781126399638)) ;
#155462=CARTESIAN_POINT('Ctrl Pts',(0.953662978710562,3.15,-1.15781126399638)) ;
#155463=CARTESIAN_POINT('',(0.953662978710562,3.45,-1.15781126399638)) ;
#155464=CARTESIAN_POINT('',(0.953662978710562,3.05,-1.15781126399638)) ;
#155465=CARTESIAN_POINT('',(1.03179971315145,3.55,-1.08875587343563)) ;
#155466=CARTESIAN_POINT('Ctrl Pts',(0.95366297871056,3.45,-1.15781126399638)) ;
#155467=CARTESIAN_POINT('Ctrl Pts',(0.95366297871056,3.45580715149871,-1.15781126399638)) ;
#155468=CARTESIAN_POINT('Ctrl Pts',(0.954069792639901,3.46165880969183,
-1.15747636843074)) ;
#155469=CARTESIAN_POINT('Ctrl Pts',(0.954880405808387,3.4674126496789,-1.15680726792462)) ;
#155470=CARTESIAN_POINT('Ctrl Pts',(0.955592557016217,3.47246759358527,
-1.15621944039835)) ;
#155471=CARTESIAN_POINT('Ctrl Pts',(0.95661557365493,3.47744631522378,-1.15537418855117)) ;
#155472=CARTESIAN_POINT('Ctrl Pts',(0.957920385817344,3.48225893605768,
-1.15429135595663)) ;
#155473=CARTESIAN_POINT('Ctrl Pts',(0.959423079246193,3.48780141482279,
-1.15304430640326)) ;
#155474=CARTESIAN_POINT('Ctrl Pts',(0.961323201468142,3.49320783601915,
-1.15146254061836)) ;
#155475=CARTESIAN_POINT('Ctrl Pts',(0.963574238618814,3.49834560049869,
-1.14957574210361)) ;
#155476=CARTESIAN_POINT('Ctrl Pts',(0.965499706648003,3.50274028640777,
-1.14796183261456)) ;
#155477=CARTESIAN_POINT('Ctrl Pts',(0.967680912999538,3.5069382066956,-1.14612540554157)) ;
#155478=CARTESIAN_POINT('Ctrl Pts',(0.970068248378237,3.51087311165944,
-1.14410121645275)) ;
#155479=CARTESIAN_POINT('Ctrl Pts',(0.972933246979058,3.51559532091264,
-1.14167202323633)) ;
#155480=CARTESIAN_POINT('Ctrl Pts',(0.976138831290364,3.52000896466724,
-1.13893531443762)) ;
#155481=CARTESIAN_POINT('Ctrl Pts',(0.979601776802484,3.52400782220666,
-1.13594901565242)) ;
#155482=CARTESIAN_POINT('Ctrl Pts',(0.982467725203496,3.52731729367563,
-1.13347754210528)) ;
#155483=CARTESIAN_POINT('Ctrl Pts',(0.985508986896838,3.53034305696182,
-1.13083582639522)) ;
#155484=CARTESIAN_POINT('Ctrl Pts',(0.988666612105885,3.53304718478134,
-1.12806840666118)) ;
#155485=CARTESIAN_POINT('Ctrl Pts',(0.992701606803651,3.53650267449006,
-1.12453203891197)) ;
#155486=CARTESIAN_POINT('Ctrl Pts',(0.996988044734313,3.53948417067186,
-1.12073641188223)) ;
#155487=CARTESIAN_POINT('Ctrl Pts',(1.00141585135915,3.54192188246042,-1.11676596479648)) ;
#155488=CARTESIAN_POINT('Ctrl Pts',(1.00487400994927,3.54382575827888,-1.11366500830503)) ;
#155489=CARTESIAN_POINT('Ctrl Pts',(1.00841776012226,3.54539884758397,-1.11045803912747)) ;
#155490=CARTESIAN_POINT('Ctrl Pts',(1.01199129263161,3.54662946216441,-1.10719177365333)) ;
#155491=CARTESIAN_POINT('Ctrl Pts',(1.016523626954,3.54819025857131,-1.10304914809285)) ;
#155492=CARTESIAN_POINT('Ctrl Pts',(1.02116533136121,3.54921942038456,-1.09875463688374)) ;
#155493=CARTESIAN_POINT('Ctrl Pts',(1.02580209629923,3.54969340754028,-1.09440854282805)) ;
#155494=CARTESIAN_POINT('Ctrl Pts',(1.02780524115375,3.54989817637043,-1.09253097170654)) ;
#155495=CARTESIAN_POINT('Ctrl Pts',(1.02980744674852,3.55,-1.09064391827031)) ;
#155496=CARTESIAN_POINT('Ctrl Pts',(1.03179971315145,3.55,-1.08875587343563)) ;
#155497=CARTESIAN_POINT('Origin',(-7.29372370581158E-16,3.55,0.)) ;
#155498=CARTESIAN_POINT('',(1.5,3.55,-1.83697019872103E-16)) ;
#155499=CARTESIAN_POINT('Origin',(9.2,0.,0.)) ;
#155500=CARTESIAN_POINT('',(8.7,-6.12323399573674E-17,0.499999999999998)) ;
#155501=CARTESIAN_POINT('Origin',(8.7,0.,0.)) ;
#155502=CARTESIAN_POINT('',(9.2,-1.22464679914735E-16,1.)) ;
#155503=CARTESIAN_POINT('Origin',(9.2,0.,0.)) ;
#155504=CARTESIAN_POINT('',(9.2,-1.22464679914735E-16,1.)) ;
#155505=CARTESIAN_POINT('Origin',(-4.,4.55,-36.59)) ;
#155506=CARTESIAN_POINT('',(-3.9,4.55,-36.49)) ;
#155507=CARTESIAN_POINT('',(-3.9,4.55,2.2)) ;
#155508=CARTESIAN_POINT('',(-3.9,4.55,-36.59)) ;
#155509=CARTESIAN_POINT('',(2.5,4.55,2.2)) ;
#155510=CARTESIAN_POINT('',(2.6,4.55,2.2)) ;
#155511=CARTESIAN_POINT('',(2.5,4.55,1.65)) ;
#155512=CARTESIAN_POINT('',(2.5,4.55,-36.59)) ;
#155513=CARTESIAN_POINT('',(1.77490703981927,4.55,1.65)) ;
#155514=CARTESIAN_POINT('Origin',(-6.24237614461351E-16,4.55,0.)) ;
#155515=CARTESIAN_POINT('Origin',(-6.24237614461351E-16,4.55,-3.81)) ;
#155516=CARTESIAN_POINT('Origin',(-6.24237614461351E-16,4.55,-7.62)) ;
#155517=CARTESIAN_POINT('Origin',(-6.24237614461351E-16,4.55,-11.43)) ;
#155518=CARTESIAN_POINT('Origin',(-6.24237614461351E-16,4.55,-15.24)) ;
#155519=CARTESIAN_POINT('Origin',(-6.24237614461351E-16,4.55,-19.05)) ;
#155520=CARTESIAN_POINT('Origin',(-6.24237614461351E-16,4.55,-22.86)) ;
#155521=CARTESIAN_POINT('Origin',(-6.24237614461351E-16,4.55,-26.67)) ;
#155522=CARTESIAN_POINT('Origin',(-5.97953925431399E-16,4.55,-30.48)) ;
#155523=CARTESIAN_POINT('Origin',(-5.97953925431399E-16,4.55,-34.29)) ;
#155524=CARTESIAN_POINT('',(2.5,4.55,-35.94)) ;
#155525=CARTESIAN_POINT('',(2.6,4.55,-35.94)) ;
#155526=CARTESIAN_POINT('',(2.5,4.55,-36.49)) ;
#155527=CARTESIAN_POINT('',(2.5,4.55,-36.59)) ;
#155528=CARTESIAN_POINT('',(-4.,4.55,-36.49)) ;
#155529=CARTESIAN_POINT('',(-2.1,4.55,-29.38)) ;
#155530=CARTESIAN_POINT('',(-1.9,4.55,-29.58)) ;
#155531=CARTESIAN_POINT('Origin',(-2.1,4.55,-29.58)) ;
#155532=CARTESIAN_POINT('',(-2.9,4.55,-29.38)) ;
#155533=CARTESIAN_POINT('',(-3.,4.55,-29.38)) ;
#155534=CARTESIAN_POINT('',(-3.1,4.55,-29.58)) ;
#155535=CARTESIAN_POINT('Origin',(-2.9,4.55,-29.58)) ;
#155536=CARTESIAN_POINT('',(-3.1,4.55,-31.38)) ;
#155537=CARTESIAN_POINT('',(-3.1,4.55,-31.48)) ;
#155538=CARTESIAN_POINT('',(-2.9,4.55,-31.58)) ;
#155539=CARTESIAN_POINT('Origin',(-2.9,4.55,-31.38)) ;
#155540=CARTESIAN_POINT('',(-2.1,4.55,-31.58)) ;
#155541=CARTESIAN_POINT('',(-2.,4.55,-31.58)) ;
#155542=CARTESIAN_POINT('',(-1.9,4.55,-31.38)) ;
#155543=CARTESIAN_POINT('Origin',(-2.1,4.55,-31.38)) ;
#155544=CARTESIAN_POINT('',(-1.9,4.55,-29.48)) ;
#155545=CARTESIAN_POINT('',(-2.1,4.55,-21.76)) ;
#155546=CARTESIAN_POINT('',(-1.9,4.55,-21.96)) ;
#155547=CARTESIAN_POINT('Origin',(-2.1,4.55,-21.96)) ;
#155548=CARTESIAN_POINT('',(-2.9,4.55,-21.76)) ;
#155549=CARTESIAN_POINT('',(-3.,4.55,-21.76)) ;
#155550=CARTESIAN_POINT('',(-3.1,4.55,-21.96)) ;
#155551=CARTESIAN_POINT('Origin',(-2.9,4.55,-21.96)) ;
#155552=CARTESIAN_POINT('',(-3.1,4.55,-23.76)) ;
#155553=CARTESIAN_POINT('',(-3.1,4.55,-23.86)) ;
#155554=CARTESIAN_POINT('',(-2.9,4.55,-23.96)) ;
#155555=CARTESIAN_POINT('Origin',(-2.9,4.55,-23.76)) ;
#155556=CARTESIAN_POINT('',(-2.1,4.55,-23.96)) ;
#155557=CARTESIAN_POINT('',(-2.,4.55,-23.96)) ;
#155558=CARTESIAN_POINT('',(-1.9,4.55,-23.76)) ;
#155559=CARTESIAN_POINT('Origin',(-2.1,4.55,-23.76)) ;
#155560=CARTESIAN_POINT('',(-1.9,4.55,-21.86)) ;
#155561=CARTESIAN_POINT('',(-2.1,4.55,-14.14)) ;
#155562=CARTESIAN_POINT('',(-1.9,4.55,-14.34)) ;
#155563=CARTESIAN_POINT('Origin',(-2.1,4.55,-14.34)) ;
#155564=CARTESIAN_POINT('',(-2.9,4.55,-14.14)) ;
#155565=CARTESIAN_POINT('',(-3.,4.55,-14.14)) ;
#155566=CARTESIAN_POINT('',(-3.1,4.55,-14.34)) ;
#155567=CARTESIAN_POINT('Origin',(-2.9,4.55,-14.34)) ;
#155568=CARTESIAN_POINT('',(-3.1,4.55,-16.14)) ;
#155569=CARTESIAN_POINT('',(-3.1,4.55,-16.24)) ;
#155570=CARTESIAN_POINT('',(-2.9,4.55,-16.34)) ;
#155571=CARTESIAN_POINT('Origin',(-2.9,4.55,-16.14)) ;
#155572=CARTESIAN_POINT('',(-2.1,4.55,-16.34)) ;
#155573=CARTESIAN_POINT('',(-2.,4.55,-16.34)) ;
#155574=CARTESIAN_POINT('',(-1.9,4.55,-16.14)) ;
#155575=CARTESIAN_POINT('Origin',(-2.1,4.55,-16.14)) ;
#155576=CARTESIAN_POINT('',(-1.9,4.55,-14.24)) ;
#155577=CARTESIAN_POINT('',(-2.1,4.55,-6.52)) ;
#155578=CARTESIAN_POINT('',(-1.9,4.55,-6.72)) ;
#155579=CARTESIAN_POINT('Origin',(-2.1,4.55,-6.72)) ;
#155580=CARTESIAN_POINT('',(-2.9,4.55,-6.52)) ;
#155581=CARTESIAN_POINT('',(-3.,4.55,-6.52)) ;
#155582=CARTESIAN_POINT('',(-3.1,4.55,-6.72)) ;
#155583=CARTESIAN_POINT('Origin',(-2.9,4.55,-6.72)) ;
#155584=CARTESIAN_POINT('',(-3.1,4.55,-8.52)) ;
#155585=CARTESIAN_POINT('',(-3.1,4.55,-8.62)) ;
#155586=CARTESIAN_POINT('',(-2.9,4.55,-8.72)) ;
#155587=CARTESIAN_POINT('Origin',(-2.9,4.55,-8.52)) ;
#155588=CARTESIAN_POINT('',(-2.1,4.55,-8.72)) ;
#155589=CARTESIAN_POINT('',(-2.,4.55,-8.72)) ;
#155590=CARTESIAN_POINT('',(-1.9,4.55,-8.52)) ;
#155591=CARTESIAN_POINT('Origin',(-2.1,4.55,-8.52)) ;
#155592=CARTESIAN_POINT('',(-1.9,4.55,-6.62)) ;
#155593=CARTESIAN_POINT('',(-2.1,4.55,1.1)) ;
#155594=CARTESIAN_POINT('',(-1.9,4.55,0.900000000000001)) ;
#155595=CARTESIAN_POINT('Origin',(-2.1,4.55,0.900000000000001)) ;
#155596=CARTESIAN_POINT('',(-2.9,4.55,1.1)) ;
#155597=CARTESIAN_POINT('',(-3.,4.55,1.1)) ;
#155598=CARTESIAN_POINT('',(-3.1,4.55,0.900000000000001)) ;
#155599=CARTESIAN_POINT('Origin',(-2.9,4.55,0.900000000000001)) ;
#155600=CARTESIAN_POINT('',(-3.1,4.55,-0.899999999999999)) ;
#155601=CARTESIAN_POINT('',(-3.1,4.55,-0.999999999999999)) ;
#155602=CARTESIAN_POINT('',(-2.9,4.55,-1.1)) ;
#155603=CARTESIAN_POINT('Origin',(-2.9,4.55,-0.899999999999999)) ;
#155604=CARTESIAN_POINT('',(-2.1,4.55,-1.1)) ;
#155605=CARTESIAN_POINT('',(-2.,4.55,-1.1)) ;
#155606=CARTESIAN_POINT('',(-1.9,4.55,-0.9)) ;
#155607=CARTESIAN_POINT('Origin',(-2.1,4.55,-0.9)) ;
#155608=CARTESIAN_POINT('',(-1.9,4.55,1.)) ;
#155609=CARTESIAN_POINT('',(-2.1,4.55,-2.71)) ;
#155610=CARTESIAN_POINT('',(-1.9,4.55,-2.91)) ;
#155611=CARTESIAN_POINT('Origin',(-2.1,4.55,-2.91)) ;
#155612=CARTESIAN_POINT('',(-2.9,4.55,-2.71)) ;
#155613=CARTESIAN_POINT('',(-3.,4.55,-2.71)) ;
#155614=CARTESIAN_POINT('',(-3.1,4.55,-2.91)) ;
#155615=CARTESIAN_POINT('Origin',(-2.9,4.55,-2.91)) ;
#155616=CARTESIAN_POINT('',(-3.1,4.55,-4.71)) ;
#155617=CARTESIAN_POINT('',(-3.1,4.55,-4.81)) ;
#155618=CARTESIAN_POINT('',(-2.9,4.55,-4.91)) ;
#155619=CARTESIAN_POINT('Origin',(-2.9,4.55,-4.71)) ;
#155620=CARTESIAN_POINT('',(-2.1,4.55,-4.91)) ;
#155621=CARTESIAN_POINT('',(-2.,4.55,-4.91)) ;
#155622=CARTESIAN_POINT('',(-1.9,4.55,-4.71)) ;
#155623=CARTESIAN_POINT('Origin',(-2.1,4.55,-4.71)) ;
#155624=CARTESIAN_POINT('',(-1.9,4.55,-2.81)) ;
#155625=CARTESIAN_POINT('',(-2.1,4.55,-10.33)) ;
#155626=CARTESIAN_POINT('',(-1.9,4.55,-10.53)) ;
#155627=CARTESIAN_POINT('Origin',(-2.1,4.55,-10.53)) ;
#155628=CARTESIAN_POINT('',(-2.9,4.55,-10.33)) ;
#155629=CARTESIAN_POINT('',(-3.,4.55,-10.33)) ;
#155630=CARTESIAN_POINT('',(-3.1,4.55,-10.53)) ;
#155631=CARTESIAN_POINT('Origin',(-2.9,4.55,-10.53)) ;
#155632=CARTESIAN_POINT('',(-3.1,4.55,-12.33)) ;
#155633=CARTESIAN_POINT('',(-3.1,4.55,-12.43)) ;
#155634=CARTESIAN_POINT('',(-2.9,4.55,-12.53)) ;
#155635=CARTESIAN_POINT('Origin',(-2.9,4.55,-12.33)) ;
#155636=CARTESIAN_POINT('',(-2.1,4.55,-12.53)) ;
#155637=CARTESIAN_POINT('',(-2.,4.55,-12.53)) ;
#155638=CARTESIAN_POINT('',(-1.9,4.55,-12.33)) ;
#155639=CARTESIAN_POINT('Origin',(-2.1,4.55,-12.33)) ;
#155640=CARTESIAN_POINT('',(-1.9,4.55,-10.43)) ;
#155641=CARTESIAN_POINT('',(-2.1,4.55,-17.95)) ;
#155642=CARTESIAN_POINT('',(-1.9,4.55,-18.15)) ;
#155643=CARTESIAN_POINT('Origin',(-2.1,4.55,-18.15)) ;
#155644=CARTESIAN_POINT('',(-2.9,4.55,-17.95)) ;
#155645=CARTESIAN_POINT('',(-3.,4.55,-17.95)) ;
#155646=CARTESIAN_POINT('',(-3.1,4.55,-18.15)) ;
#155647=CARTESIAN_POINT('Origin',(-2.9,4.55,-18.15)) ;
#155648=CARTESIAN_POINT('',(-3.1,4.55,-19.95)) ;
#155649=CARTESIAN_POINT('',(-3.1,4.55,-20.05)) ;
#155650=CARTESIAN_POINT('',(-2.9,4.55,-20.15)) ;
#155651=CARTESIAN_POINT('Origin',(-2.9,4.55,-19.95)) ;
#155652=CARTESIAN_POINT('',(-2.1,4.55,-20.15)) ;
#155653=CARTESIAN_POINT('',(-2.,4.55,-20.15)) ;
#155654=CARTESIAN_POINT('',(-1.9,4.55,-19.95)) ;
#155655=CARTESIAN_POINT('Origin',(-2.1,4.55,-19.95)) ;
#155656=CARTESIAN_POINT('',(-1.9,4.55,-18.05)) ;
#155657=CARTESIAN_POINT('',(-2.1,4.55,-25.57)) ;
#155658=CARTESIAN_POINT('',(-1.9,4.55,-25.77)) ;
#155659=CARTESIAN_POINT('Origin',(-2.1,4.55,-25.77)) ;
#155660=CARTESIAN_POINT('',(-2.9,4.55,-25.57)) ;
#155661=CARTESIAN_POINT('',(-3.,4.55,-25.57)) ;
#155662=CARTESIAN_POINT('',(-3.1,4.55,-25.77)) ;
#155663=CARTESIAN_POINT('Origin',(-2.9,4.55,-25.77)) ;
#155664=CARTESIAN_POINT('',(-3.1,4.55,-27.57)) ;
#155665=CARTESIAN_POINT('',(-3.1,4.55,-27.67)) ;
#155666=CARTESIAN_POINT('',(-2.9,4.55,-27.77)) ;
#155667=CARTESIAN_POINT('Origin',(-2.9,4.55,-27.57)) ;
#155668=CARTESIAN_POINT('',(-2.1,4.55,-27.77)) ;
#155669=CARTESIAN_POINT('',(-2.,4.55,-27.77)) ;
#155670=CARTESIAN_POINT('',(-1.9,4.55,-27.57)) ;
#155671=CARTESIAN_POINT('Origin',(-2.1,4.55,-27.57)) ;
#155672=CARTESIAN_POINT('',(-1.9,4.55,-25.67)) ;
#155673=CARTESIAN_POINT('',(-2.1,4.55,-33.19)) ;
#155674=CARTESIAN_POINT('',(-1.9,4.55,-33.39)) ;
#155675=CARTESIAN_POINT('Origin',(-2.1,4.55,-33.39)) ;
#155676=CARTESIAN_POINT('',(-2.9,4.55,-33.19)) ;
#155677=CARTESIAN_POINT('',(-3.,4.55,-33.19)) ;
#155678=CARTESIAN_POINT('',(-3.1,4.55,-33.39)) ;
#155679=CARTESIAN_POINT('Origin',(-2.9,4.55,-33.39)) ;
#155680=CARTESIAN_POINT('',(-3.1,4.55,-35.19)) ;
#155681=CARTESIAN_POINT('',(-3.1,4.55,-35.29)) ;
#155682=CARTESIAN_POINT('',(-2.9,4.55,-35.39)) ;
#155683=CARTESIAN_POINT('Origin',(-2.9,4.55,-35.19)) ;
#155684=CARTESIAN_POINT('',(-2.1,4.55,-35.39)) ;
#155685=CARTESIAN_POINT('',(-2.,4.55,-35.39)) ;
#155686=CARTESIAN_POINT('',(-1.9,4.55,-35.19)) ;
#155687=CARTESIAN_POINT('Origin',(-2.1,4.55,-35.19)) ;
#155688=CARTESIAN_POINT('',(-1.9,4.55,-33.29)) ;
#155689=CARTESIAN_POINT('Origin',(10.2,2.,-32.885)) ;
#155690=CARTESIAN_POINT('',(10.1,2.,-32.985)) ;
#155691=CARTESIAN_POINT('',(10.1,2.,-35.595)) ;
#155692=CARTESIAN_POINT('',(10.1,2.,-35.695)) ;
#155693=CARTESIAN_POINT('',(3.7,2.,-35.595)) ;
#155694=CARTESIAN_POINT('',(10.2,2.,-35.595)) ;
#155695=CARTESIAN_POINT('',(3.7,2.,-32.985)) ;
#155696=CARTESIAN_POINT('',(3.7,2.,-32.885)) ;
#155697=CARTESIAN_POINT('',(10.2,2.,-32.985)) ;
#155698=CARTESIAN_POINT('',(9.8,2.,-34.69)) ;
#155699=CARTESIAN_POINT('',(9.8,2.,-33.89)) ;
#155700=CARTESIAN_POINT('',(9.8,2.,-33.89)) ;
#155701=CARTESIAN_POINT('',(9.6,2.,-33.69)) ;
#155702=CARTESIAN_POINT('Origin',(9.6,2.,-33.89)) ;
#155703=CARTESIAN_POINT('',(7.8,2.,-33.69)) ;
#155704=CARTESIAN_POINT('',(7.8,2.,-33.69)) ;
#155705=CARTESIAN_POINT('',(7.6,2.,-33.89)) ;
#155706=CARTESIAN_POINT('Origin',(7.8,2.,-33.89)) ;
#155707=CARTESIAN_POINT('',(7.6,2.,-34.69)) ;
#155708=CARTESIAN_POINT('',(7.6,2.,-34.69)) ;
#155709=CARTESIAN_POINT('',(7.8,2.,-34.89)) ;
#155710=CARTESIAN_POINT('Origin',(7.8,2.,-34.69)) ;
#155711=CARTESIAN_POINT('',(9.6,2.,-34.89)) ;
#155712=CARTESIAN_POINT('',(9.6,2.,-34.89)) ;
#155713=CARTESIAN_POINT('Origin',(9.6,2.,-34.69)) ;
#155714=CARTESIAN_POINT('Origin',(10.2,2.,-29.075)) ;
#155715=CARTESIAN_POINT('',(10.1,2.,-29.175)) ;
#155716=CARTESIAN_POINT('',(10.1,2.,-31.785)) ;
#155717=CARTESIAN_POINT('',(10.1,2.,-31.885)) ;
#155718=CARTESIAN_POINT('',(3.7,2.,-31.785)) ;
#155719=CARTESIAN_POINT('',(10.2,2.,-31.785)) ;
#155720=CARTESIAN_POINT('',(3.7,2.,-29.175)) ;
#155721=CARTESIAN_POINT('',(3.7,2.,-29.075)) ;
#155722=CARTESIAN_POINT('',(10.2,2.,-29.175)) ;
#155723=CARTESIAN_POINT('',(9.8,2.,-30.88)) ;
#155724=CARTESIAN_POINT('',(9.8,2.,-30.08)) ;
#155725=CARTESIAN_POINT('',(9.8,2.,-30.08)) ;
#155726=CARTESIAN_POINT('',(9.6,2.,-29.88)) ;
#155727=CARTESIAN_POINT('Origin',(9.6,2.,-30.08)) ;
#155728=CARTESIAN_POINT('',(7.8,2.,-29.88)) ;
#155729=CARTESIAN_POINT('',(7.8,2.,-29.88)) ;
#155730=CARTESIAN_POINT('',(7.6,2.,-30.08)) ;
#155731=CARTESIAN_POINT('Origin',(7.8,2.,-30.08)) ;
#155732=CARTESIAN_POINT('',(7.6,2.,-30.88)) ;
#155733=CARTESIAN_POINT('',(7.6,2.,-30.88)) ;
#155734=CARTESIAN_POINT('',(7.8,2.,-31.08)) ;
#155735=CARTESIAN_POINT('Origin',(7.8,2.,-30.88)) ;
#155736=CARTESIAN_POINT('',(9.6,2.,-31.08)) ;
#155737=CARTESIAN_POINT('',(9.6,2.,-31.08)) ;
#155738=CARTESIAN_POINT('Origin',(9.6,2.,-30.88)) ;
#155739=CARTESIAN_POINT('Origin',(10.2,2.,-25.265)) ;
#155740=CARTESIAN_POINT('',(10.1,2.,-25.365)) ;
#155741=CARTESIAN_POINT('',(10.1,2.,-27.975)) ;
#155742=CARTESIAN_POINT('',(10.1,2.,-28.075)) ;
#155743=CARTESIAN_POINT('',(3.7,2.,-27.975)) ;
#155744=CARTESIAN_POINT('',(10.2,2.,-27.975)) ;
#155745=CARTESIAN_POINT('',(3.7,2.,-25.365)) ;
#155746=CARTESIAN_POINT('',(3.7,2.,-25.265)) ;
#155747=CARTESIAN_POINT('',(10.2,2.,-25.365)) ;
#155748=CARTESIAN_POINT('',(9.8,2.,-27.07)) ;
#155749=CARTESIAN_POINT('',(9.8,2.,-26.27)) ;
#155750=CARTESIAN_POINT('',(9.8,2.,-26.27)) ;
#155751=CARTESIAN_POINT('',(9.6,2.,-26.07)) ;
#155752=CARTESIAN_POINT('Origin',(9.6,2.,-26.27)) ;
#155753=CARTESIAN_POINT('',(7.8,2.,-26.07)) ;
#155754=CARTESIAN_POINT('',(7.8,2.,-26.07)) ;
#155755=CARTESIAN_POINT('',(7.6,2.,-26.27)) ;
#155756=CARTESIAN_POINT('Origin',(7.8,2.,-26.27)) ;
#155757=CARTESIAN_POINT('',(7.6,2.,-27.07)) ;
#155758=CARTESIAN_POINT('',(7.6,2.,-27.07)) ;
#155759=CARTESIAN_POINT('',(7.8,2.,-27.27)) ;
#155760=CARTESIAN_POINT('Origin',(7.8,2.,-27.07)) ;
#155761=CARTESIAN_POINT('',(9.6,2.,-27.27)) ;
#155762=CARTESIAN_POINT('',(9.6,2.,-27.27)) ;
#155763=CARTESIAN_POINT('Origin',(9.6,2.,-27.07)) ;
#155764=CARTESIAN_POINT('Origin',(10.2,2.,-21.455)) ;
#155765=CARTESIAN_POINT('',(10.1,2.,-21.555)) ;
#155766=CARTESIAN_POINT('',(10.1,2.,-24.165)) ;
#155767=CARTESIAN_POINT('',(10.1,2.,-24.265)) ;
#155768=CARTESIAN_POINT('',(3.7,2.,-24.165)) ;
#155769=CARTESIAN_POINT('',(10.2,2.,-24.165)) ;
#155770=CARTESIAN_POINT('',(3.7,2.,-21.555)) ;
#155771=CARTESIAN_POINT('',(3.7,2.,-21.455)) ;
#155772=CARTESIAN_POINT('',(10.2,2.,-21.555)) ;
#155773=CARTESIAN_POINT('',(9.8,2.,-23.26)) ;
#155774=CARTESIAN_POINT('',(9.8,2.,-22.46)) ;
#155775=CARTESIAN_POINT('',(9.8,2.,-22.46)) ;
#155776=CARTESIAN_POINT('',(9.6,2.,-22.26)) ;
#155777=CARTESIAN_POINT('Origin',(9.6,2.,-22.46)) ;
#155778=CARTESIAN_POINT('',(7.8,2.,-22.26)) ;
#155779=CARTESIAN_POINT('',(7.8,2.,-22.26)) ;
#155780=CARTESIAN_POINT('',(7.6,2.,-22.46)) ;
#155781=CARTESIAN_POINT('Origin',(7.8,2.,-22.46)) ;
#155782=CARTESIAN_POINT('',(7.6,2.,-23.26)) ;
#155783=CARTESIAN_POINT('',(7.6,2.,-23.26)) ;
#155784=CARTESIAN_POINT('',(7.8,2.,-23.46)) ;
#155785=CARTESIAN_POINT('Origin',(7.8,2.,-23.26)) ;
#155786=CARTESIAN_POINT('',(9.6,2.,-23.46)) ;
#155787=CARTESIAN_POINT('',(9.6,2.,-23.46)) ;
#155788=CARTESIAN_POINT('Origin',(9.6,2.,-23.26)) ;
#155789=CARTESIAN_POINT('Origin',(10.2,2.,-17.645)) ;
#155790=CARTESIAN_POINT('',(10.1,2.,-17.745)) ;
#155791=CARTESIAN_POINT('',(10.1,2.,-20.355)) ;
#155792=CARTESIAN_POINT('',(10.1,2.,-20.455)) ;
#155793=CARTESIAN_POINT('',(3.7,2.,-20.355)) ;
#155794=CARTESIAN_POINT('',(10.2,2.,-20.355)) ;
#155795=CARTESIAN_POINT('',(3.7,2.,-17.745)) ;
#155796=CARTESIAN_POINT('',(3.7,2.,-17.645)) ;
#155797=CARTESIAN_POINT('',(10.2,2.,-17.745)) ;
#155798=CARTESIAN_POINT('',(9.8,2.,-19.45)) ;
#155799=CARTESIAN_POINT('',(9.8,2.,-18.65)) ;
#155800=CARTESIAN_POINT('',(9.8,2.,-18.65)) ;
#155801=CARTESIAN_POINT('',(9.6,2.,-18.45)) ;
#155802=CARTESIAN_POINT('Origin',(9.6,2.,-18.65)) ;
#155803=CARTESIAN_POINT('',(7.8,2.,-18.45)) ;
#155804=CARTESIAN_POINT('',(7.8,2.,-18.45)) ;
#155805=CARTESIAN_POINT('',(7.6,2.,-18.65)) ;
#155806=CARTESIAN_POINT('Origin',(7.8,2.,-18.65)) ;
#155807=CARTESIAN_POINT('',(7.6,2.,-19.45)) ;
#155808=CARTESIAN_POINT('',(7.6,2.,-19.45)) ;
#155809=CARTESIAN_POINT('',(7.8,2.,-19.65)) ;
#155810=CARTESIAN_POINT('Origin',(7.8,2.,-19.45)) ;
#155811=CARTESIAN_POINT('',(9.6,2.,-19.65)) ;
#155812=CARTESIAN_POINT('',(9.6,2.,-19.65)) ;
#155813=CARTESIAN_POINT('Origin',(9.6,2.,-19.45)) ;
#155814=CARTESIAN_POINT('Origin',(10.2,2.,-13.835)) ;
#155815=CARTESIAN_POINT('',(10.1,2.,-13.935)) ;
#155816=CARTESIAN_POINT('',(10.1,2.,-16.545)) ;
#155817=CARTESIAN_POINT('',(10.1,2.,-16.645)) ;
#155818=CARTESIAN_POINT('',(3.7,2.,-16.545)) ;
#155819=CARTESIAN_POINT('',(10.2,2.,-16.545)) ;
#155820=CARTESIAN_POINT('',(3.7,2.,-13.935)) ;
#155821=CARTESIAN_POINT('',(3.7,2.,-13.835)) ;
#155822=CARTESIAN_POINT('',(10.2,2.,-13.935)) ;
#155823=CARTESIAN_POINT('',(9.8,2.,-15.64)) ;
#155824=CARTESIAN_POINT('',(9.8,2.,-14.84)) ;
#155825=CARTESIAN_POINT('',(9.8,2.,-14.84)) ;
#155826=CARTESIAN_POINT('',(9.6,2.,-14.64)) ;
#155827=CARTESIAN_POINT('Origin',(9.6,2.,-14.84)) ;
#155828=CARTESIAN_POINT('',(7.8,2.,-14.64)) ;
#155829=CARTESIAN_POINT('',(7.8,2.,-14.64)) ;
#155830=CARTESIAN_POINT('',(7.6,2.,-14.84)) ;
#155831=CARTESIAN_POINT('Origin',(7.8,2.,-14.84)) ;
#155832=CARTESIAN_POINT('',(7.6,2.,-15.64)) ;
#155833=CARTESIAN_POINT('',(7.6,2.,-15.64)) ;
#155834=CARTESIAN_POINT('',(7.8,2.,-15.84)) ;
#155835=CARTESIAN_POINT('Origin',(7.8,2.,-15.64)) ;
#155836=CARTESIAN_POINT('',(9.6,2.,-15.84)) ;
#155837=CARTESIAN_POINT('',(9.6,2.,-15.84)) ;
#155838=CARTESIAN_POINT('Origin',(9.6,2.,-15.64)) ;
#155839=CARTESIAN_POINT('Origin',(10.2,2.,-10.025)) ;
#155840=CARTESIAN_POINT('',(10.1,2.,-10.125)) ;
#155841=CARTESIAN_POINT('',(10.1,2.,-12.735)) ;
#155842=CARTESIAN_POINT('',(10.1,2.,-12.835)) ;
#155843=CARTESIAN_POINT('',(3.7,2.,-12.735)) ;
#155844=CARTESIAN_POINT('',(10.2,2.,-12.735)) ;
#155845=CARTESIAN_POINT('',(3.7,2.,-10.125)) ;
#155846=CARTESIAN_POINT('',(3.7,2.,-10.025)) ;
#155847=CARTESIAN_POINT('',(10.2,2.,-10.125)) ;
#155848=CARTESIAN_POINT('',(9.8,2.,-11.83)) ;
#155849=CARTESIAN_POINT('',(9.8,2.,-11.03)) ;
#155850=CARTESIAN_POINT('',(9.8,2.,-11.03)) ;
#155851=CARTESIAN_POINT('',(9.6,2.,-10.83)) ;
#155852=CARTESIAN_POINT('Origin',(9.6,2.,-11.03)) ;
#155853=CARTESIAN_POINT('',(7.8,2.,-10.83)) ;
#155854=CARTESIAN_POINT('',(7.8,2.,-10.83)) ;
#155855=CARTESIAN_POINT('',(7.6,2.,-11.03)) ;
#155856=CARTESIAN_POINT('Origin',(7.8,2.,-11.03)) ;
#155857=CARTESIAN_POINT('',(7.6,2.,-11.83)) ;
#155858=CARTESIAN_POINT('',(7.6,2.,-11.83)) ;
#155859=CARTESIAN_POINT('',(7.8,2.,-12.03)) ;
#155860=CARTESIAN_POINT('Origin',(7.8,2.,-11.83)) ;
#155861=CARTESIAN_POINT('',(9.6,2.,-12.03)) ;
#155862=CARTESIAN_POINT('',(9.6,2.,-12.03)) ;
#155863=CARTESIAN_POINT('Origin',(9.6,2.,-11.83)) ;
#155864=CARTESIAN_POINT('Origin',(10.2,2.,-6.215)) ;
#155865=CARTESIAN_POINT('',(10.1,2.,-6.315)) ;
#155866=CARTESIAN_POINT('',(10.1,2.,-8.925)) ;
#155867=CARTESIAN_POINT('',(10.1,2.,-9.025)) ;
#155868=CARTESIAN_POINT('',(3.7,2.,-8.925)) ;
#155869=CARTESIAN_POINT('',(10.2,2.,-8.925)) ;
#155870=CARTESIAN_POINT('',(3.7,2.,-6.315)) ;
#155871=CARTESIAN_POINT('',(3.7,2.,-6.215)) ;
#155872=CARTESIAN_POINT('',(10.2,2.,-6.315)) ;
#155873=CARTESIAN_POINT('',(9.8,2.,-8.02)) ;
#155874=CARTESIAN_POINT('',(9.8,2.,-7.22)) ;
#155875=CARTESIAN_POINT('',(9.8,2.,-7.22)) ;
#155876=CARTESIAN_POINT('',(9.6,2.,-7.02)) ;
#155877=CARTESIAN_POINT('Origin',(9.6,2.,-7.22)) ;
#155878=CARTESIAN_POINT('',(7.8,2.,-7.02)) ;
#155879=CARTESIAN_POINT('',(7.8,2.,-7.02)) ;
#155880=CARTESIAN_POINT('',(7.6,2.,-7.22)) ;
#155881=CARTESIAN_POINT('Origin',(7.8,2.,-7.22)) ;
#155882=CARTESIAN_POINT('',(7.6,2.,-8.02)) ;
#155883=CARTESIAN_POINT('',(7.6,2.,-8.02)) ;
#155884=CARTESIAN_POINT('',(7.8,2.,-8.22)) ;
#155885=CARTESIAN_POINT('Origin',(7.8,2.,-8.02)) ;
#155886=CARTESIAN_POINT('',(9.6,2.,-8.22)) ;
#155887=CARTESIAN_POINT('',(9.6,2.,-8.22)) ;
#155888=CARTESIAN_POINT('Origin',(9.6,2.,-8.02)) ;
#155889=CARTESIAN_POINT('Origin',(10.2,2.,-2.405)) ;
#155890=CARTESIAN_POINT('',(10.1,2.,-2.505)) ;
#155891=CARTESIAN_POINT('',(10.1,2.,-5.115)) ;
#155892=CARTESIAN_POINT('',(10.1,2.,-5.215)) ;
#155893=CARTESIAN_POINT('',(3.7,2.,-5.115)) ;
#155894=CARTESIAN_POINT('',(10.2,2.,-5.115)) ;
#155895=CARTESIAN_POINT('',(3.7,2.,-2.505)) ;
#155896=CARTESIAN_POINT('',(3.7,2.,-2.405)) ;
#155897=CARTESIAN_POINT('',(10.2,2.,-2.505)) ;
#155898=CARTESIAN_POINT('',(9.8,2.,-4.21)) ;
#155899=CARTESIAN_POINT('',(9.8,2.,-3.41)) ;
#155900=CARTESIAN_POINT('',(9.8,2.,-3.41)) ;
#155901=CARTESIAN_POINT('',(9.6,2.,-3.21)) ;
#155902=CARTESIAN_POINT('Origin',(9.6,2.,-3.41)) ;
#155903=CARTESIAN_POINT('',(7.8,2.,-3.21)) ;
#155904=CARTESIAN_POINT('',(7.8,2.,-3.21)) ;
#155905=CARTESIAN_POINT('',(7.6,2.,-3.41)) ;
#155906=CARTESIAN_POINT('Origin',(7.8,2.,-3.41)) ;
#155907=CARTESIAN_POINT('',(7.6,2.,-4.21)) ;
#155908=CARTESIAN_POINT('',(7.6,2.,-4.21)) ;
#155909=CARTESIAN_POINT('',(7.8,2.,-4.41)) ;
#155910=CARTESIAN_POINT('Origin',(7.8,2.,-4.21)) ;
#155911=CARTESIAN_POINT('',(9.6,2.,-4.41)) ;
#155912=CARTESIAN_POINT('',(9.6,2.,-4.41)) ;
#155913=CARTESIAN_POINT('Origin',(9.6,2.,-4.21)) ;
#155914=CARTESIAN_POINT('Origin',(-7.29372370581158E-16,3.55,-34.29)) ;
#155915=CARTESIAN_POINT('',(0.18330135972941,3.55,-35.807036786476)) ;
#155916=CARTESIAN_POINT('Origin',(-7.29372370581158E-16,3.55,-30.48)) ;
#155917=CARTESIAN_POINT('',(0.18330135972941,3.55,-31.997036786476)) ;
#155918=CARTESIAN_POINT('Origin',(-7.29372370581158E-16,3.55,-26.67)) ;
#155919=CARTESIAN_POINT('',(0.18330135972941,3.55,-28.187036786476)) ;
#155920=CARTESIAN_POINT('Origin',(-7.29372370581158E-16,3.55,-22.86)) ;
#155921=CARTESIAN_POINT('',(0.18330135972941,3.55,-24.377036786476)) ;
#155922=CARTESIAN_POINT('Origin',(-7.29372370581158E-16,3.55,-19.05)) ;
#155923=CARTESIAN_POINT('',(0.18330135972941,3.55,-20.567036786476)) ;
#155924=CARTESIAN_POINT('Origin',(-7.29372370581158E-16,3.55,-15.24)) ;
#155925=CARTESIAN_POINT('',(0.183301359729409,3.55,-16.757036786476)) ;
#155926=CARTESIAN_POINT('Origin',(-7.29372370581158E-16,3.55,-11.43)) ;
#155927=CARTESIAN_POINT('',(0.183301359729409,3.55,-12.947036786476)) ;
#155928=CARTESIAN_POINT('Origin',(-7.29372370581158E-16,3.55,-7.62)) ;
#155929=CARTESIAN_POINT('',(0.183301359729409,3.55,-9.13703678647597)) ;
#155930=CARTESIAN_POINT('Origin',(-7.29372370581158E-16,3.55,-3.81)) ;
#155931=CARTESIAN_POINT('',(0.183301359729409,3.55,-5.32703678647597)) ;
#155932=CARTESIAN_POINT('Origin',(3.6,7.81406971160724E-17,0.)) ;
#155933=CARTESIAN_POINT('',(3.6,2.1,-35.795)) ;
#155934=CARTESIAN_POINT('',(3.6,2.1,-36.49)) ;
#155935=CARTESIAN_POINT('',(3.6,2.1,-36.59)) ;
#155936=CARTESIAN_POINT('',(3.6,2.65,-36.49)) ;
#155937=CARTESIAN_POINT('',(3.6,7.81406971160724E-17,-36.49)) ;
#155938=CARTESIAN_POINT('',(3.6,2.65,2.2)) ;
#155939=CARTESIAN_POINT('',(3.6,2.65,-1.51)) ;
#155940=CARTESIAN_POINT('',(3.6,2.1,2.2)) ;
#155941=CARTESIAN_POINT('',(3.6,2.1,2.2)) ;
#155942=CARTESIAN_POINT('',(3.6,2.1,1.505)) ;
#155943=CARTESIAN_POINT('',(3.6,2.1,1.505)) ;
#155944=CARTESIAN_POINT('',(3.6,2.07320508075689,1.405)) ;
#155945=CARTESIAN_POINT('Origin',(3.6,1.9,1.505)) ;
#155946=CARTESIAN_POINT('',(3.6,2.1,1.305)) ;
#155947=CARTESIAN_POINT('Origin',(3.6,1.9,1.305)) ;
#155948=CARTESIAN_POINT('',(3.6,2.1,-1.305)) ;
#155949=CARTESIAN_POINT('',(3.6,2.1,0.)) ;
#155950=CARTESIAN_POINT('',(3.6,2.07320508075689,-1.405)) ;
#155951=CARTESIAN_POINT('Origin',(3.6,1.9,-1.305)) ;
#155952=CARTESIAN_POINT('',(3.6,2.1,-1.505)) ;
#155953=CARTESIAN_POINT('Origin',(3.6,1.9,-1.505)) ;
#155954=CARTESIAN_POINT('',(3.6,2.1,-2.305)) ;
#155955=CARTESIAN_POINT('',(3.6,2.1,-2.3)) ;
#155956=CARTESIAN_POINT('',(3.6,2.07320508075689,-2.405)) ;
#155957=CARTESIAN_POINT('Origin',(3.6,1.9,-2.305)) ;
#155958=CARTESIAN_POINT('',(3.6,2.1,-2.505)) ;
#155959=CARTESIAN_POINT('Origin',(3.6,1.9,-2.505)) ;
#155960=CARTESIAN_POINT('',(3.6,2.1,-5.115)) ;
#155961=CARTESIAN_POINT('',(3.6,2.1,0.)) ;
#155962=CARTESIAN_POINT('',(3.6,2.07320508075689,-5.215)) ;
#155963=CARTESIAN_POINT('Origin',(3.6,1.9,-5.115)) ;
#155964=CARTESIAN_POINT('',(3.6,2.1,-5.315)) ;
#155965=CARTESIAN_POINT('Origin',(3.6,1.9,-5.315)) ;
#155966=CARTESIAN_POINT('',(3.6,2.1,-6.115)) ;
#155967=CARTESIAN_POINT('',(3.6,2.1,-6.115)) ;
#155968=CARTESIAN_POINT('',(3.6,2.07320508075689,-6.215)) ;
#155969=CARTESIAN_POINT('Origin',(3.6,1.9,-6.115)) ;
#155970=CARTESIAN_POINT('',(3.6,2.1,-6.315)) ;
#155971=CARTESIAN_POINT('Origin',(3.6,1.9,-6.315)) ;
#155972=CARTESIAN_POINT('',(3.6,2.1,-8.925)) ;
#155973=CARTESIAN_POINT('',(3.6,2.1,0.)) ;
#155974=CARTESIAN_POINT('',(3.6,2.07320508075689,-9.025)) ;
#155975=CARTESIAN_POINT('Origin',(3.6,1.9,-8.925)) ;
#155976=CARTESIAN_POINT('',(3.6,2.1,-9.125)) ;
#155977=CARTESIAN_POINT('Origin',(3.6,1.9,-9.125)) ;
#155978=CARTESIAN_POINT('',(3.6,2.1,-9.925)) ;
#155979=CARTESIAN_POINT('',(3.6,2.1,-9.925)) ;
#155980=CARTESIAN_POINT('',(3.6,2.07320508075689,-10.025)) ;
#155981=CARTESIAN_POINT('Origin',(3.6,1.9,-9.925)) ;
#155982=CARTESIAN_POINT('',(3.6,2.1,-10.125)) ;
#155983=CARTESIAN_POINT('Origin',(3.6,1.9,-10.125)) ;
#155984=CARTESIAN_POINT('',(3.6,2.1,-12.735)) ;
#155985=CARTESIAN_POINT('',(3.6,2.1,0.)) ;
#155986=CARTESIAN_POINT('',(3.6,2.07320508075689,-12.835)) ;
#155987=CARTESIAN_POINT('Origin',(3.6,1.9,-12.735)) ;
#155988=CARTESIAN_POINT('',(3.6,2.1,-12.935)) ;
#155989=CARTESIAN_POINT('Origin',(3.6,1.9,-12.935)) ;
#155990=CARTESIAN_POINT('',(3.6,2.1,-13.735)) ;
#155991=CARTESIAN_POINT('',(3.6,2.1,-13.735)) ;
#155992=CARTESIAN_POINT('',(3.6,2.07320508075689,-13.835)) ;
#155993=CARTESIAN_POINT('Origin',(3.6,1.9,-13.735)) ;
#155994=CARTESIAN_POINT('',(3.6,2.1,-13.935)) ;
#155995=CARTESIAN_POINT('Origin',(3.6,1.9,-13.935)) ;
#155996=CARTESIAN_POINT('',(3.6,2.1,-16.545)) ;
#155997=CARTESIAN_POINT('',(3.6,2.1,0.)) ;
#155998=CARTESIAN_POINT('',(3.6,2.07320508075689,-16.645)) ;
#155999=CARTESIAN_POINT('Origin',(3.6,1.9,-16.545)) ;
#156000=CARTESIAN_POINT('',(3.6,2.1,-16.745)) ;
#156001=CARTESIAN_POINT('Origin',(3.6,1.9,-16.745)) ;
#156002=CARTESIAN_POINT('',(3.6,2.1,-17.545)) ;
#156003=CARTESIAN_POINT('',(3.6,2.1,-17.545)) ;
#156004=CARTESIAN_POINT('',(3.6,2.07320508075689,-17.645)) ;
#156005=CARTESIAN_POINT('Origin',(3.6,1.9,-17.545)) ;
#156006=CARTESIAN_POINT('',(3.6,2.1,-17.745)) ;
#156007=CARTESIAN_POINT('Origin',(3.6,1.9,-17.745)) ;
#156008=CARTESIAN_POINT('',(3.6,2.1,-20.355)) ;
#156009=CARTESIAN_POINT('',(3.6,2.1,0.)) ;
#156010=CARTESIAN_POINT('',(3.6,2.07320508075689,-20.455)) ;
#156011=CARTESIAN_POINT('Origin',(3.6,1.9,-20.355)) ;
#156012=CARTESIAN_POINT('',(3.6,2.1,-20.555)) ;
#156013=CARTESIAN_POINT('Origin',(3.6,1.9,-20.555)) ;
#156014=CARTESIAN_POINT('',(3.6,2.1,-21.355)) ;
#156015=CARTESIAN_POINT('',(3.6,2.1,-21.355)) ;
#156016=CARTESIAN_POINT('',(3.6,2.07320508075689,-21.455)) ;
#156017=CARTESIAN_POINT('Origin',(3.6,1.9,-21.355)) ;
#156018=CARTESIAN_POINT('',(3.6,2.1,-21.555)) ;
#156019=CARTESIAN_POINT('Origin',(3.6,1.9,-21.555)) ;
#156020=CARTESIAN_POINT('',(3.6,2.1,-24.165)) ;
#156021=CARTESIAN_POINT('',(3.6,2.1,0.)) ;
#156022=CARTESIAN_POINT('',(3.6,2.07320508075689,-24.265)) ;
#156023=CARTESIAN_POINT('Origin',(3.6,1.9,-24.165)) ;
#156024=CARTESIAN_POINT('',(3.6,2.1,-24.365)) ;
#156025=CARTESIAN_POINT('Origin',(3.6,1.9,-24.365)) ;
#156026=CARTESIAN_POINT('',(3.6,2.1,-25.165)) ;
#156027=CARTESIAN_POINT('',(3.6,2.1,-25.165)) ;
#156028=CARTESIAN_POINT('',(3.6,2.07320508075689,-25.265)) ;
#156029=CARTESIAN_POINT('Origin',(3.6,1.9,-25.165)) ;
#156030=CARTESIAN_POINT('',(3.6,2.1,-25.365)) ;
#156031=CARTESIAN_POINT('Origin',(3.6,1.9,-25.365)) ;
#156032=CARTESIAN_POINT('',(3.6,2.1,-27.975)) ;
#156033=CARTESIAN_POINT('',(3.6,2.1,0.)) ;
#156034=CARTESIAN_POINT('',(3.6,2.07320508075689,-28.075)) ;
#156035=CARTESIAN_POINT('Origin',(3.6,1.9,-27.975)) ;
#156036=CARTESIAN_POINT('',(3.6,2.1,-28.175)) ;
#156037=CARTESIAN_POINT('Origin',(3.6,1.9,-28.175)) ;
#156038=CARTESIAN_POINT('',(3.6,2.1,-28.975)) ;
#156039=CARTESIAN_POINT('',(3.6,2.1,-28.975)) ;
#156040=CARTESIAN_POINT('',(3.6,2.07320508075689,-29.075)) ;
#156041=CARTESIAN_POINT('Origin',(3.6,1.9,-28.975)) ;
#156042=CARTESIAN_POINT('',(3.6,2.1,-29.175)) ;
#156043=CARTESIAN_POINT('Origin',(3.6,1.9,-29.175)) ;
#156044=CARTESIAN_POINT('',(3.6,2.1,-31.785)) ;
#156045=CARTESIAN_POINT('',(3.6,2.1,0.)) ;
#156046=CARTESIAN_POINT('',(3.6,2.07320508075689,-31.885)) ;
#156047=CARTESIAN_POINT('Origin',(3.6,1.9,-31.785)) ;
#156048=CARTESIAN_POINT('',(3.6,2.1,-31.985)) ;
#156049=CARTESIAN_POINT('Origin',(3.6,1.9,-31.985)) ;
#156050=CARTESIAN_POINT('',(3.6,2.1,-32.785)) ;
#156051=CARTESIAN_POINT('',(3.6,2.1,-32.785)) ;
#156052=CARTESIAN_POINT('',(3.6,2.07320508075689,-32.885)) ;
#156053=CARTESIAN_POINT('Origin',(3.6,1.9,-32.785)) ;
#156054=CARTESIAN_POINT('',(3.6,2.1,-32.985)) ;
#156055=CARTESIAN_POINT('Origin',(3.6,1.9,-32.985)) ;
#156056=CARTESIAN_POINT('',(3.6,2.1,-35.595)) ;
#156057=CARTESIAN_POINT('',(3.6,2.1,0.)) ;
#156058=CARTESIAN_POINT('',(3.6,2.07320508075689,-35.695)) ;
#156059=CARTESIAN_POINT('Origin',(3.6,1.9,-35.595)) ;
#156060=CARTESIAN_POINT('Origin',(3.6,1.9,-35.795)) ;
#156061=CARTESIAN_POINT('Origin',(3.6,7.81406971160724E-17,0.)) ;
#156062=CARTESIAN_POINT('',(3.6,-2.35,-33.3868804065906)) ;
#156063=CARTESIAN_POINT('',(3.6,-2.32153024911032,-33.4897267659824)) ;
#156064=CARTESIAN_POINT('Origin',(3.6,-2.15,-33.3868804065906)) ;
#156065=CARTESIAN_POINT('',(3.6,-2.35,-32.985)) ;
#156066=CARTESIAN_POINT('',(3.6,-2.35,0.)) ;
#156067=CARTESIAN_POINT('',(3.6,-5.15,-32.985)) ;
#156068=CARTESIAN_POINT('',(3.6,-5.25,-32.985)) ;
#156069=CARTESIAN_POINT('',(3.6,-5.15,-35.595)) ;
#156070=CARTESIAN_POINT('',(3.6,-5.15,-35.695)) ;
#156071=CARTESIAN_POINT('',(3.6,-2.35,-35.595)) ;
#156072=CARTESIAN_POINT('',(3.6,-2.25,-35.595)) ;
#156073=CARTESIAN_POINT('',(3.6,-2.35,-35.1931195934094)) ;
#156074=CARTESIAN_POINT('',(3.6,-2.35,0.)) ;
#156075=CARTESIAN_POINT('',(3.6,-2.32153024911032,-35.0902732340176)) ;
#156076=CARTESIAN_POINT('Origin',(3.6,-2.15,-35.1931195934094)) ;
#156077=CARTESIAN_POINT('Origin',(3.6,-3.65625,-34.29)) ;
#156078=CARTESIAN_POINT('Origin',(3.6,7.81406971160724E-17,0.)) ;
#156079=CARTESIAN_POINT('',(3.6,-2.35,-29.5768804065906)) ;
#156080=CARTESIAN_POINT('',(3.6,-2.32153024911032,-29.6797267659824)) ;
#156081=CARTESIAN_POINT('Origin',(3.6,-2.15,-29.5768804065906)) ;
#156082=CARTESIAN_POINT('',(3.6,-2.35,-29.175)) ;
#156083=CARTESIAN_POINT('',(3.6,-2.35,0.)) ;
#156084=CARTESIAN_POINT('',(3.6,-5.15,-29.175)) ;
#156085=CARTESIAN_POINT('',(3.6,-5.25,-29.175)) ;
#156086=CARTESIAN_POINT('',(3.6,-5.15,-31.785)) ;
#156087=CARTESIAN_POINT('',(3.6,-5.15,-31.885)) ;
#156088=CARTESIAN_POINT('',(3.6,-2.35,-31.785)) ;
#156089=CARTESIAN_POINT('',(3.6,-2.25,-31.785)) ;
#156090=CARTESIAN_POINT('',(3.6,-2.35,-31.3831195934094)) ;
#156091=CARTESIAN_POINT('',(3.6,-2.35,0.)) ;
#156092=CARTESIAN_POINT('',(3.6,-2.32153024911032,-31.2802732340176)) ;
#156093=CARTESIAN_POINT('Origin',(3.6,-2.15,-31.3831195934094)) ;
#156094=CARTESIAN_POINT('Origin',(3.6,-3.65625,-30.48)) ;
#156095=CARTESIAN_POINT('Origin',(3.6,7.81406971160724E-17,0.)) ;
#156096=CARTESIAN_POINT('',(3.6,-2.35,-25.7668804065906)) ;
#156097=CARTESIAN_POINT('',(3.6,-2.32153024911032,-25.8697267659824)) ;
#156098=CARTESIAN_POINT('Origin',(3.6,-2.15,-25.7668804065906)) ;
#156099=CARTESIAN_POINT('',(3.6,-2.35,-25.365)) ;
#156100=CARTESIAN_POINT('',(3.6,-2.35,0.)) ;
#156101=CARTESIAN_POINT('',(3.6,-5.15,-25.365)) ;
#156102=CARTESIAN_POINT('',(3.6,-5.25,-25.365)) ;
#156103=CARTESIAN_POINT('',(3.6,-5.15,-27.975)) ;
#156104=CARTESIAN_POINT('',(3.6,-5.15,-28.075)) ;
#156105=CARTESIAN_POINT('',(3.6,-2.35,-27.975)) ;
#156106=CARTESIAN_POINT('',(3.6,-2.25,-27.975)) ;
#156107=CARTESIAN_POINT('',(3.6,-2.35,-27.5731195934094)) ;
#156108=CARTESIAN_POINT('',(3.6,-2.35,0.)) ;
#156109=CARTESIAN_POINT('',(3.6,-2.32153024911032,-27.4702732340176)) ;
#156110=CARTESIAN_POINT('Origin',(3.6,-2.15,-27.5731195934094)) ;
#156111=CARTESIAN_POINT('Origin',(3.6,-3.65625,-26.67)) ;
#156112=CARTESIAN_POINT('Origin',(3.6,7.81406971160724E-17,0.)) ;
#156113=CARTESIAN_POINT('',(3.6,-2.35,-21.9568804065906)) ;
#156114=CARTESIAN_POINT('',(3.6,-2.32153024911032,-22.0597267659824)) ;
#156115=CARTESIAN_POINT('Origin',(3.6,-2.15,-21.9568804065906)) ;
#156116=CARTESIAN_POINT('',(3.6,-2.35,-21.555)) ;
#156117=CARTESIAN_POINT('',(3.6,-2.35,0.)) ;
#156118=CARTESIAN_POINT('',(3.6,-5.15,-21.555)) ;
#156119=CARTESIAN_POINT('',(3.6,-5.25,-21.555)) ;
#156120=CARTESIAN_POINT('',(3.6,-5.15,-24.165)) ;
#156121=CARTESIAN_POINT('',(3.6,-5.15,-24.265)) ;
#156122=CARTESIAN_POINT('',(3.6,-2.35,-24.165)) ;
#156123=CARTESIAN_POINT('',(3.6,-2.25,-24.165)) ;
#156124=CARTESIAN_POINT('',(3.6,-2.35,-23.7631195934094)) ;
#156125=CARTESIAN_POINT('',(3.6,-2.35,0.)) ;
#156126=CARTESIAN_POINT('',(3.6,-2.32153024911032,-23.6602732340176)) ;
#156127=CARTESIAN_POINT('Origin',(3.6,-2.15,-23.7631195934094)) ;
#156128=CARTESIAN_POINT('Origin',(3.6,-3.65625,-22.86)) ;
#156129=CARTESIAN_POINT('Origin',(3.6,7.81406971160724E-17,0.)) ;
#156130=CARTESIAN_POINT('',(3.6,-2.35,-18.1468804065906)) ;
#156131=CARTESIAN_POINT('',(3.6,-2.32153024911032,-18.2497267659824)) ;
#156132=CARTESIAN_POINT('Origin',(3.6,-2.15,-18.1468804065906)) ;
#156133=CARTESIAN_POINT('',(3.6,-2.35,-17.745)) ;
#156134=CARTESIAN_POINT('',(3.6,-2.35,0.)) ;
#156135=CARTESIAN_POINT('',(3.6,-5.15,-17.745)) ;
#156136=CARTESIAN_POINT('',(3.6,-5.25,-17.745)) ;
#156137=CARTESIAN_POINT('',(3.6,-5.15,-20.355)) ;
#156138=CARTESIAN_POINT('',(3.6,-5.15,-20.455)) ;
#156139=CARTESIAN_POINT('',(3.6,-2.35,-20.355)) ;
#156140=CARTESIAN_POINT('',(3.6,-2.25,-20.355)) ;
#156141=CARTESIAN_POINT('',(3.6,-2.35,-19.9531195934094)) ;
#156142=CARTESIAN_POINT('',(3.6,-2.35,0.)) ;
#156143=CARTESIAN_POINT('',(3.6,-2.32153024911032,-19.8502732340176)) ;
#156144=CARTESIAN_POINT('Origin',(3.6,-2.15,-19.9531195934094)) ;
#156145=CARTESIAN_POINT('Origin',(3.6,-3.65625,-19.05)) ;
#156146=CARTESIAN_POINT('Origin',(3.6,7.81406971160724E-17,0.)) ;
#156147=CARTESIAN_POINT('',(3.6,-2.35,-14.3368804065906)) ;
#156148=CARTESIAN_POINT('',(3.6,-2.32153024911032,-14.4397267659824)) ;
#156149=CARTESIAN_POINT('Origin',(3.6,-2.15,-14.3368804065906)) ;
#156150=CARTESIAN_POINT('',(3.6,-2.35,-13.935)) ;
#156151=CARTESIAN_POINT('',(3.6,-2.35,0.)) ;
#156152=CARTESIAN_POINT('',(3.6,-5.15,-13.935)) ;
#156153=CARTESIAN_POINT('',(3.6,-5.25,-13.935)) ;
#156154=CARTESIAN_POINT('',(3.6,-5.15,-16.545)) ;
#156155=CARTESIAN_POINT('',(3.6,-5.15,-16.645)) ;
#156156=CARTESIAN_POINT('',(3.6,-2.35,-16.545)) ;
#156157=CARTESIAN_POINT('',(3.6,-2.25,-16.545)) ;
#156158=CARTESIAN_POINT('',(3.6,-2.35,-16.1431195934094)) ;
#156159=CARTESIAN_POINT('',(3.6,-2.35,0.)) ;
#156160=CARTESIAN_POINT('',(3.6,-2.32153024911032,-16.0402732340176)) ;
#156161=CARTESIAN_POINT('Origin',(3.6,-2.15,-16.1431195934094)) ;
#156162=CARTESIAN_POINT('Origin',(3.6,-3.65625,-15.24)) ;
#156163=CARTESIAN_POINT('Origin',(3.6,7.81406971160724E-17,0.)) ;
#156164=CARTESIAN_POINT('',(3.6,-2.35,-10.5268804065906)) ;
#156165=CARTESIAN_POINT('',(3.6,-2.32153024911032,-10.6297267659824)) ;
#156166=CARTESIAN_POINT('Origin',(3.6,-2.15,-10.5268804065906)) ;
#156167=CARTESIAN_POINT('',(3.6,-2.35,-10.125)) ;
#156168=CARTESIAN_POINT('',(3.6,-2.35,0.)) ;
#156169=CARTESIAN_POINT('',(3.6,-5.15,-10.125)) ;
#156170=CARTESIAN_POINT('',(3.6,-5.25,-10.125)) ;
#156171=CARTESIAN_POINT('',(3.6,-5.15,-12.735)) ;
#156172=CARTESIAN_POINT('',(3.6,-5.15,-12.835)) ;
#156173=CARTESIAN_POINT('',(3.6,-2.35,-12.735)) ;
#156174=CARTESIAN_POINT('',(3.6,-2.25,-12.735)) ;
#156175=CARTESIAN_POINT('',(3.6,-2.35,-12.3331195934094)) ;
#156176=CARTESIAN_POINT('',(3.6,-2.35,0.)) ;
#156177=CARTESIAN_POINT('',(3.6,-2.32153024911032,-12.2302732340176)) ;
#156178=CARTESIAN_POINT('Origin',(3.6,-2.15,-12.3331195934094)) ;
#156179=CARTESIAN_POINT('Origin',(3.6,-3.65625,-11.43)) ;
#156180=CARTESIAN_POINT('Origin',(3.6,7.81406971160724E-17,0.)) ;
#156181=CARTESIAN_POINT('',(3.6,-2.35,-6.71688040659058)) ;
#156182=CARTESIAN_POINT('',(3.6,-2.32153024911032,-6.8197267659824)) ;
#156183=CARTESIAN_POINT('Origin',(3.6,-2.15,-6.71688040659058)) ;
#156184=CARTESIAN_POINT('',(3.6,-2.35,-6.315)) ;
#156185=CARTESIAN_POINT('',(3.6,-2.35,0.)) ;
#156186=CARTESIAN_POINT('',(3.6,-5.15,-6.315)) ;
#156187=CARTESIAN_POINT('',(3.6,-5.25,-6.315)) ;
#156188=CARTESIAN_POINT('',(3.6,-5.15,-8.925)) ;
#156189=CARTESIAN_POINT('',(3.6,-5.15,-9.025)) ;
#156190=CARTESIAN_POINT('',(3.6,-2.35,-8.925)) ;
#156191=CARTESIAN_POINT('',(3.6,-2.25,-8.925)) ;
#156192=CARTESIAN_POINT('',(3.6,-2.35,-8.52311959340942)) ;
#156193=CARTESIAN_POINT('',(3.6,-2.35,0.)) ;
#156194=CARTESIAN_POINT('',(3.6,-2.32153024911032,-8.4202732340176)) ;
#156195=CARTESIAN_POINT('Origin',(3.6,-2.15,-8.52311959340942)) ;
#156196=CARTESIAN_POINT('Origin',(3.6,-3.65625,-7.62)) ;
#156197=CARTESIAN_POINT('Origin',(3.6,7.81406971160724E-17,0.)) ;
#156198=CARTESIAN_POINT('',(3.6,-2.35,-2.90688040659058)) ;
#156199=CARTESIAN_POINT('',(3.6,-2.32153024911032,-3.0097267659824)) ;
#156200=CARTESIAN_POINT('Origin',(3.6,-2.15,-2.90688040659058)) ;
#156201=CARTESIAN_POINT('',(3.6,-2.35,-2.505)) ;
#156202=CARTESIAN_POINT('',(3.6,-2.35,0.)) ;
#156203=CARTESIAN_POINT('',(3.6,-5.15,-2.505)) ;
#156204=CARTESIAN_POINT('',(3.6,-5.25,-2.505)) ;
#156205=CARTESIAN_POINT('',(3.6,-5.15,-5.115)) ;
#156206=CARTESIAN_POINT('',(3.6,-5.15,-5.215)) ;
#156207=CARTESIAN_POINT('',(3.6,-2.35,-5.115)) ;
#156208=CARTESIAN_POINT('',(3.6,-2.25,-5.115)) ;
#156209=CARTESIAN_POINT('',(3.6,-2.35,-4.71311959340942)) ;
#156210=CARTESIAN_POINT('',(3.6,-2.35,0.)) ;
#156211=CARTESIAN_POINT('',(3.6,-2.32153024911032,-4.6102732340176)) ;
#156212=CARTESIAN_POINT('Origin',(3.6,-2.15,-4.71311959340942)) ;
#156213=CARTESIAN_POINT('Origin',(3.6,-3.65625,-3.81)) ;
#156214=CARTESIAN_POINT('Origin',(2.6,4.55,-36.59)) ;
#156215=CARTESIAN_POINT('',(2.6,2.85,-36.49)) ;
#156216=CARTESIAN_POINT('',(2.6,4.45,-36.49)) ;
#156217=CARTESIAN_POINT('',(2.6,4.55,-36.49)) ;
#156218=CARTESIAN_POINT('',(2.6,4.45,-35.94)) ;
#156219=CARTESIAN_POINT('',(2.6,4.45,-36.59)) ;
#156220=CARTESIAN_POINT('',(2.6,2.85,-35.94)) ;
#156221=CARTESIAN_POINT('',(2.6,2.75,-35.94)) ;
#156222=CARTESIAN_POINT('',(2.6,2.85,-36.59)) ;
#156223=CARTESIAN_POINT('Origin',(2.6,4.55,-36.59)) ;
#156224=CARTESIAN_POINT('',(2.6,-6.45,2.2)) ;
#156225=CARTESIAN_POINT('',(2.6,-6.45,-36.49)) ;
#156226=CARTESIAN_POINT('',(2.6,-6.45,-36.59)) ;
#156227=CARTESIAN_POINT('',(2.6,1.9,-36.49)) ;
#156228=CARTESIAN_POINT('',(2.6,4.55,-36.49)) ;
#156229=CARTESIAN_POINT('',(2.6,1.9,-35.795)) ;
#156230=CARTESIAN_POINT('',(2.6,1.9,-36.59)) ;
#156231=CARTESIAN_POINT('',(2.6,-5.15,-35.795)) ;
#156232=CARTESIAN_POINT('',(2.6,4.55,-35.795)) ;
#156233=CARTESIAN_POINT('',(2.6,-5.35,-35.595)) ;
#156234=CARTESIAN_POINT('Origin',(2.6,-5.15,-35.595)) ;
#156235=CARTESIAN_POINT('',(2.6,-5.35,-32.985)) ;
#156236=CARTESIAN_POINT('',(2.6,-5.35,-36.59)) ;
#156237=CARTESIAN_POINT('',(2.6,-5.15,-32.785)) ;
#156238=CARTESIAN_POINT('Origin',(2.6,-5.15,-32.985)) ;
#156239=CARTESIAN_POINT('',(2.6,1.9,-32.785)) ;
#156240=CARTESIAN_POINT('',(2.6,4.55,-32.785)) ;
#156241=CARTESIAN_POINT('',(2.6,1.9,-31.985)) ;
#156242=CARTESIAN_POINT('',(2.6,1.9,-36.59)) ;
#156243=CARTESIAN_POINT('',(2.6,-5.15,-31.985)) ;
#156244=CARTESIAN_POINT('',(2.6,4.55,-31.985)) ;
#156245=CARTESIAN_POINT('',(2.6,-5.35,-31.785)) ;
#156246=CARTESIAN_POINT('Origin',(2.6,-5.15,-31.785)) ;
#156247=CARTESIAN_POINT('',(2.6,-5.35,-29.175)) ;
#156248=CARTESIAN_POINT('',(2.6,-5.35,-36.59)) ;
#156249=CARTESIAN_POINT('',(2.6,-5.15,-28.975)) ;
#156250=CARTESIAN_POINT('Origin',(2.6,-5.15,-29.175)) ;
#156251=CARTESIAN_POINT('',(2.6,1.9,-28.975)) ;
#156252=CARTESIAN_POINT('',(2.6,4.55,-28.975)) ;
#156253=CARTESIAN_POINT('',(2.6,1.9,-28.175)) ;
#156254=CARTESIAN_POINT('',(2.6,1.9,-36.59)) ;
#156255=CARTESIAN_POINT('',(2.6,-5.15,-28.175)) ;
#156256=CARTESIAN_POINT('',(2.6,4.55,-28.175)) ;
#156257=CARTESIAN_POINT('',(2.6,-5.35,-27.975)) ;
#156258=CARTESIAN_POINT('Origin',(2.6,-5.15,-27.975)) ;
#156259=CARTESIAN_POINT('',(2.6,-5.35,-25.365)) ;
#156260=CARTESIAN_POINT('',(2.6,-5.35,-36.59)) ;
#156261=CARTESIAN_POINT('',(2.6,-5.15,-25.165)) ;
#156262=CARTESIAN_POINT('Origin',(2.6,-5.15,-25.365)) ;
#156263=CARTESIAN_POINT('',(2.6,1.9,-25.165)) ;
#156264=CARTESIAN_POINT('',(2.6,4.55,-25.165)) ;
#156265=CARTESIAN_POINT('',(2.6,1.9,-24.365)) ;
#156266=CARTESIAN_POINT('',(2.6,1.89999999999999,-36.59)) ;
#156267=CARTESIAN_POINT('',(2.6,-5.15,-24.365)) ;
#156268=CARTESIAN_POINT('',(2.6,4.55,-24.365)) ;
#156269=CARTESIAN_POINT('',(2.6,-5.35,-24.165)) ;
#156270=CARTESIAN_POINT('Origin',(2.6,-5.15,-24.165)) ;
#156271=CARTESIAN_POINT('',(2.6,-5.35,-21.555)) ;
#156272=CARTESIAN_POINT('',(2.6,-5.35,-36.59)) ;
#156273=CARTESIAN_POINT('',(2.6,-5.15,-21.355)) ;
#156274=CARTESIAN_POINT('Origin',(2.6,-5.15,-21.555)) ;
#156275=CARTESIAN_POINT('',(2.6,1.9,-21.355)) ;
#156276=CARTESIAN_POINT('',(2.6,4.55,-21.355)) ;
#156277=CARTESIAN_POINT('',(2.6,1.9,-20.555)) ;
#156278=CARTESIAN_POINT('',(2.6,1.89999999999999,-36.59)) ;
#156279=CARTESIAN_POINT('',(2.6,-5.15,-20.555)) ;
#156280=CARTESIAN_POINT('',(2.6,4.55,-20.555)) ;
#156281=CARTESIAN_POINT('',(2.6,-5.35,-20.355)) ;
#156282=CARTESIAN_POINT('Origin',(2.6,-5.15,-20.355)) ;
#156283=CARTESIAN_POINT('',(2.6,-5.35,-17.745)) ;
#156284=CARTESIAN_POINT('',(2.6,-5.35,-36.59)) ;
#156285=CARTESIAN_POINT('',(2.6,-5.15,-17.545)) ;
#156286=CARTESIAN_POINT('Origin',(2.6,-5.15,-17.745)) ;
#156287=CARTESIAN_POINT('',(2.6,1.9,-17.545)) ;
#156288=CARTESIAN_POINT('',(2.6,4.55,-17.545)) ;
#156289=CARTESIAN_POINT('',(2.6,1.9,-16.745)) ;
#156290=CARTESIAN_POINT('',(2.6,1.89999999999999,-36.59)) ;
#156291=CARTESIAN_POINT('',(2.6,-5.15,-16.745)) ;
#156292=CARTESIAN_POINT('',(2.6,4.55,-16.745)) ;
#156293=CARTESIAN_POINT('',(2.6,-5.35,-16.545)) ;
#156294=CARTESIAN_POINT('Origin',(2.6,-5.15,-16.545)) ;
#156295=CARTESIAN_POINT('',(2.6,-5.35,-13.935)) ;
#156296=CARTESIAN_POINT('',(2.6,-5.35,-36.59)) ;
#156297=CARTESIAN_POINT('',(2.6,-5.15,-13.735)) ;
#156298=CARTESIAN_POINT('Origin',(2.6,-5.15,-13.935)) ;
#156299=CARTESIAN_POINT('',(2.6,1.9,-13.735)) ;
#156300=CARTESIAN_POINT('',(2.6,4.55,-13.735)) ;
#156301=CARTESIAN_POINT('',(2.6,1.9,-12.935)) ;
#156302=CARTESIAN_POINT('',(2.6,1.89999999999999,-36.59)) ;
#156303=CARTESIAN_POINT('',(2.6,-5.15,-12.935)) ;
#156304=CARTESIAN_POINT('',(2.6,4.55,-12.935)) ;
#156305=CARTESIAN_POINT('',(2.6,-5.35,-12.735)) ;
#156306=CARTESIAN_POINT('Origin',(2.6,-5.15,-12.735)) ;
#156307=CARTESIAN_POINT('',(2.6,-5.35,-10.125)) ;
#156308=CARTESIAN_POINT('',(2.6,-5.35,-36.59)) ;
#156309=CARTESIAN_POINT('',(2.6,-5.15,-9.925)) ;
#156310=CARTESIAN_POINT('Origin',(2.6,-5.15,-10.125)) ;
#156311=CARTESIAN_POINT('',(2.6,1.9,-9.925)) ;
#156312=CARTESIAN_POINT('',(2.6,4.55,-9.925)) ;
#156313=CARTESIAN_POINT('',(2.6,1.9,-9.125)) ;
#156314=CARTESIAN_POINT('',(2.6,1.89999999999999,-36.59)) ;
#156315=CARTESIAN_POINT('',(2.6,-5.15,-9.125)) ;
#156316=CARTESIAN_POINT('',(2.6,4.55,-9.125)) ;
#156317=CARTESIAN_POINT('',(2.6,-5.35,-8.925)) ;
#156318=CARTESIAN_POINT('Origin',(2.6,-5.15,-8.925)) ;
#156319=CARTESIAN_POINT('',(2.6,-5.35,-6.315)) ;
#156320=CARTESIAN_POINT('',(2.6,-5.35,-36.59)) ;
#156321=CARTESIAN_POINT('',(2.6,-5.15,-6.115)) ;
#156322=CARTESIAN_POINT('Origin',(2.6,-5.15,-6.315)) ;
#156323=CARTESIAN_POINT('',(2.6,1.9,-6.115)) ;
#156324=CARTESIAN_POINT('',(2.6,4.55,-6.115)) ;
#156325=CARTESIAN_POINT('',(2.6,1.9,-5.315)) ;
#156326=CARTESIAN_POINT('',(2.6,1.89999999999999,-36.59)) ;
#156327=CARTESIAN_POINT('',(2.6,-5.15,-5.315)) ;
#156328=CARTESIAN_POINT('',(2.6,4.55,-5.315)) ;
#156329=CARTESIAN_POINT('',(2.6,-5.35,-5.115)) ;
#156330=CARTESIAN_POINT('Origin',(2.6,-5.15,-5.115)) ;
#156331=CARTESIAN_POINT('',(2.6,-5.35,-2.505)) ;
#156332=CARTESIAN_POINT('',(2.6,-5.35,-36.59)) ;
#156333=CARTESIAN_POINT('',(2.6,-5.15,-2.305)) ;
#156334=CARTESIAN_POINT('Origin',(2.6,-5.15,-2.505)) ;
#156335=CARTESIAN_POINT('',(2.6,1.9,-2.305)) ;
#156336=CARTESIAN_POINT('',(2.6,4.55,-2.305)) ;
#156337=CARTESIAN_POINT('',(2.6,1.9,-1.505)) ;
#156338=CARTESIAN_POINT('',(2.6,1.89999999999998,-36.59)) ;
#156339=CARTESIAN_POINT('',(2.6,-5.15,-1.505)) ;
#156340=CARTESIAN_POINT('',(2.6,4.55,-1.505)) ;
#156341=CARTESIAN_POINT('',(2.6,-5.35,-1.305)) ;
#156342=CARTESIAN_POINT('Origin',(2.6,-5.15,-1.305)) ;
#156343=CARTESIAN_POINT('',(2.6,-5.35,1.305)) ;
#156344=CARTESIAN_POINT('',(2.6,-5.35,-36.59)) ;
#156345=CARTESIAN_POINT('',(2.6,-5.15,1.505)) ;
#156346=CARTESIAN_POINT('Origin',(2.6,-5.15,1.305)) ;
#156347=CARTESIAN_POINT('',(2.6,1.9,1.505)) ;
#156348=CARTESIAN_POINT('',(2.6,4.55,1.505)) ;
#156349=CARTESIAN_POINT('',(2.6,1.9,2.2)) ;
#156350=CARTESIAN_POINT('',(2.6,1.90000000000002,-36.59)) ;
#156351=CARTESIAN_POINT('',(2.6,-6.45,2.2)) ;
#156352=CARTESIAN_POINT('Origin',(3.5,2.65,0.)) ;
#156353=CARTESIAN_POINT('',(3.5,2.75,2.2)) ;
#156354=CARTESIAN_POINT('',(3.5,2.75,-36.49)) ;
#156355=CARTESIAN_POINT('',(3.5,2.75,-2.3)) ;
#156356=CARTESIAN_POINT('Origin',(3.5,2.65,2.2)) ;
#156357=CARTESIAN_POINT('Origin',(3.5,2.65,-36.49)) ;
#156358=CARTESIAN_POINT('Origin',(3.5,2.1,-1.01757522333835E-15)) ;
#156359=CARTESIAN_POINT('',(3.5,2.,-2.305)) ;
#156360=CARTESIAN_POINT('',(3.5,2.,-1.505)) ;
#156361=CARTESIAN_POINT('',(3.5,2.,-1.505)) ;
#156362=CARTESIAN_POINT('',(3.55,2.01339745962156,-2.305)) ;
#156363=CARTESIAN_POINT('Origin',(3.5,2.1,-2.305)) ;
#156364=CARTESIAN_POINT('Origin',(3.5,2.1,-2.305)) ;
#156365=CARTESIAN_POINT('',(3.55,2.01339745962156,-1.505)) ;
#156366=CARTESIAN_POINT('Origin',(3.5,2.1,-1.505)) ;
#156367=CARTESIAN_POINT('Origin',(3.5,2.1,-1.505)) ;
#156368=CARTESIAN_POINT('Origin',(-5.9,-6.55,-36.59)) ;
#156369=CARTESIAN_POINT('',(-5.9,0.35,-36.49)) ;
#156370=CARTESIAN_POINT('',(-5.9,-6.45,-36.49)) ;
#156371=CARTESIAN_POINT('',(-5.9,-6.55,-36.49)) ;
#156372=CARTESIAN_POINT('',(-5.9,-6.45,2.2)) ;
#156373=CARTESIAN_POINT('',(-5.9,-6.45,-36.59)) ;
#156374=CARTESIAN_POINT('',(-5.9,0.35,2.2)) ;
#156375=CARTESIAN_POINT('',(-5.9,0.45,2.2)) ;
#156376=CARTESIAN_POINT('',(-5.9,0.35,-36.59)) ;
#156377=CARTESIAN_POINT('',(-5.9,-5.62807764064044,-2.31)) ;
#156378=CARTESIAN_POINT('',(-5.9,-5.42192235935956,-2.11)) ;
#156379=CARTESIAN_POINT('Ctrl Pts',(-5.9,-5.62807764064044,-2.31)) ;
#156380=CARTESIAN_POINT('Ctrl Pts',(-5.9,-5.6280776389491,-2.25749316946912)) ;
#156381=CARTESIAN_POINT('Ctrl Pts',(-5.9,-5.60585949344389,-2.20560251865551)) ;
#156382=CARTESIAN_POINT('Ctrl Pts',(-5.9,-5.5295328200175,-2.13155476886987)) ;
#156383=CARTESIAN_POINT('Ctrl Pts',(-5.9,-5.47604516144825,-2.11000000149821)) ;
#156384=CARTESIAN_POINT('Ctrl Pts',(-5.9,-5.42192235935956,-2.11)) ;
#156385=CARTESIAN_POINT('',(-5.9,-5.62807764064044,-5.31)) ;
#156386=CARTESIAN_POINT('',(-5.9,-5.62807764064044,-36.59)) ;
#156387=CARTESIAN_POINT('',(-5.9,-5.42192235935956,-5.51)) ;
#156388=CARTESIAN_POINT('Ctrl Pts',(-5.9,-5.42192235935956,-5.51)) ;
#156389=CARTESIAN_POINT('Ctrl Pts',(-5.9,-5.47604516144824,-5.50999999850184)) ;
#156390=CARTESIAN_POINT('Ctrl Pts',(-5.9,-5.52953282001752,-5.48844523113013)) ;
#156391=CARTESIAN_POINT('Ctrl Pts',(-5.9,-5.60585949344386,-5.41439748134449)) ;
#156392=CARTESIAN_POINT('Ctrl Pts',(-5.9,-5.6280776389491,-5.36250683053088)) ;
#156393=CARTESIAN_POINT('Ctrl Pts',(-5.9,-5.62807764064044,-5.31)) ;
#156394=CARTESIAN_POINT('',(-5.9,-1.2914213562373,-5.51)) ;
#156395=CARTESIAN_POINT('',(-5.9,-1.04999999999999,-5.51)) ;
#156396=CARTESIAN_POINT('',(-5.9,-1.00857864376269,-5.31)) ;
#156397=CARTESIAN_POINT('Ctrl Pts',(-5.9,-1.00857864376269,-5.31)) ;
#156398=CARTESIAN_POINT('Ctrl Pts',(-5.9,-1.00857864608315,-5.36250686562998)) ;
#156399=CARTESIAN_POINT('Ctrl Pts',(-5.9,-1.03906162412146,-5.41439743459706)) ;
#156400=CARTESIAN_POINT('Ctrl Pts',(-5.9,-1.14378108835315,-5.48844527787756)) ;
#156401=CARTESIAN_POINT('Ctrl Pts',(-5.9,-1.21716543471637,-5.50999999941992)) ;
#156402=CARTESIAN_POINT('Ctrl Pts',(-5.9,-1.2914213562373,-5.51)) ;
#156403=CARTESIAN_POINT('',(-5.9,-1.00857864376269,-2.31)) ;
#156404=CARTESIAN_POINT('',(-5.9,-1.00857864376269,-36.59)) ;
#156405=CARTESIAN_POINT('',(-5.9,-1.29142135623731,-2.11)) ;
#156406=CARTESIAN_POINT('Ctrl Pts',(-5.9,-1.29142135623731,-2.11)) ;
#156407=CARTESIAN_POINT('Ctrl Pts',(-5.9,-1.21716543471638,-2.11000000058011)) ;
#156408=CARTESIAN_POINT('Ctrl Pts',(-5.9,-1.14378108835315,-2.13155472212247)) ;
#156409=CARTESIAN_POINT('Ctrl Pts',(-5.9,-1.03906162412146,-2.20560256540291)) ;
#156410=CARTESIAN_POINT('Ctrl Pts',(-5.9,-1.00857864608315,-2.25749313437004)) ;
#156411=CARTESIAN_POINT('Ctrl Pts',(-5.9,-1.00857864376269,-2.31)) ;
#156412=CARTESIAN_POINT('',(-5.9,-5.55,-2.11)) ;
#156413=CARTESIAN_POINT('',(-5.9,-5.62807764064044,-5.92)) ;
#156414=CARTESIAN_POINT('',(-5.9,-5.62807764064044,-9.32)) ;
#156415=CARTESIAN_POINT('',(-5.9,-5.62807764064044,-36.59)) ;
#156416=CARTESIAN_POINT('',(-5.9,-1.00857864376269,-9.32)) ;
#156417=CARTESIAN_POINT('',(-5.9,-1.04999999999999,-9.32)) ;
#156418=CARTESIAN_POINT('',(-5.9,-1.00857864376269,-5.92)) ;
#156419=CARTESIAN_POINT('',(-5.9,-1.00857864376269,-36.59)) ;
#156420=CARTESIAN_POINT('',(-5.9,-5.55,-5.92)) ;
#156421=CARTESIAN_POINT('',(-5.9,-5.62807764064044,-9.73)) ;
#156422=CARTESIAN_POINT('',(-5.9,-5.62807764064044,-13.13)) ;
#156423=CARTESIAN_POINT('',(-5.9,-5.62807764064044,-36.59)) ;
#156424=CARTESIAN_POINT('',(-5.9,-1.00857864376269,-13.13)) ;
#156425=CARTESIAN_POINT('',(-5.9,-1.04999999999999,-13.13)) ;
#156426=CARTESIAN_POINT('',(-5.9,-1.00857864376269,-9.73)) ;
#156427=CARTESIAN_POINT('',(-5.9,-1.00857864376269,-36.59)) ;
#156428=CARTESIAN_POINT('',(-5.9,-5.55,-9.73)) ;
#156429=CARTESIAN_POINT('',(-5.9,-5.62807764064044,-13.54)) ;
#156430=CARTESIAN_POINT('',(-5.9,-5.62807764064044,-16.94)) ;
#156431=CARTESIAN_POINT('',(-5.9,-5.62807764064044,-36.59)) ;
#156432=CARTESIAN_POINT('',(-5.9,-1.00857864376269,-16.94)) ;
#156433=CARTESIAN_POINT('',(-5.9,-1.04999999999999,-16.94)) ;
#156434=CARTESIAN_POINT('',(-5.9,-1.00857864376269,-13.54)) ;
#156435=CARTESIAN_POINT('',(-5.9,-1.00857864376269,-36.59)) ;
#156436=CARTESIAN_POINT('',(-5.9,-5.55,-13.54)) ;
#156437=CARTESIAN_POINT('',(-5.9,-5.62807764064044,-17.35)) ;
#156438=CARTESIAN_POINT('',(-5.9,-5.62807764064044,-20.75)) ;
#156439=CARTESIAN_POINT('',(-5.9,-5.62807764064044,-36.59)) ;
#156440=CARTESIAN_POINT('',(-5.9,-1.00857864376269,-20.75)) ;
#156441=CARTESIAN_POINT('',(-5.9,-1.04999999999999,-20.75)) ;
#156442=CARTESIAN_POINT('',(-5.9,-1.00857864376269,-17.35)) ;
#156443=CARTESIAN_POINT('',(-5.9,-1.00857864376269,-36.59)) ;
#156444=CARTESIAN_POINT('',(-5.9,-5.55,-17.35)) ;
#156445=CARTESIAN_POINT('',(-5.9,-5.62807764064044,-21.16)) ;
#156446=CARTESIAN_POINT('',(-5.9,-5.62807764064044,-24.56)) ;
#156447=CARTESIAN_POINT('',(-5.9,-5.62807764064044,-36.59)) ;
#156448=CARTESIAN_POINT('',(-5.9,-1.00857864376269,-24.56)) ;
#156449=CARTESIAN_POINT('',(-5.9,-1.04999999999999,-24.56)) ;
#156450=CARTESIAN_POINT('',(-5.9,-1.00857864376269,-21.16)) ;
#156451=CARTESIAN_POINT('',(-5.9,-1.00857864376269,-36.59)) ;
#156452=CARTESIAN_POINT('',(-5.9,-5.55,-21.16)) ;
#156453=CARTESIAN_POINT('',(-5.9,-5.62807764064044,-24.97)) ;
#156454=CARTESIAN_POINT('',(-5.9,-5.62807764064044,-28.37)) ;
#156455=CARTESIAN_POINT('',(-5.9,-5.62807764064044,-36.59)) ;
#156456=CARTESIAN_POINT('',(-5.9,-1.00857864376269,-28.37)) ;
#156457=CARTESIAN_POINT('',(-5.9,-1.04999999999999,-28.37)) ;
#156458=CARTESIAN_POINT('',(-5.9,-1.00857864376269,-24.97)) ;
#156459=CARTESIAN_POINT('',(-5.9,-1.00857864376269,-36.59)) ;
#156460=CARTESIAN_POINT('',(-5.9,-5.55,-24.97)) ;
#156461=CARTESIAN_POINT('',(-5.9,-5.62807764064044,-28.78)) ;
#156462=CARTESIAN_POINT('',(-5.9,-5.62807764064044,-32.18)) ;
#156463=CARTESIAN_POINT('',(-5.9,-5.62807764064044,-36.59)) ;
#156464=CARTESIAN_POINT('',(-5.9,-1.00857864376269,-32.18)) ;
#156465=CARTESIAN_POINT('',(-5.9,-1.04999999999999,-32.18)) ;
#156466=CARTESIAN_POINT('',(-5.9,-1.00857864376269,-28.78)) ;
#156467=CARTESIAN_POINT('',(-5.9,-1.00857864376269,-36.59)) ;
#156468=CARTESIAN_POINT('',(-5.9,-5.55,-28.78)) ;
#156469=CARTESIAN_POINT('',(-5.9,-5.62807764064044,-32.59)) ;
#156470=CARTESIAN_POINT('',(-5.9,-5.62807764064044,-35.99)) ;
#156471=CARTESIAN_POINT('',(-5.9,-5.62807764064044,-36.59)) ;
#156472=CARTESIAN_POINT('',(-5.9,-1.00857864376269,-35.99)) ;
#156473=CARTESIAN_POINT('',(-5.9,-1.04999999999999,-35.99)) ;
#156474=CARTESIAN_POINT('',(-5.9,-1.00857864376269,-32.59)) ;
#156475=CARTESIAN_POINT('',(-5.9,-1.00857864376269,-36.59)) ;
#156476=CARTESIAN_POINT('',(-5.9,-5.55,-32.59)) ;
#156477=CARTESIAN_POINT('',(-5.9,-5.62807764064044,1.5)) ;
#156478=CARTESIAN_POINT('',(-5.9,-5.42192235935956,1.7)) ;
#156479=CARTESIAN_POINT('Ctrl Pts',(-5.9,-5.62807764064044,1.5)) ;
#156480=CARTESIAN_POINT('Ctrl Pts',(-5.9,-5.6280776389491,1.55250683053087)) ;
#156481=CARTESIAN_POINT('Ctrl Pts',(-5.9,-5.60585949344389,1.6043974813445)) ;
#156482=CARTESIAN_POINT('Ctrl Pts',(-5.9,-5.5295328200175,1.67844523113012)) ;
#156483=CARTESIAN_POINT('Ctrl Pts',(-5.9,-5.47604516144825,1.69999999850179)) ;
#156484=CARTESIAN_POINT('Ctrl Pts',(-5.9,-5.42192235935956,1.7)) ;
#156485=CARTESIAN_POINT('',(-5.9,-5.62807764064044,-1.5)) ;
#156486=CARTESIAN_POINT('',(-5.9,-5.62807764064044,-36.59)) ;
#156487=CARTESIAN_POINT('',(-5.9,-5.42192235935956,-1.7)) ;
#156488=CARTESIAN_POINT('Ctrl Pts',(-5.9,-5.42192235935956,-1.7)) ;
#156489=CARTESIAN_POINT('Ctrl Pts',(-5.9,-5.47604516144823,-1.69999999850179)) ;
#156490=CARTESIAN_POINT('Ctrl Pts',(-5.9,-5.52953282001752,-1.67844523113013)) ;
#156491=CARTESIAN_POINT('Ctrl Pts',(-5.9,-5.60585949344386,-1.60439748134449)) ;
#156492=CARTESIAN_POINT('Ctrl Pts',(-5.9,-5.6280776389491,-1.55250683053088)) ;
#156493=CARTESIAN_POINT('Ctrl Pts',(-5.9,-5.62807764064044,-1.5)) ;
#156494=CARTESIAN_POINT('',(-5.9,-1.2914213562373,-1.7)) ;
#156495=CARTESIAN_POINT('',(-5.9,-1.04999999999999,-1.7)) ;
#156496=CARTESIAN_POINT('',(-5.9,-1.00857864376268,-1.5)) ;
#156497=CARTESIAN_POINT('Ctrl Pts',(-5.9,-1.00857864376268,-1.5)) ;
#156498=CARTESIAN_POINT('Ctrl Pts',(-5.9,-1.00857864608314,-1.55250686562996)) ;
#156499=CARTESIAN_POINT('Ctrl Pts',(-5.9,-1.03906162412144,-1.60439743459708)) ;
#156500=CARTESIAN_POINT('Ctrl Pts',(-5.9,-1.14378108835315,-1.67844527787754)) ;
#156501=CARTESIAN_POINT('Ctrl Pts',(-5.9,-1.21716543471636,-1.69999999941986)) ;
#156502=CARTESIAN_POINT('Ctrl Pts',(-5.9,-1.2914213562373,-1.7)) ;
#156503=CARTESIAN_POINT('',(-5.9,-1.00857864376268,1.5)) ;
#156504=CARTESIAN_POINT('',(-5.9,-1.00857864376268,-36.59)) ;
#156505=CARTESIAN_POINT('',(-5.9,-1.2914213562373,1.7)) ;
#156506=CARTESIAN_POINT('Ctrl Pts',(-5.9,-1.2914213562373,1.7)) ;
#156507=CARTESIAN_POINT('Ctrl Pts',(-5.9,-1.21716543471637,1.69999999941986)) ;
#156508=CARTESIAN_POINT('Ctrl Pts',(-5.9,-1.14378108835315,1.67844527787754)) ;
#156509=CARTESIAN_POINT('Ctrl Pts',(-5.9,-1.03906162412145,1.60439743459708)) ;
#156510=CARTESIAN_POINT('Ctrl Pts',(-5.9,-1.00857864608316,1.55250686562996)) ;
#156511=CARTESIAN_POINT('Ctrl Pts',(-5.9,-1.00857864376268,1.5)) ;
#156512=CARTESIAN_POINT('',(-5.9,-5.55,1.7)) ;
#156513=CARTESIAN_POINT('Origin',(10.2,2.,1.405)) ;
#156514=CARTESIAN_POINT('',(10.1,2.,1.305)) ;
#156515=CARTESIAN_POINT('',(10.1,2.,-1.305)) ;
#156516=CARTESIAN_POINT('',(10.1,2.,-1.405)) ;
#156517=CARTESIAN_POINT('',(3.7,2.,-1.305)) ;
#156518=CARTESIAN_POINT('',(10.2,2.,-1.305)) ;
#156519=CARTESIAN_POINT('',(3.7,2.,1.305)) ;
#156520=CARTESIAN_POINT('',(3.7,2.,1.405)) ;
#156521=CARTESIAN_POINT('',(10.2,2.,1.305)) ;
#156522=CARTESIAN_POINT('',(9.8,2.,-0.399999999999999)) ;
#156523=CARTESIAN_POINT('',(9.8,2.,0.399999999999999)) ;
#156524=CARTESIAN_POINT('',(9.8,2.,0.399999999999999)) ;
#156525=CARTESIAN_POINT('',(9.6,2.,0.6)) ;
#156526=CARTESIAN_POINT('Origin',(9.6,2.,0.4)) ;
#156527=CARTESIAN_POINT('',(7.8,2.,0.6)) ;
#156528=CARTESIAN_POINT('',(7.8,2.,0.6)) ;
#156529=CARTESIAN_POINT('',(7.6,2.,0.399999999999999)) ;
#156530=CARTESIAN_POINT('Origin',(7.8,2.,0.4)) ;
#156531=CARTESIAN_POINT('',(7.6,2.,-0.399999999999999)) ;
#156532=CARTESIAN_POINT('',(7.6,2.,-0.399999999999999)) ;
#156533=CARTESIAN_POINT('',(7.8,2.,-0.6)) ;
#156534=CARTESIAN_POINT('Origin',(7.8,2.,-0.4)) ;
#156535=CARTESIAN_POINT('',(9.6,2.,-0.6)) ;
#156536=CARTESIAN_POINT('',(9.6,2.,-0.6)) ;
#156537=CARTESIAN_POINT('Origin',(9.6,2.,-0.4)) ;
#156538=CARTESIAN_POINT('Origin',(2.6,4.55,-36.59)) ;
#156539=CARTESIAN_POINT('',(2.6,2.85,1.65)) ;
#156540=CARTESIAN_POINT('',(2.6,4.45,1.65)) ;
#156541=CARTESIAN_POINT('',(2.6,4.55,1.65)) ;
#156542=CARTESIAN_POINT('',(2.6,4.45,2.2)) ;
#156543=CARTESIAN_POINT('',(2.6,4.45,-36.59)) ;
#156544=CARTESIAN_POINT('',(2.6,2.85,2.2)) ;
#156545=CARTESIAN_POINT('',(2.6,2.75,2.2)) ;
#156546=CARTESIAN_POINT('',(2.6,2.85,-36.59)) ;
#156547=CARTESIAN_POINT('Origin',(-7.29372370581158E-16,3.55,0.)) ;
#156548=CARTESIAN_POINT('',(0.183301359729409,3.55,-1.51703678647597)) ;
#156549=CARTESIAN_POINT('Origin',(3.6,7.81406971160724E-17,0.)) ;
#156550=CARTESIAN_POINT('',(3.6,-2.35,1.305)) ;
#156551=CARTESIAN_POINT('',(3.6,-5.15,1.305)) ;
#156552=CARTESIAN_POINT('',(3.6,-5.25,1.305)) ;
#156553=CARTESIAN_POINT('',(3.6,-5.15,-1.305)) ;
#156554=CARTESIAN_POINT('',(3.6,-5.15,-1.405)) ;
#156555=CARTESIAN_POINT('',(3.6,-2.35,-1.305)) ;
#156556=CARTESIAN_POINT('',(3.6,-2.25,-1.305)) ;
#156557=CARTESIAN_POINT('',(3.6,-2.35,-0.903119593409422)) ;
#156558=CARTESIAN_POINT('',(3.6,-2.35,0.)) ;
#156559=CARTESIAN_POINT('',(3.6,-2.32153024911032,-0.800273234017602)) ;
#156560=CARTESIAN_POINT('Origin',(3.6,-2.15,-0.903119593409422)) ;
#156561=CARTESIAN_POINT('',(3.6,-2.32153024911032,0.800273234017602)) ;
#156562=CARTESIAN_POINT('Origin',(3.6,-3.65625,3.25260651745651E-16)) ;
#156563=CARTESIAN_POINT('',(3.6,-2.35,0.903119593409423)) ;
#156564=CARTESIAN_POINT('Origin',(3.6,-2.15,0.903119593409423)) ;
#156565=CARTESIAN_POINT('',(3.6,-2.35,0.)) ;
#156566=CARTESIAN_POINT('Origin',(-5.9,0.45,-36.59)) ;
#156567=CARTESIAN_POINT('',(-5.46221792447664,0.45,2.2)) ;
#156568=CARTESIAN_POINT('',(-5.46221792447664,0.45,-36.49)) ;
#156569=CARTESIAN_POINT('',(-5.46221792447664,0.45,-36.59)) ;
#156570=CARTESIAN_POINT('',(-5.8,0.45,-36.49)) ;
#156571=CARTESIAN_POINT('',(-5.9,0.45,-36.49)) ;
#156572=CARTESIAN_POINT('',(-5.8,0.45,2.2)) ;
#156573=CARTESIAN_POINT('',(-5.8,0.45,-36.59)) ;
#156574=CARTESIAN_POINT('',(-5.4,0.45,2.2)) ;
#156575=CARTESIAN_POINT('Origin',(-5.4,0.45,-36.59)) ;
#156576=CARTESIAN_POINT('',(-5.37250902111062,0.505815017745095,2.2)) ;
#156577=CARTESIAN_POINT('',(-3.75,3.8,2.2)) ;
#156578=CARTESIAN_POINT('',(-5.37250902111062,0.505815017745095,-36.49)) ;
#156579=CARTESIAN_POINT('',(-5.4,0.45,-36.49)) ;
#156580=CARTESIAN_POINT('',(-5.37250902111062,0.505815017745095,2.29999999999998)) ;
#156581=CARTESIAN_POINT('Origin',(-4.,3.8,-36.59)) ;
#156582=CARTESIAN_POINT('',(-4.,4.45,-36.49)) ;
#156583=CARTESIAN_POINT('',(-4.,3.9,-36.49)) ;
#156584=CARTESIAN_POINT('',(-4.,3.8,-36.49)) ;
#156585=CARTESIAN_POINT('',(-4.,3.9,2.2)) ;
#156586=CARTESIAN_POINT('',(-4.,3.9,-36.59)) ;
#156587=CARTESIAN_POINT('',(-4.,4.45,2.2)) ;
#156588=CARTESIAN_POINT('',(-4.,4.55,2.2)) ;
#156589=CARTESIAN_POINT('',(-4.,4.45,-36.59)) ;
#156590=CARTESIAN_POINT('Origin',(2.6,-6.55,-36.59)) ;
#156591=CARTESIAN_POINT('',(-5.8,-6.55,-36.49)) ;
#156592=CARTESIAN_POINT('',(2.5,-6.55,-36.49)) ;
#156593=CARTESIAN_POINT('',(2.6,-6.55,-36.49)) ;
#156594=CARTESIAN_POINT('',(2.5,-6.55,2.2)) ;
#156595=CARTESIAN_POINT('',(2.5,-6.55,-36.59)) ;
#156596=CARTESIAN_POINT('',(-5.8,-6.55,2.2)) ;
#156597=CARTESIAN_POINT('',(-5.9,-6.55,2.2)) ;
#156598=CARTESIAN_POINT('',(-5.8,-6.55,-36.59)) ;
#156599=CARTESIAN_POINT('',(-5.,-6.55,-35.39)) ;
#156600=CARTESIAN_POINT('',(-5.,-6.55,-33.19)) ;
#156601=CARTESIAN_POINT('',(-5.,-6.55,-33.29)) ;
#156602=CARTESIAN_POINT('',(-3.8,-6.55,-33.19)) ;
#156603=CARTESIAN_POINT('',(-3.9,-6.55,-33.19)) ;
#156604=CARTESIAN_POINT('',(-3.8,-6.55,-35.39)) ;
#156605=CARTESIAN_POINT('',(-3.8,-6.55,-35.29)) ;
#156606=CARTESIAN_POINT('',(-4.9,-6.55,-35.39)) ;
#156607=CARTESIAN_POINT('',(-5.,-6.55,-31.58)) ;
#156608=CARTESIAN_POINT('',(-5.,-6.55,-29.38)) ;
#156609=CARTESIAN_POINT('',(-5.,-6.55,-29.48)) ;
#156610=CARTESIAN_POINT('',(-3.8,-6.55,-29.38)) ;
#156611=CARTESIAN_POINT('',(-3.9,-6.55,-29.38)) ;
#156612=CARTESIAN_POINT('',(-3.8,-6.55,-31.58)) ;
#156613=CARTESIAN_POINT('',(-3.8,-6.55,-31.48)) ;
#156614=CARTESIAN_POINT('',(-4.9,-6.55,-31.58)) ;
#156615=CARTESIAN_POINT('',(-5.,-6.55,-27.77)) ;
#156616=CARTESIAN_POINT('',(-5.,-6.55,-25.57)) ;
#156617=CARTESIAN_POINT('',(-5.,-6.55,-25.67)) ;
#156618=CARTESIAN_POINT('',(-3.8,-6.55,-25.57)) ;
#156619=CARTESIAN_POINT('',(-3.9,-6.55,-25.57)) ;
#156620=CARTESIAN_POINT('',(-3.8,-6.55,-27.77)) ;
#156621=CARTESIAN_POINT('',(-3.8,-6.55,-27.67)) ;
#156622=CARTESIAN_POINT('',(-4.9,-6.55,-27.77)) ;
#156623=CARTESIAN_POINT('',(-5.,-6.55,-23.96)) ;
#156624=CARTESIAN_POINT('',(-5.,-6.55,-21.76)) ;
#156625=CARTESIAN_POINT('',(-5.,-6.55,-21.86)) ;
#156626=CARTESIAN_POINT('',(-3.8,-6.55,-21.76)) ;
#156627=CARTESIAN_POINT('',(-3.9,-6.55,-21.76)) ;
#156628=CARTESIAN_POINT('',(-3.8,-6.55,-23.96)) ;
#156629=CARTESIAN_POINT('',(-3.8,-6.55,-23.86)) ;
#156630=CARTESIAN_POINT('',(-4.9,-6.55,-23.96)) ;
#156631=CARTESIAN_POINT('',(-5.,-6.55,-20.15)) ;
#156632=CARTESIAN_POINT('',(-5.,-6.55,-17.95)) ;
#156633=CARTESIAN_POINT('',(-5.,-6.55,-18.05)) ;
#156634=CARTESIAN_POINT('',(-3.8,-6.55,-17.95)) ;
#156635=CARTESIAN_POINT('',(-3.9,-6.55,-17.95)) ;
#156636=CARTESIAN_POINT('',(-3.8,-6.55,-20.15)) ;
#156637=CARTESIAN_POINT('',(-3.8,-6.55,-20.05)) ;
#156638=CARTESIAN_POINT('',(-4.9,-6.55,-20.15)) ;
#156639=CARTESIAN_POINT('',(-5.,-6.55,-16.34)) ;
#156640=CARTESIAN_POINT('',(-5.,-6.55,-14.14)) ;
#156641=CARTESIAN_POINT('',(-5.,-6.55,-14.24)) ;
#156642=CARTESIAN_POINT('',(-3.8,-6.55,-14.14)) ;
#156643=CARTESIAN_POINT('',(-3.9,-6.55,-14.14)) ;
#156644=CARTESIAN_POINT('',(-3.8,-6.55,-16.34)) ;
#156645=CARTESIAN_POINT('',(-3.8,-6.55,-16.24)) ;
#156646=CARTESIAN_POINT('',(-4.9,-6.55,-16.34)) ;
#156647=CARTESIAN_POINT('',(-5.,-6.55,-12.53)) ;
#156648=CARTESIAN_POINT('',(-5.,-6.55,-10.33)) ;
#156649=CARTESIAN_POINT('',(-5.,-6.55,-10.43)) ;
#156650=CARTESIAN_POINT('',(-3.8,-6.55,-10.33)) ;
#156651=CARTESIAN_POINT('',(-3.9,-6.55,-10.33)) ;
#156652=CARTESIAN_POINT('',(-3.8,-6.55,-12.53)) ;
#156653=CARTESIAN_POINT('',(-3.8,-6.55,-12.43)) ;
#156654=CARTESIAN_POINT('',(-4.9,-6.55,-12.53)) ;
#156655=CARTESIAN_POINT('',(-5.,-6.55,-8.72)) ;
#156656=CARTESIAN_POINT('',(-5.,-6.55,-6.52)) ;
#156657=CARTESIAN_POINT('',(-5.,-6.55,-6.62)) ;
#156658=CARTESIAN_POINT('',(-3.8,-6.55,-6.52)) ;
#156659=CARTESIAN_POINT('',(-3.9,-6.55,-6.52)) ;
#156660=CARTESIAN_POINT('',(-3.8,-6.55,-8.72)) ;
#156661=CARTESIAN_POINT('',(-3.8,-6.55,-8.62)) ;
#156662=CARTESIAN_POINT('',(-4.9,-6.55,-8.72)) ;
#156663=CARTESIAN_POINT('',(-4.,-6.55,-4.91)) ;
#156664=CARTESIAN_POINT('',(-3.8,-6.55,-4.71)) ;
#156665=CARTESIAN_POINT('Origin',(-4.,-6.55,-4.71)) ;
#156666=CARTESIAN_POINT('',(-4.8,-6.55,-4.91)) ;
#156667=CARTESIAN_POINT('',(-4.9,-6.55,-4.91)) ;
#156668=CARTESIAN_POINT('',(-5.,-6.55,-4.71)) ;
#156669=CARTESIAN_POINT('Origin',(-4.8,-6.55,-4.71)) ;
#156670=CARTESIAN_POINT('',(-5.,-6.55,-2.91)) ;
#156671=CARTESIAN_POINT('',(-5.,-6.55,-2.81)) ;
#156672=CARTESIAN_POINT('',(-4.8,-6.55,-2.71)) ;
#156673=CARTESIAN_POINT('Origin',(-4.8,-6.55,-2.91)) ;
#156674=CARTESIAN_POINT('',(-4.,-6.55,-2.71)) ;
#156675=CARTESIAN_POINT('',(-3.9,-6.55,-2.71)) ;
#156676=CARTESIAN_POINT('',(-3.8,-6.55,-2.91)) ;
#156677=CARTESIAN_POINT('Origin',(-4.,-6.55,-2.91)) ;
#156678=CARTESIAN_POINT('',(-3.8,-6.55,-4.81)) ;
#156679=CARTESIAN_POINT('',(-4.,-6.55,-1.1)) ;
#156680=CARTESIAN_POINT('',(-3.8,-6.55,-0.900000000000002)) ;
#156681=CARTESIAN_POINT('Origin',(-4.,-6.55,-0.900000000000002)) ;
#156682=CARTESIAN_POINT('',(-4.8,-6.55,-1.1)) ;
#156683=CARTESIAN_POINT('',(-4.9,-6.55,-1.1)) ;
#156684=CARTESIAN_POINT('',(-5.,-6.55,-0.900000000000002)) ;
#156685=CARTESIAN_POINT('Origin',(-4.8,-6.55,-0.900000000000002)) ;
#156686=CARTESIAN_POINT('',(-5.,-6.55,0.899999999999998)) ;
#156687=CARTESIAN_POINT('',(-5.,-6.55,0.999999999999998)) ;
#156688=CARTESIAN_POINT('',(-4.8,-6.55,1.1)) ;
#156689=CARTESIAN_POINT('Origin',(-4.8,-6.55,0.899999999999998)) ;
#156690=CARTESIAN_POINT('',(-4.,-6.55,1.1)) ;
#156691=CARTESIAN_POINT('',(-3.9,-6.55,1.1)) ;
#156692=CARTESIAN_POINT('',(-3.8,-6.55,0.899999999999998)) ;
#156693=CARTESIAN_POINT('Origin',(-4.,-6.55,0.899999999999998)) ;
#156694=CARTESIAN_POINT('',(-3.8,-6.55,-1.)) ;
#156695=CARTESIAN_POINT('Origin',(0.,0.,-36.59)) ;
#156696=CARTESIAN_POINT('',(-3.9,3.9,-36.59)) ;
#156697=CARTESIAN_POINT('',(-3.9,4.45,-36.59)) ;
#156698=CARTESIAN_POINT('',(-3.9,0.,-36.59)) ;
#156699=CARTESIAN_POINT('',(2.5,4.45,-36.59)) ;
#156700=CARTESIAN_POINT('',(-5.84812080916424E-16,4.45,-36.59)) ;
#156701=CARTESIAN_POINT('',(2.5,2.85,-36.59)) ;
#156702=CARTESIAN_POINT('',(2.5,1.95351742790181E-16,-36.59)) ;
#156703=CARTESIAN_POINT('',(2.7,2.65,-36.59)) ;
#156704=CARTESIAN_POINT('Origin',(2.7,2.85,-36.59)) ;
#156705=CARTESIAN_POINT('',(3.5,2.65,-36.59)) ;
#156706=CARTESIAN_POINT('',(3.5,2.65,-36.59)) ;
#156707=CARTESIAN_POINT('',(3.5,2.1,-36.59)) ;
#156708=CARTESIAN_POINT('',(3.5,0.,-36.59)) ;
#156709=CARTESIAN_POINT('',(2.7,2.1,-36.59)) ;
#156710=CARTESIAN_POINT('',(2.7,2.1,-36.59)) ;
#156711=CARTESIAN_POINT('',(2.5,1.9,-36.59)) ;
#156712=CARTESIAN_POINT('Origin',(2.7,1.9,-36.59)) ;
#156713=CARTESIAN_POINT('',(2.5,-6.45,-36.59)) ;
#156714=CARTESIAN_POINT('',(2.5,1.95351742790181E-16,-36.59)) ;
#156715=CARTESIAN_POINT('',(-5.8,-6.45,-36.59)) ;
#156716=CARTESIAN_POINT('',(0.,-6.45,-36.59)) ;
#156717=CARTESIAN_POINT('',(-5.8,0.35,-36.59)) ;
#156718=CARTESIAN_POINT('',(-5.8,-1.4373423086665E-15,-36.59)) ;
#156719=CARTESIAN_POINT('',(-5.46221792447664,0.35,-36.59)) ;
#156720=CARTESIAN_POINT('',(0.,0.35,-36.59)) ;
#156721=CARTESIAN_POINT('',(-5.28280011774461,0.46163003549019,-36.59)) ;
#156722=CARTESIAN_POINT('Origin',(-5.46221792447664,0.55,-36.59)) ;
#156723=CARTESIAN_POINT('',(-3.58927461283679,3.9,-36.59)) ;
#156724=CARTESIAN_POINT('',(-4.43441264557625,2.18411369110472,-36.59)) ;
#156725=CARTESIAN_POINT('',(0.,3.9,-36.59)) ;
#156726=CARTESIAN_POINT('Origin',(0.,0.,2.3)) ;
#156727=CARTESIAN_POINT('',(2.5,2.85,2.3)) ;
#156728=CARTESIAN_POINT('',(2.5,4.45,2.3)) ;
#156729=CARTESIAN_POINT('',(2.5,4.55,2.3)) ;
#156730=CARTESIAN_POINT('',(-3.9,4.45,2.3)) ;
#156731=CARTESIAN_POINT('',(-3.9,4.45,2.3)) ;
#156732=CARTESIAN_POINT('',(-3.9,3.9,2.3)) ;
#156733=CARTESIAN_POINT('',(-3.9,3.8,2.3)) ;
#156734=CARTESIAN_POINT('',(-3.58927461283679,3.9,2.3)) ;
#156735=CARTESIAN_POINT('',(-3.75,3.9,2.3)) ;
#156736=CARTESIAN_POINT('',(-5.28280011774461,0.461630035490191,2.3)) ;
#156737=CARTESIAN_POINT('',(-5.31029109663398,0.405815017745095,2.3)) ;
#156738=CARTESIAN_POINT('',(-5.46221792447664,0.35,2.3)) ;
#156739=CARTESIAN_POINT('Origin',(-5.46221792447664,0.55,2.3)) ;
#156740=CARTESIAN_POINT('',(-5.8,0.35,2.3)) ;
#156741=CARTESIAN_POINT('',(-5.9,0.35,2.3)) ;
#156742=CARTESIAN_POINT('',(-5.8,-6.45,2.3)) ;
#156743=CARTESIAN_POINT('',(-5.8,-6.55,2.3)) ;
#156744=CARTESIAN_POINT('',(2.5,-6.45,2.3)) ;
#156745=CARTESIAN_POINT('',(2.6,-6.45,2.3)) ;
#156746=CARTESIAN_POINT('',(2.5,1.9,2.3)) ;
#156747=CARTESIAN_POINT('',(2.5,1.9,2.3)) ;
#156748=CARTESIAN_POINT('',(2.7,2.1,2.3)) ;
#156749=CARTESIAN_POINT('Origin',(2.7,1.9,2.3)) ;
#156750=CARTESIAN_POINT('',(3.5,2.1,2.3)) ;
#156751=CARTESIAN_POINT('',(-1.64095463943752E-16,2.1,2.3)) ;
#156752=CARTESIAN_POINT('',(3.5,2.65,2.3)) ;
#156753=CARTESIAN_POINT('',(3.5,2.65,2.3)) ;
#156754=CARTESIAN_POINT('',(2.7,2.65,2.3)) ;
#156755=CARTESIAN_POINT('',(-2.07072847357592E-16,2.65,2.3)) ;
#156756=CARTESIAN_POINT('Origin',(2.7,2.85,2.3)) ;
#156757=CARTESIAN_POINT('Origin',(-5.15,-5.05,-1.6)) ;
#156758=CARTESIAN_POINT('',(-5.8,-5.42192235935956,-1.6)) ;
#156759=CARTESIAN_POINT('',(-5.17275707706437,-5.26511162862565,-1.6)) ;
#156760=CARTESIAN_POINT('',(-5.10072415073893,-5.24710339704429,-1.6)) ;
#156761=CARTESIAN_POINT('',(-5.17275707706437,-1.91866427917293,-1.6)) ;
#156762=CARTESIAN_POINT('',(-5.17275707706437,-1.79999999999999,-1.6)) ;
#156763=CARTESIAN_POINT('',(-5.8,-1.2914213562373,-1.6)) ;
#156764=CARTESIAN_POINT('',(-3.59571067811865,-3.49571067811865,-1.6)) ;
#156765=CARTESIAN_POINT('',(-5.8,-5.55,-1.6)) ;
#156766=CARTESIAN_POINT('Origin',(-3.9,-5.05,-1.)) ;
#156767=CARTESIAN_POINT('',(-5.12948397030589,-1.91866427917293,-1.59015230574683)) ;
#156768=CARTESIAN_POINT('',(-5.12948397030589,-5.26511162862565,-1.59015230574683)) ;
#156769=CARTESIAN_POINT('',(-5.12948397030589,-5.3625,-1.59015230574683)) ;
#156770=CARTESIAN_POINT('',(-3.9,-4.95774063604919,-1.)) ;
#156771=CARTESIAN_POINT('',(-3.91783961713025,-4.96220054033175,-1.00856301622252)) ;
#156772=CARTESIAN_POINT('',(-3.9,-3.14814824947882,-1.)) ;
#156773=CARTESIAN_POINT('',(-3.9,-5.05,-1.)) ;
#156774=CARTESIAN_POINT('',(-3.04730463122257,-4.00084361825625,-0.590706222986834)) ;
#156775=CARTESIAN_POINT('Origin',(-3.9,-5.05,1.)) ;
#156776=CARTESIAN_POINT('',(-3.9,-5.05,0.900718313010847)) ;
#156777=CARTESIAN_POINT('',(-3.9,-5.05,-0.900718313010846)) ;
#156778=CARTESIAN_POINT('',(-3.9,-5.05,1.)) ;
#156779=CARTESIAN_POINT('',(-3.9,-4.95774063604919,1.)) ;
#156780=CARTESIAN_POINT('Origin',(-3.9,-4.94692235935957,0.889076603009118)) ;
#156781=CARTESIAN_POINT('',(-3.9,-3.14814824947882,1.)) ;
#156782=CARTESIAN_POINT('',(-3.9,-5.05,1.)) ;
#156783=CARTESIAN_POINT('',(-3.9,-3.05,0.923017728506055)) ;
#156784=CARTESIAN_POINT('Origin',(-3.9,-3.19142135623718,0.889076603009217)) ;
#156785=CARTESIAN_POINT('',(-3.9,-3.05,-0.923017728506055)) ;
#156786=CARTESIAN_POINT('',(-3.9,-3.05,1.)) ;
#156787=CARTESIAN_POINT('Origin',(-3.89999999999999,-3.19142135623722,-0.889076603009188)) ;
#156788=CARTESIAN_POINT('Origin',(-3.9,-4.94692235935963,-0.889076603009194)) ;
#156789=CARTESIAN_POINT('Origin',(-5.15,-5.05,1.6)) ;
#156790=CARTESIAN_POINT('',(-5.12948397030589,-5.26511162862565,1.59015230574683)) ;
#156791=CARTESIAN_POINT('',(-5.10741344341225,-5.25959399690224,1.57955845283788)) ;
#156792=CARTESIAN_POINT('',(-5.12948397030589,-1.91866427917293,1.59015230574683)) ;
#156793=CARTESIAN_POINT('',(-5.12948397030589,-1.79999999999999,1.59015230574683)) ;
#156794=CARTESIAN_POINT('',(-3.73686704155255,-3.31128120792626,0.921696179945227)) ;
#156795=CARTESIAN_POINT('Origin',(-5.9,-5.05,1.6)) ;
#156796=CARTESIAN_POINT('',(-5.17275707706436,-1.91866427917293,1.6)) ;
#156797=CARTESIAN_POINT('',(-5.17275707706436,-5.26511162862565,1.6)) ;
#156798=CARTESIAN_POINT('',(-5.17275707706436,-5.3625,1.6)) ;
#156799=CARTESIAN_POINT('',(-5.8,-5.42192235935956,1.6)) ;
#156800=CARTESIAN_POINT('',(-5.8066065036801,-5.42357398527959,1.6)) ;
#156801=CARTESIAN_POINT('',(-5.8,-1.2914213562373,1.6)) ;
#156802=CARTESIAN_POINT('',(-5.8,-1.04999999999999,1.6)) ;
#156803=CARTESIAN_POINT('',(-3.97071067811865,-3.12071067811865,1.6)) ;
#156804=CARTESIAN_POINT('Origin',(-3.89999999999997,-5.05,0.)) ;
#156805=CARTESIAN_POINT('',(-5.82425356250363,-5.53106339062591,1.5)) ;
#156806=CARTESIAN_POINT('',(-5.14850351456073,-5.36212587864019,1.5)) ;
#156807=CARTESIAN_POINT('',(-3.89999999999997,-5.05,1.5)) ;
#156808=CARTESIAN_POINT('',(-3.56560075006169,-4.96640018751543,0.74020667304046)) ;
#156809=CARTESIAN_POINT('',(-5.14850351456073,-5.36212587864019,-1.5)) ;
#156810=CARTESIAN_POINT('',(-3.56560075006169,-4.96640018751543,-0.740206673040459)) ;
#156811=CARTESIAN_POINT('',(-5.82425356250363,-5.53106339062591,-1.5)) ;
#156812=CARTESIAN_POINT('',(-3.89999999999997,-5.05,-1.5)) ;
#156813=CARTESIAN_POINT('',(-5.82425356250363,-5.53106339062591,0.)) ;
#156814=CARTESIAN_POINT('Origin',(-5.9,-1.04999999999999,-36.59)) ;
#156815=CARTESIAN_POINT('',(-5.87071067811865,-1.07928932188133,-1.5)) ;
#156816=CARTESIAN_POINT('',(-5.10204639894571,-1.84795360105428,-1.5)) ;
#156817=CARTESIAN_POINT('',(-5.9,-1.04999999999999,-1.5)) ;
#156818=CARTESIAN_POINT('',(-13.3692214357591,6.41922143575911,-5.46824401767042)) ;
#156819=CARTESIAN_POINT('',(-5.10204639894571,-1.84795360105428,1.5)) ;
#156820=CARTESIAN_POINT('',(2.37970252406874,-9.32970252406872,-2.09123948304694)) ;
#156821=CARTESIAN_POINT('',(-5.87071067811865,-1.07928932188133,1.5)) ;
#156822=CARTESIAN_POINT('',(-5.9,-1.04999999999999,1.5)) ;
#156823=CARTESIAN_POINT('',(-5.87071067811865,-1.07928932188133,-36.59)) ;
#156824=CARTESIAN_POINT('Origin',(-3.9,-6.4,0.999999999999998)) ;
#156825=CARTESIAN_POINT('',(-3.9,-6.35,0.899999999999998)) ;
#156826=CARTESIAN_POINT('',(-3.9,-6.35,-0.900000000000002)) ;
#156827=CARTESIAN_POINT('',(-3.9,-6.35,0.999999999999998)) ;
#156828=CARTESIAN_POINT('',(-3.9,-6.45,-0.900000000000002)) ;
#156829=CARTESIAN_POINT('',(-3.9,-6.55,-0.900000000000002)) ;
#156830=CARTESIAN_POINT('',(-3.9,-6.45,0.899999999999998)) ;
#156831=CARTESIAN_POINT('',(-3.9,-6.45,1.)) ;
#156832=CARTESIAN_POINT('',(-3.9,-6.25,0.899999999999998)) ;
#156833=CARTESIAN_POINT('Origin',(-4.9,-6.4,-1.)) ;
#156834=CARTESIAN_POINT('',(-4.,-6.35,-1.)) ;
#156835=CARTESIAN_POINT('',(-4.8,-6.35,-1.)) ;
#156836=CARTESIAN_POINT('',(-4.9,-6.35,-1.)) ;
#156837=CARTESIAN_POINT('',(-4.8,-6.45,-1.)) ;
#156838=CARTESIAN_POINT('',(-4.8,-6.55,-1.)) ;
#156839=CARTESIAN_POINT('',(-4.,-6.45,-1.)) ;
#156840=CARTESIAN_POINT('',(-3.9,-6.45,-1.)) ;
#156841=CARTESIAN_POINT('',(-4.,-6.25,-1.)) ;
#156842=CARTESIAN_POINT('Origin',(-4.9,-6.4,0.999999999999998)) ;
#156843=CARTESIAN_POINT('',(-4.9,-6.45,-0.900000000000002)) ;
#156844=CARTESIAN_POINT('',(-4.9,-6.35,-0.900000000000002)) ;
#156845=CARTESIAN_POINT('',(-4.9,-6.25,-0.900000000000002)) ;
#156846=CARTESIAN_POINT('',(-4.9,-6.35,0.899999999999998)) ;
#156847=CARTESIAN_POINT('',(-4.9,-6.35,0.999999999999998)) ;
#156848=CARTESIAN_POINT('',(-4.9,-6.45,0.899999999999998)) ;
#156849=CARTESIAN_POINT('',(-4.9,-6.55,0.899999999999998)) ;
#156850=CARTESIAN_POINT('',(-4.9,-6.45,-1.)) ;
#156851=CARTESIAN_POINT('Origin',(-4.9,-6.4,0.999999999999998)) ;
#156852=CARTESIAN_POINT('',(-4.8,-6.45,0.999999999999998)) ;
#156853=CARTESIAN_POINT('',(-4.8,-6.35,0.999999999999998)) ;
#156854=CARTESIAN_POINT('',(-4.8,-6.25,0.999999999999998)) ;
#156855=CARTESIAN_POINT('',(-4.,-6.35,0.999999999999998)) ;
#156856=CARTESIAN_POINT('',(-4.9,-6.35,0.999999999999998)) ;
#156857=CARTESIAN_POINT('',(-4.,-6.45,0.999999999999998)) ;
#156858=CARTESIAN_POINT('',(-4.,-6.55,0.999999999999998)) ;
#156859=CARTESIAN_POINT('',(-4.9,-6.45,0.999999999999998)) ;
#156860=CARTESIAN_POINT('Origin',(0.,-6.25,0.)) ;
#156861=CARTESIAN_POINT('',(-4.8,-6.25,0.899999999999998)) ;
#156862=CARTESIAN_POINT('',(-4.8,-6.25,-0.900000000000002)) ;
#156863=CARTESIAN_POINT('',(-4.8,-6.25,0.)) ;
#156864=CARTESIAN_POINT('',(-4.,-6.25,-0.900000000000002)) ;
#156865=CARTESIAN_POINT('',(1.95156391047391E-16,-6.25,-0.900000000000001)) ;
#156866=CARTESIAN_POINT('',(-4.,-6.25,0.899999999999998)) ;
#156867=CARTESIAN_POINT('',(-4.,-6.25,-8.67361737988403E-16)) ;
#156868=CARTESIAN_POINT('',(1.9515639104739E-16,-6.25,0.899999999999997)) ;
#156869=CARTESIAN_POINT('',(-4.65,-6.25,-0.850000000000002)) ;
#156870=CARTESIAN_POINT('',(-4.15,-6.25,-0.850000000000002)) ;
#156871=CARTESIAN_POINT('',(-4.75,-6.25,-0.850000000000002)) ;
#156872=CARTESIAN_POINT('',(-4.75,-6.25,-0.750000000000002)) ;
#156873=CARTESIAN_POINT('Origin',(-4.65,-6.25,-0.750000000000002)) ;
#156874=CARTESIAN_POINT('',(-4.75,-6.25,0.749999999999998)) ;
#156875=CARTESIAN_POINT('',(-4.75,-6.25,0.849999999999998)) ;
#156876=CARTESIAN_POINT('',(-4.65,-6.25,0.849999999999998)) ;
#156877=CARTESIAN_POINT('Origin',(-4.65,-6.25,0.749999999999998)) ;
#156878=CARTESIAN_POINT('',(-4.15,-6.25,0.849999999999998)) ;
#156879=CARTESIAN_POINT('',(-4.05,-6.25,0.849999999999998)) ;
#156880=CARTESIAN_POINT('',(-4.05,-6.25,0.749999999999998)) ;
#156881=CARTESIAN_POINT('Origin',(-4.15,-6.25,0.749999999999998)) ;
#156882=CARTESIAN_POINT('',(-4.05,-6.25,-0.750000000000002)) ;
#156883=CARTESIAN_POINT('',(-4.05,-6.25,-0.850000000000002)) ;
#156884=CARTESIAN_POINT('Origin',(-4.15,-6.25,-0.750000000000002)) ;
#156885=CARTESIAN_POINT('Origin',(-4.05,-6.25,-0.850000000000002)) ;
#156886=CARTESIAN_POINT('',(-4.05,-6.3,0.749999999999998)) ;
#156887=CARTESIAN_POINT('',(-4.05,-6.25,0.749999999999998)) ;
#156888=CARTESIAN_POINT('',(-4.05,-6.3,-0.750000000000002)) ;
#156889=CARTESIAN_POINT('',(-4.05,-6.3,-0.850000000000002)) ;
#156890=CARTESIAN_POINT('',(-4.05,-6.25,-0.750000000000002)) ;
#156891=CARTESIAN_POINT('Origin',(-4.75,-6.25,-0.850000000000002)) ;
#156892=CARTESIAN_POINT('',(-4.15,-6.3,-0.850000000000002)) ;
#156893=CARTESIAN_POINT('',(-4.15,-6.25,-0.850000000000002)) ;
#156894=CARTESIAN_POINT('',(-4.65,-6.3,-0.850000000000002)) ;
#156895=CARTESIAN_POINT('',(-4.75,-6.3,-0.850000000000002)) ;
#156896=CARTESIAN_POINT('',(-4.65,-6.25,-0.850000000000002)) ;
#156897=CARTESIAN_POINT('Origin',(-4.75,-6.25,0.849999999999998)) ;
#156898=CARTESIAN_POINT('',(-4.75,-6.3,-0.750000000000002)) ;
#156899=CARTESIAN_POINT('',(-4.75,-6.3,0.749999999999998)) ;
#156900=CARTESIAN_POINT('',(-4.75,-6.3,0.849999999999998)) ;
#156901=CARTESIAN_POINT('',(-4.75,-6.25,0.749999999999998)) ;
#156902=CARTESIAN_POINT('',(-4.75,-6.25,-0.750000000000002)) ;
#156903=CARTESIAN_POINT('Origin',(-4.05,-6.25,0.849999999999998)) ;
#156904=CARTESIAN_POINT('',(-4.65,-6.3,0.849999999999998)) ;
#156905=CARTESIAN_POINT('',(-4.65,-6.25,0.849999999999998)) ;
#156906=CARTESIAN_POINT('',(-4.15,-6.3,0.849999999999998)) ;
#156907=CARTESIAN_POINT('',(-4.05,-6.3,0.849999999999998)) ;
#156908=CARTESIAN_POINT('',(-4.15,-6.25,0.849999999999998)) ;
#156909=CARTESIAN_POINT('Origin',(0.,-6.4,0.)) ;
#156910=CARTESIAN_POINT('',(-4.15,-6.4,0.749999999999998)) ;
#156911=CARTESIAN_POINT('',(-4.65,-6.4,0.749999999999998)) ;
#156912=CARTESIAN_POINT('',(0.,-6.4,0.749999999999998)) ;
#156913=CARTESIAN_POINT('',(-4.65,-6.4,-0.750000000000002)) ;
#156914=CARTESIAN_POINT('',(-4.65,-6.4,0.)) ;
#156915=CARTESIAN_POINT('',(-4.15,-6.4,-0.750000000000002)) ;
#156916=CARTESIAN_POINT('',(0.,-6.4,-0.750000000000002)) ;
#156917=CARTESIAN_POINT('',(-4.15,-6.4,0.)) ;
#156918=CARTESIAN_POINT('Origin',(3.6,2.75,-2.3)) ;
#156919=CARTESIAN_POINT('',(2.7,2.75,-36.49)) ;
#156920=CARTESIAN_POINT('',(2.6,2.75,-36.49)) ;
#156921=CARTESIAN_POINT('',(2.7,2.75,-35.94)) ;
#156922=CARTESIAN_POINT('',(2.7,2.75,-2.3)) ;
#156923=CARTESIAN_POINT('',(2.5,2.75,-35.74)) ;
#156924=CARTESIAN_POINT('Origin',(2.5,2.75,-35.94)) ;
#156925=CARTESIAN_POINT('',(1.77490703981929,2.75,-35.74)) ;
#156926=CARTESIAN_POINT('',(2.5,2.75,1.45)) ;
#156927=CARTESIAN_POINT('',(2.6,2.75,1.45)) ;
#156928=CARTESIAN_POINT('',(2.7,2.75,1.65)) ;
#156929=CARTESIAN_POINT('Origin',(2.5,2.75,1.65)) ;
#156930=CARTESIAN_POINT('',(2.7,2.75,2.2)) ;
#156931=CARTESIAN_POINT('',(2.7,2.75,-2.3)) ;
#156932=CARTESIAN_POINT('',(3.6,2.75,2.2)) ;
#156933=CARTESIAN_POINT('Origin',(3.6,2.,2.3)) ;
#156934=CARTESIAN_POINT('',(3.5,2.,1.505)) ;
#156935=CARTESIAN_POINT('',(3.5,2.,2.2)) ;
#156936=CARTESIAN_POINT('',(3.5,2.,2.3)) ;
#156937=CARTESIAN_POINT('',(2.7,2.,2.2)) ;
#156938=CARTESIAN_POINT('',(3.6,2.,2.2)) ;
#156939=CARTESIAN_POINT('',(2.7,2.,1.505)) ;
#156940=CARTESIAN_POINT('',(2.7,2.,2.3)) ;
#156941=CARTESIAN_POINT('',(3.6,2.,1.505)) ;
#156942=CARTESIAN_POINT('Origin',(3.6,2.,1.405)) ;
#156943=CARTESIAN_POINT('',(3.7,1.9,1.405)) ;
#156944=CARTESIAN_POINT('',(3.6,1.92679491924311,1.405)) ;
#156945=CARTESIAN_POINT('Origin',(3.7,2.1,1.405)) ;
#156946=CARTESIAN_POINT('',(3.5,1.9,1.405)) ;
#156947=CARTESIAN_POINT('Origin',(3.5,2.1,1.405)) ;
#156948=CARTESIAN_POINT('',(2.7,1.9,1.405)) ;
#156949=CARTESIAN_POINT('',(2.6,1.9,1.405)) ;
#156950=CARTESIAN_POINT('',(2.7,-5.15,1.405)) ;
#156951=CARTESIAN_POINT('',(2.7,2.,1.405)) ;
#156952=CARTESIAN_POINT('',(3.5,-5.15,1.405)) ;
#156953=CARTESIAN_POINT('',(3.6,-5.15,1.405)) ;
#156954=CARTESIAN_POINT('',(3.5,-2.35,1.405)) ;
#156955=CARTESIAN_POINT('',(3.5,-2.25,1.405)) ;
#156956=CARTESIAN_POINT('',(3.7,-2.15,1.405)) ;
#156957=CARTESIAN_POINT('Origin',(3.7,-2.35,1.405)) ;
#156958=CARTESIAN_POINT('',(10.1,-2.15,1.405)) ;
#156959=CARTESIAN_POINT('',(3.6,-2.15,1.405)) ;
#156960=CARTESIAN_POINT('',(10.1,1.9,1.405)) ;
#156961=CARTESIAN_POINT('',(10.1,2.,1.405)) ;
#156962=CARTESIAN_POINT('',(3.6,1.9,1.405)) ;
#156963=CARTESIAN_POINT('Origin',(3.6,-5.25,1.405)) ;
#156964=CARTESIAN_POINT('',(3.5,-5.25,1.305)) ;
#156965=CARTESIAN_POINT('',(2.7,-5.25,1.305)) ;
#156966=CARTESIAN_POINT('',(3.6,-5.25,1.305)) ;
#156967=CARTESIAN_POINT('',(2.7,-5.25,-1.305)) ;
#156968=CARTESIAN_POINT('',(2.7,-5.25,1.405)) ;
#156969=CARTESIAN_POINT('',(3.5,-5.25,-1.305)) ;
#156970=CARTESIAN_POINT('',(3.6,-5.25,-1.305)) ;
#156971=CARTESIAN_POINT('',(3.5,-5.25,1.405)) ;
#156972=CARTESIAN_POINT('Origin',(3.6,-5.25,-1.405)) ;
#156973=CARTESIAN_POINT('',(2.7,1.9,-1.405)) ;
#156974=CARTESIAN_POINT('',(3.5,1.9,-1.405)) ;
#156975=CARTESIAN_POINT('',(3.6,1.9,-1.405)) ;
#156976=CARTESIAN_POINT('',(3.6,1.92679491924311,-1.405)) ;
#156977=CARTESIAN_POINT('Origin',(3.5,2.1,-1.405)) ;
#156978=CARTESIAN_POINT('',(3.7,1.9,-1.405)) ;
#156979=CARTESIAN_POINT('Origin',(3.7,2.1,-1.405)) ;
#156980=CARTESIAN_POINT('',(10.1,1.9,-1.405)) ;
#156981=CARTESIAN_POINT('',(3.6,1.9,-1.405)) ;
#156982=CARTESIAN_POINT('',(10.1,-2.15,-1.405)) ;
#156983=CARTESIAN_POINT('',(10.1,-2.25,-1.405)) ;
#156984=CARTESIAN_POINT('',(3.7,-2.15,-1.405)) ;
#156985=CARTESIAN_POINT('',(3.6,-2.15,-1.405)) ;
#156986=CARTESIAN_POINT('',(3.5,-2.35,-1.405)) ;
#156987=CARTESIAN_POINT('Origin',(3.7,-2.35,-1.405)) ;
#156988=CARTESIAN_POINT('',(3.5,-5.15,-1.405)) ;
#156989=CARTESIAN_POINT('',(3.5,-5.25,-1.405)) ;
#156990=CARTESIAN_POINT('',(2.7,-5.15,-1.405)) ;
#156991=CARTESIAN_POINT('',(3.6,-5.15,-1.405)) ;
#156992=CARTESIAN_POINT('',(2.7,-5.25,-1.405)) ;
#156993=CARTESIAN_POINT('Origin',(3.6,2.,-1.405)) ;
#156994=CARTESIAN_POINT('',(2.7,2.,-2.305)) ;
#156995=CARTESIAN_POINT('',(3.6,2.,-2.305)) ;
#156996=CARTESIAN_POINT('',(2.7,2.,-1.505)) ;
#156997=CARTESIAN_POINT('',(2.6,2.,-1.505)) ;
#156998=CARTESIAN_POINT('',(2.7,2.,-1.405)) ;
#156999=CARTESIAN_POINT('Origin',(10.2,-2.25,-0.875)) ;
#157000=CARTESIAN_POINT('',(10.1,-2.25,-0.903119593409422)) ;
#157001=CARTESIAN_POINT('',(3.7,-2.25,-0.903119593409422)) ;
#157002=CARTESIAN_POINT('',(10.2,-2.25,-0.903119593409422)) ;
#157003=CARTESIAN_POINT('',(3.7,-2.25,-1.305)) ;
#157004=CARTESIAN_POINT('',(3.7,-2.25,-0.875)) ;
#157005=CARTESIAN_POINT('',(10.1,-2.25,-1.305)) ;
#157006=CARTESIAN_POINT('',(10.2,-2.25,-1.305)) ;
#157007=CARTESIAN_POINT('',(10.1,-2.25,-0.875)) ;
#157008=CARTESIAN_POINT('Origin',(10.2,-2.25,1.405)) ;
#157009=CARTESIAN_POINT('',(10.1,-2.25,1.305)) ;
#157010=CARTESIAN_POINT('',(3.7,-2.25,1.305)) ;
#157011=CARTESIAN_POINT('',(10.2,-2.25,1.305)) ;
#157012=CARTESIAN_POINT('',(3.7,-2.25,0.903119593409423)) ;
#157013=CARTESIAN_POINT('',(3.7,-2.25,1.405)) ;
#157014=CARTESIAN_POINT('',(10.1,-2.25,0.903119593409423)) ;
#157015=CARTESIAN_POINT('',(10.2,-2.25,0.903119593409423)) ;
#157016=CARTESIAN_POINT('',(10.1,-2.25,1.405)) ;
#157017=CARTESIAN_POINT('Origin',(10.2,-3.65625,3.25260651745651E-16)) ;
#157018=CARTESIAN_POINT('',(10.1,-2.23576512455516,0.851696413713513)) ;
#157019=CARTESIAN_POINT('',(3.7,-2.23576512455516,0.851696413713513)) ;
#157020=CARTESIAN_POINT('',(10.2,-2.23576512455516,0.851696413713513)) ;
#157021=CARTESIAN_POINT('',(3.7,-2.23576512455516,-0.851696413713512)) ;
#157022=CARTESIAN_POINT('Origin',(3.7,-3.65625,3.25260651745651E-16)) ;
#157023=CARTESIAN_POINT('',(10.1,-2.23576512455516,-0.851696413713512)) ;
#157024=CARTESIAN_POINT('',(10.2,-2.23576512455516,-0.851696413713512)) ;
#157025=CARTESIAN_POINT('Origin',(10.1,-3.65625,3.25260651745651E-16)) ;
#157026=CARTESIAN_POINT('Origin',(10.2,-3.65625,3.25260651745651E-16)) ;
#157027=CARTESIAN_POINT('',(10.2,-2.15,1.305)) ;
#157028=CARTESIAN_POINT('',(10.2,-2.15,0.903119593409424)) ;
#157029=CARTESIAN_POINT('',(10.2,-2.15,0.875)) ;
#157030=CARTESIAN_POINT('',(10.2,-2.15,-0.903119593409424)) ;
#157031=CARTESIAN_POINT('Origin',(10.2,-3.65625,3.25260651745651E-16)) ;
#157032=CARTESIAN_POINT('',(10.2,-2.15,-1.305)) ;
#157033=CARTESIAN_POINT('',(10.2,-2.15,-1.405)) ;
#157034=CARTESIAN_POINT('',(10.2,1.9,-1.305)) ;
#157035=CARTESIAN_POINT('',(10.2,2.,-1.305)) ;
#157036=CARTESIAN_POINT('',(10.2,1.9,1.305)) ;
#157037=CARTESIAN_POINT('',(10.2,1.9,1.405)) ;
#157038=CARTESIAN_POINT('',(10.2,-2.25,1.305)) ;
#157039=CARTESIAN_POINT('Origin',(8.7,0.,0.)) ;
#157040=CARTESIAN_POINT('Origin',(-2.,4.4,-1.)) ;
#157041=CARTESIAN_POINT('',(-2.,4.35,-0.9)) ;
#157042=CARTESIAN_POINT('',(-2.,4.35,0.900000000000001)) ;
#157043=CARTESIAN_POINT('',(-2.,4.35,-1.)) ;
#157044=CARTESIAN_POINT('',(-2.,4.45,0.900000000000001)) ;
#157045=CARTESIAN_POINT('',(-2.,4.55,0.900000000000001)) ;
#157046=CARTESIAN_POINT('',(-2.,4.45,-0.9)) ;
#157047=CARTESIAN_POINT('',(-2.,4.45,-1.)) ;
#157048=CARTESIAN_POINT('',(-2.,4.25,-0.9)) ;
#157049=CARTESIAN_POINT('Origin',(-3.,4.4,1.)) ;
#157050=CARTESIAN_POINT('',(-2.9,4.45,1.)) ;
#157051=CARTESIAN_POINT('',(-2.1,4.45,1.)) ;
#157052=CARTESIAN_POINT('',(-2.,4.45,1.)) ;
#157053=CARTESIAN_POINT('',(-2.1,4.35,1.)) ;
#157054=CARTESIAN_POINT('',(-2.1,4.25,1.)) ;
#157055=CARTESIAN_POINT('',(-2.9,4.35,1.)) ;
#157056=CARTESIAN_POINT('',(-3.,4.35,1.)) ;
#157057=CARTESIAN_POINT('',(-2.9,4.55,1.)) ;
#157058=CARTESIAN_POINT('Origin',(-3.,4.4,-0.999999999999999)) ;
#157059=CARTESIAN_POINT('',(-3.,4.45,0.900000000000001)) ;
#157060=CARTESIAN_POINT('',(-3.,4.35,0.900000000000001)) ;
#157061=CARTESIAN_POINT('',(-3.,4.25,0.900000000000001)) ;
#157062=CARTESIAN_POINT('',(-3.,4.35,-0.899999999999999)) ;
#157063=CARTESIAN_POINT('',(-3.,4.35,-0.999999999999999)) ;
#157064=CARTESIAN_POINT('',(-3.,4.45,-0.899999999999999)) ;
#157065=CARTESIAN_POINT('',(-3.,4.55,-0.899999999999999)) ;
#157066=CARTESIAN_POINT('',(-3.,4.45,1.)) ;
#157067=CARTESIAN_POINT('Origin',(-3.,4.4,-0.999999999999999)) ;
#157068=CARTESIAN_POINT('',(-2.9,4.35,-0.999999999999999)) ;
#157069=CARTESIAN_POINT('',(-2.1,4.35,-1.)) ;
#157070=CARTESIAN_POINT('',(-3.,4.35,-0.999999999999999)) ;
#157071=CARTESIAN_POINT('',(-2.1,4.45,-1.)) ;
#157072=CARTESIAN_POINT('',(-2.1,4.55,-1.)) ;
#157073=CARTESIAN_POINT('',(-2.9,4.45,-0.999999999999999)) ;
#157074=CARTESIAN_POINT('',(-3.,4.45,-0.999999999999999)) ;
#157075=CARTESIAN_POINT('',(-2.9,4.25,-0.999999999999999)) ;
#157076=CARTESIAN_POINT('Origin',(0.,4.25,0.)) ;
#157077=CARTESIAN_POINT('',(-2.9,4.25,-0.899999999999999)) ;
#157078=CARTESIAN_POINT('',(-2.9,4.25,0.900000000000001)) ;
#157079=CARTESIAN_POINT('',(-2.9,4.25,1.25767452008319E-15)) ;
#157080=CARTESIAN_POINT('',(-2.1,4.25,0.900000000000001)) ;
#157081=CARTESIAN_POINT('',(-1.95156391047391E-16,4.25,0.900000000000001)) ;
#157082=CARTESIAN_POINT('',(-2.1,4.25,-0.9)) ;
#157083=CARTESIAN_POINT('',(-2.1,4.25,4.55364912443912E-16)) ;
#157084=CARTESIAN_POINT('',(-1.95156391047391E-16,4.25,-0.9)) ;
#157085=CARTESIAN_POINT('',(-2.75,4.25,0.850000000000001)) ;
#157086=CARTESIAN_POINT('',(-2.25,4.25,0.850000000000001)) ;
#157087=CARTESIAN_POINT('',(-2.85,4.25,0.850000000000001)) ;
#157088=CARTESIAN_POINT('',(-2.85,4.25,0.750000000000001)) ;
#157089=CARTESIAN_POINT('Origin',(-2.75,4.25,0.750000000000001)) ;
#157090=CARTESIAN_POINT('',(-2.85,4.25,-0.75)) ;
#157091=CARTESIAN_POINT('',(-2.85,4.25,-0.85)) ;
#157092=CARTESIAN_POINT('',(-2.75,4.25,-0.85)) ;
#157093=CARTESIAN_POINT('Origin',(-2.75,4.25,-0.75)) ;
#157094=CARTESIAN_POINT('',(-2.25,4.25,-0.85)) ;
#157095=CARTESIAN_POINT('',(-2.15,4.25,-0.85)) ;
#157096=CARTESIAN_POINT('',(-2.15,4.25,-0.75)) ;
#157097=CARTESIAN_POINT('Origin',(-2.25,4.25,-0.75)) ;
#157098=CARTESIAN_POINT('',(-2.15,4.25,0.750000000000001)) ;
#157099=CARTESIAN_POINT('',(-2.15,4.25,0.850000000000001)) ;
#157100=CARTESIAN_POINT('Origin',(-2.25,4.25,0.750000000000001)) ;
#157101=CARTESIAN_POINT('Origin',(-2.15,4.25,0.850000000000001)) ;
#157102=CARTESIAN_POINT('',(-2.15,4.3,-0.75)) ;
#157103=CARTESIAN_POINT('',(-2.15,4.3,0.750000000000001)) ;
#157104=CARTESIAN_POINT('',(-2.15,4.3,0.850000000000001)) ;
#157105=CARTESIAN_POINT('',(-2.15,4.25,0.750000000000001)) ;
#157106=CARTESIAN_POINT('',(-2.15,4.25,-0.75)) ;
#157107=CARTESIAN_POINT('Origin',(-2.85,4.25,0.850000000000001)) ;
#157108=CARTESIAN_POINT('',(-2.25,4.3,0.850000000000001)) ;
#157109=CARTESIAN_POINT('',(-2.75,4.3,0.850000000000001)) ;
#157110=CARTESIAN_POINT('',(-2.85,4.3,0.850000000000001)) ;
#157111=CARTESIAN_POINT('',(-2.75,4.25,0.850000000000001)) ;
#157112=CARTESIAN_POINT('',(-2.25,4.25,0.850000000000001)) ;
#157113=CARTESIAN_POINT('Origin',(-2.85,4.25,-0.85)) ;
#157114=CARTESIAN_POINT('',(-2.85,4.3,0.750000000000001)) ;
#157115=CARTESIAN_POINT('',(-2.85,4.25,0.750000000000001)) ;
#157116=CARTESIAN_POINT('',(-2.85,4.3,-0.75)) ;
#157117=CARTESIAN_POINT('',(-2.85,4.3,-0.85)) ;
#157118=CARTESIAN_POINT('',(-2.85,4.25,-0.75)) ;
#157119=CARTESIAN_POINT('Origin',(-2.15,4.25,-0.85)) ;
#157120=CARTESIAN_POINT('',(-2.75,4.3,-0.85)) ;
#157121=CARTESIAN_POINT('',(-2.25,4.3,-0.85)) ;
#157122=CARTESIAN_POINT('',(-2.15,4.3,-0.85)) ;
#157123=CARTESIAN_POINT('',(-2.25,4.25,-0.85)) ;
#157124=CARTESIAN_POINT('',(-2.75,4.25,-0.85)) ;
#157125=CARTESIAN_POINT('Origin',(-1.97127667724637E-17,4.4,0.)) ;
#157126=CARTESIAN_POINT('',(-2.25,4.4,-0.75)) ;
#157127=CARTESIAN_POINT('',(-2.75,4.4,-0.75)) ;
#157128=CARTESIAN_POINT('',(-1.97127667724637E-17,4.4,-0.75)) ;
#157129=CARTESIAN_POINT('',(-2.75,4.4,0.750000000000001)) ;
#157130=CARTESIAN_POINT('',(-2.75,4.4,0.)) ;
#157131=CARTESIAN_POINT('',(-2.25,4.4,0.750000000000001)) ;
#157132=CARTESIAN_POINT('',(-1.97127667724637E-17,4.4,0.750000000000001)) ;
#157133=CARTESIAN_POINT('',(-2.25,4.4,0.)) ;
#157134=CARTESIAN_POINT('Origin',(-7.29372370581158E-16,3.55,0.)) ;
#157135=CARTESIAN_POINT('',(-0.183301359729408,3.55,1.51703678647597)) ;
#157136=CARTESIAN_POINT('Origin',(-0.273932138433073,3.05,1.4747749603019)) ;
#157137=CARTESIAN_POINT('',(0.953662978710562,3.45,-1.15781126399638)) ;
#157138=CARTESIAN_POINT('',(-0.273932138433073,3.15,1.4747749603019)) ;
#157139=CARTESIAN_POINT('Origin',(-0.953662978710561,3.05,1.15781126399638)) ;
#157140=CARTESIAN_POINT('',(-0.953662978710561,3.15,1.15781126399638)) ;
#157141=CARTESIAN_POINT('',(-0.953662978710562,3.45,1.15781126399638)) ;
#157142=CARTESIAN_POINT('Origin',(-7.95081593156037E-16,3.05,0.)) ;
#157143=CARTESIAN_POINT('',(0.249234641435079,3.05,0.116220021978692)) ;
#157144=CARTESIAN_POINT('',(-0.249234641435079,3.05,-0.116220021978691)) ;
#157145=CARTESIAN_POINT('Origin',(-1.39554230456301E-15,-1.51907484122731,
-3.81)) ;
#157146=CARTESIAN_POINT('Origin',(-6.11095769946375E-16,4.45,-3.81)) ;
#157147=CARTESIAN_POINT('Origin',(-1.39554230456301E-15,-1.51907484122731,
0.)) ;
#157148=CARTESIAN_POINT('Origin',(-6.11095769946375E-16,4.45,0.)) ;
#157149=CARTESIAN_POINT('Origin',(2.6,-1.51907484122731,1.55)) ;
#157150=CARTESIAN_POINT('',(2.5,4.45,1.55)) ;
#157151=CARTESIAN_POINT('',(2.6,4.45,1.55)) ;
#157152=CARTESIAN_POINT('',(2.5,2.85,1.55)) ;
#157153=CARTESIAN_POINT('',(2.5,2.75,1.55)) ;
#157154=CARTESIAN_POINT('',(1.77490703981927,2.85,1.55)) ;
#157155=CARTESIAN_POINT('Origin',(2.6,-1.51907484122731,-35.84)) ;
#157156=CARTESIAN_POINT('',(2.5,2.85,-35.84)) ;
#157157=CARTESIAN_POINT('',(2.5,4.45,-35.84)) ;
#157158=CARTESIAN_POINT('',(2.5,4.55,-35.84)) ;
#157159=CARTESIAN_POINT('',(1.77490703981929,4.45,-35.84)) ;
#157160=CARTESIAN_POINT('',(2.6,2.85,-35.84)) ;
#157161=CARTESIAN_POINT('Origin',(1.99634453700209E-16,-1.51907484122731,
-34.29)) ;
#157162=CARTESIAN_POINT('Origin',(-5.84812080916424E-16,4.45,-34.29)) ;
#157163=CARTESIAN_POINT('Origin',(1.99634453700209E-16,-1.51907484122731,
-30.48)) ;
#157164=CARTESIAN_POINT('Origin',(-5.84812080916424E-16,4.45,-30.48)) ;
#157165=CARTESIAN_POINT('Origin',(9.6,3.,-0.4)) ;
#157166=CARTESIAN_POINT('',(9.7,2.9,-0.399999999999999)) ;
#157167=CARTESIAN_POINT('',(9.7,2.1,-0.399999999999999)) ;
#157168=CARTESIAN_POINT('',(9.7,3.,-0.399999999999999)) ;
#157169=CARTESIAN_POINT('',(9.6,2.1,-0.5)) ;
#157170=CARTESIAN_POINT('Origin',(9.6,2.1,-0.4)) ;
#157171=CARTESIAN_POINT('',(9.6,2.9,-0.5)) ;
#157172=CARTESIAN_POINT('',(9.6,3.,-0.5)) ;
#157173=CARTESIAN_POINT('Origin',(9.6,2.9,-0.4)) ;
#157174=CARTESIAN_POINT('Origin',(7.8,3.,-0.5)) ;
#157175=CARTESIAN_POINT('',(7.8,2.1,-0.5)) ;
#157176=CARTESIAN_POINT('',(7.8,2.1,-0.5)) ;
#157177=CARTESIAN_POINT('',(7.8,2.9,-0.5)) ;
#157178=CARTESIAN_POINT('',(7.8,3.,-0.5)) ;
#157179=CARTESIAN_POINT('',(7.8,2.9,-0.5)) ;
#157180=CARTESIAN_POINT('Origin',(7.8,3.,-0.4)) ;
#157181=CARTESIAN_POINT('',(7.7,2.1,-0.399999999999999)) ;
#157182=CARTESIAN_POINT('Origin',(7.8,2.1,-0.4)) ;
#157183=CARTESIAN_POINT('',(7.7,2.9,-0.399999999999999)) ;
#157184=CARTESIAN_POINT('',(7.7,3.,-0.399999999999999)) ;
#157185=CARTESIAN_POINT('Origin',(7.8,2.9,-0.4)) ;
#157186=CARTESIAN_POINT('Origin',(7.7,3.,-0.399999999999999)) ;
#157187=CARTESIAN_POINT('',(7.7,2.1,0.399999999999999)) ;
#157188=CARTESIAN_POINT('',(7.7,2.1,0.399999999999999)) ;
#157189=CARTESIAN_POINT('',(7.7,2.9,0.399999999999999)) ;
#157190=CARTESIAN_POINT('',(7.7,3.,0.399999999999999)) ;
#157191=CARTESIAN_POINT('',(7.7,2.9,-0.399999999999999)) ;
#157192=CARTESIAN_POINT('Origin',(7.8,3.,0.4)) ;
#157193=CARTESIAN_POINT('',(7.8,2.1,0.5)) ;
#157194=CARTESIAN_POINT('Origin',(7.8,2.1,0.4)) ;
#157195=CARTESIAN_POINT('',(7.8,2.9,0.5)) ;
#157196=CARTESIAN_POINT('',(7.8,3.,0.5)) ;
#157197=CARTESIAN_POINT('Origin',(7.8,2.9,0.4)) ;
#157198=CARTESIAN_POINT('Origin',(7.8,3.,0.5)) ;
#157199=CARTESIAN_POINT('',(9.6,2.1,0.5)) ;
#157200=CARTESIAN_POINT('',(9.6,2.1,0.5)) ;
#157201=CARTESIAN_POINT('',(9.6,2.9,0.5)) ;
#157202=CARTESIAN_POINT('',(9.6,3.,0.5)) ;
#157203=CARTESIAN_POINT('',(7.8,2.9,0.5)) ;
#157204=CARTESIAN_POINT('Origin',(9.6,3.,0.4)) ;
#157205=CARTESIAN_POINT('',(9.7,2.1,0.399999999999999)) ;
#157206=CARTESIAN_POINT('Origin',(9.6,2.1,0.4)) ;
#157207=CARTESIAN_POINT('',(9.7,2.9,0.399999999999999)) ;
#157208=CARTESIAN_POINT('',(9.7,3.,0.399999999999999)) ;
#157209=CARTESIAN_POINT('Origin',(9.6,2.9,0.4)) ;
#157210=CARTESIAN_POINT('Origin',(9.7,3.,-0.399999999999999)) ;
#157211=CARTESIAN_POINT('',(9.7,2.9,-0.399999999999999)) ;
#157212=CARTESIAN_POINT('',(9.7,2.1,-0.399999999999999)) ;
#157213=CARTESIAN_POINT('Origin',(9.6,3.,-0.4)) ;
#157214=CARTESIAN_POINT('',(7.8,3.,0.4)) ;
#157215=CARTESIAN_POINT('',(9.6,3.,0.4)) ;
#157216=CARTESIAN_POINT('',(9.6,3.,0.4)) ;
#157217=CARTESIAN_POINT('',(9.6,3.,-0.4)) ;
#157218=CARTESIAN_POINT('',(9.6,3.,-0.4)) ;
#157219=CARTESIAN_POINT('',(7.8,3.,-0.4)) ;
#157220=CARTESIAN_POINT('',(9.6,3.,-0.4)) ;
#157221=CARTESIAN_POINT('',(7.8,3.,-0.4)) ;
#157222=CARTESIAN_POINT('Origin',(0.,-6.45,2.2)) ;
#157223=CARTESIAN_POINT('Origin',(2.5,-6.45,2.2)) ;
#157224=CARTESIAN_POINT('Origin',(-5.8,-6.45,2.2)) ;
#157225=CARTESIAN_POINT('Origin',(-5.8,-6.45,2.2)) ;
#157226=CARTESIAN_POINT('Origin',(-5.8,-6.45,2.2)) ;
#157227=CARTESIAN_POINT('Origin',(-5.8,-6.45,2.2)) ;
#157228=CARTESIAN_POINT('Origin',(2.5,-6.45,-36.59)) ;
#157229=CARTESIAN_POINT('Origin',(2.5,-6.45,-36.49)) ;
#157230=CARTESIAN_POINT('Origin',(2.5,-6.45,2.2)) ;
#157231=CARTESIAN_POINT('Origin',(-5.8,-1.4373423086665E-15,2.2)) ;
#157232=CARTESIAN_POINT('Origin',(-5.8,0.35,2.2)) ;
#157233=CARTESIAN_POINT('Origin',(-5.8,-6.45,-36.59)) ;
#157234=CARTESIAN_POINT('Origin',(-5.8,-6.45,-36.49)) ;
#157235=CARTESIAN_POINT('Origin',(2.6,-6.45,-36.49)) ;
#157236=CARTESIAN_POINT('Origin',(2.5,-6.45,-36.49)) ;
#157237=CARTESIAN_POINT('Origin',(-5.8,-6.45,-36.49)) ;
#157238=CARTESIAN_POINT('Origin',(-3.9,0.,2.2)) ;
#157239=CARTESIAN_POINT('Origin',(-3.9,4.45,2.2)) ;
#157240=CARTESIAN_POINT('Origin',(-3.9,3.9,2.2)) ;
#157241=CARTESIAN_POINT('Origin',(0.,3.9,2.2)) ;
#157242=CARTESIAN_POINT('',(-3.9,3.80333655664151,2.22561598559651)) ;
#157243=CARTESIAN_POINT('Origin',(-3.9,3.9,2.2)) ;
#157244=CARTESIAN_POINT('',(-3.78531217125694,3.83901474997814,2.27925149386461)) ;
#157245=CARTESIAN_POINT('Origin',(-3.55328808497345,3.91119503536387,2.19250366916966)) ;
#157246=CARTESIAN_POINT('Origin',(-3.61336525333204,3.89250565174523,2.22200921288124)) ;
#157247=CARTESIAN_POINT('Origin',(-5.8,0.35,2.2)) ;
#157248=CARTESIAN_POINT('Origin',(-5.8,0.35,2.2)) ;
#157249=CARTESIAN_POINT('Origin',(-5.8,0.35,2.2)) ;
#157250=CARTESIAN_POINT('Origin',(-5.8,-6.45,-36.49)) ;
#157251=CARTESIAN_POINT('Origin',(-5.8,-6.45,-36.49)) ;
#157252=CARTESIAN_POINT('Origin',(-3.9,4.45,-36.59)) ;
#157253=CARTESIAN_POINT('Origin',(-3.9,4.45,2.2)) ;
#157254=CARTESIAN_POINT('Origin',(-3.9,4.45,-36.49)) ;
#157255=CARTESIAN_POINT('Origin',(-3.9,3.9,2.2)) ;
#157256=CARTESIAN_POINT('Origin',(-3.9,3.9,2.2)) ;
#157257=CARTESIAN_POINT('Origin',(-3.85599010415589,3.83075002080759,2.20432033664006)) ;
#157258=CARTESIAN_POINT('Origin',(-4.43441264557625,2.18411369110472,2.2)) ;
#157259=CARTESIAN_POINT('',(-3.73060297224731,3.75108317805602,2.27925149386461)) ;
#157260=CARTESIAN_POINT('Origin',(-3.59033063456527,3.89854842868432,2.20056508349004)) ;
#157261=CARTESIAN_POINT('',(-3.81328428501115,3.6639623879874,2.22561598559544)) ;
#157262=CARTESIAN_POINT('Origin',(-3.57343778044602,3.91668601355327,2.19535546435355)) ;
#157263=CARTESIAN_POINT('Origin',(-3.74596198594684,3.73501205571306,2.20243127556096)) ;
#157264=CARTESIAN_POINT('Origin',(-5.28280011774461,0.461630035490191,2.2)) ;
#157265=CARTESIAN_POINT('Origin',(0.,0.35,2.2)) ;
#157266=CARTESIAN_POINT('Origin',(-5.46221792447664,0.35,2.2)) ;
#157267=CARTESIAN_POINT('Origin',(-5.8,0.35,-36.59)) ;
#157268=CARTESIAN_POINT('Origin',(-5.8,0.35,-36.49)) ;
#157269=CARTESIAN_POINT('Origin',(-5.8,-6.55,-36.49)) ;
#157270=CARTESIAN_POINT('Origin',(-5.8,0.35,-36.49)) ;
#157271=CARTESIAN_POINT('Origin',(-3.9,3.8,-36.49)) ;
#157272=CARTESIAN_POINT('Origin',(-3.9,4.45,-36.49)) ;
#157273=CARTESIAN_POINT('Origin',(-3.9,3.9,-36.49)) ;
#157274=CARTESIAN_POINT('Origin',(-3.9,3.9,-36.59)) ;
#157275=CARTESIAN_POINT('Origin',(-3.9,3.9,-36.49)) ;
#157276=CARTESIAN_POINT('Origin',(-5.46221792447664,0.55,2.2)) ;
#157277=CARTESIAN_POINT('Origin',(-5.46221792447664,0.55,2.19999999999999)) ;
#157278=CARTESIAN_POINT('Origin',(-5.8,0.35,-36.49)) ;
#157279=CARTESIAN_POINT('Origin',(-5.8,0.35,-36.49)) ;
#157280=CARTESIAN_POINT('Origin',(-3.9,3.9,-36.49)) ;
#157281=CARTESIAN_POINT('',(-3.9,3.8033365566425,-36.5156159856002)) ;
#157282=CARTESIAN_POINT('Origin',(-3.9,3.9,-36.49)) ;
#157283=CARTESIAN_POINT('Origin',(-3.85250686906682,3.83291544204029,-36.4938003888854)) ;
#157284=CARTESIAN_POINT('Origin',(-5.46221792447664,0.55,-36.59)) ;
#157285=CARTESIAN_POINT('Origin',(-5.46221792447664,0.55,-36.49)) ;
#157286=CARTESIAN_POINT('Origin',(-5.9,0.35,-36.49)) ;
#157287=CARTESIAN_POINT('Origin',(-5.46221792447664,0.35,-36.49)) ;
#157288=CARTESIAN_POINT('Origin',(-3.75,3.9,-36.49)) ;
#157289=CARTESIAN_POINT('',(-3.7853121712506,3.83901474998012,-36.5692514938661)) ;
#157290=CARTESIAN_POINT('Origin',(-3.59104340457654,3.89969403101197,-36.4905650835037)) ;
#157291=CARTESIAN_POINT('Origin',(-3.56730827154468,3.90683433651809,-36.4853554643623)) ;
#157292=CARTESIAN_POINT('Origin',(-5.46221792447664,0.55,-36.49)) ;
#157293=CARTESIAN_POINT('Origin',(-5.28280011774461,0.46163003549019,-36.49)) ;
#157294=CARTESIAN_POINT('Origin',(-5.31029109663398,0.405815017745095,-36.49)) ;
#157295=CARTESIAN_POINT('',(-3.8132842850082,3.66396238799052,-36.5156159856002)) ;
#157296=CARTESIAN_POINT('Origin',(-3.77273229582307,3.7066162135026,-36.4964228703932)) ;
#157297=CARTESIAN_POINT('',(-3.73060297224274,3.75108317806084,-36.5692514938661)) ;
#157298=CARTESIAN_POINT('Origin',(-3.57344958540767,3.91667389310731,-36.4853617599003)) ;
#157299=CARTESIAN_POINT('Origin',(-3.59031431317769,3.89856609733425,-36.4905391368281)) ;
#157300=CARTESIAN_POINT('Origin',(10.1,-2.15,-0.903119593409422)) ;
#157301=CARTESIAN_POINT('Origin',(10.1,-2.15,-0.903119593409422)) ;
#157302=CARTESIAN_POINT('Origin',(10.1,-2.15,-0.903119593409424)) ;
#157303=CARTESIAN_POINT('Origin',(10.1,-2.15,-0.903119593409422)) ;
#157304=CARTESIAN_POINT('Origin',(10.1,-3.65625,3.25260651745651E-16)) ;
#157305=CARTESIAN_POINT('Origin',(10.1,-2.15,0.903119593409423)) ;
#157306=CARTESIAN_POINT('Origin',(10.2,-2.15,-0.903119593409422)) ;
#157307=CARTESIAN_POINT('Origin',(3.7,-2.15,-0.903119593409422)) ;
#157308=CARTESIAN_POINT('Origin',(10.1,-2.15,3.25260651745651E-16)) ;
#157309=CARTESIAN_POINT('Origin',(10.1,-2.15,-1.305)) ;
#157310=CARTESIAN_POINT('Origin',(10.1,-3.65625,-1.305)) ;
#157311=CARTESIAN_POINT('Origin',(10.1,1.9,-1.305)) ;
#157312=CARTESIAN_POINT('Origin',(10.1,-2.15,-1.305)) ;
#157313=CARTESIAN_POINT('Origin',(10.1,1.9,3.25260651745651E-16)) ;
#157314=CARTESIAN_POINT('Origin',(10.1,1.9,-1.305)) ;
#157315=CARTESIAN_POINT('Origin',(10.1,1.9,1.305)) ;
#157316=CARTESIAN_POINT('Origin',(10.1,-2.15,0.903119593409423)) ;
#157317=CARTESIAN_POINT('Origin',(10.1,-2.15,0.903119593409423)) ;
#157318=CARTESIAN_POINT('Origin',(10.1,-2.15,0.903119593409424)) ;
#157319=CARTESIAN_POINT('Origin',(3.7,-2.15,-0.903119593409422)) ;
#157320=CARTESIAN_POINT('Origin',(3.7,-2.35,-0.903119593409422)) ;
#157321=CARTESIAN_POINT('Origin',(3.7,-2.32153024911032,-0.800273234017602)) ;
#157322=CARTESIAN_POINT('Origin',(10.1,-2.15,-1.305)) ;
#157323=CARTESIAN_POINT('Origin',(10.1,-2.15,-1.305)) ;
#157324=CARTESIAN_POINT('Origin',(10.1,-3.65625,1.305)) ;
#157325=CARTESIAN_POINT('Origin',(10.1,1.9,1.305)) ;
#157326=CARTESIAN_POINT('Origin',(10.1,-2.15,1.305)) ;
#157327=CARTESIAN_POINT('Origin',(10.1,-2.15,3.25260651745651E-16)) ;
#157328=CARTESIAN_POINT('Origin',(10.1,-2.15,1.305)) ;
#157329=CARTESIAN_POINT('Origin',(10.2,-2.15,0.903119593409423)) ;
#157330=CARTESIAN_POINT('Origin',(3.7,-2.15,0.903119593409423)) ;
#157331=CARTESIAN_POINT('Origin',(3.7,-3.65625,3.25260651745651E-16)) ;
#157332=CARTESIAN_POINT('Origin',(3.7,-2.32153024911032,0.800273234017602)) ;
#157333=CARTESIAN_POINT('Origin',(3.7,-2.35,-0.875)) ;
#157334=CARTESIAN_POINT('Origin',(3.7,-2.35,-1.305)) ;
#157335=CARTESIAN_POINT('Origin',(3.6,-2.15,-1.305)) ;
#157336=CARTESIAN_POINT('Origin',(3.7,-2.15,-1.305)) ;
#157337=CARTESIAN_POINT('Origin',(10.1,-2.15,1.305)) ;
#157338=CARTESIAN_POINT('Origin',(10.1,-2.15,1.305)) ;
#157339=CARTESIAN_POINT('Origin',(3.7,-2.15,0.903119593409423)) ;
#157340=CARTESIAN_POINT('Origin',(3.7,-2.35,0.903119593409423)) ;
#157341=CARTESIAN_POINT('Origin',(3.7,-2.35,-1.305)) ;
#157342=CARTESIAN_POINT('Origin',(3.5,-2.35,-1.305)) ;
#157343=CARTESIAN_POINT('Origin',(10.2,-2.15,1.305)) ;
#157344=CARTESIAN_POINT('Origin',(3.7,-2.15,1.305)) ;
#157345=CARTESIAN_POINT('Origin',(3.7,-2.35,1.405)) ;
#157346=CARTESIAN_POINT('Origin',(3.7,-2.35,1.305)) ;
#157347=CARTESIAN_POINT('Origin',(3.5,-3.89531375123621E-17,-1.305)) ;
#157348=CARTESIAN_POINT('Origin',(3.5,-5.15,-1.305)) ;
#157349=CARTESIAN_POINT('Origin',(3.6,1.9,-1.505)) ;
#157350=CARTESIAN_POINT('Origin',(3.5,1.9,-1.505)) ;
#157351=CARTESIAN_POINT('Origin',(2.7,1.9,-1.505)) ;
#157352=CARTESIAN_POINT('Origin',(2.7,1.9,-1.405)) ;
#157353=CARTESIAN_POINT('Origin',(2.7,1.9,-1.505)) ;
#157354=CARTESIAN_POINT('Origin',(2.7,1.9,-2.305)) ;
#157355=CARTESIAN_POINT('Origin',(3.7,-2.35,1.305)) ;
#157356=CARTESIAN_POINT('Origin',(3.5,-2.35,1.305)) ;
#157357=CARTESIAN_POINT('Origin',(3.5,-5.15,-1.305)) ;
#157358=CARTESIAN_POINT('Origin',(3.5,-5.15,-1.305)) ;
#157359=CARTESIAN_POINT('Origin',(3.5,-5.15,-1.305)) ;
#157360=CARTESIAN_POINT('Origin',(2.7,1.9,-1.505)) ;
#157361=CARTESIAN_POINT('Origin',(2.7,1.9,-1.505)) ;
#157362=CARTESIAN_POINT('Origin',(3.5,-3.89531375123621E-17,1.305)) ;
#157363=CARTESIAN_POINT('Origin',(3.5,-5.15,1.305)) ;
#157364=CARTESIAN_POINT('Origin',(3.5,-5.15,0.)) ;
#157365=CARTESIAN_POINT('Origin',(3.5,-5.15,1.305)) ;
#157366=CARTESIAN_POINT('Origin',(3.6,-5.15,-1.305)) ;
#157367=CARTESIAN_POINT('Origin',(2.7,-5.15,-1.305)) ;
#157368=CARTESIAN_POINT('Origin',(2.7,-5.25,-1.505)) ;
#157369=CARTESIAN_POINT('Origin',(2.7,-5.15,-1.505)) ;
#157370=CARTESIAN_POINT('Origin',(3.5,-5.15,1.305)) ;
#157371=CARTESIAN_POINT('Origin',(3.5,-5.15,1.305)) ;
#157372=CARTESIAN_POINT('Origin',(2.7,-5.15,-1.305)) ;
#157373=CARTESIAN_POINT('Origin',(2.7,-5.35,-1.305)) ;
#157374=CARTESIAN_POINT('Origin',(2.7,1.9,2.3)) ;
#157375=CARTESIAN_POINT('Origin',(2.7,1.9,2.2)) ;
#157376=CARTESIAN_POINT('Origin',(2.7,1.9,1.505)) ;
#157377=CARTESIAN_POINT('Origin',(3.6,1.9,1.505)) ;
#157378=CARTESIAN_POINT('Origin',(3.5,1.9,1.505)) ;
#157379=CARTESIAN_POINT('Origin',(2.7,1.9,1.505)) ;
#157380=CARTESIAN_POINT('Origin',(3.6,-5.15,1.305)) ;
#157381=CARTESIAN_POINT('Origin',(2.7,-5.15,1.305)) ;
#157382=CARTESIAN_POINT('Origin',(2.7,-5.35,1.405)) ;
#157383=CARTESIAN_POINT('Origin',(2.7,-5.35,1.305)) ;
#157384=CARTESIAN_POINT('Origin',(2.7,1.9,1.505)) ;
#157385=CARTESIAN_POINT('Origin',(2.7,1.9,1.505)) ;
#157386=CARTESIAN_POINT('Origin',(2.7,-5.15,1.305)) ;
#157387=CARTESIAN_POINT('Origin',(2.7,-5.15,1.505)) ;
#157388=CARTESIAN_POINT('Origin',(2.7,2.,1.505)) ;
#157389=CARTESIAN_POINT('Origin',(7.8,2.1,-0.4)) ;
#157390=CARTESIAN_POINT('Origin',(7.8,2.1,-0.6)) ;
#157391=CARTESIAN_POINT('Origin',(7.6,2.1,-0.399999999999999)) ;
#157392=CARTESIAN_POINT('Origin',(7.6,2.1,-0.399999999999999)) ;
#157393=CARTESIAN_POINT('Origin',(7.6,2.1,0.399999999999999)) ;
#157394=CARTESIAN_POINT('Origin',(7.8,2.1,-0.6)) ;
#157395=CARTESIAN_POINT('Origin',(9.6,2.1,-0.6)) ;
#157396=CARTESIAN_POINT('Origin',(7.8,2.1,0.4)) ;
#157397=CARTESIAN_POINT('Origin',(7.8,2.1,0.6)) ;
#157398=CARTESIAN_POINT('Origin',(9.6,2.1,-0.4)) ;
#157399=CARTESIAN_POINT('Origin',(9.8,2.1,-0.399999999999999)) ;
#157400=CARTESIAN_POINT('Origin',(7.8,2.1,0.6)) ;
#157401=CARTESIAN_POINT('Origin',(9.6,2.1,0.6)) ;
#157402=CARTESIAN_POINT('Origin',(9.8,2.1,-0.399999999999999)) ;
#157403=CARTESIAN_POINT('Origin',(9.8,2.1,0.399999999999999)) ;
#157404=CARTESIAN_POINT('Origin',(9.6,2.1,0.4)) ;
#157405=CARTESIAN_POINT('Origin',(-4.9,-6.45,1.1)) ;
#157406=CARTESIAN_POINT('Origin',(-4.,-6.45,1.1)) ;
#157407=CARTESIAN_POINT('Origin',(-4.8,-6.45,1.1)) ;
#157408=CARTESIAN_POINT('Origin',(-4.8,-6.45,0.899999999999998)) ;
#157409=CARTESIAN_POINT('Origin',(-5.,-6.45,0.899999999999998)) ;
#157410=CARTESIAN_POINT('Origin',(-4.8,-6.45,0.899999999999998)) ;
#157411=CARTESIAN_POINT('Origin',(-4.,-6.45,0.899999999999998)) ;
#157412=CARTESIAN_POINT('Origin',(-4.,-6.45,0.899999999999998)) ;
#157413=CARTESIAN_POINT('Origin',(-3.8,-6.45,0.899999999999998)) ;
#157414=CARTESIAN_POINT('Origin',(-5.,-6.45,0.999999999999998)) ;
#157415=CARTESIAN_POINT('Origin',(-5.,-6.45,-0.900000000000002)) ;
#157416=CARTESIAN_POINT('Origin',(-4.8,-6.4,0.899999999999998)) ;
#157417=CARTESIAN_POINT('Origin',(-4.8,-6.35,0.899999999999998)) ;
#157418=CARTESIAN_POINT('Origin',(1.9515639104739E-16,-6.35,0.899999999999997)) ;
#157419=CARTESIAN_POINT('Origin',(-4.,-6.35,0.899999999999998)) ;
#157420=CARTESIAN_POINT('Origin',(-4.8,-6.35,0.899999999999998)) ;
#157421=CARTESIAN_POINT('Origin',(-4.,-6.4,0.899999999999998)) ;
#157422=CARTESIAN_POINT('Origin',(-4.,-6.35,0.899999999999998)) ;
#157423=CARTESIAN_POINT('Origin',(-3.8,-6.45,0.999999999999998)) ;
#157424=CARTESIAN_POINT('Origin',(-3.8,-6.45,-0.900000000000002)) ;
#157425=CARTESIAN_POINT('Origin',(-4.9,-6.45,-1.1)) ;
#157426=CARTESIAN_POINT('Origin',(-4.8,-6.45,-1.1)) ;
#157427=CARTESIAN_POINT('Origin',(-4.,-6.45,-1.1)) ;
#157428=CARTESIAN_POINT('Origin',(-4.8,-6.45,-0.900000000000002)) ;
#157429=CARTESIAN_POINT('Origin',(-4.8,-6.45,-0.900000000000002)) ;
#157430=CARTESIAN_POINT('Origin',(-4.8,-6.35,0.899999999999998)) ;
#157431=CARTESIAN_POINT('Origin',(-4.8,-6.35,0.899999999999998)) ;
#157432=CARTESIAN_POINT('Origin',(-4.,-6.35,0.899999999999998)) ;
#157433=CARTESIAN_POINT('Origin',(-4.,-6.35,0.899999999999998)) ;
#157434=CARTESIAN_POINT('Origin',(-4.,-6.45,-0.900000000000002)) ;
#157435=CARTESIAN_POINT('Origin',(-4.,-6.45,-0.900000000000002)) ;
#157436=CARTESIAN_POINT('Origin',(-4.8,-6.4,-0.900000000000002)) ;
#157437=CARTESIAN_POINT('Origin',(-4.8,-6.35,-0.900000000000002)) ;
#157438=CARTESIAN_POINT('Origin',(-4.8,-6.35,0.)) ;
#157439=CARTESIAN_POINT('Origin',(-4.8,-6.35,-0.900000000000002)) ;
#157440=CARTESIAN_POINT('Origin',(-4.,-6.35,-8.67361737988403E-16)) ;
#157441=CARTESIAN_POINT('Origin',(-4.,-6.35,-0.900000000000002)) ;
#157442=CARTESIAN_POINT('Origin',(-4.,-6.4,-0.900000000000002)) ;
#157443=CARTESIAN_POINT('Origin',(-4.,-6.35,-0.900000000000002)) ;
#157444=CARTESIAN_POINT('Origin',(-4.8,-6.35,-0.900000000000002)) ;
#157445=CARTESIAN_POINT('Origin',(-4.8,-6.35,-0.900000000000002)) ;
#157446=CARTESIAN_POINT('Origin',(-4.,-6.35,-0.900000000000002)) ;
#157447=CARTESIAN_POINT('Origin',(-4.,-6.35,-0.900000000000002)) ;
#157448=CARTESIAN_POINT('Origin',(1.95156391047391E-16,-6.35,-0.900000000000001)) ;
#157449=CARTESIAN_POINT('Origin',(-4.15,-6.25,0.749999999999998)) ;
#157450=CARTESIAN_POINT('Origin',(-4.15,-6.3,0.749999999999998)) ;
#157451=CARTESIAN_POINT('Origin',(-4.15,-6.3,0.)) ;
#157452=CARTESIAN_POINT('Origin',(-4.15,-6.3,-0.750000000000002)) ;
#157453=CARTESIAN_POINT('Origin',(-4.15,-6.3,0.749999999999998)) ;
#157454=CARTESIAN_POINT('Origin',(-4.15,-6.25,-0.750000000000002)) ;
#157455=CARTESIAN_POINT('Origin',(-4.15,-6.3,-0.750000000000002)) ;
#157456=CARTESIAN_POINT('Origin',(-4.15,-6.3,0.749999999999998)) ;
#157457=CARTESIAN_POINT('Origin',(-4.15,-6.3,0.749999999999998)) ;
#157458=CARTESIAN_POINT('Origin',(-4.15,-6.3,-0.750000000000002)) ;
#157459=CARTESIAN_POINT('Origin',(-4.15,-6.3,-0.750000000000002)) ;
#157460=CARTESIAN_POINT('Origin',(-4.65,-6.25,0.749999999999998)) ;
#157461=CARTESIAN_POINT('Origin',(-4.65,-6.3,0.749999999999998)) ;
#157462=CARTESIAN_POINT('Origin',(0.,-6.3,0.749999999999998)) ;
#157463=CARTESIAN_POINT('Origin',(-4.65,-6.3,0.749999999999998)) ;
#157464=CARTESIAN_POINT('Origin',(0.,-6.3,-0.750000000000002)) ;
#157465=CARTESIAN_POINT('Origin',(-4.65,-6.3,-0.750000000000002)) ;
#157466=CARTESIAN_POINT('Origin',(-4.65,-6.25,-0.750000000000002)) ;
#157467=CARTESIAN_POINT('Origin',(-4.65,-6.3,-0.750000000000002)) ;
#157468=CARTESIAN_POINT('Origin',(-4.65,-6.3,0.749999999999998)) ;
#157469=CARTESIAN_POINT('Origin',(-4.65,-6.3,0.749999999999998)) ;
#157470=CARTESIAN_POINT('Origin',(-4.65,-6.3,-0.750000000000002)) ;
#157471=CARTESIAN_POINT('Origin',(-4.65,-6.3,-0.750000000000002)) ;
#157472=CARTESIAN_POINT('Origin',(-4.65,-6.3,0.)) ;
#157473=CARTESIAN_POINT('Origin',(-3.09057773798104,-4.00084361825625,-0.500553917240007)) ;
#157474=CARTESIAN_POINT('Origin',(-5.17275707706437,-1.91866427917293,-1.5)) ;
#157475=CARTESIAN_POINT('Origin',(-5.17275707706437,-1.91866427917293,-1.5)) ;
#157476=CARTESIAN_POINT('Origin',(-5.17275707706437,-1.91866427917293,-1.5)) ;
#157477=CARTESIAN_POINT('Origin',(-5.17275707706437,-1.91866427917293,-1.5)) ;
#157478=CARTESIAN_POINT('Origin',(-3.59571067811865,-3.49571067811865,-1.5)) ;
#157479=CARTESIAN_POINT('Ctrl Pts',(-5.8,-1.2914213562373,-1.6)) ;
#157480=CARTESIAN_POINT('Ctrl Pts',(-5.81856398038093,-1.23572941509445,
-1.6)) ;
#157481=CARTESIAN_POINT('Ctrl Pts',(-5.83691006697102,-1.18069115532419,
-1.58922263893877)) ;
#157482=CARTESIAN_POINT('Ctrl Pts',(-5.86308993302897,-1.1021515571504,
-1.55219871729854)) ;
#157483=CARTESIAN_POINT('Ctrl Pts',(-5.87071067695841,-1.07928932304158,
-1.5262534328036)) ;
#157484=CARTESIAN_POINT('Ctrl Pts',(-5.87071067811865,-1.07928932188133,
-1.5)) ;
#157485=CARTESIAN_POINT('Origin',(-5.17275707706437,-5.05,-1.5)) ;
#157486=CARTESIAN_POINT('Origin',(-5.17275707706437,-5.26511162862565,-1.5)) ;
#157487=CARTESIAN_POINT('Origin',(-3.96111272388873,-4.96220054033175,-0.918410710475694)) ;
#157488=CARTESIAN_POINT('Origin',(-5.17275707706437,-5.26511162862565,-1.5)) ;
#157489=CARTESIAN_POINT('Ctrl Pts',(-5.9,-1.00857864376268,-1.5)) ;
#157490=CARTESIAN_POINT('Ctrl Pts',(-5.9,-1.04999999999999,-1.5)) ;
#157491=CARTESIAN_POINT('Ctrl Pts',(-5.87071067811865,-1.07928932188133,
-1.5)) ;
#157492=CARTESIAN_POINT('Ctrl Pts',(-5.9,-1.00857864608314,-1.55250686562996)) ;
#157493=CARTESIAN_POINT('Ctrl Pts',(-5.9,-1.05000000261917,-1.53717194963254)) ;
#157494=CARTESIAN_POINT('Ctrl Pts',(-5.87071067695841,-1.07928932304158,
-1.5262534328036)) ;
#157495=CARTESIAN_POINT('Ctrl Pts',(-5.9,-1.03906162412144,-1.60439743459708)) ;
#157496=CARTESIAN_POINT('Ctrl Pts',(-5.9,-1.08015861705713,-1.57457207120097)) ;
#157497=CARTESIAN_POINT('Ctrl Pts',(-5.86308993302897,-1.1021515571504,
-1.55219871729854)) ;
#157498=CARTESIAN_POINT('Ctrl Pts',(-5.9,-1.14378108835315,-1.67844527787754)) ;
#157499=CARTESIAN_POINT('Ctrl Pts',(-5.9,-1.17342005527962,-1.61578812462635)) ;
#157500=CARTESIAN_POINT('Ctrl Pts',(-5.83691006697102,-1.18069115532419,
-1.58922263893877)) ;
#157501=CARTESIAN_POINT('Ctrl Pts',(-5.9,-1.21716543471636,-1.69999999941986)) ;
#157502=CARTESIAN_POINT('Ctrl Pts',(-5.9,-1.24006789214486,-1.61711774888611)) ;
#157503=CARTESIAN_POINT('Ctrl Pts',(-5.81856398038093,-1.23572941509445,
-1.6)) ;
#157504=CARTESIAN_POINT('Ctrl Pts',(-5.9,-1.2914213562373,-1.7)) ;
#157505=CARTESIAN_POINT('Ctrl Pts',(-5.9,-1.2914213562373,-1.6)) ;
#157506=CARTESIAN_POINT('Ctrl Pts',(-5.8,-1.2914213562373,-1.6)) ;
#157507=CARTESIAN_POINT('Origin',(-5.8,-1.2914213562373,-1.7)) ;
#157508=CARTESIAN_POINT('Origin',(-5.8,-1.00857864376268,-1.5)) ;
#157509=CARTESIAN_POINT('Origin',(-5.17275707706437,-5.26511162862565,-1.5)) ;
#157510=CARTESIAN_POINT('Origin',(-5.17275707706437,-5.26511162862565,-1.5)) ;
#157511=CARTESIAN_POINT('Origin',(-3.78014014831103,-3.31128120792626,0.8315438741984)) ;
#157512=CARTESIAN_POINT('Origin',(-5.17275707706436,-1.91866427917293,1.5)) ;
#157513=CARTESIAN_POINT('Origin',(-3.97071067811865,-3.12071067811865,1.5)) ;
#157514=CARTESIAN_POINT('Ctrl Pts',(-5.87071067811865,-1.07928932188133,
1.5)) ;
#157515=CARTESIAN_POINT('Ctrl Pts',(-5.8707106769584,-1.07928932304159,
1.52625343280361)) ;
#157516=CARTESIAN_POINT('Ctrl Pts',(-5.86308993302895,-1.10215155715041,
1.55219871729854)) ;
#157517=CARTESIAN_POINT('Ctrl Pts',(-5.83691006697104,-1.18069115532418,
1.58922263893878)) ;
#157518=CARTESIAN_POINT('Ctrl Pts',(-5.81856398038092,-1.23572941509446,
1.6)) ;
#157519=CARTESIAN_POINT('Ctrl Pts',(-5.8,-1.2914213562373,1.6)) ;
#157520=CARTESIAN_POINT('Origin',(-5.17275707706436,-1.91866427917293,1.5)) ;
#157521=CARTESIAN_POINT('Origin',(-5.8,-1.00857864376268,-36.59)) ;
#157522=CARTESIAN_POINT('Origin',(-5.8,-1.00857864376268,1.5)) ;
#157523=CARTESIAN_POINT('Origin',(-5.8,-6.55,-1.7)) ;
#157524=CARTESIAN_POINT('Origin',(-5.8,-5.42192235935956,-1.7)) ;
#157525=CARTESIAN_POINT('Origin',(-5.10072415073893,-5.24710339704429,-1.5)) ;
#157526=CARTESIAN_POINT('Origin',(-5.80000000000002,-5.42192235935965,-1.50000000000007)) ;
#157527=CARTESIAN_POINT('Origin',(-5.17275707706436,-1.91866427917293,1.5)) ;
#157528=CARTESIAN_POINT('Origin',(-5.17275707706436,-1.91866427917293,1.5)) ;
#157529=CARTESIAN_POINT('Ctrl Pts',(-5.9,-1.2914213562373,1.7)) ;
#157530=CARTESIAN_POINT('Ctrl Pts',(-5.9,-1.2914213562373,1.6)) ;
#157531=CARTESIAN_POINT('Ctrl Pts',(-5.8,-1.2914213562373,1.6)) ;
#157532=CARTESIAN_POINT('Ctrl Pts',(-5.9,-1.21716543471637,1.69999999941986)) ;
#157533=CARTESIAN_POINT('Ctrl Pts',(-5.9,-1.24006789214486,1.6171177488861)) ;
#157534=CARTESIAN_POINT('Ctrl Pts',(-5.81856398038092,-1.23572941509446,
1.6)) ;
#157535=CARTESIAN_POINT('Ctrl Pts',(-5.9,-1.14378108835315,1.67844527787754)) ;
#157536=CARTESIAN_POINT('Ctrl Pts',(-5.9,-1.17342005527961,1.61578812462635)) ;
#157537=CARTESIAN_POINT('Ctrl Pts',(-5.83691006697104,-1.18069115532418,
1.58922263893878)) ;
#157538=CARTESIAN_POINT('Ctrl Pts',(-5.9,-1.03906162412145,1.60439743459708)) ;
#157539=CARTESIAN_POINT('Ctrl Pts',(-5.9,-1.08015861705713,1.57457207120097)) ;
#157540=CARTESIAN_POINT('Ctrl Pts',(-5.86308993302895,-1.10215155715041,
1.55219871729854)) ;
#157541=CARTESIAN_POINT('Ctrl Pts',(-5.9,-1.00857864608316,1.55250686562996)) ;
#157542=CARTESIAN_POINT('Ctrl Pts',(-5.9,-1.05000000261919,1.53717194963254)) ;
#157543=CARTESIAN_POINT('Ctrl Pts',(-5.8707106769584,-1.07928932304159,
1.52625343280361)) ;
#157544=CARTESIAN_POINT('Ctrl Pts',(-5.9,-1.00857864376268,1.5)) ;
#157545=CARTESIAN_POINT('Ctrl Pts',(-5.9,-1.04999999999999,1.5)) ;
#157546=CARTESIAN_POINT('Ctrl Pts',(-5.87071067811865,-1.07928932188133,
1.5)) ;
#157547=CARTESIAN_POINT('Origin',(-5.8,-1.2914213562373,1.7)) ;
#157548=CARTESIAN_POINT('Ctrl Pts',(-5.9,-5.42181243301045,-1.69999997036252)) ;
#157549=CARTESIAN_POINT('Ctrl Pts',(-5.9,-5.42186418462486,-1.5999118155266)) ;
#157550=CARTESIAN_POINT('Ctrl Pts',(-5.79991187715164,-5.42186416305549,
-1.60000002317701)) ;
#157551=CARTESIAN_POINT('Ctrl Pts',(-5.9,-5.47597273077135,-1.70002917711601)) ;
#157552=CARTESIAN_POINT('Ctrl Pts',(-5.9,-5.44963575044052,-1.60611310490823)) ;
#157553=CARTESIAN_POINT('Ctrl Pts',(-5.80628621775607,-5.45053795385126,
-1.60000983135988)) ;
#157554=CARTESIAN_POINT('Ctrl Pts',(-5.9,-5.5295069829522,-1.67847029676528)) ;
#157555=CARTESIAN_POINT('Ctrl Pts',(-5.90000000000002,-5.48352164712825,
-1.60029821762257)) ;
#157556=CARTESIAN_POINT('Ctrl Pts',(-5.81258729511711,-5.47887520585224,
-1.58922629545968)) ;
#157557=CARTESIAN_POINT('Ctrl Pts',(-5.9,-5.60588533050918,-1.60437241570934)) ;
#157558=CARTESIAN_POINT('Ctrl Pts',(-5.89999999999997,-5.53371219741587,
-1.56246819784151)) ;
#157559=CARTESIAN_POINT('Ctrl Pts',(-5.82157770712951,-5.51930255765375,
-1.55217766736415)) ;
#157560=CARTESIAN_POINT('Ctrl Pts',(-5.9,-5.62810771557601,-1.55243656245292)) ;
#157561=CARTESIAN_POINT('Ctrl Pts',(-5.9,-5.54996909580657,-1.5314248414507)) ;
#157562=CARTESIAN_POINT('Ctrl Pts',(-5.8241936039171,-5.53106345572106,
-1.52621391054005)) ;
#157563=CARTESIAN_POINT('Ctrl Pts',(-5.9,-5.62807761009112,-1.49989335577685)) ;
#157564=CARTESIAN_POINT('Ctrl Pts',(-5.9,-5.54994729905278,-1.49993608021398)) ;
#157565=CARTESIAN_POINT('Ctrl Pts',(-5.82419006898363,-5.53104752404526,
-1.49994668678336)) ;
#157566=CARTESIAN_POINT('Origin',(-5.8,-5.62807764064044,-1.5)) ;
#157567=CARTESIAN_POINT('Origin',(-5.15068655017073,-5.25959399690224,1.48940614709106)) ;
#157568=CARTESIAN_POINT('Origin',(-5.17275707706436,-5.26511162862565,1.5)) ;
#157569=CARTESIAN_POINT('Origin',(-5.17275707706436,-5.05,1.5)) ;
#157570=CARTESIAN_POINT('Origin',(-5.17275707706436,-5.26511162862565,1.5)) ;
#157571=CARTESIAN_POINT('Origin',(-5.8,-5.05,1.7)) ;
#157572=CARTESIAN_POINT('Origin',(-5.8,-5.42192235935956,1.7)) ;
#157573=CARTESIAN_POINT('Origin',(-5.8,-5.62807764064044,-36.59)) ;
#157574=CARTESIAN_POINT('Origin',(-5.8,-5.62807764064044,1.5)) ;
#157575=CARTESIAN_POINT('Origin',(-5.17275707706436,-5.26511162862565,1.5)) ;
#157576=CARTESIAN_POINT('Origin',(-5.17275707706436,-5.26511162862565,1.5)) ;
#157577=CARTESIAN_POINT('Ctrl Pts',(-5.9,-5.62807761009112,1.49989335577687)) ;
#157578=CARTESIAN_POINT('Ctrl Pts',(-5.9,-5.54994729905279,1.49993608021399)) ;
#157579=CARTESIAN_POINT('Ctrl Pts',(-5.82419006898364,-5.53104752404526,
1.49994668678337)) ;
#157580=CARTESIAN_POINT('Ctrl Pts',(-5.9,-5.62810771557601,1.55243656245293)) ;
#157581=CARTESIAN_POINT('Ctrl Pts',(-5.9,-5.54996909580664,1.5314248414507)) ;
#157582=CARTESIAN_POINT('Ctrl Pts',(-5.82419360391714,-5.53106345572106,
1.52621391054006)) ;
#157583=CARTESIAN_POINT('Ctrl Pts',(-5.9,-5.6058853305092,1.60437241570935)) ;
#157584=CARTESIAN_POINT('Ctrl Pts',(-5.89999999999997,-5.53371219741588,
1.56246819784153)) ;
#157585=CARTESIAN_POINT('Ctrl Pts',(-5.82157770712952,-5.51930255765375,
1.55217766736414)) ;
#157586=CARTESIAN_POINT('Ctrl Pts',(-5.9,-5.52950698295218,1.67847029676527)) ;
#157587=CARTESIAN_POINT('Ctrl Pts',(-5.90000000000002,-5.48352164712826,
1.60029821762257)) ;
#157588=CARTESIAN_POINT('Ctrl Pts',(-5.81258729511712,-5.47887520585224,
1.58922629545969)) ;
#157589=CARTESIAN_POINT('Ctrl Pts',(-5.9,-5.47597273077138,1.700029177116)) ;
#157590=CARTESIAN_POINT('Ctrl Pts',(-5.9,-5.44963575044054,1.60611310490826)) ;
#157591=CARTESIAN_POINT('Ctrl Pts',(-5.80628621775611,-5.45053795385126,
1.60000983135988)) ;
#157592=CARTESIAN_POINT('Ctrl Pts',(-5.9,-5.42181243301047,1.69999997036252)) ;
#157593=CARTESIAN_POINT('Ctrl Pts',(-5.9,-5.42186418462487,1.59991181552662)) ;
#157594=CARTESIAN_POINT('Ctrl Pts',(-5.79991187715165,-5.4218641630555,
1.60000002317701)) ;
#157595=CARTESIAN_POINT('Origin',(-5.80000000000001,-5.42192235935961,1.50000000000005)) ;
#157596=CARTESIAN_POINT('Origin',(-5.8066065036801,-5.42357398527959,1.5)) ;
#157597=CARTESIAN_POINT('Origin',(-3.,4.45,-1.1)) ;
#157598=CARTESIAN_POINT('Origin',(-2.1,4.45,-1.1)) ;
#157599=CARTESIAN_POINT('Origin',(-2.9,4.45,-1.1)) ;
#157600=CARTESIAN_POINT('Origin',(-2.9,4.45,-0.899999999999999)) ;
#157601=CARTESIAN_POINT('Origin',(-3.1,4.45,-0.899999999999999)) ;
#157602=CARTESIAN_POINT('Origin',(-2.9,4.45,-0.899999999999999)) ;
#157603=CARTESIAN_POINT('Origin',(-2.1,4.45,-0.9)) ;
#157604=CARTESIAN_POINT('Origin',(-2.1,4.45,-0.9)) ;
#157605=CARTESIAN_POINT('Origin',(-1.9,4.45,-0.9)) ;
#157606=CARTESIAN_POINT('Origin',(-3.1,4.45,-0.999999999999999)) ;
#157607=CARTESIAN_POINT('Origin',(-3.1,4.45,0.900000000000001)) ;
#157608=CARTESIAN_POINT('Origin',(-2.9,4.4,-0.899999999999999)) ;
#157609=CARTESIAN_POINT('Origin',(-2.9,4.35,-0.899999999999999)) ;
#157610=CARTESIAN_POINT('Origin',(-1.95156391047391E-16,4.35,-0.9)) ;
#157611=CARTESIAN_POINT('Origin',(-2.1,4.35,-0.9)) ;
#157612=CARTESIAN_POINT('Origin',(-2.9,4.35,-0.899999999999999)) ;
#157613=CARTESIAN_POINT('Origin',(-2.1,4.4,-0.9)) ;
#157614=CARTESIAN_POINT('Origin',(-2.1,4.35,-0.9)) ;
#157615=CARTESIAN_POINT('Origin',(-1.9,4.45,-1.)) ;
#157616=CARTESIAN_POINT('Origin',(-1.9,4.45,0.900000000000001)) ;
#157617=CARTESIAN_POINT('Origin',(-3.,4.45,1.1)) ;
#157618=CARTESIAN_POINT('Origin',(-2.9,4.45,1.1)) ;
#157619=CARTESIAN_POINT('Origin',(-2.1,4.45,1.1)) ;
#157620=CARTESIAN_POINT('Origin',(-2.9,4.45,0.900000000000001)) ;
#157621=CARTESIAN_POINT('Origin',(-2.9,4.45,0.900000000000001)) ;
#157622=CARTESIAN_POINT('Origin',(-2.9,4.35,-0.899999999999999)) ;
#157623=CARTESIAN_POINT('Origin',(-2.9,4.35,-0.899999999999999)) ;
#157624=CARTESIAN_POINT('Origin',(-2.1,4.35,-0.9)) ;
#157625=CARTESIAN_POINT('Origin',(-2.1,4.35,-0.9)) ;
#157626=CARTESIAN_POINT('Origin',(-2.1,4.45,0.900000000000001)) ;
#157627=CARTESIAN_POINT('Origin',(-2.1,4.45,0.900000000000001)) ;
#157628=CARTESIAN_POINT('Origin',(-2.9,4.4,0.900000000000001)) ;
#157629=CARTESIAN_POINT('Origin',(-2.9,4.35,0.900000000000001)) ;
#157630=CARTESIAN_POINT('Origin',(-2.9,4.35,1.25767452008319E-15)) ;
#157631=CARTESIAN_POINT('Origin',(-2.9,4.35,0.900000000000001)) ;
#157632=CARTESIAN_POINT('Origin',(-2.1,4.35,4.55364912443912E-16)) ;
#157633=CARTESIAN_POINT('Origin',(-2.1,4.35,0.900000000000001)) ;
#157634=CARTESIAN_POINT('Origin',(-2.1,4.4,0.900000000000001)) ;
#157635=CARTESIAN_POINT('Origin',(-2.1,4.35,0.900000000000001)) ;
#157636=CARTESIAN_POINT('Origin',(-2.9,4.35,0.900000000000001)) ;
#157637=CARTESIAN_POINT('Origin',(-2.9,4.35,0.900000000000001)) ;
#157638=CARTESIAN_POINT('Origin',(-2.1,4.35,0.900000000000001)) ;
#157639=CARTESIAN_POINT('Origin',(-2.1,4.35,0.900000000000001)) ;
#157640=CARTESIAN_POINT('Origin',(-1.95156391047391E-16,4.35,0.900000000000001)) ;
#157641=CARTESIAN_POINT('Origin',(-2.25,4.25,-0.75)) ;
#157642=CARTESIAN_POINT('Origin',(-2.25,4.3,-0.75)) ;
#157643=CARTESIAN_POINT('Origin',(-2.25,4.3,0.)) ;
#157644=CARTESIAN_POINT('Origin',(-2.25,4.3,0.750000000000001)) ;
#157645=CARTESIAN_POINT('Origin',(-2.25,4.3,-0.75)) ;
#157646=CARTESIAN_POINT('Origin',(-2.25,4.25,0.750000000000001)) ;
#157647=CARTESIAN_POINT('Origin',(-2.25,4.3,0.750000000000001)) ;
#157648=CARTESIAN_POINT('Origin',(-2.25,4.3,-0.75)) ;
#157649=CARTESIAN_POINT('Origin',(-2.25,4.3,-0.75)) ;
#157650=CARTESIAN_POINT('Origin',(-2.25,4.3,0.750000000000001)) ;
#157651=CARTESIAN_POINT('Origin',(-2.25,4.3,0.750000000000001)) ;
#157652=CARTESIAN_POINT('Origin',(-2.75,4.25,-0.75)) ;
#157653=CARTESIAN_POINT('Origin',(-2.75,4.3,-0.75)) ;
#157654=CARTESIAN_POINT('Origin',(-1.97127667724637E-17,4.3,-0.75)) ;
#157655=CARTESIAN_POINT('Origin',(-2.75,4.3,-0.75)) ;
#157656=CARTESIAN_POINT('Origin',(-1.97127667724637E-17,4.3,0.750000000000001)) ;
#157657=CARTESIAN_POINT('Origin',(-2.75,4.3,0.750000000000001)) ;
#157658=CARTESIAN_POINT('Origin',(-2.75,4.25,0.750000000000001)) ;
#157659=CARTESIAN_POINT('Origin',(-2.75,4.3,0.750000000000001)) ;
#157660=CARTESIAN_POINT('Origin',(-2.75,4.3,-0.75)) ;
#157661=CARTESIAN_POINT('Origin',(-2.75,4.3,-0.75)) ;
#157662=CARTESIAN_POINT('Origin',(-2.75,4.3,0.750000000000001)) ;
#157663=CARTESIAN_POINT('Origin',(-2.75,4.3,0.750000000000001)) ;
#157664=CARTESIAN_POINT('Origin',(-2.75,4.3,0.)) ;
#157665=CARTESIAN_POINT('Origin',(7.8,2.9,-0.4)) ;
#157666=CARTESIAN_POINT('Origin',(7.8,2.9,-0.399999999999999)) ;
#157667=CARTESIAN_POINT('Origin',(7.8,2.9,0.4)) ;
#157668=CARTESIAN_POINT('Origin',(7.8,2.9,0.4)) ;
#157669=CARTESIAN_POINT('Origin',(7.8,2.9,0.4)) ;
#157670=CARTESIAN_POINT('Origin',(7.8,2.9,-0.4)) ;
#157671=CARTESIAN_POINT('Origin',(7.8,2.9,-0.4)) ;
#157672=CARTESIAN_POINT('Origin',(9.6,2.9,0.4)) ;
#157673=CARTESIAN_POINT('Origin',(9.6,2.9,0.4)) ;
#157674=CARTESIAN_POINT('Origin',(9.6,2.9,-0.4)) ;
#157675=CARTESIAN_POINT('Origin',(9.6,2.9,-0.4)) ;
#157676=CARTESIAN_POINT('Origin',(9.6,2.9,0.4)) ;
#157677=CARTESIAN_POINT('Origin',(9.6,2.9,0.4)) ;
#157678=CARTESIAN_POINT('Origin',(9.6,2.9,-0.4)) ;
#157679=CARTESIAN_POINT('Origin',(9.6,2.9,-0.4)) ;
#157680=CARTESIAN_POINT('Origin',(9.6,2.9,-0.4)) ;
#157681=CARTESIAN_POINT('Origin',(-0.183301359729408,3.45,1.51703678647597)) ;
#157682=CARTESIAN_POINT('Origin',(0.249234641435079,3.15,0.116220021978692)) ;
#157683=CARTESIAN_POINT('Origin',(-0.249234641435079,3.15,-0.116220021978691)) ;
#157684=CARTESIAN_POINT('Origin',(-1.04429375741423,3.45,1.11554943782231)) ;
#157685=CARTESIAN_POINT('Origin',(3.7,2.1,1.405)) ;
#157686=CARTESIAN_POINT('Origin',(3.7,2.1,-1.305)) ;
#157687=CARTESIAN_POINT('Origin',(3.7,2.1,1.305)) ;
#157688=CARTESIAN_POINT('Origin',(3.5,1.9,-1.505)) ;
#157689=CARTESIAN_POINT('Ctrl Pts',(3.6,2.07320508075689,-1.405)) ;
#157690=CARTESIAN_POINT('Ctrl Pts',(3.6,2.07265589924994,-1.40785357667012)) ;
#157691=CARTESIAN_POINT('Ctrl Pts',(3.59994554076638,2.07202433860048,-1.41069358004935)) ;
#157692=CARTESIAN_POINT('Ctrl Pts',(3.59971739924421,2.07059366100574,-1.41637921497761)) ;
#157693=CARTESIAN_POINT('Ctrl Pts',(3.59954156373429,2.06979274847061,-1.41921873634692)) ;
#157694=CARTESIAN_POINT('Ctrl Pts',(3.59880783141188,2.06712577191666,-1.42778089072516)) ;
#157695=CARTESIAN_POINT('Ctrl Pts',(3.59804129495589,2.06501902766395,-1.43341713644376)) ;
#157696=CARTESIAN_POINT('Ctrl Pts',(3.59624340061598,2.06105248659392,-1.44263353946359)) ;
#157697=CARTESIAN_POINT('Ctrl Pts',(3.59536494855695,2.05931170891995,-1.44632347138735)) ;
#157698=CARTESIAN_POINT('Ctrl Pts',(3.5928372720244,2.05479606436795,-1.455199432059)) ;
#157699=CARTESIAN_POINT('Ctrl Pts',(3.59099650883093,2.05188276467124,-1.46034424200706)) ;
#157700=CARTESIAN_POINT('Ctrl Pts',(3.58838944624309,2.04823719194674,-1.46622737667939)) ;
#157701=CARTESIAN_POINT('Ctrl Pts',(3.58794537962076,2.04762948672744,-1.46719091385134)) ;
#157702=CARTESIAN_POINT('Ctrl Pts',(3.58597371492279,2.04498948329048,-1.47130665172963)) ;
#157703=CARTESIAN_POINT('Ctrl Pts',(3.58430396743904,2.04289920268562,-1.47439316248021)) ;
#157704=CARTESIAN_POINT('Ctrl Pts',(3.58008903321357,2.03798436571146,-1.48128092067897)) ;
#157705=CARTESIAN_POINT('Ctrl Pts',(3.57743593401588,2.03513945367721,-1.48500157292061)) ;
#157706=CARTESIAN_POINT('Ctrl Pts',(3.57357563759669,2.03136250950851,-1.48958640159683)) ;
#157707=CARTESIAN_POINT('Ctrl Pts',(3.57257888733677,2.03041544381404,-1.4907065689314)) ;
#157708=CARTESIAN_POINT('Ctrl Pts',(3.56956839719837,2.02764175140689,-1.49390390778887)) ;
#157709=CARTESIAN_POINT('Ctrl Pts',(3.56746189551945,2.0258155454478,-1.49598430067905)) ;
#157710=CARTESIAN_POINT('Ctrl Pts',(3.56503628433181,2.02384076964141,-1.49802226003861)) ;
#157711=CARTESIAN_POINT('Ctrl Pts',(3.5648141102349,2.02366103014354,-1.49820583968788)) ;
#157712=CARTESIAN_POINT('Ctrl Pts',(3.56285239425757,2.0220841692406,-1.49979838212051)) ;
#157713=CARTESIAN_POINT('Ctrl Pts',(3.56093641846876,2.02061618613969,-1.5011871777518)) ;
#157714=CARTESIAN_POINT('Ctrl Pts',(3.55879736620766,2.01908299720835,-1.50237714025468)) ;
#157715=CARTESIAN_POINT('Ctrl Pts',(3.55867935922407,2.0189987330146,-1.50244171035243)) ;
#157716=CARTESIAN_POINT('Ctrl Pts',(3.5578895339955,2.01843691186419,-1.50286648337378)) ;
#157717=CARTESIAN_POINT('Ctrl Pts',(3.55720723474254,2.01796200020269,-1.503197549106)) ;
#157718=CARTESIAN_POINT('Ctrl Pts',(3.5550912564315,2.01652382826845,-1.50409794445158)) ;
#157719=CARTESIAN_POINT('Ctrl Pts',(3.55356547969789,2.01553571874064,-1.50460356135169)) ;
#157720=CARTESIAN_POINT('Ctrl Pts',(3.55133342567602,2.01417771500981,-1.50494476439962)) ;
#157721=CARTESIAN_POINT('Ctrl Pts',(3.55066861961528,2.01378348733642,-1.50499963178873)) ;
#157722=CARTESIAN_POINT('Ctrl Pts',(3.55,2.01339745962156,-1.505)) ;
#157723=CARTESIAN_POINT('Origin',(3.5,2.1,1.01757522333835E-15)) ;
#157724=CARTESIAN_POINT('Origin',(3.5,2.1,2.2)) ;
#157725=CARTESIAN_POINT('',(3.55,2.01339745962156,1.505)) ;
#157726=CARTESIAN_POINT('Origin',(3.5,2.1,1.505)) ;
#157727=CARTESIAN_POINT('Origin',(3.5,2.1,1.505)) ;
#157728=CARTESIAN_POINT('Origin',(3.5,1.9,1.505)) ;
#157729=CARTESIAN_POINT('Ctrl Pts',(3.55,2.01339745962156,1.505)) ;
#157730=CARTESIAN_POINT('Ctrl Pts',(3.55164546205118,2.01434746757975,1.505)) ;
#157731=CARTESIAN_POINT('Ctrl Pts',(3.55326668047441,2.01534654795451,1.50466702196971)) ;
#157732=CARTESIAN_POINT('Ctrl Pts',(3.55550702654634,2.01680421826673,1.50390173831696)) ;
#157733=CARTESIAN_POINT('Ctrl Pts',(3.55618577699068,2.01725684095079,1.50362640393618)) ;
#157734=CARTESIAN_POINT('Ctrl Pts',(3.55727967686454,2.01800266699454,1.5031321699042)) ;
#157735=CARTESIAN_POINT('Ctrl Pts',(3.55771141786834,2.01830156212325,1.50292168105742)) ;
#157736=CARTESIAN_POINT('Ctrl Pts',(3.5620282181816,2.02133211263483,1.50082930890279)) ;
#157737=CARTESIAN_POINT('Ctrl Pts',(3.56570108751482,2.02427663140642,1.4977560683717)) ;
#157738=CARTESIAN_POINT('Ctrl Pts',(3.56990347726565,2.02797441535149,1.49359799526151)) ;
#157739=CARTESIAN_POINT('Ctrl Pts',(3.57072473561128,2.02871480216323,1.49275040226905)) ;
#157740=CARTESIAN_POINT('Ctrl Pts',(3.5738286330762,2.03157464832067,1.48945828106714)) ;
#157741=CARTESIAN_POINT('Ctrl Pts',(3.5759706937612,2.03369481096682,1.48686226564267)) ;
#157742=CARTESIAN_POINT('Ctrl Pts',(3.58156103639367,2.03956384830232,1.47924188322025)) ;
#157743=CARTESIAN_POINT('Ctrl Pts',(3.58475859790494,2.04336775308648,1.47384516147842)) ;
#157744=CARTESIAN_POINT('Ctrl Pts',(3.58897725231935,2.0490105592432,1.46504516569941)) ;
#157745=CARTESIAN_POINT('Ctrl Pts',(3.59034871903171,2.05099358132072,1.46177746615682)) ;
#157746=CARTESIAN_POINT('Ctrl Pts',(3.5936548829273,2.05613355260445,1.45275077139164)) ;
#157747=CARTESIAN_POINT('Ctrl Pts',(3.59534780095526,2.05919518104046,1.44675628838969)) ;
#157748=CARTESIAN_POINT('Ctrl Pts',(3.59674625886212,2.06216860863465,1.44003955337032)) ;
#157749=CARTESIAN_POINT('Ctrl Pts',(3.59685725281059,2.06240883133061,1.43948968489037)) ;
#157750=CARTESIAN_POINT('Ctrl Pts',(3.59768573690243,2.06423460359408,1.43525346237999)) ;
#157751=CARTESIAN_POINT('Ctrl Pts',(3.59826864191792,2.06571343564803,1.43147600284345)) ;
#157752=CARTESIAN_POINT('Ctrl Pts',(3.59959273712775,2.06963221119414,1.42031698563094)) ;
#157753=CARTESIAN_POINT('Ctrl Pts',(3.6,2.07172309150643,1.4127006420342)) ;
#157754=CARTESIAN_POINT('Ctrl Pts',(3.6,2.07320508075689,1.405)) ;
#157755=CARTESIAN_POINT('Origin',(3.7,2.1,-1.305)) ;
#157756=CARTESIAN_POINT('',(3.7,1.98660254037844,-1.355)) ;
#157757=CARTESIAN_POINT('Ctrl Pts',(3.60000000000001,1.92679491924311,-1.405)) ;
#157758=CARTESIAN_POINT('Ctrl Pts',(3.60642117639485,1.92803067521647,-1.405)) ;
#157759=CARTESIAN_POINT('Ctrl Pts',(3.61278477806503,1.92968896670923,-1.40472281361407)) ;
#157760=CARTESIAN_POINT('Ctrl Pts',(3.61897283239529,1.93170032347262,-1.40412352491366)) ;
#157761=CARTESIAN_POINT('Ctrl Pts',(3.62020584678442,1.93210110079269,-1.40400411232427)) ;
#157762=CARTESIAN_POINT('Ctrl Pts',(3.62143195421093,1.93251577262755,-1.40387200280826)) ;
#157763=CARTESIAN_POINT('Ctrl Pts',(3.62265032708637,1.93294361409314,-1.40372698243403)) ;
#157764=CARTESIAN_POINT('Ctrl Pts',(3.62647624625549,1.9342871164786,-1.40327159128008)) ;
#157765=CARTESIAN_POINT('Ctrl Pts',(3.63025346237246,1.93576539638805,-1.40268573681767)) ;
#157766=CARTESIAN_POINT('Ctrl Pts',(3.6339385638818,1.93735364065939,-1.40196503626974)) ;
#157767=CARTESIAN_POINT('Ctrl Pts',(3.63907793749077,1.93956866259897,-1.40095992165713)) ;
#157768=CARTESIAN_POINT('Ctrl Pts',(3.64410916187591,1.94202076919908,-1.39967872244964)) ;
#157769=CARTESIAN_POINT('Ctrl Pts',(3.64894317395077,1.94461872744763,-1.39812217773587)) ;
#157770=CARTESIAN_POINT('Ctrl Pts',(3.64993855309172,1.94515367717668,-1.39780166712976)) ;
#157771=CARTESIAN_POINT('Ctrl Pts',(3.65092568100083,1.94569474416709,-1.39746960315684)) ;
#157772=CARTESIAN_POINT('Ctrl Pts',(3.65190395907102,1.94624104404953,-1.3971261809367)) ;
#157773=CARTESIAN_POINT('Ctrl Pts',(3.65241342868356,1.94652554719634,-1.39694733282514)) ;
#157774=CARTESIAN_POINT('Ctrl Pts',(3.65292046817501,1.9468114778021,-1.39676540573999)) ;
#157775=CARTESIAN_POINT('Ctrl Pts',(3.6534249821411,1.94709871486666,-1.39658043363331)) ;
#157776=CARTESIAN_POINT('Ctrl Pts',(3.65677402871197,1.94900544167845,-1.39535255840841)) ;
#157777=CARTESIAN_POINT('Ctrl Pts',(3.66003813592315,1.95098496635821,-1.39398063668092)) ;
#157778=CARTESIAN_POINT('Ctrl Pts',(3.66320312645637,1.95301617633166,-1.39246240139399)) ;
#157779=CARTESIAN_POINT('Ctrl Pts',(3.66757373088802,1.9558211184692,-1.39036583718514)) ;
#157780=CARTESIAN_POINT('Ctrl Pts',(3.67181875309355,1.95875330073059,-1.38796612617098)) ;
#157781=CARTESIAN_POINT('Ctrl Pts',(3.67584388612499,1.96174615985042,-1.38526003578587)) ;
#157782=CARTESIAN_POINT('Ctrl Pts',(3.67661208162767,1.96231734616851,-1.38474357919985)) ;
#157783=CARTESIAN_POINT('Ctrl Pts',(3.67737237849352,1.96289065080917,-1.38421601587673)) ;
#157784=CARTESIAN_POINT('Ctrl Pts',(3.67812428214755,1.96346549105992,-1.38367739883589)) ;
#157785=CARTESIAN_POINT('Ctrl Pts',(3.6785349394885,1.96377944400799,-1.38338322944251)) ;
#157786=CARTESIAN_POINT('Ctrl Pts',(3.67894301851534,1.96409388168819,-1.38308575174331)) ;
#157787=CARTESIAN_POINT('Ctrl Pts',(3.67934840022277,1.96440871854256,-1.38278496939811)) ;
#157788=CARTESIAN_POINT('Ctrl Pts',(3.68198440184427,1.96645595067818,-1.38082912695353)) ;
#157789=CARTESIAN_POINT('Ctrl Pts',(3.68449751351864,1.96851545671307,-1.37873828347164)) ;
#157790=CARTESIAN_POINT('Ctrl Pts',(3.68685379133723,1.97055696562013,-1.37652085039877)) ;
#157791=CARTESIAN_POINT('Ctrl Pts',(3.68896164651385,1.97238323800784,-1.37453720155032)) ;
#157792=CARTESIAN_POINT('Ctrl Pts',(3.69104797813205,1.97419718002547,-1.37244243877984)) ;
#157793=CARTESIAN_POINT('Ctrl Pts',(3.69290978292492,1.97598569412168,-1.37024500103231)) ;
#157794=CARTESIAN_POINT('Ctrl Pts',(3.69362192319645,1.97666980070416,-1.36940448116677)) ;
#157795=CARTESIAN_POINT('Ctrl Pts',(3.6943016327186,1.97734979318971,-1.36854897561524)) ;
#157796=CARTESIAN_POINT('Ctrl Pts',(3.69493905694205,1.97802369895108,-1.36767908836304)) ;
#157797=CARTESIAN_POINT('Ctrl Pts',(3.69605143900785,1.9791997456958,-1.36616103030527)) ;
#157798=CARTESIAN_POINT('Ctrl Pts',(3.69703421735413,1.98035885502255,-1.3645986233173)) ;
#157799=CARTESIAN_POINT('Ctrl Pts',(3.6978475066491,1.98151165953424,-1.36295719153115)) ;
#157800=CARTESIAN_POINT('Ctrl Pts',(3.69841279947844,1.98231293913809,-1.36181628186433)) ;
#157801=CARTESIAN_POINT('Ctrl Pts',(3.69890310384956,1.98311438470601,-1.3606332480121)) ;
#157802=CARTESIAN_POINT('Ctrl Pts',(3.69929098301997,1.9839378326546,-1.35935810707453)) ;
#157803=CARTESIAN_POINT('Ctrl Pts',(3.69936193271527,1.98408845528532,-1.35912486211608)) ;
#157804=CARTESIAN_POINT('Ctrl Pts',(3.69942931950318,1.98423979370567,-1.35888851468589)) ;
#157805=CARTESIAN_POINT('Ctrl Pts',(3.69949277412725,1.98439195189923,-1.35864873028525)) ;
#157806=CARTESIAN_POINT('Ctrl Pts',(3.69967702385849,1.98483376534754,-1.35795248139834)) ;
#157807=CARTESIAN_POINT('Ctrl Pts',(3.69981936684304,1.98527475083258,-1.35723933425854)) ;
#157808=CARTESIAN_POINT('Ctrl Pts',(3.69990669142683,1.98570953653121,-1.35651584102814)) ;
#157809=CARTESIAN_POINT('Ctrl Pts',(3.69996666908332,1.98600816294479,-1.35601891992581)) ;
#157810=CARTESIAN_POINT('Ctrl Pts',(3.7,1.98630780592129,-1.35551049505453)) ;
#157811=CARTESIAN_POINT('Ctrl Pts',(3.7,1.98660254037844,-1.355)) ;
#157812=CARTESIAN_POINT('Origin',(3.7,1.9,-1.305)) ;
#157813=CARTESIAN_POINT('Origin',(10.2,1.9,-1.305)) ;
#157814=CARTESIAN_POINT('Origin',(3.7,1.9,-1.305)) ;
#157815=CARTESIAN_POINT('Origin',(10.1,1.9,-1.305)) ;
#157816=CARTESIAN_POINT('Origin',(10.1,1.9,-1.305)) ;
#157817=CARTESIAN_POINT('Origin',(3.7,2.1,1.305)) ;
#157818=CARTESIAN_POINT('',(3.7,1.98660254037844,1.355)) ;
#157819=CARTESIAN_POINT('Origin',(3.7,1.9,1.305)) ;
#157820=CARTESIAN_POINT('Ctrl Pts',(3.7,1.98660254037844,1.355)) ;
#157821=CARTESIAN_POINT('Ctrl Pts',(3.69999911718144,1.98567700534182,1.35660307370761)) ;
#157822=CARTESIAN_POINT('Ctrl Pts',(3.69968163901485,1.984703699336,1.35818199771545)) ;
#157823=CARTESIAN_POINT('Ctrl Pts',(3.69895427931585,1.98325895404995,1.36040554395919)) ;
#157824=CARTESIAN_POINT('Ctrl Pts',(3.69867650892745,1.98278649590681,1.36111390157608)) ;
#157825=CARTESIAN_POINT('Ctrl Pts',(3.69717970712967,1.9804354328423,1.36455908121567)) ;
#157826=CARTESIAN_POINT('Ctrl Pts',(3.69541014605544,1.97847095301992,1.36717587915573)) ;
#157827=CARTESIAN_POINT('Ctrl Pts',(3.69146029518774,1.97457001268155,1.37202655649097)) ;
#157828=CARTESIAN_POINT('Ctrl Pts',(3.68915436790411,1.97254004967205,1.37436779312348)) ;
#157829=CARTESIAN_POINT('Ctrl Pts',(3.68263623161791,1.96688850447179,1.38050008154324)) ;
#157830=CARTESIAN_POINT('Ctrl Pts',(3.67796661383157,1.96321337091311,1.38402074771694)) ;
#157831=CARTESIAN_POINT('Ctrl Pts',(3.67279117399676,1.95950210067475,1.38723765660546)) ;
#157832=CARTESIAN_POINT('Ctrl Pts',(3.67252519027993,1.95931231248682,1.38740119094185)) ;
#157833=CARTESIAN_POINT('Ctrl Pts',(3.6693311210617,1.95704457126181,1.38934379569321)) ;
#157834=CARTESIAN_POINT('Ctrl Pts',(3.66628216680077,1.95498580453519,1.39099038776091)) ;
#157835=CARTESIAN_POINT('Ctrl Pts',(3.65739884032376,1.94929644648107,1.39524097578772)) ;
#157836=CARTESIAN_POINT('Ctrl Pts',(3.65126071410426,1.94574201114262,1.39752886673119)) ;
#157837=CARTESIAN_POINT('Ctrl Pts',(3.64132315686417,1.94068746317945,1.40036203409875)) ;
#157838=CARTESIAN_POINT('Ctrl Pts',(3.63763353946351,1.93894751340588,1.40124340061523)) ;
#157839=CARTESIAN_POINT('Ctrl Pts',(3.62813871250318,1.93486114467727,1.40309560864189)) ;
#157840=CARTESIAN_POINT('Ctrl Pts',(3.62220485293006,1.93266004719379,1.4038846559585)) ;
#157841=CARTESIAN_POINT('Ctrl Pts',(3.61359543742329,1.93003167234286,1.40457978254887)) ;
#157842=CARTESIAN_POINT('Ctrl Pts',(3.61101642177011,1.92931331154714,1.40473301744682)) ;
#157843=CARTESIAN_POINT('Ctrl Pts',(3.60562851963646,1.92796119665945,1.40494674322732)) ;
#157844=CARTESIAN_POINT('Ctrl Pts',(3.60282089026139,1.92733781012841,1.405)) ;
#157845=CARTESIAN_POINT('Ctrl Pts',(3.6,1.92679491924311,1.405)) ;
#157846=CARTESIAN_POINT('Origin',(3.6,1.9,1.305)) ;
#157847=CARTESIAN_POINT('Origin',(3.7,1.9,1.305)) ;
#157848=CARTESIAN_POINT('Origin',(10.1,1.9,1.305)) ;
#157849=CARTESIAN_POINT('Origin',(10.1,1.9,1.305)) ;
#157850=CARTESIAN_POINT('Origin',(3.7,1.9,-1.305)) ;
#157851=CARTESIAN_POINT('Origin',(3.7,2.07320508075689,-1.405)) ;
#157852=CARTESIAN_POINT('Ctrl Pts',(3.60000659411846,1.92678349789492,-1.40500000086965)) ;
#157853=CARTESIAN_POINT('Ctrl Pts',(3.55,2.01339745962156,-1.40498681089333)) ;
#157854=CARTESIAN_POINT('Ctrl Pts',(3.55,2.01339745962156,-1.505)) ;
#157855=CARTESIAN_POINT('Ctrl Pts',(3.61192169694494,1.92907674455598,-1.4050005173338)) ;
#157856=CARTESIAN_POINT('Ctrl Pts',(3.55199190475227,2.01454315814788,-1.40100027733254)) ;
#157857=CARTESIAN_POINT('Ctrl Pts',(3.55795064586849,2.01798776715396,-1.5049956215502)) ;
#157858=CARTESIAN_POINT('Ctrl Pts',(3.62341406508537,1.93280912529606,-1.4040249033077)) ;
#157859=CARTESIAN_POINT('Ctrl Pts',(3.55602946562208,2.01072041298289,-1.3966898307659)) ;
#157860=CARTESIAN_POINT('Ctrl Pts',(3.56528619664567,2.02370799306987,-1.49863885617462)) ;
#157861=CARTESIAN_POINT('Ctrl Pts',(3.64447698054259,1.94188479470202,-1.39990697186185)) ;
#157862=CARTESIAN_POINT('Ctrl Pts',(3.56481337003729,2.00521659408682,-1.3881887406645)) ;
#157863=CARTESIAN_POINT('Ctrl Pts',(3.5778513142626,2.03528605841761,-1.48516115437406)) ;
#157864=CARTESIAN_POINT('Ctrl Pts',(3.6543438360007,1.94732274903781,-1.39671544038559)) ;
#157865=CARTESIAN_POINT('Ctrl Pts',(3.56964037752545,2.00254785926568,-1.38373800427671)) ;
#157866=CARTESIAN_POINT('Ctrl Pts',(3.58324299321411,2.04133793352501,-1.4770289695647)) ;
#157867=CARTESIAN_POINT('Ctrl Pts',(3.67209270719132,1.95869361548257,-1.3882138841634)) ;
#157868=CARTESIAN_POINT('Ctrl Pts',(3.57877657372944,1.99742369139614,-1.37460192490957)) ;
#157869=CARTESIAN_POINT('Ctrl Pts',(3.59173571364126,2.05270412132581,-1.4592738450102)) ;
#157870=CARTESIAN_POINT('Ctrl Pts',(3.68022412057907,1.96474917806412,-1.38281520426601)) ;
#157871=CARTESIAN_POINT('Ctrl Pts',(3.58322866085249,1.9947527117803,-1.36977362629675)) ;
#157872=CARTESIAN_POINT('Ctrl Pts',(3.59492343714209,2.05814036366738,-1.449399963424)) ;
#157873=CARTESIAN_POINT('Ctrl Pts',(3.693683649568,1.97632149420531,-1.37024886281709)) ;
#157874=CARTESIAN_POINT('Ctrl Pts',(3.59172551342568,1.98925228662578,-1.36099928071625)) ;
#157875=CARTESIAN_POINT('Ctrl Pts',(3.59903094645825,2.06720241143976,-1.42834396451164)) ;
#157876=CARTESIAN_POINT('Ctrl Pts',(3.70000914724963,1.98195813651218,-1.36304434431452)) ;
#157877=CARTESIAN_POINT('Ctrl Pts',(3.59596384548938,1.98543049140365,-1.35700954448628)) ;
#157878=CARTESIAN_POINT('Ctrl Pts',(3.6,2.07088547209221,-1.41705281147587)) ;
#157879=CARTESIAN_POINT('Ctrl Pts',(3.70001318823691,1.98660254113158,-1.35500000043482)) ;
#157880=CARTESIAN_POINT('Ctrl Pts',(3.6,1.98659111827701,-1.35499340544666)) ;
#157881=CARTESIAN_POINT('Ctrl Pts',(3.6,2.07320508075689,-1.405)) ;
#157882=CARTESIAN_POINT('Origin',(3.6,1.92679491924311,-1.505)) ;
#157883=CARTESIAN_POINT('Origin',(3.5,2.1,-1.505)) ;
#157884=CARTESIAN_POINT('Origin',(3.7,1.9,1.305)) ;
#157885=CARTESIAN_POINT('Origin',(3.7,2.07320508075689,1.405)) ;
#157886=CARTESIAN_POINT('Ctrl Pts',(3.70000000000001,1.98660254037844,1.355)) ;
#157887=CARTESIAN_POINT('Ctrl Pts',(3.59998681089333,1.98660254037844,1.355)) ;
#157888=CARTESIAN_POINT('Ctrl Pts',(3.60000000086965,2.07321650210508,1.40500659411846)) ;
#157889=CARTESIAN_POINT('Ctrl Pts',(3.69999562155021,1.98201223284605,1.36295064586848)) ;
#157890=CARTESIAN_POINT('Ctrl Pts',(3.59600027733256,1.98545684185208,1.35699190475226)) ;
#157891=CARTESIAN_POINT('Ctrl Pts',(3.60000051733381,2.07092325544402,1.41692169694494)) ;
#157892=CARTESIAN_POINT('Ctrl Pts',(3.69363885617462,1.97629200693013,1.37028619664567)) ;
#157893=CARTESIAN_POINT('Ctrl Pts',(3.5916898307659,1.98927958701711,1.36102946562208)) ;
#157894=CARTESIAN_POINT('Ctrl Pts',(3.59902490330771,2.06719087470394,1.42841406508537)) ;
#157895=CARTESIAN_POINT('Ctrl Pts',(3.68016115437407,1.9647139415824,1.3828513142626)) ;
#157896=CARTESIAN_POINT('Ctrl Pts',(3.58318874066451,1.99478340591318,1.36981337003728)) ;
#157897=CARTESIAN_POINT('Ctrl Pts',(3.59490697186185,2.05811520529798,1.44947698054259)) ;
#157898=CARTESIAN_POINT('Ctrl Pts',(3.67202896956471,1.95866206647499,1.38824299321411)) ;
#157899=CARTESIAN_POINT('Ctrl Pts',(3.57873800427672,1.99745214073432,1.37464037752545)) ;
#157900=CARTESIAN_POINT('Ctrl Pts',(3.59171544038559,2.05267725096219,1.45934383600069)) ;
#157901=CARTESIAN_POINT('Ctrl Pts',(3.6542738450102,1.94729587867419,1.39673571364126)) ;
#157902=CARTESIAN_POINT('Ctrl Pts',(3.56960192490957,2.00257630860386,1.38377657372944)) ;
#157903=CARTESIAN_POINT('Ctrl Pts',(3.5832138841634,2.04130638451743,1.47709270719132)) ;
#157904=CARTESIAN_POINT('Ctrl Pts',(3.644399963424,1.94185963633262,1.39992343714209)) ;
#157905=CARTESIAN_POINT('Ctrl Pts',(3.56477362629675,2.0052472882197,1.38822866085248)) ;
#157906=CARTESIAN_POINT('Ctrl Pts',(3.57781520426602,2.03525082193588,1.48522412057907)) ;
#157907=CARTESIAN_POINT('Ctrl Pts',(3.62334396451164,1.93279758856024,1.40403094645824)) ;
#157908=CARTESIAN_POINT('Ctrl Pts',(3.55599928071625,2.01074771337423,1.39672551342568)) ;
#157909=CARTESIAN_POINT('Ctrl Pts',(3.5652488628171,2.02367850579469,1.498683649568)) ;
#157910=CARTESIAN_POINT('Ctrl Pts',(3.61205281147587,1.92911452790779,1.405)) ;
#157911=CARTESIAN_POINT('Ctrl Pts',(3.55200954448627,2.01456950859638,1.40096384548938)) ;
#157912=CARTESIAN_POINT('Ctrl Pts',(3.55804434431452,2.01804186348783,1.50500914724966)) ;
#157913=CARTESIAN_POINT('Ctrl Pts',(3.6,1.92679491924311,1.405)) ;
#157914=CARTESIAN_POINT('Ctrl Pts',(3.54999340544667,2.01340888172299,1.405)) ;
#157915=CARTESIAN_POINT('Ctrl Pts',(3.55000000043483,2.01339745886842,1.50501318823691)) ;
#157916=CARTESIAN_POINT('Origin',(3.6,1.92679491924311,1.505)) ;
#157917=CARTESIAN_POINT('Origin',(3.5,2.1,1.505)) ;
#157918=CARTESIAN_POINT('Origin',(-5.15,-5.05,-35.89)) ;
#157919=CARTESIAN_POINT('',(-5.8,-1.29142135623731,-35.89)) ;
#157920=CARTESIAN_POINT('',(-5.8,-5.42192235935956,-35.89)) ;
#157921=CARTESIAN_POINT('',(-5.8,-5.55,-35.89)) ;
#157922=CARTESIAN_POINT('',(-5.17275707706435,-5.26511162862565,-35.89)) ;
#157923=CARTESIAN_POINT('',(-5.10072415073893,-5.24710339704429,-35.89)) ;
#157924=CARTESIAN_POINT('',(-5.17275707706435,-1.91866427917295,-35.89)) ;
#157925=CARTESIAN_POINT('',(-5.17275707706435,-1.8,-35.89)) ;
#157926=CARTESIAN_POINT('',(-3.59571067811865,-3.49571067811865,-35.89)) ;
#157927=CARTESIAN_POINT('Origin',(-3.9,-5.05,-35.29)) ;
#157928=CARTESIAN_POINT('',(-5.12948397030587,-1.91866427917295,-35.8801523057468)) ;
#157929=CARTESIAN_POINT('',(-5.12948397030587,-5.26511162862565,-35.8801523057468)) ;
#157930=CARTESIAN_POINT('',(-5.12948397030587,-5.3625,-35.8801523057468)) ;
#157931=CARTESIAN_POINT('',(-3.9,-4.95774063604919,-35.29)) ;
#157932=CARTESIAN_POINT('',(-3.91783961713025,-4.96220054033175,-35.2985630162225)) ;
#157933=CARTESIAN_POINT('',(-3.9,-3.14814824947882,-35.29)) ;
#157934=CARTESIAN_POINT('',(-3.9,-5.05,-35.29)) ;
#157935=CARTESIAN_POINT('',(-3.04730463122257,-4.00084361825625,-34.8807062229868)) ;
#157936=CARTESIAN_POINT('Origin',(-3.9,-5.05,-33.29)) ;
#157937=CARTESIAN_POINT('',(-3.9,-5.05,-33.3892816869892)) ;
#157938=CARTESIAN_POINT('',(-3.9,-5.05,-35.1907183130108)) ;
#157939=CARTESIAN_POINT('',(-3.9,-5.05,-33.29)) ;
#157940=CARTESIAN_POINT('',(-3.9,-4.95774063604919,-33.29)) ;
#157941=CARTESIAN_POINT('Origin',(-3.9,-4.94692235935959,-33.4009233969909)) ;
#157942=CARTESIAN_POINT('',(-3.9,-3.14814824947882,-33.29)) ;
#157943=CARTESIAN_POINT('',(-3.9,-5.05,-33.29)) ;
#157944=CARTESIAN_POINT('',(-3.9,-3.05,-33.3669822714939)) ;
#157945=CARTESIAN_POINT('Origin',(-3.89999999999999,-3.1914213562364,-33.4009233969901)) ;
#157946=CARTESIAN_POINT('',(-3.9,-3.05,-35.2130177285061)) ;
#157947=CARTESIAN_POINT('',(-3.9,-3.05,-33.29)) ;
#157948=CARTESIAN_POINT('Origin',(-3.89999999999999,-3.19142135623724,-35.1790766030092)) ;
#157949=CARTESIAN_POINT('Origin',(-3.89999999999999,-4.94692235935948,-35.1790766030091)) ;
#157950=CARTESIAN_POINT('Origin',(-5.15,-5.05,-32.69)) ;
#157951=CARTESIAN_POINT('',(-5.12948397030588,-5.26511162862565,-32.6998476942532)) ;
#157952=CARTESIAN_POINT('',(-5.10741344341225,-5.25959399690224,-32.7104415471621)) ;
#157953=CARTESIAN_POINT('',(-5.12948397030588,-1.91866427917294,-32.6998476942532)) ;
#157954=CARTESIAN_POINT('',(-5.12948397030588,-1.79999999999999,-32.6998476942532)) ;
#157955=CARTESIAN_POINT('',(-3.73686704155256,-3.31128120792626,-33.3683038200548)) ;
#157956=CARTESIAN_POINT('Origin',(-5.9,-5.05,-32.69)) ;
#157957=CARTESIAN_POINT('',(-5.8,-5.42192235935956,-32.69)) ;
#157958=CARTESIAN_POINT('',(-5.8,-1.29142135623731,-32.69)) ;
#157959=CARTESIAN_POINT('',(-5.8,-1.04999999999999,-32.69)) ;
#157960=CARTESIAN_POINT('',(-5.17275707706436,-1.91866427917294,-32.69)) ;
#157961=CARTESIAN_POINT('',(-3.97071067811865,-3.12071067811865,-32.69)) ;
#157962=CARTESIAN_POINT('',(-5.17275707706436,-5.26511162862565,-32.69)) ;
#157963=CARTESIAN_POINT('',(-5.17275707706436,-5.3625,-32.69)) ;
#157964=CARTESIAN_POINT('',(-5.8066065036801,-5.42357398527959,-32.69)) ;
#157965=CARTESIAN_POINT('Origin',(-5.15,-5.05,-32.08)) ;
#157966=CARTESIAN_POINT('',(-5.8,-1.29142135623731,-32.08)) ;
#157967=CARTESIAN_POINT('',(-5.8,-5.42192235935956,-32.08)) ;
#157968=CARTESIAN_POINT('',(-5.8,-5.55,-32.08)) ;
#157969=CARTESIAN_POINT('',(-5.17275707706435,-5.26511162862565,-32.08)) ;
#157970=CARTESIAN_POINT('',(-5.10072415073893,-5.24710339704429,-32.08)) ;
#157971=CARTESIAN_POINT('',(-5.17275707706435,-1.91866427917295,-32.08)) ;
#157972=CARTESIAN_POINT('',(-5.17275707706435,-1.8,-32.08)) ;
#157973=CARTESIAN_POINT('',(-3.59571067811865,-3.49571067811865,-32.08)) ;
#157974=CARTESIAN_POINT('Origin',(-3.9,-5.05,-31.48)) ;
#157975=CARTESIAN_POINT('',(-5.12948397030587,-1.91866427917295,-32.0701523057468)) ;
#157976=CARTESIAN_POINT('',(-5.12948397030587,-5.26511162862565,-32.0701523057468)) ;
#157977=CARTESIAN_POINT('',(-5.12948397030587,-5.3625,-32.0701523057468)) ;
#157978=CARTESIAN_POINT('',(-3.9,-4.95774063604919,-31.48)) ;
#157979=CARTESIAN_POINT('',(-3.91783961713025,-4.96220054033175,-31.4885630162225)) ;
#157980=CARTESIAN_POINT('',(-3.9,-3.14814824947882,-31.48)) ;
#157981=CARTESIAN_POINT('',(-3.9,-5.05,-31.48)) ;
#157982=CARTESIAN_POINT('',(-3.04730463122257,-4.00084361825625,-31.0707062229868)) ;
#157983=CARTESIAN_POINT('Origin',(-3.9,-5.05,-29.48)) ;
#157984=CARTESIAN_POINT('',(-3.9,-5.05,-29.5792816869892)) ;
#157985=CARTESIAN_POINT('',(-3.9,-5.05,-31.3807183130108)) ;
#157986=CARTESIAN_POINT('',(-3.9,-5.05,-29.48)) ;
#157987=CARTESIAN_POINT('',(-3.9,-4.95774063604918,-29.48)) ;
#157988=CARTESIAN_POINT('Origin',(-3.9,-4.94692235935937,-29.5909233969911)) ;
#157989=CARTESIAN_POINT('',(-3.9,-3.14814824947882,-29.48)) ;
#157990=CARTESIAN_POINT('',(-3.9,-5.05,-29.48)) ;
#157991=CARTESIAN_POINT('',(-3.9,-3.05,-29.5569822714939)) ;
#157992=CARTESIAN_POINT('Origin',(-3.9,-3.19142135623589,-29.5909233969898)) ;
#157993=CARTESIAN_POINT('',(-3.9,-3.05,-31.4030177285061)) ;
#157994=CARTESIAN_POINT('',(-3.9,-3.05,-29.48)) ;
#157995=CARTESIAN_POINT('Origin',(-3.89999999999999,-3.19142135623673,-31.3690766030095)) ;
#157996=CARTESIAN_POINT('Origin',(-3.89999999999999,-4.94692235935935,-31.3690766030089)) ;
#157997=CARTESIAN_POINT('Origin',(-5.15,-5.05,-28.88)) ;
#157998=CARTESIAN_POINT('',(-5.12948397030589,-5.26511162862565,-28.8898476942532)) ;
#157999=CARTESIAN_POINT('',(-5.10741344341225,-5.25959399690224,-28.9004415471621)) ;
#158000=CARTESIAN_POINT('',(-5.12948397030589,-1.91866427917294,-28.8898476942532)) ;
#158001=CARTESIAN_POINT('',(-5.12948397030589,-1.79999999999999,-28.8898476942532)) ;
#158002=CARTESIAN_POINT('',(-3.73686704155256,-3.31128120792626,-29.5583038200548)) ;
#158003=CARTESIAN_POINT('Origin',(-5.9,-5.05,-28.88)) ;
#158004=CARTESIAN_POINT('',(-5.8,-5.42192235935956,-28.88)) ;
#158005=CARTESIAN_POINT('',(-5.8,-1.29142135623731,-28.88)) ;
#158006=CARTESIAN_POINT('',(-5.8,-1.04999999999999,-28.88)) ;
#158007=CARTESIAN_POINT('',(-5.17275707706436,-1.91866427917294,-28.88)) ;
#158008=CARTESIAN_POINT('',(-3.97071067811865,-3.12071067811865,-28.88)) ;
#158009=CARTESIAN_POINT('',(-5.17275707706436,-5.26511162862565,-28.88)) ;
#158010=CARTESIAN_POINT('',(-5.17275707706436,-5.3625,-28.88)) ;
#158011=CARTESIAN_POINT('',(-5.8066065036801,-5.42357398527959,-28.88)) ;
#158012=CARTESIAN_POINT('Origin',(-5.15,-5.05,-28.27)) ;
#158013=CARTESIAN_POINT('',(-5.8,-1.29142135623731,-28.27)) ;
#158014=CARTESIAN_POINT('',(-5.8,-5.42192235935956,-28.27)) ;
#158015=CARTESIAN_POINT('',(-5.8,-5.55,-28.27)) ;
#158016=CARTESIAN_POINT('',(-5.17275707706436,-5.26511162862565,-28.27)) ;
#158017=CARTESIAN_POINT('',(-5.10072415073893,-5.24710339704429,-28.27)) ;
#158018=CARTESIAN_POINT('',(-5.17275707706436,-1.91866427917293,-28.27)) ;
#158019=CARTESIAN_POINT('',(-5.17275707706436,-1.79999999999999,-28.27)) ;
#158020=CARTESIAN_POINT('',(-3.59571067811865,-3.49571067811865,-28.27)) ;
#158021=CARTESIAN_POINT('Origin',(-3.9,-5.05,-27.67)) ;
#158022=CARTESIAN_POINT('',(-5.12948397030589,-1.91866427917293,-28.2601523057468)) ;
#158023=CARTESIAN_POINT('',(-5.12948397030589,-5.26511162862565,-28.2601523057468)) ;
#158024=CARTESIAN_POINT('',(-5.12948397030589,-5.3625,-28.2601523057468)) ;
#158025=CARTESIAN_POINT('',(-3.9,-4.95774063604919,-27.67)) ;
#158026=CARTESIAN_POINT('',(-3.91783961713025,-4.96220054033175,-27.6785630162225)) ;
#158027=CARTESIAN_POINT('',(-3.9,-3.14814824947882,-27.67)) ;
#158028=CARTESIAN_POINT('',(-3.9,-5.05,-27.67)) ;
#158029=CARTESIAN_POINT('',(-3.04730463122257,-4.00084361825625,-27.2607062229868)) ;
#158030=CARTESIAN_POINT('Origin',(-3.9,-5.05,-25.67)) ;
#158031=CARTESIAN_POINT('',(-3.9,-5.05,-25.7692816869891)) ;
#158032=CARTESIAN_POINT('',(-3.9,-5.05,-27.5707183130108)) ;
#158033=CARTESIAN_POINT('',(-3.9,-5.05,-25.67)) ;
#158034=CARTESIAN_POINT('',(-3.9,-4.95774063604918,-25.67)) ;
#158035=CARTESIAN_POINT('Origin',(-3.9,-4.94692235935943,-25.780923396991)) ;
#158036=CARTESIAN_POINT('',(-3.9,-3.14814824947882,-25.67)) ;
#158037=CARTESIAN_POINT('',(-3.9,-5.05,-25.67)) ;
#158038=CARTESIAN_POINT('',(-3.9,-3.05,-25.7469822714939)) ;
#158039=CARTESIAN_POINT('Origin',(-3.9,-3.1914213562362,-25.7809233969901)) ;
#158040=CARTESIAN_POINT('',(-3.9,-3.05,-27.5930177285061)) ;
#158041=CARTESIAN_POINT('',(-3.9,-3.05,-25.67)) ;
#158042=CARTESIAN_POINT('Origin',(-3.9,-3.19142135623739,-27.559076603009)) ;
#158043=CARTESIAN_POINT('Origin',(-3.9,-4.94692235935962,-27.5590766030092)) ;
#158044=CARTESIAN_POINT('Origin',(-5.15,-5.05,-25.07)) ;
#158045=CARTESIAN_POINT('',(-5.12948397030589,-5.26511162862565,-25.0798476942532)) ;
#158046=CARTESIAN_POINT('',(-5.10741344341225,-5.25959399690224,-25.0904415471621)) ;
#158047=CARTESIAN_POINT('',(-5.12948397030589,-1.91866427917294,-25.0798476942532)) ;
#158048=CARTESIAN_POINT('',(-5.12948397030589,-1.79999999999999,-25.0798476942532)) ;
#158049=CARTESIAN_POINT('',(-3.73686704155256,-3.31128120792626,-25.7483038200548)) ;
#158050=CARTESIAN_POINT('Origin',(-5.9,-5.05,-25.07)) ;
#158051=CARTESIAN_POINT('',(-5.8,-5.42192235935956,-25.07)) ;
#158052=CARTESIAN_POINT('',(-5.8,-1.29142135623731,-25.07)) ;
#158053=CARTESIAN_POINT('',(-5.8,-1.04999999999999,-25.07)) ;
#158054=CARTESIAN_POINT('',(-5.17275707706436,-1.91866427917294,-25.07)) ;
#158055=CARTESIAN_POINT('',(-3.97071067811865,-3.12071067811865,-25.07)) ;
#158056=CARTESIAN_POINT('',(-5.17275707706436,-5.26511162862565,-25.07)) ;
#158057=CARTESIAN_POINT('',(-5.17275707706436,-5.3625,-25.07)) ;
#158058=CARTESIAN_POINT('',(-5.8066065036801,-5.42357398527959,-25.07)) ;
#158059=CARTESIAN_POINT('Origin',(-5.15,-5.05,-24.46)) ;
#158060=CARTESIAN_POINT('',(-5.8,-1.29142135623731,-24.46)) ;
#158061=CARTESIAN_POINT('',(-5.8,-5.42192235935956,-24.46)) ;
#158062=CARTESIAN_POINT('',(-5.8,-5.55,-24.46)) ;
#158063=CARTESIAN_POINT('',(-5.17275707706436,-5.26511162862565,-24.46)) ;
#158064=CARTESIAN_POINT('',(-5.10072415073893,-5.24710339704429,-24.46)) ;
#158065=CARTESIAN_POINT('',(-5.17275707706436,-1.91866427917293,-24.46)) ;
#158066=CARTESIAN_POINT('',(-5.17275707706436,-1.79999999999999,-24.46)) ;
#158067=CARTESIAN_POINT('',(-3.59571067811865,-3.49571067811865,-24.46)) ;
#158068=CARTESIAN_POINT('Origin',(-3.9,-5.05,-23.86)) ;
#158069=CARTESIAN_POINT('',(-5.12948397030589,-1.91866427917293,-24.4501523057468)) ;
#158070=CARTESIAN_POINT('',(-5.12948397030589,-5.26511162862565,-24.4501523057468)) ;
#158071=CARTESIAN_POINT('',(-5.12948397030589,-5.3625,-24.4501523057468)) ;
#158072=CARTESIAN_POINT('',(-3.9,-4.95774063604919,-23.86)) ;
#158073=CARTESIAN_POINT('',(-3.91783961713025,-4.96220054033175,-23.8685630162225)) ;
#158074=CARTESIAN_POINT('',(-3.9,-3.14814824947882,-23.86)) ;
#158075=CARTESIAN_POINT('',(-3.9,-5.05,-23.86)) ;
#158076=CARTESIAN_POINT('',(-3.04730463122257,-4.00084361825625,-23.4507062229868)) ;
#158077=CARTESIAN_POINT('Origin',(-3.9,-5.05,-21.86)) ;
#158078=CARTESIAN_POINT('',(-3.9,-5.05,-21.9592816869892)) ;
#158079=CARTESIAN_POINT('',(-3.9,-5.05,-23.7607183130108)) ;
#158080=CARTESIAN_POINT('',(-3.9,-5.05,-21.86)) ;
#158081=CARTESIAN_POINT('',(-3.9,-4.95774063604918,-21.86)) ;
#158082=CARTESIAN_POINT('Origin',(-3.9,-4.94692235935955,-21.9709233969909)) ;
#158083=CARTESIAN_POINT('',(-3.9,-3.14814824947882,-21.86)) ;
#158084=CARTESIAN_POINT('',(-3.9,-5.05,-21.86)) ;
#158085=CARTESIAN_POINT('',(-3.9,-3.05,-21.9369822714939)) ;
#158086=CARTESIAN_POINT('Origin',(-3.9,-3.19142135623605,-21.97092339699)) ;
#158087=CARTESIAN_POINT('',(-3.9,-3.05,-23.7830177285061)) ;
#158088=CARTESIAN_POINT('',(-3.9,-3.05,-21.86)) ;
#158089=CARTESIAN_POINT('Origin',(-3.9,-3.19142135623773,-23.7490766030088)) ;
#158090=CARTESIAN_POINT('Origin',(-3.9,-4.94692235935942,-23.749076603009)) ;
#158091=CARTESIAN_POINT('Origin',(-5.15,-5.05,-21.26)) ;
#158092=CARTESIAN_POINT('',(-5.12948397030589,-5.26511162862565,-21.2698476942532)) ;
#158093=CARTESIAN_POINT('',(-5.10741344341225,-5.25959399690224,-21.2804415471621)) ;
#158094=CARTESIAN_POINT('',(-5.12948397030589,-1.91866427917294,-21.2698476942532)) ;
#158095=CARTESIAN_POINT('',(-5.12948397030589,-1.79999999999999,-21.2698476942532)) ;
#158096=CARTESIAN_POINT('',(-3.73686704155256,-3.31128120792626,-21.9383038200548)) ;
#158097=CARTESIAN_POINT('Origin',(-5.9,-5.05,-21.26)) ;
#158098=CARTESIAN_POINT('',(-5.8,-5.42192235935956,-21.26)) ;
#158099=CARTESIAN_POINT('',(-5.8,-1.29142135623731,-21.26)) ;
#158100=CARTESIAN_POINT('',(-5.8,-1.04999999999999,-21.26)) ;
#158101=CARTESIAN_POINT('',(-5.17275707706436,-1.91866427917294,-21.26)) ;
#158102=CARTESIAN_POINT('',(-3.97071067811865,-3.12071067811865,-21.26)) ;
#158103=CARTESIAN_POINT('',(-5.17275707706436,-5.26511162862565,-21.26)) ;
#158104=CARTESIAN_POINT('',(-5.17275707706436,-5.3625,-21.26)) ;
#158105=CARTESIAN_POINT('',(-5.8066065036801,-5.42357398527959,-21.26)) ;
#158106=CARTESIAN_POINT('Origin',(-5.15,-5.05,-20.65)) ;
#158107=CARTESIAN_POINT('',(-5.8,-1.29142135623731,-20.65)) ;
#158108=CARTESIAN_POINT('',(-5.8,-5.42192235935956,-20.65)) ;
#158109=CARTESIAN_POINT('',(-5.8,-5.55,-20.65)) ;
#158110=CARTESIAN_POINT('',(-5.17275707706436,-5.26511162862565,-20.65)) ;
#158111=CARTESIAN_POINT('',(-5.10072415073893,-5.24710339704429,-20.65)) ;
#158112=CARTESIAN_POINT('',(-5.17275707706436,-1.91866427917293,-20.65)) ;
#158113=CARTESIAN_POINT('',(-5.17275707706436,-1.79999999999999,-20.65)) ;
#158114=CARTESIAN_POINT('',(-3.59571067811865,-3.49571067811865,-20.65)) ;
#158115=CARTESIAN_POINT('Origin',(-3.9,-5.05,-20.05)) ;
#158116=CARTESIAN_POINT('',(-5.12948397030589,-1.91866427917293,-20.6401523057468)) ;
#158117=CARTESIAN_POINT('',(-5.12948397030589,-5.26511162862565,-20.6401523057468)) ;
#158118=CARTESIAN_POINT('',(-5.12948397030589,-5.3625,-20.6401523057468)) ;
#158119=CARTESIAN_POINT('',(-3.9,-4.95774063604919,-20.05)) ;
#158120=CARTESIAN_POINT('',(-3.91783961713025,-4.96220054033175,-20.0585630162225)) ;
#158121=CARTESIAN_POINT('',(-3.9,-3.14814824947882,-20.05)) ;
#158122=CARTESIAN_POINT('',(-3.9,-5.05,-20.05)) ;
#158123=CARTESIAN_POINT('',(-3.04730463122257,-4.00084361825625,-19.6407062229868)) ;
#158124=CARTESIAN_POINT('Origin',(-3.9,-5.05,-18.05)) ;
#158125=CARTESIAN_POINT('',(-3.9,-5.05,-18.1492816869892)) ;
#158126=CARTESIAN_POINT('',(-3.9,-5.05,-19.9507183130109)) ;
#158127=CARTESIAN_POINT('',(-3.9,-5.05,-18.05)) ;
#158128=CARTESIAN_POINT('',(-3.9,-4.95774063604918,-18.05)) ;
#158129=CARTESIAN_POINT('Origin',(-3.9,-4.94692235935955,-18.1609233969909)) ;
#158130=CARTESIAN_POINT('',(-3.9,-3.14814824947882,-18.05)) ;
#158131=CARTESIAN_POINT('',(-3.9,-5.05,-18.05)) ;
#158132=CARTESIAN_POINT('',(-3.9,-3.05,-18.1269822714939)) ;
#158133=CARTESIAN_POINT('Origin',(-3.9,-3.19142135623647,-18.1609233969903)) ;
#158134=CARTESIAN_POINT('',(-3.9,-3.05,-19.9730177285061)) ;
#158135=CARTESIAN_POINT('',(-3.9,-3.05,-18.05)) ;
#158136=CARTESIAN_POINT('Origin',(-3.9,-3.19142135623653,-19.9390766030097)) ;
#158137=CARTESIAN_POINT('Origin',(-3.89999999999999,-4.9469223593596,-19.9390766030092)) ;
#158138=CARTESIAN_POINT('Origin',(-5.15,-5.05,-17.45)) ;
#158139=CARTESIAN_POINT('',(-5.12948397030589,-5.26511162862565,-17.4598476942532)) ;
#158140=CARTESIAN_POINT('',(-5.10741344341225,-5.25959399690224,-17.4704415471621)) ;
#158141=CARTESIAN_POINT('',(-5.12948397030589,-1.91866427917294,-17.4598476942532)) ;
#158142=CARTESIAN_POINT('',(-5.12948397030589,-1.79999999999999,-17.4598476942532)) ;
#158143=CARTESIAN_POINT('',(-3.73686704155256,-3.31128120792626,-18.1283038200548)) ;
#158144=CARTESIAN_POINT('Origin',(-5.9,-5.05,-17.45)) ;
#158145=CARTESIAN_POINT('',(-5.8,-5.42192235935956,-17.45)) ;
#158146=CARTESIAN_POINT('',(-5.8,-1.29142135623731,-17.45)) ;
#158147=CARTESIAN_POINT('',(-5.8,-1.04999999999999,-17.45)) ;
#158148=CARTESIAN_POINT('',(-5.17275707706436,-1.91866427917294,-17.45)) ;
#158149=CARTESIAN_POINT('',(-3.97071067811865,-3.12071067811865,-17.45)) ;
#158150=CARTESIAN_POINT('',(-5.17275707706436,-5.26511162862565,-17.45)) ;
#158151=CARTESIAN_POINT('',(-5.17275707706436,-5.3625,-17.45)) ;
#158152=CARTESIAN_POINT('',(-5.8066065036801,-5.42357398527959,-17.45)) ;
#158153=CARTESIAN_POINT('Origin',(-5.15,-5.05,-16.84)) ;
#158154=CARTESIAN_POINT('',(-5.8,-1.29142135623731,-16.84)) ;
#158155=CARTESIAN_POINT('',(-5.8,-5.42192235935956,-16.84)) ;
#158156=CARTESIAN_POINT('',(-5.8,-5.55,-16.84)) ;
#158157=CARTESIAN_POINT('',(-5.17275707706436,-5.26511162862565,-16.84)) ;
#158158=CARTESIAN_POINT('',(-5.10072415073893,-5.24710339704429,-16.84)) ;
#158159=CARTESIAN_POINT('',(-5.17275707706436,-1.91866427917293,-16.84)) ;
#158160=CARTESIAN_POINT('',(-5.17275707706436,-1.79999999999999,-16.84)) ;
#158161=CARTESIAN_POINT('',(-3.59571067811865,-3.49571067811865,-16.84)) ;
#158162=CARTESIAN_POINT('Origin',(-3.9,-5.05,-16.24)) ;
#158163=CARTESIAN_POINT('',(-5.12948397030589,-1.91866427917293,-16.8301523057468)) ;
#158164=CARTESIAN_POINT('',(-5.12948397030589,-5.26511162862565,-16.8301523057468)) ;
#158165=CARTESIAN_POINT('',(-5.12948397030589,-5.3625,-16.8301523057468)) ;
#158166=CARTESIAN_POINT('',(-3.9,-4.95774063604919,-16.24)) ;
#158167=CARTESIAN_POINT('',(-3.91783961713025,-4.96220054033175,-16.2485630162225)) ;
#158168=CARTESIAN_POINT('',(-3.9,-3.14814824947882,-16.24)) ;
#158169=CARTESIAN_POINT('',(-3.9,-5.05,-16.24)) ;
#158170=CARTESIAN_POINT('',(-3.04730463122257,-4.00084361825625,-15.8307062229868)) ;
#158171=CARTESIAN_POINT('Origin',(-3.9,-5.05,-14.24)) ;
#158172=CARTESIAN_POINT('',(-3.9,-5.05,-14.3392816869892)) ;
#158173=CARTESIAN_POINT('',(-3.9,-5.05,-16.1407183130109)) ;
#158174=CARTESIAN_POINT('',(-3.9,-5.05,-14.24)) ;
#158175=CARTESIAN_POINT('',(-3.9,-4.95774063604919,-14.24)) ;
#158176=CARTESIAN_POINT('Origin',(-3.9,-4.94692235935948,-14.3509233969909)) ;
#158177=CARTESIAN_POINT('',(-3.9,-3.14814824947882,-14.24)) ;
#158178=CARTESIAN_POINT('',(-3.9,-5.05,-14.24)) ;
#158179=CARTESIAN_POINT('',(-3.9,-3.05,-14.3169822714939)) ;
#158180=CARTESIAN_POINT('Origin',(-3.9,-3.19142135623778,-14.3509233969912)) ;
#158181=CARTESIAN_POINT('',(-3.9,-3.05,-16.1630177285061)) ;
#158182=CARTESIAN_POINT('',(-3.9,-3.05,-14.24)) ;
#158183=CARTESIAN_POINT('Origin',(-3.9,-3.19142135623662,-16.1290766030096)) ;
#158184=CARTESIAN_POINT('Origin',(-3.89999999999999,-4.9469223593597,-16.1290766030092)) ;
#158185=CARTESIAN_POINT('Origin',(-5.15,-5.05,-13.64)) ;
#158186=CARTESIAN_POINT('',(-5.12948397030589,-5.26511162862565,-13.6498476942532)) ;
#158187=CARTESIAN_POINT('',(-5.10741344341225,-5.25959399690224,-13.6604415471621)) ;
#158188=CARTESIAN_POINT('',(-5.12948397030589,-1.91866427917294,-13.6498476942532)) ;
#158189=CARTESIAN_POINT('',(-5.12948397030589,-1.79999999999999,-13.6498476942532)) ;
#158190=CARTESIAN_POINT('',(-3.73686704155256,-3.31128120792626,-14.3183038200548)) ;
#158191=CARTESIAN_POINT('Origin',(-5.9,-5.05,-13.64)) ;
#158192=CARTESIAN_POINT('',(-5.8,-5.42192235935956,-13.64)) ;
#158193=CARTESIAN_POINT('',(-5.8,-1.29142135623731,-13.64)) ;
#158194=CARTESIAN_POINT('',(-5.8,-1.04999999999999,-13.64)) ;
#158195=CARTESIAN_POINT('',(-5.17275707706436,-1.91866427917294,-13.64)) ;
#158196=CARTESIAN_POINT('',(-3.97071067811865,-3.12071067811865,-13.64)) ;
#158197=CARTESIAN_POINT('',(-5.17275707706436,-5.26511162862565,-13.64)) ;
#158198=CARTESIAN_POINT('',(-5.17275707706436,-5.3625,-13.64)) ;
#158199=CARTESIAN_POINT('',(-5.8066065036801,-5.42357398527959,-13.64)) ;
#158200=CARTESIAN_POINT('Origin',(-5.15,-5.05,-13.03)) ;
#158201=CARTESIAN_POINT('',(-5.8,-1.29142135623731,-13.03)) ;
#158202=CARTESIAN_POINT('',(-5.8,-5.42192235935956,-13.03)) ;
#158203=CARTESIAN_POINT('',(-5.8,-5.55,-13.03)) ;
#158204=CARTESIAN_POINT('',(-5.17275707706436,-5.26511162862565,-13.03)) ;
#158205=CARTESIAN_POINT('',(-5.10072415073893,-5.24710339704429,-13.03)) ;
#158206=CARTESIAN_POINT('',(-5.17275707706436,-1.91866427917293,-13.03)) ;
#158207=CARTESIAN_POINT('',(-5.17275707706436,-1.79999999999999,-13.03)) ;
#158208=CARTESIAN_POINT('',(-3.59571067811865,-3.49571067811865,-13.03)) ;
#158209=CARTESIAN_POINT('Origin',(-3.9,-5.05,-12.43)) ;
#158210=CARTESIAN_POINT('',(-5.12948397030589,-1.91866427917294,-13.0201523057468)) ;
#158211=CARTESIAN_POINT('',(-5.12948397030589,-5.26511162862565,-13.0201523057468)) ;
#158212=CARTESIAN_POINT('',(-5.12948397030589,-5.3625,-13.0201523057468)) ;
#158213=CARTESIAN_POINT('',(-3.9,-4.95774063604919,-12.43)) ;
#158214=CARTESIAN_POINT('',(-3.91783961713025,-4.96220054033175,-12.4385630162225)) ;
#158215=CARTESIAN_POINT('',(-3.9,-3.14814824947882,-12.43)) ;
#158216=CARTESIAN_POINT('',(-3.9,-5.05,-12.43)) ;
#158217=CARTESIAN_POINT('',(-3.04730463122257,-4.00084361825625,-12.0207062229868)) ;
#158218=CARTESIAN_POINT('Origin',(-3.9,-5.05,-10.43)) ;
#158219=CARTESIAN_POINT('',(-3.9,-5.05,-10.5292816869892)) ;
#158220=CARTESIAN_POINT('',(-3.9,-5.05,-12.3307183130108)) ;
#158221=CARTESIAN_POINT('',(-3.9,-5.05,-10.43)) ;
#158222=CARTESIAN_POINT('',(-3.9,-4.95774063604919,-10.43)) ;
#158223=CARTESIAN_POINT('Origin',(-3.9,-4.94692235935962,-10.5409233969908)) ;
#158224=CARTESIAN_POINT('',(-3.9,-3.14814824947882,-10.43)) ;
#158225=CARTESIAN_POINT('',(-3.9,-5.05,-10.43)) ;
#158226=CARTESIAN_POINT('',(-3.9,-3.05,-10.5069822714939)) ;
#158227=CARTESIAN_POINT('Origin',(-3.9,-3.19142135623743,-10.540923396991)) ;
#158228=CARTESIAN_POINT('',(-3.9,-3.05,-12.3530177285061)) ;
#158229=CARTESIAN_POINT('',(-3.9,-3.05,-10.43)) ;
#158230=CARTESIAN_POINT('Origin',(-3.9,-3.19142135623734,-12.3190766030091)) ;
#158231=CARTESIAN_POINT('Origin',(-3.89999999999999,-4.94692235935969,-12.3190766030093)) ;
#158232=CARTESIAN_POINT('Origin',(-5.15,-5.05,-9.83)) ;
#158233=CARTESIAN_POINT('',(-5.12948397030589,-5.26511162862565,-9.83984769425317)) ;
#158234=CARTESIAN_POINT('',(-5.10741344341225,-5.25959399690224,-9.85044154716212)) ;
#158235=CARTESIAN_POINT('',(-5.12948397030589,-1.91866427917294,-9.83984769425317)) ;
#158236=CARTESIAN_POINT('',(-5.12948397030589,-1.79999999999999,-9.83984769425317)) ;
#158237=CARTESIAN_POINT('',(-3.73686704155256,-3.31128120792626,-10.5083038200548)) ;
#158238=CARTESIAN_POINT('Origin',(-5.9,-5.05,-9.83)) ;
#158239=CARTESIAN_POINT('',(-5.8,-5.42192235935956,-9.83)) ;
#158240=CARTESIAN_POINT('',(-5.8,-1.29142135623731,-9.83)) ;
#158241=CARTESIAN_POINT('',(-5.8,-1.04999999999999,-9.83)) ;
#158242=CARTESIAN_POINT('',(-5.17275707706436,-1.91866427917294,-9.83)) ;
#158243=CARTESIAN_POINT('',(-3.97071067811865,-3.12071067811865,-9.83)) ;
#158244=CARTESIAN_POINT('',(-5.17275707706436,-5.26511162862565,-9.83)) ;
#158245=CARTESIAN_POINT('',(-5.17275707706436,-5.3625,-9.83)) ;
#158246=CARTESIAN_POINT('',(-5.8066065036801,-5.42357398527959,-9.83)) ;
#158247=CARTESIAN_POINT('Origin',(-5.15,-5.05,-9.22)) ;
#158248=CARTESIAN_POINT('',(-5.8,-1.29142135623731,-9.22)) ;
#158249=CARTESIAN_POINT('',(-5.8,-5.42192235935956,-9.22)) ;
#158250=CARTESIAN_POINT('',(-5.8,-5.55,-9.22)) ;
#158251=CARTESIAN_POINT('',(-5.17275707706437,-5.26511162862565,-9.22)) ;
#158252=CARTESIAN_POINT('',(-5.10072415073893,-5.24710339704429,-9.22)) ;
#158253=CARTESIAN_POINT('',(-5.17275707706437,-1.91866427917293,-9.22)) ;
#158254=CARTESIAN_POINT('',(-5.17275707706437,-1.79999999999999,-9.22)) ;
#158255=CARTESIAN_POINT('',(-3.59571067811865,-3.49571067811865,-9.22)) ;
#158256=CARTESIAN_POINT('Origin',(-3.9,-5.05,-8.62)) ;
#158257=CARTESIAN_POINT('',(-5.12948397030589,-1.91866427917293,-9.21015230574683)) ;
#158258=CARTESIAN_POINT('',(-5.12948397030589,-5.26511162862565,-9.21015230574683)) ;
#158259=CARTESIAN_POINT('',(-5.12948397030589,-5.3625,-9.21015230574683)) ;
#158260=CARTESIAN_POINT('',(-3.9,-4.95774063604919,-8.62)) ;
#158261=CARTESIAN_POINT('',(-3.91783961713025,-4.96220054033175,-8.62856301622252)) ;
#158262=CARTESIAN_POINT('',(-3.9,-3.14814824947882,-8.62)) ;
#158263=CARTESIAN_POINT('',(-3.9,-5.05,-8.62)) ;
#158264=CARTESIAN_POINT('',(-3.04730463122257,-4.00084361825625,-8.21070622298683)) ;
#158265=CARTESIAN_POINT('Origin',(-3.9,-5.05,-6.62)) ;
#158266=CARTESIAN_POINT('',(-3.9,-5.05,-6.71928168698915)) ;
#158267=CARTESIAN_POINT('',(-3.9,-5.05,-8.52071831301085)) ;
#158268=CARTESIAN_POINT('',(-3.9,-5.05,-6.62)) ;
#158269=CARTESIAN_POINT('',(-3.9,-4.95774063604918,-6.62)) ;
#158270=CARTESIAN_POINT('Origin',(-3.9,-4.94692235935954,-6.7309233969909)) ;
#158271=CARTESIAN_POINT('',(-3.9,-3.14814824947882,-6.62)) ;
#158272=CARTESIAN_POINT('',(-3.9,-5.05,-6.62)) ;
#158273=CARTESIAN_POINT('',(-3.9,-3.05,-6.69698227149394)) ;
#158274=CARTESIAN_POINT('Origin',(-3.9,-3.19142135623718,-6.73092339699078)) ;
#158275=CARTESIAN_POINT('',(-3.9,-3.05,-8.54301772850605)) ;
#158276=CARTESIAN_POINT('',(-3.9,-3.05,-6.62)) ;
#158277=CARTESIAN_POINT('Origin',(-3.9,-3.19142135623772,-8.5090766030088)) ;
#158278=CARTESIAN_POINT('Origin',(-3.89999999999999,-4.94692235935958,-8.50907660300914)) ;
#158279=CARTESIAN_POINT('Origin',(-5.15,-5.05,-6.02)) ;
#158280=CARTESIAN_POINT('',(-5.12948397030589,-5.26511162862565,-6.02984769425317)) ;
#158281=CARTESIAN_POINT('',(-5.10741344341225,-5.25959399690224,-6.04044154716212)) ;
#158282=CARTESIAN_POINT('',(-5.12948397030589,-1.91866427917294,-6.02984769425317)) ;
#158283=CARTESIAN_POINT('',(-5.12948397030589,-1.79999999999999,-6.02984769425317)) ;
#158284=CARTESIAN_POINT('',(-3.73686704155256,-3.31128120792626,-6.69830382005477)) ;
#158285=CARTESIAN_POINT('Origin',(-5.9,-5.05,-6.02)) ;
#158286=CARTESIAN_POINT('',(-5.8,-5.42192235935956,-6.02)) ;
#158287=CARTESIAN_POINT('',(-5.8,-1.29142135623731,-6.02)) ;
#158288=CARTESIAN_POINT('',(-5.8,-1.04999999999999,-6.02)) ;
#158289=CARTESIAN_POINT('',(-5.17275707706436,-1.91866427917294,-6.02)) ;
#158290=CARTESIAN_POINT('',(-3.97071067811865,-3.12071067811865,-6.02)) ;
#158291=CARTESIAN_POINT('',(-5.17275707706436,-5.26511162862565,-6.02)) ;
#158292=CARTESIAN_POINT('',(-5.17275707706436,-5.3625,-6.02)) ;
#158293=CARTESIAN_POINT('',(-5.8066065036801,-5.42357398527959,-6.02)) ;
#158294=CARTESIAN_POINT('Origin',(-5.15,-5.05,-5.41)) ;
#158295=CARTESIAN_POINT('',(-5.8,-5.42192235935956,-5.41)) ;
#158296=CARTESIAN_POINT('',(-5.17275707706436,-5.26511162862565,-5.41)) ;
#158297=CARTESIAN_POINT('',(-5.10072415073893,-5.24710339704429,-5.41)) ;
#158298=CARTESIAN_POINT('',(-5.17275707706436,-1.91866427917294,-5.41)) ;
#158299=CARTESIAN_POINT('',(-5.17275707706436,-1.79999999999999,-5.41)) ;
#158300=CARTESIAN_POINT('',(-5.8,-1.2914213562373,-5.41)) ;
#158301=CARTESIAN_POINT('',(-3.59571067811865,-3.49571067811865,-5.41)) ;
#158302=CARTESIAN_POINT('',(-5.8,-5.55,-5.41)) ;
#158303=CARTESIAN_POINT('Origin',(-3.9,-5.05,-4.81)) ;
#158304=CARTESIAN_POINT('',(-5.12948397030589,-1.91866427917294,-5.40015230574683)) ;
#158305=CARTESIAN_POINT('',(-5.12948397030589,-5.26511162862565,-5.40015230574683)) ;
#158306=CARTESIAN_POINT('',(-5.12948397030589,-5.3625,-5.40015230574683)) ;
#158307=CARTESIAN_POINT('',(-3.9,-4.95774063604919,-4.81)) ;
#158308=CARTESIAN_POINT('',(-3.91783961713025,-4.96220054033175,-4.81856301622252)) ;
#158309=CARTESIAN_POINT('',(-3.9,-3.14814824947882,-4.81)) ;
#158310=CARTESIAN_POINT('',(-3.9,-5.05,-4.81)) ;
#158311=CARTESIAN_POINT('',(-3.04730463122257,-4.00084361825625,-4.40070622298683)) ;
#158312=CARTESIAN_POINT('Origin',(-3.9,-5.05,-2.81)) ;
#158313=CARTESIAN_POINT('',(-3.9,-5.05,-2.90928168698915)) ;
#158314=CARTESIAN_POINT('',(-3.9,-5.05,-4.71071831301085)) ;
#158315=CARTESIAN_POINT('',(-3.9,-5.05,-2.81)) ;
#158316=CARTESIAN_POINT('',(-3.9,-4.95774063604919,-2.81)) ;
#158317=CARTESIAN_POINT('Origin',(-3.9,-4.94692235935961,-2.92092339699082)) ;
#158318=CARTESIAN_POINT('',(-3.9,-3.14814824947882,-2.81)) ;
#158319=CARTESIAN_POINT('',(-3.9,-5.05,-2.81)) ;
#158320=CARTESIAN_POINT('',(-3.9,-3.05,-2.88698227149394)) ;
#158321=CARTESIAN_POINT('Origin',(-3.9,-3.19142135623728,-2.92092339699086)) ;
#158322=CARTESIAN_POINT('',(-3.9,-3.05,-4.73301772850606)) ;
#158323=CARTESIAN_POINT('',(-3.9,-3.05,-2.81)) ;
#158324=CARTESIAN_POINT('Origin',(-3.9,-3.19142135623729,-4.69907660300913)) ;
#158325=CARTESIAN_POINT('Origin',(-3.9,-4.94692235935959,-4.69907660300915)) ;
#158326=CARTESIAN_POINT('Origin',(-5.15,-5.05,-2.21)) ;
#158327=CARTESIAN_POINT('',(-5.12948397030589,-5.26511162862565,-2.21984769425317)) ;
#158328=CARTESIAN_POINT('',(-5.10741344341225,-5.25959399690224,-2.23044154716212)) ;
#158329=CARTESIAN_POINT('',(-5.12948397030589,-1.91866427917294,-2.21984769425317)) ;
#158330=CARTESIAN_POINT('',(-5.12948397030589,-1.79999999999999,-2.21984769425317)) ;
#158331=CARTESIAN_POINT('',(-3.73686704155256,-3.31128120792626,-2.88830382005477)) ;
#158332=CARTESIAN_POINT('Origin',(-5.9,-5.05,-2.21)) ;
#158333=CARTESIAN_POINT('',(-5.17275707706436,-1.91866427917294,-2.21)) ;
#158334=CARTESIAN_POINT('',(-5.17275707706436,-5.26511162862565,-2.21)) ;
#158335=CARTESIAN_POINT('',(-5.17275707706436,-5.3625,-2.21)) ;
#158336=CARTESIAN_POINT('',(-5.8,-5.42192235935956,-2.21)) ;
#158337=CARTESIAN_POINT('',(-5.8066065036801,-5.42357398527959,-2.21)) ;
#158338=CARTESIAN_POINT('',(-5.8,-1.29142135623731,-2.21)) ;
#158339=CARTESIAN_POINT('',(-5.8,-1.04999999999999,-2.21)) ;
#158340=CARTESIAN_POINT('',(-3.97071067811865,-3.12071067811865,-2.21)) ;
#158341=CARTESIAN_POINT('Origin',(-3.89999999999997,-5.05,-3.81)) ;
#158342=CARTESIAN_POINT('',(-5.82425356250363,-5.53106339062591,-2.31)) ;
#158343=CARTESIAN_POINT('',(-5.14850351456073,-5.36212587864019,-2.31)) ;
#158344=CARTESIAN_POINT('',(-3.89999999999997,-5.05,-2.31)) ;
#158345=CARTESIAN_POINT('',(-3.56560075006169,-4.96640018751543,-3.06979332695954)) ;
#158346=CARTESIAN_POINT('',(-5.14850351456073,-5.36212587864019,-5.31)) ;
#158347=CARTESIAN_POINT('',(-3.56560075006169,-4.96640018751543,-4.55020667304046)) ;
#158348=CARTESIAN_POINT('',(-5.82425356250363,-5.53106339062591,-5.31)) ;
#158349=CARTESIAN_POINT('',(-3.89999999999997,-5.05,-5.31)) ;
#158350=CARTESIAN_POINT('',(-5.82425356250363,-5.53106339062591,-3.81)) ;
#158351=CARTESIAN_POINT('Origin',(-3.89999999999997,-5.05,-7.62)) ;
#158352=CARTESIAN_POINT('',(-5.82425356250363,-5.53106339062591,-9.12597149997094)) ;
#158353=CARTESIAN_POINT('',(-5.82425356250363,-5.53106339062591,-6.11402850002907)) ;
#158354=CARTESIAN_POINT('',(-5.82425356250363,-5.53106339062591,-7.62)) ;
#158355=CARTESIAN_POINT('',(-5.77574643749636,-5.51893660937409,-6.12)) ;
#158356=CARTESIAN_POINT('Origin',(-5.7814888808097,-5.52037222020246,-5.96664642007523)) ;
#158357=CARTESIAN_POINT('',(-5.14850351456073,-5.36212587864019,-6.12)) ;
#158358=CARTESIAN_POINT('',(-3.89999999999997,-5.05,-6.12)) ;
#158359=CARTESIAN_POINT('',(-3.56560075006169,-4.96640018751543,-6.87979332695954)) ;
#158360=CARTESIAN_POINT('',(-5.14850351456074,-5.36212587864019,-9.12)) ;
#158361=CARTESIAN_POINT('',(-3.56560075006169,-4.96640018751543,-8.36020667304046)) ;
#158362=CARTESIAN_POINT('',(-5.77574643749636,-5.51893660937409,-9.12)) ;
#158363=CARTESIAN_POINT('',(-3.89999999999997,-5.05,-9.12)) ;
#158364=CARTESIAN_POINT('Origin',(-5.78148888079898,-5.52037222019986,-9.27335357990704)) ;
#158365=CARTESIAN_POINT('Origin',(-3.89999999999997,-5.05,-11.43)) ;
#158366=CARTESIAN_POINT('',(-5.82425356250363,-5.53106339062591,-12.9359714999709)) ;
#158367=CARTESIAN_POINT('',(-5.82425356250363,-5.53106339062591,-9.92402850002907)) ;
#158368=CARTESIAN_POINT('',(-5.82425356250363,-5.53106339062591,-11.43)) ;
#158369=CARTESIAN_POINT('',(-5.77574643749636,-5.51893660937409,-9.93)) ;
#158370=CARTESIAN_POINT('Origin',(-5.78148888078994,-5.52037222019747,-9.77664642000976)) ;
#158371=CARTESIAN_POINT('',(-5.14850351456073,-5.36212587864019,-9.93)) ;
#158372=CARTESIAN_POINT('',(-3.89999999999997,-5.05,-9.93)) ;
#158373=CARTESIAN_POINT('',(-3.56560075006169,-4.96640018751543,-10.6897933269595)) ;
#158374=CARTESIAN_POINT('',(-5.14850351456073,-5.36212587864019,-12.93)) ;
#158375=CARTESIAN_POINT('',(-3.56560075006169,-4.96640018751543,-12.1702066730405)) ;
#158376=CARTESIAN_POINT('',(-5.77574643749636,-5.51893660937409,-12.93)) ;
#158377=CARTESIAN_POINT('',(-3.89999999999997,-5.05,-12.93)) ;
#158378=CARTESIAN_POINT('Origin',(-5.78148888076761,-5.52037222019189,-13.0833535801862)) ;
#158379=CARTESIAN_POINT('Origin',(-3.89999999999997,-5.05,-15.24)) ;
#158380=CARTESIAN_POINT('',(-5.82425356250363,-5.53106339062591,-16.7459714999709)) ;
#158381=CARTESIAN_POINT('',(-5.82425356250363,-5.53106339062591,-13.7340285000291)) ;
#158382=CARTESIAN_POINT('',(-5.82425356250363,-5.53106339062591,-15.24)) ;
#158383=CARTESIAN_POINT('',(-5.77574643749636,-5.51893660937409,-13.74)) ;
#158384=CARTESIAN_POINT('Origin',(-5.78148888075282,-5.52037222018823,-13.5866464197048)) ;
#158385=CARTESIAN_POINT('',(-5.14850351456073,-5.36212587864019,-13.74)) ;
#158386=CARTESIAN_POINT('',(-3.89999999999997,-5.05,-13.74)) ;
#158387=CARTESIAN_POINT('',(-3.56560075006169,-4.96640018751543,-14.4997933269595)) ;
#158388=CARTESIAN_POINT('',(-5.14850351456073,-5.36212587864019,-16.74)) ;
#158389=CARTESIAN_POINT('',(-3.56560075006169,-4.96640018751543,-15.9802066730405)) ;
#158390=CARTESIAN_POINT('',(-5.77574643749636,-5.51893660937409,-16.74)) ;
#158391=CARTESIAN_POINT('',(-3.89999999999997,-5.05,-16.74)) ;
#158392=CARTESIAN_POINT('Origin',(-5.78148888084216,-5.52037222021054,-16.8933535798564)) ;
#158393=CARTESIAN_POINT('Origin',(-3.89999999999997,-5.05,-19.05)) ;
#158394=CARTESIAN_POINT('',(-5.82425356250363,-5.53106339062591,-20.5559714999709)) ;
#158395=CARTESIAN_POINT('',(-5.82425356250363,-5.53106339062591,-17.5440285000291)) ;
#158396=CARTESIAN_POINT('',(-5.82425356250363,-5.53106339062591,-19.05)) ;
#158397=CARTESIAN_POINT('',(-5.77574643749636,-5.51893660937409,-17.55)) ;
#158398=CARTESIAN_POINT('Origin',(-5.78148888084565,-5.52037222021153,-17.3966464201892)) ;
#158399=CARTESIAN_POINT('',(-5.14850351456074,-5.36212587864019,-17.55)) ;
#158400=CARTESIAN_POINT('',(-3.89999999999997,-5.05,-17.55)) ;
#158401=CARTESIAN_POINT('',(-3.56560075006169,-4.96640018751543,-18.3097933269595)) ;
#158402=CARTESIAN_POINT('',(-5.14850351456073,-5.36212587864019,-20.55)) ;
#158403=CARTESIAN_POINT('',(-3.56560075006169,-4.96640018751543,-19.7902066730405)) ;
#158404=CARTESIAN_POINT('',(-5.77574643749636,-5.51893660937409,-20.55)) ;
#158405=CARTESIAN_POINT('',(-3.89999999999997,-5.05,-20.55)) ;
#158406=CARTESIAN_POINT('Origin',(-5.78148888080932,-5.52037222020243,-20.7033535801353)) ;
#158407=CARTESIAN_POINT('Origin',(-3.89999999999997,-5.05,-22.86)) ;
#158408=CARTESIAN_POINT('',(-5.82425356250363,-5.53106339062591,-24.3659714999709)) ;
#158409=CARTESIAN_POINT('',(-5.82425356250363,-5.53106339062591,-21.3540285000291)) ;
#158410=CARTESIAN_POINT('',(-5.82425356250363,-5.53106339062591,-22.86)) ;
#158411=CARTESIAN_POINT('',(-5.77574643749636,-5.51893660937409,-21.36)) ;
#158412=CARTESIAN_POINT('Origin',(-5.7814888808788,-5.52037222021982,-21.2066464204715)) ;
#158413=CARTESIAN_POINT('',(-5.14850351456074,-5.36212587864019,-21.36)) ;
#158414=CARTESIAN_POINT('',(-3.89999999999997,-5.05,-21.36)) ;
#158415=CARTESIAN_POINT('',(-3.56560075006169,-4.96640018751543,-22.1197933269595)) ;
#158416=CARTESIAN_POINT('',(-5.14850351456073,-5.36212587864019,-24.36)) ;
#158417=CARTESIAN_POINT('',(-3.56560075006169,-4.96640018751543,-23.6002066730405)) ;
#158418=CARTESIAN_POINT('',(-5.77574643749636,-5.51893660937409,-24.36)) ;
#158419=CARTESIAN_POINT('',(-3.89999999999997,-5.05,-24.36)) ;
#158420=CARTESIAN_POINT('Origin',(-5.7814888808248,-5.5203722202062,-24.513353580007)) ;
#158421=CARTESIAN_POINT('Origin',(-3.89999999999997,-5.05,-26.67)) ;
#158422=CARTESIAN_POINT('',(-5.82425356250363,-5.53106339062591,-28.1759714999709)) ;
#158423=CARTESIAN_POINT('',(-5.82425356250363,-5.53106339062591,-25.1640285000291)) ;
#158424=CARTESIAN_POINT('',(-5.82425356250363,-5.53106339062591,-26.67)) ;
#158425=CARTESIAN_POINT('',(-5.77574643749636,-5.51893660937409,-25.17)) ;
#158426=CARTESIAN_POINT('Origin',(-5.78148888089162,-5.52037222022287,-25.016646420512)) ;
#158427=CARTESIAN_POINT('',(-5.14850351456074,-5.36212587864019,-25.17)) ;
#158428=CARTESIAN_POINT('',(-3.89999999999997,-5.05,-25.17)) ;
#158429=CARTESIAN_POINT('',(-3.56560075006169,-4.96640018751543,-25.9297933269595)) ;
#158430=CARTESIAN_POINT('',(-5.14850351456073,-5.36212587864019,-28.17)) ;
#158431=CARTESIAN_POINT('',(-3.56560075006169,-4.96640018751543,-27.4102066730405)) ;
#158432=CARTESIAN_POINT('',(-5.77574643749636,-5.51893660937409,-28.17)) ;
#158433=CARTESIAN_POINT('',(-3.89999999999997,-5.05,-28.17)) ;
#158434=CARTESIAN_POINT('Origin',(-5.78148888087819,-5.52037222021968,-28.3233535795358)) ;
#158435=CARTESIAN_POINT('Origin',(-3.89999999999997,-5.05,-30.48)) ;
#158436=CARTESIAN_POINT('',(-5.82425356250363,-5.53106339062591,-31.9859714999709)) ;
#158437=CARTESIAN_POINT('',(-5.82425356250363,-5.53106339062591,-28.9740285000291)) ;
#158438=CARTESIAN_POINT('',(-5.82425356250363,-5.53106339062591,-30.48)) ;
#158439=CARTESIAN_POINT('',(-5.77574643749636,-5.51893660937409,-28.98)) ;
#158440=CARTESIAN_POINT('Origin',(-5.78148888086266,-5.52037222021575,-28.8266464203985)) ;
#158441=CARTESIAN_POINT('',(-5.14850351456074,-5.36212587864019,-28.98)) ;
#158442=CARTESIAN_POINT('',(-3.89999999999997,-5.05,-28.98)) ;
#158443=CARTESIAN_POINT('',(-3.56560075006169,-4.96640018751543,-29.7397933269595)) ;
#158444=CARTESIAN_POINT('',(-5.14850351456071,-5.36212587864018,-31.98)) ;
#158445=CARTESIAN_POINT('',(-3.56560075006169,-4.96640018751543,-31.2202066730405)) ;
#158446=CARTESIAN_POINT('',(-5.77574643749636,-5.51893660937409,-31.98)) ;
#158447=CARTESIAN_POINT('',(-3.89999999999997,-5.05,-31.98)) ;
#158448=CARTESIAN_POINT('Origin',(-5.78148888079375,-5.52037222019844,-32.1333535799531)) ;
#158449=CARTESIAN_POINT('Origin',(-3.89999999999997,-5.05,-34.29)) ;
#158450=CARTESIAN_POINT('',(-5.82425356250363,-5.53106339062591,-35.7959714999709)) ;
#158451=CARTESIAN_POINT('',(-5.82425356250363,-5.53106339062591,-32.7840285000291)) ;
#158452=CARTESIAN_POINT('',(-5.82425356250363,-5.53106339062591,-34.29)) ;
#158453=CARTESIAN_POINT('',(-5.77574643749636,-5.51893660937409,-32.79)) ;
#158454=CARTESIAN_POINT('Origin',(-5.7814888807851,-5.52037222019633,-32.6366464199968)) ;
#158455=CARTESIAN_POINT('',(-5.14850351456072,-5.36212587864018,-32.79)) ;
#158456=CARTESIAN_POINT('',(-3.89999999999997,-5.05,-32.79)) ;
#158457=CARTESIAN_POINT('',(-3.56560075006169,-4.96640018751543,-33.5497933269595)) ;
#158458=CARTESIAN_POINT('',(-5.14850351456071,-5.36212587864018,-35.79)) ;
#158459=CARTESIAN_POINT('',(-3.56560075006169,-4.96640018751543,-35.0302066730405)) ;
#158460=CARTESIAN_POINT('',(-5.77574643749636,-5.51893660937409,-35.79)) ;
#158461=CARTESIAN_POINT('',(-3.89999999999997,-5.05,-35.79)) ;
#158462=CARTESIAN_POINT('Origin',(-5.78148888079367,-5.52037222019848,-35.9433535799528)) ;
#158463=CARTESIAN_POINT('Origin',(-5.9,-1.04999999999999,-36.59)) ;
#158464=CARTESIAN_POINT('',(-5.87071067811865,-1.07928932188134,-5.31)) ;
#158465=CARTESIAN_POINT('',(-5.10204639894571,-1.84795360105428,-5.31)) ;
#158466=CARTESIAN_POINT('',(-5.9,-1.04999999999999,-5.31)) ;
#158467=CARTESIAN_POINT('',(-12.5492788245683,5.59927882456828,-8.88467156429883)) ;
#158468=CARTESIAN_POINT('',(-5.10204639894571,-1.84795360105428,-2.31)) ;
#158469=CARTESIAN_POINT('',(1.55975991287794,-8.50975991287791,-5.50766702967535)) ;
#158470=CARTESIAN_POINT('',(-5.87071067811865,-1.07928932188134,-2.31)) ;
#158471=CARTESIAN_POINT('',(-5.9,-1.04999999999999,-2.31)) ;
#158472=CARTESIAN_POINT('',(-5.87071067811865,-1.07928932188134,-36.59)) ;
#158473=CARTESIAN_POINT('Origin',(-5.9,-1.04999999999999,-36.59)) ;
#158474=CARTESIAN_POINT('',(-5.87071067811865,-1.07928932188134,-6.06142135623731)) ;
#158475=CARTESIAN_POINT('',(-5.87071067811865,-1.07928932188134,-9.17857864376271)) ;
#158476=CARTESIAN_POINT('',(-5.87071067811865,-1.07928932188134,-36.59)) ;
#158477=CARTESIAN_POINT('',(-5.72928932188134,-1.22071067811865,-9.12)) ;
#158478=CARTESIAN_POINT('Origin',(-5.74291017058518,-1.2070898294148,-9.28714114800675)) ;
#158479=CARTESIAN_POINT('',(-5.10204639894571,-1.84795360105428,-9.12)) ;
#158480=CARTESIAN_POINT('',(-5.9,-1.04999999999999,-9.12)) ;
#158481=CARTESIAN_POINT('',(-11.7293362133775,4.77933621337747,-12.3010991109272)) ;
#158482=CARTESIAN_POINT('',(-5.10204639894571,-1.84795360105428,-6.12)) ;
#158483=CARTESIAN_POINT('',(0.739817301687122,-7.68981730168709,-8.92409457630375)) ;
#158484=CARTESIAN_POINT('',(-5.72928932188134,-1.22071067811865,-6.12)) ;
#158485=CARTESIAN_POINT('',(-5.9,-1.04999999999999,-6.12)) ;
#158486=CARTESIAN_POINT('Origin',(-5.74291017058796,-1.20708982941201,-5.95285885199633)) ;
#158487=CARTESIAN_POINT('Origin',(-5.9,-1.04999999999999,-36.59)) ;
#158488=CARTESIAN_POINT('',(-5.87071067811865,-1.07928932188134,-9.87142135623731)) ;
#158489=CARTESIAN_POINT('',(-5.87071067811865,-1.07928932188134,-12.9885786437627)) ;
#158490=CARTESIAN_POINT('',(-5.87071067811865,-1.07928932188134,-36.59)) ;
#158491=CARTESIAN_POINT('',(-5.72928932188134,-1.22071067811865,-12.93)) ;
#158492=CARTESIAN_POINT('Origin',(-5.74291017058355,-1.20708982941644,-13.0971411480106)) ;
#158493=CARTESIAN_POINT('',(-5.10204639894571,-1.84795360105428,-12.93)) ;
#158494=CARTESIAN_POINT('',(-5.9,-1.04999999999999,-12.93)) ;
#158495=CARTESIAN_POINT('',(-10.9093936021867,3.95939360218665,-15.7175266575557)) ;
#158496=CARTESIAN_POINT('',(-5.10204639894571,-1.84795360105428,-9.93)) ;
#158497=CARTESIAN_POINT('',(-0.0801253095036982,-6.86987469049627,-12.3405221229322)) ;
#158498=CARTESIAN_POINT('',(-5.72928932188134,-1.22071067811865,-9.93)) ;
#158499=CARTESIAN_POINT('',(-5.9,-1.04999999999999,-9.93)) ;
#158500=CARTESIAN_POINT('Origin',(-5.74291017058447,-1.20708982941551,-9.76285885199229)) ;
#158501=CARTESIAN_POINT('Origin',(-5.9,-1.04999999999999,-36.59)) ;
#158502=CARTESIAN_POINT('',(-5.87071067811865,-1.07928932188134,-13.6814213562373)) ;
#158503=CARTESIAN_POINT('',(-5.87071067811865,-1.07928932188134,-16.7985786437627)) ;
#158504=CARTESIAN_POINT('',(-5.87071067811865,-1.07928932188134,-36.59)) ;
#158505=CARTESIAN_POINT('',(-5.72928932188134,-1.22071067811865,-16.74)) ;
#158506=CARTESIAN_POINT('Origin',(-5.74291017058335,-1.20708982941664,-16.9071411480136)) ;
#158507=CARTESIAN_POINT('',(-5.10204639894571,-1.84795360105428,-16.74)) ;
#158508=CARTESIAN_POINT('',(-5.9,-1.04999999999999,-16.74)) ;
#158509=CARTESIAN_POINT('',(-10.0894509909958,3.13945099099583,-19.1339542041841)) ;
#158510=CARTESIAN_POINT('',(-5.10204639894571,-1.84795360105428,-13.74)) ;
#158511=CARTESIAN_POINT('',(-0.900067920694518,-6.04993207930546,-15.7569496695606)) ;
#158512=CARTESIAN_POINT('',(-5.72928932188134,-1.22071067811865,-13.74)) ;
#158513=CARTESIAN_POINT('',(-5.9,-1.04999999999999,-13.74)) ;
#158514=CARTESIAN_POINT('Origin',(-5.74291017058507,-1.20708982941492,-13.5728588519939)) ;
#158515=CARTESIAN_POINT('Origin',(-5.9,-1.04999999999999,-36.59)) ;
#158516=CARTESIAN_POINT('',(-5.87071067811865,-1.07928932188134,-17.4914213562373)) ;
#158517=CARTESIAN_POINT('',(-5.87071067811865,-1.07928932188134,-20.6085786437627)) ;
#158518=CARTESIAN_POINT('',(-5.87071067811865,-1.07928932188134,-36.59)) ;
#158519=CARTESIAN_POINT('',(-5.72928932188134,-1.22071067811865,-20.55)) ;
#158520=CARTESIAN_POINT('Origin',(-5.74291017058427,-1.20708982941573,-20.7171411480115)) ;
#158521=CARTESIAN_POINT('',(-5.10204639894571,-1.84795360105428,-20.55)) ;
#158522=CARTESIAN_POINT('',(-5.9,-1.04999999999999,-20.55)) ;
#158523=CARTESIAN_POINT('',(-9.26950837980502,2.31950837980501,-22.5503817508125)) ;
#158524=CARTESIAN_POINT('',(-5.10204639894571,-1.84795360105428,-17.55)) ;
#158525=CARTESIAN_POINT('',(-1.72001053188534,-5.22998946811464,-19.173377216189)) ;
#158526=CARTESIAN_POINT('',(-5.72928932188134,-1.22071067811865,-17.55)) ;
#158527=CARTESIAN_POINT('',(-5.9,-1.04999999999999,-17.55)) ;
#158528=CARTESIAN_POINT('Origin',(-5.74291017058526,-1.20708982941474,-17.3828588519974)) ;
#158529=CARTESIAN_POINT('Origin',(-5.9,-1.04999999999999,-36.59)) ;
#158530=CARTESIAN_POINT('',(-5.87071067811865,-1.07928932188134,-21.3014213562373)) ;
#158531=CARTESIAN_POINT('',(-5.87071067811865,-1.07928932188134,-24.4185786437627)) ;
#158532=CARTESIAN_POINT('',(-5.87071067811865,-1.07928932188134,-36.59)) ;
#158533=CARTESIAN_POINT('',(-5.72928932188134,-1.22071067811865,-24.36)) ;
#158534=CARTESIAN_POINT('Origin',(-5.74291017058376,-1.20708982941625,-24.5271411480123)) ;
#158535=CARTESIAN_POINT('',(-5.10204639894571,-1.84795360105428,-24.36)) ;
#158536=CARTESIAN_POINT('',(-5.9,-1.04999999999999,-24.36)) ;
#158537=CARTESIAN_POINT('',(-8.4495657686142,1.49956576861419,-25.9668092974409)) ;
#158538=CARTESIAN_POINT('',(-5.10204639894571,-1.84795360105428,-21.36)) ;
#158539=CARTESIAN_POINT('',(-2.53995314307616,-4.41004685692382,-22.5898047628174)) ;
#158540=CARTESIAN_POINT('',(-5.72928932188134,-1.22071067811865,-21.36)) ;
#158541=CARTESIAN_POINT('',(-5.9,-1.04999999999999,-21.36)) ;
#158542=CARTESIAN_POINT('Origin',(-5.74291017058452,-1.20708982941547,-21.1928588519956)) ;
#158543=CARTESIAN_POINT('Origin',(-5.9,-1.04999999999999,-36.59)) ;
#158544=CARTESIAN_POINT('',(-5.87071067811865,-1.07928932188134,-25.1114213562373)) ;
#158545=CARTESIAN_POINT('',(-5.87071067811865,-1.07928932188134,-28.2285786437627)) ;
#158546=CARTESIAN_POINT('',(-5.87071067811865,-1.07928932188134,-36.59)) ;
#158547=CARTESIAN_POINT('',(-5.72928932188134,-1.22071067811865,-28.17)) ;
#158548=CARTESIAN_POINT('Origin',(-5.74291017058572,-1.20708982941426,-28.3371411480073)) ;
#158549=CARTESIAN_POINT('',(-5.10204639894571,-1.84795360105428,-28.17)) ;
#158550=CARTESIAN_POINT('',(-5.9,-1.04999999999999,-28.17)) ;
#158551=CARTESIAN_POINT('',(-7.62962315742338,0.679623157423377,-29.3832368440693)) ;
#158552=CARTESIAN_POINT('',(-5.10204639894571,-1.84795360105428,-25.17)) ;
#158553=CARTESIAN_POINT('',(-3.35989575426698,-3.590104245733,-26.0062323094458)) ;
#158554=CARTESIAN_POINT('',(-5.72928932188134,-1.22071067811865,-25.17)) ;
#158555=CARTESIAN_POINT('',(-5.9,-1.04999999999999,-25.17)) ;
#158556=CARTESIAN_POINT('Origin',(-5.7429101705851,-1.20708982941489,-25.0028588519971)) ;
#158557=CARTESIAN_POINT('Origin',(-5.9,-1.04999999999999,-36.59)) ;
#158558=CARTESIAN_POINT('',(-5.87071067811865,-1.07928932188134,-28.9214213562373)) ;
#158559=CARTESIAN_POINT('',(-5.87071067811865,-1.07928932188134,-32.0385786437627)) ;
#158560=CARTESIAN_POINT('',(-5.87071067811865,-1.07928932188134,-36.59)) ;
#158561=CARTESIAN_POINT('',(-5.72928932188134,-1.22071067811865,-31.98)) ;
#158562=CARTESIAN_POINT('Origin',(-5.74291017059717,-1.20708982940281,-32.147141147996)) ;
#158563=CARTESIAN_POINT('',(-5.1020463989457,-1.84795360105429,-31.98)) ;
#158564=CARTESIAN_POINT('',(-5.9,-1.04999999999999,-31.98)) ;
#158565=CARTESIAN_POINT('',(-6.80968054623256,-0.14031945376744,-32.7996643906977)) ;
#158566=CARTESIAN_POINT('',(-5.10204639894571,-1.84795360105428,-28.98)) ;
#158567=CARTESIAN_POINT('',(-4.1798383654578,-2.77016163454219,-29.4226598560742)) ;
#158568=CARTESIAN_POINT('',(-5.72928932188134,-1.22071067811865,-28.98)) ;
#158569=CARTESIAN_POINT('',(-5.9,-1.04999999999999,-28.98)) ;
#158570=CARTESIAN_POINT('Origin',(-5.74291017058634,-1.20708982941365,-28.8128588519997)) ;
#158571=CARTESIAN_POINT('Origin',(-5.9,-1.04999999999999,-36.59)) ;
#158572=CARTESIAN_POINT('',(-5.87071067811865,-1.07928932188134,-32.7314213562373)) ;
#158573=CARTESIAN_POINT('',(-5.87071067811865,-1.07928932188134,-35.8485786437627)) ;
#158574=CARTESIAN_POINT('',(-5.87071067811865,-1.07928932188134,-36.59)) ;
#158575=CARTESIAN_POINT('',(-5.72928932188134,-1.22071067811865,-35.79)) ;
#158576=CARTESIAN_POINT('Origin',(-5.74291017059454,-1.20708982940546,-35.9571411480018)) ;
#158577=CARTESIAN_POINT('',(-5.1020463989457,-1.84795360105429,-35.79)) ;
#158578=CARTESIAN_POINT('',(-5.9,-1.04999999999999,-35.79)) ;
#158579=CARTESIAN_POINT('',(-5.98973793504174,-0.960262064958257,-36.2160919373261)) ;
#158580=CARTESIAN_POINT('',(-5.1020463989457,-1.84795360105429,-32.79)) ;
#158581=CARTESIAN_POINT('',(-4.99978097664862,-1.95021902335137,-32.8390874027026)) ;
#158582=CARTESIAN_POINT('',(-5.72928932188134,-1.22071067811865,-32.79)) ;
#158583=CARTESIAN_POINT('',(-5.9,-1.04999999999999,-32.79)) ;
#158584=CARTESIAN_POINT('Origin',(-5.74291017059665,-1.20708982940334,-32.622858852003)) ;
#158585=CARTESIAN_POINT('Origin',(-3.9,-6.4,-33.29)) ;
#158586=CARTESIAN_POINT('',(-3.9,-6.45,-35.19)) ;
#158587=CARTESIAN_POINT('',(-3.9,-6.45,-33.39)) ;
#158588=CARTESIAN_POINT('',(-3.9,-6.45,-33.29)) ;
#158589=CARTESIAN_POINT('',(-3.9,-6.35,-33.39)) ;
#158590=CARTESIAN_POINT('',(-3.9,-6.25,-33.39)) ;
#158591=CARTESIAN_POINT('',(-3.9,-6.35,-35.19)) ;
#158592=CARTESIAN_POINT('',(-3.9,-6.35,-33.29)) ;
#158593=CARTESIAN_POINT('',(-3.9,-6.45,-35.19)) ;
#158594=CARTESIAN_POINT('Origin',(-4.9,-6.4,-35.29)) ;
#158595=CARTESIAN_POINT('',(-4.,-6.35,-35.29)) ;
#158596=CARTESIAN_POINT('',(-4.8,-6.35,-35.29)) ;
#158597=CARTESIAN_POINT('',(-4.9,-6.35,-35.29)) ;
#158598=CARTESIAN_POINT('',(-4.8,-6.45,-35.29)) ;
#158599=CARTESIAN_POINT('',(-4.8,-6.45,-35.29)) ;
#158600=CARTESIAN_POINT('',(-4.,-6.45,-35.29)) ;
#158601=CARTESIAN_POINT('',(-3.9,-6.45,-35.29)) ;
#158602=CARTESIAN_POINT('',(-4.,-6.25,-35.29)) ;
#158603=CARTESIAN_POINT('Origin',(-4.9,-6.4,-33.29)) ;
#158604=CARTESIAN_POINT('',(-4.9,-6.45,-33.39)) ;
#158605=CARTESIAN_POINT('',(-4.9,-6.45,-35.19)) ;
#158606=CARTESIAN_POINT('',(-4.9,-6.45,-35.29)) ;
#158607=CARTESIAN_POINT('',(-4.9,-6.35,-35.19)) ;
#158608=CARTESIAN_POINT('',(-4.9,-6.25,-35.19)) ;
#158609=CARTESIAN_POINT('',(-4.9,-6.35,-33.39)) ;
#158610=CARTESIAN_POINT('',(-4.9,-6.35,-33.29)) ;
#158611=CARTESIAN_POINT('',(-4.9,-6.45,-33.39)) ;
#158612=CARTESIAN_POINT('Origin',(-4.9,-6.4,-33.29)) ;
#158613=CARTESIAN_POINT('',(-4.,-6.45,-33.29)) ;
#158614=CARTESIAN_POINT('',(-4.8,-6.45,-33.29)) ;
#158615=CARTESIAN_POINT('',(-4.9,-6.45,-33.29)) ;
#158616=CARTESIAN_POINT('',(-4.8,-6.35,-33.29)) ;
#158617=CARTESIAN_POINT('',(-4.8,-6.25,-33.29)) ;
#158618=CARTESIAN_POINT('',(-4.,-6.35,-33.29)) ;
#158619=CARTESIAN_POINT('',(-4.9,-6.35,-33.29)) ;
#158620=CARTESIAN_POINT('',(-4.,-6.45,-33.29)) ;
#158621=CARTESIAN_POINT('Origin',(-3.9,-6.4,-29.48)) ;
#158622=CARTESIAN_POINT('',(-3.9,-6.45,-31.38)) ;
#158623=CARTESIAN_POINT('',(-3.9,-6.45,-29.58)) ;
#158624=CARTESIAN_POINT('',(-3.9,-6.45,-29.48)) ;
#158625=CARTESIAN_POINT('',(-3.9,-6.35,-29.58)) ;
#158626=CARTESIAN_POINT('',(-3.9,-6.25,-29.58)) ;
#158627=CARTESIAN_POINT('',(-3.9,-6.35,-31.38)) ;
#158628=CARTESIAN_POINT('',(-3.9,-6.35,-29.48)) ;
#158629=CARTESIAN_POINT('',(-3.9,-6.45,-31.38)) ;
#158630=CARTESIAN_POINT('Origin',(-4.9,-6.4,-31.48)) ;
#158631=CARTESIAN_POINT('',(-4.,-6.35,-31.48)) ;
#158632=CARTESIAN_POINT('',(-4.8,-6.35,-31.48)) ;
#158633=CARTESIAN_POINT('',(-4.9,-6.35,-31.48)) ;
#158634=CARTESIAN_POINT('',(-4.8,-6.45,-31.48)) ;
#158635=CARTESIAN_POINT('',(-4.8,-6.45,-31.48)) ;
#158636=CARTESIAN_POINT('',(-4.,-6.45,-31.48)) ;
#158637=CARTESIAN_POINT('',(-3.9,-6.45,-31.48)) ;
#158638=CARTESIAN_POINT('',(-4.,-6.25,-31.48)) ;
#158639=CARTESIAN_POINT('Origin',(-4.9,-6.4,-29.48)) ;
#158640=CARTESIAN_POINT('',(-4.9,-6.45,-29.58)) ;
#158641=CARTESIAN_POINT('',(-4.9,-6.45,-31.38)) ;
#158642=CARTESIAN_POINT('',(-4.9,-6.45,-31.48)) ;
#158643=CARTESIAN_POINT('',(-4.9,-6.35,-31.38)) ;
#158644=CARTESIAN_POINT('',(-4.9,-6.25,-31.38)) ;
#158645=CARTESIAN_POINT('',(-4.9,-6.35,-29.58)) ;
#158646=CARTESIAN_POINT('',(-4.9,-6.35,-29.48)) ;
#158647=CARTESIAN_POINT('',(-4.9,-6.45,-29.58)) ;
#158648=CARTESIAN_POINT('Origin',(-4.9,-6.4,-29.48)) ;
#158649=CARTESIAN_POINT('',(-4.,-6.45,-29.48)) ;
#158650=CARTESIAN_POINT('',(-4.8,-6.45,-29.48)) ;
#158651=CARTESIAN_POINT('',(-4.9,-6.45,-29.48)) ;
#158652=CARTESIAN_POINT('',(-4.8,-6.35,-29.48)) ;
#158653=CARTESIAN_POINT('',(-4.8,-6.25,-29.48)) ;
#158654=CARTESIAN_POINT('',(-4.,-6.35,-29.48)) ;
#158655=CARTESIAN_POINT('',(-4.9,-6.35,-29.48)) ;
#158656=CARTESIAN_POINT('',(-4.,-6.45,-29.48)) ;
#158657=CARTESIAN_POINT('Origin',(-3.9,-6.4,-25.67)) ;
#158658=CARTESIAN_POINT('',(-3.9,-6.45,-27.57)) ;
#158659=CARTESIAN_POINT('',(-3.9,-6.45,-25.77)) ;
#158660=CARTESIAN_POINT('',(-3.9,-6.45,-25.67)) ;
#158661=CARTESIAN_POINT('',(-3.9,-6.35,-25.77)) ;
#158662=CARTESIAN_POINT('',(-3.9,-6.25,-25.77)) ;
#158663=CARTESIAN_POINT('',(-3.9,-6.35,-27.57)) ;
#158664=CARTESIAN_POINT('',(-3.9,-6.35,-25.67)) ;
#158665=CARTESIAN_POINT('',(-3.9,-6.45,-27.57)) ;
#158666=CARTESIAN_POINT('Origin',(-4.9,-6.4,-27.67)) ;
#158667=CARTESIAN_POINT('',(-4.,-6.35,-27.67)) ;
#158668=CARTESIAN_POINT('',(-4.8,-6.35,-27.67)) ;
#158669=CARTESIAN_POINT('',(-4.9,-6.35,-27.67)) ;
#158670=CARTESIAN_POINT('',(-4.8,-6.45,-27.67)) ;
#158671=CARTESIAN_POINT('',(-4.8,-6.45,-27.67)) ;
#158672=CARTESIAN_POINT('',(-4.,-6.45,-27.67)) ;
#158673=CARTESIAN_POINT('',(-3.9,-6.45,-27.67)) ;
#158674=CARTESIAN_POINT('',(-4.,-6.25,-27.67)) ;
#158675=CARTESIAN_POINT('Origin',(-4.9,-6.4,-25.67)) ;
#158676=CARTESIAN_POINT('',(-4.9,-6.45,-25.77)) ;
#158677=CARTESIAN_POINT('',(-4.9,-6.45,-27.57)) ;
#158678=CARTESIAN_POINT('',(-4.9,-6.45,-27.67)) ;
#158679=CARTESIAN_POINT('',(-4.9,-6.35,-27.57)) ;
#158680=CARTESIAN_POINT('',(-4.9,-6.25,-27.57)) ;
#158681=CARTESIAN_POINT('',(-4.9,-6.35,-25.77)) ;
#158682=CARTESIAN_POINT('',(-4.9,-6.35,-25.67)) ;
#158683=CARTESIAN_POINT('',(-4.9,-6.45,-25.77)) ;
#158684=CARTESIAN_POINT('Origin',(-4.9,-6.4,-25.67)) ;
#158685=CARTESIAN_POINT('',(-4.,-6.45,-25.67)) ;
#158686=CARTESIAN_POINT('',(-4.8,-6.45,-25.67)) ;
#158687=CARTESIAN_POINT('',(-4.9,-6.45,-25.67)) ;
#158688=CARTESIAN_POINT('',(-4.8,-6.35,-25.67)) ;
#158689=CARTESIAN_POINT('',(-4.8,-6.25,-25.67)) ;
#158690=CARTESIAN_POINT('',(-4.,-6.35,-25.67)) ;
#158691=CARTESIAN_POINT('',(-4.9,-6.35,-25.67)) ;
#158692=CARTESIAN_POINT('',(-4.,-6.45,-25.67)) ;
#158693=CARTESIAN_POINT('Origin',(-3.9,-6.4,-21.86)) ;
#158694=CARTESIAN_POINT('',(-3.9,-6.45,-23.76)) ;
#158695=CARTESIAN_POINT('',(-3.9,-6.45,-21.96)) ;
#158696=CARTESIAN_POINT('',(-3.9,-6.45,-21.86)) ;
#158697=CARTESIAN_POINT('',(-3.9,-6.35,-21.96)) ;
#158698=CARTESIAN_POINT('',(-3.9,-6.25,-21.96)) ;
#158699=CARTESIAN_POINT('',(-3.9,-6.35,-23.76)) ;
#158700=CARTESIAN_POINT('',(-3.9,-6.35,-21.86)) ;
#158701=CARTESIAN_POINT('',(-3.9,-6.45,-23.76)) ;
#158702=CARTESIAN_POINT('Origin',(-4.9,-6.4,-23.86)) ;
#158703=CARTESIAN_POINT('',(-4.,-6.35,-23.86)) ;
#158704=CARTESIAN_POINT('',(-4.8,-6.35,-23.86)) ;
#158705=CARTESIAN_POINT('',(-4.9,-6.35,-23.86)) ;
#158706=CARTESIAN_POINT('',(-4.8,-6.45,-23.86)) ;
#158707=CARTESIAN_POINT('',(-4.8,-6.45,-23.86)) ;
#158708=CARTESIAN_POINT('',(-4.,-6.45,-23.86)) ;
#158709=CARTESIAN_POINT('',(-3.9,-6.45,-23.86)) ;
#158710=CARTESIAN_POINT('',(-4.,-6.25,-23.86)) ;
#158711=CARTESIAN_POINT('Origin',(-4.9,-6.4,-21.86)) ;
#158712=CARTESIAN_POINT('',(-4.9,-6.45,-21.96)) ;
#158713=CARTESIAN_POINT('',(-4.9,-6.45,-23.76)) ;
#158714=CARTESIAN_POINT('',(-4.9,-6.45,-23.86)) ;
#158715=CARTESIAN_POINT('',(-4.9,-6.35,-23.76)) ;
#158716=CARTESIAN_POINT('',(-4.9,-6.25,-23.76)) ;
#158717=CARTESIAN_POINT('',(-4.9,-6.35,-21.96)) ;
#158718=CARTESIAN_POINT('',(-4.9,-6.35,-21.86)) ;
#158719=CARTESIAN_POINT('',(-4.9,-6.45,-21.96)) ;
#158720=CARTESIAN_POINT('Origin',(-4.9,-6.4,-21.86)) ;
#158721=CARTESIAN_POINT('',(-4.,-6.45,-21.86)) ;
#158722=CARTESIAN_POINT('',(-4.8,-6.45,-21.86)) ;
#158723=CARTESIAN_POINT('',(-4.9,-6.45,-21.86)) ;
#158724=CARTESIAN_POINT('',(-4.8,-6.35,-21.86)) ;
#158725=CARTESIAN_POINT('',(-4.8,-6.25,-21.86)) ;
#158726=CARTESIAN_POINT('',(-4.,-6.35,-21.86)) ;
#158727=CARTESIAN_POINT('',(-4.9,-6.35,-21.86)) ;
#158728=CARTESIAN_POINT('',(-4.,-6.45,-21.86)) ;
#158729=CARTESIAN_POINT('Origin',(-3.9,-6.4,-18.05)) ;
#158730=CARTESIAN_POINT('',(-3.9,-6.45,-19.95)) ;
#158731=CARTESIAN_POINT('',(-3.9,-6.45,-18.15)) ;
#158732=CARTESIAN_POINT('',(-3.9,-6.45,-18.05)) ;
#158733=CARTESIAN_POINT('',(-3.9,-6.35,-18.15)) ;
#158734=CARTESIAN_POINT('',(-3.9,-6.25,-18.15)) ;
#158735=CARTESIAN_POINT('',(-3.9,-6.35,-19.95)) ;
#158736=CARTESIAN_POINT('',(-3.9,-6.35,-18.05)) ;
#158737=CARTESIAN_POINT('',(-3.9,-6.45,-19.95)) ;
#158738=CARTESIAN_POINT('Origin',(-4.9,-6.4,-20.05)) ;
#158739=CARTESIAN_POINT('',(-4.,-6.35,-20.05)) ;
#158740=CARTESIAN_POINT('',(-4.8,-6.35,-20.05)) ;
#158741=CARTESIAN_POINT('',(-4.9,-6.35,-20.05)) ;
#158742=CARTESIAN_POINT('',(-4.8,-6.45,-20.05)) ;
#158743=CARTESIAN_POINT('',(-4.8,-6.45,-20.05)) ;
#158744=CARTESIAN_POINT('',(-4.,-6.45,-20.05)) ;
#158745=CARTESIAN_POINT('',(-3.9,-6.45,-20.05)) ;
#158746=CARTESIAN_POINT('',(-4.,-6.25,-20.05)) ;
#158747=CARTESIAN_POINT('Origin',(-4.9,-6.4,-18.05)) ;
#158748=CARTESIAN_POINT('',(-4.9,-6.45,-18.15)) ;
#158749=CARTESIAN_POINT('',(-4.9,-6.45,-19.95)) ;
#158750=CARTESIAN_POINT('',(-4.9,-6.45,-20.05)) ;
#158751=CARTESIAN_POINT('',(-4.9,-6.35,-19.95)) ;
#158752=CARTESIAN_POINT('',(-4.9,-6.25,-19.95)) ;
#158753=CARTESIAN_POINT('',(-4.9,-6.35,-18.15)) ;
#158754=CARTESIAN_POINT('',(-4.9,-6.35,-18.05)) ;
#158755=CARTESIAN_POINT('',(-4.9,-6.45,-18.15)) ;
#158756=CARTESIAN_POINT('Origin',(-4.9,-6.4,-18.05)) ;
#158757=CARTESIAN_POINT('',(-4.,-6.45,-18.05)) ;
#158758=CARTESIAN_POINT('',(-4.8,-6.45,-18.05)) ;
#158759=CARTESIAN_POINT('',(-4.9,-6.45,-18.05)) ;
#158760=CARTESIAN_POINT('',(-4.8,-6.35,-18.05)) ;
#158761=CARTESIAN_POINT('',(-4.8,-6.25,-18.05)) ;
#158762=CARTESIAN_POINT('',(-4.,-6.35,-18.05)) ;
#158763=CARTESIAN_POINT('',(-4.9,-6.35,-18.05)) ;
#158764=CARTESIAN_POINT('',(-4.,-6.45,-18.05)) ;
#158765=CARTESIAN_POINT('Origin',(-3.9,-6.4,-14.24)) ;
#158766=CARTESIAN_POINT('',(-3.9,-6.45,-16.14)) ;
#158767=CARTESIAN_POINT('',(-3.9,-6.45,-14.34)) ;
#158768=CARTESIAN_POINT('',(-3.9,-6.45,-14.24)) ;
#158769=CARTESIAN_POINT('',(-3.9,-6.35,-14.34)) ;
#158770=CARTESIAN_POINT('',(-3.9,-6.25,-14.34)) ;
#158771=CARTESIAN_POINT('',(-3.9,-6.35,-16.14)) ;
#158772=CARTESIAN_POINT('',(-3.9,-6.35,-14.24)) ;
#158773=CARTESIAN_POINT('',(-3.9,-6.45,-16.14)) ;
#158774=CARTESIAN_POINT('Origin',(-4.9,-6.4,-16.24)) ;
#158775=CARTESIAN_POINT('',(-4.,-6.35,-16.24)) ;
#158776=CARTESIAN_POINT('',(-4.8,-6.35,-16.24)) ;
#158777=CARTESIAN_POINT('',(-4.9,-6.35,-16.24)) ;
#158778=CARTESIAN_POINT('',(-4.8,-6.45,-16.24)) ;
#158779=CARTESIAN_POINT('',(-4.8,-6.45,-16.24)) ;
#158780=CARTESIAN_POINT('',(-4.,-6.45,-16.24)) ;
#158781=CARTESIAN_POINT('',(-3.9,-6.45,-16.24)) ;
#158782=CARTESIAN_POINT('',(-4.,-6.25,-16.24)) ;
#158783=CARTESIAN_POINT('Origin',(-4.9,-6.4,-14.24)) ;
#158784=CARTESIAN_POINT('',(-4.9,-6.45,-14.34)) ;
#158785=CARTESIAN_POINT('',(-4.9,-6.45,-16.14)) ;
#158786=CARTESIAN_POINT('',(-4.9,-6.45,-16.24)) ;
#158787=CARTESIAN_POINT('',(-4.9,-6.35,-16.14)) ;
#158788=CARTESIAN_POINT('',(-4.9,-6.25,-16.14)) ;
#158789=CARTESIAN_POINT('',(-4.9,-6.35,-14.34)) ;
#158790=CARTESIAN_POINT('',(-4.9,-6.35,-14.24)) ;
#158791=CARTESIAN_POINT('',(-4.9,-6.45,-14.34)) ;
#158792=CARTESIAN_POINT('Origin',(-4.9,-6.4,-14.24)) ;
#158793=CARTESIAN_POINT('',(-4.,-6.45,-14.24)) ;
#158794=CARTESIAN_POINT('',(-4.8,-6.45,-14.24)) ;
#158795=CARTESIAN_POINT('',(-4.9,-6.45,-14.24)) ;
#158796=CARTESIAN_POINT('',(-4.8,-6.35,-14.24)) ;
#158797=CARTESIAN_POINT('',(-4.8,-6.25,-14.24)) ;
#158798=CARTESIAN_POINT('',(-4.,-6.35,-14.24)) ;
#158799=CARTESIAN_POINT('',(-4.9,-6.35,-14.24)) ;
#158800=CARTESIAN_POINT('',(-4.,-6.45,-14.24)) ;
#158801=CARTESIAN_POINT('Origin',(-3.9,-6.4,-10.43)) ;
#158802=CARTESIAN_POINT('',(-3.9,-6.45,-12.33)) ;
#158803=CARTESIAN_POINT('',(-3.9,-6.45,-10.53)) ;
#158804=CARTESIAN_POINT('',(-3.9,-6.45,-10.43)) ;
#158805=CARTESIAN_POINT('',(-3.9,-6.35,-10.53)) ;
#158806=CARTESIAN_POINT('',(-3.9,-6.25,-10.53)) ;
#158807=CARTESIAN_POINT('',(-3.9,-6.35,-12.33)) ;
#158808=CARTESIAN_POINT('',(-3.9,-6.35,-10.43)) ;
#158809=CARTESIAN_POINT('',(-3.9,-6.45,-12.33)) ;
#158810=CARTESIAN_POINT('Origin',(-4.9,-6.4,-12.43)) ;
#158811=CARTESIAN_POINT('',(-4.,-6.35,-12.43)) ;
#158812=CARTESIAN_POINT('',(-4.8,-6.35,-12.43)) ;
#158813=CARTESIAN_POINT('',(-4.9,-6.35,-12.43)) ;
#158814=CARTESIAN_POINT('',(-4.8,-6.45,-12.43)) ;
#158815=CARTESIAN_POINT('',(-4.8,-6.45,-12.43)) ;
#158816=CARTESIAN_POINT('',(-4.,-6.45,-12.43)) ;
#158817=CARTESIAN_POINT('',(-3.9,-6.45,-12.43)) ;
#158818=CARTESIAN_POINT('',(-4.,-6.25,-12.43)) ;
#158819=CARTESIAN_POINT('Origin',(-4.9,-6.4,-10.43)) ;
#158820=CARTESIAN_POINT('',(-4.9,-6.45,-10.53)) ;
#158821=CARTESIAN_POINT('',(-4.9,-6.45,-12.33)) ;
#158822=CARTESIAN_POINT('',(-4.9,-6.45,-12.43)) ;
#158823=CARTESIAN_POINT('',(-4.9,-6.35,-12.33)) ;
#158824=CARTESIAN_POINT('',(-4.9,-6.25,-12.33)) ;
#158825=CARTESIAN_POINT('',(-4.9,-6.35,-10.53)) ;
#158826=CARTESIAN_POINT('',(-4.9,-6.35,-10.43)) ;
#158827=CARTESIAN_POINT('',(-4.9,-6.45,-10.53)) ;
#158828=CARTESIAN_POINT('Origin',(-4.9,-6.4,-10.43)) ;
#158829=CARTESIAN_POINT('',(-4.,-6.45,-10.43)) ;
#158830=CARTESIAN_POINT('',(-4.8,-6.45,-10.43)) ;
#158831=CARTESIAN_POINT('',(-4.9,-6.45,-10.43)) ;
#158832=CARTESIAN_POINT('',(-4.8,-6.35,-10.43)) ;
#158833=CARTESIAN_POINT('',(-4.8,-6.25,-10.43)) ;
#158834=CARTESIAN_POINT('',(-4.,-6.35,-10.43)) ;
#158835=CARTESIAN_POINT('',(-4.9,-6.35,-10.43)) ;
#158836=CARTESIAN_POINT('',(-4.,-6.45,-10.43)) ;
#158837=CARTESIAN_POINT('Origin',(-3.9,-6.4,-6.62)) ;
#158838=CARTESIAN_POINT('',(-3.9,-6.45,-8.52)) ;
#158839=CARTESIAN_POINT('',(-3.9,-6.45,-6.72)) ;
#158840=CARTESIAN_POINT('',(-3.9,-6.45,-6.62)) ;
#158841=CARTESIAN_POINT('',(-3.9,-6.35,-6.72)) ;
#158842=CARTESIAN_POINT('',(-3.9,-6.25,-6.72)) ;
#158843=CARTESIAN_POINT('',(-3.9,-6.35,-8.52)) ;
#158844=CARTESIAN_POINT('',(-3.9,-6.35,-6.62)) ;
#158845=CARTESIAN_POINT('',(-3.9,-6.45,-8.52)) ;
#158846=CARTESIAN_POINT('Origin',(-4.9,-6.4,-8.62)) ;
#158847=CARTESIAN_POINT('',(-4.,-6.35,-8.62)) ;
#158848=CARTESIAN_POINT('',(-4.8,-6.35,-8.62)) ;
#158849=CARTESIAN_POINT('',(-4.9,-6.35,-8.62)) ;
#158850=CARTESIAN_POINT('',(-4.8,-6.45,-8.62)) ;
#158851=CARTESIAN_POINT('',(-4.8,-6.45,-8.62)) ;
#158852=CARTESIAN_POINT('',(-4.,-6.45,-8.62)) ;
#158853=CARTESIAN_POINT('',(-3.9,-6.45,-8.62)) ;
#158854=CARTESIAN_POINT('',(-4.,-6.25,-8.62)) ;
#158855=CARTESIAN_POINT('Origin',(-4.9,-6.4,-6.62)) ;
#158856=CARTESIAN_POINT('',(-4.9,-6.45,-6.72)) ;
#158857=CARTESIAN_POINT('',(-4.9,-6.45,-8.52)) ;
#158858=CARTESIAN_POINT('',(-4.9,-6.45,-8.62)) ;
#158859=CARTESIAN_POINT('',(-4.9,-6.35,-8.52)) ;
#158860=CARTESIAN_POINT('',(-4.9,-6.25,-8.52)) ;
#158861=CARTESIAN_POINT('',(-4.9,-6.35,-6.72)) ;
#158862=CARTESIAN_POINT('',(-4.9,-6.35,-6.62)) ;
#158863=CARTESIAN_POINT('',(-4.9,-6.45,-6.72)) ;
#158864=CARTESIAN_POINT('Origin',(-4.9,-6.4,-6.62)) ;
#158865=CARTESIAN_POINT('',(-4.,-6.45,-6.62)) ;
#158866=CARTESIAN_POINT('',(-4.8,-6.45,-6.62)) ;
#158867=CARTESIAN_POINT('',(-4.9,-6.45,-6.62)) ;
#158868=CARTESIAN_POINT('',(-4.8,-6.35,-6.62)) ;
#158869=CARTESIAN_POINT('',(-4.8,-6.25,-6.62)) ;
#158870=CARTESIAN_POINT('',(-4.,-6.35,-6.62)) ;
#158871=CARTESIAN_POINT('',(-4.9,-6.35,-6.62)) ;
#158872=CARTESIAN_POINT('',(-4.,-6.45,-6.62)) ;
#158873=CARTESIAN_POINT('Origin',(-3.9,-6.4,-2.81)) ;
#158874=CARTESIAN_POINT('',(-3.9,-6.35,-2.91)) ;
#158875=CARTESIAN_POINT('',(-3.9,-6.35,-4.71)) ;
#158876=CARTESIAN_POINT('',(-3.9,-6.35,-2.81)) ;
#158877=CARTESIAN_POINT('',(-3.9,-6.45,-4.71)) ;
#158878=CARTESIAN_POINT('',(-3.9,-6.55,-4.71)) ;
#158879=CARTESIAN_POINT('',(-3.9,-6.45,-2.91)) ;
#158880=CARTESIAN_POINT('',(-3.9,-6.45,-2.81)) ;
#158881=CARTESIAN_POINT('',(-3.9,-6.25,-2.91)) ;
#158882=CARTESIAN_POINT('Origin',(-4.9,-6.4,-4.81)) ;
#158883=CARTESIAN_POINT('',(-4.,-6.35,-4.81)) ;
#158884=CARTESIAN_POINT('',(-4.8,-6.35,-4.81)) ;
#158885=CARTESIAN_POINT('',(-4.9,-6.35,-4.81)) ;
#158886=CARTESIAN_POINT('',(-4.8,-6.45,-4.81)) ;
#158887=CARTESIAN_POINT('',(-4.8,-6.55,-4.81)) ;
#158888=CARTESIAN_POINT('',(-4.,-6.45,-4.81)) ;
#158889=CARTESIAN_POINT('',(-3.9,-6.45,-4.81)) ;
#158890=CARTESIAN_POINT('',(-4.,-6.25,-4.81)) ;
#158891=CARTESIAN_POINT('Origin',(-4.9,-6.4,-2.81)) ;
#158892=CARTESIAN_POINT('',(-4.9,-6.45,-4.71)) ;
#158893=CARTESIAN_POINT('',(-4.9,-6.35,-4.71)) ;
#158894=CARTESIAN_POINT('',(-4.9,-6.25,-4.71)) ;
#158895=CARTESIAN_POINT('',(-4.9,-6.35,-2.91)) ;
#158896=CARTESIAN_POINT('',(-4.9,-6.35,-2.81)) ;
#158897=CARTESIAN_POINT('',(-4.9,-6.45,-2.91)) ;
#158898=CARTESIAN_POINT('',(-4.9,-6.55,-2.91)) ;
#158899=CARTESIAN_POINT('',(-4.9,-6.45,-4.81)) ;
#158900=CARTESIAN_POINT('Origin',(-4.9,-6.4,-2.81)) ;
#158901=CARTESIAN_POINT('',(-4.8,-6.45,-2.81)) ;
#158902=CARTESIAN_POINT('',(-4.8,-6.35,-2.81)) ;
#158903=CARTESIAN_POINT('',(-4.8,-6.25,-2.81)) ;
#158904=CARTESIAN_POINT('',(-4.,-6.35,-2.81)) ;
#158905=CARTESIAN_POINT('',(-4.9,-6.35,-2.81)) ;
#158906=CARTESIAN_POINT('',(-4.,-6.45,-2.81)) ;
#158907=CARTESIAN_POINT('',(-4.,-6.55,-2.81)) ;
#158908=CARTESIAN_POINT('',(-4.9,-6.45,-2.81)) ;
#158909=CARTESIAN_POINT('Origin',(0.,-6.25,-3.81)) ;
#158910=CARTESIAN_POINT('',(-4.8,-6.25,-2.91)) ;
#158911=CARTESIAN_POINT('',(-4.8,-6.25,-4.71)) ;
#158912=CARTESIAN_POINT('',(-4.8,-6.25,-3.81)) ;
#158913=CARTESIAN_POINT('',(-4.,-6.25,-4.71)) ;
#158914=CARTESIAN_POINT('',(1.95156391047391E-16,-6.25,-4.71)) ;
#158915=CARTESIAN_POINT('',(-4.,-6.25,-2.91)) ;
#158916=CARTESIAN_POINT('',(-4.,-6.25,-3.81)) ;
#158917=CARTESIAN_POINT('',(1.9515639104739E-16,-6.25,-2.91)) ;
#158918=CARTESIAN_POINT('',(-4.65,-6.25,-4.66)) ;
#158919=CARTESIAN_POINT('',(-4.15,-6.25,-4.66)) ;
#158920=CARTESIAN_POINT('',(-4.75,-6.25,-4.66)) ;
#158921=CARTESIAN_POINT('',(-4.75,-6.25,-4.56)) ;
#158922=CARTESIAN_POINT('Origin',(-4.65,-6.25,-4.56)) ;
#158923=CARTESIAN_POINT('',(-4.75,-6.25,-3.06)) ;
#158924=CARTESIAN_POINT('',(-4.75,-6.25,-2.96)) ;
#158925=CARTESIAN_POINT('',(-4.65,-6.25,-2.96)) ;
#158926=CARTESIAN_POINT('Origin',(-4.65,-6.25,-3.06)) ;
#158927=CARTESIAN_POINT('',(-4.15,-6.25,-2.96)) ;
#158928=CARTESIAN_POINT('',(-4.05,-6.25,-2.96)) ;
#158929=CARTESIAN_POINT('',(-4.05,-6.25,-3.06)) ;
#158930=CARTESIAN_POINT('Origin',(-4.15,-6.25,-3.06)) ;
#158931=CARTESIAN_POINT('',(-4.05,-6.25,-4.56)) ;
#158932=CARTESIAN_POINT('',(-4.05,-6.25,-4.66)) ;
#158933=CARTESIAN_POINT('Origin',(-4.15,-6.25,-4.56)) ;
#158934=CARTESIAN_POINT('Origin',(-4.05,-6.25,-4.66)) ;
#158935=CARTESIAN_POINT('',(-4.05,-6.3,-3.06)) ;
#158936=CARTESIAN_POINT('',(-4.05,-6.25,-3.06)) ;
#158937=CARTESIAN_POINT('',(-4.05,-6.3,-4.56)) ;
#158938=CARTESIAN_POINT('',(-4.05,-6.3,-4.66)) ;
#158939=CARTESIAN_POINT('',(-4.05,-6.25,-4.56)) ;
#158940=CARTESIAN_POINT('Origin',(-4.75,-6.25,-4.66)) ;
#158941=CARTESIAN_POINT('',(-4.15,-6.3,-4.66)) ;
#158942=CARTESIAN_POINT('',(-4.15,-6.25,-4.66)) ;
#158943=CARTESIAN_POINT('',(-4.65,-6.3,-4.66)) ;
#158944=CARTESIAN_POINT('',(-4.75,-6.3,-4.66)) ;
#158945=CARTESIAN_POINT('',(-4.65,-6.25,-4.66)) ;
#158946=CARTESIAN_POINT('Origin',(-4.75,-6.25,-2.96)) ;
#158947=CARTESIAN_POINT('',(-4.75,-6.3,-4.56)) ;
#158948=CARTESIAN_POINT('',(-4.75,-6.3,-3.06)) ;
#158949=CARTESIAN_POINT('',(-4.75,-6.3,-2.96)) ;
#158950=CARTESIAN_POINT('',(-4.75,-6.25,-3.06)) ;
#158951=CARTESIAN_POINT('',(-4.75,-6.25,-4.56)) ;
#158952=CARTESIAN_POINT('Origin',(-4.05,-6.25,-2.96)) ;
#158953=CARTESIAN_POINT('',(-4.65,-6.3,-2.96)) ;
#158954=CARTESIAN_POINT('',(-4.65,-6.25,-2.96)) ;
#158955=CARTESIAN_POINT('',(-4.15,-6.3,-2.96)) ;
#158956=CARTESIAN_POINT('',(-4.05,-6.3,-2.96)) ;
#158957=CARTESIAN_POINT('',(-4.15,-6.25,-2.96)) ;
#158958=CARTESIAN_POINT('Origin',(0.,-6.25,-7.62)) ;
#158959=CARTESIAN_POINT('',(-4.8,-6.25,-6.72)) ;
#158960=CARTESIAN_POINT('',(-4.8,-6.25,-8.52)) ;
#158961=CARTESIAN_POINT('',(-4.8,-6.25,-7.62)) ;
#158962=CARTESIAN_POINT('',(-4.,-6.25,-8.52)) ;
#158963=CARTESIAN_POINT('',(1.95156391047391E-16,-6.25,-8.52)) ;
#158964=CARTESIAN_POINT('',(-4.,-6.25,-6.72)) ;
#158965=CARTESIAN_POINT('',(-4.,-6.25,-7.62)) ;
#158966=CARTESIAN_POINT('',(1.9515639104739E-16,-6.25,-6.72000000000001)) ;
#158967=CARTESIAN_POINT('',(-4.65,-6.25,-8.47)) ;
#158968=CARTESIAN_POINT('',(-4.15,-6.25,-8.47)) ;
#158969=CARTESIAN_POINT('',(-4.75,-6.25,-8.47)) ;
#158970=CARTESIAN_POINT('',(-4.75,-6.25,-8.37)) ;
#158971=CARTESIAN_POINT('Origin',(-4.65,-6.25,-8.37)) ;
#158972=CARTESIAN_POINT('',(-4.75,-6.25,-6.87)) ;
#158973=CARTESIAN_POINT('',(-4.75,-6.25,-6.77)) ;
#158974=CARTESIAN_POINT('',(-4.65,-6.25,-6.77)) ;
#158975=CARTESIAN_POINT('Origin',(-4.65,-6.25,-6.87)) ;
#158976=CARTESIAN_POINT('',(-4.15,-6.25,-6.77)) ;
#158977=CARTESIAN_POINT('',(-4.05,-6.25,-6.77)) ;
#158978=CARTESIAN_POINT('',(-4.05,-6.25,-6.87)) ;
#158979=CARTESIAN_POINT('Origin',(-4.15,-6.25,-6.87)) ;
#158980=CARTESIAN_POINT('',(-4.05,-6.25,-8.37)) ;
#158981=CARTESIAN_POINT('',(-4.05,-6.25,-8.47)) ;
#158982=CARTESIAN_POINT('Origin',(-4.15,-6.25,-8.37)) ;
#158983=CARTESIAN_POINT('Origin',(-4.05,-6.25,-8.47)) ;
#158984=CARTESIAN_POINT('',(-4.05,-6.3,-6.87)) ;
#158985=CARTESIAN_POINT('',(-4.05,-6.25,-6.87)) ;
#158986=CARTESIAN_POINT('',(-4.05,-6.3,-8.37)) ;
#158987=CARTESIAN_POINT('',(-4.05,-6.3,-8.47)) ;
#158988=CARTESIAN_POINT('',(-4.05,-6.25,-8.37)) ;
#158989=CARTESIAN_POINT('Origin',(-4.75,-6.25,-8.47)) ;
#158990=CARTESIAN_POINT('',(-4.15,-6.3,-8.47)) ;
#158991=CARTESIAN_POINT('',(-4.15,-6.25,-8.47)) ;
#158992=CARTESIAN_POINT('',(-4.65,-6.3,-8.47)) ;
#158993=CARTESIAN_POINT('',(-4.75,-6.3,-8.47)) ;
#158994=CARTESIAN_POINT('',(-4.65,-6.25,-8.47)) ;
#158995=CARTESIAN_POINT('Origin',(-4.75,-6.25,-6.77)) ;
#158996=CARTESIAN_POINT('',(-4.75,-6.3,-8.37)) ;
#158997=CARTESIAN_POINT('',(-4.75,-6.3,-6.87)) ;
#158998=CARTESIAN_POINT('',(-4.75,-6.3,-6.77)) ;
#158999=CARTESIAN_POINT('',(-4.75,-6.25,-6.87)) ;
#159000=CARTESIAN_POINT('',(-4.75,-6.25,-8.37)) ;
#159001=CARTESIAN_POINT('Origin',(-4.05,-6.25,-6.77)) ;
#159002=CARTESIAN_POINT('',(-4.65,-6.3,-6.77)) ;
#159003=CARTESIAN_POINT('',(-4.65,-6.25,-6.77)) ;
#159004=CARTESIAN_POINT('',(-4.15,-6.3,-6.77)) ;
#159005=CARTESIAN_POINT('',(-4.05,-6.3,-6.77)) ;
#159006=CARTESIAN_POINT('',(-4.15,-6.25,-6.77)) ;
#159007=CARTESIAN_POINT('Origin',(0.,-6.25,-11.43)) ;
#159008=CARTESIAN_POINT('',(-4.8,-6.25,-10.53)) ;
#159009=CARTESIAN_POINT('',(-4.8,-6.25,-12.33)) ;
#159010=CARTESIAN_POINT('',(-4.8,-6.25,-11.43)) ;
#159011=CARTESIAN_POINT('',(-4.,-6.25,-12.33)) ;
#159012=CARTESIAN_POINT('',(1.95156391047391E-16,-6.25,-12.33)) ;
#159013=CARTESIAN_POINT('',(-4.,-6.25,-10.53)) ;
#159014=CARTESIAN_POINT('',(-4.,-6.25,-11.43)) ;
#159015=CARTESIAN_POINT('',(1.9515639104739E-16,-6.25,-10.53)) ;
#159016=CARTESIAN_POINT('',(-4.65,-6.25,-12.28)) ;
#159017=CARTESIAN_POINT('',(-4.15,-6.25,-12.28)) ;
#159018=CARTESIAN_POINT('',(-4.75,-6.25,-12.28)) ;
#159019=CARTESIAN_POINT('',(-4.75,-6.25,-12.18)) ;
#159020=CARTESIAN_POINT('Origin',(-4.65,-6.25,-12.18)) ;
#159021=CARTESIAN_POINT('',(-4.75,-6.25,-10.68)) ;
#159022=CARTESIAN_POINT('',(-4.75,-6.25,-10.58)) ;
#159023=CARTESIAN_POINT('',(-4.65,-6.25,-10.58)) ;
#159024=CARTESIAN_POINT('Origin',(-4.65,-6.25,-10.68)) ;
#159025=CARTESIAN_POINT('',(-4.15,-6.25,-10.58)) ;
#159026=CARTESIAN_POINT('',(-4.05,-6.25,-10.58)) ;
#159027=CARTESIAN_POINT('',(-4.05,-6.25,-10.68)) ;
#159028=CARTESIAN_POINT('Origin',(-4.15,-6.25,-10.68)) ;
#159029=CARTESIAN_POINT('',(-4.05,-6.25,-12.18)) ;
#159030=CARTESIAN_POINT('',(-4.05,-6.25,-12.28)) ;
#159031=CARTESIAN_POINT('Origin',(-4.15,-6.25,-12.18)) ;
#159032=CARTESIAN_POINT('Origin',(-4.05,-6.25,-12.28)) ;
#159033=CARTESIAN_POINT('',(-4.05,-6.3,-10.68)) ;
#159034=CARTESIAN_POINT('',(-4.05,-6.25,-10.68)) ;
#159035=CARTESIAN_POINT('',(-4.05,-6.3,-12.18)) ;
#159036=CARTESIAN_POINT('',(-4.05,-6.3,-12.28)) ;
#159037=CARTESIAN_POINT('',(-4.05,-6.25,-12.18)) ;
#159038=CARTESIAN_POINT('Origin',(-4.75,-6.25,-12.28)) ;
#159039=CARTESIAN_POINT('',(-4.15,-6.3,-12.28)) ;
#159040=CARTESIAN_POINT('',(-4.15,-6.25,-12.28)) ;
#159041=CARTESIAN_POINT('',(-4.65,-6.3,-12.28)) ;
#159042=CARTESIAN_POINT('',(-4.75,-6.3,-12.28)) ;
#159043=CARTESIAN_POINT('',(-4.65,-6.25,-12.28)) ;
#159044=CARTESIAN_POINT('Origin',(-4.75,-6.25,-10.58)) ;
#159045=CARTESIAN_POINT('',(-4.75,-6.3,-12.18)) ;
#159046=CARTESIAN_POINT('',(-4.75,-6.3,-10.68)) ;
#159047=CARTESIAN_POINT('',(-4.75,-6.3,-10.58)) ;
#159048=CARTESIAN_POINT('',(-4.75,-6.25,-10.68)) ;
#159049=CARTESIAN_POINT('',(-4.75,-6.25,-12.18)) ;
#159050=CARTESIAN_POINT('Origin',(-4.05,-6.25,-10.58)) ;
#159051=CARTESIAN_POINT('',(-4.65,-6.3,-10.58)) ;
#159052=CARTESIAN_POINT('',(-4.65,-6.25,-10.58)) ;
#159053=CARTESIAN_POINT('',(-4.15,-6.3,-10.58)) ;
#159054=CARTESIAN_POINT('',(-4.05,-6.3,-10.58)) ;
#159055=CARTESIAN_POINT('',(-4.15,-6.25,-10.58)) ;
#159056=CARTESIAN_POINT('Origin',(0.,-6.25,-15.24)) ;
#159057=CARTESIAN_POINT('',(-4.8,-6.25,-14.34)) ;
#159058=CARTESIAN_POINT('',(-4.8,-6.25,-16.14)) ;
#159059=CARTESIAN_POINT('',(-4.8,-6.25,-15.24)) ;
#159060=CARTESIAN_POINT('',(-4.,-6.25,-16.14)) ;
#159061=CARTESIAN_POINT('',(1.95156391047391E-16,-6.25,-16.14)) ;
#159062=CARTESIAN_POINT('',(-4.,-6.25,-14.34)) ;
#159063=CARTESIAN_POINT('',(-4.,-6.25,-15.24)) ;
#159064=CARTESIAN_POINT('',(1.9515639104739E-16,-6.25,-14.34)) ;
#159065=CARTESIAN_POINT('',(-4.65,-6.25,-16.09)) ;
#159066=CARTESIAN_POINT('',(-4.15,-6.25,-16.09)) ;
#159067=CARTESIAN_POINT('',(-4.75,-6.25,-16.09)) ;
#159068=CARTESIAN_POINT('',(-4.75,-6.25,-15.99)) ;
#159069=CARTESIAN_POINT('Origin',(-4.65,-6.25,-15.99)) ;
#159070=CARTESIAN_POINT('',(-4.75,-6.25,-14.49)) ;
#159071=CARTESIAN_POINT('',(-4.75,-6.25,-14.39)) ;
#159072=CARTESIAN_POINT('',(-4.65,-6.25,-14.39)) ;
#159073=CARTESIAN_POINT('Origin',(-4.65,-6.25,-14.49)) ;
#159074=CARTESIAN_POINT('',(-4.15,-6.25,-14.39)) ;
#159075=CARTESIAN_POINT('',(-4.05,-6.25,-14.39)) ;
#159076=CARTESIAN_POINT('',(-4.05,-6.25,-14.49)) ;
#159077=CARTESIAN_POINT('Origin',(-4.15,-6.25,-14.49)) ;
#159078=CARTESIAN_POINT('',(-4.05,-6.25,-15.99)) ;
#159079=CARTESIAN_POINT('',(-4.05,-6.25,-16.09)) ;
#159080=CARTESIAN_POINT('Origin',(-4.15,-6.25,-15.99)) ;
#159081=CARTESIAN_POINT('Origin',(-4.05,-6.25,-16.09)) ;
#159082=CARTESIAN_POINT('',(-4.05,-6.3,-14.49)) ;
#159083=CARTESIAN_POINT('',(-4.05,-6.25,-14.49)) ;
#159084=CARTESIAN_POINT('',(-4.05,-6.3,-15.99)) ;
#159085=CARTESIAN_POINT('',(-4.05,-6.3,-16.09)) ;
#159086=CARTESIAN_POINT('',(-4.05,-6.25,-15.99)) ;
#159087=CARTESIAN_POINT('Origin',(-4.75,-6.25,-16.09)) ;
#159088=CARTESIAN_POINT('',(-4.15,-6.3,-16.09)) ;
#159089=CARTESIAN_POINT('',(-4.15,-6.25,-16.09)) ;
#159090=CARTESIAN_POINT('',(-4.65,-6.3,-16.09)) ;
#159091=CARTESIAN_POINT('',(-4.75,-6.3,-16.09)) ;
#159092=CARTESIAN_POINT('',(-4.65,-6.25,-16.09)) ;
#159093=CARTESIAN_POINT('Origin',(-4.75,-6.25,-14.39)) ;
#159094=CARTESIAN_POINT('',(-4.75,-6.3,-15.99)) ;
#159095=CARTESIAN_POINT('',(-4.75,-6.3,-14.49)) ;
#159096=CARTESIAN_POINT('',(-4.75,-6.3,-14.39)) ;
#159097=CARTESIAN_POINT('',(-4.75,-6.25,-14.49)) ;
#159098=CARTESIAN_POINT('',(-4.75,-6.25,-15.99)) ;
#159099=CARTESIAN_POINT('Origin',(-4.05,-6.25,-14.39)) ;
#159100=CARTESIAN_POINT('',(-4.65,-6.3,-14.39)) ;
#159101=CARTESIAN_POINT('',(-4.65,-6.25,-14.39)) ;
#159102=CARTESIAN_POINT('',(-4.15,-6.3,-14.39)) ;
#159103=CARTESIAN_POINT('',(-4.05,-6.3,-14.39)) ;
#159104=CARTESIAN_POINT('',(-4.15,-6.25,-14.39)) ;
#159105=CARTESIAN_POINT('Origin',(0.,-6.25,-19.05)) ;
#159106=CARTESIAN_POINT('',(-4.8,-6.25,-18.15)) ;
#159107=CARTESIAN_POINT('',(-4.8,-6.25,-19.95)) ;
#159108=CARTESIAN_POINT('',(-4.8,-6.25,-19.05)) ;
#159109=CARTESIAN_POINT('',(-4.,-6.25,-19.95)) ;
#159110=CARTESIAN_POINT('',(1.95156391047391E-16,-6.25,-19.95)) ;
#159111=CARTESIAN_POINT('',(-4.,-6.25,-18.15)) ;
#159112=CARTESIAN_POINT('',(-4.,-6.25,-19.05)) ;
#159113=CARTESIAN_POINT('',(1.9515639104739E-16,-6.25,-18.15)) ;
#159114=CARTESIAN_POINT('',(-4.65,-6.25,-19.9)) ;
#159115=CARTESIAN_POINT('',(-4.15,-6.25,-19.9)) ;
#159116=CARTESIAN_POINT('',(-4.75,-6.25,-19.9)) ;
#159117=CARTESIAN_POINT('',(-4.75,-6.25,-19.8)) ;
#159118=CARTESIAN_POINT('Origin',(-4.65,-6.25,-19.8)) ;
#159119=CARTESIAN_POINT('',(-4.75,-6.25,-18.3)) ;
#159120=CARTESIAN_POINT('',(-4.75,-6.25,-18.2)) ;
#159121=CARTESIAN_POINT('',(-4.65,-6.25,-18.2)) ;
#159122=CARTESIAN_POINT('Origin',(-4.65,-6.25,-18.3)) ;
#159123=CARTESIAN_POINT('',(-4.15,-6.25,-18.2)) ;
#159124=CARTESIAN_POINT('',(-4.05,-6.25,-18.2)) ;
#159125=CARTESIAN_POINT('',(-4.05,-6.25,-18.3)) ;
#159126=CARTESIAN_POINT('Origin',(-4.15,-6.25,-18.3)) ;
#159127=CARTESIAN_POINT('',(-4.05,-6.25,-19.8)) ;
#159128=CARTESIAN_POINT('',(-4.05,-6.25,-19.9)) ;
#159129=CARTESIAN_POINT('Origin',(-4.15,-6.25,-19.8)) ;
#159130=CARTESIAN_POINT('Origin',(-4.05,-6.25,-19.9)) ;
#159131=CARTESIAN_POINT('',(-4.05,-6.3,-18.3)) ;
#159132=CARTESIAN_POINT('',(-4.05,-6.25,-18.3)) ;
#159133=CARTESIAN_POINT('',(-4.05,-6.3,-19.8)) ;
#159134=CARTESIAN_POINT('',(-4.05,-6.3,-19.9)) ;
#159135=CARTESIAN_POINT('',(-4.05,-6.25,-19.8)) ;
#159136=CARTESIAN_POINT('Origin',(-4.75,-6.25,-19.9)) ;
#159137=CARTESIAN_POINT('',(-4.15,-6.3,-19.9)) ;
#159138=CARTESIAN_POINT('',(-4.15,-6.25,-19.9)) ;
#159139=CARTESIAN_POINT('',(-4.65,-6.3,-19.9)) ;
#159140=CARTESIAN_POINT('',(-4.75,-6.3,-19.9)) ;
#159141=CARTESIAN_POINT('',(-4.65,-6.25,-19.9)) ;
#159142=CARTESIAN_POINT('Origin',(-4.75,-6.25,-18.2)) ;
#159143=CARTESIAN_POINT('',(-4.75,-6.3,-19.8)) ;
#159144=CARTESIAN_POINT('',(-4.75,-6.3,-18.3)) ;
#159145=CARTESIAN_POINT('',(-4.75,-6.3,-18.2)) ;
#159146=CARTESIAN_POINT('',(-4.75,-6.25,-18.3)) ;
#159147=CARTESIAN_POINT('',(-4.75,-6.25,-19.8)) ;
#159148=CARTESIAN_POINT('Origin',(-4.05,-6.25,-18.2)) ;
#159149=CARTESIAN_POINT('',(-4.65,-6.3,-18.2)) ;
#159150=CARTESIAN_POINT('',(-4.65,-6.25,-18.2)) ;
#159151=CARTESIAN_POINT('',(-4.15,-6.3,-18.2)) ;
#159152=CARTESIAN_POINT('',(-4.05,-6.3,-18.2)) ;
#159153=CARTESIAN_POINT('',(-4.15,-6.25,-18.2)) ;
#159154=CARTESIAN_POINT('Origin',(0.,-6.25,-22.86)) ;
#159155=CARTESIAN_POINT('',(-4.8,-6.25,-21.96)) ;
#159156=CARTESIAN_POINT('',(-4.8,-6.25,-23.76)) ;
#159157=CARTESIAN_POINT('',(-4.8,-6.25,-22.86)) ;
#159158=CARTESIAN_POINT('',(-4.,-6.25,-23.76)) ;
#159159=CARTESIAN_POINT('',(1.95156391047391E-16,-6.25,-23.76)) ;
#159160=CARTESIAN_POINT('',(-4.,-6.25,-21.96)) ;
#159161=CARTESIAN_POINT('',(-4.,-6.25,-22.86)) ;
#159162=CARTESIAN_POINT('',(1.9515639104739E-16,-6.25,-21.96)) ;
#159163=CARTESIAN_POINT('',(-4.65,-6.25,-23.71)) ;
#159164=CARTESIAN_POINT('',(-4.15,-6.25,-23.71)) ;
#159165=CARTESIAN_POINT('',(-4.75,-6.25,-23.71)) ;
#159166=CARTESIAN_POINT('',(-4.75,-6.25,-23.61)) ;
#159167=CARTESIAN_POINT('Origin',(-4.65,-6.25,-23.61)) ;
#159168=CARTESIAN_POINT('',(-4.75,-6.25,-22.11)) ;
#159169=CARTESIAN_POINT('',(-4.75,-6.25,-22.01)) ;
#159170=CARTESIAN_POINT('',(-4.65,-6.25,-22.01)) ;
#159171=CARTESIAN_POINT('Origin',(-4.65,-6.25,-22.11)) ;
#159172=CARTESIAN_POINT('',(-4.15,-6.25,-22.01)) ;
#159173=CARTESIAN_POINT('',(-4.05,-6.25,-22.01)) ;
#159174=CARTESIAN_POINT('',(-4.05,-6.25,-22.11)) ;
#159175=CARTESIAN_POINT('Origin',(-4.15,-6.25,-22.11)) ;
#159176=CARTESIAN_POINT('',(-4.05,-6.25,-23.61)) ;
#159177=CARTESIAN_POINT('',(-4.05,-6.25,-23.71)) ;
#159178=CARTESIAN_POINT('Origin',(-4.15,-6.25,-23.61)) ;
#159179=CARTESIAN_POINT('Origin',(-4.05,-6.25,-23.71)) ;
#159180=CARTESIAN_POINT('',(-4.05,-6.3,-22.11)) ;
#159181=CARTESIAN_POINT('',(-4.05,-6.25,-22.11)) ;
#159182=CARTESIAN_POINT('',(-4.05,-6.3,-23.61)) ;
#159183=CARTESIAN_POINT('',(-4.05,-6.3,-23.71)) ;
#159184=CARTESIAN_POINT('',(-4.05,-6.25,-23.61)) ;
#159185=CARTESIAN_POINT('Origin',(-4.75,-6.25,-23.71)) ;
#159186=CARTESIAN_POINT('',(-4.15,-6.3,-23.71)) ;
#159187=CARTESIAN_POINT('',(-4.15,-6.25,-23.71)) ;
#159188=CARTESIAN_POINT('',(-4.65,-6.3,-23.71)) ;
#159189=CARTESIAN_POINT('',(-4.75,-6.3,-23.71)) ;
#159190=CARTESIAN_POINT('',(-4.65,-6.25,-23.71)) ;
#159191=CARTESIAN_POINT('Origin',(-4.75,-6.25,-22.01)) ;
#159192=CARTESIAN_POINT('',(-4.75,-6.3,-23.61)) ;
#159193=CARTESIAN_POINT('',(-4.75,-6.3,-22.11)) ;
#159194=CARTESIAN_POINT('',(-4.75,-6.3,-22.01)) ;
#159195=CARTESIAN_POINT('',(-4.75,-6.25,-22.11)) ;
#159196=CARTESIAN_POINT('',(-4.75,-6.25,-23.61)) ;
#159197=CARTESIAN_POINT('Origin',(-4.05,-6.25,-22.01)) ;
#159198=CARTESIAN_POINT('',(-4.65,-6.3,-22.01)) ;
#159199=CARTESIAN_POINT('',(-4.65,-6.25,-22.01)) ;
#159200=CARTESIAN_POINT('',(-4.15,-6.3,-22.01)) ;
#159201=CARTESIAN_POINT('',(-4.05,-6.3,-22.01)) ;
#159202=CARTESIAN_POINT('',(-4.15,-6.25,-22.01)) ;
#159203=CARTESIAN_POINT('Origin',(0.,-6.25,-26.67)) ;
#159204=CARTESIAN_POINT('',(-4.8,-6.25,-25.77)) ;
#159205=CARTESIAN_POINT('',(-4.8,-6.25,-27.57)) ;
#159206=CARTESIAN_POINT('',(-4.8,-6.25,-26.67)) ;
#159207=CARTESIAN_POINT('',(-4.,-6.25,-27.57)) ;
#159208=CARTESIAN_POINT('',(1.95156391047391E-16,-6.25,-27.57)) ;
#159209=CARTESIAN_POINT('',(-4.,-6.25,-25.77)) ;
#159210=CARTESIAN_POINT('',(-4.,-6.25,-26.67)) ;
#159211=CARTESIAN_POINT('',(1.9515639104739E-16,-6.25,-25.77)) ;
#159212=CARTESIAN_POINT('',(-4.65,-6.25,-27.52)) ;
#159213=CARTESIAN_POINT('',(-4.15,-6.25,-27.52)) ;
#159214=CARTESIAN_POINT('',(-4.75,-6.25,-27.52)) ;
#159215=CARTESIAN_POINT('',(-4.75,-6.25,-27.42)) ;
#159216=CARTESIAN_POINT('Origin',(-4.65,-6.25,-27.42)) ;
#159217=CARTESIAN_POINT('',(-4.75,-6.25,-25.92)) ;
#159218=CARTESIAN_POINT('',(-4.75,-6.25,-25.82)) ;
#159219=CARTESIAN_POINT('',(-4.65,-6.25,-25.82)) ;
#159220=CARTESIAN_POINT('Origin',(-4.65,-6.25,-25.92)) ;
#159221=CARTESIAN_POINT('',(-4.15,-6.25,-25.82)) ;
#159222=CARTESIAN_POINT('',(-4.05,-6.25,-25.82)) ;
#159223=CARTESIAN_POINT('',(-4.05,-6.25,-25.92)) ;
#159224=CARTESIAN_POINT('Origin',(-4.15,-6.25,-25.92)) ;
#159225=CARTESIAN_POINT('',(-4.05,-6.25,-27.42)) ;
#159226=CARTESIAN_POINT('',(-4.05,-6.25,-27.52)) ;
#159227=CARTESIAN_POINT('Origin',(-4.15,-6.25,-27.42)) ;
#159228=CARTESIAN_POINT('Origin',(-4.05,-6.25,-27.52)) ;
#159229=CARTESIAN_POINT('',(-4.05,-6.3,-25.92)) ;
#159230=CARTESIAN_POINT('',(-4.05,-6.25,-25.92)) ;
#159231=CARTESIAN_POINT('',(-4.05,-6.3,-27.42)) ;
#159232=CARTESIAN_POINT('',(-4.05,-6.3,-27.52)) ;
#159233=CARTESIAN_POINT('',(-4.05,-6.25,-27.42)) ;
#159234=CARTESIAN_POINT('Origin',(-4.75,-6.25,-27.52)) ;
#159235=CARTESIAN_POINT('',(-4.15,-6.3,-27.52)) ;
#159236=CARTESIAN_POINT('',(-4.15,-6.25,-27.52)) ;
#159237=CARTESIAN_POINT('',(-4.65,-6.3,-27.52)) ;
#159238=CARTESIAN_POINT('',(-4.75,-6.3,-27.52)) ;
#159239=CARTESIAN_POINT('',(-4.65,-6.25,-27.52)) ;
#159240=CARTESIAN_POINT('Origin',(-4.75,-6.25,-25.82)) ;
#159241=CARTESIAN_POINT('',(-4.75,-6.3,-27.42)) ;
#159242=CARTESIAN_POINT('',(-4.75,-6.3,-25.92)) ;
#159243=CARTESIAN_POINT('',(-4.75,-6.3,-25.82)) ;
#159244=CARTESIAN_POINT('',(-4.75,-6.25,-25.92)) ;
#159245=CARTESIAN_POINT('',(-4.75,-6.25,-27.42)) ;
#159246=CARTESIAN_POINT('Origin',(-4.05,-6.25,-25.82)) ;
#159247=CARTESIAN_POINT('',(-4.65,-6.3,-25.82)) ;
#159248=CARTESIAN_POINT('',(-4.65,-6.25,-25.82)) ;
#159249=CARTESIAN_POINT('',(-4.15,-6.3,-25.82)) ;
#159250=CARTESIAN_POINT('',(-4.05,-6.3,-25.82)) ;
#159251=CARTESIAN_POINT('',(-4.15,-6.25,-25.82)) ;
#159252=CARTESIAN_POINT('Origin',(0.,-6.25,-30.48)) ;
#159253=CARTESIAN_POINT('',(-4.8,-6.25,-29.58)) ;
#159254=CARTESIAN_POINT('',(-4.8,-6.25,-31.38)) ;
#159255=CARTESIAN_POINT('',(-4.8,-6.25,-30.48)) ;
#159256=CARTESIAN_POINT('',(-4.,-6.25,-31.38)) ;
#159257=CARTESIAN_POINT('',(1.9515639104739E-16,-6.25,-31.38)) ;
#159258=CARTESIAN_POINT('',(-4.,-6.25,-29.58)) ;
#159259=CARTESIAN_POINT('',(-4.,-6.25,-30.48)) ;
#159260=CARTESIAN_POINT('',(1.9515639104739E-16,-6.25,-29.58)) ;
#159261=CARTESIAN_POINT('',(-4.65,-6.25,-31.33)) ;
#159262=CARTESIAN_POINT('',(-4.15,-6.25,-31.33)) ;
#159263=CARTESIAN_POINT('',(-4.75,-6.25,-31.33)) ;
#159264=CARTESIAN_POINT('',(-4.75,-6.25,-31.23)) ;
#159265=CARTESIAN_POINT('Origin',(-4.65,-6.25,-31.23)) ;
#159266=CARTESIAN_POINT('',(-4.75,-6.25,-29.73)) ;
#159267=CARTESIAN_POINT('',(-4.75,-6.25,-29.63)) ;
#159268=CARTESIAN_POINT('',(-4.65,-6.25,-29.63)) ;
#159269=CARTESIAN_POINT('Origin',(-4.65,-6.25,-29.73)) ;
#159270=CARTESIAN_POINT('',(-4.15,-6.25,-29.63)) ;
#159271=CARTESIAN_POINT('',(-4.05,-6.25,-29.63)) ;
#159272=CARTESIAN_POINT('',(-4.05,-6.25,-29.73)) ;
#159273=CARTESIAN_POINT('Origin',(-4.15,-6.25,-29.73)) ;
#159274=CARTESIAN_POINT('',(-4.05,-6.25,-31.23)) ;
#159275=CARTESIAN_POINT('',(-4.05,-6.25,-31.33)) ;
#159276=CARTESIAN_POINT('Origin',(-4.15,-6.25,-31.23)) ;
#159277=CARTESIAN_POINT('Origin',(-4.05,-6.25,-31.33)) ;
#159278=CARTESIAN_POINT('',(-4.05,-6.3,-29.73)) ;
#159279=CARTESIAN_POINT('',(-4.05,-6.25,-29.73)) ;
#159280=CARTESIAN_POINT('',(-4.05,-6.3,-31.23)) ;
#159281=CARTESIAN_POINT('',(-4.05,-6.3,-31.33)) ;
#159282=CARTESIAN_POINT('',(-4.05,-6.25,-31.23)) ;
#159283=CARTESIAN_POINT('Origin',(-4.75,-6.25,-31.33)) ;
#159284=CARTESIAN_POINT('',(-4.15,-6.3,-31.33)) ;
#159285=CARTESIAN_POINT('',(-4.15,-6.25,-31.33)) ;
#159286=CARTESIAN_POINT('',(-4.65,-6.3,-31.33)) ;
#159287=CARTESIAN_POINT('',(-4.75,-6.3,-31.33)) ;
#159288=CARTESIAN_POINT('',(-4.65,-6.25,-31.33)) ;
#159289=CARTESIAN_POINT('Origin',(-4.75,-6.25,-29.63)) ;
#159290=CARTESIAN_POINT('',(-4.75,-6.3,-31.23)) ;
#159291=CARTESIAN_POINT('',(-4.75,-6.3,-29.73)) ;
#159292=CARTESIAN_POINT('',(-4.75,-6.3,-29.63)) ;
#159293=CARTESIAN_POINT('',(-4.75,-6.25,-29.73)) ;
#159294=CARTESIAN_POINT('',(-4.75,-6.25,-31.23)) ;
#159295=CARTESIAN_POINT('Origin',(-4.05,-6.25,-29.63)) ;
#159296=CARTESIAN_POINT('',(-4.65,-6.3,-29.63)) ;
#159297=CARTESIAN_POINT('',(-4.65,-6.25,-29.63)) ;
#159298=CARTESIAN_POINT('',(-4.15,-6.3,-29.63)) ;
#159299=CARTESIAN_POINT('',(-4.05,-6.3,-29.63)) ;
#159300=CARTESIAN_POINT('',(-4.15,-6.25,-29.63)) ;
#159301=CARTESIAN_POINT('Origin',(0.,-6.25,-34.29)) ;
#159302=CARTESIAN_POINT('',(-4.8,-6.25,-33.39)) ;
#159303=CARTESIAN_POINT('',(-4.8,-6.25,-35.19)) ;
#159304=CARTESIAN_POINT('',(-4.8,-6.25,-34.29)) ;
#159305=CARTESIAN_POINT('',(-4.,-6.25,-35.19)) ;
#159306=CARTESIAN_POINT('',(1.9515639104739E-16,-6.25,-35.19)) ;
#159307=CARTESIAN_POINT('',(-4.,-6.25,-33.39)) ;
#159308=CARTESIAN_POINT('',(-4.,-6.25,-34.29)) ;
#159309=CARTESIAN_POINT('',(1.9515639104739E-16,-6.25,-33.39)) ;
#159310=CARTESIAN_POINT('',(-4.65,-6.25,-35.14)) ;
#159311=CARTESIAN_POINT('',(-4.15,-6.25,-35.14)) ;
#159312=CARTESIAN_POINT('',(-4.75,-6.25,-35.14)) ;
#159313=CARTESIAN_POINT('',(-4.75,-6.25,-35.04)) ;
#159314=CARTESIAN_POINT('Origin',(-4.65,-6.25,-35.04)) ;
#159315=CARTESIAN_POINT('',(-4.75,-6.25,-33.54)) ;
#159316=CARTESIAN_POINT('',(-4.75,-6.25,-33.44)) ;
#159317=CARTESIAN_POINT('',(-4.65,-6.25,-33.44)) ;
#159318=CARTESIAN_POINT('Origin',(-4.65,-6.25,-33.54)) ;
#159319=CARTESIAN_POINT('',(-4.15,-6.25,-33.44)) ;
#159320=CARTESIAN_POINT('',(-4.05,-6.25,-33.44)) ;
#159321=CARTESIAN_POINT('',(-4.05,-6.25,-33.54)) ;
#159322=CARTESIAN_POINT('Origin',(-4.15,-6.25,-33.54)) ;
#159323=CARTESIAN_POINT('',(-4.05,-6.25,-35.04)) ;
#159324=CARTESIAN_POINT('',(-4.05,-6.25,-35.14)) ;
#159325=CARTESIAN_POINT('Origin',(-4.15,-6.25,-35.04)) ;
#159326=CARTESIAN_POINT('Origin',(-4.05,-6.25,-35.14)) ;
#159327=CARTESIAN_POINT('',(-4.05,-6.3,-33.54)) ;
#159328=CARTESIAN_POINT('',(-4.05,-6.25,-33.54)) ;
#159329=CARTESIAN_POINT('',(-4.05,-6.3,-35.04)) ;
#159330=CARTESIAN_POINT('',(-4.05,-6.3,-35.14)) ;
#159331=CARTESIAN_POINT('',(-4.05,-6.25,-35.04)) ;
#159332=CARTESIAN_POINT('Origin',(-4.75,-6.25,-35.14)) ;
#159333=CARTESIAN_POINT('',(-4.15,-6.3,-35.14)) ;
#159334=CARTESIAN_POINT('',(-4.15,-6.25,-35.14)) ;
#159335=CARTESIAN_POINT('',(-4.65,-6.3,-35.14)) ;
#159336=CARTESIAN_POINT('',(-4.75,-6.3,-35.14)) ;
#159337=CARTESIAN_POINT('',(-4.65,-6.25,-35.14)) ;
#159338=CARTESIAN_POINT('Origin',(-4.75,-6.25,-33.44)) ;
#159339=CARTESIAN_POINT('',(-4.75,-6.3,-35.04)) ;
#159340=CARTESIAN_POINT('',(-4.75,-6.3,-33.54)) ;
#159341=CARTESIAN_POINT('',(-4.75,-6.3,-33.44)) ;
#159342=CARTESIAN_POINT('',(-4.75,-6.25,-33.54)) ;
#159343=CARTESIAN_POINT('',(-4.75,-6.25,-35.04)) ;
#159344=CARTESIAN_POINT('Origin',(-4.05,-6.25,-33.44)) ;
#159345=CARTESIAN_POINT('',(-4.65,-6.3,-33.44)) ;
#159346=CARTESIAN_POINT('',(-4.65,-6.25,-33.44)) ;
#159347=CARTESIAN_POINT('',(-4.15,-6.3,-33.44)) ;
#159348=CARTESIAN_POINT('',(-4.05,-6.3,-33.44)) ;
#159349=CARTESIAN_POINT('',(-4.15,-6.25,-33.44)) ;
#159350=CARTESIAN_POINT('Origin',(0.,-6.4,-3.81)) ;
#159351=CARTESIAN_POINT('',(-4.15,-6.4,-3.06)) ;
#159352=CARTESIAN_POINT('',(-4.65,-6.4,-3.06)) ;
#159353=CARTESIAN_POINT('',(0.,-6.4,-3.06)) ;
#159354=CARTESIAN_POINT('',(-4.65,-6.4,-4.56)) ;
#159355=CARTESIAN_POINT('',(-4.65,-6.4,-3.81)) ;
#159356=CARTESIAN_POINT('',(-4.15,-6.4,-4.56)) ;
#159357=CARTESIAN_POINT('',(0.,-6.4,-4.56)) ;
#159358=CARTESIAN_POINT('',(-4.15,-6.4,-3.81)) ;
#159359=CARTESIAN_POINT('Origin',(0.,-6.4,-7.62)) ;
#159360=CARTESIAN_POINT('',(-4.15,-6.4,-6.87)) ;
#159361=CARTESIAN_POINT('',(-4.65,-6.4,-6.87)) ;
#159362=CARTESIAN_POINT('',(0.,-6.4,-6.87)) ;
#159363=CARTESIAN_POINT('',(-4.65,-6.4,-8.37)) ;
#159364=CARTESIAN_POINT('',(-4.65,-6.4,-7.62)) ;
#159365=CARTESIAN_POINT('',(-4.15,-6.4,-8.37)) ;
#159366=CARTESIAN_POINT('',(0.,-6.4,-8.37)) ;
#159367=CARTESIAN_POINT('',(-4.15,-6.4,-7.62)) ;
#159368=CARTESIAN_POINT('Origin',(0.,-6.4,-11.43)) ;
#159369=CARTESIAN_POINT('',(-4.15,-6.4,-10.68)) ;
#159370=CARTESIAN_POINT('',(-4.65,-6.4,-10.68)) ;
#159371=CARTESIAN_POINT('',(0.,-6.4,-10.68)) ;
#159372=CARTESIAN_POINT('',(-4.65,-6.4,-12.18)) ;
#159373=CARTESIAN_POINT('',(-4.65,-6.4,-11.43)) ;
#159374=CARTESIAN_POINT('',(-4.15,-6.4,-12.18)) ;
#159375=CARTESIAN_POINT('',(0.,-6.4,-12.18)) ;
#159376=CARTESIAN_POINT('',(-4.15,-6.4,-11.43)) ;
#159377=CARTESIAN_POINT('Origin',(0.,-6.4,-15.24)) ;
#159378=CARTESIAN_POINT('',(-4.15,-6.4,-14.49)) ;
#159379=CARTESIAN_POINT('',(-4.65,-6.4,-14.49)) ;
#159380=CARTESIAN_POINT('',(0.,-6.4,-14.49)) ;
#159381=CARTESIAN_POINT('',(-4.65,-6.4,-15.99)) ;
#159382=CARTESIAN_POINT('',(-4.65,-6.4,-15.24)) ;
#159383=CARTESIAN_POINT('',(-4.15,-6.4,-15.99)) ;
#159384=CARTESIAN_POINT('',(0.,-6.4,-15.99)) ;
#159385=CARTESIAN_POINT('',(-4.15,-6.4,-15.24)) ;
#159386=CARTESIAN_POINT('Origin',(0.,-6.4,-19.05)) ;
#159387=CARTESIAN_POINT('',(-4.15,-6.4,-18.3)) ;
#159388=CARTESIAN_POINT('',(-4.65,-6.4,-18.3)) ;
#159389=CARTESIAN_POINT('',(0.,-6.4,-18.3)) ;
#159390=CARTESIAN_POINT('',(-4.65,-6.4,-19.8)) ;
#159391=CARTESIAN_POINT('',(-4.65,-6.4,-19.05)) ;
#159392=CARTESIAN_POINT('',(-4.15,-6.4,-19.8)) ;
#159393=CARTESIAN_POINT('',(0.,-6.4,-19.8)) ;
#159394=CARTESIAN_POINT('',(-4.15,-6.4,-19.05)) ;
#159395=CARTESIAN_POINT('Origin',(0.,-6.4,-22.86)) ;
#159396=CARTESIAN_POINT('',(-4.15,-6.4,-22.11)) ;
#159397=CARTESIAN_POINT('',(-4.65,-6.4,-22.11)) ;
#159398=CARTESIAN_POINT('',(0.,-6.4,-22.11)) ;
#159399=CARTESIAN_POINT('',(-4.65,-6.4,-23.61)) ;
#159400=CARTESIAN_POINT('',(-4.65,-6.4,-22.86)) ;
#159401=CARTESIAN_POINT('',(-4.15,-6.4,-23.61)) ;
#159402=CARTESIAN_POINT('',(0.,-6.4,-23.61)) ;
#159403=CARTESIAN_POINT('',(-4.15,-6.4,-22.86)) ;
#159404=CARTESIAN_POINT('Origin',(0.,-6.4,-26.67)) ;
#159405=CARTESIAN_POINT('',(-4.15,-6.4,-25.92)) ;
#159406=CARTESIAN_POINT('',(-4.65,-6.4,-25.92)) ;
#159407=CARTESIAN_POINT('',(0.,-6.4,-25.92)) ;
#159408=CARTESIAN_POINT('',(-4.65,-6.4,-27.42)) ;
#159409=CARTESIAN_POINT('',(-4.65,-6.4,-26.67)) ;
#159410=CARTESIAN_POINT('',(-4.15,-6.4,-27.42)) ;
#159411=CARTESIAN_POINT('',(0.,-6.4,-27.42)) ;
#159412=CARTESIAN_POINT('',(-4.15,-6.4,-26.67)) ;
#159413=CARTESIAN_POINT('Origin',(0.,-6.4,-30.48)) ;
#159414=CARTESIAN_POINT('',(-4.15,-6.4,-29.73)) ;
#159415=CARTESIAN_POINT('',(-4.65,-6.4,-29.73)) ;
#159416=CARTESIAN_POINT('',(0.,-6.4,-29.73)) ;
#159417=CARTESIAN_POINT('',(-4.65,-6.4,-31.23)) ;
#159418=CARTESIAN_POINT('',(-4.65,-6.4,-30.48)) ;
#159419=CARTESIAN_POINT('',(-4.15,-6.4,-31.23)) ;
#159420=CARTESIAN_POINT('',(0.,-6.4,-31.23)) ;
#159421=CARTESIAN_POINT('',(-4.15,-6.4,-30.48)) ;
#159422=CARTESIAN_POINT('Origin',(0.,-6.4,-34.29)) ;
#159423=CARTESIAN_POINT('',(-4.15,-6.4,-33.54)) ;
#159424=CARTESIAN_POINT('',(-4.65,-6.4,-33.54)) ;
#159425=CARTESIAN_POINT('',(0.,-6.4,-33.54)) ;
#159426=CARTESIAN_POINT('',(-4.65,-6.4,-35.04)) ;
#159427=CARTESIAN_POINT('',(-4.65,-6.4,-34.29)) ;
#159428=CARTESIAN_POINT('',(-4.15,-6.4,-35.04)) ;
#159429=CARTESIAN_POINT('',(0.,-6.4,-35.04)) ;
#159430=CARTESIAN_POINT('',(-4.15,-6.4,-34.29)) ;
#159431=CARTESIAN_POINT('Origin',(3.6,2.,-2.405)) ;
#159432=CARTESIAN_POINT('',(3.7,1.9,-2.405)) ;
#159433=CARTESIAN_POINT('',(3.6,1.92679491924311,-2.405)) ;
#159434=CARTESIAN_POINT('Origin',(3.7,2.1,-2.405)) ;
#159435=CARTESIAN_POINT('',(3.5,1.9,-2.405)) ;
#159436=CARTESIAN_POINT('Origin',(3.5,2.1,-2.405)) ;
#159437=CARTESIAN_POINT('',(2.7,1.9,-2.405)) ;
#159438=CARTESIAN_POINT('',(2.6,1.9,-2.405)) ;
#159439=CARTESIAN_POINT('',(2.7,-5.15,-2.405)) ;
#159440=CARTESIAN_POINT('',(2.7,2.,-2.405)) ;
#159441=CARTESIAN_POINT('',(3.5,-5.15,-2.405)) ;
#159442=CARTESIAN_POINT('',(3.6,-5.15,-2.405)) ;
#159443=CARTESIAN_POINT('',(3.5,-2.35,-2.405)) ;
#159444=CARTESIAN_POINT('',(3.5,-2.25,-2.405)) ;
#159445=CARTESIAN_POINT('',(3.7,-2.15,-2.405)) ;
#159446=CARTESIAN_POINT('Origin',(3.7,-2.35,-2.405)) ;
#159447=CARTESIAN_POINT('',(10.1,-2.15,-2.405)) ;
#159448=CARTESIAN_POINT('',(3.6,-2.15,-2.405)) ;
#159449=CARTESIAN_POINT('',(10.1,1.9,-2.405)) ;
#159450=CARTESIAN_POINT('',(10.1,2.,-2.405)) ;
#159451=CARTESIAN_POINT('',(3.6,1.9,-2.405)) ;
#159452=CARTESIAN_POINT('Origin',(3.6,-5.25,-2.405)) ;
#159453=CARTESIAN_POINT('',(3.5,-5.25,-2.505)) ;
#159454=CARTESIAN_POINT('',(2.7,-5.25,-2.505)) ;
#159455=CARTESIAN_POINT('',(3.6,-5.25,-2.505)) ;
#159456=CARTESIAN_POINT('',(2.7,-5.25,-5.115)) ;
#159457=CARTESIAN_POINT('',(2.7,-5.25,-2.405)) ;
#159458=CARTESIAN_POINT('',(3.5,-5.25,-5.115)) ;
#159459=CARTESIAN_POINT('',(3.6,-5.25,-5.115)) ;
#159460=CARTESIAN_POINT('',(3.5,-5.25,-2.405)) ;
#159461=CARTESIAN_POINT('Origin',(3.6,-5.25,-5.215)) ;
#159462=CARTESIAN_POINT('',(2.7,1.9,-5.215)) ;
#159463=CARTESIAN_POINT('',(3.5,1.9,-5.215)) ;
#159464=CARTESIAN_POINT('',(3.6,1.9,-5.215)) ;
#159465=CARTESIAN_POINT('',(3.6,1.92679491924311,-5.215)) ;
#159466=CARTESIAN_POINT('Origin',(3.5,2.1,-5.215)) ;
#159467=CARTESIAN_POINT('',(3.7,1.9,-5.215)) ;
#159468=CARTESIAN_POINT('Origin',(3.7,2.1,-5.215)) ;
#159469=CARTESIAN_POINT('',(10.1,1.9,-5.215)) ;
#159470=CARTESIAN_POINT('',(3.6,1.9,-5.215)) ;
#159471=CARTESIAN_POINT('',(10.1,-2.15,-5.215)) ;
#159472=CARTESIAN_POINT('',(10.1,-2.25,-5.215)) ;
#159473=CARTESIAN_POINT('',(3.7,-2.15,-5.215)) ;
#159474=CARTESIAN_POINT('',(3.6,-2.15,-5.215)) ;
#159475=CARTESIAN_POINT('',(3.5,-2.35,-5.215)) ;
#159476=CARTESIAN_POINT('Origin',(3.7,-2.35,-5.215)) ;
#159477=CARTESIAN_POINT('',(3.5,-5.15,-5.215)) ;
#159478=CARTESIAN_POINT('',(3.5,-5.25,-5.215)) ;
#159479=CARTESIAN_POINT('',(2.7,-5.15,-5.215)) ;
#159480=CARTESIAN_POINT('',(3.6,-5.15,-5.215)) ;
#159481=CARTESIAN_POINT('',(2.7,-5.25,-5.215)) ;
#159482=CARTESIAN_POINT('Origin',(3.6,2.,-5.215)) ;
#159483=CARTESIAN_POINT('',(2.7,2.,-6.115)) ;
#159484=CARTESIAN_POINT('',(3.5,2.,-6.115)) ;
#159485=CARTESIAN_POINT('',(3.6,2.,-6.115)) ;
#159486=CARTESIAN_POINT('',(3.5,2.,-5.315)) ;
#159487=CARTESIAN_POINT('',(3.5,2.,-5.315)) ;
#159488=CARTESIAN_POINT('',(2.7,2.,-5.315)) ;
#159489=CARTESIAN_POINT('',(2.6,2.,-5.315)) ;
#159490=CARTESIAN_POINT('',(2.7,2.,-5.215)) ;
#159491=CARTESIAN_POINT('Origin',(3.6,2.,-6.215)) ;
#159492=CARTESIAN_POINT('',(3.7,1.9,-6.215)) ;
#159493=CARTESIAN_POINT('',(3.6,1.92679491924311,-6.215)) ;
#159494=CARTESIAN_POINT('Origin',(3.7,2.1,-6.215)) ;
#159495=CARTESIAN_POINT('',(3.5,1.9,-6.215)) ;
#159496=CARTESIAN_POINT('Origin',(3.5,2.1,-6.215)) ;
#159497=CARTESIAN_POINT('',(2.7,1.9,-6.215)) ;
#159498=CARTESIAN_POINT('',(2.7,1.9,-6.215)) ;
#159499=CARTESIAN_POINT('',(2.7,-5.15,-6.215)) ;
#159500=CARTESIAN_POINT('',(2.7,2.,-6.215)) ;
#159501=CARTESIAN_POINT('',(3.5,-5.15,-6.215)) ;
#159502=CARTESIAN_POINT('',(3.6,-5.15,-6.215)) ;
#159503=CARTESIAN_POINT('',(3.5,-2.35,-6.215)) ;
#159504=CARTESIAN_POINT('',(3.5,-2.25,-6.215)) ;
#159505=CARTESIAN_POINT('',(3.7,-2.15,-6.215)) ;
#159506=CARTESIAN_POINT('Origin',(3.7,-2.35,-6.215)) ;
#159507=CARTESIAN_POINT('',(10.1,-2.15,-6.215)) ;
#159508=CARTESIAN_POINT('',(3.6,-2.15,-6.215)) ;
#159509=CARTESIAN_POINT('',(10.1,1.9,-6.215)) ;
#159510=CARTESIAN_POINT('',(10.1,2.,-6.215)) ;
#159511=CARTESIAN_POINT('',(3.6,1.9,-6.215)) ;
#159512=CARTESIAN_POINT('Origin',(3.6,-5.25,-6.215)) ;
#159513=CARTESIAN_POINT('',(3.5,-5.25,-6.315)) ;
#159514=CARTESIAN_POINT('',(2.7,-5.25,-6.315)) ;
#159515=CARTESIAN_POINT('',(3.6,-5.25,-6.315)) ;
#159516=CARTESIAN_POINT('',(2.7,-5.25,-8.925)) ;
#159517=CARTESIAN_POINT('',(2.7,-5.25,-6.215)) ;
#159518=CARTESIAN_POINT('',(3.5,-5.25,-8.925)) ;
#159519=CARTESIAN_POINT('',(3.6,-5.25,-8.925)) ;
#159520=CARTESIAN_POINT('',(3.5,-5.25,-6.215)) ;
#159521=CARTESIAN_POINT('Origin',(3.6,-5.25,-9.025)) ;
#159522=CARTESIAN_POINT('',(2.7,1.9,-9.025)) ;
#159523=CARTESIAN_POINT('',(3.5,1.9,-9.025)) ;
#159524=CARTESIAN_POINT('',(3.6,1.9,-9.025)) ;
#159525=CARTESIAN_POINT('',(3.6,1.92679491924311,-9.025)) ;
#159526=CARTESIAN_POINT('Origin',(3.5,2.1,-9.025)) ;
#159527=CARTESIAN_POINT('',(3.7,1.9,-9.025)) ;
#159528=CARTESIAN_POINT('Origin',(3.7,2.1,-9.025)) ;
#159529=CARTESIAN_POINT('',(10.1,1.9,-9.025)) ;
#159530=CARTESIAN_POINT('',(3.6,1.9,-9.025)) ;
#159531=CARTESIAN_POINT('',(10.1,-2.15,-9.025)) ;
#159532=CARTESIAN_POINT('',(10.1,-2.25,-9.025)) ;
#159533=CARTESIAN_POINT('',(3.7,-2.15,-9.025)) ;
#159534=CARTESIAN_POINT('',(3.6,-2.15,-9.025)) ;
#159535=CARTESIAN_POINT('',(3.5,-2.35,-9.025)) ;
#159536=CARTESIAN_POINT('Origin',(3.7,-2.35,-9.025)) ;
#159537=CARTESIAN_POINT('',(3.5,-5.15,-9.025)) ;
#159538=CARTESIAN_POINT('',(3.5,-5.25,-9.025)) ;
#159539=CARTESIAN_POINT('',(2.7,-5.15,-9.025)) ;
#159540=CARTESIAN_POINT('',(3.6,-5.15,-9.025)) ;
#159541=CARTESIAN_POINT('',(2.7,-5.25,-9.025)) ;
#159542=CARTESIAN_POINT('Origin',(3.6,2.,-9.025)) ;
#159543=CARTESIAN_POINT('',(2.7,2.,-9.925)) ;
#159544=CARTESIAN_POINT('',(3.5,2.,-9.925)) ;
#159545=CARTESIAN_POINT('',(3.6,2.,-9.925)) ;
#159546=CARTESIAN_POINT('',(3.5,2.,-9.125)) ;
#159547=CARTESIAN_POINT('',(3.5,2.,-9.125)) ;
#159548=CARTESIAN_POINT('',(2.7,2.,-9.125)) ;
#159549=CARTESIAN_POINT('',(2.6,2.,-9.125)) ;
#159550=CARTESIAN_POINT('',(2.7,2.,-9.025)) ;
#159551=CARTESIAN_POINT('Origin',(3.6,2.,-10.025)) ;
#159552=CARTESIAN_POINT('',(3.7,1.9,-10.025)) ;
#159553=CARTESIAN_POINT('',(3.6,1.92679491924311,-10.025)) ;
#159554=CARTESIAN_POINT('Origin',(3.7,2.1,-10.025)) ;
#159555=CARTESIAN_POINT('',(3.5,1.9,-10.025)) ;
#159556=CARTESIAN_POINT('Origin',(3.5,2.1,-10.025)) ;
#159557=CARTESIAN_POINT('',(2.7,1.9,-10.025)) ;
#159558=CARTESIAN_POINT('',(2.7,1.9,-10.025)) ;
#159559=CARTESIAN_POINT('',(2.7,-5.15,-10.025)) ;
#159560=CARTESIAN_POINT('',(2.7,2.,-10.025)) ;
#159561=CARTESIAN_POINT('',(3.5,-5.15,-10.025)) ;
#159562=CARTESIAN_POINT('',(3.6,-5.15,-10.025)) ;
#159563=CARTESIAN_POINT('',(3.5,-2.35,-10.025)) ;
#159564=CARTESIAN_POINT('',(3.5,-2.25,-10.025)) ;
#159565=CARTESIAN_POINT('',(3.7,-2.15,-10.025)) ;
#159566=CARTESIAN_POINT('Origin',(3.7,-2.35,-10.025)) ;
#159567=CARTESIAN_POINT('',(10.1,-2.15,-10.025)) ;
#159568=CARTESIAN_POINT('',(3.6,-2.15,-10.025)) ;
#159569=CARTESIAN_POINT('',(10.1,1.9,-10.025)) ;
#159570=CARTESIAN_POINT('',(10.1,2.,-10.025)) ;
#159571=CARTESIAN_POINT('',(3.6,1.9,-10.025)) ;
#159572=CARTESIAN_POINT('Origin',(3.6,-5.25,-10.025)) ;
#159573=CARTESIAN_POINT('',(3.5,-5.25,-10.125)) ;
#159574=CARTESIAN_POINT('',(2.7,-5.25,-10.125)) ;
#159575=CARTESIAN_POINT('',(3.6,-5.25,-10.125)) ;
#159576=CARTESIAN_POINT('',(2.7,-5.25,-12.735)) ;
#159577=CARTESIAN_POINT('',(2.7,-5.25,-10.025)) ;
#159578=CARTESIAN_POINT('',(3.5,-5.25,-12.735)) ;
#159579=CARTESIAN_POINT('',(3.6,-5.25,-12.735)) ;
#159580=CARTESIAN_POINT('',(3.5,-5.25,-10.025)) ;
#159581=CARTESIAN_POINT('Origin',(3.6,-5.25,-12.835)) ;
#159582=CARTESIAN_POINT('',(2.7,1.9,-12.835)) ;
#159583=CARTESIAN_POINT('',(3.5,1.9,-12.835)) ;
#159584=CARTESIAN_POINT('',(3.6,1.9,-12.835)) ;
#159585=CARTESIAN_POINT('',(3.6,1.92679491924311,-12.835)) ;
#159586=CARTESIAN_POINT('Origin',(3.5,2.1,-12.835)) ;
#159587=CARTESIAN_POINT('',(3.7,1.9,-12.835)) ;
#159588=CARTESIAN_POINT('Origin',(3.7,2.1,-12.835)) ;
#159589=CARTESIAN_POINT('',(10.1,1.9,-12.835)) ;
#159590=CARTESIAN_POINT('',(3.6,1.9,-12.835)) ;
#159591=CARTESIAN_POINT('',(10.1,-2.15,-12.835)) ;
#159592=CARTESIAN_POINT('',(10.1,-2.25,-12.835)) ;
#159593=CARTESIAN_POINT('',(3.7,-2.15,-12.835)) ;
#159594=CARTESIAN_POINT('',(3.6,-2.15,-12.835)) ;
#159595=CARTESIAN_POINT('',(3.5,-2.35,-12.835)) ;
#159596=CARTESIAN_POINT('Origin',(3.7,-2.35,-12.835)) ;
#159597=CARTESIAN_POINT('',(3.5,-5.15,-12.835)) ;
#159598=CARTESIAN_POINT('',(3.5,-5.25,-12.835)) ;
#159599=CARTESIAN_POINT('',(2.7,-5.15,-12.835)) ;
#159600=CARTESIAN_POINT('',(3.6,-5.15,-12.835)) ;
#159601=CARTESIAN_POINT('',(2.7,-5.25,-12.835)) ;
#159602=CARTESIAN_POINT('Origin',(3.6,2.,-12.835)) ;
#159603=CARTESIAN_POINT('',(2.7,2.,-13.735)) ;
#159604=CARTESIAN_POINT('',(3.5,2.,-13.735)) ;
#159605=CARTESIAN_POINT('',(3.6,2.,-13.735)) ;
#159606=CARTESIAN_POINT('',(3.5,2.,-12.935)) ;
#159607=CARTESIAN_POINT('',(3.5,2.,-12.935)) ;
#159608=CARTESIAN_POINT('',(2.7,2.,-12.935)) ;
#159609=CARTESIAN_POINT('',(2.6,2.,-12.935)) ;
#159610=CARTESIAN_POINT('',(2.7,2.,-12.835)) ;
#159611=CARTESIAN_POINT('Origin',(3.6,2.,-13.835)) ;
#159612=CARTESIAN_POINT('',(3.7,1.9,-13.835)) ;
#159613=CARTESIAN_POINT('',(3.6,1.92679491924311,-13.835)) ;
#159614=CARTESIAN_POINT('Origin',(3.7,2.1,-13.835)) ;
#159615=CARTESIAN_POINT('',(3.5,1.9,-13.835)) ;
#159616=CARTESIAN_POINT('Origin',(3.5,2.1,-13.835)) ;
#159617=CARTESIAN_POINT('',(2.7,1.9,-13.835)) ;
#159618=CARTESIAN_POINT('',(2.7,1.9,-13.835)) ;
#159619=CARTESIAN_POINT('',(2.7,-5.15,-13.835)) ;
#159620=CARTESIAN_POINT('',(2.7,2.,-13.835)) ;
#159621=CARTESIAN_POINT('',(3.5,-5.15,-13.835)) ;
#159622=CARTESIAN_POINT('',(3.6,-5.15,-13.835)) ;
#159623=CARTESIAN_POINT('',(3.5,-2.35,-13.835)) ;
#159624=CARTESIAN_POINT('',(3.5,-2.25,-13.835)) ;
#159625=CARTESIAN_POINT('',(3.7,-2.15,-13.835)) ;
#159626=CARTESIAN_POINT('Origin',(3.7,-2.35,-13.835)) ;
#159627=CARTESIAN_POINT('',(10.1,-2.15,-13.835)) ;
#159628=CARTESIAN_POINT('',(3.6,-2.15,-13.835)) ;
#159629=CARTESIAN_POINT('',(10.1,1.9,-13.835)) ;
#159630=CARTESIAN_POINT('',(10.1,2.,-13.835)) ;
#159631=CARTESIAN_POINT('',(3.6,1.9,-13.835)) ;
#159632=CARTESIAN_POINT('Origin',(3.6,-5.25,-13.835)) ;
#159633=CARTESIAN_POINT('',(3.5,-5.25,-13.935)) ;
#159634=CARTESIAN_POINT('',(2.7,-5.25,-13.935)) ;
#159635=CARTESIAN_POINT('',(3.6,-5.25,-13.935)) ;
#159636=CARTESIAN_POINT('',(2.7,-5.25,-16.545)) ;
#159637=CARTESIAN_POINT('',(2.7,-5.25,-13.835)) ;
#159638=CARTESIAN_POINT('',(3.5,-5.25,-16.545)) ;
#159639=CARTESIAN_POINT('',(3.6,-5.25,-16.545)) ;
#159640=CARTESIAN_POINT('',(3.5,-5.25,-13.835)) ;
#159641=CARTESIAN_POINT('Origin',(3.6,-5.25,-16.645)) ;
#159642=CARTESIAN_POINT('',(2.7,1.9,-16.645)) ;
#159643=CARTESIAN_POINT('',(3.5,1.9,-16.645)) ;
#159644=CARTESIAN_POINT('',(3.6,1.9,-16.645)) ;
#159645=CARTESIAN_POINT('',(3.6,1.92679491924311,-16.645)) ;
#159646=CARTESIAN_POINT('Origin',(3.5,2.1,-16.645)) ;
#159647=CARTESIAN_POINT('',(3.7,1.9,-16.645)) ;
#159648=CARTESIAN_POINT('Origin',(3.7,2.1,-16.645)) ;
#159649=CARTESIAN_POINT('',(10.1,1.9,-16.645)) ;
#159650=CARTESIAN_POINT('',(3.6,1.9,-16.645)) ;
#159651=CARTESIAN_POINT('',(10.1,-2.15,-16.645)) ;
#159652=CARTESIAN_POINT('',(10.1,-2.25,-16.645)) ;
#159653=CARTESIAN_POINT('',(3.7,-2.15,-16.645)) ;
#159654=CARTESIAN_POINT('',(3.6,-2.15,-16.645)) ;
#159655=CARTESIAN_POINT('',(3.5,-2.35,-16.645)) ;
#159656=CARTESIAN_POINT('Origin',(3.7,-2.35,-16.645)) ;
#159657=CARTESIAN_POINT('',(3.5,-5.15,-16.645)) ;
#159658=CARTESIAN_POINT('',(3.5,-5.25,-16.645)) ;
#159659=CARTESIAN_POINT('',(2.7,-5.15,-16.645)) ;
#159660=CARTESIAN_POINT('',(3.6,-5.15,-16.645)) ;
#159661=CARTESIAN_POINT('',(2.7,-5.25,-16.645)) ;
#159662=CARTESIAN_POINT('Origin',(3.6,2.,-16.645)) ;
#159663=CARTESIAN_POINT('',(2.7,2.,-17.545)) ;
#159664=CARTESIAN_POINT('',(3.5,2.,-17.545)) ;
#159665=CARTESIAN_POINT('',(3.6,2.,-17.545)) ;
#159666=CARTESIAN_POINT('',(3.5,2.,-16.745)) ;
#159667=CARTESIAN_POINT('',(3.5,2.,-16.745)) ;
#159668=CARTESIAN_POINT('',(2.7,2.,-16.745)) ;
#159669=CARTESIAN_POINT('',(2.6,2.,-16.745)) ;
#159670=CARTESIAN_POINT('',(2.7,2.,-16.645)) ;
#159671=CARTESIAN_POINT('Origin',(3.6,2.,-17.645)) ;
#159672=CARTESIAN_POINT('',(3.7,1.9,-17.645)) ;
#159673=CARTESIAN_POINT('',(3.6,1.92679491924311,-17.645)) ;
#159674=CARTESIAN_POINT('Origin',(3.7,2.1,-17.645)) ;
#159675=CARTESIAN_POINT('',(3.5,1.9,-17.645)) ;
#159676=CARTESIAN_POINT('Origin',(3.5,2.1,-17.645)) ;
#159677=CARTESIAN_POINT('',(2.7,1.9,-17.645)) ;
#159678=CARTESIAN_POINT('',(2.7,1.9,-17.645)) ;
#159679=CARTESIAN_POINT('',(2.7,-5.15,-17.645)) ;
#159680=CARTESIAN_POINT('',(2.7,2.,-17.645)) ;
#159681=CARTESIAN_POINT('',(3.5,-5.15,-17.645)) ;
#159682=CARTESIAN_POINT('',(3.6,-5.15,-17.645)) ;
#159683=CARTESIAN_POINT('',(3.5,-2.35,-17.645)) ;
#159684=CARTESIAN_POINT('',(3.5,-2.25,-17.645)) ;
#159685=CARTESIAN_POINT('',(3.7,-2.15,-17.645)) ;
#159686=CARTESIAN_POINT('Origin',(3.7,-2.35,-17.645)) ;
#159687=CARTESIAN_POINT('',(10.1,-2.15,-17.645)) ;
#159688=CARTESIAN_POINT('',(3.6,-2.15,-17.645)) ;
#159689=CARTESIAN_POINT('',(10.1,1.9,-17.645)) ;
#159690=CARTESIAN_POINT('',(10.1,2.,-17.645)) ;
#159691=CARTESIAN_POINT('',(3.6,1.9,-17.645)) ;
#159692=CARTESIAN_POINT('Origin',(3.6,-5.25,-17.645)) ;
#159693=CARTESIAN_POINT('',(3.5,-5.25,-17.745)) ;
#159694=CARTESIAN_POINT('',(2.7,-5.25,-17.745)) ;
#159695=CARTESIAN_POINT('',(3.6,-5.25,-17.745)) ;
#159696=CARTESIAN_POINT('',(2.7,-5.25,-20.355)) ;
#159697=CARTESIAN_POINT('',(2.7,-5.25,-17.645)) ;
#159698=CARTESIAN_POINT('',(3.5,-5.25,-20.355)) ;
#159699=CARTESIAN_POINT('',(3.6,-5.25,-20.355)) ;
#159700=CARTESIAN_POINT('',(3.5,-5.25,-17.645)) ;
#159701=CARTESIAN_POINT('Origin',(3.6,-5.25,-20.455)) ;
#159702=CARTESIAN_POINT('',(2.7,1.9,-20.455)) ;
#159703=CARTESIAN_POINT('',(3.5,1.9,-20.455)) ;
#159704=CARTESIAN_POINT('',(3.6,1.9,-20.455)) ;
#159705=CARTESIAN_POINT('',(3.6,1.92679491924311,-20.455)) ;
#159706=CARTESIAN_POINT('Origin',(3.5,2.1,-20.455)) ;
#159707=CARTESIAN_POINT('',(3.7,1.9,-20.455)) ;
#159708=CARTESIAN_POINT('Origin',(3.7,2.1,-20.455)) ;
#159709=CARTESIAN_POINT('',(10.1,1.9,-20.455)) ;
#159710=CARTESIAN_POINT('',(3.6,1.9,-20.455)) ;
#159711=CARTESIAN_POINT('',(10.1,-2.15,-20.455)) ;
#159712=CARTESIAN_POINT('',(10.1,-2.25,-20.455)) ;
#159713=CARTESIAN_POINT('',(3.7,-2.15,-20.455)) ;
#159714=CARTESIAN_POINT('',(3.6,-2.15,-20.455)) ;
#159715=CARTESIAN_POINT('',(3.5,-2.35,-20.455)) ;
#159716=CARTESIAN_POINT('Origin',(3.7,-2.35,-20.455)) ;
#159717=CARTESIAN_POINT('',(3.5,-5.15,-20.455)) ;
#159718=CARTESIAN_POINT('',(3.5,-5.25,-20.455)) ;
#159719=CARTESIAN_POINT('',(2.7,-5.15,-20.455)) ;
#159720=CARTESIAN_POINT('',(3.6,-5.15,-20.455)) ;
#159721=CARTESIAN_POINT('',(2.7,-5.25,-20.455)) ;
#159722=CARTESIAN_POINT('Origin',(3.6,2.,-20.455)) ;
#159723=CARTESIAN_POINT('',(2.7,2.,-21.355)) ;
#159724=CARTESIAN_POINT('',(3.5,2.,-21.355)) ;
#159725=CARTESIAN_POINT('',(3.6,2.,-21.355)) ;
#159726=CARTESIAN_POINT('',(3.5,2.,-20.555)) ;
#159727=CARTESIAN_POINT('',(3.5,2.,-20.555)) ;
#159728=CARTESIAN_POINT('',(2.7,2.,-20.555)) ;
#159729=CARTESIAN_POINT('',(2.6,2.,-20.555)) ;
#159730=CARTESIAN_POINT('',(2.7,2.,-20.455)) ;
#159731=CARTESIAN_POINT('Origin',(3.6,2.,-21.455)) ;
#159732=CARTESIAN_POINT('',(3.7,1.9,-21.455)) ;
#159733=CARTESIAN_POINT('',(3.6,1.92679491924311,-21.455)) ;
#159734=CARTESIAN_POINT('Origin',(3.7,2.1,-21.455)) ;
#159735=CARTESIAN_POINT('',(3.5,1.9,-21.455)) ;
#159736=CARTESIAN_POINT('Origin',(3.5,2.1,-21.455)) ;
#159737=CARTESIAN_POINT('',(2.7,1.9,-21.455)) ;
#159738=CARTESIAN_POINT('',(2.7,1.9,-21.455)) ;
#159739=CARTESIAN_POINT('',(2.7,-5.15,-21.455)) ;
#159740=CARTESIAN_POINT('',(2.7,2.,-21.455)) ;
#159741=CARTESIAN_POINT('',(3.5,-5.15,-21.455)) ;
#159742=CARTESIAN_POINT('',(3.6,-5.15,-21.455)) ;
#159743=CARTESIAN_POINT('',(3.5,-2.35,-21.455)) ;
#159744=CARTESIAN_POINT('',(3.5,-2.25,-21.455)) ;
#159745=CARTESIAN_POINT('',(3.7,-2.15,-21.455)) ;
#159746=CARTESIAN_POINT('Origin',(3.7,-2.35,-21.455)) ;
#159747=CARTESIAN_POINT('',(10.1,-2.15,-21.455)) ;
#159748=CARTESIAN_POINT('',(3.6,-2.15,-21.455)) ;
#159749=CARTESIAN_POINT('',(10.1,1.9,-21.455)) ;
#159750=CARTESIAN_POINT('',(10.1,2.,-21.455)) ;
#159751=CARTESIAN_POINT('',(3.6,1.9,-21.455)) ;
#159752=CARTESIAN_POINT('Origin',(3.6,-5.25,-21.455)) ;
#159753=CARTESIAN_POINT('',(3.5,-5.25,-21.555)) ;
#159754=CARTESIAN_POINT('',(2.7,-5.25,-21.555)) ;
#159755=CARTESIAN_POINT('',(3.6,-5.25,-21.555)) ;
#159756=CARTESIAN_POINT('',(2.7,-5.25,-24.165)) ;
#159757=CARTESIAN_POINT('',(2.7,-5.25,-21.455)) ;
#159758=CARTESIAN_POINT('',(3.5,-5.25,-24.165)) ;
#159759=CARTESIAN_POINT('',(3.6,-5.25,-24.165)) ;
#159760=CARTESIAN_POINT('',(3.5,-5.25,-21.455)) ;
#159761=CARTESIAN_POINT('Origin',(3.6,-5.25,-24.265)) ;
#159762=CARTESIAN_POINT('',(2.7,1.9,-24.265)) ;
#159763=CARTESIAN_POINT('',(3.5,1.9,-24.265)) ;
#159764=CARTESIAN_POINT('',(3.6,1.9,-24.265)) ;
#159765=CARTESIAN_POINT('',(3.6,1.92679491924311,-24.265)) ;
#159766=CARTESIAN_POINT('Origin',(3.5,2.1,-24.265)) ;
#159767=CARTESIAN_POINT('',(3.7,1.9,-24.265)) ;
#159768=CARTESIAN_POINT('Origin',(3.7,2.1,-24.265)) ;
#159769=CARTESIAN_POINT('',(10.1,1.9,-24.265)) ;
#159770=CARTESIAN_POINT('',(3.6,1.9,-24.265)) ;
#159771=CARTESIAN_POINT('',(10.1,-2.15,-24.265)) ;
#159772=CARTESIAN_POINT('',(10.1,-2.25,-24.265)) ;
#159773=CARTESIAN_POINT('',(3.7,-2.15,-24.265)) ;
#159774=CARTESIAN_POINT('',(3.6,-2.15,-24.265)) ;
#159775=CARTESIAN_POINT('',(3.5,-2.35,-24.265)) ;
#159776=CARTESIAN_POINT('Origin',(3.7,-2.35,-24.265)) ;
#159777=CARTESIAN_POINT('',(3.5,-5.15,-24.265)) ;
#159778=CARTESIAN_POINT('',(3.5,-5.25,-24.265)) ;
#159779=CARTESIAN_POINT('',(2.7,-5.15,-24.265)) ;
#159780=CARTESIAN_POINT('',(3.6,-5.15,-24.265)) ;
#159781=CARTESIAN_POINT('',(2.7,-5.25,-24.265)) ;
#159782=CARTESIAN_POINT('Origin',(3.6,2.,-24.265)) ;
#159783=CARTESIAN_POINT('',(2.7,2.,-25.165)) ;
#159784=CARTESIAN_POINT('',(3.5,2.,-25.165)) ;
#159785=CARTESIAN_POINT('',(3.6,2.,-25.165)) ;
#159786=CARTESIAN_POINT('',(3.5,2.,-24.365)) ;
#159787=CARTESIAN_POINT('',(3.5,2.,-24.365)) ;
#159788=CARTESIAN_POINT('',(2.7,2.,-24.365)) ;
#159789=CARTESIAN_POINT('',(2.6,2.,-24.365)) ;
#159790=CARTESIAN_POINT('',(2.7,2.,-24.265)) ;
#159791=CARTESIAN_POINT('Origin',(3.6,2.,-25.265)) ;
#159792=CARTESIAN_POINT('',(3.7,1.9,-25.265)) ;
#159793=CARTESIAN_POINT('',(3.6,1.92679491924311,-25.265)) ;
#159794=CARTESIAN_POINT('Origin',(3.7,2.1,-25.265)) ;
#159795=CARTESIAN_POINT('',(3.5,1.9,-25.265)) ;
#159796=CARTESIAN_POINT('Origin',(3.5,2.1,-25.265)) ;
#159797=CARTESIAN_POINT('',(2.7,1.9,-25.265)) ;
#159798=CARTESIAN_POINT('',(2.7,1.9,-25.265)) ;
#159799=CARTESIAN_POINT('',(2.7,-5.15,-25.265)) ;
#159800=CARTESIAN_POINT('',(2.7,2.,-25.265)) ;
#159801=CARTESIAN_POINT('',(3.5,-5.15,-25.265)) ;
#159802=CARTESIAN_POINT('',(3.6,-5.15,-25.265)) ;
#159803=CARTESIAN_POINT('',(3.5,-2.35,-25.265)) ;
#159804=CARTESIAN_POINT('',(3.5,-2.25,-25.265)) ;
#159805=CARTESIAN_POINT('',(3.7,-2.15,-25.265)) ;
#159806=CARTESIAN_POINT('Origin',(3.7,-2.35,-25.265)) ;
#159807=CARTESIAN_POINT('',(10.1,-2.15,-25.265)) ;
#159808=CARTESIAN_POINT('',(3.6,-2.15,-25.265)) ;
#159809=CARTESIAN_POINT('',(10.1,1.9,-25.265)) ;
#159810=CARTESIAN_POINT('',(10.1,2.,-25.265)) ;
#159811=CARTESIAN_POINT('',(3.6,1.9,-25.265)) ;
#159812=CARTESIAN_POINT('Origin',(3.6,-5.25,-25.265)) ;
#159813=CARTESIAN_POINT('',(3.5,-5.25,-25.365)) ;
#159814=CARTESIAN_POINT('',(2.7,-5.25,-25.365)) ;
#159815=CARTESIAN_POINT('',(3.6,-5.25,-25.365)) ;
#159816=CARTESIAN_POINT('',(2.7,-5.25,-27.975)) ;
#159817=CARTESIAN_POINT('',(2.7,-5.25,-25.265)) ;
#159818=CARTESIAN_POINT('',(3.5,-5.25,-27.975)) ;
#159819=CARTESIAN_POINT('',(3.6,-5.25,-27.975)) ;
#159820=CARTESIAN_POINT('',(3.5,-5.25,-25.265)) ;
#159821=CARTESIAN_POINT('Origin',(3.6,-5.25,-28.075)) ;
#159822=CARTESIAN_POINT('',(2.7,1.9,-28.075)) ;
#159823=CARTESIAN_POINT('',(3.5,1.9,-28.075)) ;
#159824=CARTESIAN_POINT('',(3.6,1.9,-28.075)) ;
#159825=CARTESIAN_POINT('',(3.6,1.92679491924311,-28.075)) ;
#159826=CARTESIAN_POINT('Origin',(3.5,2.1,-28.075)) ;
#159827=CARTESIAN_POINT('',(3.7,1.9,-28.075)) ;
#159828=CARTESIAN_POINT('Origin',(3.7,2.1,-28.075)) ;
#159829=CARTESIAN_POINT('',(10.1,1.9,-28.075)) ;
#159830=CARTESIAN_POINT('',(3.6,1.9,-28.075)) ;
#159831=CARTESIAN_POINT('',(10.1,-2.15,-28.075)) ;
#159832=CARTESIAN_POINT('',(10.1,-2.25,-28.075)) ;
#159833=CARTESIAN_POINT('',(3.7,-2.15,-28.075)) ;
#159834=CARTESIAN_POINT('',(3.6,-2.15,-28.075)) ;
#159835=CARTESIAN_POINT('',(3.5,-2.35,-28.075)) ;
#159836=CARTESIAN_POINT('Origin',(3.7,-2.35,-28.075)) ;
#159837=CARTESIAN_POINT('',(3.5,-5.15,-28.075)) ;
#159838=CARTESIAN_POINT('',(3.5,-5.25,-28.075)) ;
#159839=CARTESIAN_POINT('',(2.7,-5.15,-28.075)) ;
#159840=CARTESIAN_POINT('',(3.6,-5.15,-28.075)) ;
#159841=CARTESIAN_POINT('',(2.7,-5.25,-28.075)) ;
#159842=CARTESIAN_POINT('Origin',(3.6,2.,-28.075)) ;
#159843=CARTESIAN_POINT('',(2.7,2.,-28.975)) ;
#159844=CARTESIAN_POINT('',(3.5,2.,-28.975)) ;
#159845=CARTESIAN_POINT('',(3.6,2.,-28.975)) ;
#159846=CARTESIAN_POINT('',(3.5,2.,-28.175)) ;
#159847=CARTESIAN_POINT('',(3.5,2.,-28.175)) ;
#159848=CARTESIAN_POINT('',(2.7,2.,-28.175)) ;
#159849=CARTESIAN_POINT('',(2.6,2.,-28.175)) ;
#159850=CARTESIAN_POINT('',(2.7,2.,-28.075)) ;
#159851=CARTESIAN_POINT('Origin',(3.6,2.,-29.075)) ;
#159852=CARTESIAN_POINT('',(3.7,1.9,-29.075)) ;
#159853=CARTESIAN_POINT('',(3.6,1.92679491924311,-29.075)) ;
#159854=CARTESIAN_POINT('Origin',(3.7,2.1,-29.075)) ;
#159855=CARTESIAN_POINT('',(3.5,1.9,-29.075)) ;
#159856=CARTESIAN_POINT('Origin',(3.5,2.1,-29.075)) ;
#159857=CARTESIAN_POINT('',(2.7,1.9,-29.075)) ;
#159858=CARTESIAN_POINT('',(2.7,1.9,-29.075)) ;
#159859=CARTESIAN_POINT('',(2.7,-5.15,-29.075)) ;
#159860=CARTESIAN_POINT('',(2.7,2.,-29.075)) ;
#159861=CARTESIAN_POINT('',(3.5,-5.15,-29.075)) ;
#159862=CARTESIAN_POINT('',(3.6,-5.15,-29.075)) ;
#159863=CARTESIAN_POINT('',(3.5,-2.35,-29.075)) ;
#159864=CARTESIAN_POINT('',(3.5,-2.25,-29.075)) ;
#159865=CARTESIAN_POINT('',(3.7,-2.15,-29.075)) ;
#159866=CARTESIAN_POINT('Origin',(3.7,-2.35,-29.075)) ;
#159867=CARTESIAN_POINT('',(10.1,-2.15,-29.075)) ;
#159868=CARTESIAN_POINT('',(3.6,-2.15,-29.075)) ;
#159869=CARTESIAN_POINT('',(10.1,1.9,-29.075)) ;
#159870=CARTESIAN_POINT('',(10.1,2.,-29.075)) ;
#159871=CARTESIAN_POINT('',(3.6,1.9,-29.075)) ;
#159872=CARTESIAN_POINT('Origin',(3.6,-5.25,-29.075)) ;
#159873=CARTESIAN_POINT('',(3.5,-5.25,-29.175)) ;
#159874=CARTESIAN_POINT('',(2.7,-5.25,-29.175)) ;
#159875=CARTESIAN_POINT('',(3.6,-5.25,-29.175)) ;
#159876=CARTESIAN_POINT('',(2.7,-5.25,-31.785)) ;
#159877=CARTESIAN_POINT('',(2.7,-5.25,-29.075)) ;
#159878=CARTESIAN_POINT('',(3.5,-5.25,-31.785)) ;
#159879=CARTESIAN_POINT('',(3.6,-5.25,-31.785)) ;
#159880=CARTESIAN_POINT('',(3.5,-5.25,-29.075)) ;
#159881=CARTESIAN_POINT('Origin',(3.6,-5.25,-31.885)) ;
#159882=CARTESIAN_POINT('',(2.7,1.9,-31.885)) ;
#159883=CARTESIAN_POINT('',(3.5,1.9,-31.885)) ;
#159884=CARTESIAN_POINT('',(3.6,1.9,-31.885)) ;
#159885=CARTESIAN_POINT('',(3.6,1.92679491924311,-31.885)) ;
#159886=CARTESIAN_POINT('Origin',(3.5,2.1,-31.885)) ;
#159887=CARTESIAN_POINT('',(3.7,1.9,-31.885)) ;
#159888=CARTESIAN_POINT('Origin',(3.7,2.1,-31.885)) ;
#159889=CARTESIAN_POINT('',(10.1,1.9,-31.885)) ;
#159890=CARTESIAN_POINT('',(3.6,1.9,-31.885)) ;
#159891=CARTESIAN_POINT('',(10.1,-2.15,-31.885)) ;
#159892=CARTESIAN_POINT('',(10.1,-2.25,-31.885)) ;
#159893=CARTESIAN_POINT('',(3.7,-2.15,-31.885)) ;
#159894=CARTESIAN_POINT('',(3.6,-2.15,-31.885)) ;
#159895=CARTESIAN_POINT('',(3.5,-2.35,-31.885)) ;
#159896=CARTESIAN_POINT('Origin',(3.7,-2.35,-31.885)) ;
#159897=CARTESIAN_POINT('',(3.5,-5.15,-31.885)) ;
#159898=CARTESIAN_POINT('',(3.5,-5.25,-31.885)) ;
#159899=CARTESIAN_POINT('',(2.7,-5.15,-31.885)) ;
#159900=CARTESIAN_POINT('',(3.6,-5.15,-31.885)) ;
#159901=CARTESIAN_POINT('',(2.7,-5.25,-31.885)) ;
#159902=CARTESIAN_POINT('Origin',(3.6,2.,-31.885)) ;
#159903=CARTESIAN_POINT('',(2.7,2.,-32.785)) ;
#159904=CARTESIAN_POINT('',(3.5,2.,-32.785)) ;
#159905=CARTESIAN_POINT('',(3.6,2.,-32.785)) ;
#159906=CARTESIAN_POINT('',(3.5,2.,-31.985)) ;
#159907=CARTESIAN_POINT('',(3.5,2.,-31.985)) ;
#159908=CARTESIAN_POINT('',(2.7,2.,-31.985)) ;
#159909=CARTESIAN_POINT('',(2.6,2.,-31.985)) ;
#159910=CARTESIAN_POINT('',(2.7,2.,-31.885)) ;
#159911=CARTESIAN_POINT('Origin',(3.6,2.,-32.885)) ;
#159912=CARTESIAN_POINT('',(3.7,1.9,-32.885)) ;
#159913=CARTESIAN_POINT('',(3.6,1.92679491924311,-32.885)) ;
#159914=CARTESIAN_POINT('Origin',(3.7,2.1,-32.885)) ;
#159915=CARTESIAN_POINT('',(3.5,1.9,-32.885)) ;
#159916=CARTESIAN_POINT('Origin',(3.5,2.1,-32.885)) ;
#159917=CARTESIAN_POINT('',(2.7,1.9,-32.885)) ;
#159918=CARTESIAN_POINT('',(2.7,1.9,-32.885)) ;
#159919=CARTESIAN_POINT('',(2.7,-5.15,-32.885)) ;
#159920=CARTESIAN_POINT('',(2.7,2.,-32.885)) ;
#159921=CARTESIAN_POINT('',(3.5,-5.15,-32.885)) ;
#159922=CARTESIAN_POINT('',(3.6,-5.15,-32.885)) ;
#159923=CARTESIAN_POINT('',(3.5,-2.35,-32.885)) ;
#159924=CARTESIAN_POINT('',(3.5,-2.25,-32.885)) ;
#159925=CARTESIAN_POINT('',(3.7,-2.15,-32.885)) ;
#159926=CARTESIAN_POINT('Origin',(3.7,-2.35,-32.885)) ;
#159927=CARTESIAN_POINT('',(10.1,-2.15,-32.885)) ;
#159928=CARTESIAN_POINT('',(3.6,-2.15,-32.885)) ;
#159929=CARTESIAN_POINT('',(10.1,1.9,-32.885)) ;
#159930=CARTESIAN_POINT('',(10.1,2.,-32.885)) ;
#159931=CARTESIAN_POINT('',(3.6,1.9,-32.885)) ;
#159932=CARTESIAN_POINT('Origin',(3.6,-5.25,-32.885)) ;
#159933=CARTESIAN_POINT('',(3.5,-5.25,-32.985)) ;
#159934=CARTESIAN_POINT('',(2.7,-5.25,-32.985)) ;
#159935=CARTESIAN_POINT('',(3.6,-5.25,-32.985)) ;
#159936=CARTESIAN_POINT('',(2.7,-5.25,-35.595)) ;
#159937=CARTESIAN_POINT('',(2.7,-5.25,-32.885)) ;
#159938=CARTESIAN_POINT('',(3.5,-5.25,-35.595)) ;
#159939=CARTESIAN_POINT('',(3.6,-5.25,-35.595)) ;
#159940=CARTESIAN_POINT('',(3.5,-5.25,-32.885)) ;
#159941=CARTESIAN_POINT('Origin',(3.6,-5.25,-35.695)) ;
#159942=CARTESIAN_POINT('',(2.7,1.9,-35.695)) ;
#159943=CARTESIAN_POINT('',(3.5,1.9,-35.695)) ;
#159944=CARTESIAN_POINT('',(3.6,1.9,-35.695)) ;
#159945=CARTESIAN_POINT('',(3.6,1.92679491924311,-35.695)) ;
#159946=CARTESIAN_POINT('Origin',(3.5,2.1,-35.695)) ;
#159947=CARTESIAN_POINT('',(3.7,1.9,-35.695)) ;
#159948=CARTESIAN_POINT('Origin',(3.7,2.1,-35.695)) ;
#159949=CARTESIAN_POINT('',(10.1,1.9,-35.695)) ;
#159950=CARTESIAN_POINT('',(3.6,1.9,-35.695)) ;
#159951=CARTESIAN_POINT('',(10.1,-2.15,-35.695)) ;
#159952=CARTESIAN_POINT('',(10.1,-2.25,-35.695)) ;
#159953=CARTESIAN_POINT('',(3.7,-2.15,-35.695)) ;
#159954=CARTESIAN_POINT('',(3.6,-2.15,-35.695)) ;
#159955=CARTESIAN_POINT('',(3.5,-2.35,-35.695)) ;
#159956=CARTESIAN_POINT('Origin',(3.7,-2.35,-35.695)) ;
#159957=CARTESIAN_POINT('',(3.5,-5.15,-35.695)) ;
#159958=CARTESIAN_POINT('',(3.5,-5.25,-35.695)) ;
#159959=CARTESIAN_POINT('',(2.7,-5.15,-35.695)) ;
#159960=CARTESIAN_POINT('',(3.6,-5.15,-35.695)) ;
#159961=CARTESIAN_POINT('',(2.7,-5.25,-35.695)) ;
#159962=CARTESIAN_POINT('Origin',(3.6,2.,-35.695)) ;
#159963=CARTESIAN_POINT('',(2.7,2.,-35.795)) ;
#159964=CARTESIAN_POINT('',(2.7,2.,-36.49)) ;
#159965=CARTESIAN_POINT('',(2.7,2.,-35.695)) ;
#159966=CARTESIAN_POINT('',(3.5,2.,-36.49)) ;
#159967=CARTESIAN_POINT('',(3.5,2.,-36.49)) ;
#159968=CARTESIAN_POINT('',(3.5,2.,-35.795)) ;
#159969=CARTESIAN_POINT('',(3.5,2.,-35.795)) ;
#159970=CARTESIAN_POINT('',(2.6,2.,-35.795)) ;
#159971=CARTESIAN_POINT('Origin',(10.2,-2.25,-4.685)) ;
#159972=CARTESIAN_POINT('',(10.1,-2.25,-4.71311959340942)) ;
#159973=CARTESIAN_POINT('',(3.7,-2.25,-4.71311959340942)) ;
#159974=CARTESIAN_POINT('',(10.2,-2.25,-4.71311959340942)) ;
#159975=CARTESIAN_POINT('',(3.7,-2.25,-5.115)) ;
#159976=CARTESIAN_POINT('',(3.7,-2.25,-4.685)) ;
#159977=CARTESIAN_POINT('',(10.1,-2.25,-5.115)) ;
#159978=CARTESIAN_POINT('',(10.2,-2.25,-5.115)) ;
#159979=CARTESIAN_POINT('',(10.1,-2.25,-4.685)) ;
#159980=CARTESIAN_POINT('Origin',(10.2,-2.25,-2.405)) ;
#159981=CARTESIAN_POINT('',(10.1,-2.25,-2.505)) ;
#159982=CARTESIAN_POINT('',(3.7,-2.25,-2.505)) ;
#159983=CARTESIAN_POINT('',(10.2,-2.25,-2.505)) ;
#159984=CARTESIAN_POINT('',(3.7,-2.25,-2.90688040659058)) ;
#159985=CARTESIAN_POINT('',(3.7,-2.25,-2.405)) ;
#159986=CARTESIAN_POINT('',(10.1,-2.25,-2.90688040659058)) ;
#159987=CARTESIAN_POINT('',(10.2,-2.25,-2.90688040659058)) ;
#159988=CARTESIAN_POINT('',(10.1,-2.25,-2.405)) ;
#159989=CARTESIAN_POINT('Origin',(10.2,-3.65625,-3.81)) ;
#159990=CARTESIAN_POINT('',(10.1,-2.23576512455516,-2.95830358628649)) ;
#159991=CARTESIAN_POINT('',(3.7,-2.23576512455516,-2.95830358628649)) ;
#159992=CARTESIAN_POINT('',(10.2,-2.23576512455516,-2.95830358628649)) ;
#159993=CARTESIAN_POINT('',(3.7,-2.23576512455516,-4.66169641371351)) ;
#159994=CARTESIAN_POINT('Origin',(3.7,-3.65625,-3.81)) ;
#159995=CARTESIAN_POINT('',(10.1,-2.23576512455516,-4.66169641371351)) ;
#159996=CARTESIAN_POINT('',(10.2,-2.23576512455516,-4.66169641371351)) ;
#159997=CARTESIAN_POINT('Origin',(10.1,-3.65625,-3.81)) ;
#159998=CARTESIAN_POINT('Origin',(10.2,-3.65625,-3.81)) ;
#159999=CARTESIAN_POINT('',(10.2,-2.15,-2.505)) ;
#160000=CARTESIAN_POINT('',(10.2,-2.15,-2.90688040659058)) ;
#160001=CARTESIAN_POINT('',(10.2,-2.15,-2.935)) ;
#160002=CARTESIAN_POINT('',(10.2,-2.15,-4.71311959340942)) ;
#160003=CARTESIAN_POINT('Origin',(10.2,-3.65625,-3.81)) ;
#160004=CARTESIAN_POINT('',(10.2,-2.15,-5.115)) ;
#160005=CARTESIAN_POINT('',(10.2,-2.15,-5.215)) ;
#160006=CARTESIAN_POINT('',(10.2,1.9,-5.115)) ;
#160007=CARTESIAN_POINT('',(10.2,2.,-5.115)) ;
#160008=CARTESIAN_POINT('',(10.2,1.9,-2.505)) ;
#160009=CARTESIAN_POINT('',(10.2,1.9,-2.405)) ;
#160010=CARTESIAN_POINT('',(10.2,-2.25,-2.505)) ;
#160011=CARTESIAN_POINT('Origin',(10.2,-2.25,-8.495)) ;
#160012=CARTESIAN_POINT('',(10.1,-2.25,-8.52311959340942)) ;
#160013=CARTESIAN_POINT('',(3.7,-2.25,-8.52311959340942)) ;
#160014=CARTESIAN_POINT('',(10.2,-2.25,-8.52311959340942)) ;
#160015=CARTESIAN_POINT('',(3.7,-2.25,-8.925)) ;
#160016=CARTESIAN_POINT('',(3.7,-2.25,-8.495)) ;
#160017=CARTESIAN_POINT('',(10.1,-2.25,-8.925)) ;
#160018=CARTESIAN_POINT('',(10.2,-2.25,-8.925)) ;
#160019=CARTESIAN_POINT('',(10.1,-2.25,-8.495)) ;
#160020=CARTESIAN_POINT('Origin',(10.2,-2.25,-6.215)) ;
#160021=CARTESIAN_POINT('',(10.1,-2.25,-6.315)) ;
#160022=CARTESIAN_POINT('',(3.7,-2.25,-6.315)) ;
#160023=CARTESIAN_POINT('',(10.2,-2.25,-6.315)) ;
#160024=CARTESIAN_POINT('',(3.7,-2.25,-6.71688040659058)) ;
#160025=CARTESIAN_POINT('',(3.7,-2.25,-6.215)) ;
#160026=CARTESIAN_POINT('',(10.1,-2.25,-6.71688040659058)) ;
#160027=CARTESIAN_POINT('',(10.2,-2.25,-6.71688040659058)) ;
#160028=CARTESIAN_POINT('',(10.1,-2.25,-6.215)) ;
#160029=CARTESIAN_POINT('Origin',(10.2,-3.65625,-7.62)) ;
#160030=CARTESIAN_POINT('',(10.1,-2.23576512455516,-6.76830358628649)) ;
#160031=CARTESIAN_POINT('',(3.7,-2.23576512455516,-6.76830358628649)) ;
#160032=CARTESIAN_POINT('',(10.2,-2.23576512455516,-6.76830358628649)) ;
#160033=CARTESIAN_POINT('',(3.7,-2.23576512455516,-8.47169641371351)) ;
#160034=CARTESIAN_POINT('Origin',(3.7,-3.65625,-7.62)) ;
#160035=CARTESIAN_POINT('',(10.1,-2.23576512455516,-8.47169641371351)) ;
#160036=CARTESIAN_POINT('',(10.2,-2.23576512455516,-8.47169641371351)) ;
#160037=CARTESIAN_POINT('Origin',(10.1,-3.65625,-7.62)) ;
#160038=CARTESIAN_POINT('Origin',(10.2,-3.65625,-7.62)) ;
#160039=CARTESIAN_POINT('',(10.2,-2.15,-6.315)) ;
#160040=CARTESIAN_POINT('',(10.2,-2.15,-6.71688040659058)) ;
#160041=CARTESIAN_POINT('',(10.2,-2.15,-6.745)) ;
#160042=CARTESIAN_POINT('',(10.2,-2.15,-8.52311959340943)) ;
#160043=CARTESIAN_POINT('Origin',(10.2,-3.65625,-7.62)) ;
#160044=CARTESIAN_POINT('',(10.2,-2.15,-8.925)) ;
#160045=CARTESIAN_POINT('',(10.2,-2.15,-9.025)) ;
#160046=CARTESIAN_POINT('',(10.2,1.9,-8.925)) ;
#160047=CARTESIAN_POINT('',(10.2,2.,-8.925)) ;
#160048=CARTESIAN_POINT('',(10.2,1.9,-6.315)) ;
#160049=CARTESIAN_POINT('',(10.2,1.9,-6.215)) ;
#160050=CARTESIAN_POINT('',(10.2,-2.25,-6.315)) ;
#160051=CARTESIAN_POINT('Origin',(10.2,-2.25,-12.305)) ;
#160052=CARTESIAN_POINT('',(10.1,-2.25,-12.3331195934094)) ;
#160053=CARTESIAN_POINT('',(3.7,-2.25,-12.3331195934094)) ;
#160054=CARTESIAN_POINT('',(10.2,-2.25,-12.3331195934094)) ;
#160055=CARTESIAN_POINT('',(3.7,-2.25,-12.735)) ;
#160056=CARTESIAN_POINT('',(3.7,-2.25,-12.305)) ;
#160057=CARTESIAN_POINT('',(10.1,-2.25,-12.735)) ;
#160058=CARTESIAN_POINT('',(10.2,-2.25,-12.735)) ;
#160059=CARTESIAN_POINT('',(10.1,-2.25,-12.305)) ;
#160060=CARTESIAN_POINT('Origin',(10.2,-2.25,-10.025)) ;
#160061=CARTESIAN_POINT('',(10.1,-2.25,-10.125)) ;
#160062=CARTESIAN_POINT('',(3.7,-2.25,-10.125)) ;
#160063=CARTESIAN_POINT('',(10.2,-2.25,-10.125)) ;
#160064=CARTESIAN_POINT('',(3.7,-2.25,-10.5268804065906)) ;
#160065=CARTESIAN_POINT('',(3.7,-2.25,-10.025)) ;
#160066=CARTESIAN_POINT('',(10.1,-2.25,-10.5268804065906)) ;
#160067=CARTESIAN_POINT('',(10.2,-2.25,-10.5268804065906)) ;
#160068=CARTESIAN_POINT('',(10.1,-2.25,-10.025)) ;
#160069=CARTESIAN_POINT('Origin',(10.2,-3.65625,-11.43)) ;
#160070=CARTESIAN_POINT('',(10.1,-2.23576512455516,-10.5783035862865)) ;
#160071=CARTESIAN_POINT('',(3.7,-2.23576512455516,-10.5783035862865)) ;
#160072=CARTESIAN_POINT('',(10.2,-2.23576512455516,-10.5783035862865)) ;
#160073=CARTESIAN_POINT('',(3.7,-2.23576512455516,-12.2816964137135)) ;
#160074=CARTESIAN_POINT('Origin',(3.7,-3.65625,-11.43)) ;
#160075=CARTESIAN_POINT('',(10.1,-2.23576512455516,-12.2816964137135)) ;
#160076=CARTESIAN_POINT('',(10.2,-2.23576512455516,-12.2816964137135)) ;
#160077=CARTESIAN_POINT('Origin',(10.1,-3.65625,-11.43)) ;
#160078=CARTESIAN_POINT('Origin',(10.2,-3.65625,-11.43)) ;
#160079=CARTESIAN_POINT('',(10.2,-2.15,-10.125)) ;
#160080=CARTESIAN_POINT('',(10.2,-2.15,-10.5268804065906)) ;
#160081=CARTESIAN_POINT('',(10.2,-2.15,-10.555)) ;
#160082=CARTESIAN_POINT('',(10.2,-2.15,-12.3331195934094)) ;
#160083=CARTESIAN_POINT('Origin',(10.2,-3.65625,-11.43)) ;
#160084=CARTESIAN_POINT('',(10.2,-2.15,-12.735)) ;
#160085=CARTESIAN_POINT('',(10.2,-2.15,-12.835)) ;
#160086=CARTESIAN_POINT('',(10.2,1.9,-12.735)) ;
#160087=CARTESIAN_POINT('',(10.2,2.,-12.735)) ;
#160088=CARTESIAN_POINT('',(10.2,1.9,-10.125)) ;
#160089=CARTESIAN_POINT('',(10.2,1.9,-10.025)) ;
#160090=CARTESIAN_POINT('',(10.2,-2.25,-10.125)) ;
#160091=CARTESIAN_POINT('Origin',(10.2,-2.25,-16.115)) ;
#160092=CARTESIAN_POINT('',(10.1,-2.25,-16.1431195934094)) ;
#160093=CARTESIAN_POINT('',(3.7,-2.25,-16.1431195934094)) ;
#160094=CARTESIAN_POINT('',(10.2,-2.25,-16.1431195934094)) ;
#160095=CARTESIAN_POINT('',(3.7,-2.25,-16.545)) ;
#160096=CARTESIAN_POINT('',(3.7,-2.25,-16.115)) ;
#160097=CARTESIAN_POINT('',(10.1,-2.25,-16.545)) ;
#160098=CARTESIAN_POINT('',(10.2,-2.25,-16.545)) ;
#160099=CARTESIAN_POINT('',(10.1,-2.25,-16.115)) ;
#160100=CARTESIAN_POINT('Origin',(10.2,-2.25,-13.835)) ;
#160101=CARTESIAN_POINT('',(10.1,-2.25,-13.935)) ;
#160102=CARTESIAN_POINT('',(3.7,-2.25,-13.935)) ;
#160103=CARTESIAN_POINT('',(10.2,-2.25,-13.935)) ;
#160104=CARTESIAN_POINT('',(3.7,-2.25,-14.3368804065906)) ;
#160105=CARTESIAN_POINT('',(3.7,-2.25,-13.835)) ;
#160106=CARTESIAN_POINT('',(10.1,-2.25,-14.3368804065906)) ;
#160107=CARTESIAN_POINT('',(10.2,-2.25,-14.3368804065906)) ;
#160108=CARTESIAN_POINT('',(10.1,-2.25,-13.835)) ;
#160109=CARTESIAN_POINT('Origin',(10.2,-3.65625,-15.24)) ;
#160110=CARTESIAN_POINT('',(10.1,-2.23576512455516,-14.3883035862865)) ;
#160111=CARTESIAN_POINT('',(3.7,-2.23576512455516,-14.3883035862865)) ;
#160112=CARTESIAN_POINT('',(10.2,-2.23576512455516,-14.3883035862865)) ;
#160113=CARTESIAN_POINT('',(3.7,-2.23576512455516,-16.0916964137135)) ;
#160114=CARTESIAN_POINT('Origin',(3.7,-3.65625,-15.24)) ;
#160115=CARTESIAN_POINT('',(10.1,-2.23576512455516,-16.0916964137135)) ;
#160116=CARTESIAN_POINT('',(10.2,-2.23576512455516,-16.0916964137135)) ;
#160117=CARTESIAN_POINT('Origin',(10.1,-3.65625,-15.24)) ;
#160118=CARTESIAN_POINT('Origin',(10.2,-3.65625,-15.24)) ;
#160119=CARTESIAN_POINT('',(10.2,-2.15,-13.935)) ;
#160120=CARTESIAN_POINT('',(10.2,-2.15,-14.3368804065906)) ;
#160121=CARTESIAN_POINT('',(10.2,-2.15,-14.365)) ;
#160122=CARTESIAN_POINT('',(10.2,-2.15,-16.1431195934094)) ;
#160123=CARTESIAN_POINT('Origin',(10.2,-3.65625,-15.24)) ;
#160124=CARTESIAN_POINT('',(10.2,-2.15,-16.545)) ;
#160125=CARTESIAN_POINT('',(10.2,-2.15,-16.645)) ;
#160126=CARTESIAN_POINT('',(10.2,1.9,-16.545)) ;
#160127=CARTESIAN_POINT('',(10.2,2.,-16.545)) ;
#160128=CARTESIAN_POINT('',(10.2,1.9,-13.935)) ;
#160129=CARTESIAN_POINT('',(10.2,1.9,-13.835)) ;
#160130=CARTESIAN_POINT('',(10.2,-2.25,-13.935)) ;
#160131=CARTESIAN_POINT('Origin',(10.2,-2.25,-19.925)) ;
#160132=CARTESIAN_POINT('',(10.1,-2.25,-19.9531195934094)) ;
#160133=CARTESIAN_POINT('',(3.7,-2.25,-19.9531195934094)) ;
#160134=CARTESIAN_POINT('',(10.2,-2.25,-19.9531195934094)) ;
#160135=CARTESIAN_POINT('',(3.7,-2.25,-20.355)) ;
#160136=CARTESIAN_POINT('',(3.7,-2.25,-19.925)) ;
#160137=CARTESIAN_POINT('',(10.1,-2.25,-20.355)) ;
#160138=CARTESIAN_POINT('',(10.2,-2.25,-20.355)) ;
#160139=CARTESIAN_POINT('',(10.1,-2.25,-19.925)) ;
#160140=CARTESIAN_POINT('Origin',(10.2,-2.25,-17.645)) ;
#160141=CARTESIAN_POINT('',(10.1,-2.25,-17.745)) ;
#160142=CARTESIAN_POINT('',(3.7,-2.25,-17.745)) ;
#160143=CARTESIAN_POINT('',(10.2,-2.25,-17.745)) ;
#160144=CARTESIAN_POINT('',(3.7,-2.25,-18.1468804065906)) ;
#160145=CARTESIAN_POINT('',(3.7,-2.25,-17.645)) ;
#160146=CARTESIAN_POINT('',(10.1,-2.25,-18.1468804065906)) ;
#160147=CARTESIAN_POINT('',(10.2,-2.25,-18.1468804065906)) ;
#160148=CARTESIAN_POINT('',(10.1,-2.25,-17.645)) ;
#160149=CARTESIAN_POINT('Origin',(10.2,-3.65625,-19.05)) ;
#160150=CARTESIAN_POINT('',(10.1,-2.23576512455516,-18.1983035862865)) ;
#160151=CARTESIAN_POINT('',(3.7,-2.23576512455516,-18.1983035862865)) ;
#160152=CARTESIAN_POINT('',(10.2,-2.23576512455516,-18.1983035862865)) ;
#160153=CARTESIAN_POINT('',(3.7,-2.23576512455516,-19.9016964137135)) ;
#160154=CARTESIAN_POINT('Origin',(3.7,-3.65625,-19.05)) ;
#160155=CARTESIAN_POINT('',(10.1,-2.23576512455516,-19.9016964137135)) ;
#160156=CARTESIAN_POINT('',(10.2,-2.23576512455516,-19.9016964137135)) ;
#160157=CARTESIAN_POINT('Origin',(10.1,-3.65625,-19.05)) ;
#160158=CARTESIAN_POINT('Origin',(10.2,-3.65625,-19.05)) ;
#160159=CARTESIAN_POINT('',(10.2,-2.15,-17.745)) ;
#160160=CARTESIAN_POINT('',(10.2,-2.15,-18.1468804065906)) ;
#160161=CARTESIAN_POINT('',(10.2,-2.15,-18.175)) ;
#160162=CARTESIAN_POINT('',(10.2,-2.15,-19.9531195934094)) ;
#160163=CARTESIAN_POINT('Origin',(10.2,-3.65625,-19.05)) ;
#160164=CARTESIAN_POINT('',(10.2,-2.15,-20.355)) ;
#160165=CARTESIAN_POINT('',(10.2,-2.15,-20.455)) ;
#160166=CARTESIAN_POINT('',(10.2,1.9,-20.355)) ;
#160167=CARTESIAN_POINT('',(10.2,2.,-20.355)) ;
#160168=CARTESIAN_POINT('',(10.2,1.9,-17.745)) ;
#160169=CARTESIAN_POINT('',(10.2,1.9,-17.645)) ;
#160170=CARTESIAN_POINT('',(10.2,-2.25,-17.745)) ;
#160171=CARTESIAN_POINT('Origin',(10.2,-2.25,-23.735)) ;
#160172=CARTESIAN_POINT('',(10.1,-2.25,-23.7631195934094)) ;
#160173=CARTESIAN_POINT('',(3.7,-2.25,-23.7631195934094)) ;
#160174=CARTESIAN_POINT('',(10.2,-2.25,-23.7631195934094)) ;
#160175=CARTESIAN_POINT('',(3.7,-2.25,-24.165)) ;
#160176=CARTESIAN_POINT('',(3.7,-2.25,-23.735)) ;
#160177=CARTESIAN_POINT('',(10.1,-2.25,-24.165)) ;
#160178=CARTESIAN_POINT('',(10.2,-2.25,-24.165)) ;
#160179=CARTESIAN_POINT('',(10.1,-2.25,-23.735)) ;
#160180=CARTESIAN_POINT('Origin',(10.2,-2.25,-21.455)) ;
#160181=CARTESIAN_POINT('',(10.1,-2.25,-21.555)) ;
#160182=CARTESIAN_POINT('',(3.7,-2.25,-21.555)) ;
#160183=CARTESIAN_POINT('',(10.2,-2.25,-21.555)) ;
#160184=CARTESIAN_POINT('',(3.7,-2.25,-21.9568804065906)) ;
#160185=CARTESIAN_POINT('',(3.7,-2.25,-21.455)) ;
#160186=CARTESIAN_POINT('',(10.1,-2.25,-21.9568804065906)) ;
#160187=CARTESIAN_POINT('',(10.2,-2.25,-21.9568804065906)) ;
#160188=CARTESIAN_POINT('',(10.1,-2.25,-21.455)) ;
#160189=CARTESIAN_POINT('Origin',(10.2,-3.65625,-22.86)) ;
#160190=CARTESIAN_POINT('',(10.1,-2.23576512455516,-22.0083035862865)) ;
#160191=CARTESIAN_POINT('',(3.7,-2.23576512455516,-22.0083035862865)) ;
#160192=CARTESIAN_POINT('',(10.2,-2.23576512455516,-22.0083035862865)) ;
#160193=CARTESIAN_POINT('',(3.7,-2.23576512455516,-23.7116964137135)) ;
#160194=CARTESIAN_POINT('Origin',(3.7,-3.65625,-22.86)) ;
#160195=CARTESIAN_POINT('',(10.1,-2.23576512455516,-23.7116964137135)) ;
#160196=CARTESIAN_POINT('',(10.2,-2.23576512455516,-23.7116964137135)) ;
#160197=CARTESIAN_POINT('Origin',(10.1,-3.65625,-22.86)) ;
#160198=CARTESIAN_POINT('Origin',(10.2,-3.65625,-22.86)) ;
#160199=CARTESIAN_POINT('',(10.2,-2.15,-21.555)) ;
#160200=CARTESIAN_POINT('',(10.2,-2.15,-21.9568804065906)) ;
#160201=CARTESIAN_POINT('',(10.2,-2.15,-21.985)) ;
#160202=CARTESIAN_POINT('',(10.2,-2.15,-23.7631195934094)) ;
#160203=CARTESIAN_POINT('Origin',(10.2,-3.65625,-22.86)) ;
#160204=CARTESIAN_POINT('',(10.2,-2.15,-24.165)) ;
#160205=CARTESIAN_POINT('',(10.2,-2.15,-24.265)) ;
#160206=CARTESIAN_POINT('',(10.2,1.9,-24.165)) ;
#160207=CARTESIAN_POINT('',(10.2,2.,-24.165)) ;
#160208=CARTESIAN_POINT('',(10.2,1.9,-21.555)) ;
#160209=CARTESIAN_POINT('',(10.2,1.9,-21.455)) ;
#160210=CARTESIAN_POINT('',(10.2,-2.25,-21.555)) ;
#160211=CARTESIAN_POINT('Origin',(10.2,-2.25,-27.545)) ;
#160212=CARTESIAN_POINT('',(10.1,-2.25,-27.5731195934094)) ;
#160213=CARTESIAN_POINT('',(3.7,-2.25,-27.5731195934094)) ;
#160214=CARTESIAN_POINT('',(10.2,-2.25,-27.5731195934094)) ;
#160215=CARTESIAN_POINT('',(3.7,-2.25,-27.975)) ;
#160216=CARTESIAN_POINT('',(3.7,-2.25,-27.545)) ;
#160217=CARTESIAN_POINT('',(10.1,-2.25,-27.975)) ;
#160218=CARTESIAN_POINT('',(10.2,-2.25,-27.975)) ;
#160219=CARTESIAN_POINT('',(10.1,-2.25,-27.545)) ;
#160220=CARTESIAN_POINT('Origin',(10.2,-2.25,-25.265)) ;
#160221=CARTESIAN_POINT('',(10.1,-2.25,-25.365)) ;
#160222=CARTESIAN_POINT('',(3.7,-2.25,-25.365)) ;
#160223=CARTESIAN_POINT('',(10.2,-2.25,-25.365)) ;
#160224=CARTESIAN_POINT('',(3.7,-2.25,-25.7668804065906)) ;
#160225=CARTESIAN_POINT('',(3.7,-2.25,-25.265)) ;
#160226=CARTESIAN_POINT('',(10.1,-2.25,-25.7668804065906)) ;
#160227=CARTESIAN_POINT('',(10.2,-2.25,-25.7668804065906)) ;
#160228=CARTESIAN_POINT('',(10.1,-2.25,-25.265)) ;
#160229=CARTESIAN_POINT('Origin',(10.2,-3.65625,-26.67)) ;
#160230=CARTESIAN_POINT('',(10.1,-2.23576512455516,-25.8183035862865)) ;
#160231=CARTESIAN_POINT('',(3.7,-2.23576512455516,-25.8183035862865)) ;
#160232=CARTESIAN_POINT('',(10.2,-2.23576512455516,-25.8183035862865)) ;
#160233=CARTESIAN_POINT('',(3.7,-2.23576512455516,-27.5216964137135)) ;
#160234=CARTESIAN_POINT('Origin',(3.7,-3.65625,-26.67)) ;
#160235=CARTESIAN_POINT('',(10.1,-2.23576512455516,-27.5216964137135)) ;
#160236=CARTESIAN_POINT('',(10.2,-2.23576512455516,-27.5216964137135)) ;
#160237=CARTESIAN_POINT('Origin',(10.1,-3.65625,-26.67)) ;
#160238=CARTESIAN_POINT('Origin',(10.2,-3.65625,-26.67)) ;
#160239=CARTESIAN_POINT('',(10.2,-2.15,-25.365)) ;
#160240=CARTESIAN_POINT('',(10.2,-2.15,-25.7668804065906)) ;
#160241=CARTESIAN_POINT('',(10.2,-2.15,-25.795)) ;
#160242=CARTESIAN_POINT('',(10.2,-2.15,-27.5731195934094)) ;
#160243=CARTESIAN_POINT('Origin',(10.2,-3.65625,-26.67)) ;
#160244=CARTESIAN_POINT('',(10.2,-2.15,-27.975)) ;
#160245=CARTESIAN_POINT('',(10.2,-2.15,-28.075)) ;
#160246=CARTESIAN_POINT('',(10.2,1.9,-27.975)) ;
#160247=CARTESIAN_POINT('',(10.2,2.,-27.975)) ;
#160248=CARTESIAN_POINT('',(10.2,1.9,-25.365)) ;
#160249=CARTESIAN_POINT('',(10.2,1.9,-25.265)) ;
#160250=CARTESIAN_POINT('',(10.2,-2.25,-25.365)) ;
#160251=CARTESIAN_POINT('Origin',(10.2,-2.25,-31.355)) ;
#160252=CARTESIAN_POINT('',(10.1,-2.25,-31.3831195934094)) ;
#160253=CARTESIAN_POINT('',(3.7,-2.25,-31.3831195934094)) ;
#160254=CARTESIAN_POINT('',(10.2,-2.25,-31.3831195934094)) ;
#160255=CARTESIAN_POINT('',(3.7,-2.25,-31.785)) ;
#160256=CARTESIAN_POINT('',(3.7,-2.25,-31.355)) ;
#160257=CARTESIAN_POINT('',(10.1,-2.25,-31.785)) ;
#160258=CARTESIAN_POINT('',(10.2,-2.25,-31.785)) ;
#160259=CARTESIAN_POINT('',(10.1,-2.25,-31.355)) ;
#160260=CARTESIAN_POINT('Origin',(10.2,-2.25,-29.075)) ;
#160261=CARTESIAN_POINT('',(10.1,-2.25,-29.175)) ;
#160262=CARTESIAN_POINT('',(3.7,-2.25,-29.175)) ;
#160263=CARTESIAN_POINT('',(10.2,-2.25,-29.175)) ;
#160264=CARTESIAN_POINT('',(3.7,-2.25,-29.5768804065906)) ;
#160265=CARTESIAN_POINT('',(3.7,-2.25,-29.075)) ;
#160266=CARTESIAN_POINT('',(10.1,-2.25,-29.5768804065906)) ;
#160267=CARTESIAN_POINT('',(10.2,-2.25,-29.5768804065906)) ;
#160268=CARTESIAN_POINT('',(10.1,-2.25,-29.075)) ;
#160269=CARTESIAN_POINT('Origin',(10.2,-3.65625,-30.48)) ;
#160270=CARTESIAN_POINT('',(10.1,-2.23576512455516,-29.6283035862865)) ;
#160271=CARTESIAN_POINT('',(3.7,-2.23576512455516,-29.6283035862865)) ;
#160272=CARTESIAN_POINT('',(10.2,-2.23576512455516,-29.6283035862865)) ;
#160273=CARTESIAN_POINT('',(3.7,-2.23576512455516,-31.3316964137135)) ;
#160274=CARTESIAN_POINT('Origin',(3.7,-3.65625,-30.48)) ;
#160275=CARTESIAN_POINT('',(10.1,-2.23576512455516,-31.3316964137135)) ;
#160276=CARTESIAN_POINT('',(10.2,-2.23576512455516,-31.3316964137135)) ;
#160277=CARTESIAN_POINT('Origin',(10.1,-3.65625,-30.48)) ;
#160278=CARTESIAN_POINT('Origin',(10.2,-3.65625,-30.48)) ;
#160279=CARTESIAN_POINT('',(10.2,-2.15,-29.175)) ;
#160280=CARTESIAN_POINT('',(10.2,-2.15,-29.5768804065906)) ;
#160281=CARTESIAN_POINT('',(10.2,-2.15,-29.605)) ;
#160282=CARTESIAN_POINT('',(10.2,-2.15,-31.3831195934094)) ;
#160283=CARTESIAN_POINT('Origin',(10.2,-3.65625,-30.48)) ;
#160284=CARTESIAN_POINT('',(10.2,-2.15,-31.785)) ;
#160285=CARTESIAN_POINT('',(10.2,-2.15,-31.885)) ;
#160286=CARTESIAN_POINT('',(10.2,1.9,-31.785)) ;
#160287=CARTESIAN_POINT('',(10.2,2.,-31.785)) ;
#160288=CARTESIAN_POINT('',(10.2,1.9,-29.175)) ;
#160289=CARTESIAN_POINT('',(10.2,1.9,-29.075)) ;
#160290=CARTESIAN_POINT('',(10.2,-2.25,-29.175)) ;
#160291=CARTESIAN_POINT('Origin',(10.2,-2.25,-35.165)) ;
#160292=CARTESIAN_POINT('',(10.1,-2.25,-35.1931195934094)) ;
#160293=CARTESIAN_POINT('',(3.7,-2.25,-35.1931195934094)) ;
#160294=CARTESIAN_POINT('',(10.2,-2.25,-35.1931195934094)) ;
#160295=CARTESIAN_POINT('',(3.7,-2.25,-35.595)) ;
#160296=CARTESIAN_POINT('',(3.7,-2.25,-35.165)) ;
#160297=CARTESIAN_POINT('',(10.1,-2.25,-35.595)) ;
#160298=CARTESIAN_POINT('',(10.2,-2.25,-35.595)) ;
#160299=CARTESIAN_POINT('',(10.1,-2.25,-35.165)) ;
#160300=CARTESIAN_POINT('Origin',(10.2,-2.25,-32.885)) ;
#160301=CARTESIAN_POINT('',(10.1,-2.25,-32.985)) ;
#160302=CARTESIAN_POINT('',(3.7,-2.25,-32.985)) ;
#160303=CARTESIAN_POINT('',(10.2,-2.25,-32.985)) ;
#160304=CARTESIAN_POINT('',(3.7,-2.25,-33.3868804065906)) ;
#160305=CARTESIAN_POINT('',(3.7,-2.25,-32.885)) ;
#160306=CARTESIAN_POINT('',(10.1,-2.25,-33.3868804065906)) ;
#160307=CARTESIAN_POINT('',(10.2,-2.25,-33.3868804065906)) ;
#160308=CARTESIAN_POINT('',(10.1,-2.25,-32.885)) ;
#160309=CARTESIAN_POINT('Origin',(10.2,-3.65625,-34.29)) ;
#160310=CARTESIAN_POINT('',(10.1,-2.23576512455516,-33.4383035862865)) ;
#160311=CARTESIAN_POINT('',(3.7,-2.23576512455516,-33.4383035862865)) ;
#160312=CARTESIAN_POINT('',(10.2,-2.23576512455516,-33.4383035862865)) ;
#160313=CARTESIAN_POINT('',(3.7,-2.23576512455516,-35.1416964137135)) ;
#160314=CARTESIAN_POINT('Origin',(3.7,-3.65625,-34.29)) ;
#160315=CARTESIAN_POINT('',(10.1,-2.23576512455516,-35.1416964137135)) ;
#160316=CARTESIAN_POINT('',(10.2,-2.23576512455516,-35.1416964137135)) ;
#160317=CARTESIAN_POINT('Origin',(10.1,-3.65625,-34.29)) ;
#160318=CARTESIAN_POINT('Origin',(10.2,-3.65625,-34.29)) ;
#160319=CARTESIAN_POINT('',(10.2,-2.15,-32.985)) ;
#160320=CARTESIAN_POINT('',(10.2,-2.15,-33.3868804065906)) ;
#160321=CARTESIAN_POINT('',(10.2,-2.15,-33.415)) ;
#160322=CARTESIAN_POINT('',(10.2,-2.15,-35.1931195934094)) ;
#160323=CARTESIAN_POINT('Origin',(10.2,-3.65625,-34.29)) ;
#160324=CARTESIAN_POINT('',(10.2,-2.15,-35.595)) ;
#160325=CARTESIAN_POINT('',(10.2,-2.15,-35.695)) ;
#160326=CARTESIAN_POINT('',(10.2,1.9,-35.595)) ;
#160327=CARTESIAN_POINT('',(10.2,2.,-35.595)) ;
#160328=CARTESIAN_POINT('',(10.2,1.9,-32.985)) ;
#160329=CARTESIAN_POINT('',(10.2,1.9,-32.885)) ;
#160330=CARTESIAN_POINT('',(10.2,-2.25,-32.985)) ;
#160331=CARTESIAN_POINT('Origin',(8.7,0.,-3.81)) ;
#160332=CARTESIAN_POINT('Origin',(8.7,0.,-7.62)) ;
#160333=CARTESIAN_POINT('Origin',(8.7,0.,-11.43)) ;
#160334=CARTESIAN_POINT('Origin',(8.7,0.,-15.24)) ;
#160335=CARTESIAN_POINT('Origin',(8.7,0.,-19.05)) ;
#160336=CARTESIAN_POINT('Origin',(8.7,0.,-22.86)) ;
#160337=CARTESIAN_POINT('Origin',(8.7,0.,-26.67)) ;
#160338=CARTESIAN_POINT('Origin',(8.7,0.,-30.48)) ;
#160339=CARTESIAN_POINT('Origin',(8.7,0.,-34.29)) ;
#160340=CARTESIAN_POINT('Origin',(-2.,4.4,-35.29)) ;
#160341=CARTESIAN_POINT('',(-2.,4.35,-35.19)) ;
#160342=CARTESIAN_POINT('',(-2.,4.35,-33.39)) ;
#160343=CARTESIAN_POINT('',(-2.,4.35,-35.29)) ;
#160344=CARTESIAN_POINT('',(-2.,4.45,-33.39)) ;
#160345=CARTESIAN_POINT('',(-2.,4.55,-33.39)) ;
#160346=CARTESIAN_POINT('',(-2.,4.45,-35.19)) ;
#160347=CARTESIAN_POINT('',(-2.,4.45,-35.29)) ;
#160348=CARTESIAN_POINT('',(-2.,4.25,-35.19)) ;
#160349=CARTESIAN_POINT('Origin',(-3.,4.4,-33.29)) ;
#160350=CARTESIAN_POINT('',(-2.9,4.45,-33.29)) ;
#160351=CARTESIAN_POINT('',(-2.1,4.45,-33.29)) ;
#160352=CARTESIAN_POINT('',(-2.,4.45,-33.29)) ;
#160353=CARTESIAN_POINT('',(-2.1,4.35,-33.29)) ;
#160354=CARTESIAN_POINT('',(-2.1,4.25,-33.29)) ;
#160355=CARTESIAN_POINT('',(-2.9,4.35,-33.29)) ;
#160356=CARTESIAN_POINT('',(-3.,4.35,-33.29)) ;
#160357=CARTESIAN_POINT('',(-2.9,4.55,-33.29)) ;
#160358=CARTESIAN_POINT('Origin',(-3.,4.4,-35.29)) ;
#160359=CARTESIAN_POINT('',(-3.,4.45,-33.39)) ;
#160360=CARTESIAN_POINT('',(-3.,4.35,-33.39)) ;
#160361=CARTESIAN_POINT('',(-3.,4.25,-33.39)) ;
#160362=CARTESIAN_POINT('',(-3.,4.35,-35.19)) ;
#160363=CARTESIAN_POINT('',(-3.,4.35,-35.29)) ;
#160364=CARTESIAN_POINT('',(-3.,4.45,-35.19)) ;
#160365=CARTESIAN_POINT('',(-3.,4.55,-35.19)) ;
#160366=CARTESIAN_POINT('',(-3.,4.45,-33.29)) ;
#160367=CARTESIAN_POINT('Origin',(-3.,4.4,-35.29)) ;
#160368=CARTESIAN_POINT('',(-2.9,4.35,-35.29)) ;
#160369=CARTESIAN_POINT('',(-2.1,4.35,-35.29)) ;
#160370=CARTESIAN_POINT('',(-3.,4.35,-35.29)) ;
#160371=CARTESIAN_POINT('',(-2.1,4.45,-35.29)) ;
#160372=CARTESIAN_POINT('',(-2.1,4.55,-35.29)) ;
#160373=CARTESIAN_POINT('',(-2.9,4.45,-35.29)) ;
#160374=CARTESIAN_POINT('',(-3.,4.45,-35.29)) ;
#160375=CARTESIAN_POINT('',(-2.9,4.25,-35.29)) ;
#160376=CARTESIAN_POINT('Origin',(-2.,4.4,-31.48)) ;
#160377=CARTESIAN_POINT('',(-2.,4.35,-31.38)) ;
#160378=CARTESIAN_POINT('',(-2.,4.35,-29.58)) ;
#160379=CARTESIAN_POINT('',(-2.,4.35,-31.48)) ;
#160380=CARTESIAN_POINT('',(-2.,4.45,-29.58)) ;
#160381=CARTESIAN_POINT('',(-2.,4.55,-29.58)) ;
#160382=CARTESIAN_POINT('',(-2.,4.45,-31.38)) ;
#160383=CARTESIAN_POINT('',(-2.,4.45,-31.48)) ;
#160384=CARTESIAN_POINT('',(-2.,4.25,-31.38)) ;
#160385=CARTESIAN_POINT('Origin',(-3.,4.4,-29.48)) ;
#160386=CARTESIAN_POINT('',(-2.9,4.45,-29.48)) ;
#160387=CARTESIAN_POINT('',(-2.1,4.45,-29.48)) ;
#160388=CARTESIAN_POINT('',(-2.,4.45,-29.48)) ;
#160389=CARTESIAN_POINT('',(-2.1,4.35,-29.48)) ;
#160390=CARTESIAN_POINT('',(-2.1,4.25,-29.48)) ;
#160391=CARTESIAN_POINT('',(-2.9,4.35,-29.48)) ;
#160392=CARTESIAN_POINT('',(-3.,4.35,-29.48)) ;
#160393=CARTESIAN_POINT('',(-2.9,4.55,-29.48)) ;
#160394=CARTESIAN_POINT('Origin',(-3.,4.4,-31.48)) ;
#160395=CARTESIAN_POINT('',(-3.,4.45,-29.58)) ;
#160396=CARTESIAN_POINT('',(-3.,4.35,-29.58)) ;
#160397=CARTESIAN_POINT('',(-3.,4.25,-29.58)) ;
#160398=CARTESIAN_POINT('',(-3.,4.35,-31.38)) ;
#160399=CARTESIAN_POINT('',(-3.,4.35,-31.48)) ;
#160400=CARTESIAN_POINT('',(-3.,4.45,-31.38)) ;
#160401=CARTESIAN_POINT('',(-3.,4.55,-31.38)) ;
#160402=CARTESIAN_POINT('',(-3.,4.45,-29.48)) ;
#160403=CARTESIAN_POINT('Origin',(-3.,4.4,-31.48)) ;
#160404=CARTESIAN_POINT('',(-2.9,4.35,-31.48)) ;
#160405=CARTESIAN_POINT('',(-2.1,4.35,-31.48)) ;
#160406=CARTESIAN_POINT('',(-3.,4.35,-31.48)) ;
#160407=CARTESIAN_POINT('',(-2.1,4.45,-31.48)) ;
#160408=CARTESIAN_POINT('',(-2.1,4.55,-31.48)) ;
#160409=CARTESIAN_POINT('',(-2.9,4.45,-31.48)) ;
#160410=CARTESIAN_POINT('',(-3.,4.45,-31.48)) ;
#160411=CARTESIAN_POINT('',(-2.9,4.25,-31.48)) ;
#160412=CARTESIAN_POINT('Origin',(-2.,4.4,-27.67)) ;
#160413=CARTESIAN_POINT('',(-2.,4.35,-27.57)) ;
#160414=CARTESIAN_POINT('',(-2.,4.35,-25.77)) ;
#160415=CARTESIAN_POINT('',(-2.,4.35,-27.67)) ;
#160416=CARTESIAN_POINT('',(-2.,4.45,-25.77)) ;
#160417=CARTESIAN_POINT('',(-2.,4.55,-25.77)) ;
#160418=CARTESIAN_POINT('',(-2.,4.45,-27.57)) ;
#160419=CARTESIAN_POINT('',(-2.,4.45,-27.67)) ;
#160420=CARTESIAN_POINT('',(-2.,4.25,-27.57)) ;
#160421=CARTESIAN_POINT('Origin',(-3.,4.4,-25.67)) ;
#160422=CARTESIAN_POINT('',(-2.9,4.45,-25.67)) ;
#160423=CARTESIAN_POINT('',(-2.1,4.45,-25.67)) ;
#160424=CARTESIAN_POINT('',(-2.,4.45,-25.67)) ;
#160425=CARTESIAN_POINT('',(-2.1,4.35,-25.67)) ;
#160426=CARTESIAN_POINT('',(-2.1,4.25,-25.67)) ;
#160427=CARTESIAN_POINT('',(-2.9,4.35,-25.67)) ;
#160428=CARTESIAN_POINT('',(-3.,4.35,-25.67)) ;
#160429=CARTESIAN_POINT('',(-2.9,4.55,-25.67)) ;
#160430=CARTESIAN_POINT('Origin',(-3.,4.4,-27.67)) ;
#160431=CARTESIAN_POINT('',(-3.,4.45,-25.77)) ;
#160432=CARTESIAN_POINT('',(-3.,4.35,-25.77)) ;
#160433=CARTESIAN_POINT('',(-3.,4.25,-25.77)) ;
#160434=CARTESIAN_POINT('',(-3.,4.35,-27.57)) ;
#160435=CARTESIAN_POINT('',(-3.,4.35,-27.67)) ;
#160436=CARTESIAN_POINT('',(-3.,4.45,-27.57)) ;
#160437=CARTESIAN_POINT('',(-3.,4.55,-27.57)) ;
#160438=CARTESIAN_POINT('',(-3.,4.45,-25.67)) ;
#160439=CARTESIAN_POINT('Origin',(-3.,4.4,-27.67)) ;
#160440=CARTESIAN_POINT('',(-2.9,4.35,-27.67)) ;
#160441=CARTESIAN_POINT('',(-2.1,4.35,-27.67)) ;
#160442=CARTESIAN_POINT('',(-3.,4.35,-27.67)) ;
#160443=CARTESIAN_POINT('',(-2.1,4.45,-27.67)) ;
#160444=CARTESIAN_POINT('',(-2.1,4.55,-27.67)) ;
#160445=CARTESIAN_POINT('',(-2.9,4.45,-27.67)) ;
#160446=CARTESIAN_POINT('',(-3.,4.45,-27.67)) ;
#160447=CARTESIAN_POINT('',(-2.9,4.25,-27.67)) ;
#160448=CARTESIAN_POINT('Origin',(-2.,4.4,-23.86)) ;
#160449=CARTESIAN_POINT('',(-2.,4.35,-23.76)) ;
#160450=CARTESIAN_POINT('',(-2.,4.35,-21.96)) ;
#160451=CARTESIAN_POINT('',(-2.,4.35,-23.86)) ;
#160452=CARTESIAN_POINT('',(-2.,4.45,-21.96)) ;
#160453=CARTESIAN_POINT('',(-2.,4.55,-21.96)) ;
#160454=CARTESIAN_POINT('',(-2.,4.45,-23.76)) ;
#160455=CARTESIAN_POINT('',(-2.,4.45,-23.86)) ;
#160456=CARTESIAN_POINT('',(-2.,4.25,-23.76)) ;
#160457=CARTESIAN_POINT('Origin',(-3.,4.4,-21.86)) ;
#160458=CARTESIAN_POINT('',(-2.9,4.45,-21.86)) ;
#160459=CARTESIAN_POINT('',(-2.1,4.45,-21.86)) ;
#160460=CARTESIAN_POINT('',(-2.,4.45,-21.86)) ;
#160461=CARTESIAN_POINT('',(-2.1,4.35,-21.86)) ;
#160462=CARTESIAN_POINT('',(-2.1,4.25,-21.86)) ;
#160463=CARTESIAN_POINT('',(-2.9,4.35,-21.86)) ;
#160464=CARTESIAN_POINT('',(-3.,4.35,-21.86)) ;
#160465=CARTESIAN_POINT('',(-2.9,4.55,-21.86)) ;
#160466=CARTESIAN_POINT('Origin',(-3.,4.4,-23.86)) ;
#160467=CARTESIAN_POINT('',(-3.,4.45,-21.96)) ;
#160468=CARTESIAN_POINT('',(-3.,4.35,-21.96)) ;
#160469=CARTESIAN_POINT('',(-3.,4.25,-21.96)) ;
#160470=CARTESIAN_POINT('',(-3.,4.35,-23.76)) ;
#160471=CARTESIAN_POINT('',(-3.,4.35,-23.86)) ;
#160472=CARTESIAN_POINT('',(-3.,4.45,-23.76)) ;
#160473=CARTESIAN_POINT('',(-3.,4.55,-23.76)) ;
#160474=CARTESIAN_POINT('',(-3.,4.45,-21.86)) ;
#160475=CARTESIAN_POINT('Origin',(-3.,4.4,-23.86)) ;
#160476=CARTESIAN_POINT('',(-2.9,4.35,-23.86)) ;
#160477=CARTESIAN_POINT('',(-2.1,4.35,-23.86)) ;
#160478=CARTESIAN_POINT('',(-3.,4.35,-23.86)) ;
#160479=CARTESIAN_POINT('',(-2.1,4.45,-23.86)) ;
#160480=CARTESIAN_POINT('',(-2.1,4.55,-23.86)) ;
#160481=CARTESIAN_POINT('',(-2.9,4.45,-23.86)) ;
#160482=CARTESIAN_POINT('',(-3.,4.45,-23.86)) ;
#160483=CARTESIAN_POINT('',(-2.9,4.25,-23.86)) ;
#160484=CARTESIAN_POINT('Origin',(-2.,4.4,-20.05)) ;
#160485=CARTESIAN_POINT('',(-2.,4.35,-19.95)) ;
#160486=CARTESIAN_POINT('',(-2.,4.35,-18.15)) ;
#160487=CARTESIAN_POINT('',(-2.,4.35,-20.05)) ;
#160488=CARTESIAN_POINT('',(-2.,4.45,-18.15)) ;
#160489=CARTESIAN_POINT('',(-2.,4.55,-18.15)) ;
#160490=CARTESIAN_POINT('',(-2.,4.45,-19.95)) ;
#160491=CARTESIAN_POINT('',(-2.,4.45,-20.05)) ;
#160492=CARTESIAN_POINT('',(-2.,4.25,-19.95)) ;
#160493=CARTESIAN_POINT('Origin',(-3.,4.4,-18.05)) ;
#160494=CARTESIAN_POINT('',(-2.9,4.45,-18.05)) ;
#160495=CARTESIAN_POINT('',(-2.1,4.45,-18.05)) ;
#160496=CARTESIAN_POINT('',(-2.,4.45,-18.05)) ;
#160497=CARTESIAN_POINT('',(-2.1,4.35,-18.05)) ;
#160498=CARTESIAN_POINT('',(-2.1,4.25,-18.05)) ;
#160499=CARTESIAN_POINT('',(-2.9,4.35,-18.05)) ;
#160500=CARTESIAN_POINT('',(-3.,4.35,-18.05)) ;
#160501=CARTESIAN_POINT('',(-2.9,4.55,-18.05)) ;
#160502=CARTESIAN_POINT('Origin',(-3.,4.4,-20.05)) ;
#160503=CARTESIAN_POINT('',(-3.,4.45,-18.15)) ;
#160504=CARTESIAN_POINT('',(-3.,4.35,-18.15)) ;
#160505=CARTESIAN_POINT('',(-3.,4.25,-18.15)) ;
#160506=CARTESIAN_POINT('',(-3.,4.35,-19.95)) ;
#160507=CARTESIAN_POINT('',(-3.,4.35,-20.05)) ;
#160508=CARTESIAN_POINT('',(-3.,4.45,-19.95)) ;
#160509=CARTESIAN_POINT('',(-3.,4.55,-19.95)) ;
#160510=CARTESIAN_POINT('',(-3.,4.45,-18.05)) ;
#160511=CARTESIAN_POINT('Origin',(-3.,4.4,-20.05)) ;
#160512=CARTESIAN_POINT('',(-2.9,4.35,-20.05)) ;
#160513=CARTESIAN_POINT('',(-2.1,4.35,-20.05)) ;
#160514=CARTESIAN_POINT('',(-3.,4.35,-20.05)) ;
#160515=CARTESIAN_POINT('',(-2.1,4.45,-20.05)) ;
#160516=CARTESIAN_POINT('',(-2.1,4.55,-20.05)) ;
#160517=CARTESIAN_POINT('',(-2.9,4.45,-20.05)) ;
#160518=CARTESIAN_POINT('',(-3.,4.45,-20.05)) ;
#160519=CARTESIAN_POINT('',(-2.9,4.25,-20.05)) ;
#160520=CARTESIAN_POINT('Origin',(-2.,4.4,-16.24)) ;
#160521=CARTESIAN_POINT('',(-2.,4.35,-16.14)) ;
#160522=CARTESIAN_POINT('',(-2.,4.35,-14.34)) ;
#160523=CARTESIAN_POINT('',(-2.,4.35,-16.24)) ;
#160524=CARTESIAN_POINT('',(-2.,4.45,-14.34)) ;
#160525=CARTESIAN_POINT('',(-2.,4.55,-14.34)) ;
#160526=CARTESIAN_POINT('',(-2.,4.45,-16.14)) ;
#160527=CARTESIAN_POINT('',(-2.,4.45,-16.24)) ;
#160528=CARTESIAN_POINT('',(-2.,4.25,-16.14)) ;
#160529=CARTESIAN_POINT('Origin',(-3.,4.4,-14.24)) ;
#160530=CARTESIAN_POINT('',(-2.9,4.45,-14.24)) ;
#160531=CARTESIAN_POINT('',(-2.1,4.45,-14.24)) ;
#160532=CARTESIAN_POINT('',(-2.,4.45,-14.24)) ;
#160533=CARTESIAN_POINT('',(-2.1,4.35,-14.24)) ;
#160534=CARTESIAN_POINT('',(-2.1,4.25,-14.24)) ;
#160535=CARTESIAN_POINT('',(-2.9,4.35,-14.24)) ;
#160536=CARTESIAN_POINT('',(-3.,4.35,-14.24)) ;
#160537=CARTESIAN_POINT('',(-2.9,4.55,-14.24)) ;
#160538=CARTESIAN_POINT('Origin',(-3.,4.4,-16.24)) ;
#160539=CARTESIAN_POINT('',(-3.,4.45,-14.34)) ;
#160540=CARTESIAN_POINT('',(-3.,4.35,-14.34)) ;
#160541=CARTESIAN_POINT('',(-3.,4.25,-14.34)) ;
#160542=CARTESIAN_POINT('',(-3.,4.35,-16.14)) ;
#160543=CARTESIAN_POINT('',(-3.,4.35,-16.24)) ;
#160544=CARTESIAN_POINT('',(-3.,4.45,-16.14)) ;
#160545=CARTESIAN_POINT('',(-3.,4.55,-16.14)) ;
#160546=CARTESIAN_POINT('',(-3.,4.45,-14.24)) ;
#160547=CARTESIAN_POINT('Origin',(-3.,4.4,-16.24)) ;
#160548=CARTESIAN_POINT('',(-2.9,4.35,-16.24)) ;
#160549=CARTESIAN_POINT('',(-2.1,4.35,-16.24)) ;
#160550=CARTESIAN_POINT('',(-3.,4.35,-16.24)) ;
#160551=CARTESIAN_POINT('',(-2.1,4.45,-16.24)) ;
#160552=CARTESIAN_POINT('',(-2.1,4.55,-16.24)) ;
#160553=CARTESIAN_POINT('',(-2.9,4.45,-16.24)) ;
#160554=CARTESIAN_POINT('',(-3.,4.45,-16.24)) ;
#160555=CARTESIAN_POINT('',(-2.9,4.25,-16.24)) ;
#160556=CARTESIAN_POINT('Origin',(-2.,4.4,-12.43)) ;
#160557=CARTESIAN_POINT('',(-2.,4.35,-12.33)) ;
#160558=CARTESIAN_POINT('',(-2.,4.35,-10.53)) ;
#160559=CARTESIAN_POINT('',(-2.,4.35,-12.43)) ;
#160560=CARTESIAN_POINT('',(-2.,4.45,-10.53)) ;
#160561=CARTESIAN_POINT('',(-2.,4.55,-10.53)) ;
#160562=CARTESIAN_POINT('',(-2.,4.45,-12.33)) ;
#160563=CARTESIAN_POINT('',(-2.,4.45,-12.43)) ;
#160564=CARTESIAN_POINT('',(-2.,4.25,-12.33)) ;
#160565=CARTESIAN_POINT('Origin',(-3.,4.4,-10.43)) ;
#160566=CARTESIAN_POINT('',(-2.9,4.45,-10.43)) ;
#160567=CARTESIAN_POINT('',(-2.1,4.45,-10.43)) ;
#160568=CARTESIAN_POINT('',(-2.,4.45,-10.43)) ;
#160569=CARTESIAN_POINT('',(-2.1,4.35,-10.43)) ;
#160570=CARTESIAN_POINT('',(-2.1,4.25,-10.43)) ;
#160571=CARTESIAN_POINT('',(-2.9,4.35,-10.43)) ;
#160572=CARTESIAN_POINT('',(-3.,4.35,-10.43)) ;
#160573=CARTESIAN_POINT('',(-2.9,4.55,-10.43)) ;
#160574=CARTESIAN_POINT('Origin',(-3.,4.4,-12.43)) ;
#160575=CARTESIAN_POINT('',(-3.,4.45,-10.53)) ;
#160576=CARTESIAN_POINT('',(-3.,4.35,-10.53)) ;
#160577=CARTESIAN_POINT('',(-3.,4.25,-10.53)) ;
#160578=CARTESIAN_POINT('',(-3.,4.35,-12.33)) ;
#160579=CARTESIAN_POINT('',(-3.,4.35,-12.43)) ;
#160580=CARTESIAN_POINT('',(-3.,4.45,-12.33)) ;
#160581=CARTESIAN_POINT('',(-3.,4.55,-12.33)) ;
#160582=CARTESIAN_POINT('',(-3.,4.45,-10.43)) ;
#160583=CARTESIAN_POINT('Origin',(-3.,4.4,-12.43)) ;
#160584=CARTESIAN_POINT('',(-2.9,4.35,-12.43)) ;
#160585=CARTESIAN_POINT('',(-2.1,4.35,-12.43)) ;
#160586=CARTESIAN_POINT('',(-3.,4.35,-12.43)) ;
#160587=CARTESIAN_POINT('',(-2.1,4.45,-12.43)) ;
#160588=CARTESIAN_POINT('',(-2.1,4.55,-12.43)) ;
#160589=CARTESIAN_POINT('',(-2.9,4.45,-12.43)) ;
#160590=CARTESIAN_POINT('',(-3.,4.45,-12.43)) ;
#160591=CARTESIAN_POINT('',(-2.9,4.25,-12.43)) ;
#160592=CARTESIAN_POINT('Origin',(-2.,4.4,-8.62)) ;
#160593=CARTESIAN_POINT('',(-2.,4.35,-8.52)) ;
#160594=CARTESIAN_POINT('',(-2.,4.35,-6.72)) ;
#160595=CARTESIAN_POINT('',(-2.,4.35,-8.62)) ;
#160596=CARTESIAN_POINT('',(-2.,4.45,-6.72)) ;
#160597=CARTESIAN_POINT('',(-2.,4.55,-6.72)) ;
#160598=CARTESIAN_POINT('',(-2.,4.45,-8.52)) ;
#160599=CARTESIAN_POINT('',(-2.,4.45,-8.62)) ;
#160600=CARTESIAN_POINT('',(-2.,4.25,-8.52)) ;
#160601=CARTESIAN_POINT('Origin',(-3.,4.4,-6.62)) ;
#160602=CARTESIAN_POINT('',(-2.9,4.45,-6.62)) ;
#160603=CARTESIAN_POINT('',(-2.1,4.45,-6.62)) ;
#160604=CARTESIAN_POINT('',(-2.,4.45,-6.62)) ;
#160605=CARTESIAN_POINT('',(-2.1,4.35,-6.62)) ;
#160606=CARTESIAN_POINT('',(-2.1,4.25,-6.62)) ;
#160607=CARTESIAN_POINT('',(-2.9,4.35,-6.62)) ;
#160608=CARTESIAN_POINT('',(-3.,4.35,-6.62)) ;
#160609=CARTESIAN_POINT('',(-2.9,4.55,-6.62)) ;
#160610=CARTESIAN_POINT('Origin',(-3.,4.4,-8.62)) ;
#160611=CARTESIAN_POINT('',(-3.,4.45,-6.72)) ;
#160612=CARTESIAN_POINT('',(-3.,4.35,-6.72)) ;
#160613=CARTESIAN_POINT('',(-3.,4.25,-6.72)) ;
#160614=CARTESIAN_POINT('',(-3.,4.35,-8.52)) ;
#160615=CARTESIAN_POINT('',(-3.,4.35,-8.62)) ;
#160616=CARTESIAN_POINT('',(-3.,4.45,-8.52)) ;
#160617=CARTESIAN_POINT('',(-3.,4.55,-8.52)) ;
#160618=CARTESIAN_POINT('',(-3.,4.45,-6.62)) ;
#160619=CARTESIAN_POINT('Origin',(-3.,4.4,-8.62)) ;
#160620=CARTESIAN_POINT('',(-2.9,4.35,-8.62)) ;
#160621=CARTESIAN_POINT('',(-2.1,4.35,-8.62)) ;
#160622=CARTESIAN_POINT('',(-3.,4.35,-8.62)) ;
#160623=CARTESIAN_POINT('',(-2.1,4.45,-8.62)) ;
#160624=CARTESIAN_POINT('',(-2.1,4.55,-8.62)) ;
#160625=CARTESIAN_POINT('',(-2.9,4.45,-8.62)) ;
#160626=CARTESIAN_POINT('',(-3.,4.45,-8.62)) ;
#160627=CARTESIAN_POINT('',(-2.9,4.25,-8.62)) ;
#160628=CARTESIAN_POINT('Origin',(-2.,4.4,-4.81)) ;
#160629=CARTESIAN_POINT('',(-2.,4.35,-4.71)) ;
#160630=CARTESIAN_POINT('',(-2.,4.35,-2.91)) ;
#160631=CARTESIAN_POINT('',(-2.,4.35,-4.81)) ;
#160632=CARTESIAN_POINT('',(-2.,4.45,-2.91)) ;
#160633=CARTESIAN_POINT('',(-2.,4.55,-2.91)) ;
#160634=CARTESIAN_POINT('',(-2.,4.45,-4.71)) ;
#160635=CARTESIAN_POINT('',(-2.,4.45,-4.81)) ;
#160636=CARTESIAN_POINT('',(-2.,4.25,-4.71)) ;
#160637=CARTESIAN_POINT('Origin',(-3.,4.4,-2.81)) ;
#160638=CARTESIAN_POINT('',(-2.9,4.45,-2.81)) ;
#160639=CARTESIAN_POINT('',(-2.1,4.45,-2.81)) ;
#160640=CARTESIAN_POINT('',(-2.,4.45,-2.81)) ;
#160641=CARTESIAN_POINT('',(-2.1,4.35,-2.81)) ;
#160642=CARTESIAN_POINT('',(-2.1,4.25,-2.81)) ;
#160643=CARTESIAN_POINT('',(-2.9,4.35,-2.81)) ;
#160644=CARTESIAN_POINT('',(-3.,4.35,-2.81)) ;
#160645=CARTESIAN_POINT('',(-2.9,4.55,-2.81)) ;
#160646=CARTESIAN_POINT('Origin',(-3.,4.4,-4.81)) ;
#160647=CARTESIAN_POINT('',(-3.,4.45,-2.91)) ;
#160648=CARTESIAN_POINT('',(-3.,4.35,-2.91)) ;
#160649=CARTESIAN_POINT('',(-3.,4.25,-2.91)) ;
#160650=CARTESIAN_POINT('',(-3.,4.35,-4.71)) ;
#160651=CARTESIAN_POINT('',(-3.,4.35,-4.81)) ;
#160652=CARTESIAN_POINT('',(-3.,4.45,-4.71)) ;
#160653=CARTESIAN_POINT('',(-3.,4.55,-4.71)) ;
#160654=CARTESIAN_POINT('',(-3.,4.45,-2.81)) ;
#160655=CARTESIAN_POINT('Origin',(-3.,4.4,-4.81)) ;
#160656=CARTESIAN_POINT('',(-2.9,4.35,-4.81)) ;
#160657=CARTESIAN_POINT('',(-2.1,4.35,-4.81)) ;
#160658=CARTESIAN_POINT('',(-3.,4.35,-4.81)) ;
#160659=CARTESIAN_POINT('',(-2.1,4.45,-4.81)) ;
#160660=CARTESIAN_POINT('',(-2.1,4.55,-4.81)) ;
#160661=CARTESIAN_POINT('',(-2.9,4.45,-4.81)) ;
#160662=CARTESIAN_POINT('',(-3.,4.45,-4.81)) ;
#160663=CARTESIAN_POINT('',(-2.9,4.25,-4.81)) ;
#160664=CARTESIAN_POINT('Origin',(0.,4.25,-3.81)) ;
#160665=CARTESIAN_POINT('',(-2.9,4.25,-4.71)) ;
#160666=CARTESIAN_POINT('',(-2.9,4.25,-2.91)) ;
#160667=CARTESIAN_POINT('',(-2.9,4.25,-3.81)) ;
#160668=CARTESIAN_POINT('',(-2.1,4.25,-2.91)) ;
#160669=CARTESIAN_POINT('',(-1.95156391047391E-16,4.25,-2.91)) ;
#160670=CARTESIAN_POINT('',(-2.1,4.25,-4.71)) ;
#160671=CARTESIAN_POINT('',(-2.1,4.25,-3.81)) ;
#160672=CARTESIAN_POINT('',(-1.95156391047391E-16,4.25,-4.71)) ;
#160673=CARTESIAN_POINT('',(-2.75,4.25,-2.96)) ;
#160674=CARTESIAN_POINT('',(-2.25,4.25,-2.96)) ;
#160675=CARTESIAN_POINT('',(-2.85,4.25,-2.96)) ;
#160676=CARTESIAN_POINT('',(-2.85,4.25,-3.06)) ;
#160677=CARTESIAN_POINT('Origin',(-2.75,4.25,-3.06)) ;
#160678=CARTESIAN_POINT('',(-2.85,4.25,-4.56)) ;
#160679=CARTESIAN_POINT('',(-2.85,4.25,-4.66)) ;
#160680=CARTESIAN_POINT('',(-2.75,4.25,-4.66)) ;
#160681=CARTESIAN_POINT('Origin',(-2.75,4.25,-4.56)) ;
#160682=CARTESIAN_POINT('',(-2.25,4.25,-4.66)) ;
#160683=CARTESIAN_POINT('',(-2.15,4.25,-4.66)) ;
#160684=CARTESIAN_POINT('',(-2.15,4.25,-4.56)) ;
#160685=CARTESIAN_POINT('Origin',(-2.25,4.25,-4.56)) ;
#160686=CARTESIAN_POINT('',(-2.15,4.25,-3.06)) ;
#160687=CARTESIAN_POINT('',(-2.15,4.25,-2.96)) ;
#160688=CARTESIAN_POINT('Origin',(-2.25,4.25,-3.06)) ;
#160689=CARTESIAN_POINT('Origin',(-2.15,4.25,-2.96)) ;
#160690=CARTESIAN_POINT('',(-2.15,4.3,-4.56)) ;
#160691=CARTESIAN_POINT('',(-2.15,4.3,-3.06)) ;
#160692=CARTESIAN_POINT('',(-2.15,4.3,-2.96)) ;
#160693=CARTESIAN_POINT('',(-2.15,4.25,-3.06)) ;
#160694=CARTESIAN_POINT('',(-2.15,4.25,-4.56)) ;
#160695=CARTESIAN_POINT('Origin',(-2.85,4.25,-2.96)) ;
#160696=CARTESIAN_POINT('',(-2.25,4.3,-2.96)) ;
#160697=CARTESIAN_POINT('',(-2.75,4.3,-2.96)) ;
#160698=CARTESIAN_POINT('',(-2.85,4.3,-2.96)) ;
#160699=CARTESIAN_POINT('',(-2.75,4.25,-2.96)) ;
#160700=CARTESIAN_POINT('',(-2.25,4.25,-2.96)) ;
#160701=CARTESIAN_POINT('Origin',(-2.85,4.25,-4.66)) ;
#160702=CARTESIAN_POINT('',(-2.85,4.3,-3.06)) ;
#160703=CARTESIAN_POINT('',(-2.85,4.25,-3.06)) ;
#160704=CARTESIAN_POINT('',(-2.85,4.3,-4.56)) ;
#160705=CARTESIAN_POINT('',(-2.85,4.3,-4.66)) ;
#160706=CARTESIAN_POINT('',(-2.85,4.25,-4.56)) ;
#160707=CARTESIAN_POINT('Origin',(-2.15,4.25,-4.66)) ;
#160708=CARTESIAN_POINT('',(-2.75,4.3,-4.66)) ;
#160709=CARTESIAN_POINT('',(-2.25,4.3,-4.66)) ;
#160710=CARTESIAN_POINT('',(-2.15,4.3,-4.66)) ;
#160711=CARTESIAN_POINT('',(-2.25,4.25,-4.66)) ;
#160712=CARTESIAN_POINT('',(-2.75,4.25,-4.66)) ;
#160713=CARTESIAN_POINT('Origin',(0.,4.25,-7.62)) ;
#160714=CARTESIAN_POINT('',(-2.9,4.25,-8.52)) ;
#160715=CARTESIAN_POINT('',(-2.9,4.25,-6.72)) ;
#160716=CARTESIAN_POINT('',(-2.9,4.25,-7.62)) ;
#160717=CARTESIAN_POINT('',(-2.1,4.25,-6.72)) ;
#160718=CARTESIAN_POINT('',(-1.95156391047391E-16,4.25,-6.72)) ;
#160719=CARTESIAN_POINT('',(-2.1,4.25,-8.52)) ;
#160720=CARTESIAN_POINT('',(-2.1,4.25,-7.62)) ;
#160721=CARTESIAN_POINT('',(-1.95156391047391E-16,4.25,-8.52)) ;
#160722=CARTESIAN_POINT('',(-2.75,4.25,-6.77)) ;
#160723=CARTESIAN_POINT('',(-2.25,4.25,-6.77)) ;
#160724=CARTESIAN_POINT('',(-2.85,4.25,-6.77)) ;
#160725=CARTESIAN_POINT('',(-2.85,4.25,-6.87)) ;
#160726=CARTESIAN_POINT('Origin',(-2.75,4.25,-6.87)) ;
#160727=CARTESIAN_POINT('',(-2.85,4.25,-8.37)) ;
#160728=CARTESIAN_POINT('',(-2.85,4.25,-8.47)) ;
#160729=CARTESIAN_POINT('',(-2.75,4.25,-8.47)) ;
#160730=CARTESIAN_POINT('Origin',(-2.75,4.25,-8.37)) ;
#160731=CARTESIAN_POINT('',(-2.25,4.25,-8.47)) ;
#160732=CARTESIAN_POINT('',(-2.15,4.25,-8.47)) ;
#160733=CARTESIAN_POINT('',(-2.15,4.25,-8.37)) ;
#160734=CARTESIAN_POINT('Origin',(-2.25,4.25,-8.37)) ;
#160735=CARTESIAN_POINT('',(-2.15,4.25,-6.87)) ;
#160736=CARTESIAN_POINT('',(-2.15,4.25,-6.77)) ;
#160737=CARTESIAN_POINT('Origin',(-2.25,4.25,-6.87)) ;
#160738=CARTESIAN_POINT('Origin',(-2.15,4.25,-6.77)) ;
#160739=CARTESIAN_POINT('',(-2.15,4.3,-8.37)) ;
#160740=CARTESIAN_POINT('',(-2.15,4.3,-6.87)) ;
#160741=CARTESIAN_POINT('',(-2.15,4.3,-6.77)) ;
#160742=CARTESIAN_POINT('',(-2.15,4.25,-6.87)) ;
#160743=CARTESIAN_POINT('',(-2.15,4.25,-8.37)) ;
#160744=CARTESIAN_POINT('Origin',(-2.85,4.25,-6.77)) ;
#160745=CARTESIAN_POINT('',(-2.25,4.3,-6.77)) ;
#160746=CARTESIAN_POINT('',(-2.75,4.3,-6.77)) ;
#160747=CARTESIAN_POINT('',(-2.85,4.3,-6.77)) ;
#160748=CARTESIAN_POINT('',(-2.75,4.25,-6.77)) ;
#160749=CARTESIAN_POINT('',(-2.25,4.25,-6.77)) ;
#160750=CARTESIAN_POINT('Origin',(-2.85,4.25,-8.47)) ;
#160751=CARTESIAN_POINT('',(-2.85,4.3,-6.87)) ;
#160752=CARTESIAN_POINT('',(-2.85,4.25,-6.87)) ;
#160753=CARTESIAN_POINT('',(-2.85,4.3,-8.37)) ;
#160754=CARTESIAN_POINT('',(-2.85,4.3,-8.47)) ;
#160755=CARTESIAN_POINT('',(-2.85,4.25,-8.37)) ;
#160756=CARTESIAN_POINT('Origin',(-2.15,4.25,-8.47)) ;
#160757=CARTESIAN_POINT('',(-2.75,4.3,-8.47)) ;
#160758=CARTESIAN_POINT('',(-2.25,4.3,-8.47)) ;
#160759=CARTESIAN_POINT('',(-2.15,4.3,-8.47)) ;
#160760=CARTESIAN_POINT('',(-2.25,4.25,-8.47)) ;
#160761=CARTESIAN_POINT('',(-2.75,4.25,-8.47)) ;
#160762=CARTESIAN_POINT('Origin',(0.,4.25,-11.43)) ;
#160763=CARTESIAN_POINT('',(-2.9,4.25,-12.33)) ;
#160764=CARTESIAN_POINT('',(-2.9,4.25,-10.53)) ;
#160765=CARTESIAN_POINT('',(-2.9,4.25,-11.43)) ;
#160766=CARTESIAN_POINT('',(-2.1,4.25,-10.53)) ;
#160767=CARTESIAN_POINT('',(-1.95156391047391E-16,4.25,-10.53)) ;
#160768=CARTESIAN_POINT('',(-2.1,4.25,-12.33)) ;
#160769=CARTESIAN_POINT('',(-2.1,4.25,-11.43)) ;
#160770=CARTESIAN_POINT('',(-1.95156391047391E-16,4.25,-12.33)) ;
#160771=CARTESIAN_POINT('',(-2.75,4.25,-10.58)) ;
#160772=CARTESIAN_POINT('',(-2.25,4.25,-10.58)) ;
#160773=CARTESIAN_POINT('',(-2.85,4.25,-10.58)) ;
#160774=CARTESIAN_POINT('',(-2.85,4.25,-10.68)) ;
#160775=CARTESIAN_POINT('Origin',(-2.75,4.25,-10.68)) ;
#160776=CARTESIAN_POINT('',(-2.85,4.25,-12.18)) ;
#160777=CARTESIAN_POINT('',(-2.85,4.25,-12.28)) ;
#160778=CARTESIAN_POINT('',(-2.75,4.25,-12.28)) ;
#160779=CARTESIAN_POINT('Origin',(-2.75,4.25,-12.18)) ;
#160780=CARTESIAN_POINT('',(-2.25,4.25,-12.28)) ;
#160781=CARTESIAN_POINT('',(-2.15,4.25,-12.28)) ;
#160782=CARTESIAN_POINT('',(-2.15,4.25,-12.18)) ;
#160783=CARTESIAN_POINT('Origin',(-2.25,4.25,-12.18)) ;
#160784=CARTESIAN_POINT('',(-2.15,4.25,-10.68)) ;
#160785=CARTESIAN_POINT('',(-2.15,4.25,-10.58)) ;
#160786=CARTESIAN_POINT('Origin',(-2.25,4.25,-10.68)) ;
#160787=CARTESIAN_POINT('Origin',(-2.15,4.25,-10.58)) ;
#160788=CARTESIAN_POINT('',(-2.15,4.3,-12.18)) ;
#160789=CARTESIAN_POINT('',(-2.15,4.3,-10.68)) ;
#160790=CARTESIAN_POINT('',(-2.15,4.3,-10.58)) ;
#160791=CARTESIAN_POINT('',(-2.15,4.25,-10.68)) ;
#160792=CARTESIAN_POINT('',(-2.15,4.25,-12.18)) ;
#160793=CARTESIAN_POINT('Origin',(-2.85,4.25,-10.58)) ;
#160794=CARTESIAN_POINT('',(-2.25,4.3,-10.58)) ;
#160795=CARTESIAN_POINT('',(-2.75,4.3,-10.58)) ;
#160796=CARTESIAN_POINT('',(-2.85,4.3,-10.58)) ;
#160797=CARTESIAN_POINT('',(-2.75,4.25,-10.58)) ;
#160798=CARTESIAN_POINT('',(-2.25,4.25,-10.58)) ;
#160799=CARTESIAN_POINT('Origin',(-2.85,4.25,-12.28)) ;
#160800=CARTESIAN_POINT('',(-2.85,4.3,-10.68)) ;
#160801=CARTESIAN_POINT('',(-2.85,4.25,-10.68)) ;
#160802=CARTESIAN_POINT('',(-2.85,4.3,-12.18)) ;
#160803=CARTESIAN_POINT('',(-2.85,4.3,-12.28)) ;
#160804=CARTESIAN_POINT('',(-2.85,4.25,-12.18)) ;
#160805=CARTESIAN_POINT('Origin',(-2.15,4.25,-12.28)) ;
#160806=CARTESIAN_POINT('',(-2.75,4.3,-12.28)) ;
#160807=CARTESIAN_POINT('',(-2.25,4.3,-12.28)) ;
#160808=CARTESIAN_POINT('',(-2.15,4.3,-12.28)) ;
#160809=CARTESIAN_POINT('',(-2.25,4.25,-12.28)) ;
#160810=CARTESIAN_POINT('',(-2.75,4.25,-12.28)) ;
#160811=CARTESIAN_POINT('Origin',(0.,4.25,-15.24)) ;
#160812=CARTESIAN_POINT('',(-2.9,4.25,-16.14)) ;
#160813=CARTESIAN_POINT('',(-2.9,4.25,-14.34)) ;
#160814=CARTESIAN_POINT('',(-2.9,4.25,-15.24)) ;
#160815=CARTESIAN_POINT('',(-2.1,4.25,-14.34)) ;
#160816=CARTESIAN_POINT('',(-1.95156391047391E-16,4.25,-14.34)) ;
#160817=CARTESIAN_POINT('',(-2.1,4.25,-16.14)) ;
#160818=CARTESIAN_POINT('',(-2.1,4.25,-15.24)) ;
#160819=CARTESIAN_POINT('',(-1.95156391047391E-16,4.25,-16.14)) ;
#160820=CARTESIAN_POINT('',(-2.75,4.25,-14.39)) ;
#160821=CARTESIAN_POINT('',(-2.25,4.25,-14.39)) ;
#160822=CARTESIAN_POINT('',(-2.85,4.25,-14.39)) ;
#160823=CARTESIAN_POINT('',(-2.85,4.25,-14.49)) ;
#160824=CARTESIAN_POINT('Origin',(-2.75,4.25,-14.49)) ;
#160825=CARTESIAN_POINT('',(-2.85,4.25,-15.99)) ;
#160826=CARTESIAN_POINT('',(-2.85,4.25,-16.09)) ;
#160827=CARTESIAN_POINT('',(-2.75,4.25,-16.09)) ;
#160828=CARTESIAN_POINT('Origin',(-2.75,4.25,-15.99)) ;
#160829=CARTESIAN_POINT('',(-2.25,4.25,-16.09)) ;
#160830=CARTESIAN_POINT('',(-2.15,4.25,-16.09)) ;
#160831=CARTESIAN_POINT('',(-2.15,4.25,-15.99)) ;
#160832=CARTESIAN_POINT('Origin',(-2.25,4.25,-15.99)) ;
#160833=CARTESIAN_POINT('',(-2.15,4.25,-14.49)) ;
#160834=CARTESIAN_POINT('',(-2.15,4.25,-14.39)) ;
#160835=CARTESIAN_POINT('Origin',(-2.25,4.25,-14.49)) ;
#160836=CARTESIAN_POINT('Origin',(-2.15,4.25,-14.39)) ;
#160837=CARTESIAN_POINT('',(-2.15,4.3,-15.99)) ;
#160838=CARTESIAN_POINT('',(-2.15,4.3,-14.49)) ;
#160839=CARTESIAN_POINT('',(-2.15,4.3,-14.39)) ;
#160840=CARTESIAN_POINT('',(-2.15,4.25,-14.49)) ;
#160841=CARTESIAN_POINT('',(-2.15,4.25,-15.99)) ;
#160842=CARTESIAN_POINT('Origin',(-2.85,4.25,-14.39)) ;
#160843=CARTESIAN_POINT('',(-2.25,4.3,-14.39)) ;
#160844=CARTESIAN_POINT('',(-2.75,4.3,-14.39)) ;
#160845=CARTESIAN_POINT('',(-2.85,4.3,-14.39)) ;
#160846=CARTESIAN_POINT('',(-2.75,4.25,-14.39)) ;
#160847=CARTESIAN_POINT('',(-2.25,4.25,-14.39)) ;
#160848=CARTESIAN_POINT('Origin',(-2.85,4.25,-16.09)) ;
#160849=CARTESIAN_POINT('',(-2.85,4.3,-14.49)) ;
#160850=CARTESIAN_POINT('',(-2.85,4.25,-14.49)) ;
#160851=CARTESIAN_POINT('',(-2.85,4.3,-15.99)) ;
#160852=CARTESIAN_POINT('',(-2.85,4.3,-16.09)) ;
#160853=CARTESIAN_POINT('',(-2.85,4.25,-15.99)) ;
#160854=CARTESIAN_POINT('Origin',(-2.15,4.25,-16.09)) ;
#160855=CARTESIAN_POINT('',(-2.75,4.3,-16.09)) ;
#160856=CARTESIAN_POINT('',(-2.25,4.3,-16.09)) ;
#160857=CARTESIAN_POINT('',(-2.15,4.3,-16.09)) ;
#160858=CARTESIAN_POINT('',(-2.25,4.25,-16.09)) ;
#160859=CARTESIAN_POINT('',(-2.75,4.25,-16.09)) ;
#160860=CARTESIAN_POINT('Origin',(0.,4.25,-19.05)) ;
#160861=CARTESIAN_POINT('',(-2.9,4.25,-19.95)) ;
#160862=CARTESIAN_POINT('',(-2.9,4.25,-18.15)) ;
#160863=CARTESIAN_POINT('',(-2.9,4.25,-19.05)) ;
#160864=CARTESIAN_POINT('',(-2.1,4.25,-18.15)) ;
#160865=CARTESIAN_POINT('',(-1.95156391047391E-16,4.25,-18.15)) ;
#160866=CARTESIAN_POINT('',(-2.1,4.25,-19.95)) ;
#160867=CARTESIAN_POINT('',(-2.1,4.25,-19.05)) ;
#160868=CARTESIAN_POINT('',(-1.95156391047391E-16,4.25,-19.95)) ;
#160869=CARTESIAN_POINT('',(-2.75,4.25,-18.2)) ;
#160870=CARTESIAN_POINT('',(-2.25,4.25,-18.2)) ;
#160871=CARTESIAN_POINT('',(-2.85,4.25,-18.2)) ;
#160872=CARTESIAN_POINT('',(-2.85,4.25,-18.3)) ;
#160873=CARTESIAN_POINT('Origin',(-2.75,4.25,-18.3)) ;
#160874=CARTESIAN_POINT('',(-2.85,4.25,-19.8)) ;
#160875=CARTESIAN_POINT('',(-2.85,4.25,-19.9)) ;
#160876=CARTESIAN_POINT('',(-2.75,4.25,-19.9)) ;
#160877=CARTESIAN_POINT('Origin',(-2.75,4.25,-19.8)) ;
#160878=CARTESIAN_POINT('',(-2.25,4.25,-19.9)) ;
#160879=CARTESIAN_POINT('',(-2.15,4.25,-19.9)) ;
#160880=CARTESIAN_POINT('',(-2.15,4.25,-19.8)) ;
#160881=CARTESIAN_POINT('Origin',(-2.25,4.25,-19.8)) ;
#160882=CARTESIAN_POINT('',(-2.15,4.25,-18.3)) ;
#160883=CARTESIAN_POINT('',(-2.15,4.25,-18.2)) ;
#160884=CARTESIAN_POINT('Origin',(-2.25,4.25,-18.3)) ;
#160885=CARTESIAN_POINT('Origin',(-2.15,4.25,-18.2)) ;
#160886=CARTESIAN_POINT('',(-2.15,4.3,-19.8)) ;
#160887=CARTESIAN_POINT('',(-2.15,4.3,-18.3)) ;
#160888=CARTESIAN_POINT('',(-2.15,4.3,-18.2)) ;
#160889=CARTESIAN_POINT('',(-2.15,4.25,-18.3)) ;
#160890=CARTESIAN_POINT('',(-2.15,4.25,-19.8)) ;
#160891=CARTESIAN_POINT('Origin',(-2.85,4.25,-18.2)) ;
#160892=CARTESIAN_POINT('',(-2.25,4.3,-18.2)) ;
#160893=CARTESIAN_POINT('',(-2.75,4.3,-18.2)) ;
#160894=CARTESIAN_POINT('',(-2.85,4.3,-18.2)) ;
#160895=CARTESIAN_POINT('',(-2.75,4.25,-18.2)) ;
#160896=CARTESIAN_POINT('',(-2.25,4.25,-18.2)) ;
#160897=CARTESIAN_POINT('Origin',(-2.85,4.25,-19.9)) ;
#160898=CARTESIAN_POINT('',(-2.85,4.3,-18.3)) ;
#160899=CARTESIAN_POINT('',(-2.85,4.25,-18.3)) ;
#160900=CARTESIAN_POINT('',(-2.85,4.3,-19.8)) ;
#160901=CARTESIAN_POINT('',(-2.85,4.3,-19.9)) ;
#160902=CARTESIAN_POINT('',(-2.85,4.25,-19.8)) ;
#160903=CARTESIAN_POINT('Origin',(-2.15,4.25,-19.9)) ;
#160904=CARTESIAN_POINT('',(-2.75,4.3,-19.9)) ;
#160905=CARTESIAN_POINT('',(-2.25,4.3,-19.9)) ;
#160906=CARTESIAN_POINT('',(-2.15,4.3,-19.9)) ;
#160907=CARTESIAN_POINT('',(-2.25,4.25,-19.9)) ;
#160908=CARTESIAN_POINT('',(-2.75,4.25,-19.9)) ;
#160909=CARTESIAN_POINT('Origin',(0.,4.25,-22.86)) ;
#160910=CARTESIAN_POINT('',(-2.9,4.25,-23.76)) ;
#160911=CARTESIAN_POINT('',(-2.9,4.25,-21.96)) ;
#160912=CARTESIAN_POINT('',(-2.9,4.25,-22.86)) ;
#160913=CARTESIAN_POINT('',(-2.1,4.25,-21.96)) ;
#160914=CARTESIAN_POINT('',(-1.95156391047391E-16,4.25,-21.96)) ;
#160915=CARTESIAN_POINT('',(-2.1,4.25,-23.76)) ;
#160916=CARTESIAN_POINT('',(-2.1,4.25,-22.86)) ;
#160917=CARTESIAN_POINT('',(-1.95156391047391E-16,4.25,-23.76)) ;
#160918=CARTESIAN_POINT('',(-2.75,4.25,-22.01)) ;
#160919=CARTESIAN_POINT('',(-2.25,4.25,-22.01)) ;
#160920=CARTESIAN_POINT('',(-2.85,4.25,-22.01)) ;
#160921=CARTESIAN_POINT('',(-2.85,4.25,-22.11)) ;
#160922=CARTESIAN_POINT('Origin',(-2.75,4.25,-22.11)) ;
#160923=CARTESIAN_POINT('',(-2.85,4.25,-23.61)) ;
#160924=CARTESIAN_POINT('',(-2.85,4.25,-23.71)) ;
#160925=CARTESIAN_POINT('',(-2.75,4.25,-23.71)) ;
#160926=CARTESIAN_POINT('Origin',(-2.75,4.25,-23.61)) ;
#160927=CARTESIAN_POINT('',(-2.25,4.25,-23.71)) ;
#160928=CARTESIAN_POINT('',(-2.15,4.25,-23.71)) ;
#160929=CARTESIAN_POINT('',(-2.15,4.25,-23.61)) ;
#160930=CARTESIAN_POINT('Origin',(-2.25,4.25,-23.61)) ;
#160931=CARTESIAN_POINT('',(-2.15,4.25,-22.11)) ;
#160932=CARTESIAN_POINT('',(-2.15,4.25,-22.01)) ;
#160933=CARTESIAN_POINT('Origin',(-2.25,4.25,-22.11)) ;
#160934=CARTESIAN_POINT('Origin',(-2.15,4.25,-22.01)) ;
#160935=CARTESIAN_POINT('',(-2.15,4.3,-23.61)) ;
#160936=CARTESIAN_POINT('',(-2.15,4.3,-22.11)) ;
#160937=CARTESIAN_POINT('',(-2.15,4.3,-22.01)) ;
#160938=CARTESIAN_POINT('',(-2.15,4.25,-22.11)) ;
#160939=CARTESIAN_POINT('',(-2.15,4.25,-23.61)) ;
#160940=CARTESIAN_POINT('Origin',(-2.85,4.25,-22.01)) ;
#160941=CARTESIAN_POINT('',(-2.25,4.3,-22.01)) ;
#160942=CARTESIAN_POINT('',(-2.75,4.3,-22.01)) ;
#160943=CARTESIAN_POINT('',(-2.85,4.3,-22.01)) ;
#160944=CARTESIAN_POINT('',(-2.75,4.25,-22.01)) ;
#160945=CARTESIAN_POINT('',(-2.25,4.25,-22.01)) ;
#160946=CARTESIAN_POINT('Origin',(-2.85,4.25,-23.71)) ;
#160947=CARTESIAN_POINT('',(-2.85,4.3,-22.11)) ;
#160948=CARTESIAN_POINT('',(-2.85,4.25,-22.11)) ;
#160949=CARTESIAN_POINT('',(-2.85,4.3,-23.61)) ;
#160950=CARTESIAN_POINT('',(-2.85,4.3,-23.71)) ;
#160951=CARTESIAN_POINT('',(-2.85,4.25,-23.61)) ;
#160952=CARTESIAN_POINT('Origin',(-2.15,4.25,-23.71)) ;
#160953=CARTESIAN_POINT('',(-2.75,4.3,-23.71)) ;
#160954=CARTESIAN_POINT('',(-2.25,4.3,-23.71)) ;
#160955=CARTESIAN_POINT('',(-2.15,4.3,-23.71)) ;
#160956=CARTESIAN_POINT('',(-2.25,4.25,-23.71)) ;
#160957=CARTESIAN_POINT('',(-2.75,4.25,-23.71)) ;
#160958=CARTESIAN_POINT('Origin',(0.,4.25,-26.67)) ;
#160959=CARTESIAN_POINT('',(-2.9,4.25,-27.57)) ;
#160960=CARTESIAN_POINT('',(-2.9,4.25,-25.77)) ;
#160961=CARTESIAN_POINT('',(-2.9,4.25,-26.67)) ;
#160962=CARTESIAN_POINT('',(-2.1,4.25,-25.77)) ;
#160963=CARTESIAN_POINT('',(-1.95156391047391E-16,4.25,-25.77)) ;
#160964=CARTESIAN_POINT('',(-2.1,4.25,-27.57)) ;
#160965=CARTESIAN_POINT('',(-2.1,4.25,-26.67)) ;
#160966=CARTESIAN_POINT('',(-1.95156391047391E-16,4.25,-27.57)) ;
#160967=CARTESIAN_POINT('',(-2.75,4.25,-25.82)) ;
#160968=CARTESIAN_POINT('',(-2.25,4.25,-25.82)) ;
#160969=CARTESIAN_POINT('',(-2.85,4.25,-25.82)) ;
#160970=CARTESIAN_POINT('',(-2.85,4.25,-25.92)) ;
#160971=CARTESIAN_POINT('Origin',(-2.75,4.25,-25.92)) ;
#160972=CARTESIAN_POINT('',(-2.85,4.25,-27.42)) ;
#160973=CARTESIAN_POINT('',(-2.85,4.25,-27.52)) ;
#160974=CARTESIAN_POINT('',(-2.75,4.25,-27.52)) ;
#160975=CARTESIAN_POINT('Origin',(-2.75,4.25,-27.42)) ;
#160976=CARTESIAN_POINT('',(-2.25,4.25,-27.52)) ;
#160977=CARTESIAN_POINT('',(-2.15,4.25,-27.52)) ;
#160978=CARTESIAN_POINT('',(-2.15,4.25,-27.42)) ;
#160979=CARTESIAN_POINT('Origin',(-2.25,4.25,-27.42)) ;
#160980=CARTESIAN_POINT('',(-2.15,4.25,-25.92)) ;
#160981=CARTESIAN_POINT('',(-2.15,4.25,-25.82)) ;
#160982=CARTESIAN_POINT('Origin',(-2.25,4.25,-25.92)) ;
#160983=CARTESIAN_POINT('Origin',(-2.15,4.25,-25.82)) ;
#160984=CARTESIAN_POINT('',(-2.15,4.3,-27.42)) ;
#160985=CARTESIAN_POINT('',(-2.15,4.3,-25.92)) ;
#160986=CARTESIAN_POINT('',(-2.15,4.3,-25.82)) ;
#160987=CARTESIAN_POINT('',(-2.15,4.25,-25.92)) ;
#160988=CARTESIAN_POINT('',(-2.15,4.25,-27.42)) ;
#160989=CARTESIAN_POINT('Origin',(-2.85,4.25,-25.82)) ;
#160990=CARTESIAN_POINT('',(-2.25,4.3,-25.82)) ;
#160991=CARTESIAN_POINT('',(-2.75,4.3,-25.82)) ;
#160992=CARTESIAN_POINT('',(-2.85,4.3,-25.82)) ;
#160993=CARTESIAN_POINT('',(-2.75,4.25,-25.82)) ;
#160994=CARTESIAN_POINT('',(-2.25,4.25,-25.82)) ;
#160995=CARTESIAN_POINT('Origin',(-2.85,4.25,-27.52)) ;
#160996=CARTESIAN_POINT('',(-2.85,4.3,-25.92)) ;
#160997=CARTESIAN_POINT('',(-2.85,4.25,-25.92)) ;
#160998=CARTESIAN_POINT('',(-2.85,4.3,-27.42)) ;
#160999=CARTESIAN_POINT('',(-2.85,4.3,-27.52)) ;
#161000=CARTESIAN_POINT('',(-2.85,4.25,-27.42)) ;
#161001=CARTESIAN_POINT('Origin',(-2.15,4.25,-27.52)) ;
#161002=CARTESIAN_POINT('',(-2.75,4.3,-27.52)) ;
#161003=CARTESIAN_POINT('',(-2.25,4.3,-27.52)) ;
#161004=CARTESIAN_POINT('',(-2.15,4.3,-27.52)) ;
#161005=CARTESIAN_POINT('',(-2.25,4.25,-27.52)) ;
#161006=CARTESIAN_POINT('',(-2.75,4.25,-27.52)) ;
#161007=CARTESIAN_POINT('Origin',(0.,4.25,-30.48)) ;
#161008=CARTESIAN_POINT('',(-2.9,4.25,-31.38)) ;
#161009=CARTESIAN_POINT('',(-2.9,4.25,-29.58)) ;
#161010=CARTESIAN_POINT('',(-2.9,4.25,-30.48)) ;
#161011=CARTESIAN_POINT('',(-2.1,4.25,-29.58)) ;
#161012=CARTESIAN_POINT('',(-1.95156391047391E-16,4.25,-29.58)) ;
#161013=CARTESIAN_POINT('',(-2.1,4.25,-31.38)) ;
#161014=CARTESIAN_POINT('',(-2.1,4.25,-30.48)) ;
#161015=CARTESIAN_POINT('',(-1.95156391047391E-16,4.25,-31.38)) ;
#161016=CARTESIAN_POINT('',(-2.75,4.25,-29.63)) ;
#161017=CARTESIAN_POINT('',(-2.25,4.25,-29.63)) ;
#161018=CARTESIAN_POINT('',(-2.85,4.25,-29.63)) ;
#161019=CARTESIAN_POINT('',(-2.85,4.25,-29.73)) ;
#161020=CARTESIAN_POINT('Origin',(-2.75,4.25,-29.73)) ;
#161021=CARTESIAN_POINT('',(-2.85,4.25,-31.23)) ;
#161022=CARTESIAN_POINT('',(-2.85,4.25,-31.33)) ;
#161023=CARTESIAN_POINT('',(-2.75,4.25,-31.33)) ;
#161024=CARTESIAN_POINT('Origin',(-2.75,4.25,-31.23)) ;
#161025=CARTESIAN_POINT('',(-2.25,4.25,-31.33)) ;
#161026=CARTESIAN_POINT('',(-2.15,4.25,-31.33)) ;
#161027=CARTESIAN_POINT('',(-2.15,4.25,-31.23)) ;
#161028=CARTESIAN_POINT('Origin',(-2.25,4.25,-31.23)) ;
#161029=CARTESIAN_POINT('',(-2.15,4.25,-29.73)) ;
#161030=CARTESIAN_POINT('',(-2.15,4.25,-29.63)) ;
#161031=CARTESIAN_POINT('Origin',(-2.25,4.25,-29.73)) ;
#161032=CARTESIAN_POINT('Origin',(-2.15,4.25,-29.63)) ;
#161033=CARTESIAN_POINT('',(-2.15,4.3,-31.23)) ;
#161034=CARTESIAN_POINT('',(-2.15,4.3,-29.73)) ;
#161035=CARTESIAN_POINT('',(-2.15,4.3,-29.63)) ;
#161036=CARTESIAN_POINT('',(-2.15,4.25,-29.73)) ;
#161037=CARTESIAN_POINT('',(-2.15,4.25,-31.23)) ;
#161038=CARTESIAN_POINT('Origin',(-2.85,4.25,-29.63)) ;
#161039=CARTESIAN_POINT('',(-2.25,4.3,-29.63)) ;
#161040=CARTESIAN_POINT('',(-2.75,4.3,-29.63)) ;
#161041=CARTESIAN_POINT('',(-2.85,4.3,-29.63)) ;
#161042=CARTESIAN_POINT('',(-2.75,4.25,-29.63)) ;
#161043=CARTESIAN_POINT('',(-2.25,4.25,-29.63)) ;
#161044=CARTESIAN_POINT('Origin',(-2.85,4.25,-31.33)) ;
#161045=CARTESIAN_POINT('',(-2.85,4.3,-29.73)) ;
#161046=CARTESIAN_POINT('',(-2.85,4.25,-29.73)) ;
#161047=CARTESIAN_POINT('',(-2.85,4.3,-31.23)) ;
#161048=CARTESIAN_POINT('',(-2.85,4.3,-31.33)) ;
#161049=CARTESIAN_POINT('',(-2.85,4.25,-31.23)) ;
#161050=CARTESIAN_POINT('Origin',(-2.15,4.25,-31.33)) ;
#161051=CARTESIAN_POINT('',(-2.75,4.3,-31.33)) ;
#161052=CARTESIAN_POINT('',(-2.25,4.3,-31.33)) ;
#161053=CARTESIAN_POINT('',(-2.15,4.3,-31.33)) ;
#161054=CARTESIAN_POINT('',(-2.25,4.25,-31.33)) ;
#161055=CARTESIAN_POINT('',(-2.75,4.25,-31.33)) ;
#161056=CARTESIAN_POINT('Origin',(0.,4.25,-34.29)) ;
#161057=CARTESIAN_POINT('',(-2.9,4.25,-35.19)) ;
#161058=CARTESIAN_POINT('',(-2.9,4.25,-33.39)) ;
#161059=CARTESIAN_POINT('',(-2.9,4.25,-34.29)) ;
#161060=CARTESIAN_POINT('',(-2.1,4.25,-33.39)) ;
#161061=CARTESIAN_POINT('',(-1.95156391047391E-16,4.25,-33.39)) ;
#161062=CARTESIAN_POINT('',(-2.1,4.25,-35.19)) ;
#161063=CARTESIAN_POINT('',(-2.1,4.25,-34.29)) ;
#161064=CARTESIAN_POINT('',(-1.95156391047391E-16,4.25,-35.19)) ;
#161065=CARTESIAN_POINT('',(-2.75,4.25,-33.44)) ;
#161066=CARTESIAN_POINT('',(-2.25,4.25,-33.44)) ;
#161067=CARTESIAN_POINT('',(-2.85,4.25,-33.44)) ;
#161068=CARTESIAN_POINT('',(-2.85,4.25,-33.54)) ;
#161069=CARTESIAN_POINT('Origin',(-2.75,4.25,-33.54)) ;
#161070=CARTESIAN_POINT('',(-2.85,4.25,-35.04)) ;
#161071=CARTESIAN_POINT('',(-2.85,4.25,-35.14)) ;
#161072=CARTESIAN_POINT('',(-2.75,4.25,-35.14)) ;
#161073=CARTESIAN_POINT('Origin',(-2.75,4.25,-35.04)) ;
#161074=CARTESIAN_POINT('',(-2.25,4.25,-35.14)) ;
#161075=CARTESIAN_POINT('',(-2.15,4.25,-35.14)) ;
#161076=CARTESIAN_POINT('',(-2.15,4.25,-35.04)) ;
#161077=CARTESIAN_POINT('Origin',(-2.25,4.25,-35.04)) ;
#161078=CARTESIAN_POINT('',(-2.15,4.25,-33.54)) ;
#161079=CARTESIAN_POINT('',(-2.15,4.25,-33.44)) ;
#161080=CARTESIAN_POINT('Origin',(-2.25,4.25,-33.54)) ;
#161081=CARTESIAN_POINT('Origin',(-2.15,4.25,-33.44)) ;
#161082=CARTESIAN_POINT('',(-2.15,4.3,-35.04)) ;
#161083=CARTESIAN_POINT('',(-2.15,4.3,-33.54)) ;
#161084=CARTESIAN_POINT('',(-2.15,4.3,-33.44)) ;
#161085=CARTESIAN_POINT('',(-2.15,4.25,-33.54)) ;
#161086=CARTESIAN_POINT('',(-2.15,4.25,-35.04)) ;
#161087=CARTESIAN_POINT('Origin',(-2.85,4.25,-33.44)) ;
#161088=CARTESIAN_POINT('',(-2.25,4.3,-33.44)) ;
#161089=CARTESIAN_POINT('',(-2.75,4.3,-33.44)) ;
#161090=CARTESIAN_POINT('',(-2.85,4.3,-33.44)) ;
#161091=CARTESIAN_POINT('',(-2.75,4.25,-33.44)) ;
#161092=CARTESIAN_POINT('',(-2.25,4.25,-33.44)) ;
#161093=CARTESIAN_POINT('Origin',(-2.85,4.25,-35.14)) ;
#161094=CARTESIAN_POINT('',(-2.85,4.3,-33.54)) ;
#161095=CARTESIAN_POINT('',(-2.85,4.25,-33.54)) ;
#161096=CARTESIAN_POINT('',(-2.85,4.3,-35.04)) ;
#161097=CARTESIAN_POINT('',(-2.85,4.3,-35.14)) ;
#161098=CARTESIAN_POINT('',(-2.85,4.25,-35.04)) ;
#161099=CARTESIAN_POINT('Origin',(-2.15,4.25,-35.14)) ;
#161100=CARTESIAN_POINT('',(-2.75,4.3,-35.14)) ;
#161101=CARTESIAN_POINT('',(-2.25,4.3,-35.14)) ;
#161102=CARTESIAN_POINT('',(-2.15,4.3,-35.14)) ;
#161103=CARTESIAN_POINT('',(-2.25,4.25,-35.14)) ;
#161104=CARTESIAN_POINT('',(-2.75,4.25,-35.14)) ;
#161105=CARTESIAN_POINT('Origin',(-1.97127667724637E-17,4.4,-3.81)) ;
#161106=CARTESIAN_POINT('',(-2.25,4.4,-4.56)) ;
#161107=CARTESIAN_POINT('',(-2.75,4.4,-4.56)) ;
#161108=CARTESIAN_POINT('',(-1.97127667724637E-17,4.4,-4.56)) ;
#161109=CARTESIAN_POINT('',(-2.75,4.4,-3.06)) ;
#161110=CARTESIAN_POINT('',(-2.75,4.4,-3.81)) ;
#161111=CARTESIAN_POINT('',(-2.25,4.4,-3.06)) ;
#161112=CARTESIAN_POINT('',(-1.97127667724637E-17,4.4,-3.06)) ;
#161113=CARTESIAN_POINT('',(-2.25,4.4,-3.81)) ;
#161114=CARTESIAN_POINT('Origin',(-1.97127667724637E-17,4.4,-7.62)) ;
#161115=CARTESIAN_POINT('',(-2.25,4.4,-8.37)) ;
#161116=CARTESIAN_POINT('',(-2.75,4.4,-8.37)) ;
#161117=CARTESIAN_POINT('',(-1.97127667724637E-17,4.4,-8.37)) ;
#161118=CARTESIAN_POINT('',(-2.75,4.4,-6.87)) ;
#161119=CARTESIAN_POINT('',(-2.75,4.4,-7.62)) ;
#161120=CARTESIAN_POINT('',(-2.25,4.4,-6.87)) ;
#161121=CARTESIAN_POINT('',(-1.97127667724637E-17,4.4,-6.87)) ;
#161122=CARTESIAN_POINT('',(-2.25,4.4,-7.62)) ;
#161123=CARTESIAN_POINT('Origin',(-1.97127667724637E-17,4.4,-11.43)) ;
#161124=CARTESIAN_POINT('',(-2.25,4.4,-12.18)) ;
#161125=CARTESIAN_POINT('',(-2.75,4.4,-12.18)) ;
#161126=CARTESIAN_POINT('',(-1.97127667724637E-17,4.4,-12.18)) ;
#161127=CARTESIAN_POINT('',(-2.75,4.4,-10.68)) ;
#161128=CARTESIAN_POINT('',(-2.75,4.4,-11.43)) ;
#161129=CARTESIAN_POINT('',(-2.25,4.4,-10.68)) ;
#161130=CARTESIAN_POINT('',(-1.97127667724637E-17,4.4,-10.68)) ;
#161131=CARTESIAN_POINT('',(-2.25,4.4,-11.43)) ;
#161132=CARTESIAN_POINT('Origin',(-1.97127667724637E-17,4.4,-15.24)) ;
#161133=CARTESIAN_POINT('',(-2.25,4.4,-15.99)) ;
#161134=CARTESIAN_POINT('',(-2.75,4.4,-15.99)) ;
#161135=CARTESIAN_POINT('',(-1.97127667724637E-17,4.4,-15.99)) ;
#161136=CARTESIAN_POINT('',(-2.75,4.4,-14.49)) ;
#161137=CARTESIAN_POINT('',(-2.75,4.4,-15.24)) ;
#161138=CARTESIAN_POINT('',(-2.25,4.4,-14.49)) ;
#161139=CARTESIAN_POINT('',(-1.97127667724637E-17,4.4,-14.49)) ;
#161140=CARTESIAN_POINT('',(-2.25,4.4,-15.24)) ;
#161141=CARTESIAN_POINT('Origin',(-1.97127667724637E-17,4.4,-19.05)) ;
#161142=CARTESIAN_POINT('',(-2.25,4.4,-19.8)) ;
#161143=CARTESIAN_POINT('',(-2.75,4.4,-19.8)) ;
#161144=CARTESIAN_POINT('',(-1.97127667724637E-17,4.4,-19.8)) ;
#161145=CARTESIAN_POINT('',(-2.75,4.4,-18.3)) ;
#161146=CARTESIAN_POINT('',(-2.75,4.4,-19.05)) ;
#161147=CARTESIAN_POINT('',(-2.25,4.4,-18.3)) ;
#161148=CARTESIAN_POINT('',(-1.97127667724637E-17,4.4,-18.3)) ;
#161149=CARTESIAN_POINT('',(-2.25,4.4,-19.05)) ;
#161150=CARTESIAN_POINT('Origin',(-1.97127667724637E-17,4.4,-22.86)) ;
#161151=CARTESIAN_POINT('',(-2.25,4.4,-23.61)) ;
#161152=CARTESIAN_POINT('',(-2.75,4.4,-23.61)) ;
#161153=CARTESIAN_POINT('',(-1.97127667724637E-17,4.4,-23.61)) ;
#161154=CARTESIAN_POINT('',(-2.75,4.4,-22.11)) ;
#161155=CARTESIAN_POINT('',(-2.75,4.4,-22.86)) ;
#161156=CARTESIAN_POINT('',(-2.25,4.4,-22.11)) ;
#161157=CARTESIAN_POINT('',(-1.97127667724637E-17,4.4,-22.11)) ;
#161158=CARTESIAN_POINT('',(-2.25,4.4,-22.86)) ;
#161159=CARTESIAN_POINT('Origin',(-1.97127667724637E-17,4.4,-26.67)) ;
#161160=CARTESIAN_POINT('',(-2.25,4.4,-27.42)) ;
#161161=CARTESIAN_POINT('',(-2.75,4.4,-27.42)) ;
#161162=CARTESIAN_POINT('',(-1.97127667724637E-17,4.4,-27.42)) ;
#161163=CARTESIAN_POINT('',(-2.75,4.4,-25.92)) ;
#161164=CARTESIAN_POINT('',(-2.75,4.4,-26.67)) ;
#161165=CARTESIAN_POINT('',(-2.25,4.4,-25.92)) ;
#161166=CARTESIAN_POINT('',(-1.97127667724637E-17,4.4,-25.92)) ;
#161167=CARTESIAN_POINT('',(-2.25,4.4,-26.67)) ;
#161168=CARTESIAN_POINT('Origin',(-1.97127667724637E-17,4.4,-30.48)) ;
#161169=CARTESIAN_POINT('',(-2.25,4.4,-31.23)) ;
#161170=CARTESIAN_POINT('',(-2.75,4.4,-31.23)) ;
#161171=CARTESIAN_POINT('',(-1.97127667724637E-17,4.4,-31.23)) ;
#161172=CARTESIAN_POINT('',(-2.75,4.4,-29.73)) ;
#161173=CARTESIAN_POINT('',(-2.75,4.4,-30.48)) ;
#161174=CARTESIAN_POINT('',(-2.25,4.4,-29.73)) ;
#161175=CARTESIAN_POINT('',(-1.97127667724637E-17,4.4,-29.73)) ;
#161176=CARTESIAN_POINT('',(-2.25,4.4,-30.48)) ;
#161177=CARTESIAN_POINT('Origin',(-1.97127667724637E-17,4.4,-34.29)) ;
#161178=CARTESIAN_POINT('',(-2.25,4.4,-35.04)) ;
#161179=CARTESIAN_POINT('',(-2.75,4.4,-35.04)) ;
#161180=CARTESIAN_POINT('',(-1.97127667724637E-17,4.4,-35.04)) ;
#161181=CARTESIAN_POINT('',(-2.75,4.4,-33.54)) ;
#161182=CARTESIAN_POINT('',(-2.75,4.4,-34.29)) ;
#161183=CARTESIAN_POINT('',(-2.25,4.4,-33.54)) ;
#161184=CARTESIAN_POINT('',(-1.97127667724637E-17,4.4,-33.54)) ;
#161185=CARTESIAN_POINT('',(-2.25,4.4,-34.29)) ;
#161186=CARTESIAN_POINT('Origin',(-7.29372370581158E-16,3.55,-34.29)) ;
#161187=CARTESIAN_POINT('',(-0.183301359729408,3.55,-32.772963213524)) ;
#161188=CARTESIAN_POINT('Origin',(-7.29372370581158E-16,3.55,-30.48)) ;
#161189=CARTESIAN_POINT('',(-0.183301359729408,3.55,-28.962963213524)) ;
#161190=CARTESIAN_POINT('Origin',(-7.29372370581158E-16,3.55,-26.67)) ;
#161191=CARTESIAN_POINT('',(-0.183301359729408,3.55,-25.152963213524)) ;
#161192=CARTESIAN_POINT('Origin',(-7.29372370581158E-16,3.55,-22.86)) ;
#161193=CARTESIAN_POINT('',(-0.183301359729408,3.55,-21.342963213524)) ;
#161194=CARTESIAN_POINT('Origin',(-7.29372370581158E-16,3.55,-19.05)) ;
#161195=CARTESIAN_POINT('',(-0.183301359729408,3.55,-17.532963213524)) ;
#161196=CARTESIAN_POINT('Origin',(-7.29372370581158E-16,3.55,-15.24)) ;
#161197=CARTESIAN_POINT('',(-0.183301359729408,3.55,-13.722963213524)) ;
#161198=CARTESIAN_POINT('Origin',(-7.29372370581158E-16,3.55,-11.43)) ;
#161199=CARTESIAN_POINT('',(-0.183301359729408,3.55,-9.91296321352402)) ;
#161200=CARTESIAN_POINT('Origin',(-7.29372370581158E-16,3.55,-7.62)) ;
#161201=CARTESIAN_POINT('',(-0.183301359729408,3.55,-6.10296321352403)) ;
#161202=CARTESIAN_POINT('Origin',(-7.29372370581158E-16,3.55,-3.81)) ;
#161203=CARTESIAN_POINT('',(-0.183301359729408,3.55,-2.29296321352403)) ;
#161204=CARTESIAN_POINT('Origin',(-0.273932138433073,3.05,-2.3352250396981)) ;
#161205=CARTESIAN_POINT('',(0.953662978710562,3.45,-4.96781126399638)) ;
#161206=CARTESIAN_POINT('',(-0.273932138433073,3.15,-2.3352250396981)) ;
#161207=CARTESIAN_POINT('Origin',(-0.953662978710561,3.05,-2.65218873600362)) ;
#161208=CARTESIAN_POINT('',(-0.953662978710561,3.15,-2.65218873600362)) ;
#161209=CARTESIAN_POINT('',(-0.953662978710562,3.45,-2.65218873600362)) ;
#161210=CARTESIAN_POINT('Origin',(-7.95081593156037E-16,3.05,-3.81)) ;
#161211=CARTESIAN_POINT('',(0.249234641435079,3.05,-3.69377997802131)) ;
#161212=CARTESIAN_POINT('',(-0.249234641435079,3.05,-3.92622002197869)) ;
#161213=CARTESIAN_POINT('Origin',(-0.273932138433073,3.05,-6.1452250396981)) ;
#161214=CARTESIAN_POINT('',(0.953662978710562,3.45,-8.77781126399638)) ;
#161215=CARTESIAN_POINT('',(-0.273932138433073,3.15,-6.1452250396981)) ;
#161216=CARTESIAN_POINT('Origin',(-0.953662978710561,3.05,-6.46218873600362)) ;
#161217=CARTESIAN_POINT('',(-0.953662978710561,3.15,-6.46218873600362)) ;
#161218=CARTESIAN_POINT('',(-0.953662978710562,3.45,-6.46218873600362)) ;
#161219=CARTESIAN_POINT('Origin',(-7.95081593156037E-16,3.05,-7.62)) ;
#161220=CARTESIAN_POINT('',(0.249234641435079,3.05,-7.50377997802131)) ;
#161221=CARTESIAN_POINT('',(-0.249234641435079,3.05,-7.73622002197869)) ;
#161222=CARTESIAN_POINT('Origin',(-0.273932138433073,3.05,-9.9552250396981)) ;
#161223=CARTESIAN_POINT('',(0.953662978710562,3.45,-12.5878112639964)) ;
#161224=CARTESIAN_POINT('',(-0.273932138433073,3.15,-9.9552250396981)) ;
#161225=CARTESIAN_POINT('Origin',(-0.953662978710561,3.05,-10.2721887360036)) ;
#161226=CARTESIAN_POINT('',(-0.953662978710561,3.15,-10.2721887360036)) ;
#161227=CARTESIAN_POINT('',(-0.953662978710561,3.45,-10.2721887360036)) ;
#161228=CARTESIAN_POINT('Origin',(-7.95081593156037E-16,3.05,-11.43)) ;
#161229=CARTESIAN_POINT('',(0.249234641435079,3.05,-11.3137799780213)) ;
#161230=CARTESIAN_POINT('',(-0.249234641435079,3.05,-11.5462200219787)) ;
#161231=CARTESIAN_POINT('Origin',(-0.273932138433073,3.05,-13.7652250396981)) ;
#161232=CARTESIAN_POINT('',(0.953662978710563,3.45,-16.3978112639964)) ;
#161233=CARTESIAN_POINT('',(-0.273932138433073,3.15,-13.7652250396981)) ;
#161234=CARTESIAN_POINT('Origin',(-0.953662978710561,3.05,-14.0821887360036)) ;
#161235=CARTESIAN_POINT('',(-0.953662978710561,3.15,-14.0821887360036)) ;
#161236=CARTESIAN_POINT('',(-0.953662978710561,3.45,-14.0821887360036)) ;
#161237=CARTESIAN_POINT('Origin',(-7.95081593156037E-16,3.05,-15.24)) ;
#161238=CARTESIAN_POINT('',(0.249234641435079,3.05,-15.1237799780213)) ;
#161239=CARTESIAN_POINT('',(-0.249234641435079,3.05,-15.3562200219787)) ;
#161240=CARTESIAN_POINT('Origin',(-0.273932138433073,3.05,-17.5752250396981)) ;
#161241=CARTESIAN_POINT('',(0.953662978710563,3.45,-20.2078112639964)) ;
#161242=CARTESIAN_POINT('',(-0.273932138433073,3.15,-17.5752250396981)) ;
#161243=CARTESIAN_POINT('Origin',(-0.953662978710561,3.05,-17.8921887360036)) ;
#161244=CARTESIAN_POINT('',(-0.953662978710561,3.15,-17.8921887360036)) ;
#161245=CARTESIAN_POINT('',(-0.953662978710561,3.45,-17.8921887360036)) ;
#161246=CARTESIAN_POINT('Origin',(-7.95081593156037E-16,3.05,-19.05)) ;
#161247=CARTESIAN_POINT('',(0.249234641435081,3.05,-18.9337799780213)) ;
#161248=CARTESIAN_POINT('',(-0.249234641435079,3.05,-19.1662200219787)) ;
#161249=CARTESIAN_POINT('Origin',(-0.273932138433073,3.05,-21.3852250396981)) ;
#161250=CARTESIAN_POINT('',(0.953662978710563,3.45,-24.0178112639964)) ;
#161251=CARTESIAN_POINT('',(-0.273932138433073,3.15,-21.3852250396981)) ;
#161252=CARTESIAN_POINT('Origin',(-0.953662978710561,3.05,-21.7021887360036)) ;
#161253=CARTESIAN_POINT('',(-0.953662978710561,3.15,-21.7021887360036)) ;
#161254=CARTESIAN_POINT('',(-0.953662978710561,3.45,-21.7021887360036)) ;
#161255=CARTESIAN_POINT('Origin',(-7.95081593156037E-16,3.05,-22.86)) ;
#161256=CARTESIAN_POINT('',(0.249234641435081,3.05,-22.7437799780213)) ;
#161257=CARTESIAN_POINT('',(-0.249234641435079,3.05,-22.9762200219787)) ;
#161258=CARTESIAN_POINT('Origin',(-0.273932138433073,3.05,-25.1952250396981)) ;
#161259=CARTESIAN_POINT('',(0.953662978710563,3.45,-27.8278112639964)) ;
#161260=CARTESIAN_POINT('',(-0.273932138433073,3.15,-25.1952250396981)) ;
#161261=CARTESIAN_POINT('Origin',(-0.953662978710561,3.05,-25.5121887360036)) ;
#161262=CARTESIAN_POINT('',(-0.953662978710561,3.15,-25.5121887360036)) ;
#161263=CARTESIAN_POINT('',(-0.953662978710561,3.45,-25.5121887360036)) ;
#161264=CARTESIAN_POINT('Origin',(-7.95081593156037E-16,3.05,-26.67)) ;
#161265=CARTESIAN_POINT('',(0.249234641435081,3.05,-26.5537799780213)) ;
#161266=CARTESIAN_POINT('',(-0.249234641435079,3.05,-26.7862200219787)) ;
#161267=CARTESIAN_POINT('Origin',(-0.273932138433073,3.05,-29.0052250396981)) ;
#161268=CARTESIAN_POINT('',(0.953662978710563,3.45,-31.6378112639964)) ;
#161269=CARTESIAN_POINT('',(-0.273932138433073,3.15,-29.0052250396981)) ;
#161270=CARTESIAN_POINT('Origin',(-0.953662978710561,3.05,-29.3221887360036)) ;
#161271=CARTESIAN_POINT('',(-0.953662978710561,3.15,-29.3221887360036)) ;
#161272=CARTESIAN_POINT('',(-0.953662978710561,3.45,-29.3221887360036)) ;
#161273=CARTESIAN_POINT('Origin',(-7.95081593156037E-16,3.05,-30.48)) ;
#161274=CARTESIAN_POINT('',(0.249234641435081,3.05,-30.3637799780213)) ;
#161275=CARTESIAN_POINT('',(-0.249234641435079,3.05,-30.5962200219787)) ;
#161276=CARTESIAN_POINT('Origin',(-0.273932138433073,3.05,-32.8152250396981)) ;
#161277=CARTESIAN_POINT('',(0.953662978710563,3.45,-35.4478112639964)) ;
#161278=CARTESIAN_POINT('',(-0.273932138433073,3.15,-32.8152250396981)) ;
#161279=CARTESIAN_POINT('Origin',(-0.953662978710561,3.05,-33.1321887360036)) ;
#161280=CARTESIAN_POINT('',(-0.953662978710561,3.15,-33.1321887360036)) ;
#161281=CARTESIAN_POINT('',(-0.953662978710561,3.45,-33.1321887360036)) ;
#161282=CARTESIAN_POINT('Origin',(-7.95081593156037E-16,3.05,-34.29)) ;
#161283=CARTESIAN_POINT('',(0.24923464143508,3.05,-34.1737799780213)) ;
#161284=CARTESIAN_POINT('',(-0.249234641435079,3.05,-34.4062200219787)) ;
#161285=CARTESIAN_POINT('Origin',(9.6,3.,-4.21)) ;
#161286=CARTESIAN_POINT('',(9.7,2.9,-4.21)) ;
#161287=CARTESIAN_POINT('',(9.7,2.1,-4.21)) ;
#161288=CARTESIAN_POINT('',(9.7,3.,-4.21)) ;
#161289=CARTESIAN_POINT('',(9.6,2.1,-4.31)) ;
#161290=CARTESIAN_POINT('Origin',(9.6,2.1,-4.21)) ;
#161291=CARTESIAN_POINT('',(9.6,2.9,-4.31)) ;
#161292=CARTESIAN_POINT('',(9.6,3.,-4.31)) ;
#161293=CARTESIAN_POINT('Origin',(9.6,2.9,-4.21)) ;
#161294=CARTESIAN_POINT('Origin',(7.8,3.,-4.31)) ;
#161295=CARTESIAN_POINT('',(7.8,2.1,-4.31)) ;
#161296=CARTESIAN_POINT('',(7.8,2.1,-4.31)) ;
#161297=CARTESIAN_POINT('',(7.8,2.9,-4.31)) ;
#161298=CARTESIAN_POINT('',(7.8,3.,-4.31)) ;
#161299=CARTESIAN_POINT('',(7.8,2.9,-4.31)) ;
#161300=CARTESIAN_POINT('Origin',(7.8,3.,-4.21)) ;
#161301=CARTESIAN_POINT('',(7.7,2.1,-4.21)) ;
#161302=CARTESIAN_POINT('Origin',(7.8,2.1,-4.21)) ;
#161303=CARTESIAN_POINT('',(7.7,2.9,-4.21)) ;
#161304=CARTESIAN_POINT('',(7.7,3.,-4.21)) ;
#161305=CARTESIAN_POINT('Origin',(7.8,2.9,-4.21)) ;
#161306=CARTESIAN_POINT('Origin',(7.7,3.,-4.21)) ;
#161307=CARTESIAN_POINT('',(7.7,2.1,-3.41)) ;
#161308=CARTESIAN_POINT('',(7.7,2.1,-3.41)) ;
#161309=CARTESIAN_POINT('',(7.7,2.9,-3.41)) ;
#161310=CARTESIAN_POINT('',(7.7,3.,-3.41)) ;
#161311=CARTESIAN_POINT('',(7.7,2.9,-4.21)) ;
#161312=CARTESIAN_POINT('Origin',(7.8,3.,-3.41)) ;
#161313=CARTESIAN_POINT('',(7.8,2.1,-3.31)) ;
#161314=CARTESIAN_POINT('Origin',(7.8,2.1,-3.41)) ;
#161315=CARTESIAN_POINT('',(7.8,2.9,-3.31)) ;
#161316=CARTESIAN_POINT('',(7.8,3.,-3.31)) ;
#161317=CARTESIAN_POINT('Origin',(7.8,2.9,-3.41)) ;
#161318=CARTESIAN_POINT('Origin',(7.8,3.,-3.31)) ;
#161319=CARTESIAN_POINT('',(9.6,2.1,-3.31)) ;
#161320=CARTESIAN_POINT('',(9.6,2.1,-3.31)) ;
#161321=CARTESIAN_POINT('',(9.6,2.9,-3.31)) ;
#161322=CARTESIAN_POINT('',(9.6,3.,-3.31)) ;
#161323=CARTESIAN_POINT('',(7.8,2.9,-3.31)) ;
#161324=CARTESIAN_POINT('Origin',(9.6,3.,-3.41)) ;
#161325=CARTESIAN_POINT('',(9.7,2.1,-3.41)) ;
#161326=CARTESIAN_POINT('Origin',(9.6,2.1,-3.41)) ;
#161327=CARTESIAN_POINT('',(9.7,2.9,-3.41)) ;
#161328=CARTESIAN_POINT('',(9.7,3.,-3.41)) ;
#161329=CARTESIAN_POINT('Origin',(9.6,2.9,-3.41)) ;
#161330=CARTESIAN_POINT('Origin',(9.7,3.,-4.21)) ;
#161331=CARTESIAN_POINT('',(9.7,2.9,-4.21)) ;
#161332=CARTESIAN_POINT('',(9.7,2.1,-4.21)) ;
#161333=CARTESIAN_POINT('Origin',(9.6,3.,-4.21)) ;
#161334=CARTESIAN_POINT('',(7.8,3.,-3.41)) ;
#161335=CARTESIAN_POINT('',(9.6,3.,-3.41)) ;
#161336=CARTESIAN_POINT('',(9.6,3.,-3.41)) ;
#161337=CARTESIAN_POINT('',(9.6,3.,-4.21)) ;
#161338=CARTESIAN_POINT('',(9.6,3.,-4.21)) ;
#161339=CARTESIAN_POINT('',(7.8,3.,-4.21)) ;
#161340=CARTESIAN_POINT('',(9.6,3.,-4.21)) ;
#161341=CARTESIAN_POINT('',(7.8,3.,-4.21)) ;
#161342=CARTESIAN_POINT('Origin',(9.6,3.,-8.02)) ;
#161343=CARTESIAN_POINT('',(9.7,2.9,-8.02)) ;
#161344=CARTESIAN_POINT('',(9.7,2.1,-8.02)) ;
#161345=CARTESIAN_POINT('',(9.7,3.,-8.02)) ;
#161346=CARTESIAN_POINT('',(9.6,2.1,-8.12)) ;
#161347=CARTESIAN_POINT('Origin',(9.6,2.1,-8.02)) ;
#161348=CARTESIAN_POINT('',(9.6,2.9,-8.12)) ;
#161349=CARTESIAN_POINT('',(9.6,3.,-8.12)) ;
#161350=CARTESIAN_POINT('Origin',(9.6,2.9,-8.02)) ;
#161351=CARTESIAN_POINT('Origin',(7.8,3.,-8.12)) ;
#161352=CARTESIAN_POINT('',(7.8,2.1,-8.12)) ;
#161353=CARTESIAN_POINT('',(7.8,2.1,-8.12)) ;
#161354=CARTESIAN_POINT('',(7.8,2.9,-8.12)) ;
#161355=CARTESIAN_POINT('',(7.8,3.,-8.12)) ;
#161356=CARTESIAN_POINT('',(7.8,2.9,-8.12)) ;
#161357=CARTESIAN_POINT('Origin',(7.8,3.,-8.02)) ;
#161358=CARTESIAN_POINT('',(7.7,2.1,-8.02)) ;
#161359=CARTESIAN_POINT('Origin',(7.8,2.1,-8.02)) ;
#161360=CARTESIAN_POINT('',(7.7,2.9,-8.02)) ;
#161361=CARTESIAN_POINT('',(7.7,3.,-8.02)) ;
#161362=CARTESIAN_POINT('Origin',(7.8,2.9,-8.02)) ;
#161363=CARTESIAN_POINT('Origin',(7.7,3.,-8.02)) ;
#161364=CARTESIAN_POINT('',(7.7,2.1,-7.22)) ;
#161365=CARTESIAN_POINT('',(7.7,2.1,-7.22)) ;
#161366=CARTESIAN_POINT('',(7.7,2.9,-7.22)) ;
#161367=CARTESIAN_POINT('',(7.7,3.,-7.22)) ;
#161368=CARTESIAN_POINT('',(7.7,2.9,-8.02)) ;
#161369=CARTESIAN_POINT('Origin',(7.8,3.,-7.22)) ;
#161370=CARTESIAN_POINT('',(7.8,2.1,-7.12)) ;
#161371=CARTESIAN_POINT('Origin',(7.8,2.1,-7.22)) ;
#161372=CARTESIAN_POINT('',(7.8,2.9,-7.12)) ;
#161373=CARTESIAN_POINT('',(7.8,3.,-7.12)) ;
#161374=CARTESIAN_POINT('Origin',(7.8,2.9,-7.22)) ;
#161375=CARTESIAN_POINT('Origin',(7.8,3.,-7.12)) ;
#161376=CARTESIAN_POINT('',(9.6,2.1,-7.12)) ;
#161377=CARTESIAN_POINT('',(9.6,2.1,-7.12)) ;
#161378=CARTESIAN_POINT('',(9.6,2.9,-7.12)) ;
#161379=CARTESIAN_POINT('',(9.6,3.,-7.12)) ;
#161380=CARTESIAN_POINT('',(7.8,2.9,-7.12)) ;
#161381=CARTESIAN_POINT('Origin',(9.6,3.,-7.22)) ;
#161382=CARTESIAN_POINT('',(9.7,2.1,-7.22)) ;
#161383=CARTESIAN_POINT('Origin',(9.6,2.1,-7.22)) ;
#161384=CARTESIAN_POINT('',(9.7,2.9,-7.22)) ;
#161385=CARTESIAN_POINT('',(9.7,3.,-7.22)) ;
#161386=CARTESIAN_POINT('Origin',(9.6,2.9,-7.22)) ;
#161387=CARTESIAN_POINT('Origin',(9.7,3.,-8.02)) ;
#161388=CARTESIAN_POINT('',(9.7,2.9,-8.02)) ;
#161389=CARTESIAN_POINT('',(9.7,2.1,-8.02)) ;
#161390=CARTESIAN_POINT('Origin',(9.6,3.,-8.02)) ;
#161391=CARTESIAN_POINT('',(7.8,3.,-7.22)) ;
#161392=CARTESIAN_POINT('',(9.6,3.,-7.22)) ;
#161393=CARTESIAN_POINT('',(9.6,3.,-7.22)) ;
#161394=CARTESIAN_POINT('',(9.6,3.,-8.02)) ;
#161395=CARTESIAN_POINT('',(9.6,3.,-8.02)) ;
#161396=CARTESIAN_POINT('',(7.8,3.,-8.02)) ;
#161397=CARTESIAN_POINT('',(9.6,3.,-8.02)) ;
#161398=CARTESIAN_POINT('',(7.8,3.,-8.02)) ;
#161399=CARTESIAN_POINT('Origin',(9.6,3.,-11.83)) ;
#161400=CARTESIAN_POINT('',(9.7,2.9,-11.83)) ;
#161401=CARTESIAN_POINT('',(9.7,2.1,-11.83)) ;
#161402=CARTESIAN_POINT('',(9.7,3.,-11.83)) ;
#161403=CARTESIAN_POINT('',(9.6,2.1,-11.93)) ;
#161404=CARTESIAN_POINT('Origin',(9.6,2.1,-11.83)) ;
#161405=CARTESIAN_POINT('',(9.6,2.9,-11.93)) ;
#161406=CARTESIAN_POINT('',(9.6,3.,-11.93)) ;
#161407=CARTESIAN_POINT('Origin',(9.6,2.9,-11.83)) ;
#161408=CARTESIAN_POINT('Origin',(7.8,3.,-11.93)) ;
#161409=CARTESIAN_POINT('',(7.8,2.1,-11.93)) ;
#161410=CARTESIAN_POINT('',(7.8,2.1,-11.93)) ;
#161411=CARTESIAN_POINT('',(7.8,2.9,-11.93)) ;
#161412=CARTESIAN_POINT('',(7.8,3.,-11.93)) ;
#161413=CARTESIAN_POINT('',(7.8,2.9,-11.93)) ;
#161414=CARTESIAN_POINT('Origin',(7.8,3.,-11.83)) ;
#161415=CARTESIAN_POINT('',(7.7,2.1,-11.83)) ;
#161416=CARTESIAN_POINT('Origin',(7.8,2.1,-11.83)) ;
#161417=CARTESIAN_POINT('',(7.7,2.9,-11.83)) ;
#161418=CARTESIAN_POINT('',(7.7,3.,-11.83)) ;
#161419=CARTESIAN_POINT('Origin',(7.8,2.9,-11.83)) ;
#161420=CARTESIAN_POINT('Origin',(7.7,3.,-11.83)) ;
#161421=CARTESIAN_POINT('',(7.7,2.1,-11.03)) ;
#161422=CARTESIAN_POINT('',(7.7,2.1,-11.03)) ;
#161423=CARTESIAN_POINT('',(7.7,2.9,-11.03)) ;
#161424=CARTESIAN_POINT('',(7.7,3.,-11.03)) ;
#161425=CARTESIAN_POINT('',(7.7,2.9,-11.83)) ;
#161426=CARTESIAN_POINT('Origin',(7.8,3.,-11.03)) ;
#161427=CARTESIAN_POINT('',(7.8,2.1,-10.93)) ;
#161428=CARTESIAN_POINT('Origin',(7.8,2.1,-11.03)) ;
#161429=CARTESIAN_POINT('',(7.8,2.9,-10.93)) ;
#161430=CARTESIAN_POINT('',(7.8,3.,-10.93)) ;
#161431=CARTESIAN_POINT('Origin',(7.8,2.9,-11.03)) ;
#161432=CARTESIAN_POINT('Origin',(7.8,3.,-10.93)) ;
#161433=CARTESIAN_POINT('',(9.6,2.1,-10.93)) ;
#161434=CARTESIAN_POINT('',(9.6,2.1,-10.93)) ;
#161435=CARTESIAN_POINT('',(9.6,2.9,-10.93)) ;
#161436=CARTESIAN_POINT('',(9.6,3.,-10.93)) ;
#161437=CARTESIAN_POINT('',(7.8,2.9,-10.93)) ;
#161438=CARTESIAN_POINT('Origin',(9.6,3.,-11.03)) ;
#161439=CARTESIAN_POINT('',(9.7,2.1,-11.03)) ;
#161440=CARTESIAN_POINT('Origin',(9.6,2.1,-11.03)) ;
#161441=CARTESIAN_POINT('',(9.7,2.9,-11.03)) ;
#161442=CARTESIAN_POINT('',(9.7,3.,-11.03)) ;
#161443=CARTESIAN_POINT('Origin',(9.6,2.9,-11.03)) ;
#161444=CARTESIAN_POINT('Origin',(9.7,3.,-11.83)) ;
#161445=CARTESIAN_POINT('',(9.7,2.9,-11.83)) ;
#161446=CARTESIAN_POINT('',(9.7,2.1,-11.83)) ;
#161447=CARTESIAN_POINT('Origin',(9.6,3.,-11.83)) ;
#161448=CARTESIAN_POINT('',(7.8,3.,-11.03)) ;
#161449=CARTESIAN_POINT('',(9.6,3.,-11.03)) ;
#161450=CARTESIAN_POINT('',(9.6,3.,-11.03)) ;
#161451=CARTESIAN_POINT('',(9.6,3.,-11.83)) ;
#161452=CARTESIAN_POINT('',(9.6,3.,-11.83)) ;
#161453=CARTESIAN_POINT('',(7.8,3.,-11.83)) ;
#161454=CARTESIAN_POINT('',(9.6,3.,-11.83)) ;
#161455=CARTESIAN_POINT('',(7.8,3.,-11.83)) ;
#161456=CARTESIAN_POINT('Origin',(9.6,3.,-15.64)) ;
#161457=CARTESIAN_POINT('',(9.7,2.9,-15.64)) ;
#161458=CARTESIAN_POINT('',(9.7,2.1,-15.64)) ;
#161459=CARTESIAN_POINT('',(9.7,3.,-15.64)) ;
#161460=CARTESIAN_POINT('',(9.6,2.1,-15.74)) ;
#161461=CARTESIAN_POINT('Origin',(9.6,2.1,-15.64)) ;
#161462=CARTESIAN_POINT('',(9.6,2.9,-15.74)) ;
#161463=CARTESIAN_POINT('',(9.6,3.,-15.74)) ;
#161464=CARTESIAN_POINT('Origin',(9.6,2.9,-15.64)) ;
#161465=CARTESIAN_POINT('Origin',(7.8,3.,-15.74)) ;
#161466=CARTESIAN_POINT('',(7.8,2.1,-15.74)) ;
#161467=CARTESIAN_POINT('',(7.8,2.1,-15.74)) ;
#161468=CARTESIAN_POINT('',(7.8,2.9,-15.74)) ;
#161469=CARTESIAN_POINT('',(7.8,3.,-15.74)) ;
#161470=CARTESIAN_POINT('',(7.8,2.9,-15.74)) ;
#161471=CARTESIAN_POINT('Origin',(7.8,3.,-15.64)) ;
#161472=CARTESIAN_POINT('',(7.7,2.1,-15.64)) ;
#161473=CARTESIAN_POINT('Origin',(7.8,2.1,-15.64)) ;
#161474=CARTESIAN_POINT('',(7.7,2.9,-15.64)) ;
#161475=CARTESIAN_POINT('',(7.7,3.,-15.64)) ;
#161476=CARTESIAN_POINT('Origin',(7.8,2.9,-15.64)) ;
#161477=CARTESIAN_POINT('Origin',(7.7,3.,-15.64)) ;
#161478=CARTESIAN_POINT('',(7.7,2.1,-14.84)) ;
#161479=CARTESIAN_POINT('',(7.7,2.1,-14.84)) ;
#161480=CARTESIAN_POINT('',(7.7,2.9,-14.84)) ;
#161481=CARTESIAN_POINT('',(7.7,3.,-14.84)) ;
#161482=CARTESIAN_POINT('',(7.7,2.9,-15.64)) ;
#161483=CARTESIAN_POINT('Origin',(7.8,3.,-14.84)) ;
#161484=CARTESIAN_POINT('',(7.8,2.1,-14.74)) ;
#161485=CARTESIAN_POINT('Origin',(7.8,2.1,-14.84)) ;
#161486=CARTESIAN_POINT('',(7.8,2.9,-14.74)) ;
#161487=CARTESIAN_POINT('',(7.8,3.,-14.74)) ;
#161488=CARTESIAN_POINT('Origin',(7.8,2.9,-14.84)) ;
#161489=CARTESIAN_POINT('Origin',(7.8,3.,-14.74)) ;
#161490=CARTESIAN_POINT('',(9.6,2.1,-14.74)) ;
#161491=CARTESIAN_POINT('',(9.6,2.1,-14.74)) ;
#161492=CARTESIAN_POINT('',(9.6,2.9,-14.74)) ;
#161493=CARTESIAN_POINT('',(9.6,3.,-14.74)) ;
#161494=CARTESIAN_POINT('',(7.8,2.9,-14.74)) ;
#161495=CARTESIAN_POINT('Origin',(9.6,3.,-14.84)) ;
#161496=CARTESIAN_POINT('',(9.7,2.1,-14.84)) ;
#161497=CARTESIAN_POINT('Origin',(9.6,2.1,-14.84)) ;
#161498=CARTESIAN_POINT('',(9.7,2.9,-14.84)) ;
#161499=CARTESIAN_POINT('',(9.7,3.,-14.84)) ;
#161500=CARTESIAN_POINT('Origin',(9.6,2.9,-14.84)) ;
#161501=CARTESIAN_POINT('Origin',(9.7,3.,-15.64)) ;
#161502=CARTESIAN_POINT('',(9.7,2.9,-15.64)) ;
#161503=CARTESIAN_POINT('',(9.7,2.1,-15.64)) ;
#161504=CARTESIAN_POINT('Origin',(9.6,3.,-15.64)) ;
#161505=CARTESIAN_POINT('',(7.8,3.,-14.84)) ;
#161506=CARTESIAN_POINT('',(9.6,3.,-14.84)) ;
#161507=CARTESIAN_POINT('',(9.6,3.,-14.84)) ;
#161508=CARTESIAN_POINT('',(9.6,3.,-15.64)) ;
#161509=CARTESIAN_POINT('',(9.6,3.,-15.64)) ;
#161510=CARTESIAN_POINT('',(7.8,3.,-15.64)) ;
#161511=CARTESIAN_POINT('',(9.6,3.,-15.64)) ;
#161512=CARTESIAN_POINT('',(7.8,3.,-15.64)) ;
#161513=CARTESIAN_POINT('Origin',(9.6,3.,-19.45)) ;
#161514=CARTESIAN_POINT('',(9.7,2.9,-19.45)) ;
#161515=CARTESIAN_POINT('',(9.7,2.1,-19.45)) ;
#161516=CARTESIAN_POINT('',(9.7,3.,-19.45)) ;
#161517=CARTESIAN_POINT('',(9.6,2.1,-19.55)) ;
#161518=CARTESIAN_POINT('Origin',(9.6,2.1,-19.45)) ;
#161519=CARTESIAN_POINT('',(9.6,2.9,-19.55)) ;
#161520=CARTESIAN_POINT('',(9.6,3.,-19.55)) ;
#161521=CARTESIAN_POINT('Origin',(9.6,2.9,-19.45)) ;
#161522=CARTESIAN_POINT('Origin',(7.8,3.,-19.55)) ;
#161523=CARTESIAN_POINT('',(7.8,2.1,-19.55)) ;
#161524=CARTESIAN_POINT('',(7.8,2.1,-19.55)) ;
#161525=CARTESIAN_POINT('',(7.8,2.9,-19.55)) ;
#161526=CARTESIAN_POINT('',(7.8,3.,-19.55)) ;
#161527=CARTESIAN_POINT('',(7.8,2.9,-19.55)) ;
#161528=CARTESIAN_POINT('Origin',(7.8,3.,-19.45)) ;
#161529=CARTESIAN_POINT('',(7.7,2.1,-19.45)) ;
#161530=CARTESIAN_POINT('Origin',(7.8,2.1,-19.45)) ;
#161531=CARTESIAN_POINT('',(7.7,2.9,-19.45)) ;
#161532=CARTESIAN_POINT('',(7.7,3.,-19.45)) ;
#161533=CARTESIAN_POINT('Origin',(7.8,2.9,-19.45)) ;
#161534=CARTESIAN_POINT('Origin',(7.7,3.,-19.45)) ;
#161535=CARTESIAN_POINT('',(7.7,2.1,-18.65)) ;
#161536=CARTESIAN_POINT('',(7.7,2.1,-18.65)) ;
#161537=CARTESIAN_POINT('',(7.7,2.9,-18.65)) ;
#161538=CARTESIAN_POINT('',(7.7,3.,-18.65)) ;
#161539=CARTESIAN_POINT('',(7.7,2.9,-19.45)) ;
#161540=CARTESIAN_POINT('Origin',(7.8,3.,-18.65)) ;
#161541=CARTESIAN_POINT('',(7.8,2.1,-18.55)) ;
#161542=CARTESIAN_POINT('Origin',(7.8,2.1,-18.65)) ;
#161543=CARTESIAN_POINT('',(7.8,2.9,-18.55)) ;
#161544=CARTESIAN_POINT('',(7.8,3.,-18.55)) ;
#161545=CARTESIAN_POINT('Origin',(7.8,2.9,-18.65)) ;
#161546=CARTESIAN_POINT('Origin',(7.8,3.,-18.55)) ;
#161547=CARTESIAN_POINT('',(9.6,2.1,-18.55)) ;
#161548=CARTESIAN_POINT('',(9.6,2.1,-18.55)) ;
#161549=CARTESIAN_POINT('',(9.6,2.9,-18.55)) ;
#161550=CARTESIAN_POINT('',(9.6,3.,-18.55)) ;
#161551=CARTESIAN_POINT('',(7.8,2.9,-18.55)) ;
#161552=CARTESIAN_POINT('Origin',(9.6,3.,-18.65)) ;
#161553=CARTESIAN_POINT('',(9.7,2.1,-18.65)) ;
#161554=CARTESIAN_POINT('Origin',(9.6,2.1,-18.65)) ;
#161555=CARTESIAN_POINT('',(9.7,2.9,-18.65)) ;
#161556=CARTESIAN_POINT('',(9.7,3.,-18.65)) ;
#161557=CARTESIAN_POINT('Origin',(9.6,2.9,-18.65)) ;
#161558=CARTESIAN_POINT('Origin',(9.7,3.,-19.45)) ;
#161559=CARTESIAN_POINT('',(9.7,2.9,-19.45)) ;
#161560=CARTESIAN_POINT('',(9.7,2.1,-19.45)) ;
#161561=CARTESIAN_POINT('Origin',(9.6,3.,-19.45)) ;
#161562=CARTESIAN_POINT('',(7.8,3.,-18.65)) ;
#161563=CARTESIAN_POINT('',(9.6,3.,-18.65)) ;
#161564=CARTESIAN_POINT('',(9.6,3.,-18.65)) ;
#161565=CARTESIAN_POINT('',(9.6,3.,-19.45)) ;
#161566=CARTESIAN_POINT('',(9.6,3.,-19.45)) ;
#161567=CARTESIAN_POINT('',(7.8,3.,-19.45)) ;
#161568=CARTESIAN_POINT('',(9.6,3.,-19.45)) ;
#161569=CARTESIAN_POINT('',(7.8,3.,-19.45)) ;
#161570=CARTESIAN_POINT('Origin',(9.6,3.,-23.26)) ;
#161571=CARTESIAN_POINT('',(9.7,2.9,-23.26)) ;
#161572=CARTESIAN_POINT('',(9.7,2.1,-23.26)) ;
#161573=CARTESIAN_POINT('',(9.7,3.,-23.26)) ;
#161574=CARTESIAN_POINT('',(9.6,2.1,-23.36)) ;
#161575=CARTESIAN_POINT('Origin',(9.6,2.1,-23.26)) ;
#161576=CARTESIAN_POINT('',(9.6,2.9,-23.36)) ;
#161577=CARTESIAN_POINT('',(9.6,3.,-23.36)) ;
#161578=CARTESIAN_POINT('Origin',(9.6,2.9,-23.26)) ;
#161579=CARTESIAN_POINT('Origin',(7.8,3.,-23.36)) ;
#161580=CARTESIAN_POINT('',(7.8,2.1,-23.36)) ;
#161581=CARTESIAN_POINT('',(7.8,2.1,-23.36)) ;
#161582=CARTESIAN_POINT('',(7.8,2.9,-23.36)) ;
#161583=CARTESIAN_POINT('',(7.8,3.,-23.36)) ;
#161584=CARTESIAN_POINT('',(7.8,2.9,-23.36)) ;
#161585=CARTESIAN_POINT('Origin',(7.8,3.,-23.26)) ;
#161586=CARTESIAN_POINT('',(7.7,2.1,-23.26)) ;
#161587=CARTESIAN_POINT('Origin',(7.8,2.1,-23.26)) ;
#161588=CARTESIAN_POINT('',(7.7,2.9,-23.26)) ;
#161589=CARTESIAN_POINT('',(7.7,3.,-23.26)) ;
#161590=CARTESIAN_POINT('Origin',(7.8,2.9,-23.26)) ;
#161591=CARTESIAN_POINT('Origin',(7.7,3.,-23.26)) ;
#161592=CARTESIAN_POINT('',(7.7,2.1,-22.46)) ;
#161593=CARTESIAN_POINT('',(7.7,2.1,-22.46)) ;
#161594=CARTESIAN_POINT('',(7.7,2.9,-22.46)) ;
#161595=CARTESIAN_POINT('',(7.7,3.,-22.46)) ;
#161596=CARTESIAN_POINT('',(7.7,2.9,-23.26)) ;
#161597=CARTESIAN_POINT('Origin',(7.8,3.,-22.46)) ;
#161598=CARTESIAN_POINT('',(7.8,2.1,-22.36)) ;
#161599=CARTESIAN_POINT('Origin',(7.8,2.1,-22.46)) ;
#161600=CARTESIAN_POINT('',(7.8,2.9,-22.36)) ;
#161601=CARTESIAN_POINT('',(7.8,3.,-22.36)) ;
#161602=CARTESIAN_POINT('Origin',(7.8,2.9,-22.46)) ;
#161603=CARTESIAN_POINT('Origin',(7.8,3.,-22.36)) ;
#161604=CARTESIAN_POINT('',(9.6,2.1,-22.36)) ;
#161605=CARTESIAN_POINT('',(9.6,2.1,-22.36)) ;
#161606=CARTESIAN_POINT('',(9.6,2.9,-22.36)) ;
#161607=CARTESIAN_POINT('',(9.6,3.,-22.36)) ;
#161608=CARTESIAN_POINT('',(7.8,2.9,-22.36)) ;
#161609=CARTESIAN_POINT('Origin',(9.6,3.,-22.46)) ;
#161610=CARTESIAN_POINT('',(9.7,2.1,-22.46)) ;
#161611=CARTESIAN_POINT('Origin',(9.6,2.1,-22.46)) ;
#161612=CARTESIAN_POINT('',(9.7,2.9,-22.46)) ;
#161613=CARTESIAN_POINT('',(9.7,3.,-22.46)) ;
#161614=CARTESIAN_POINT('Origin',(9.6,2.9,-22.46)) ;
#161615=CARTESIAN_POINT('Origin',(9.7,3.,-23.26)) ;
#161616=CARTESIAN_POINT('',(9.7,2.9,-23.26)) ;
#161617=CARTESIAN_POINT('',(9.7,2.1,-23.26)) ;
#161618=CARTESIAN_POINT('Origin',(9.6,3.,-23.26)) ;
#161619=CARTESIAN_POINT('',(7.8,3.,-22.46)) ;
#161620=CARTESIAN_POINT('',(9.6,3.,-22.46)) ;
#161621=CARTESIAN_POINT('',(9.6,3.,-22.46)) ;
#161622=CARTESIAN_POINT('',(9.6,3.,-23.26)) ;
#161623=CARTESIAN_POINT('',(9.6,3.,-23.26)) ;
#161624=CARTESIAN_POINT('',(7.8,3.,-23.26)) ;
#161625=CARTESIAN_POINT('',(9.6,3.,-23.26)) ;
#161626=CARTESIAN_POINT('',(7.8,3.,-23.26)) ;
#161627=CARTESIAN_POINT('Origin',(9.6,3.,-27.07)) ;
#161628=CARTESIAN_POINT('',(9.7,2.9,-27.07)) ;
#161629=CARTESIAN_POINT('',(9.7,2.1,-27.07)) ;
#161630=CARTESIAN_POINT('',(9.7,3.,-27.07)) ;
#161631=CARTESIAN_POINT('',(9.6,2.1,-27.17)) ;
#161632=CARTESIAN_POINT('Origin',(9.6,2.1,-27.07)) ;
#161633=CARTESIAN_POINT('',(9.6,2.9,-27.17)) ;
#161634=CARTESIAN_POINT('',(9.6,3.,-27.17)) ;
#161635=CARTESIAN_POINT('Origin',(9.6,2.9,-27.07)) ;
#161636=CARTESIAN_POINT('Origin',(7.8,3.,-27.17)) ;
#161637=CARTESIAN_POINT('',(7.8,2.1,-27.17)) ;
#161638=CARTESIAN_POINT('',(7.8,2.1,-27.17)) ;
#161639=CARTESIAN_POINT('',(7.8,2.9,-27.17)) ;
#161640=CARTESIAN_POINT('',(7.8,3.,-27.17)) ;
#161641=CARTESIAN_POINT('',(7.8,2.9,-27.17)) ;
#161642=CARTESIAN_POINT('Origin',(7.8,3.,-27.07)) ;
#161643=CARTESIAN_POINT('',(7.7,2.1,-27.07)) ;
#161644=CARTESIAN_POINT('Origin',(7.8,2.1,-27.07)) ;
#161645=CARTESIAN_POINT('',(7.7,2.9,-27.07)) ;
#161646=CARTESIAN_POINT('',(7.7,3.,-27.07)) ;
#161647=CARTESIAN_POINT('Origin',(7.8,2.9,-27.07)) ;
#161648=CARTESIAN_POINT('Origin',(7.7,3.,-27.07)) ;
#161649=CARTESIAN_POINT('',(7.7,2.1,-26.27)) ;
#161650=CARTESIAN_POINT('',(7.7,2.1,-26.27)) ;
#161651=CARTESIAN_POINT('',(7.7,2.9,-26.27)) ;
#161652=CARTESIAN_POINT('',(7.7,3.,-26.27)) ;
#161653=CARTESIAN_POINT('',(7.7,2.9,-27.07)) ;
#161654=CARTESIAN_POINT('Origin',(7.8,3.,-26.27)) ;
#161655=CARTESIAN_POINT('',(7.8,2.1,-26.17)) ;
#161656=CARTESIAN_POINT('Origin',(7.8,2.1,-26.27)) ;
#161657=CARTESIAN_POINT('',(7.8,2.9,-26.17)) ;
#161658=CARTESIAN_POINT('',(7.8,3.,-26.17)) ;
#161659=CARTESIAN_POINT('Origin',(7.8,2.9,-26.27)) ;
#161660=CARTESIAN_POINT('Origin',(7.8,3.,-26.17)) ;
#161661=CARTESIAN_POINT('',(9.6,2.1,-26.17)) ;
#161662=CARTESIAN_POINT('',(9.6,2.1,-26.17)) ;
#161663=CARTESIAN_POINT('',(9.6,2.9,-26.17)) ;
#161664=CARTESIAN_POINT('',(9.6,3.,-26.17)) ;
#161665=CARTESIAN_POINT('',(7.8,2.9,-26.17)) ;
#161666=CARTESIAN_POINT('Origin',(9.6,3.,-26.27)) ;
#161667=CARTESIAN_POINT('',(9.7,2.1,-26.27)) ;
#161668=CARTESIAN_POINT('Origin',(9.6,2.1,-26.27)) ;
#161669=CARTESIAN_POINT('',(9.7,2.9,-26.27)) ;
#161670=CARTESIAN_POINT('',(9.7,3.,-26.27)) ;
#161671=CARTESIAN_POINT('Origin',(9.6,2.9,-26.27)) ;
#161672=CARTESIAN_POINT('Origin',(9.7,3.,-27.07)) ;
#161673=CARTESIAN_POINT('',(9.7,2.9,-27.07)) ;
#161674=CARTESIAN_POINT('',(9.7,2.1,-27.07)) ;
#161675=CARTESIAN_POINT('Origin',(9.6,3.,-27.07)) ;
#161676=CARTESIAN_POINT('',(7.8,3.,-26.27)) ;
#161677=CARTESIAN_POINT('',(9.6,3.,-26.27)) ;
#161678=CARTESIAN_POINT('',(9.6,3.,-26.27)) ;
#161679=CARTESIAN_POINT('',(9.6,3.,-27.07)) ;
#161680=CARTESIAN_POINT('',(9.6,3.,-27.07)) ;
#161681=CARTESIAN_POINT('',(7.8,3.,-27.07)) ;
#161682=CARTESIAN_POINT('',(9.6,3.,-27.07)) ;
#161683=CARTESIAN_POINT('',(7.8,3.,-27.07)) ;
#161684=CARTESIAN_POINT('Origin',(9.6,3.,-30.88)) ;
#161685=CARTESIAN_POINT('',(9.7,2.9,-30.88)) ;
#161686=CARTESIAN_POINT('',(9.7,2.1,-30.88)) ;
#161687=CARTESIAN_POINT('',(9.7,3.,-30.88)) ;
#161688=CARTESIAN_POINT('',(9.6,2.1,-30.98)) ;
#161689=CARTESIAN_POINT('Origin',(9.6,2.1,-30.88)) ;
#161690=CARTESIAN_POINT('',(9.6,2.9,-30.98)) ;
#161691=CARTESIAN_POINT('',(9.6,3.,-30.98)) ;
#161692=CARTESIAN_POINT('Origin',(9.6,2.9,-30.88)) ;
#161693=CARTESIAN_POINT('Origin',(7.8,3.,-30.98)) ;
#161694=CARTESIAN_POINT('',(7.8,2.1,-30.98)) ;
#161695=CARTESIAN_POINT('',(7.8,2.1,-30.98)) ;
#161696=CARTESIAN_POINT('',(7.8,2.9,-30.98)) ;
#161697=CARTESIAN_POINT('',(7.8,3.,-30.98)) ;
#161698=CARTESIAN_POINT('',(7.8,2.9,-30.98)) ;
#161699=CARTESIAN_POINT('Origin',(7.8,3.,-30.88)) ;
#161700=CARTESIAN_POINT('',(7.7,2.1,-30.88)) ;
#161701=CARTESIAN_POINT('Origin',(7.8,2.1,-30.88)) ;
#161702=CARTESIAN_POINT('',(7.7,2.9,-30.88)) ;
#161703=CARTESIAN_POINT('',(7.7,3.,-30.88)) ;
#161704=CARTESIAN_POINT('Origin',(7.8,2.9,-30.88)) ;
#161705=CARTESIAN_POINT('Origin',(7.7,3.,-30.88)) ;
#161706=CARTESIAN_POINT('',(7.7,2.1,-30.08)) ;
#161707=CARTESIAN_POINT('',(7.7,2.1,-30.08)) ;
#161708=CARTESIAN_POINT('',(7.7,2.9,-30.08)) ;
#161709=CARTESIAN_POINT('',(7.7,3.,-30.08)) ;
#161710=CARTESIAN_POINT('',(7.7,2.9,-30.88)) ;
#161711=CARTESIAN_POINT('Origin',(7.8,3.,-30.08)) ;
#161712=CARTESIAN_POINT('',(7.8,2.1,-29.98)) ;
#161713=CARTESIAN_POINT('Origin',(7.8,2.1,-30.08)) ;
#161714=CARTESIAN_POINT('',(7.8,2.9,-29.98)) ;
#161715=CARTESIAN_POINT('',(7.8,3.,-29.98)) ;
#161716=CARTESIAN_POINT('Origin',(7.8,2.9,-30.08)) ;
#161717=CARTESIAN_POINT('Origin',(7.8,3.,-29.98)) ;
#161718=CARTESIAN_POINT('',(9.6,2.1,-29.98)) ;
#161719=CARTESIAN_POINT('',(9.6,2.1,-29.98)) ;
#161720=CARTESIAN_POINT('',(9.6,2.9,-29.98)) ;
#161721=CARTESIAN_POINT('',(9.6,3.,-29.98)) ;
#161722=CARTESIAN_POINT('',(7.8,2.9,-29.98)) ;
#161723=CARTESIAN_POINT('Origin',(9.6,3.,-30.08)) ;
#161724=CARTESIAN_POINT('',(9.7,2.1,-30.08)) ;
#161725=CARTESIAN_POINT('Origin',(9.6,2.1,-30.08)) ;
#161726=CARTESIAN_POINT('',(9.7,2.9,-30.08)) ;
#161727=CARTESIAN_POINT('',(9.7,3.,-30.08)) ;
#161728=CARTESIAN_POINT('Origin',(9.6,2.9,-30.08)) ;
#161729=CARTESIAN_POINT('Origin',(9.7,3.,-30.88)) ;
#161730=CARTESIAN_POINT('',(9.7,2.9,-30.88)) ;
#161731=CARTESIAN_POINT('',(9.7,2.1,-30.88)) ;
#161732=CARTESIAN_POINT('Origin',(9.6,3.,-30.88)) ;
#161733=CARTESIAN_POINT('',(7.8,3.,-30.08)) ;
#161734=CARTESIAN_POINT('',(9.6,3.,-30.08)) ;
#161735=CARTESIAN_POINT('',(9.6,3.,-30.08)) ;
#161736=CARTESIAN_POINT('',(9.6,3.,-30.88)) ;
#161737=CARTESIAN_POINT('',(9.6,3.,-30.88)) ;
#161738=CARTESIAN_POINT('',(7.8,3.,-30.88)) ;
#161739=CARTESIAN_POINT('',(9.6,3.,-30.88)) ;
#161740=CARTESIAN_POINT('',(7.8,3.,-30.88)) ;
#161741=CARTESIAN_POINT('Origin',(9.6,3.,-34.69)) ;
#161742=CARTESIAN_POINT('',(9.7,2.9,-34.69)) ;
#161743=CARTESIAN_POINT('',(9.7,2.1,-34.69)) ;
#161744=CARTESIAN_POINT('',(9.7,3.,-34.69)) ;
#161745=CARTESIAN_POINT('',(9.6,2.1,-34.79)) ;
#161746=CARTESIAN_POINT('Origin',(9.6,2.1,-34.69)) ;
#161747=CARTESIAN_POINT('',(9.6,2.9,-34.79)) ;
#161748=CARTESIAN_POINT('',(9.6,3.,-34.79)) ;
#161749=CARTESIAN_POINT('Origin',(9.6,2.9,-34.69)) ;
#161750=CARTESIAN_POINT('Origin',(7.8,3.,-34.79)) ;
#161751=CARTESIAN_POINT('',(7.8,2.1,-34.79)) ;
#161752=CARTESIAN_POINT('',(7.8,2.1,-34.79)) ;
#161753=CARTESIAN_POINT('',(7.8,2.9,-34.79)) ;
#161754=CARTESIAN_POINT('',(7.8,3.,-34.79)) ;
#161755=CARTESIAN_POINT('',(7.8,2.9,-34.79)) ;
#161756=CARTESIAN_POINT('Origin',(7.8,3.,-34.69)) ;
#161757=CARTESIAN_POINT('',(7.7,2.1,-34.69)) ;
#161758=CARTESIAN_POINT('Origin',(7.8,2.1,-34.69)) ;
#161759=CARTESIAN_POINT('',(7.7,2.9,-34.69)) ;
#161760=CARTESIAN_POINT('',(7.7,3.,-34.69)) ;
#161761=CARTESIAN_POINT('Origin',(7.8,2.9,-34.69)) ;
#161762=CARTESIAN_POINT('Origin',(7.7,3.,-34.69)) ;
#161763=CARTESIAN_POINT('',(7.7,2.1,-33.89)) ;
#161764=CARTESIAN_POINT('',(7.7,2.1,-33.89)) ;
#161765=CARTESIAN_POINT('',(7.7,2.9,-33.89)) ;
#161766=CARTESIAN_POINT('',(7.7,3.,-33.89)) ;
#161767=CARTESIAN_POINT('',(7.7,2.9,-34.69)) ;
#161768=CARTESIAN_POINT('Origin',(7.8,3.,-33.89)) ;
#161769=CARTESIAN_POINT('',(7.8,2.1,-33.79)) ;
#161770=CARTESIAN_POINT('Origin',(7.8,2.1,-33.89)) ;
#161771=CARTESIAN_POINT('',(7.8,2.9,-33.79)) ;
#161772=CARTESIAN_POINT('',(7.8,3.,-33.79)) ;
#161773=CARTESIAN_POINT('Origin',(7.8,2.9,-33.89)) ;
#161774=CARTESIAN_POINT('Origin',(7.8,3.,-33.79)) ;
#161775=CARTESIAN_POINT('',(9.6,2.1,-33.79)) ;
#161776=CARTESIAN_POINT('',(9.6,2.1,-33.79)) ;
#161777=CARTESIAN_POINT('',(9.6,2.9,-33.79)) ;
#161778=CARTESIAN_POINT('',(9.6,3.,-33.79)) ;
#161779=CARTESIAN_POINT('',(7.8,2.9,-33.79)) ;
#161780=CARTESIAN_POINT('Origin',(9.6,3.,-33.89)) ;
#161781=CARTESIAN_POINT('',(9.7,2.1,-33.89)) ;
#161782=CARTESIAN_POINT('Origin',(9.6,2.1,-33.89)) ;
#161783=CARTESIAN_POINT('',(9.7,2.9,-33.89)) ;
#161784=CARTESIAN_POINT('',(9.7,3.,-33.89)) ;
#161785=CARTESIAN_POINT('Origin',(9.6,2.9,-33.89)) ;
#161786=CARTESIAN_POINT('Origin',(9.7,3.,-34.69)) ;
#161787=CARTESIAN_POINT('',(9.7,2.9,-34.69)) ;
#161788=CARTESIAN_POINT('',(9.7,2.1,-34.69)) ;
#161789=CARTESIAN_POINT('Origin',(9.6,3.,-34.69)) ;
#161790=CARTESIAN_POINT('',(7.8,3.,-33.89)) ;
#161791=CARTESIAN_POINT('',(9.6,3.,-33.89)) ;
#161792=CARTESIAN_POINT('',(9.6,3.,-33.89)) ;
#161793=CARTESIAN_POINT('',(9.6,3.,-34.69)) ;
#161794=CARTESIAN_POINT('',(9.6,3.,-34.69)) ;
#161795=CARTESIAN_POINT('',(7.8,3.,-34.69)) ;
#161796=CARTESIAN_POINT('',(9.6,3.,-34.69)) ;
#161797=CARTESIAN_POINT('',(7.8,3.,-34.69)) ;
#161798=CARTESIAN_POINT('Origin',(10.1,-2.15,-4.71311959340942)) ;
#161799=CARTESIAN_POINT('Origin',(10.1,-2.15,-4.71311959340942)) ;
#161800=CARTESIAN_POINT('Origin',(10.1,-2.15,-4.71311959340942)) ;
#161801=CARTESIAN_POINT('Origin',(10.1,-2.15,-4.71311959340942)) ;
#161802=CARTESIAN_POINT('Origin',(10.1,-3.65625,-3.81)) ;
#161803=CARTESIAN_POINT('Origin',(10.1,-2.15,-2.90688040659058)) ;
#161804=CARTESIAN_POINT('Origin',(10.2,-2.15,-4.71311959340942)) ;
#161805=CARTESIAN_POINT('Origin',(3.7,-2.15,-4.71311959340942)) ;
#161806=CARTESIAN_POINT('Origin',(10.1,-2.15,-3.81)) ;
#161807=CARTESIAN_POINT('Origin',(10.1,-2.15,-5.115)) ;
#161808=CARTESIAN_POINT('Origin',(10.1,-3.65625,-5.115)) ;
#161809=CARTESIAN_POINT('Origin',(10.1,1.9,-5.115)) ;
#161810=CARTESIAN_POINT('Origin',(10.1,-2.15,-5.115)) ;
#161811=CARTESIAN_POINT('Origin',(10.1,1.9,-3.81)) ;
#161812=CARTESIAN_POINT('Origin',(10.1,1.9,-5.115)) ;
#161813=CARTESIAN_POINT('Origin',(10.1,1.9,-2.505)) ;
#161814=CARTESIAN_POINT('Origin',(10.1,-2.15,-2.90688040659058)) ;
#161815=CARTESIAN_POINT('Origin',(10.1,-2.15,-2.90688040659058)) ;
#161816=CARTESIAN_POINT('Origin',(10.1,-2.15,-2.90688040659058)) ;
#161817=CARTESIAN_POINT('Origin',(3.7,-2.15,-4.71311959340942)) ;
#161818=CARTESIAN_POINT('Origin',(3.7,-2.35,-4.71311959340942)) ;
#161819=CARTESIAN_POINT('Origin',(3.7,-2.32153024911032,-4.6102732340176)) ;
#161820=CARTESIAN_POINT('Origin',(10.1,-2.15,-5.115)) ;
#161821=CARTESIAN_POINT('Origin',(10.1,-2.15,-5.115)) ;
#161822=CARTESIAN_POINT('Origin',(10.1,-3.65625,-2.505)) ;
#161823=CARTESIAN_POINT('Origin',(10.1,1.9,-2.505)) ;
#161824=CARTESIAN_POINT('Origin',(10.1,-2.15,-2.505)) ;
#161825=CARTESIAN_POINT('Origin',(10.1,-2.15,-3.81)) ;
#161826=CARTESIAN_POINT('Origin',(10.1,-2.15,-2.505)) ;
#161827=CARTESIAN_POINT('Origin',(10.2,-2.15,-2.90688040659058)) ;
#161828=CARTESIAN_POINT('Origin',(3.7,-2.15,-2.90688040659058)) ;
#161829=CARTESIAN_POINT('Origin',(3.7,-3.65625,-3.81)) ;
#161830=CARTESIAN_POINT('Origin',(3.7,-2.32153024911032,-3.0097267659824)) ;
#161831=CARTESIAN_POINT('Origin',(3.7,-2.35,-4.685)) ;
#161832=CARTESIAN_POINT('Origin',(3.7,-2.35,-5.115)) ;
#161833=CARTESIAN_POINT('Origin',(3.6,-2.15,-5.115)) ;
#161834=CARTESIAN_POINT('Origin',(3.7,-2.15,-5.115)) ;
#161835=CARTESIAN_POINT('Origin',(10.1,-2.15,-2.505)) ;
#161836=CARTESIAN_POINT('Origin',(10.1,-2.15,-2.505)) ;
#161837=CARTESIAN_POINT('Origin',(3.7,-2.15,-2.90688040659058)) ;
#161838=CARTESIAN_POINT('Origin',(3.7,-2.35,-2.90688040659058)) ;
#161839=CARTESIAN_POINT('Origin',(3.7,-2.35,-5.115)) ;
#161840=CARTESIAN_POINT('Origin',(3.5,-2.35,-5.115)) ;
#161841=CARTESIAN_POINT('Origin',(10.2,-2.15,-2.505)) ;
#161842=CARTESIAN_POINT('Origin',(3.7,-2.15,-2.505)) ;
#161843=CARTESIAN_POINT('Origin',(3.7,-2.35,-2.405)) ;
#161844=CARTESIAN_POINT('Origin',(3.7,-2.35,-2.505)) ;
#161845=CARTESIAN_POINT('Origin',(3.5,-3.80813298381585E-16,-5.115)) ;
#161846=CARTESIAN_POINT('Origin',(3.5,-5.15,-5.115)) ;
#161847=CARTESIAN_POINT('Origin',(3.6,1.9,-5.315)) ;
#161848=CARTESIAN_POINT('Origin',(3.5,1.9,-5.315)) ;
#161849=CARTESIAN_POINT('Origin',(2.7,1.9,-5.315)) ;
#161850=CARTESIAN_POINT('Origin',(2.7,1.9,-5.215)) ;
#161851=CARTESIAN_POINT('Origin',(2.7,1.9,-6.115)) ;
#161852=CARTESIAN_POINT('Origin',(2.7,1.9,-5.315)) ;
#161853=CARTESIAN_POINT('Origin',(3.7,-2.35,-2.505)) ;
#161854=CARTESIAN_POINT('Origin',(3.5,-2.35,-2.505)) ;
#161855=CARTESIAN_POINT('Origin',(3.5,-5.15,-5.115)) ;
#161856=CARTESIAN_POINT('Origin',(3.5,-5.15,-5.115)) ;
#161857=CARTESIAN_POINT('Origin',(3.5,-5.15,-5.115)) ;
#161858=CARTESIAN_POINT('Origin',(2.7,1.9,-5.315)) ;
#161859=CARTESIAN_POINT('Origin',(2.7,1.9,-5.315)) ;
#161860=CARTESIAN_POINT('Origin',(3.5,3.0290702335686E-16,-2.505)) ;
#161861=CARTESIAN_POINT('Origin',(3.5,-5.15,-2.505)) ;
#161862=CARTESIAN_POINT('Origin',(3.5,-5.15,0.)) ;
#161863=CARTESIAN_POINT('Origin',(3.5,-5.15,-2.505)) ;
#161864=CARTESIAN_POINT('Origin',(3.6,-5.15,-5.115)) ;
#161865=CARTESIAN_POINT('Origin',(2.7,-5.15,-5.115)) ;
#161866=CARTESIAN_POINT('Origin',(2.7,-5.25,-5.315)) ;
#161867=CARTESIAN_POINT('Origin',(2.7,-5.15,-5.315)) ;
#161868=CARTESIAN_POINT('Origin',(3.5,-5.15,-2.505)) ;
#161869=CARTESIAN_POINT('Origin',(3.5,-5.15,-2.505)) ;
#161870=CARTESIAN_POINT('Origin',(2.7,-5.15,-5.115)) ;
#161871=CARTESIAN_POINT('Origin',(2.7,-5.35,-5.115)) ;
#161872=CARTESIAN_POINT('Origin',(3.6,1.9,-2.305)) ;
#161873=CARTESIAN_POINT('Origin',(3.5,1.9,-2.305)) ;
#161874=CARTESIAN_POINT('Origin',(2.7,1.9,-2.305)) ;
#161875=CARTESIAN_POINT('Origin',(3.6,-5.15,-2.505)) ;
#161876=CARTESIAN_POINT('Origin',(2.7,-5.15,-2.505)) ;
#161877=CARTESIAN_POINT('Origin',(2.7,-5.35,-2.405)) ;
#161878=CARTESIAN_POINT('Origin',(2.7,-5.35,-2.505)) ;
#161879=CARTESIAN_POINT('Origin',(2.7,1.9,-2.305)) ;
#161880=CARTESIAN_POINT('Origin',(2.7,1.9,-2.305)) ;
#161881=CARTESIAN_POINT('Origin',(2.7,-5.15,-2.505)) ;
#161882=CARTESIAN_POINT('Origin',(2.7,-5.15,-2.305)) ;
#161883=CARTESIAN_POINT('Origin',(2.7,2.,-2.305)) ;
#161884=CARTESIAN_POINT('Origin',(7.8,2.1,-4.21)) ;
#161885=CARTESIAN_POINT('Origin',(7.8,2.1,-4.41)) ;
#161886=CARTESIAN_POINT('Origin',(7.6,2.1,-4.21)) ;
#161887=CARTESIAN_POINT('Origin',(7.6,2.1,-4.21)) ;
#161888=CARTESIAN_POINT('Origin',(7.6,2.1,-3.41)) ;
#161889=CARTESIAN_POINT('Origin',(7.8,2.1,-4.41)) ;
#161890=CARTESIAN_POINT('Origin',(9.6,2.1,-4.41)) ;
#161891=CARTESIAN_POINT('Origin',(7.8,2.1,-3.41)) ;
#161892=CARTESIAN_POINT('Origin',(7.8,2.1,-3.21)) ;
#161893=CARTESIAN_POINT('Origin',(9.6,2.1,-4.21)) ;
#161894=CARTESIAN_POINT('Origin',(9.8,2.1,-4.21)) ;
#161895=CARTESIAN_POINT('Origin',(7.8,2.1,-3.21)) ;
#161896=CARTESIAN_POINT('Origin',(9.6,2.1,-3.21)) ;
#161897=CARTESIAN_POINT('Origin',(9.8,2.1,-4.21)) ;
#161898=CARTESIAN_POINT('Origin',(9.8,2.1,-3.41)) ;
#161899=CARTESIAN_POINT('Origin',(9.6,2.1,-3.41)) ;
#161900=CARTESIAN_POINT('Origin',(-4.9,-6.45,-35.39)) ;
#161901=CARTESIAN_POINT('',(-4.85857864376269,-6.52071067811866,-35.3192893218814)) ;
#161902=CARTESIAN_POINT('Origin',(-5.01417009506433,-6.44703459697317,-35.3970866853867)) ;
#161903=CARTESIAN_POINT('Ctrl Pts',(-4.85857864376269,-6.52071067811868,
-35.3192893218814)) ;
#161904=CARTESIAN_POINT('Ctrl Pts',(-4.86759079869274,-6.5252167555837,
-35.3237953993464)) ;
#161905=CARTESIAN_POINT('Ctrl Pts',(-4.87748625817285,-6.52928079264427,
-35.3287264816717)) ;
#161906=CARTESIAN_POINT('Ctrl Pts',(-4.89811277057011,-6.53624680748678,
-35.3390208825486)) ;
#161907=CARTESIAN_POINT('Ctrl Pts',(-4.90880509433771,-6.53918030781879,
-35.3443639841507)) ;
#161908=CARTESIAN_POINT('Ctrl Pts',(-4.92101859322336,-6.54185985500363,
-35.3504747545345)) ;
#161909=CARTESIAN_POINT('Ctrl Pts',(-4.92228751722852,-6.54213045061265,
-35.3511097099098)) ;
#161910=CARTESIAN_POINT('Ctrl Pts',(-4.9350493700286,-6.54477467909837,
-35.3574962891342)) ;
#161911=CARTESIAN_POINT('Ctrl Pts',(-4.94677936428208,-6.54657370273658,
-35.3633715724064)) ;
#161912=CARTESIAN_POINT('Ctrl Pts',(-4.96920025888411,-6.5489600764314,
-35.3745957747614)) ;
#161913=CARTESIAN_POINT('Ctrl Pts',(-4.97990192168179,-6.5496301025519,
-35.3799500759452)) ;
#161914=CARTESIAN_POINT('Ctrl Pts',(-4.99357116034318,-6.54996164986963,
-35.3867855738171)) ;
#161915=CARTESIAN_POINT('Ctrl Pts',(-4.99680282631925,-6.55,-35.3884014131596)) ;
#161916=CARTESIAN_POINT('Ctrl Pts',(-5.,-6.55,-35.39)) ;
#161917=CARTESIAN_POINT('',(-3.94142135623684,-6.52071067811842,-35.3192893218811)) ;
#161918=CARTESIAN_POINT('Ctrl Pts',(-3.8,-6.55,-35.39)) ;
#161919=CARTESIAN_POINT('Ctrl Pts',(-3.81016571653571,-6.55,-35.3849171417321)) ;
#161920=CARTESIAN_POINT('Ctrl Pts',(-3.82068315091917,-6.54961031187957,
-35.3796576838579)) ;
#161921=CARTESIAN_POINT('Ctrl Pts',(-3.84304266527945,-6.54783411578236,
-35.3684679497194)) ;
#161922=CARTESIAN_POINT('Ctrl Pts',(-3.85491327259758,-6.54635217950662,
-35.3625227617952)) ;
#161923=CARTESIAN_POINT('Ctrl Pts',(-3.87771616261517,-6.54231439116937,
-35.3511067603977)) ;
#161924=CARTESIAN_POINT('Ctrl Pts',(-3.88866251834261,-6.53982180675303,
-35.345629861311)) ;
#161925=CARTESIAN_POINT('Ctrl Pts',(-3.90045005710787,-6.53645537933612,
-35.3397406960422)) ;
#161926=CARTESIAN_POINT('Ctrl Pts',(-3.90170928105007,-6.53608665347898,
-35.3391116827677)) ;
#161927=CARTESIAN_POINT('Ctrl Pts',(-3.91388077026579,-6.53243308776766,
-35.333032751352)) ;
#161928=CARTESIAN_POINT('Ctrl Pts',(-3.92429308263634,-6.52859969139749,
-35.3278422384292)) ;
#161929=CARTESIAN_POINT('Ctrl Pts',(-3.93645488997201,-6.52312881451524,
-35.3217711869642)) ;
#161930=CARTESIAN_POINT('Ctrl Pts',(-3.93897066587108,-6.52193602330131,
-35.320514667064)) ;
#161931=CARTESIAN_POINT('Ctrl Pts',(-3.94142135623684,-6.52071067811842,
-35.3192893218811)) ;
#161932=CARTESIAN_POINT('Origin',(-3.78571994569831,-6.44700925664017,-35.397142104249)) ;
#161933=CARTESIAN_POINT('Origin',(-3.8,-6.45,-33.29)) ;
#161934=CARTESIAN_POINT('',(-3.87071067811865,-6.52071067811866,-33.3314213562373)) ;
#161935=CARTESIAN_POINT('Ctrl Pts',(-3.8,-6.55,-33.19)) ;
#161936=CARTESIAN_POINT('Ctrl Pts',(-3.80508285826794,-6.55,-33.2001657165359)) ;
#161937=CARTESIAN_POINT('Ctrl Pts',(-3.81034231614204,-6.54961031187957,
-33.2106831509196)) ;
#161938=CARTESIAN_POINT('Ctrl Pts',(-3.82153205028074,-6.54783411578234,
-33.2330426652806)) ;
#161939=CARTESIAN_POINT('Ctrl Pts',(-3.82747723820518,-6.54635217950653,
-33.2449132725992)) ;
#161940=CARTESIAN_POINT('Ctrl Pts',(-3.83889323960396,-6.54231439116874,
-33.2677161626196)) ;
#161941=CARTESIAN_POINT('Ctrl Pts',(-3.84437013869177,-6.53982180675175,
-33.2786625183492)) ;
#161942=CARTESIAN_POINT('Ctrl Pts',(-3.8502593039605,-6.53645537933455,
-33.2904500571143)) ;
#161943=CARTESIAN_POINT('Ctrl Pts',(-3.85088831723394,-6.53608665347802,
-33.2917092810543)) ;
#161944=CARTESIAN_POINT('Ctrl Pts',(-3.85696724864837,-6.53243308776737,
-33.3038807702676)) ;
#161945=CARTESIAN_POINT('Ctrl Pts',(-3.86215776157101,-6.52859969139729,
-33.3142930826378)) ;
#161946=CARTESIAN_POINT('Ctrl Pts',(-3.86822881303577,-6.52312881451525,
-33.3264548899729)) ;
#161947=CARTESIAN_POINT('Ctrl Pts',(-3.86948533293589,-6.52193602330142,
-33.3289706658718)) ;
#161948=CARTESIAN_POINT('Ctrl Pts',(-3.87071067811865,-6.52071067811866,
-33.3314213562373)) ;
#161949=CARTESIAN_POINT('Origin',(-3.79285789576313,-6.44700925664404,-33.1757199457244)) ;
#161950=CARTESIAN_POINT('',(-3.87071067811865,-6.52071067811866,-35.2485786437627)) ;
#161951=CARTESIAN_POINT('Origin',(-3.79291331463517,-6.44703459698217,-35.4041700950208)) ;
#161952=CARTESIAN_POINT('Ctrl Pts',(-3.87071067811865,-6.52071067811866,
-35.2485786437627)) ;
#161953=CARTESIAN_POINT('Ctrl Pts',(-3.86620460065363,-6.52521675558368,
-35.2575907986928)) ;
#161954=CARTESIAN_POINT('Ctrl Pts',(-3.86127351832835,-6.52928079264423,
-35.2674862581729)) ;
#161955=CARTESIAN_POINT('Ctrl Pts',(-3.85097911745215,-6.5362468074863,
-35.2881127705688)) ;
#161956=CARTESIAN_POINT('Ctrl Pts',(-3.84563601585079,-6.53918030781798,
-35.2988050943349)) ;
#161957=CARTESIAN_POINT('Ctrl Pts',(-3.83952524546706,-6.54185985500296,
-35.3110185932205)) ;
#161958=CARTESIAN_POINT('Ctrl Pts',(-3.83889029009099,-6.5421304506123,
-35.3122875172271)) ;
#161959=CARTESIAN_POINT('Ctrl Pts',(-3.832503710866,-6.54477467909831,-35.3250493700286)) ;
#161960=CARTESIAN_POINT('Ctrl Pts',(-3.82662842759374,-6.54657370273655,
-35.336779364282)) ;
#161961=CARTESIAN_POINT('Ctrl Pts',(-3.81540422523868,-6.54896007643138,
-35.3592002588841)) ;
#161962=CARTESIAN_POINT('Ctrl Pts',(-3.81004992405483,-6.54963010255189,
-35.3699019216818)) ;
#161963=CARTESIAN_POINT('Ctrl Pts',(-3.80321442618285,-6.54996164986963,
-35.3835711603432)) ;
#161964=CARTESIAN_POINT('Ctrl Pts',(-3.80159858684037,-6.55,-35.3868028263193)) ;
#161965=CARTESIAN_POINT('Ctrl Pts',(-3.8,-6.55,-35.39)) ;
#161966=CARTESIAN_POINT('Origin',(-5.,-6.45,-33.29)) ;
#161967=CARTESIAN_POINT('',(-4.92928932188134,-6.52071067811866,-35.2485786437627)) ;
#161968=CARTESIAN_POINT('Ctrl Pts',(-5.,-6.55,-35.39)) ;
#161969=CARTESIAN_POINT('Ctrl Pts',(-4.99491714173205,-6.55,-35.3798342834641)) ;
#161970=CARTESIAN_POINT('Ctrl Pts',(-4.98965768385794,-6.54961031187957,
-35.3693168490804)) ;
#161971=CARTESIAN_POINT('Ctrl Pts',(-4.97846794971924,-6.54783411578233,
-35.3469573347195)) ;
#161972=CARTESIAN_POINT('Ctrl Pts',(-4.9725227617948,-6.54635217950652,
-35.3350867274009)) ;
#161973=CARTESIAN_POINT('Ctrl Pts',(-4.96110676039595,-6.54231439116871,
-35.3122838373804)) ;
#161974=CARTESIAN_POINT('Ctrl Pts',(-4.95562986130807,-6.53982180675168,
-35.3013374816505)) ;
#161975=CARTESIAN_POINT('Ctrl Pts',(-4.94974069603936,-6.53645537933446,
-35.2895499428855)) ;
#161976=CARTESIAN_POINT('Ctrl Pts',(-4.949111682766,-6.53608665347798,-35.2882907189456)) ;
#161977=CARTESIAN_POINT('Ctrl Pts',(-4.94303275135165,-6.53243308776738,
-35.2761192297325)) ;
#161978=CARTESIAN_POINT('Ctrl Pts',(-4.93784223842901,-6.52859969139732,
-35.2657069173623)) ;
#161979=CARTESIAN_POINT('Ctrl Pts',(-4.93177118696425,-6.52312881451527,
-35.2535451100271)) ;
#161980=CARTESIAN_POINT('Ctrl Pts',(-4.93051466706411,-6.52193602330142,
-35.2510293341283)) ;
#161981=CARTESIAN_POINT('Ctrl Pts',(-4.92928932188135,-6.52071067811866,
-35.2485786437627)) ;
#161982=CARTESIAN_POINT('Origin',(-5.007142104231,-6.44700925664598,-35.4042800542639)) ;
#161983=CARTESIAN_POINT('',(-4.92928932188135,-6.52071067811866,-33.3314213562373)) ;
#161984=CARTESIAN_POINT('Origin',(-5.00708668535334,-6.44703459698616,-33.1758299050023)) ;
#161985=CARTESIAN_POINT('Ctrl Pts',(-4.92928932188135,-6.52071067811866,
-33.3314213562373)) ;
#161986=CARTESIAN_POINT('Ctrl Pts',(-4.93379539934637,-6.52521675558368,
-33.3224092013072)) ;
#161987=CARTESIAN_POINT('Ctrl Pts',(-4.93872648167165,-6.52928079264423,
-33.3125137418271)) ;
#161988=CARTESIAN_POINT('Ctrl Pts',(-4.94902088254777,-6.53624680748625,
-33.2918872294312)) ;
#161989=CARTESIAN_POINT('Ctrl Pts',(-4.95436398414905,-6.53918030781789,
-33.2811949056653)) ;
#161990=CARTESIAN_POINT('Ctrl Pts',(-4.96047475453277,-6.54185985500289,
-33.2689814067798)) ;
#161991=CARTESIAN_POINT('Ctrl Pts',(-4.96110970990891,-6.54213045061226,
-33.2677124827731)) ;
#161992=CARTESIAN_POINT('Ctrl Pts',(-4.96749628913395,-6.5447746790983,
-33.2549506299714)) ;
#161993=CARTESIAN_POINT('Ctrl Pts',(-4.97337157240622,-6.54657370273654,
-33.2432206357179)) ;
#161994=CARTESIAN_POINT('Ctrl Pts',(-4.98459577476128,-6.54896007643137,
-33.2207997411159)) ;
#161995=CARTESIAN_POINT('Ctrl Pts',(-4.98995007594513,-6.54963010255189,
-33.2100980783182)) ;
#161996=CARTESIAN_POINT('Ctrl Pts',(-4.99678557381713,-6.54996164986963,
-33.1964288396568)) ;
#161997=CARTESIAN_POINT('Ctrl Pts',(-4.99840141315962,-6.55,-33.1931971736808)) ;
#161998=CARTESIAN_POINT('Ctrl Pts',(-5.,-6.55,-33.19)) ;
#161999=CARTESIAN_POINT('Origin',(-4.9,-6.45,-33.19)) ;
#162000=CARTESIAN_POINT('',(-4.85857864376269,-6.52071067811865,-33.2607106781187)) ;
#162001=CARTESIAN_POINT('Ctrl Pts',(-5.,-6.55,-33.19)) ;
#162002=CARTESIAN_POINT('Ctrl Pts',(-4.98983428346409,-6.55,-33.1950828582679)) ;
#162003=CARTESIAN_POINT('Ctrl Pts',(-4.97931684908043,-6.54961031187958,
-33.200342316142)) ;
#162004=CARTESIAN_POINT('Ctrl Pts',(-4.95695733471947,-6.54783411578237,
-33.2115320502806)) ;
#162005=CARTESIAN_POINT('Ctrl Pts',(-4.94508672740085,-6.54635217950657,
-33.217477238205)) ;
#162006=CARTESIAN_POINT('Ctrl Pts',(-4.92228383738129,-6.54231439116894,
-33.2288932396034)) ;
#162007=CARTESIAN_POINT('Ctrl Pts',(-4.91133748165239,-6.53982180675217,
-33.2343701386909)) ;
#162008=CARTESIAN_POINT('Ctrl Pts',(-4.89954994288722,-6.53645537933505,
-33.2402593039596)) ;
#162009=CARTESIAN_POINT('Ctrl Pts',(-4.8982907189464,-6.5360866534783,-33.2408883172335)) ;
#162010=CARTESIAN_POINT('Ctrl Pts',(-4.88611922973238,-6.53243308776742,
-33.2469672486483)) ;
#162011=CARTESIAN_POINT('Ctrl Pts',(-4.87570691736216,-6.52859969139732,
-33.252157761571)) ;
#162012=CARTESIAN_POINT('Ctrl Pts',(-4.86354511002705,-6.52312881451524,
-33.2582288130358)) ;
#162013=CARTESIAN_POINT('Ctrl Pts',(-4.86102933412822,-6.52193602330141,
-33.2594853329359)) ;
#162014=CARTESIAN_POINT('Ctrl Pts',(-4.85857864376269,-6.52071067811863,
-33.2607106781187)) ;
#162015=CARTESIAN_POINT('Origin',(-5.01428005430853,-6.44700925663641,-33.1828578957469)) ;
#162016=CARTESIAN_POINT('',(-3.94142135623684,-6.52071067811842,-33.2607106781189)) ;
#162017=CARTESIAN_POINT('Origin',(-3.7858299049171,-6.44703459697097,-33.1829133146053)) ;
#162018=CARTESIAN_POINT('Ctrl Pts',(-3.94142135623684,-6.52071067811842,
-33.2607106781189)) ;
#162019=CARTESIAN_POINT('Ctrl Pts',(-3.93240920130662,-6.52521675558355,
-33.2562046006538)) ;
#162020=CARTESIAN_POINT('Ctrl Pts',(-3.92251374182629,-6.52928079264416,
-33.2512735183285)) ;
#162021=CARTESIAN_POINT('Ctrl Pts',(-3.90188722942757,-6.53624680748717,
-33.2409791174509)) ;
#162022=CARTESIAN_POINT('Ctrl Pts',(-3.89119490565864,-6.53918030781945,
-33.2356360158481)) ;
#162023=CARTESIAN_POINT('Ctrl Pts',(-3.87898140677303,-6.54185985500413,
-33.2295252454643)) ;
#162024=CARTESIAN_POINT('Ctrl Pts',(-3.87771248276927,-6.54213045061284,
-33.2288902900897)) ;
#162025=CARTESIAN_POINT('Ctrl Pts',(-3.86495062997103,-6.54477467909819,
-33.2225037108663)) ;
#162026=CARTESIAN_POINT('Ctrl Pts',(-3.85322063571802,-6.54657370273639,
-33.2166284275943)) ;
#162027=CARTESIAN_POINT('Ctrl Pts',(-3.83079974111668,-6.54896007643127,
-33.2054042252394)) ;
#162028=CARTESIAN_POINT('Ctrl Pts',(-3.82009807831922,-6.54963010255182,
-33.2000499240556)) ;
#162029=CARTESIAN_POINT('Ctrl Pts',(-3.80642883965762,-6.54996164986962,
-33.1932144261834)) ;
#162030=CARTESIAN_POINT('Ctrl Pts',(-3.80319717368114,-6.55,-33.1915985868406)) ;
#162031=CARTESIAN_POINT('Ctrl Pts',(-3.8,-6.55,-33.19)) ;
#162032=CARTESIAN_POINT('Origin',(-4.9,-6.45,-31.58)) ;
#162033=CARTESIAN_POINT('',(-4.85857864376269,-6.52071067811866,-31.5092893218814)) ;
#162034=CARTESIAN_POINT('Origin',(-5.01417009505135,-6.44703459697586,-31.5870866853803)) ;
#162035=CARTESIAN_POINT('Ctrl Pts',(-4.85857864376269,-6.52071067811868,
-31.5092893218814)) ;
#162036=CARTESIAN_POINT('Ctrl Pts',(-4.86759079869273,-6.5252167555837,
-31.5137953993464)) ;
#162037=CARTESIAN_POINT('Ctrl Pts',(-4.87748625817284,-6.52928079264427,
-31.5187264816717)) ;
#162038=CARTESIAN_POINT('Ctrl Pts',(-4.89811277056898,-6.53624680748639,
-31.529020882548)) ;
#162039=CARTESIAN_POINT('Ctrl Pts',(-4.90880509433532,-6.53918030781814,
-31.5343639841495)) ;
#162040=CARTESIAN_POINT('Ctrl Pts',(-4.92101859322092,-6.54185985500311,
-31.5404747545333)) ;
#162041=CARTESIAN_POINT('Ctrl Pts',(-4.9222875172273,-6.5421304506124,-31.5411097099092)) ;
#162042=CARTESIAN_POINT('Ctrl Pts',(-4.9350493700286,-6.54477467909837,
-31.5474962891341)) ;
#162043=CARTESIAN_POINT('Ctrl Pts',(-4.94677936428206,-6.54657370273659,
-31.5533715724064)) ;
#162044=CARTESIAN_POINT('Ctrl Pts',(-4.96920025888408,-6.5489600764314,
-31.5645957747614)) ;
#162045=CARTESIAN_POINT('Ctrl Pts',(-4.97990192168176,-6.5496301025519,
-31.5699500759452)) ;
#162046=CARTESIAN_POINT('Ctrl Pts',(-4.99357116034316,-6.54996164986963,
-31.5767855738171)) ;
#162047=CARTESIAN_POINT('Ctrl Pts',(-4.99680282631924,-6.55,-31.5784014131596)) ;
#162048=CARTESIAN_POINT('Ctrl Pts',(-5.,-6.55,-31.58)) ;
#162049=CARTESIAN_POINT('',(-3.94142135623683,-6.52071067811842,-31.5092893218811)) ;
#162050=CARTESIAN_POINT('Ctrl Pts',(-3.8,-6.55,-31.58)) ;
#162051=CARTESIAN_POINT('Ctrl Pts',(-3.81016571653571,-6.55,-31.5749171417321)) ;
#162052=CARTESIAN_POINT('Ctrl Pts',(-3.82068315091917,-6.54961031187957,
-31.5696576838579)) ;
#162053=CARTESIAN_POINT('Ctrl Pts',(-3.84304266527945,-6.54783411578236,
-31.5584679497194)) ;
#162054=CARTESIAN_POINT('Ctrl Pts',(-3.85491327259759,-6.54635217950662,
-31.5525227617952)) ;
#162055=CARTESIAN_POINT('Ctrl Pts',(-3.87771616261546,-6.54231439116932,
-31.5411067603976)) ;
#162056=CARTESIAN_POINT('Ctrl Pts',(-3.88866251834317,-6.53982180675291,
-31.5356298613107)) ;
#162057=CARTESIAN_POINT('Ctrl Pts',(-3.90045005710841,-6.53645537933597,
-31.5297406960419)) ;
#162058=CARTESIAN_POINT('Ctrl Pts',(-3.90170928105035,-6.5360866534789,
-31.5291116827675)) ;
#162059=CARTESIAN_POINT('Ctrl Pts',(-3.9138807702658,-6.53243308776766,
-31.523032751352)) ;
#162060=CARTESIAN_POINT('Ctrl Pts',(-3.92429308263635,-6.5285996913975,
-31.5178422384292)) ;
#162061=CARTESIAN_POINT('Ctrl Pts',(-3.93645488997202,-6.52312881451524,
-31.5117711869642)) ;
#162062=CARTESIAN_POINT('Ctrl Pts',(-3.93897066587108,-6.52193602330131,
-31.510514667064)) ;
#162063=CARTESIAN_POINT('Ctrl Pts',(-3.94142135623683,-6.52071067811842,
-31.5092893218811)) ;
#162064=CARTESIAN_POINT('Origin',(-3.78571994569106,-6.44700925663902,-31.5871421042526)) ;
#162065=CARTESIAN_POINT('Origin',(-3.8,-6.45,-29.48)) ;
#162066=CARTESIAN_POINT('',(-3.87071067811865,-6.52071067811866,-29.5214213562373)) ;
#162067=CARTESIAN_POINT('Ctrl Pts',(-3.8,-6.55,-29.38)) ;
#162068=CARTESIAN_POINT('Ctrl Pts',(-3.80508285826792,-6.55,-29.3901657165359)) ;
#162069=CARTESIAN_POINT('Ctrl Pts',(-3.81034231614199,-6.54961031187958,
-29.4006831509195)) ;
#162070=CARTESIAN_POINT('Ctrl Pts',(-3.82153205028065,-6.54783411578235,
-29.4230426652804)) ;
#162071=CARTESIAN_POINT('Ctrl Pts',(-3.82747723820507,-6.54635217950656,
-29.4349132725989)) ;
#162072=CARTESIAN_POINT('Ctrl Pts',(-3.83889323960381,-6.5423143911688,
-29.4577161626192)) ;
#162073=CARTESIAN_POINT('Ctrl Pts',(-3.8443701386916,-6.53982180675183,
-29.4686625183489)) ;
#162074=CARTESIAN_POINT('Ctrl Pts',(-3.85025930396034,-6.53645537933464,
-29.480450057114)) ;
#162075=CARTESIAN_POINT('Ctrl Pts',(-3.8508883172338,-6.5360866534781,-29.4817092810541)) ;
#162076=CARTESIAN_POINT('Ctrl Pts',(-3.85696724864826,-6.53243308776744,
-29.4938807702674)) ;
#162077=CARTESIAN_POINT('Ctrl Pts',(-3.86215776157091,-6.52859969139737,
-29.5042930826376)) ;
#162078=CARTESIAN_POINT('Ctrl Pts',(-3.86822881303572,-6.5231288145153,
-29.5164548899728)) ;
#162079=CARTESIAN_POINT('Ctrl Pts',(-3.86948533293586,-6.52193602330145,
-29.5189706658717)) ;
#162080=CARTESIAN_POINT('Ctrl Pts',(-3.87071067811865,-6.52071067811866,
-29.5214213562373)) ;
#162081=CARTESIAN_POINT('Origin',(-3.7928578957674,-6.44700925664559,-29.3657199457331)) ;
#162082=CARTESIAN_POINT('',(-3.87071067811865,-6.52071067811866,-31.4385786437627)) ;
#162083=CARTESIAN_POINT('Origin',(-3.79291331463673,-6.44703459698258,-31.5941700950176)) ;
#162084=CARTESIAN_POINT('Ctrl Pts',(-3.87071067811865,-6.52071067811866,
-31.4385786437627)) ;
#162085=CARTESIAN_POINT('Ctrl Pts',(-3.86620460065363,-6.52521675558368,
-31.4475907986928)) ;
#162086=CARTESIAN_POINT('Ctrl Pts',(-3.86127351832835,-6.52928079264423,
-31.4574862581729)) ;
#162087=CARTESIAN_POINT('Ctrl Pts',(-3.85097911745211,-6.53624680748632,
-31.4781127705689)) ;
#162088=CARTESIAN_POINT('Ctrl Pts',(-3.84563601585071,-6.53918030781802,
-31.4888050943351)) ;
#162089=CARTESIAN_POINT('Ctrl Pts',(-3.83952524546698,-6.541859855003,-31.5010185932206)) ;
#162090=CARTESIAN_POINT('Ctrl Pts',(-3.83889029009095,-6.54213045061232,
-31.5022875172272)) ;
#162091=CARTESIAN_POINT('Ctrl Pts',(-3.832503710866,-6.54477467909831,-31.5150493700286)) ;
#162092=CARTESIAN_POINT('Ctrl Pts',(-3.82662842759373,-6.54657370273655,
-31.5267793642821)) ;
#162093=CARTESIAN_POINT('Ctrl Pts',(-3.81540422523867,-6.54896007643138,
-31.5492002588841)) ;
#162094=CARTESIAN_POINT('Ctrl Pts',(-3.81004992405483,-6.54963010255189,
-31.5599019216818)) ;
#162095=CARTESIAN_POINT('Ctrl Pts',(-3.80321442618285,-6.54996164986963,
-31.5735711603432)) ;
#162096=CARTESIAN_POINT('Ctrl Pts',(-3.80159858684036,-6.55,-31.5768028263193)) ;
#162097=CARTESIAN_POINT('Ctrl Pts',(-3.8,-6.55,-31.58)) ;
#162098=CARTESIAN_POINT('Origin',(-5.,-6.45,-29.48)) ;
#162099=CARTESIAN_POINT('',(-4.92928932188134,-6.52071067811866,-31.4385786437627)) ;
#162100=CARTESIAN_POINT('Ctrl Pts',(-5.,-6.55,-31.58)) ;
#162101=CARTESIAN_POINT('Ctrl Pts',(-4.99491714173205,-6.55,-31.5698342834641)) ;
#162102=CARTESIAN_POINT('Ctrl Pts',(-4.98965768385794,-6.54961031187957,
-31.5593168490804)) ;
#162103=CARTESIAN_POINT('Ctrl Pts',(-4.97846794971924,-6.54783411578233,
-31.5369573347195)) ;
#162104=CARTESIAN_POINT('Ctrl Pts',(-4.9725227617948,-6.54635217950652,
-31.5250867274009)) ;
#162105=CARTESIAN_POINT('Ctrl Pts',(-4.96110676039594,-6.54231439116871,
-31.5022838373803)) ;
#162106=CARTESIAN_POINT('Ctrl Pts',(-4.95562986130805,-6.53982180675167,
-31.4913374816505)) ;
#162107=CARTESIAN_POINT('Ctrl Pts',(-4.94974069603934,-6.53645537933445,
-31.4795499428854)) ;
#162108=CARTESIAN_POINT('Ctrl Pts',(-4.94911168276599,-6.53608665347797,
-31.4782907189456)) ;
#162109=CARTESIAN_POINT('Ctrl Pts',(-4.94303275135165,-6.53243308776738,
-31.4661192297325)) ;
#162110=CARTESIAN_POINT('Ctrl Pts',(-4.93784223842901,-6.52859969139731,
-31.4557069173623)) ;
#162111=CARTESIAN_POINT('Ctrl Pts',(-4.93177118696424,-6.52312881451526,
-31.4435451100271)) ;
#162112=CARTESIAN_POINT('Ctrl Pts',(-4.93051466706411,-6.52193602330142,
-31.4410293341282)) ;
#162113=CARTESIAN_POINT('Ctrl Pts',(-4.92928932188135,-6.52071067811866,
-31.4385786437627)) ;
#162114=CARTESIAN_POINT('Origin',(-5.0071421042338,-6.44700925664485,-31.5942800542696)) ;
#162115=CARTESIAN_POINT('',(-4.92928932188133,-6.52071067811864,-29.5214213562373)) ;
#162116=CARTESIAN_POINT('Origin',(-5.00708668536686,-6.44703459698117,-29.3658299049752)) ;
#162117=CARTESIAN_POINT('Ctrl Pts',(-4.92928932188133,-6.52071067811864,
-29.5214213562373)) ;
#162118=CARTESIAN_POINT('Ctrl Pts',(-4.93379539934636,-6.52521675558367,
-29.5124092013072)) ;
#162119=CARTESIAN_POINT('Ctrl Pts',(-4.93872648167164,-6.52928079264422,
-29.5025137418271)) ;
#162120=CARTESIAN_POINT('Ctrl Pts',(-4.94902088254797,-6.53624680748638,
-29.4818872294309)) ;
#162121=CARTESIAN_POINT('Ctrl Pts',(-4.95436398414947,-6.53918030781812,
-29.4711949056645)) ;
#162122=CARTESIAN_POINT('Ctrl Pts',(-4.9604747545332,-6.54185985500307,
-29.4589814067789)) ;
#162123=CARTESIAN_POINT('Ctrl Pts',(-4.96110970990912,-6.54213045061235,
-29.4577124827726)) ;
#162124=CARTESIAN_POINT('Ctrl Pts',(-4.96749628913392,-6.54477467909829,
-29.4449506299714)) ;
#162125=CARTESIAN_POINT('Ctrl Pts',(-4.97337157240617,-6.54657370273652,
-29.433220635718)) ;
#162126=CARTESIAN_POINT('Ctrl Pts',(-4.98459577476118,-6.54896007643136,
-29.4107997411161)) ;
#162127=CARTESIAN_POINT('Ctrl Pts',(-4.989950075945,-6.54963010255188,-29.4000980783185)) ;
#162128=CARTESIAN_POINT('Ctrl Pts',(-4.99678557381703,-6.54996164986962,
-29.386428839657)) ;
#162129=CARTESIAN_POINT('Ctrl Pts',(-4.99840141315957,-6.55,-29.3831971736808)) ;
#162130=CARTESIAN_POINT('Ctrl Pts',(-5.,-6.55,-29.38)) ;
#162131=CARTESIAN_POINT('Origin',(-4.9,-6.45,-29.38)) ;
#162132=CARTESIAN_POINT('',(-4.85857864376276,-6.52071067811862,-29.4507106781187)) ;
#162133=CARTESIAN_POINT('Ctrl Pts',(-5.,-6.55,-29.38)) ;
#162134=CARTESIAN_POINT('Ctrl Pts',(-4.98983428346421,-6.55,-29.3850828582679)) ;
#162135=CARTESIAN_POINT('Ctrl Pts',(-4.97931684908067,-6.54961031187958,
-29.390342316142)) ;
#162136=CARTESIAN_POINT('Ctrl Pts',(-4.95695733471996,-6.54783411578236,
-29.4015320502806)) ;
#162137=CARTESIAN_POINT('Ctrl Pts',(-4.94508672740148,-6.54635217950657,
-29.407477238205)) ;
#162138=CARTESIAN_POINT('Ctrl Pts',(-4.92228383737806,-6.54231439116827,
-29.4188932396053)) ;
#162139=CARTESIAN_POINT('Ctrl Pts',(-4.91133748164525,-6.53982180675044,
-29.4243701386947)) ;
#162140=CARTESIAN_POINT('Ctrl Pts',(-4.89954994288043,-6.53645537933293,
-29.4302593039633)) ;
#162141=CARTESIAN_POINT('Ctrl Pts',(-4.89829071894342,-6.53608665347727,
-29.4308883172352)) ;
#162142=CARTESIAN_POINT('Ctrl Pts',(-4.88611922973308,-6.53243308776751,
-29.4369672486482)) ;
#162143=CARTESIAN_POINT('Ctrl Pts',(-4.87570691736278,-6.52859969139747,
-29.4421577615708)) ;
#162144=CARTESIAN_POINT('Ctrl Pts',(-4.86354511002741,-6.52312881451534,
-29.4482288130357)) ;
#162145=CARTESIAN_POINT('Ctrl Pts',(-4.86102933412843,-6.52193602330143,
-29.4494853329359)) ;
#162146=CARTESIAN_POINT('Ctrl Pts',(-4.85857864376276,-6.52071067811861,
-29.4507106781187)) ;
#162147=CARTESIAN_POINT('Origin',(-5.01428005428586,-6.44700925664139,-29.3728578957581)) ;
#162148=CARTESIAN_POINT('',(-3.94142135623731,-6.52071067811866,-29.4507106781187)) ;
#162149=CARTESIAN_POINT('Origin',(-3.78582990494928,-6.44703459697472,-29.3729133146205)) ;
#162150=CARTESIAN_POINT('Ctrl Pts',(-3.94142135623731,-6.52071067811863,
-29.4507106781187)) ;
#162151=CARTESIAN_POINT('Ctrl Pts',(-3.93240920130726,-6.52521675558369,
-29.4462046006536)) ;
#162152=CARTESIAN_POINT('Ctrl Pts',(-3.92251374182714,-6.5292807926442,
-29.4412735183284)) ;
#162153=CARTESIAN_POINT('Ctrl Pts',(-3.90188722943347,-6.5362468074855,
-29.4309791174533)) ;
#162154=CARTESIAN_POINT('Ctrl Pts',(-3.89119490566987,-6.53918030781666,
-29.4256360158532)) ;
#162155=CARTESIAN_POINT('Ctrl Pts',(-3.87898140678443,-6.5418598550019,
-29.4195252454696)) ;
#162156=CARTESIAN_POINT('Ctrl Pts',(-3.8777124827754,-6.54213045061177,
-29.4188902900923)) ;
#162157=CARTESIAN_POINT('Ctrl Pts',(-3.86495062997147,-6.54477467909826,
-29.4125037108661)) ;
#162158=CARTESIAN_POINT('Ctrl Pts',(-3.85322063571804,-6.54657370273652,
-29.4066284275938)) ;
#162159=CARTESIAN_POINT('Ctrl Pts',(-3.83079974111613,-6.54896007643135,
-29.3954042252389)) ;
#162160=CARTESIAN_POINT('Ctrl Pts',(-3.82009807831852,-6.54963010255187,
-29.3900499240551)) ;
#162161=CARTESIAN_POINT('Ctrl Pts',(-3.80642883965707,-6.54996164986962,
-29.383214426183)) ;
#162162=CARTESIAN_POINT('Ctrl Pts',(-3.80319717368087,-6.55,-29.3815985868404)) ;
#162163=CARTESIAN_POINT('Ctrl Pts',(-3.8,-6.55,-29.38)) ;
#162164=CARTESIAN_POINT('Origin',(-4.9,-6.45,-27.77)) ;
#162165=CARTESIAN_POINT('',(-4.85857864376276,-6.52071067811862,-27.6992893218813)) ;
#162166=CARTESIAN_POINT('Origin',(-5.01417009503991,-6.4470345969778,-27.7770866853742)) ;
#162167=CARTESIAN_POINT('Ctrl Pts',(-4.85857864376276,-6.52071067811861,
-27.6992893218813)) ;
#162168=CARTESIAN_POINT('Ctrl Pts',(-4.86759079869284,-6.52521675558363,
-27.7037953993463)) ;
#162169=CARTESIAN_POINT('Ctrl Pts',(-4.877486258173,-6.52928079264421,-27.7087264816716)) ;
#162170=CARTESIAN_POINT('Ctrl Pts',(-4.89811277056682,-6.53624680748554,
-27.7190208825467)) ;
#162171=CARTESIAN_POINT('Ctrl Pts',(-4.90880509433053,-6.53918030781672,
-27.7243639841469)) ;
#162172=CARTESIAN_POINT('Ctrl Pts',(-4.92101859321596,-6.54185985500196,
-27.7304747545306)) ;
#162173=CARTESIAN_POINT('Ctrl Pts',(-4.92228751722488,-6.5421304506118,
-27.7311097099078)) ;
#162174=CARTESIAN_POINT('Ctrl Pts',(-4.93504937002862,-6.54477467909826,
-27.7374962891339)) ;
#162175=CARTESIAN_POINT('Ctrl Pts',(-4.94677936428197,-6.5465737027365,
-27.7433715724061)) ;
#162176=CARTESIAN_POINT('Ctrl Pts',(-4.96920025888377,-6.54896007643133,
-27.754595774761)) ;
#162177=CARTESIAN_POINT('Ctrl Pts',(-4.97990192168136,-6.54963010255186,
-27.7599500759448)) ;
#162178=CARTESIAN_POINT('Ctrl Pts',(-4.99357116034283,-6.54996164986962,
-27.766785573817)) ;
#162179=CARTESIAN_POINT('Ctrl Pts',(-4.99680282631908,-6.55,-27.7684014131595)) ;
#162180=CARTESIAN_POINT('Ctrl Pts',(-5.,-6.55,-27.77)) ;
#162181=CARTESIAN_POINT('',(-3.94142135623731,-6.52071067811866,-27.6992893218813)) ;
#162182=CARTESIAN_POINT('Ctrl Pts',(-3.8,-6.55,-27.77)) ;
#162183=CARTESIAN_POINT('Ctrl Pts',(-3.81016571653584,-6.55,-27.7649171417321)) ;
#162184=CARTESIAN_POINT('Ctrl Pts',(-3.82068315091945,-6.54961031187958,
-27.759657683858)) ;
#162185=CARTESIAN_POINT('Ctrl Pts',(-3.84304266528029,-6.54783411578235,
-27.7484679497193)) ;
#162186=CARTESIAN_POINT('Ctrl Pts',(-3.85491327259885,-6.54635217950657,
-27.742522761795)) ;
#162187=CARTESIAN_POINT('Ctrl Pts',(-3.87771616262343,-6.54231439116804,
-27.731106760394)) ;
#162188=CARTESIAN_POINT('Ctrl Pts',(-3.88866251835728,-6.53982180674991,
-27.7256298613042)) ;
#162189=CARTESIAN_POINT('Ctrl Pts',(-3.900450057122,-6.53645537933228,-27.7197406960356)) ;
#162190=CARTESIAN_POINT('Ctrl Pts',(-3.901709281058,-6.5360866534769,-27.7191116827642)) ;
#162191=CARTESIAN_POINT('Ctrl Pts',(-3.91388077026728,-6.53243308776744,
-27.7130327513517)) ;
#162192=CARTESIAN_POINT('Ctrl Pts',(-3.92429308263753,-6.5285996913974,
-27.7078422384291)) ;
#162193=CARTESIAN_POINT('Ctrl Pts',(-3.93645488997278,-6.52312881451533,
-27.7017711869643)) ;
#162194=CARTESIAN_POINT('Ctrl Pts',(-3.9389706658717,-6.52193602330143,
-27.7005146670641)) ;
#162195=CARTESIAN_POINT('Ctrl Pts',(-3.94142135623731,-6.52071067811863,
-27.6992893218813)) ;
#162196=CARTESIAN_POINT('Origin',(-3.78571994570707,-6.44700925663904,-27.7771421042453)) ;
#162197=CARTESIAN_POINT('Origin',(-3.8,-6.45,-25.67)) ;
#162198=CARTESIAN_POINT('',(-3.87071067811865,-6.52071067811866,-25.7114213562373)) ;
#162199=CARTESIAN_POINT('Ctrl Pts',(-3.8,-6.55,-25.57)) ;
#162200=CARTESIAN_POINT('Ctrl Pts',(-3.80508285826791,-6.55,-25.5801657165359)) ;
#162201=CARTESIAN_POINT('Ctrl Pts',(-3.81034231614198,-6.54961031187958,
-25.5906831509195)) ;
#162202=CARTESIAN_POINT('Ctrl Pts',(-3.82153205028064,-6.54783411578236,
-25.6130426652803)) ;
#162203=CARTESIAN_POINT('Ctrl Pts',(-3.82747723820505,-6.54635217950656,
-25.6249132725989)) ;
#162204=CARTESIAN_POINT('Ctrl Pts',(-3.83889323960423,-6.54231439116865,
-25.6477161626201)) ;
#162205=CARTESIAN_POINT('Ctrl Pts',(-3.84437013869244,-6.53982180675145,
-25.6586625183506)) ;
#162206=CARTESIAN_POINT('Ctrl Pts',(-3.85025930396114,-6.53645537933417,
-25.6704500571156)) ;
#162207=CARTESIAN_POINT('Ctrl Pts',(-3.8508883172342,-6.53608665347786,
-25.6717092810549)) ;
#162208=CARTESIAN_POINT('Ctrl Pts',(-3.85696724864826,-6.53243308776744,
-25.6838807702674)) ;
#162209=CARTESIAN_POINT('Ctrl Pts',(-3.86215776157091,-6.52859969139737,
-25.6942930826377)) ;
#162210=CARTESIAN_POINT('Ctrl Pts',(-3.86822881303572,-6.5231288145153,
-25.7064548899729)) ;
#162211=CARTESIAN_POINT('Ctrl Pts',(-3.86948533293586,-6.52193602330144,
-25.7089706658717)) ;
#162212=CARTESIAN_POINT('Ctrl Pts',(-3.87071067811865,-6.52071067811866,
-25.7114213562373)) ;
#162213=CARTESIAN_POINT('Origin',(-3.79285789576216,-6.44700925664358,-25.5557199457226)) ;
#162214=CARTESIAN_POINT('',(-3.87071067811865,-6.52071067811866,-27.6285786437627)) ;
#162215=CARTESIAN_POINT('Origin',(-3.79291331463346,-6.4470345969815,-27.7841700950241)) ;
#162216=CARTESIAN_POINT('Ctrl Pts',(-3.87071067811865,-6.52071067811866,
-27.6285786437627)) ;
#162217=CARTESIAN_POINT('Ctrl Pts',(-3.86620460065363,-6.52521675558368,
-27.6375907986927)) ;
#162218=CARTESIAN_POINT('Ctrl Pts',(-3.86127351832835,-6.52928079264423,
-27.6474862581729)) ;
#162219=CARTESIAN_POINT('Ctrl Pts',(-3.85097911745203,-6.53624680748638,
-27.668112770569)) ;
#162220=CARTESIAN_POINT('Ctrl Pts',(-3.84563601585054,-6.53918030781812,
-27.6788050943354)) ;
#162221=CARTESIAN_POINT('Ctrl Pts',(-3.8395252454668,-6.54185985500308,
-27.6910185932209)) ;
#162222=CARTESIAN_POINT('Ctrl Pts',(-3.83889029009086,-6.54213045061235,
-27.6922875172273)) ;
#162223=CARTESIAN_POINT('Ctrl Pts',(-3.83250371086603,-6.5447746790983,
-27.7050493700285)) ;
#162224=CARTESIAN_POINT('Ctrl Pts',(-3.82662842759379,-6.54657370273653,
-27.716779364282)) ;
#162225=CARTESIAN_POINT('Ctrl Pts',(-3.81540422523878,-6.54896007643136,
-27.7392002588839)) ;
#162226=CARTESIAN_POINT('Ctrl Pts',(-3.81004992405496,-6.54963010255188,
-27.7499019216815)) ;
#162227=CARTESIAN_POINT('Ctrl Pts',(-3.80321442618296,-6.54996164986962,
-27.763571160343)) ;
#162228=CARTESIAN_POINT('Ctrl Pts',(-3.80159858684042,-6.55,-27.7668028263191)) ;
#162229=CARTESIAN_POINT('Ctrl Pts',(-3.8,-6.55,-27.77)) ;
#162230=CARTESIAN_POINT('Origin',(-5.,-6.45,-25.67)) ;
#162231=CARTESIAN_POINT('',(-4.92928932188133,-6.52071067811864,-27.6285786437627)) ;
#162232=CARTESIAN_POINT('Ctrl Pts',(-5.,-6.55,-27.77)) ;
#162233=CARTESIAN_POINT('Ctrl Pts',(-4.99491714173208,-6.55,-27.7598342834642)) ;
#162234=CARTESIAN_POINT('Ctrl Pts',(-4.989657683858,-6.54961031187958,-27.7493168490806)) ;
#162235=CARTESIAN_POINT('Ctrl Pts',(-4.97846794971935,-6.54783411578236,
-27.7269573347198)) ;
#162236=CARTESIAN_POINT('Ctrl Pts',(-4.97252276179495,-6.54635217950656,
-27.7150867274012)) ;
#162237=CARTESIAN_POINT('Ctrl Pts',(-4.96110676039612,-6.54231439116878,
-27.6922838373808)) ;
#162238=CARTESIAN_POINT('Ctrl Pts',(-4.95562986130823,-6.53982180675176,
-27.6813374816509)) ;
#162239=CARTESIAN_POINT('Ctrl Pts',(-4.94974069603951,-6.53645537933455,
-27.6695499428858)) ;
#162240=CARTESIAN_POINT('Ctrl Pts',(-4.94911168276615,-6.53608665347807,
-27.6682907189459)) ;
#162241=CARTESIAN_POINT('Ctrl Pts',(-4.94303275135179,-6.53243308776748,
-27.6561192297328)) ;
#162242=CARTESIAN_POINT('Ctrl Pts',(-4.93784223842914,-6.52859969139742,
-27.6457069173625)) ;
#162243=CARTESIAN_POINT('Ctrl Pts',(-4.93177118696431,-6.52312881451532,
-27.6335451100273)) ;
#162244=CARTESIAN_POINT('Ctrl Pts',(-4.93051466706414,-6.52193602330145,
-27.6310293341283)) ;
#162245=CARTESIAN_POINT('Ctrl Pts',(-4.92928932188133,-6.52071067811864,
-27.6285786437627)) ;
#162246=CARTESIAN_POINT('Origin',(-5.00714210424853,-6.44700925663946,-27.7842800542989)) ;
#162247=CARTESIAN_POINT('',(-4.92928932188133,-6.52071067811864,-25.7114213562373)) ;
#162248=CARTESIAN_POINT('Origin',(-5.00708668536615,-6.44703459698157,-25.5558299049765)) ;
#162249=CARTESIAN_POINT('Ctrl Pts',(-4.92928932188133,-6.52071067811864,
-25.7114213562373)) ;
#162250=CARTESIAN_POINT('Ctrl Pts',(-4.93379539934636,-6.52521675558367,
-25.7024092013072)) ;
#162251=CARTESIAN_POINT('Ctrl Pts',(-4.93872648167164,-6.52928079264422,
-25.6925137418271)) ;
#162252=CARTESIAN_POINT('Ctrl Pts',(-4.9490208825476,-6.53624680748613,
-25.6718872294316)) ;
#162253=CARTESIAN_POINT('Ctrl Pts',(-4.95436398414871,-6.53918030781771,
-25.661194905666)) ;
#162254=CARTESIAN_POINT('Ctrl Pts',(-4.96047475453242,-6.54185985500274,
-25.6489814067805)) ;
#162255=CARTESIAN_POINT('Ctrl Pts',(-4.96110970990874,-6.54213045061219,
-25.6477124827734)) ;
#162256=CARTESIAN_POINT('Ctrl Pts',(-4.96749628913393,-6.54477467909829,
-25.6349506299714)) ;
#162257=CARTESIAN_POINT('Ctrl Pts',(-4.97337157240618,-6.54657370273652,
-25.623220635718)) ;
#162258=CARTESIAN_POINT('Ctrl Pts',(-4.98459577476119,-6.54896007643136,
-25.6007997411161)) ;
#162259=CARTESIAN_POINT('Ctrl Pts',(-4.98995007594501,-6.54963010255188,
-25.5900980783184)) ;
#162260=CARTESIAN_POINT('Ctrl Pts',(-4.99678557381703,-6.54996164986962,
-25.576428839657)) ;
#162261=CARTESIAN_POINT('Ctrl Pts',(-4.99840141315958,-6.55,-25.5731971736808)) ;
#162262=CARTESIAN_POINT('Ctrl Pts',(-5.,-6.55,-25.57)) ;
#162263=CARTESIAN_POINT('Origin',(-4.9,-6.45,-25.57)) ;
#162264=CARTESIAN_POINT('',(-4.85857864376276,-6.52071067811862,-25.6407106781187)) ;
#162265=CARTESIAN_POINT('Ctrl Pts',(-5.,-6.55,-25.57)) ;
#162266=CARTESIAN_POINT('Ctrl Pts',(-4.9898342834642,-6.55,-25.5750828582679)) ;
#162267=CARTESIAN_POINT('Ctrl Pts',(-4.97931684908064,-6.54961031187958,
-25.580342316142)) ;
#162268=CARTESIAN_POINT('Ctrl Pts',(-4.95695733471992,-6.54783411578236,
-25.5915320502806)) ;
#162269=CARTESIAN_POINT('Ctrl Pts',(-4.94508672740143,-6.54635217950657,
-25.597477238205)) ;
#162270=CARTESIAN_POINT('Ctrl Pts',(-4.92228383737812,-6.54231439116829,
-25.6088932396053)) ;
#162271=CARTESIAN_POINT('Ctrl Pts',(-4.91133748164544,-6.5398218067505,
-25.6143701386945)) ;
#162272=CARTESIAN_POINT('Ctrl Pts',(-4.89954994288061,-6.536455379333,-25.6202593039631)) ;
#162273=CARTESIAN_POINT('Ctrl Pts',(-4.89829071894348,-6.5360866534773,
-25.6208883172351)) ;
#162274=CARTESIAN_POINT('Ctrl Pts',(-4.88611922973303,-6.53243308776751,
-25.6269672486482)) ;
#162275=CARTESIAN_POINT('Ctrl Pts',(-4.87570691736273,-6.52859969139746,
-25.6321577615708)) ;
#162276=CARTESIAN_POINT('Ctrl Pts',(-4.86354511002739,-6.52312881451533,
-25.6382288130357)) ;
#162277=CARTESIAN_POINT('Ctrl Pts',(-4.86102933412842,-6.52193602330143,
-25.6394853329359)) ;
#162278=CARTESIAN_POINT('Ctrl Pts',(-4.85857864376276,-6.52071067811862,
-25.6407106781187)) ;
#162279=CARTESIAN_POINT('Origin',(-5.01428005427684,-6.44700925664322,-25.5628578957626)) ;
#162280=CARTESIAN_POINT('',(-3.94142135623731,-6.52071067811866,-25.6407106781187)) ;
#162281=CARTESIAN_POINT('Origin',(-3.78582990495265,-6.44703459697566,-25.5629133146221)) ;
#162282=CARTESIAN_POINT('Ctrl Pts',(-3.94142135623731,-6.52071067811864,
-25.6407106781187)) ;
#162283=CARTESIAN_POINT('Ctrl Pts',(-3.93240920130726,-6.52521675558369,
-25.6362046006536)) ;
#162284=CARTESIAN_POINT('Ctrl Pts',(-3.92251374182714,-6.52928079264421,
-25.6312735183284)) ;
#162285=CARTESIAN_POINT('Ctrl Pts',(-3.90188722943356,-6.53624680748547,
-25.6209791174534)) ;
#162286=CARTESIAN_POINT('Ctrl Pts',(-3.89119490567006,-6.53918030781661,
-25.6156360158533)) ;
#162287=CARTESIAN_POINT('Ctrl Pts',(-3.87898140678463,-6.54185985500186,
-25.6095252454697)) ;
#162288=CARTESIAN_POINT('Ctrl Pts',(-3.8777124827755,-6.54213045061175,
-25.6088902900923)) ;
#162289=CARTESIAN_POINT('Ctrl Pts',(-3.86495062997148,-6.54477467909826,
-25.6025037108661)) ;
#162290=CARTESIAN_POINT('Ctrl Pts',(-3.85322063571806,-6.54657370273652,
-25.5966284275938)) ;
#162291=CARTESIAN_POINT('Ctrl Pts',(-3.83079974111614,-6.54896007643135,
-25.5854042252389)) ;
#162292=CARTESIAN_POINT('Ctrl Pts',(-3.82009807831852,-6.54963010255187,
-25.5800499240551)) ;
#162293=CARTESIAN_POINT('Ctrl Pts',(-3.80642883965707,-6.54996164986963,
-25.573214426183)) ;
#162294=CARTESIAN_POINT('Ctrl Pts',(-3.80319717368087,-6.55,-25.5715985868404)) ;
#162295=CARTESIAN_POINT('Ctrl Pts',(-3.8,-6.55,-25.57)) ;
#162296=CARTESIAN_POINT('Origin',(-4.9,-6.45,-23.96)) ;
#162297=CARTESIAN_POINT('',(-4.85857864376276,-6.52071067811862,-23.8892893218813)) ;
#162298=CARTESIAN_POINT('Origin',(-5.01417009504266,-6.44703459697728,-23.9670866853756)) ;
#162299=CARTESIAN_POINT('Ctrl Pts',(-4.85857864376276,-6.52071067811861,
-23.8892893218813)) ;
#162300=CARTESIAN_POINT('Ctrl Pts',(-4.86759079869285,-6.52521675558364,
-23.8937953993463)) ;
#162301=CARTESIAN_POINT('Ctrl Pts',(-4.87748625817302,-6.52928079264421,
-23.8987264816716)) ;
#162302=CARTESIAN_POINT('Ctrl Pts',(-4.8981127705669,-6.53624680748557,
-23.9090208825468)) ;
#162303=CARTESIAN_POINT('Ctrl Pts',(-4.90880509433068,-6.53918030781676,
-23.914363984147)) ;
#162304=CARTESIAN_POINT('Ctrl Pts',(-4.92101859321611,-6.54185985500198,
-23.9204747545306)) ;
#162305=CARTESIAN_POINT('Ctrl Pts',(-4.92228751722495,-6.54213045061181,
-23.9211097099078)) ;
#162306=CARTESIAN_POINT('Ctrl Pts',(-4.93504937002862,-6.54477467909826,
-23.9274962891339)) ;
#162307=CARTESIAN_POINT('Ctrl Pts',(-4.94677936428196,-6.5465737027365,
-23.9333715724061)) ;
#162308=CARTESIAN_POINT('Ctrl Pts',(-4.96920025888376,-6.54896007643133,
-23.944595774761)) ;
#162309=CARTESIAN_POINT('Ctrl Pts',(-4.97990192168134,-6.54963010255186,
-23.9499500759448)) ;
#162310=CARTESIAN_POINT('Ctrl Pts',(-4.99357116034282,-6.54996164986962,
-23.9567855738169)) ;
#162311=CARTESIAN_POINT('Ctrl Pts',(-4.99680282631907,-6.55,-23.9584014131595)) ;
#162312=CARTESIAN_POINT('Ctrl Pts',(-5.,-6.55,-23.96)) ;
#162313=CARTESIAN_POINT('',(-3.94142135623731,-6.52071067811866,-23.8892893218813)) ;
#162314=CARTESIAN_POINT('Ctrl Pts',(-3.8,-6.55,-23.96)) ;
#162315=CARTESIAN_POINT('Ctrl Pts',(-3.81016571653584,-6.55,-23.9549171417321)) ;
#162316=CARTESIAN_POINT('Ctrl Pts',(-3.82068315091944,-6.54961031187958,
-23.949657683858)) ;
#162317=CARTESIAN_POINT('Ctrl Pts',(-3.84304266528028,-6.54783411578234,
-23.9384679497193)) ;
#162318=CARTESIAN_POINT('Ctrl Pts',(-3.85491327259884,-6.54635217950657,
-23.932522761795)) ;
#162319=CARTESIAN_POINT('Ctrl Pts',(-3.87771616262351,-6.54231439116802,
-23.921106760394)) ;
#162320=CARTESIAN_POINT('Ctrl Pts',(-3.88866251835745,-6.53982180674987,
-23.9156298613041)) ;
#162321=CARTESIAN_POINT('Ctrl Pts',(-3.90045005712217,-6.53645537933222,
-23.9097406960355)) ;
#162322=CARTESIAN_POINT('Ctrl Pts',(-3.90170928105808,-6.53608665347687,
-23.9091116827642)) ;
#162323=CARTESIAN_POINT('Ctrl Pts',(-3.91388077026727,-6.53243308776744,
-23.9030327513517)) ;
#162324=CARTESIAN_POINT('Ctrl Pts',(-3.92429308263752,-6.5285996913974,
-23.8978422384291)) ;
#162325=CARTESIAN_POINT('Ctrl Pts',(-3.93645488997277,-6.52312881451532,
-23.8917711869643)) ;
#162326=CARTESIAN_POINT('Ctrl Pts',(-3.93897066587169,-6.52193602330143,
-23.8905146670641)) ;
#162327=CARTESIAN_POINT('Ctrl Pts',(-3.94142135623731,-6.52071067811863,
-23.8892893218813)) ;
#162328=CARTESIAN_POINT('Origin',(-3.78571994570344,-6.44700925663849,-23.9671421042471)) ;
#162329=CARTESIAN_POINT('Origin',(-3.8,-6.45,-21.86)) ;
#162330=CARTESIAN_POINT('',(-3.87071067811865,-6.52071067811866,-21.9014213562373)) ;
#162331=CARTESIAN_POINT('Ctrl Pts',(-3.8,-6.55,-21.76)) ;
#162332=CARTESIAN_POINT('Ctrl Pts',(-3.80508285826791,-6.55,-21.7701657165358)) ;
#162333=CARTESIAN_POINT('Ctrl Pts',(-3.81034231614198,-6.54961031187958,
-21.7806831509195)) ;
#162334=CARTESIAN_POINT('Ctrl Pts',(-3.82153205028064,-6.54783411578236,
-21.8030426652803)) ;
#162335=CARTESIAN_POINT('Ctrl Pts',(-3.82747723820505,-6.54635217950656,
-21.8149132725989)) ;
#162336=CARTESIAN_POINT('Ctrl Pts',(-3.83889323960399,-6.54231439116874,
-21.8377161626196)) ;
#162337=CARTESIAN_POINT('Ctrl Pts',(-3.84437013869197,-6.53982180675166,
-21.8486625183496)) ;
#162338=CARTESIAN_POINT('Ctrl Pts',(-3.8502593039607,-6.53645537933443,
-21.8604500571147)) ;
#162339=CARTESIAN_POINT('Ctrl Pts',(-3.85088831723398,-6.53608665347799,
-21.8617092810544)) ;
#162340=CARTESIAN_POINT('Ctrl Pts',(-3.85696724864826,-6.53243308776744,
-21.8738807702674)) ;
#162341=CARTESIAN_POINT('Ctrl Pts',(-3.86215776157091,-6.52859969139738,
-21.8842930826377)) ;
#162342=CARTESIAN_POINT('Ctrl Pts',(-3.86822881303572,-6.5231288145153,
-21.8964548899729)) ;
#162343=CARTESIAN_POINT('Ctrl Pts',(-3.86948533293587,-6.52193602330144,
-21.8989706658717)) ;
#162344=CARTESIAN_POINT('Ctrl Pts',(-3.87071067811865,-6.52071067811866,
-21.9014213562373)) ;
#162345=CARTESIAN_POINT('Origin',(-3.79285789575771,-6.44700925664161,-21.7457199457137)) ;
#162346=CARTESIAN_POINT('',(-3.87071067811865,-6.52071067811866,-23.8185786437627)) ;
#162347=CARTESIAN_POINT('Origin',(-3.79291331460805,-6.44703459697049,-23.9741700950758)) ;
#162348=CARTESIAN_POINT('Ctrl Pts',(-3.87071067811865,-6.52071067811866,
-23.8185786437627)) ;
#162349=CARTESIAN_POINT('Ctrl Pts',(-3.86620460065363,-6.52521675558368,
-23.8275907986927)) ;
#162350=CARTESIAN_POINT('Ctrl Pts',(-3.86127351832836,-6.52928079264422,
-23.8374862581728)) ;
#162351=CARTESIAN_POINT('Ctrl Pts',(-3.85097911745241,-6.53624680748612,
-23.8581127705683)) ;
#162352=CARTESIAN_POINT('Ctrl Pts',(-3.84563601585132,-6.53918030781769,
-23.8688050943338)) ;
#162353=CARTESIAN_POINT('Ctrl Pts',(-3.8395252454676,-6.54185985500273,
-23.8810185932193)) ;
#162354=CARTESIAN_POINT('Ctrl Pts',(-3.83889029009126,-6.54213045061219,
-23.8822875172265)) ;
#162355=CARTESIAN_POINT('Ctrl Pts',(-3.83250371086603,-6.5447746790983,
-23.8950493700285)) ;
#162356=CARTESIAN_POINT('Ctrl Pts',(-3.82662842759379,-6.54657370273653,
-23.906779364282)) ;
#162357=CARTESIAN_POINT('Ctrl Pts',(-3.81540422523878,-6.54896007643136,
-23.9292002588839)) ;
#162358=CARTESIAN_POINT('Ctrl Pts',(-3.81004992405496,-6.54963010255188,
-23.9399019216815)) ;
#162359=CARTESIAN_POINT('Ctrl Pts',(-3.80321442618295,-6.54996164986962,
-23.953571160343)) ;
#162360=CARTESIAN_POINT('Ctrl Pts',(-3.80159858684042,-6.55,-23.9568028263192)) ;
#162361=CARTESIAN_POINT('Ctrl Pts',(-3.8,-6.55,-23.96)) ;
#162362=CARTESIAN_POINT('Origin',(-5.,-6.45,-21.86)) ;
#162363=CARTESIAN_POINT('',(-4.92928932188133,-6.52071067811864,-23.8185786437627)) ;
#162364=CARTESIAN_POINT('Ctrl Pts',(-5.,-6.55,-23.96)) ;
#162365=CARTESIAN_POINT('Ctrl Pts',(-4.99491714173208,-6.55,-23.9498342834642)) ;
#162366=CARTESIAN_POINT('Ctrl Pts',(-4.989657683858,-6.54961031187958,-23.9393168490806)) ;
#162367=CARTESIAN_POINT('Ctrl Pts',(-4.97846794971936,-6.54783411578236,
-23.9169573347198)) ;
#162368=CARTESIAN_POINT('Ctrl Pts',(-4.97252276179495,-6.54635217950656,
-23.9050867274012)) ;
#162369=CARTESIAN_POINT('Ctrl Pts',(-4.96110676039623,-6.54231439116882,
-23.882283837381)) ;
#162370=CARTESIAN_POINT('Ctrl Pts',(-4.95562986130845,-6.53982180675186,
-23.8713374816513)) ;
#162371=CARTESIAN_POINT('Ctrl Pts',(-4.94974069603971,-6.53645537933467,
-23.8595499428862)) ;
#162372=CARTESIAN_POINT('Ctrl Pts',(-4.94911168276625,-6.53608665347813,
-23.8582907189461)) ;
#162373=CARTESIAN_POINT('Ctrl Pts',(-4.94303275135179,-6.53243308776748,
-23.8461192297328)) ;
#162374=CARTESIAN_POINT('Ctrl Pts',(-4.93784223842914,-6.52859969139742,
-23.8357069173625)) ;
#162375=CARTESIAN_POINT('Ctrl Pts',(-4.93177118696431,-6.52312881451533,
-23.8235451100273)) ;
#162376=CARTESIAN_POINT('Ctrl Pts',(-4.93051466706414,-6.52193602330145,
-23.8210293341283)) ;
#162377=CARTESIAN_POINT('Ctrl Pts',(-4.92928932188133,-6.52071067811864,
-23.8185786437627)) ;
#162378=CARTESIAN_POINT('Origin',(-5.00714210424667,-6.44700925664039,-23.9742800542952)) ;
#162379=CARTESIAN_POINT('',(-4.92928932188133,-6.52071067811864,-21.9014213562373)) ;
#162380=CARTESIAN_POINT('Origin',(-5.00708668537149,-6.44703459697967,-21.7458299049658)) ;
#162381=CARTESIAN_POINT('Ctrl Pts',(-4.92928932188133,-6.52071067811864,
-21.9014213562373)) ;
#162382=CARTESIAN_POINT('Ctrl Pts',(-4.93379539934636,-6.52521675558367,
-21.8924092013072)) ;
#162383=CARTESIAN_POINT('Ctrl Pts',(-4.93872648167163,-6.52928079264421,
-21.8825137418271)) ;
#162384=CARTESIAN_POINT('Ctrl Pts',(-4.94902088254783,-6.53624680748629,
-21.8618872294312)) ;
#162385=CARTESIAN_POINT('Ctrl Pts',(-4.9543639841492,-6.53918030781798,
-21.851194905665)) ;
#162386=CARTESIAN_POINT('Ctrl Pts',(-4.96047475453293,-6.54185985500296,
-21.8389814067794)) ;
#162387=CARTESIAN_POINT('Ctrl Pts',(-4.96110970990898,-6.54213045061229,
-21.8377124827729)) ;
#162388=CARTESIAN_POINT('Ctrl Pts',(-4.96749628913391,-6.54477467909828,
-21.8249506299714)) ;
#162389=CARTESIAN_POINT('Ctrl Pts',(-4.97337157240615,-6.54657370273652,
-21.813220635718)) ;
#162390=CARTESIAN_POINT('Ctrl Pts',(-4.98459577476116,-6.54896007643135,
-21.7907997411161)) ;
#162391=CARTESIAN_POINT('Ctrl Pts',(-4.98995007594499,-6.54963010255188,
-21.7800980783185)) ;
#162392=CARTESIAN_POINT('Ctrl Pts',(-4.99678557381703,-6.54996164986962,
-21.766428839657)) ;
#162393=CARTESIAN_POINT('Ctrl Pts',(-4.99840141315957,-6.55,-21.7631971736809)) ;
#162394=CARTESIAN_POINT('Ctrl Pts',(-5.,-6.55,-21.76)) ;
#162395=CARTESIAN_POINT('Origin',(-4.9,-6.45,-21.76)) ;
#162396=CARTESIAN_POINT('',(-4.85857864376276,-6.52071067811862,-21.8307106781187)) ;
#162397=CARTESIAN_POINT('Ctrl Pts',(-5.,-6.55,-21.76)) ;
#162398=CARTESIAN_POINT('Ctrl Pts',(-4.98983428346421,-6.55,-21.7650828582679)) ;
#162399=CARTESIAN_POINT('Ctrl Pts',(-4.97931684908065,-6.54961031187958,
-21.770342316142)) ;
#162400=CARTESIAN_POINT('Ctrl Pts',(-4.95695733471994,-6.54783411578236,
-21.7815320502806)) ;
#162401=CARTESIAN_POINT('Ctrl Pts',(-4.94508672740146,-6.54635217950657,
-21.787477238205)) ;
#162402=CARTESIAN_POINT('Ctrl Pts',(-4.92228383737779,-6.54231439116823,
-21.7988932396055)) ;
#162403=CARTESIAN_POINT('Ctrl Pts',(-4.91133748164475,-6.53982180675033,
-21.8043701386949)) ;
#162404=CARTESIAN_POINT('Ctrl Pts',(-4.89954994287995,-6.5364553793328,
-21.8102593039635)) ;
#162405=CARTESIAN_POINT('Ctrl Pts',(-4.89829071894318,-6.5360866534772,
-21.8108883172353)) ;
#162406=CARTESIAN_POINT('Ctrl Pts',(-4.88611922973306,-6.53243308776752,
-21.8169672486482)) ;
#162407=CARTESIAN_POINT('Ctrl Pts',(-4.87570691736276,-6.52859969139747,
-21.8221577615708)) ;
#162408=CARTESIAN_POINT('Ctrl Pts',(-4.86354511002741,-6.52312881451533,
-21.8282288130357)) ;
#162409=CARTESIAN_POINT('Ctrl Pts',(-4.86102933412843,-6.52193602330143,
-21.8294853329359)) ;
#162410=CARTESIAN_POINT('Ctrl Pts',(-4.85857864376276,-6.52071067811862,
-21.8307106781187)) ;
#162411=CARTESIAN_POINT('Origin',(-5.01428005428387,-6.44700925664178,-21.7528578957592)) ;
#162412=CARTESIAN_POINT('',(-3.94142135623731,-6.52071067811866,-21.8307106781187)) ;
#162413=CARTESIAN_POINT('Origin',(-3.7858299049486,-6.44703459697488,-21.7529133146201)) ;
#162414=CARTESIAN_POINT('Ctrl Pts',(-3.94142135623731,-6.52071067811864,
-21.8307106781187)) ;
#162415=CARTESIAN_POINT('Ctrl Pts',(-3.93240920130726,-6.52521675558369,
-21.8262046006536)) ;
#162416=CARTESIAN_POINT('Ctrl Pts',(-3.92251374182714,-6.52928079264421,
-21.8212735183284)) ;
#162417=CARTESIAN_POINT('Ctrl Pts',(-3.901887229432,-6.536246807486,-21.8109791174526)) ;
#162418=CARTESIAN_POINT('Ctrl Pts',(-3.89119490566676,-6.53918030781751,
-21.8056360158517)) ;
#162419=CARTESIAN_POINT('Ctrl Pts',(-3.87898140678124,-6.54185985500259,
-21.7995252454679)) ;
#162420=CARTESIAN_POINT('Ctrl Pts',(-3.8777124827738,-6.54213045061211,
-21.7988902900914)) ;
#162421=CARTESIAN_POINT('Ctrl Pts',(-3.86495062997147,-6.5447746790983,
-21.7925037108661)) ;
#162422=CARTESIAN_POINT('Ctrl Pts',(-3.85322063571804,-6.54657370273652,
-21.7866284275938)) ;
#162423=CARTESIAN_POINT('Ctrl Pts',(-3.83079974111613,-6.54896007643135,
-21.7754042252389)) ;
#162424=CARTESIAN_POINT('Ctrl Pts',(-3.82009807831852,-6.54963010255187,
-21.7700499240551)) ;
#162425=CARTESIAN_POINT('Ctrl Pts',(-3.80642883965707,-6.54996164986963,
-21.763214426183)) ;
#162426=CARTESIAN_POINT('Ctrl Pts',(-3.80319717368087,-6.55,-21.7615985868404)) ;
#162427=CARTESIAN_POINT('Ctrl Pts',(-3.8,-6.55,-21.76)) ;
#162428=CARTESIAN_POINT('Origin',(-4.9,-6.45,-20.15)) ;
#162429=CARTESIAN_POINT('',(-4.85857864376276,-6.52071067811862,-20.0792893218813)) ;
#162430=CARTESIAN_POINT('Origin',(-5.01417009505195,-6.44703459697568,-20.1570866853802)) ;
#162431=CARTESIAN_POINT('Ctrl Pts',(-4.85857864376276,-6.52071067811862,
-20.0792893218813)) ;
#162432=CARTESIAN_POINT('Ctrl Pts',(-4.86759079869283,-6.52521675558363,
-20.0837953993463)) ;
#162433=CARTESIAN_POINT('Ctrl Pts',(-4.87748625817297,-6.5292807926442,
-20.0887264816716)) ;
#162434=CARTESIAN_POINT('Ctrl Pts',(-4.89811277056717,-6.53624680748567,
-20.0990208825469)) ;
#162435=CARTESIAN_POINT('Ctrl Pts',(-4.90880509433133,-6.53918030781695,
-20.1043639841473)) ;
#162436=CARTESIAN_POINT('Ctrl Pts',(-4.92101859321678,-6.54185985500213,
-20.110474754531)) ;
#162437=CARTESIAN_POINT('Ctrl Pts',(-4.92228751722526,-6.54213045061188,
-20.111109709908)) ;
#162438=CARTESIAN_POINT('Ctrl Pts',(-4.93504937002857,-6.54477467909826,
-20.1174962891339)) ;
#162439=CARTESIAN_POINT('Ctrl Pts',(-4.94677936428192,-6.5465737027365,
-20.1233715724061)) ;
#162440=CARTESIAN_POINT('Ctrl Pts',(-4.96920025888373,-6.54896007643133,
-20.134595774761)) ;
#162441=CARTESIAN_POINT('Ctrl Pts',(-4.97990192168131,-6.54963010255186,
-20.1399500759448)) ;
#162442=CARTESIAN_POINT('Ctrl Pts',(-4.9935711603428,-6.54996164986962,
-20.1467855738169)) ;
#162443=CARTESIAN_POINT('Ctrl Pts',(-4.99680282631906,-6.55,-20.1484014131595)) ;
#162444=CARTESIAN_POINT('Ctrl Pts',(-5.,-6.55,-20.15)) ;
#162445=CARTESIAN_POINT('',(-3.94142135623731,-6.52071067811866,-20.0792893218813)) ;
#162446=CARTESIAN_POINT('Ctrl Pts',(-3.8,-6.55,-20.15)) ;
#162447=CARTESIAN_POINT('Ctrl Pts',(-3.81016571653584,-6.55,-20.1449171417321)) ;
#162448=CARTESIAN_POINT('Ctrl Pts',(-3.82068315091945,-6.54961031187958,
-20.139657683858)) ;
#162449=CARTESIAN_POINT('Ctrl Pts',(-3.84304266528029,-6.54783411578235,
-20.1284679497193)) ;
#162450=CARTESIAN_POINT('Ctrl Pts',(-3.85491327259885,-6.54635217950657,
-20.122522761795)) ;
#162451=CARTESIAN_POINT('Ctrl Pts',(-3.87771616262406,-6.54231439116792,
-20.1111067603937)) ;
#162452=CARTESIAN_POINT('Ctrl Pts',(-3.88866251835853,-6.53982180674963,
-20.1056298613036)) ;
#162453=CARTESIAN_POINT('Ctrl Pts',(-3.9004500571232,-6.53645537933192,
-20.099740696035)) ;
#162454=CARTESIAN_POINT('Ctrl Pts',(-3.90170928105859,-6.53608665347672,
-20.0991116827639)) ;
#162455=CARTESIAN_POINT('Ctrl Pts',(-3.91388077026728,-6.53243308776744,
-20.0930327513517)) ;
#162456=CARTESIAN_POINT('Ctrl Pts',(-3.92429308263753,-6.5285996913974,
-20.0878422384291)) ;
#162457=CARTESIAN_POINT('Ctrl Pts',(-3.93645488997278,-6.52312881451532,
-20.0817711869643)) ;
#162458=CARTESIAN_POINT('Ctrl Pts',(-3.9389706658717,-6.52193602330149,
-20.0805146670642)) ;
#162459=CARTESIAN_POINT('Ctrl Pts',(-3.94142135623731,-6.52071067811864,
-20.0792893218813)) ;
#162460=CARTESIAN_POINT('Origin',(-3.78571994570446,-6.44700925663872,-20.1571421042466)) ;
#162461=CARTESIAN_POINT('Origin',(-3.8,-6.45,-18.05)) ;
#162462=CARTESIAN_POINT('',(-3.87071067811865,-6.52071067811866,-18.0914213562373)) ;
#162463=CARTESIAN_POINT('Ctrl Pts',(-3.8,-6.55,-17.95)) ;
#162464=CARTESIAN_POINT('Ctrl Pts',(-3.80508285826791,-6.55,-17.9601657165359)) ;
#162465=CARTESIAN_POINT('Ctrl Pts',(-3.81034231614198,-6.54961031187958,
-17.9706831509195)) ;
#162466=CARTESIAN_POINT('Ctrl Pts',(-3.82153205028063,-6.54783411578236,
-17.9930426652803)) ;
#162467=CARTESIAN_POINT('Ctrl Pts',(-3.82747723820505,-6.54635217950656,
-18.0049132725989)) ;
#162468=CARTESIAN_POINT('Ctrl Pts',(-3.83889323960378,-6.54231439116881,
-18.0277161626192)) ;
#162469=CARTESIAN_POINT('Ctrl Pts',(-3.84437013869156,-6.53982180675185,
-18.0386625183488)) ;
#162470=CARTESIAN_POINT('Ctrl Pts',(-3.8502593039603,-6.53645537933466,
-18.0504500571139)) ;
#162471=CARTESIAN_POINT('Ctrl Pts',(-3.85088831723378,-6.53608665347812,
-18.051709281054)) ;
#162472=CARTESIAN_POINT('Ctrl Pts',(-3.85696724864825,-6.53243308776745,
-18.0638807702674)) ;
#162473=CARTESIAN_POINT('Ctrl Pts',(-3.86215776157091,-6.52859969139737,
-18.0742930826376)) ;
#162474=CARTESIAN_POINT('Ctrl Pts',(-3.86822881303572,-6.5231288145153,
-18.0864548899729)) ;
#162475=CARTESIAN_POINT('Ctrl Pts',(-3.86948533293586,-6.52193602330144,
-18.0889706658717)) ;
#162476=CARTESIAN_POINT('Ctrl Pts',(-3.87071067811865,-6.52071067811866,
-18.0914213562373)) ;
#162477=CARTESIAN_POINT('Origin',(-3.79285789576042,-6.44700925664281,-17.9357199457191)) ;
#162478=CARTESIAN_POINT('',(-3.87071067811865,-6.52071067811866,-20.0085786437627)) ;
#162479=CARTESIAN_POINT('Origin',(-3.79291331463951,-6.4470345969837,-20.164170095012)) ;
#162480=CARTESIAN_POINT('Ctrl Pts',(-3.87071067811865,-6.52071067811866,
-20.0085786437627)) ;
#162481=CARTESIAN_POINT('Ctrl Pts',(-3.86620460065363,-6.52521675558368,
-20.0175907986927)) ;
#162482=CARTESIAN_POINT('Ctrl Pts',(-3.86127351832835,-6.52928079264423,
-20.0274862581729)) ;
#162483=CARTESIAN_POINT('Ctrl Pts',(-3.85097911745214,-6.5362468074863,
-20.0481127705688)) ;
#162484=CARTESIAN_POINT('Ctrl Pts',(-3.84563601585077,-6.53918030781799,
-20.0588050943349)) ;
#162485=CARTESIAN_POINT('Ctrl Pts',(-3.83952524546704,-6.54185985500297,
-20.0710185932205)) ;
#162486=CARTESIAN_POINT('Ctrl Pts',(-3.83889029009097,-6.54213045061231,
-20.0722875172271)) ;
#162487=CARTESIAN_POINT('Ctrl Pts',(-3.83250371086602,-6.5447746790983,
-20.0850493700286)) ;
#162488=CARTESIAN_POINT('Ctrl Pts',(-3.82662842759378,-6.54657370273654,
-20.096779364282)) ;
#162489=CARTESIAN_POINT('Ctrl Pts',(-3.81540422523877,-6.54896007643136,
-20.1192002588839)) ;
#162490=CARTESIAN_POINT('Ctrl Pts',(-3.81004992405495,-6.54963010255188,
-20.1299019216816)) ;
#162491=CARTESIAN_POINT('Ctrl Pts',(-3.80321442618295,-6.54996164986962,
-20.143571160343)) ;
#162492=CARTESIAN_POINT('Ctrl Pts',(-3.80159858684041,-6.55,-20.1468028263192)) ;
#162493=CARTESIAN_POINT('Ctrl Pts',(-3.8,-6.55,-20.15)) ;
#162494=CARTESIAN_POINT('Origin',(-5.,-6.45,-18.05)) ;
#162495=CARTESIAN_POINT('',(-4.92928932188133,-6.52071067811864,-20.0085786437627)) ;
#162496=CARTESIAN_POINT('Ctrl Pts',(-5.,-6.55,-20.15)) ;
#162497=CARTESIAN_POINT('Ctrl Pts',(-4.99491714173208,-6.55,-20.1398342834642)) ;
#162498=CARTESIAN_POINT('Ctrl Pts',(-4.98965768385801,-6.54961031187958,
-20.1293168490806)) ;
#162499=CARTESIAN_POINT('Ctrl Pts',(-4.97846794971936,-6.54783411578236,
-20.1069573347198)) ;
#162500=CARTESIAN_POINT('Ctrl Pts',(-4.97252276179496,-6.54635217950657,
-20.0950867274012)) ;
#162501=CARTESIAN_POINT('Ctrl Pts',(-4.9611067603961,-6.54231439116877,
-20.0722838373807)) ;
#162502=CARTESIAN_POINT('Ctrl Pts',(-4.95562986130818,-6.53982180675173,
-20.0613374816508)) ;
#162503=CARTESIAN_POINT('Ctrl Pts',(-4.94974069603945,-6.53645537933452,
-20.0495499428857)) ;
#162504=CARTESIAN_POINT('Ctrl Pts',(-4.94911168276612,-6.53608665347806,
-20.0482907189459)) ;
#162505=CARTESIAN_POINT('Ctrl Pts',(-4.94303275135179,-6.53243308776748,
-20.0361192297328)) ;
#162506=CARTESIAN_POINT('Ctrl Pts',(-4.93784223842913,-6.52859969139741,
-20.0257069173625)) ;
#162507=CARTESIAN_POINT('Ctrl Pts',(-4.9317711869643,-6.52312881451532,
-20.0135451100273)) ;
#162508=CARTESIAN_POINT('Ctrl Pts',(-4.93051466706414,-6.52193602330145,
-20.0110293341283)) ;
#162509=CARTESIAN_POINT('Ctrl Pts',(-4.92928932188133,-6.52071067811864,
-20.0085786437627)) ;
#162510=CARTESIAN_POINT('Origin',(-5.00714210424655,-6.44700925664027,-20.1642800542949)) ;
#162511=CARTESIAN_POINT('',(-4.92928932188133,-6.52071067811864,-18.0914213562373)) ;
#162512=CARTESIAN_POINT('Origin',(-5.00708668537412,-6.44703459697887,-17.9358299049606)) ;
#162513=CARTESIAN_POINT('Ctrl Pts',(-4.92928932188133,-6.52071067811864,
-18.0914213562373)) ;
#162514=CARTESIAN_POINT('Ctrl Pts',(-4.93379539934636,-6.52521675558368,
-18.0824092013072)) ;
#162515=CARTESIAN_POINT('Ctrl Pts',(-4.93872648167165,-6.52928079264423,
-18.0725137418271)) ;
#162516=CARTESIAN_POINT('Ctrl Pts',(-4.94902088254759,-6.53624680748613,
-18.0518872294316)) ;
#162517=CARTESIAN_POINT('Ctrl Pts',(-4.95436398414867,-6.53918030781768,
-18.0411949056661)) ;
#162518=CARTESIAN_POINT('Ctrl Pts',(-4.96047475453238,-6.54185985500273,
-18.0289814067806)) ;
#162519=CARTESIAN_POINT('Ctrl Pts',(-4.96110970990873,-6.54213045061218,
-18.0277124827734)) ;
#162520=CARTESIAN_POINT('Ctrl Pts',(-4.96749628913394,-6.54477467909829,
-18.0149506299714)) ;
#162521=CARTESIAN_POINT('Ctrl Pts',(-4.97337157240618,-6.54657370273652,
-18.003220635718)) ;
#162522=CARTESIAN_POINT('Ctrl Pts',(-4.98459577476118,-6.54896007643136,
-17.9807997411161)) ;
#162523=CARTESIAN_POINT('Ctrl Pts',(-4.989950075945,-6.54963010255188,-17.9700980783185)) ;
#162524=CARTESIAN_POINT('Ctrl Pts',(-4.99678557381704,-6.54996164986962,
-17.956428839657)) ;
#162525=CARTESIAN_POINT('Ctrl Pts',(-4.99840141315957,-6.55,-17.9531971736809)) ;
#162526=CARTESIAN_POINT('Ctrl Pts',(-5.,-6.55,-17.95)) ;
#162527=CARTESIAN_POINT('Origin',(-4.9,-6.45,-17.95)) ;
#162528=CARTESIAN_POINT('',(-4.85857864376276,-6.52071067811862,-18.0207106781187)) ;
#162529=CARTESIAN_POINT('Ctrl Pts',(-5.,-6.55,-17.95)) ;
#162530=CARTESIAN_POINT('Ctrl Pts',(-4.98983428346421,-6.55,-17.9550828582679)) ;
#162531=CARTESIAN_POINT('Ctrl Pts',(-4.97931684908065,-6.54961031187958,
-17.960342316142)) ;
#162532=CARTESIAN_POINT('Ctrl Pts',(-4.95695733471993,-6.54783411578236,
-17.9715320502806)) ;
#162533=CARTESIAN_POINT('Ctrl Pts',(-4.94508672740146,-6.54635217950657,
-17.977477238205)) ;
#162534=CARTESIAN_POINT('Ctrl Pts',(-4.92228383737789,-6.54231439116824,
-17.9888932396054)) ;
#162535=CARTESIAN_POINT('Ctrl Pts',(-4.91133748164494,-6.53982180675038,
-17.9943701386948)) ;
#162536=CARTESIAN_POINT('Ctrl Pts',(-4.89954994288014,-6.53645537933285,
-18.0002593039634)) ;
#162537=CARTESIAN_POINT('Ctrl Pts',(-4.89829071894327,-6.53608665347723,
-18.0008883172352)) ;
#162538=CARTESIAN_POINT('Ctrl Pts',(-4.88611922973307,-6.53243308776751,
-18.0069672486482)) ;
#162539=CARTESIAN_POINT('Ctrl Pts',(-4.87570691736276,-6.52859969139747,
-18.0121577615708)) ;
#162540=CARTESIAN_POINT('Ctrl Pts',(-4.8635451100274,-6.52312881451533,
-18.0182288130357)) ;
#162541=CARTESIAN_POINT('Ctrl Pts',(-4.86102933412843,-6.52193602330143,
-18.0194853329359)) ;
#162542=CARTESIAN_POINT('Ctrl Pts',(-4.85857864376276,-6.52071067811861,
-18.0207106781187)) ;
#162543=CARTESIAN_POINT('Origin',(-5.01428005427931,-6.44700925664276,-17.9428578957614)) ;
#162544=CARTESIAN_POINT('',(-3.94142135623731,-6.52071067811866,-18.0207106781187)) ;
#162545=CARTESIAN_POINT('Origin',(-3.78582990494094,-6.44703459697309,-17.9429133146163)) ;
#162546=CARTESIAN_POINT('Ctrl Pts',(-3.94142135623731,-6.52071067811863,
-18.0207106781187)) ;
#162547=CARTESIAN_POINT('Ctrl Pts',(-3.93240920130726,-6.52521675558369,
-18.0162046006536)) ;
#162548=CARTESIAN_POINT('Ctrl Pts',(-3.92251374182714,-6.52928079264421,
-18.0112735183284)) ;
#162549=CARTESIAN_POINT('Ctrl Pts',(-3.90188722943185,-6.53624680748605,
-18.0009791174525)) ;
#162550=CARTESIAN_POINT('Ctrl Pts',(-3.89119490566645,-6.53918030781759,
-17.9956360158515)) ;
#162551=CARTESIAN_POINT('Ctrl Pts',(-3.87898140678092,-6.54185985500266,
-17.9895252454678)) ;
#162552=CARTESIAN_POINT('Ctrl Pts',(-3.87771248277363,-6.54213045061215,
-17.9888902900914)) ;
#162553=CARTESIAN_POINT('Ctrl Pts',(-3.86495062997146,-6.5447746790983,
-17.982503710866)) ;
#162554=CARTESIAN_POINT('Ctrl Pts',(-3.85322063571804,-6.54657370273652,
-17.9766284275938)) ;
#162555=CARTESIAN_POINT('Ctrl Pts',(-3.83079974111613,-6.54896007643134,
-17.9654042252389)) ;
#162556=CARTESIAN_POINT('Ctrl Pts',(-3.82009807831851,-6.54963010255187,
-17.9600499240551)) ;
#162557=CARTESIAN_POINT('Ctrl Pts',(-3.80642883965706,-6.54996164986962,
-17.953214426183)) ;
#162558=CARTESIAN_POINT('Ctrl Pts',(-3.80319717368087,-6.55,-17.9515985868404)) ;
#162559=CARTESIAN_POINT('Ctrl Pts',(-3.8,-6.55,-17.95)) ;
#162560=CARTESIAN_POINT('Origin',(-4.9,-6.45,-16.34)) ;
#162561=CARTESIAN_POINT('',(-4.85857864376276,-6.52071067811862,-16.2692893218813)) ;
#162562=CARTESIAN_POINT('Origin',(-5.01417009504985,-6.44703459697582,-16.3470866853791)) ;
#162563=CARTESIAN_POINT('Ctrl Pts',(-4.85857864376276,-6.52071067811861,
-16.2692893218813)) ;
#162564=CARTESIAN_POINT('Ctrl Pts',(-4.86759079869283,-6.52521675558363,
-16.2737953993463)) ;
#162565=CARTESIAN_POINT('Ctrl Pts',(-4.87748625817297,-6.5292807926442,
-16.2787264816716)) ;
#162566=CARTESIAN_POINT('Ctrl Pts',(-4.89811277056686,-6.53624680748557,
-16.2890208825468)) ;
#162567=CARTESIAN_POINT('Ctrl Pts',(-4.90880509433066,-6.53918030781677,
-16.294363984147)) ;
#162568=CARTESIAN_POINT('Ctrl Pts',(-4.92101859321609,-6.54185985500199,
-16.3004747545307)) ;
#162569=CARTESIAN_POINT('Ctrl Pts',(-4.92228751722491,-6.54213045061181,
-16.3011097099078)) ;
#162570=CARTESIAN_POINT('Ctrl Pts',(-4.93504937002856,-6.54477467909826,
-16.3074962891339)) ;
#162571=CARTESIAN_POINT('Ctrl Pts',(-4.94677936428192,-6.5465737027365,
-16.3133715724061)) ;
#162572=CARTESIAN_POINT('Ctrl Pts',(-4.96920025888373,-6.54896007643133,
-16.324595774761)) ;
#162573=CARTESIAN_POINT('Ctrl Pts',(-4.97990192168131,-6.54963010255186,
-16.3299500759448)) ;
#162574=CARTESIAN_POINT('Ctrl Pts',(-4.9935711603428,-6.54996164986962,
-16.3367855738169)) ;
#162575=CARTESIAN_POINT('Ctrl Pts',(-4.99680282631906,-6.55,-16.3384014131595)) ;
#162576=CARTESIAN_POINT('Ctrl Pts',(-5.,-6.55,-16.34)) ;
#162577=CARTESIAN_POINT('',(-3.94142135623731,-6.52071067811866,-16.2692893218813)) ;
#162578=CARTESIAN_POINT('Ctrl Pts',(-3.8,-6.55,-16.34)) ;
#162579=CARTESIAN_POINT('Ctrl Pts',(-3.81016571653584,-6.55,-16.3349171417321)) ;
#162580=CARTESIAN_POINT('Ctrl Pts',(-3.82068315091945,-6.54961031187958,
-16.329657683858)) ;
#162581=CARTESIAN_POINT('Ctrl Pts',(-3.84304266528029,-6.54783411578235,
-16.3184679497193)) ;
#162582=CARTESIAN_POINT('Ctrl Pts',(-3.85491327259885,-6.54635217950657,
-16.312522761795)) ;
#162583=CARTESIAN_POINT('Ctrl Pts',(-3.87771616262369,-6.54231439116799,
-16.3011067603939)) ;
#162584=CARTESIAN_POINT('Ctrl Pts',(-3.8886625183578,-6.53982180674979,
-16.2956298613039)) ;
#162585=CARTESIAN_POINT('Ctrl Pts',(-3.9004500571225,-6.53645537933213,
-16.2897406960354)) ;
#162586=CARTESIAN_POINT('Ctrl Pts',(-3.90170928105824,-6.53608665347683,
-16.2891116827641)) ;
#162587=CARTESIAN_POINT('Ctrl Pts',(-3.91388077026727,-6.53243308776745,
-16.2830327513517)) ;
#162588=CARTESIAN_POINT('Ctrl Pts',(-3.92429308263753,-6.5285996913974,
-16.2778422384291)) ;
#162589=CARTESIAN_POINT('Ctrl Pts',(-3.93645488997277,-6.52312881451532,
-16.2717711869643)) ;
#162590=CARTESIAN_POINT('Ctrl Pts',(-3.93897066587169,-6.52193602330143,
-16.2705146670641)) ;
#162591=CARTESIAN_POINT('Ctrl Pts',(-3.94142135623731,-6.52071067811863,
-16.2692893218813)) ;
#162592=CARTESIAN_POINT('Origin',(-3.78571994570709,-6.44700925663911,-16.3471421042453)) ;
#162593=CARTESIAN_POINT('Origin',(-3.8,-6.45,-14.24)) ;
#162594=CARTESIAN_POINT('',(-3.87071067811867,-6.52071067811863,-14.2814213562373)) ;
#162595=CARTESIAN_POINT('Ctrl Pts',(-3.8,-6.55,-14.14)) ;
#162596=CARTESIAN_POINT('Ctrl Pts',(-3.80508285826792,-6.55,-14.1501657165358)) ;
#162597=CARTESIAN_POINT('Ctrl Pts',(-3.810342316142,-6.54961031187958,-14.1606831509194)) ;
#162598=CARTESIAN_POINT('Ctrl Pts',(-3.82153205028064,-6.54783411578236,
-14.1830426652802)) ;
#162599=CARTESIAN_POINT('Ctrl Pts',(-3.82747723820505,-6.54635217950656,
-14.1949132725988)) ;
#162600=CARTESIAN_POINT('Ctrl Pts',(-3.8388932396039,-6.54231439116878,
-14.2177161626193)) ;
#162601=CARTESIAN_POINT('Ctrl Pts',(-3.84437013869181,-6.53982180675174,
-14.2286625183492)) ;
#162602=CARTESIAN_POINT('Ctrl Pts',(-3.85025930396054,-6.53645537933452,
-14.2404500571143)) ;
#162603=CARTESIAN_POINT('Ctrl Pts',(-3.85088831723387,-6.53608665347806,
-14.2417092810541)) ;
#162604=CARTESIAN_POINT('Ctrl Pts',(-3.85696724864822,-6.53243308776747,
-14.2538807702672)) ;
#162605=CARTESIAN_POINT('Ctrl Pts',(-3.86215776157089,-6.5285996913974,
-14.2642930826375)) ;
#162606=CARTESIAN_POINT('Ctrl Pts',(-3.86822881303571,-6.52312881451531,
-14.2764548899728)) ;
#162607=CARTESIAN_POINT('Ctrl Pts',(-3.86948533293587,-6.52193602330144,
-14.2789706658717)) ;
#162608=CARTESIAN_POINT('Ctrl Pts',(-3.87071067811867,-6.52071067811864,
-14.2814213562373)) ;
#162609=CARTESIAN_POINT('Origin',(-3.7928578957324,-6.44700925663102,-14.1257199456631)) ;
#162610=CARTESIAN_POINT('',(-3.87071067811865,-6.52071067811866,-16.1985786437627)) ;
#162611=CARTESIAN_POINT('Origin',(-3.79291331463642,-6.44703459698195,-16.3541700950182)) ;
#162612=CARTESIAN_POINT('Ctrl Pts',(-3.87071067811865,-6.52071067811866,
-16.1985786437627)) ;
#162613=CARTESIAN_POINT('Ctrl Pts',(-3.86620460065363,-6.52521675558368,
-16.2075907986927)) ;
#162614=CARTESIAN_POINT('Ctrl Pts',(-3.86127351832835,-6.52928079264423,
-16.2174862581729)) ;
#162615=CARTESIAN_POINT('Ctrl Pts',(-3.85097911745215,-6.53624680748629,
-16.2381127705688)) ;
#162616=CARTESIAN_POINT('Ctrl Pts',(-3.8456360158508,-6.53918030781797,
-16.2488050943348)) ;
#162617=CARTESIAN_POINT('Ctrl Pts',(-3.83952524546706,-6.54185985500296,
-16.2610185932204)) ;
#162618=CARTESIAN_POINT('Ctrl Pts',(-3.83889029009099,-6.5421304506123,
-16.262287517227)) ;
#162619=CARTESIAN_POINT('Ctrl Pts',(-3.83250371086603,-6.5447746790983,
-16.2750493700286)) ;
#162620=CARTESIAN_POINT('Ctrl Pts',(-3.82662842759378,-6.54657370273654,
-16.286779364282)) ;
#162621=CARTESIAN_POINT('Ctrl Pts',(-3.81540422523877,-6.54896007643136,
-16.3092002588839)) ;
#162622=CARTESIAN_POINT('Ctrl Pts',(-3.81004992405495,-6.54963010255188,
-16.3199019216816)) ;
#162623=CARTESIAN_POINT('Ctrl Pts',(-3.80321442618295,-6.54996164986963,
-16.333571160343)) ;
#162624=CARTESIAN_POINT('Ctrl Pts',(-3.80159858684041,-6.55,-16.3368028263192)) ;
#162625=CARTESIAN_POINT('Ctrl Pts',(-3.8,-6.55,-16.34)) ;
#162626=CARTESIAN_POINT('Origin',(-5.,-6.45,-14.24)) ;
#162627=CARTESIAN_POINT('',(-4.92928932188133,-6.52071067811864,-16.1985786437627)) ;
#162628=CARTESIAN_POINT('Ctrl Pts',(-5.,-6.55,-16.34)) ;
#162629=CARTESIAN_POINT('Ctrl Pts',(-4.99491714173208,-6.55,-16.3298342834642)) ;
#162630=CARTESIAN_POINT('Ctrl Pts',(-4.989657683858,-6.54961031187958,-16.3193168490806)) ;
#162631=CARTESIAN_POINT('Ctrl Pts',(-4.97846794971935,-6.54783411578236,
-16.2969573347197)) ;
#162632=CARTESIAN_POINT('Ctrl Pts',(-4.97252276179495,-6.54635217950656,
-16.2850867274012)) ;
#162633=CARTESIAN_POINT('Ctrl Pts',(-4.96110676039589,-6.5423143911687,
-16.2622838373803)) ;
#162634=CARTESIAN_POINT('Ctrl Pts',(-4.95562986130779,-6.53982180675155,
-16.25133748165)) ;
#162635=CARTESIAN_POINT('Ctrl Pts',(-4.94974069603908,-6.5364553793343,
-16.239549942885)) ;
#162636=CARTESIAN_POINT('Ctrl Pts',(-4.94911168276594,-6.53608665347795,
-16.2382907189455)) ;
#162637=CARTESIAN_POINT('Ctrl Pts',(-4.94303275135179,-6.53243308776748,
-16.2261192297328)) ;
#162638=CARTESIAN_POINT('Ctrl Pts',(-4.93784223842914,-6.52859969139742,
-16.2157069173625)) ;
#162639=CARTESIAN_POINT('Ctrl Pts',(-4.93177118696431,-6.52312881451533,
-16.2035451100273)) ;
#162640=CARTESIAN_POINT('Ctrl Pts',(-4.93051466706414,-6.52193602330145,
-16.2010293341283)) ;
#162641=CARTESIAN_POINT('Ctrl Pts',(-4.92928932188133,-6.52071067811864,
-16.1985786437627)) ;
#162642=CARTESIAN_POINT('Origin',(-5.0071421042461,-6.44700925664031,-16.354280054294)) ;
#162643=CARTESIAN_POINT('',(-4.9292893218813,-6.52071067811861,-14.2814213562372)) ;
#162644=CARTESIAN_POINT('Origin',(-5.00708668537856,-6.44703459697599,-14.1258299049512)) ;
#162645=CARTESIAN_POINT('Ctrl Pts',(-4.9292893218813,-6.52071067811861,
-14.2814213562372)) ;
#162646=CARTESIAN_POINT('Ctrl Pts',(-4.93379539934635,-6.52521675558366,
-14.2724092013071)) ;
#162647=CARTESIAN_POINT('Ctrl Pts',(-4.93872648167166,-6.52928079264424,
-14.2625137418269)) ;
#162648=CARTESIAN_POINT('Ctrl Pts',(-4.94902088254798,-6.53624680748638,
-14.2418872294307)) ;
#162649=CARTESIAN_POINT('Ctrl Pts',(-4.95436398414945,-6.53918030781811,
-14.2311949056644)) ;
#162650=CARTESIAN_POINT('Ctrl Pts',(-4.96047475453317,-6.54185985500306,
-14.2189814067788)) ;
#162651=CARTESIAN_POINT('Ctrl Pts',(-4.96110970990912,-6.54213045061234,
-14.2177124827724)) ;
#162652=CARTESIAN_POINT('Ctrl Pts',(-4.96749628913392,-6.54477467909828,
-14.2049506299712)) ;
#162653=CARTESIAN_POINT('Ctrl Pts',(-4.97337157240614,-6.54657370273651,
-14.1932206357179)) ;
#162654=CARTESIAN_POINT('Ctrl Pts',(-4.98459577476115,-6.54896007643135,
-14.170799741116)) ;
#162655=CARTESIAN_POINT('Ctrl Pts',(-4.98995007594499,-6.54963010255188,
-14.1600980783184)) ;
#162656=CARTESIAN_POINT('Ctrl Pts',(-4.99678557381703,-6.54996164986962,
-14.146428839657)) ;
#162657=CARTESIAN_POINT('Ctrl Pts',(-4.99840141315957,-6.55,-14.1431971736808)) ;
#162658=CARTESIAN_POINT('Ctrl Pts',(-5.,-6.55,-14.14)) ;
#162659=CARTESIAN_POINT('Origin',(-4.9,-6.45,-14.14)) ;
#162660=CARTESIAN_POINT('',(-4.85857864376269,-6.52071067811866,-14.2107106781187)) ;
#162661=CARTESIAN_POINT('Ctrl Pts',(-5.,-6.55,-14.14)) ;
#162662=CARTESIAN_POINT('Ctrl Pts',(-4.98983428346412,-6.55,-14.1450828582679)) ;
#162663=CARTESIAN_POINT('Ctrl Pts',(-4.97931684908049,-6.54961031187958,
-14.150342316142)) ;
#162664=CARTESIAN_POINT('Ctrl Pts',(-4.95695733471958,-6.54783411578236,
-14.1615320502806)) ;
#162665=CARTESIAN_POINT('Ctrl Pts',(-4.94508672740099,-6.54635217950657,
-14.167477238205)) ;
#162666=CARTESIAN_POINT('Ctrl Pts',(-4.92228383738157,-6.54231439116896,
-14.1788932396034)) ;
#162667=CARTESIAN_POINT('Ctrl Pts',(-4.91133748165278,-6.53982180675222,
-14.1843701386908)) ;
#162668=CARTESIAN_POINT('Ctrl Pts',(-4.8995499428876,-6.53645537933512,
-14.1902593039595)) ;
#162669=CARTESIAN_POINT('Ctrl Pts',(-4.89829071894667,-6.53608665347833,
-14.1908883172334)) ;
#162670=CARTESIAN_POINT('Ctrl Pts',(-4.88611922973252,-6.53243308776743,
-14.1969672486483)) ;
#162671=CARTESIAN_POINT('Ctrl Pts',(-4.87570691736228,-6.52859969139738,
-14.2021577615709)) ;
#162672=CARTESIAN_POINT('Ctrl Pts',(-4.86354511002712,-6.5231288145153,
-14.2082288130357)) ;
#162673=CARTESIAN_POINT('Ctrl Pts',(-4.86102933412825,-6.52193602330142,
-14.2094853329359)) ;
#162674=CARTESIAN_POINT('Ctrl Pts',(-4.85857864376269,-6.52071067811863,
-14.2107106781187)) ;
#162675=CARTESIAN_POINT('Origin',(-5.01428005427037,-6.44700925664399,-14.1328578957658)) ;
#162676=CARTESIAN_POINT('',(-3.94142135623725,-6.52071067811863,-14.2107106781187)) ;
#162677=CARTESIAN_POINT('Origin',(-3.78582990492081,-6.44703459697004,-14.1329133146062)) ;
#162678=CARTESIAN_POINT('Ctrl Pts',(-3.94142135623725,-6.52071067811862,
-14.2107106781187)) ;
#162679=CARTESIAN_POINT('Ctrl Pts',(-3.93240920130718,-6.52521675558364,
-14.2062046006537)) ;
#162680=CARTESIAN_POINT('Ctrl Pts',(-3.92251374182704,-6.52928079264421,
-14.2012735183284)) ;
#162681=CARTESIAN_POINT('Ctrl Pts',(-3.90188722943303,-6.53624680748561,
-14.1909791174532)) ;
#162682=CARTESIAN_POINT('Ctrl Pts',(-3.89119490566909,-6.53918030781684,
-14.1856360158529)) ;
#162683=CARTESIAN_POINT('Ctrl Pts',(-3.87898140678365,-6.54185985500205,
-14.1795252454692)) ;
#162684=CARTESIAN_POINT('Ctrl Pts',(-3.87771248277495,-6.54213045061184,
-14.1788902900921)) ;
#162685=CARTESIAN_POINT('Ctrl Pts',(-3.8649506299714,-6.54477467909827,
-14.1725037108661)) ;
#162686=CARTESIAN_POINT('Ctrl Pts',(-3.85322063571803,-6.5465737027365,
-14.1666284275939)) ;
#162687=CARTESIAN_POINT('Ctrl Pts',(-3.83079974111618,-6.54896007643135,
-14.1554042252389)) ;
#162688=CARTESIAN_POINT('Ctrl Pts',(-3.82009807831857,-6.54963010255187,
-14.1500499240551)) ;
#162689=CARTESIAN_POINT('Ctrl Pts',(-3.80642883965711,-6.54996164986962,
-14.1432144261831)) ;
#162690=CARTESIAN_POINT('Ctrl Pts',(-3.80319717368089,-6.55,-14.1415985868405)) ;
#162691=CARTESIAN_POINT('Ctrl Pts',(-3.8,-6.55,-14.14)) ;
#162692=CARTESIAN_POINT('Origin',(-4.9,-6.45,-12.53)) ;
#162693=CARTESIAN_POINT('',(-4.85857864376269,-6.52071067811866,-12.4592893218813)) ;
#162694=CARTESIAN_POINT('Origin',(-5.01417009504273,-6.44703459697676,-12.5370866853755)) ;
#162695=CARTESIAN_POINT('Ctrl Pts',(-4.85857864376269,-6.52071067811863,
-12.4592893218813)) ;
#162696=CARTESIAN_POINT('Ctrl Pts',(-4.86759079869274,-6.5252167555837,
-12.4637953993464)) ;
#162697=CARTESIAN_POINT('Ctrl Pts',(-4.87748625817285,-6.52928079264422,
-12.4687264816716)) ;
#162698=CARTESIAN_POINT('Ctrl Pts',(-4.89811277056884,-6.53624680748634,
-12.4790208825479)) ;
#162699=CARTESIAN_POINT('Ctrl Pts',(-4.90880509433502,-6.53918030781804,
-12.4843639841493)) ;
#162700=CARTESIAN_POINT('Ctrl Pts',(-4.9210185932206,-6.54185985500302,
-12.4904747545331)) ;
#162701=CARTESIAN_POINT('Ctrl Pts',(-4.92228751722714,-6.54213045061234,
-12.4911097099091)) ;
#162702=CARTESIAN_POINT('Ctrl Pts',(-4.93504937002859,-6.54477467909833,
-12.4974962891341)) ;
#162703=CARTESIAN_POINT('Ctrl Pts',(-4.94677936428205,-6.54657370273655,
-12.5033715724063)) ;
#162704=CARTESIAN_POINT('Ctrl Pts',(-4.96920025888403,-6.54896007643138,
-12.5145957747613)) ;
#162705=CARTESIAN_POINT('Ctrl Pts',(-4.97990192168169,-6.54963010255189,
-12.5199500759451)) ;
#162706=CARTESIAN_POINT('Ctrl Pts',(-4.99357116034309,-6.54996164986963,
-12.5267855738171)) ;
#162707=CARTESIAN_POINT('Ctrl Pts',(-4.99680282631921,-6.55,-12.5284014131596)) ;
#162708=CARTESIAN_POINT('Ctrl Pts',(-5.,-6.55,-12.53)) ;
#162709=CARTESIAN_POINT('',(-3.94142135623725,-6.52071067811863,-12.4592893218813)) ;
#162710=CARTESIAN_POINT('Ctrl Pts',(-3.8,-6.55,-12.53)) ;
#162711=CARTESIAN_POINT('Ctrl Pts',(-3.81016571653583,-6.55,-12.5249171417321)) ;
#162712=CARTESIAN_POINT('Ctrl Pts',(-3.82068315091943,-6.54961031187958,
-12.519657683858)) ;
#162713=CARTESIAN_POINT('Ctrl Pts',(-3.84304266528023,-6.54783411578235,
-12.5084679497193)) ;
#162714=CARTESIAN_POINT('Ctrl Pts',(-3.85491327259876,-6.54635217950657,
-12.502522761795)) ;
#162715=CARTESIAN_POINT('Ctrl Pts',(-3.87771616262383,-6.54231439116795,
-12.4911067603938)) ;
#162716=CARTESIAN_POINT('Ctrl Pts',(-3.8886625183582,-6.53982180674967,
-12.4856298613037)) ;
#162717=CARTESIAN_POINT('Ctrl Pts',(-3.90045005712288,-6.53645537933199,
-12.4797406960351)) ;
#162718=CARTESIAN_POINT('Ctrl Pts',(-3.90170928105837,-6.53608665347676,
-12.479111682764)) ;
#162719=CARTESIAN_POINT('Ctrl Pts',(-3.91388077026718,-6.53243308776745,
-12.4730327513517)) ;
#162720=CARTESIAN_POINT('Ctrl Pts',(-3.92429308263747,-6.52859969139739,
-12.4678422384291)) ;
#162721=CARTESIAN_POINT('Ctrl Pts',(-3.93645488997274,-6.52312881451531,
-12.4617711869643)) ;
#162722=CARTESIAN_POINT('Ctrl Pts',(-3.93897066587165,-6.52193602330142,
-12.4605146670641)) ;
#162723=CARTESIAN_POINT('Ctrl Pts',(-3.94142135623725,-6.52071067811862,
-12.4592893218813)) ;
#162724=CARTESIAN_POINT('Origin',(-3.78571994569861,-6.44700925663807,-12.5371421042496)) ;
#162725=CARTESIAN_POINT('Origin',(-3.8,-6.45,-10.43)) ;
#162726=CARTESIAN_POINT('',(-3.87071067811867,-6.52071067811864,-10.4714213562373)) ;
#162727=CARTESIAN_POINT('Ctrl Pts',(-3.8,-6.55,-10.33)) ;
#162728=CARTESIAN_POINT('Ctrl Pts',(-3.80508285826792,-6.55,-10.3401657165358)) ;
#162729=CARTESIAN_POINT('Ctrl Pts',(-3.810342316142,-6.54961031187958,-10.3506831509194)) ;
#162730=CARTESIAN_POINT('Ctrl Pts',(-3.82153205028064,-6.54783411578236,
-10.3730426652802)) ;
#162731=CARTESIAN_POINT('Ctrl Pts',(-3.82747723820505,-6.54635217950656,
-10.3849132725988)) ;
#162732=CARTESIAN_POINT('Ctrl Pts',(-3.83889323960397,-6.54231439116875,
-10.4077161626194)) ;
#162733=CARTESIAN_POINT('Ctrl Pts',(-3.84437013869195,-6.53982180675168,
-10.4186625183494)) ;
#162734=CARTESIAN_POINT('Ctrl Pts',(-3.85025930396067,-6.53645537933445,
-10.4304500571145)) ;
#162735=CARTESIAN_POINT('Ctrl Pts',(-3.85088831723394,-6.53608665347802,
-10.4317092810542)) ;
#162736=CARTESIAN_POINT('Ctrl Pts',(-3.85696724864823,-6.53243308776747,
-10.4438807702672)) ;
#162737=CARTESIAN_POINT('Ctrl Pts',(-3.86215776157089,-6.5285996913974,
-10.4542930826375)) ;
#162738=CARTESIAN_POINT('Ctrl Pts',(-3.86822881303571,-6.5231288145153,
-10.4664548899728)) ;
#162739=CARTESIAN_POINT('Ctrl Pts',(-3.86948533293587,-6.52193602330144,
-10.4689706658717)) ;
#162740=CARTESIAN_POINT('Ctrl Pts',(-3.87071067811867,-6.52071067811864,
-10.4714213562373)) ;
#162741=CARTESIAN_POINT('Origin',(-3.79285789573469,-6.44700925663192,-10.3157199456678)) ;
#162742=CARTESIAN_POINT('',(-3.87071067811865,-6.52071067811866,-12.3885786437627)) ;
#162743=CARTESIAN_POINT('Origin',(-3.79291331463695,-6.44703459698198,-12.544170095017)) ;
#162744=CARTESIAN_POINT('Ctrl Pts',(-3.87071067811865,-6.52071067811866,
-12.3885786437627)) ;
#162745=CARTESIAN_POINT('Ctrl Pts',(-3.86620460065363,-6.52521675558368,
-12.3975907986927)) ;
#162746=CARTESIAN_POINT('Ctrl Pts',(-3.86127351832835,-6.52928079264423,
-12.4074862581729)) ;
#162747=CARTESIAN_POINT('Ctrl Pts',(-3.8509791174523,-6.5362468074862,-12.4281127705685)) ;
#162748=CARTESIAN_POINT('Ctrl Pts',(-3.84563601585109,-6.53918030781781,
-12.4388050943343)) ;
#162749=CARTESIAN_POINT('Ctrl Pts',(-3.83952524546737,-6.54185985500283,
-12.4510185932199)) ;
#162750=CARTESIAN_POINT('Ctrl Pts',(-3.83889029009115,-6.54213045061223,
-12.4522875172268)) ;
#162751=CARTESIAN_POINT('Ctrl Pts',(-3.83250371086605,-6.54477467909829,
-12.4650493700286)) ;
#162752=CARTESIAN_POINT('Ctrl Pts',(-3.8266284275938,-6.54657370273653,
-12.476779364282)) ;
#162753=CARTESIAN_POINT('Ctrl Pts',(-3.81540422523879,-6.54896007643136,
-12.499200258884)) ;
#162754=CARTESIAN_POINT('Ctrl Pts',(-3.81004992405497,-6.54963010255188,
-12.5099019216816)) ;
#162755=CARTESIAN_POINT('Ctrl Pts',(-3.80321442618295,-6.54996164986962,
-12.523571160343)) ;
#162756=CARTESIAN_POINT('Ctrl Pts',(-3.80159858684041,-6.55,-12.5268028263192)) ;
#162757=CARTESIAN_POINT('Ctrl Pts',(-3.8,-6.55,-12.53)) ;
#162758=CARTESIAN_POINT('Origin',(-5.,-6.45,-10.43)) ;
#162759=CARTESIAN_POINT('',(-4.9292893218813,-6.52071067811861,-12.3885786437628)) ;
#162760=CARTESIAN_POINT('Ctrl Pts',(-5.,-6.55,-12.53)) ;
#162761=CARTESIAN_POINT('Ctrl Pts',(-4.99491714173206,-6.55,-12.5198342834642)) ;
#162762=CARTESIAN_POINT('Ctrl Pts',(-4.98965768385797,-6.54961031187957,
-12.5093168490806)) ;
#162763=CARTESIAN_POINT('Ctrl Pts',(-4.97846794971932,-6.54783411578235,
-12.4869573347198)) ;
#162764=CARTESIAN_POINT('Ctrl Pts',(-4.97252276179494,-6.54635217950656,
-12.4750867274013)) ;
#162765=CARTESIAN_POINT('Ctrl Pts',(-4.96110676039596,-6.54231439116872,
-12.4522838373806)) ;
#162766=CARTESIAN_POINT('Ctrl Pts',(-4.95562986130792,-6.53982180675161,
-12.4413374816505)) ;
#162767=CARTESIAN_POINT('Ctrl Pts',(-4.94974069603921,-6.53645537933438,
-12.4295499428854)) ;
#162768=CARTESIAN_POINT('Ctrl Pts',(-4.94911168276601,-6.53608665347799,
-12.4282907189459)) ;
#162769=CARTESIAN_POINT('Ctrl Pts',(-4.94303275135178,-6.53243308776748,
-12.416119229733)) ;
#162770=CARTESIAN_POINT('Ctrl Pts',(-4.93784223842911,-6.52859969139739,
-12.4057069173626)) ;
#162771=CARTESIAN_POINT('Ctrl Pts',(-4.93177118696427,-6.52312881451529,
-12.3935451100273)) ;
#162772=CARTESIAN_POINT('Ctrl Pts',(-4.9305146670641,-6.52193602330142,
-12.3910293341284)) ;
#162773=CARTESIAN_POINT('Ctrl Pts',(-4.9292893218813,-6.52071067811861,
-12.3885786437628)) ;
#162774=CARTESIAN_POINT('Origin',(-5.00714210425336,-6.44700925663617,-12.5442800543089)) ;
#162775=CARTESIAN_POINT('',(-4.9292893218813,-6.52071067811861,-10.4714213562372)) ;
#162776=CARTESIAN_POINT('Origin',(-5.00708668538065,-6.44703459697523,-10.3158299049469)) ;
#162777=CARTESIAN_POINT('Ctrl Pts',(-4.9292893218813,-6.52071067811861,
-10.4714213562372)) ;
#162778=CARTESIAN_POINT('Ctrl Pts',(-4.93379539934634,-6.52521675558366,
-10.4624092013071)) ;
#162779=CARTESIAN_POINT('Ctrl Pts',(-4.93872648167164,-6.52928079264423,
-10.4525137418269)) ;
#162780=CARTESIAN_POINT('Ctrl Pts',(-4.94902088254777,-6.53624680748624,
-10.4318872294311)) ;
#162781=CARTESIAN_POINT('Ctrl Pts',(-4.95436398414903,-6.53918030781788,
-10.4211949056652)) ;
#162782=CARTESIAN_POINT('Ctrl Pts',(-4.96047475453275,-6.54185985500288,
-10.4089814067796)) ;
#162783=CARTESIAN_POINT('Ctrl Pts',(-4.96110970990889,-6.54213045061225,
-10.4077124827729)) ;
#162784=CARTESIAN_POINT('Ctrl Pts',(-4.9674962891339,-6.54477467909827,
-10.3949506299713)) ;
#162785=CARTESIAN_POINT('Ctrl Pts',(-4.97337157240611,-6.5465737027365,
-10.3832206357179)) ;
#162786=CARTESIAN_POINT('Ctrl Pts',(-4.98459577476111,-6.54896007643135,
-10.3607997411161)) ;
#162787=CARTESIAN_POINT('Ctrl Pts',(-4.98995007594495,-6.54963010255187,
-10.3500980783185)) ;
#162788=CARTESIAN_POINT('Ctrl Pts',(-4.99678557381701,-6.54996164986962,
-10.3364288396571)) ;
#162789=CARTESIAN_POINT('Ctrl Pts',(-4.99840141315956,-6.55,-10.3331971736809)) ;
#162790=CARTESIAN_POINT('Ctrl Pts',(-5.,-6.55,-10.33)) ;
#162791=CARTESIAN_POINT('Origin',(-4.9,-6.45,-10.33)) ;
#162792=CARTESIAN_POINT('',(-4.85857864376269,-6.52071067811866,-10.4007106781187)) ;
#162793=CARTESIAN_POINT('Ctrl Pts',(-5.,-6.55,-10.33)) ;
#162794=CARTESIAN_POINT('Ctrl Pts',(-4.98983428346413,-6.55,-10.3350828582679)) ;
#162795=CARTESIAN_POINT('Ctrl Pts',(-4.9793168490805,-6.54961031187958,
-10.340342316142)) ;
#162796=CARTESIAN_POINT('Ctrl Pts',(-4.9569573347196,-6.54783411578236,
-10.3515320502806)) ;
#162797=CARTESIAN_POINT('Ctrl Pts',(-4.94508672740101,-6.54635217950657,
-10.357477238205)) ;
#162798=CARTESIAN_POINT('Ctrl Pts',(-4.9222838373818,-6.542314391169,-10.3688932396033)) ;
#162799=CARTESIAN_POINT('Ctrl Pts',(-4.91133748165322,-6.53982180675231,
-10.3743701386905)) ;
#162800=CARTESIAN_POINT('Ctrl Pts',(-4.89954994288802,-6.53645537933523,
-10.3802593039593)) ;
#162801=CARTESIAN_POINT('Ctrl Pts',(-4.89829071894688,-6.53608665347839,
-10.3808883172333)) ;
#162802=CARTESIAN_POINT('Ctrl Pts',(-4.88611922973253,-6.53243308776743,
-10.3869672486483)) ;
#162803=CARTESIAN_POINT('Ctrl Pts',(-4.87570691736229,-6.52859969139738,
-10.3921577615709)) ;
#162804=CARTESIAN_POINT('Ctrl Pts',(-4.86354511002712,-6.5231288145153,
-10.3982288130357)) ;
#162805=CARTESIAN_POINT('Ctrl Pts',(-4.86102933412825,-6.52193602330142,
-10.3994853329359)) ;
#162806=CARTESIAN_POINT('Ctrl Pts',(-4.85857864376269,-6.52071067811863,
-10.4007106781187)) ;
#162807=CARTESIAN_POINT('Origin',(-5.01428005429581,-6.44700925663878,-10.3228578957533)) ;
#162808=CARTESIAN_POINT('',(-3.94142135623724,-6.52071067811862,-10.4007106781187)) ;
#162809=CARTESIAN_POINT('Origin',(-3.78582990492664,-6.44703459697108,-10.3229133146092)) ;
#162810=CARTESIAN_POINT('Ctrl Pts',(-3.94142135623724,-6.52071067811862,
-10.4007106781187)) ;
#162811=CARTESIAN_POINT('Ctrl Pts',(-3.93240920130719,-6.52521675558363,
-10.3962046006537)) ;
#162812=CARTESIAN_POINT('Ctrl Pts',(-3.92251374182705,-6.52928079264421,
-10.3912735183284)) ;
#162813=CARTESIAN_POINT('Ctrl Pts',(-3.90188722943306,-6.53624680748561,
-10.3809791174532)) ;
#162814=CARTESIAN_POINT('Ctrl Pts',(-3.89119490566911,-6.53918030781684,
-10.3756360158529)) ;
#162815=CARTESIAN_POINT('Ctrl Pts',(-3.87898140678367,-6.54185985500205,
-10.3695252454692)) ;
#162816=CARTESIAN_POINT('Ctrl Pts',(-3.87771248277498,-6.54213045061184,
-10.3688902900921)) ;
#162817=CARTESIAN_POINT('Ctrl Pts',(-3.86495062997144,-6.54477467909826,
-10.3625037108661)) ;
#162818=CARTESIAN_POINT('Ctrl Pts',(-3.85322063571806,-6.5465737027365,
-10.3566284275939)) ;
#162819=CARTESIAN_POINT('Ctrl Pts',(-3.83079974111621,-6.54896007643133,
-10.345404225239)) ;
#162820=CARTESIAN_POINT('Ctrl Pts',(-3.82009807831861,-6.54963010255187,
-10.3400499240551)) ;
#162821=CARTESIAN_POINT('Ctrl Pts',(-3.80642883965713,-6.54996164986962,
-10.3332144261831)) ;
#162822=CARTESIAN_POINT('Ctrl Pts',(-3.8031971736809,-6.55,-10.3315985868405)) ;
#162823=CARTESIAN_POINT('Ctrl Pts',(-3.8,-6.55,-10.33)) ;
#162824=CARTESIAN_POINT('Origin',(-4.9,-6.45,-8.72)) ;
#162825=CARTESIAN_POINT('',(-4.85857864376269,-6.52071067811866,-8.64928932188135)) ;
#162826=CARTESIAN_POINT('Origin',(-5.0141700950508,-6.44703459697536,-8.72708668537973)) ;
#162827=CARTESIAN_POINT('Ctrl Pts',(-4.85857864376269,-6.52071067811865,
-8.64928932188135)) ;
#162828=CARTESIAN_POINT('Ctrl Pts',(-4.86759079869274,-6.52521675558369,
-8.65379539934638)) ;
#162829=CARTESIAN_POINT('Ctrl Pts',(-4.87748625817286,-6.52928079264424,
-8.65872648167166)) ;
#162830=CARTESIAN_POINT('Ctrl Pts',(-4.89811277056854,-6.53624680748623,
-8.66902088254776)) ;
#162831=CARTESIAN_POINT('Ctrl Pts',(-4.90880509433436,-6.53918030781786,
-8.67436398414899)) ;
#162832=CARTESIAN_POINT('Ctrl Pts',(-4.92101859321993,-6.54185985500287,
-8.68047475453273)) ;
#162833=CARTESIAN_POINT('Ctrl Pts',(-4.92228751722681,-6.54213045061227,
-8.68110970990893)) ;
#162834=CARTESIAN_POINT('Ctrl Pts',(-4.93504937002862,-6.54477467909833,
-8.68749628913405)) ;
#162835=CARTESIAN_POINT('Ctrl Pts',(-4.94677936428208,-6.54657370273656,
-8.69337157240631)) ;
#162836=CARTESIAN_POINT('Ctrl Pts',(-4.96920025888408,-6.54896007643138,
-8.70459577476134)) ;
#162837=CARTESIAN_POINT('Ctrl Pts',(-4.97990192168174,-6.54963010255189,
-8.70995007594516)) ;
#162838=CARTESIAN_POINT('Ctrl Pts',(-4.99357116034313,-6.54996164986963,
-8.71678557381714)) ;
#162839=CARTESIAN_POINT('Ctrl Pts',(-4.99680282631923,-6.55,-8.71840141315963)) ;
#162840=CARTESIAN_POINT('Ctrl Pts',(-5.,-6.55,-8.72)) ;
#162841=CARTESIAN_POINT('',(-3.94142135623725,-6.52071067811863,-8.64928932188132)) ;
#162842=CARTESIAN_POINT('Ctrl Pts',(-3.8,-6.55,-8.72)) ;
#162843=CARTESIAN_POINT('Ctrl Pts',(-3.81016571653583,-6.55,-8.71491714173207)) ;
#162844=CARTESIAN_POINT('Ctrl Pts',(-3.82068315091943,-6.54961031187958,
-8.70965768385799)) ;
#162845=CARTESIAN_POINT('Ctrl Pts',(-3.84304266528024,-6.54783411578235,
-8.69846794971933)) ;
#162846=CARTESIAN_POINT('Ctrl Pts',(-3.85491327259876,-6.54635217950656,
-8.69252276179493)) ;
#162847=CARTESIAN_POINT('Ctrl Pts',(-3.87771616261911,-6.5423143911688,
-8.68110676039617)) ;
#162848=CARTESIAN_POINT('Ctrl Pts',(-3.88866251834886,-6.5398218067518,
-8.67562986130833)) ;
#162849=CARTESIAN_POINT('Ctrl Pts',(-3.90045005711395,-6.53645537933461,
-8.66974069603961)) ;
#162850=CARTESIAN_POINT('Ctrl Pts',(-3.90170928105393,-6.5360866534781,
-8.66911168276619)) ;
#162851=CARTESIAN_POINT('Ctrl Pts',(-3.91388077026719,-6.53243308776746,
-8.66303275135177)) ;
#162852=CARTESIAN_POINT('Ctrl Pts',(-3.92429308263748,-6.52859969139739,
-8.6578422384291)) ;
#162853=CARTESIAN_POINT('Ctrl Pts',(-3.93645488997274,-6.5231288145153,
-8.65177118696428)) ;
#162854=CARTESIAN_POINT('Ctrl Pts',(-3.93897066587165,-6.52193602330143,
-8.65051466706412)) ;
#162855=CARTESIAN_POINT('Ctrl Pts',(-3.94142135623725,-6.52071067811863,
-8.64928932188132)) ;
#162856=CARTESIAN_POINT('Origin',(-3.78571994570435,-6.44700925663925,-8.72714210424676)) ;
#162857=CARTESIAN_POINT('Origin',(-3.8,-6.45,-6.62)) ;
#162858=CARTESIAN_POINT('',(-3.87071067811865,-6.52071067811866,-6.66142135623731)) ;
#162859=CARTESIAN_POINT('Ctrl Pts',(-3.8,-6.55,-6.52)) ;
#162860=CARTESIAN_POINT('Ctrl Pts',(-3.80508285826792,-6.55,-6.53016571653586)) ;
#162861=CARTESIAN_POINT('Ctrl Pts',(-3.810342316142,-6.54961031187958,-6.54068315091949)) ;
#162862=CARTESIAN_POINT('Ctrl Pts',(-3.82153205028068,-6.54783411578235,
-6.56304266528037)) ;
#162863=CARTESIAN_POINT('Ctrl Pts',(-3.8274772382051,-6.54635217950655,
-6.57491327259895)) ;
#162864=CARTESIAN_POINT('Ctrl Pts',(-3.83889323960401,-6.54231439116873,
-6.59771616261959)) ;
#162865=CARTESIAN_POINT('Ctrl Pts',(-3.84437013869196,-6.53982180675167,
-6.6086625183496)) ;
#162866=CARTESIAN_POINT('Ctrl Pts',(-3.85025930396068,-6.53645537933444,
-6.62045005711466)) ;
#162867=CARTESIAN_POINT('Ctrl Pts',(-3.85088831723398,-6.53608665347799,
-6.62170928105441)) ;
#162868=CARTESIAN_POINT('Ctrl Pts',(-3.85696724864827,-6.53243308776743,
-6.6338807702674)) ;
#162869=CARTESIAN_POINT('Ctrl Pts',(-3.86215776157092,-6.52859969139737,
-6.64429308263765)) ;
#162870=CARTESIAN_POINT('Ctrl Pts',(-3.86822881303572,-6.5231288145153,
-6.65645488997285)) ;
#162871=CARTESIAN_POINT('Ctrl Pts',(-3.86948533293586,-6.52193602330144,
-6.65897066587173)) ;
#162872=CARTESIAN_POINT('Ctrl Pts',(-3.87071067811865,-6.52071067811866,
-6.66142135623731)) ;
#162873=CARTESIAN_POINT('Origin',(-3.79285789575055,-6.44700925663822,-6.5057199456992)) ;
#162874=CARTESIAN_POINT('',(-3.87071067811865,-6.52071067811866,-8.57857864376269)) ;
#162875=CARTESIAN_POINT('Origin',(-3.79291331460542,-6.44703459696871,-8.73417009508047)) ;
#162876=CARTESIAN_POINT('Ctrl Pts',(-3.87071067811865,-6.52071067811866,
-8.57857864376269)) ;
#162877=CARTESIAN_POINT('Ctrl Pts',(-3.86620460065363,-6.52521675558368,
-8.58759079869274)) ;
#162878=CARTESIAN_POINT('Ctrl Pts',(-3.86127351832835,-6.52928079264423,
-8.59748625817286)) ;
#162879=CARTESIAN_POINT('Ctrl Pts',(-3.85097911745197,-6.53624680748642,
-8.61811277056917)) ;
#162880=CARTESIAN_POINT('Ctrl Pts',(-3.84563601585041,-6.53918030781819,
-8.62880509433569)) ;
#162881=CARTESIAN_POINT('Ctrl Pts',(-3.83952524546667,-6.54185985500313,
-8.64101859322128)) ;
#162882=CARTESIAN_POINT('Ctrl Pts',(-3.8388902900908,-6.54213045061238,
-8.64228751722748)) ;
#162883=CARTESIAN_POINT('Ctrl Pts',(-3.83250371086605,-6.5447746790983,
-8.65504937002858)) ;
#162884=CARTESIAN_POINT('Ctrl Pts',(-3.8266284275938,-6.54657370273653,
-8.66677936428201)) ;
#162885=CARTESIAN_POINT('Ctrl Pts',(-3.8154042252388,-6.54896007643136,
-8.68920025888395)) ;
#162886=CARTESIAN_POINT('Ctrl Pts',(-3.81004992405497,-6.54963010255188,
-8.69990192168157)) ;
#162887=CARTESIAN_POINT('Ctrl Pts',(-3.80321442618295,-6.54996164986962,
-8.713571160343)) ;
#162888=CARTESIAN_POINT('Ctrl Pts',(-3.80159858684042,-6.55,-8.71680282631917)) ;
#162889=CARTESIAN_POINT('Ctrl Pts',(-3.8,-6.55,-8.72)) ;
#162890=CARTESIAN_POINT('Origin',(-5.,-6.45,-6.62)) ;
#162891=CARTESIAN_POINT('',(-4.9292893218813,-6.52071067811861,-8.57857864376279)) ;
#162892=CARTESIAN_POINT('Ctrl Pts',(-5.,-6.55,-8.72)) ;
#162893=CARTESIAN_POINT('Ctrl Pts',(-4.99491714173206,-6.55,-8.70983428346417)) ;
#162894=CARTESIAN_POINT('Ctrl Pts',(-4.98965768385797,-6.54961031187957,
-8.69931684908058)) ;
#162895=CARTESIAN_POINT('Ctrl Pts',(-4.97846794971931,-6.54783411578235,
-8.67695733471982)) ;
#162896=CARTESIAN_POINT('Ctrl Pts',(-4.97252276179493,-6.54635217950656,
-8.66508672740134)) ;
#162897=CARTESIAN_POINT('Ctrl Pts',(-4.96110676039608,-6.54231439116877,
-8.64228383738083)) ;
#162898=CARTESIAN_POINT('Ctrl Pts',(-4.95562986130815,-6.53982180675172,
-8.63133748165089)) ;
#162899=CARTESIAN_POINT('Ctrl Pts',(-4.94974069603943,-6.53645537933451,
-8.61954994288583)) ;
#162900=CARTESIAN_POINT('Ctrl Pts',(-4.94911168276612,-6.53608665347805,
-8.61829071894605)) ;
#162901=CARTESIAN_POINT('Ctrl Pts',(-4.94303275135178,-6.53243308776748,
-8.60611922973296)) ;
#162902=CARTESIAN_POINT('Ctrl Pts',(-4.93784223842912,-6.5285996913974,
-8.59570691736265)) ;
#162903=CARTESIAN_POINT('Ctrl Pts',(-4.93177118696428,-6.5231288145153,
-8.58354511002734)) ;
#162904=CARTESIAN_POINT('Ctrl Pts',(-4.9305146670641,-6.52193602330142,
-8.58102933412841)) ;
#162905=CARTESIAN_POINT('Ctrl Pts',(-4.9292893218813,-6.52071067811861,
-8.57857864376279)) ;
#162906=CARTESIAN_POINT('Origin',(-5.00714210425842,-6.4470092566342,-8.73428005431905)) ;
#162907=CARTESIAN_POINT('',(-4.92928932188132,-6.52071067811863,-6.66142135623726)) ;
#162908=CARTESIAN_POINT('Origin',(-5.007086685383,-6.44703459697434,-6.50582990494236)) ;
#162909=CARTESIAN_POINT('Ctrl Pts',(-4.92928932188132,-6.52071067811863,
-6.66142135623726)) ;
#162910=CARTESIAN_POINT('Ctrl Pts',(-4.93379539934634,-6.52521675558365,
-6.6524092013072)) ;
#162911=CARTESIAN_POINT('Ctrl Pts',(-4.93872648167162,-6.5292807926442,
-6.64251374182708)) ;
#162912=CARTESIAN_POINT('Ctrl Pts',(-4.94902088254778,-6.53624680748625,
-6.62188722943121)) ;
#162913=CARTESIAN_POINT('Ctrl Pts',(-4.9543639841491,-6.53918030781792,
-6.61119490566518)) ;
#162914=CARTESIAN_POINT('Ctrl Pts',(-4.96047475453282,-6.54185985500291,
-6.59898140677963)) ;
#162915=CARTESIAN_POINT('Ctrl Pts',(-4.96110970990891,-6.54213045061226,
-6.59771248277296)) ;
#162916=CARTESIAN_POINT('Ctrl Pts',(-4.96749628913387,-6.54477467909827,
-6.58495062997146)) ;
#162917=CARTESIAN_POINT('Ctrl Pts',(-4.9733715724061,-6.5465737027365,-6.57322063571808)) ;
#162918=CARTESIAN_POINT('Ctrl Pts',(-4.98459577476108,-6.54896007643134,
-6.55079974111622)) ;
#162919=CARTESIAN_POINT('Ctrl Pts',(-4.98995007594491,-6.54963010255187,
-6.54009807831861)) ;
#162920=CARTESIAN_POINT('Ctrl Pts',(-4.99678557381697,-6.54996164986962,
-6.52642883965713)) ;
#162921=CARTESIAN_POINT('Ctrl Pts',(-4.99840141315954,-6.55,-6.5231971736809)) ;
#162922=CARTESIAN_POINT('Ctrl Pts',(-5.,-6.55,-6.52)) ;
#162923=CARTESIAN_POINT('Origin',(-4.9,-6.45,-6.52)) ;
#162924=CARTESIAN_POINT('',(-4.85857864376269,-6.52071067811866,-6.59071067811866)) ;
#162925=CARTESIAN_POINT('Ctrl Pts',(-5.,-6.55,-6.52)) ;
#162926=CARTESIAN_POINT('Ctrl Pts',(-4.98983428346415,-6.55,-6.52508285826791)) ;
#162927=CARTESIAN_POINT('Ctrl Pts',(-4.97931684908054,-6.54961031187958,
-6.53034231614198)) ;
#162928=CARTESIAN_POINT('Ctrl Pts',(-4.95695733471967,-6.54783411578236,
-6.54153205028064)) ;
#162929=CARTESIAN_POINT('Ctrl Pts',(-4.9450867274011,-6.54635217950656,
-6.54747723820505)) ;
#162930=CARTESIAN_POINT('Ctrl Pts',(-4.92228383738093,-6.54231439116883,
-6.55889323960373)) ;
#162931=CARTESIAN_POINT('Ctrl Pts',(-4.91133748165139,-6.5398218067519,
-6.56437013869147)) ;
#162932=CARTESIAN_POINT('Ctrl Pts',(-4.89954994288627,-6.53645537933471,
-6.57025930396021)) ;
#162933=CARTESIAN_POINT('Ctrl Pts',(-4.89829071894607,-6.53608665347814,
-6.57088831723374)) ;
#162934=CARTESIAN_POINT('Ctrl Pts',(-4.88611922973263,-6.53243308776745,
-6.57696724864825)) ;
#162935=CARTESIAN_POINT('Ctrl Pts',(-4.87570691736238,-6.52859969139738,
-6.5821577615709)) ;
#162936=CARTESIAN_POINT('Ctrl Pts',(-4.86354511002717,-6.5231288145153,
-6.58822881303571)) ;
#162937=CARTESIAN_POINT('Ctrl Pts',(-4.86102933412828,-6.52193602330145,
-6.58948533293586)) ;
#162938=CARTESIAN_POINT('Ctrl Pts',(-4.85857864376269,-6.52071067811865,
-6.59071067811866)) ;
#162939=CARTESIAN_POINT('Origin',(-5.0142800542992,-6.44700925663862,-6.51285789575134)) ;
#162940=CARTESIAN_POINT('',(-3.94142135623721,-6.52071067811861,-6.59071067811871)) ;
#162941=CARTESIAN_POINT('Origin',(-3.78582990493307,-6.44703459697233,-6.51291331461247)) ;
#162942=CARTESIAN_POINT('Ctrl Pts',(-3.94142135623721,-6.52071067811861,
-6.5907106781187)) ;
#162943=CARTESIAN_POINT('Ctrl Pts',(-3.93240920130712,-6.52521675558366,
-6.58620460065366)) ;
#162944=CARTESIAN_POINT('Ctrl Pts',(-3.92251374182695,-6.52928079264422,
-6.58127351832836)) ;
#162945=CARTESIAN_POINT('Ctrl Pts',(-3.90188722943119,-6.53624680748622,
-6.57097911745226)) ;
#162946=CARTESIAN_POINT('Ctrl Pts',(-3.89119490566534,-6.53918030781785,
-6.56563601585102)) ;
#162947=CARTESIAN_POINT('Ctrl Pts',(-3.8789814067798,-6.54185985500286,
-6.55952524546731)) ;
#162948=CARTESIAN_POINT('Ctrl Pts',(-3.87771248277297,-6.54213045061224,
-6.55889029009113)) ;
#162949=CARTESIAN_POINT('Ctrl Pts',(-3.86495062997132,-6.54477467909828,
-6.5525037108661)) ;
#162950=CARTESIAN_POINT('Ctrl Pts',(-3.85322063571796,-6.54657370273651,
-6.54662842759388)) ;
#162951=CARTESIAN_POINT('Ctrl Pts',(-3.83079974111614,-6.54896007643134,
-6.5354042252389)) ;
#162952=CARTESIAN_POINT('Ctrl Pts',(-3.82009807831854,-6.54963010255187,
-6.53004992405507)) ;
#162953=CARTESIAN_POINT('Ctrl Pts',(-3.80642883965709,-6.54996164986962,
-6.52321442618302)) ;
#162954=CARTESIAN_POINT('Ctrl Pts',(-3.80319717368088,-6.55,-6.52159858684045)) ;
#162955=CARTESIAN_POINT('Ctrl Pts',(-3.8,-6.55,-6.52)) ;
#162956=CARTESIAN_POINT('Origin',(-4.9,-6.45,-2.71)) ;
#162957=CARTESIAN_POINT('Origin',(-4.,-6.45,-2.71)) ;
#162958=CARTESIAN_POINT('Origin',(-4.8,-6.45,-2.71)) ;
#162959=CARTESIAN_POINT('Origin',(-4.8,-6.45,-2.91)) ;
#162960=CARTESIAN_POINT('Origin',(-5.,-6.45,-2.91)) ;
#162961=CARTESIAN_POINT('Origin',(-4.8,-6.45,-2.91)) ;
#162962=CARTESIAN_POINT('Origin',(-4.,-6.45,-2.91)) ;
#162963=CARTESIAN_POINT('Origin',(-4.,-6.45,-2.91)) ;
#162964=CARTESIAN_POINT('Origin',(-3.8,-6.45,-2.91)) ;
#162965=CARTESIAN_POINT('Origin',(-5.,-6.45,-2.81)) ;
#162966=CARTESIAN_POINT('Origin',(-5.,-6.45,-4.71)) ;
#162967=CARTESIAN_POINT('Origin',(-4.8,-6.4,-2.91)) ;
#162968=CARTESIAN_POINT('Origin',(-4.8,-6.35,-2.91)) ;
#162969=CARTESIAN_POINT('Origin',(1.9515639104739E-16,-6.35,-2.91)) ;
#162970=CARTESIAN_POINT('Origin',(-4.,-6.35,-2.91)) ;
#162971=CARTESIAN_POINT('Origin',(-4.8,-6.35,-2.91)) ;
#162972=CARTESIAN_POINT('Origin',(-4.,-6.4,-2.91)) ;
#162973=CARTESIAN_POINT('Origin',(-4.,-6.35,-2.91)) ;
#162974=CARTESIAN_POINT('Origin',(-3.8,-6.45,-2.81)) ;
#162975=CARTESIAN_POINT('Origin',(-3.8,-6.45,-4.71)) ;
#162976=CARTESIAN_POINT('Origin',(-4.9,-6.45,-4.91)) ;
#162977=CARTESIAN_POINT('Origin',(-4.8,-6.45,-4.91)) ;
#162978=CARTESIAN_POINT('Origin',(-4.,-6.45,-4.91)) ;
#162979=CARTESIAN_POINT('Origin',(-4.8,-6.45,-4.71)) ;
#162980=CARTESIAN_POINT('Origin',(-4.8,-6.45,-4.71)) ;
#162981=CARTESIAN_POINT('Origin',(-4.8,-6.35,-2.91)) ;
#162982=CARTESIAN_POINT('Origin',(-4.8,-6.35,-2.91)) ;
#162983=CARTESIAN_POINT('Origin',(-4.,-6.35,-2.91)) ;
#162984=CARTESIAN_POINT('Origin',(-4.,-6.35,-2.91)) ;
#162985=CARTESIAN_POINT('Origin',(-4.,-6.45,-4.71)) ;
#162986=CARTESIAN_POINT('Origin',(-4.,-6.45,-4.71)) ;
#162987=CARTESIAN_POINT('Origin',(-4.8,-6.4,-4.71)) ;
#162988=CARTESIAN_POINT('Origin',(-4.8,-6.35,-4.71)) ;
#162989=CARTESIAN_POINT('Origin',(-4.8,-6.35,-3.81)) ;
#162990=CARTESIAN_POINT('Origin',(-4.8,-6.35,-4.71)) ;
#162991=CARTESIAN_POINT('Origin',(-4.,-6.35,-3.81)) ;
#162992=CARTESIAN_POINT('Origin',(-4.,-6.35,-4.71)) ;
#162993=CARTESIAN_POINT('Origin',(-4.,-6.4,-4.71)) ;
#162994=CARTESIAN_POINT('Origin',(-4.,-6.35,-4.71)) ;
#162995=CARTESIAN_POINT('Origin',(-4.8,-6.35,-4.71)) ;
#162996=CARTESIAN_POINT('Origin',(-4.8,-6.35,-4.71)) ;
#162997=CARTESIAN_POINT('Origin',(-4.,-6.35,-4.71)) ;
#162998=CARTESIAN_POINT('Origin',(-4.,-6.35,-4.71)) ;
#162999=CARTESIAN_POINT('Origin',(1.95156391047391E-16,-6.35,-4.71)) ;
#163000=CARTESIAN_POINT('Origin',(-4.15,-6.25,-3.06)) ;
#163001=CARTESIAN_POINT('Origin',(-4.15,-6.3,-3.06)) ;
#163002=CARTESIAN_POINT('Origin',(-4.15,-6.3,-3.81)) ;
#163003=CARTESIAN_POINT('Origin',(-4.15,-6.3,-4.56)) ;
#163004=CARTESIAN_POINT('Origin',(-4.15,-6.3,-3.06)) ;
#163005=CARTESIAN_POINT('Origin',(-4.15,-6.25,-4.56)) ;
#163006=CARTESIAN_POINT('Origin',(-4.15,-6.3,-4.56)) ;
#163007=CARTESIAN_POINT('Origin',(-4.15,-6.3,-3.06)) ;
#163008=CARTESIAN_POINT('Origin',(-4.15,-6.3,-3.06)) ;
#163009=CARTESIAN_POINT('Origin',(-4.15,-6.3,-4.56)) ;
#163010=CARTESIAN_POINT('Origin',(-4.15,-6.3,-4.56)) ;
#163011=CARTESIAN_POINT('Origin',(-4.65,-6.25,-3.06)) ;
#163012=CARTESIAN_POINT('Origin',(-4.65,-6.3,-3.06)) ;
#163013=CARTESIAN_POINT('Origin',(0.,-6.3,-3.06)) ;
#163014=CARTESIAN_POINT('Origin',(-4.65,-6.3,-3.06)) ;
#163015=CARTESIAN_POINT('Origin',(0.,-6.3,-4.56)) ;
#163016=CARTESIAN_POINT('Origin',(-4.65,-6.3,-4.56)) ;
#163017=CARTESIAN_POINT('Origin',(-4.65,-6.25,-4.56)) ;
#163018=CARTESIAN_POINT('Origin',(-4.65,-6.3,-4.56)) ;
#163019=CARTESIAN_POINT('Origin',(-4.65,-6.3,-3.06)) ;
#163020=CARTESIAN_POINT('Origin',(-4.65,-6.3,-3.06)) ;
#163021=CARTESIAN_POINT('Origin',(-4.65,-6.3,-4.56)) ;
#163022=CARTESIAN_POINT('Origin',(-4.65,-6.3,-4.56)) ;
#163023=CARTESIAN_POINT('Origin',(-4.65,-6.3,-3.81)) ;
#163024=CARTESIAN_POINT('Origin',(-3.09057773798104,-4.00084361825625,-4.31055391724001)) ;
#163025=CARTESIAN_POINT('Origin',(-5.17275707706436,-1.91866427917294,-5.31)) ;
#163026=CARTESIAN_POINT('Origin',(-5.17275707706436,-1.91866427917294,-5.31)) ;
#163027=CARTESIAN_POINT('Origin',(-5.17275707706436,-1.91866427917294,-5.31)) ;
#163028=CARTESIAN_POINT('Origin',(-5.17275707706436,-1.91866427917294,-5.31)) ;
#163029=CARTESIAN_POINT('Origin',(-3.59571067811865,-3.49571067811865,-5.31)) ;
#163030=CARTESIAN_POINT('Ctrl Pts',(-5.8,-1.2914213562373,-5.41)) ;
#163031=CARTESIAN_POINT('Ctrl Pts',(-5.81856398038092,-1.23572941509446,
-5.41)) ;
#163032=CARTESIAN_POINT('Ctrl Pts',(-5.83691006697105,-1.1806911553242,
-5.39922263893878)) ;
#163033=CARTESIAN_POINT('Ctrl Pts',(-5.86308993302895,-1.10215155715041,
-5.36219871729853)) ;
#163034=CARTESIAN_POINT('Ctrl Pts',(-5.8707106769584,-1.0792893230416,-5.33625343280361)) ;
#163035=CARTESIAN_POINT('Ctrl Pts',(-5.87071067811865,-1.07928932188134,
-5.31)) ;
#163036=CARTESIAN_POINT('Origin',(-5.17275707706436,-5.05,-5.31)) ;
#163037=CARTESIAN_POINT('Origin',(-5.17275707706436,-5.26511162862565,-5.31)) ;
#163038=CARTESIAN_POINT('Origin',(-3.96111272388873,-4.96220054033175,-4.72841071047569)) ;
#163039=CARTESIAN_POINT('Origin',(-5.17275707706436,-5.26511162862565,-5.31)) ;
#163040=CARTESIAN_POINT('Ctrl Pts',(-5.9,-1.00857864376269,-5.31)) ;
#163041=CARTESIAN_POINT('Ctrl Pts',(-5.9,-1.04999999999999,-5.31)) ;
#163042=CARTESIAN_POINT('Ctrl Pts',(-5.87071067811865,-1.07928932188134,
-5.31)) ;
#163043=CARTESIAN_POINT('Ctrl Pts',(-5.9,-1.00857864608315,-5.36250686562998)) ;
#163044=CARTESIAN_POINT('Ctrl Pts',(-5.9,-1.0500000026192,-5.34717194963253)) ;
#163045=CARTESIAN_POINT('Ctrl Pts',(-5.8707106769584,-1.0792893230416,-5.33625343280361)) ;
#163046=CARTESIAN_POINT('Ctrl Pts',(-5.9,-1.03906162412146,-5.41439743459706)) ;
#163047=CARTESIAN_POINT('Ctrl Pts',(-5.9,-1.08015861705713,-5.38457207120098)) ;
#163048=CARTESIAN_POINT('Ctrl Pts',(-5.86308993302894,-1.10215155715041,
-5.36219871729853)) ;
#163049=CARTESIAN_POINT('Ctrl Pts',(-5.9,-1.14378108835315,-5.48844527787756)) ;
#163050=CARTESIAN_POINT('Ctrl Pts',(-5.9,-1.17342005527962,-5.42578812462634)) ;
#163051=CARTESIAN_POINT('Ctrl Pts',(-5.83691006697105,-1.1806911553242,
-5.39922263893878)) ;
#163052=CARTESIAN_POINT('Ctrl Pts',(-5.9,-1.21716543471637,-5.50999999941992)) ;
#163053=CARTESIAN_POINT('Ctrl Pts',(-5.89999999999991,-1.24006789214487,
-5.42711774888614)) ;
#163054=CARTESIAN_POINT('Ctrl Pts',(-5.81856398038092,-1.23572941509446,
-5.41)) ;
#163055=CARTESIAN_POINT('Ctrl Pts',(-5.9,-1.2914213562373,-5.51)) ;
#163056=CARTESIAN_POINT('Ctrl Pts',(-5.9,-1.2914213562373,-5.41)) ;
#163057=CARTESIAN_POINT('Ctrl Pts',(-5.8,-1.2914213562373,-5.41)) ;
#163058=CARTESIAN_POINT('Origin',(-5.8,-1.2914213562373,-5.51)) ;
#163059=CARTESIAN_POINT('Origin',(-5.8,-1.00857864376269,-5.31)) ;
#163060=CARTESIAN_POINT('Origin',(-5.17275707706436,-5.26511162862565,-5.31)) ;
#163061=CARTESIAN_POINT('Origin',(-5.17275707706436,-5.26511162862565,-5.31)) ;
#163062=CARTESIAN_POINT('Origin',(-3.78014014831103,-3.31128120792626,-2.9784561258016)) ;
#163063=CARTESIAN_POINT('Origin',(-5.17275707706436,-1.91866427917294,-2.31)) ;
#163064=CARTESIAN_POINT('Origin',(-3.97071067811865,-3.12071067811865,-2.31)) ;
#163065=CARTESIAN_POINT('Ctrl Pts',(-5.87071067811865,-1.07928932188134,
-2.31)) ;
#163066=CARTESIAN_POINT('Ctrl Pts',(-5.87071067695842,-1.07928932304157,
-2.28374656719639)) ;
#163067=CARTESIAN_POINT('Ctrl Pts',(-5.86308993302895,-1.10215155715042,
-2.25780128270147)) ;
#163068=CARTESIAN_POINT('Ctrl Pts',(-5.83691006697105,-1.18069115532419,
-2.22077736106122)) ;
#163069=CARTESIAN_POINT('Ctrl Pts',(-5.81856398038092,-1.23572941509447,
-2.21)) ;
#163070=CARTESIAN_POINT('Ctrl Pts',(-5.8,-1.29142135623731,-2.21)) ;
#163071=CARTESIAN_POINT('Origin',(-5.17275707706436,-1.91866427917294,-2.31)) ;
#163072=CARTESIAN_POINT('Origin',(-5.8,-1.00857864376269,-36.59)) ;
#163073=CARTESIAN_POINT('Origin',(-5.8,-1.00857864376269,-2.31)) ;
#163074=CARTESIAN_POINT('Origin',(-5.8,-6.55,-5.51)) ;
#163075=CARTESIAN_POINT('Origin',(-5.8,-5.42192235935956,-5.51)) ;
#163076=CARTESIAN_POINT('Origin',(-5.10072415073893,-5.24710339704429,-5.31)) ;
#163077=CARTESIAN_POINT('Origin',(-5.80000000000002,-5.42192235935964,-5.31000000000008)) ;
#163078=CARTESIAN_POINT('Origin',(-5.17275707706436,-1.91866427917293,-2.31)) ;
#163079=CARTESIAN_POINT('Origin',(-5.17275707706436,-1.91866427917294,-2.31)) ;
#163080=CARTESIAN_POINT('Ctrl Pts',(-5.9,-1.29142135623731,-2.11)) ;
#163081=CARTESIAN_POINT('Ctrl Pts',(-5.9,-1.29142135623731,-2.21)) ;
#163082=CARTESIAN_POINT('Ctrl Pts',(-5.8,-1.29142135623731,-2.21)) ;
#163083=CARTESIAN_POINT('Ctrl Pts',(-5.9,-1.21716543471638,-2.11000000058011)) ;
#163084=CARTESIAN_POINT('Ctrl Pts',(-5.9,-1.24006789214487,-2.19288225111391)) ;
#163085=CARTESIAN_POINT('Ctrl Pts',(-5.81856398038092,-1.23572941509447,
-2.21)) ;
#163086=CARTESIAN_POINT('Ctrl Pts',(-5.9,-1.14378108835315,-2.13155472212247)) ;
#163087=CARTESIAN_POINT('Ctrl Pts',(-5.9,-1.1734200552796,-2.19421187537365)) ;
#163088=CARTESIAN_POINT('Ctrl Pts',(-5.83691006697105,-1.18069115532419,
-2.22077736106122)) ;
#163089=CARTESIAN_POINT('Ctrl Pts',(-5.9,-1.03906162412146,-2.20560256540291)) ;
#163090=CARTESIAN_POINT('Ctrl Pts',(-5.9,-1.08015861705715,-2.23542792879904)) ;
#163091=CARTESIAN_POINT('Ctrl Pts',(-5.86308993302895,-1.10215155715042,
-2.25780128270147)) ;
#163092=CARTESIAN_POINT('Ctrl Pts',(-5.9,-1.00857864608315,-2.25749313437004)) ;
#163093=CARTESIAN_POINT('Ctrl Pts',(-5.9,-1.05000000261917,-2.27282805036745)) ;
#163094=CARTESIAN_POINT('Ctrl Pts',(-5.87071067695842,-1.07928932304157,
-2.28374656719639)) ;
#163095=CARTESIAN_POINT('Ctrl Pts',(-5.9,-1.00857864376269,-2.31)) ;
#163096=CARTESIAN_POINT('Ctrl Pts',(-5.9,-1.05,-2.31)) ;
#163097=CARTESIAN_POINT('Ctrl Pts',(-5.87071067811865,-1.07928932188134,
-2.31)) ;
#163098=CARTESIAN_POINT('Origin',(-5.8,-1.29142135623731,-2.11)) ;
#163099=CARTESIAN_POINT('Ctrl Pts',(-5.9,-5.42181243301045,-5.50999997036252)) ;
#163100=CARTESIAN_POINT('Ctrl Pts',(-5.9,-5.42186418462486,-5.4099118155266)) ;
#163101=CARTESIAN_POINT('Ctrl Pts',(-5.79991187715164,-5.42186416305549,
-5.41000002317701)) ;
#163102=CARTESIAN_POINT('Ctrl Pts',(-5.9,-5.47597273077136,-5.51002917711606)) ;
#163103=CARTESIAN_POINT('Ctrl Pts',(-5.89999999999995,-5.44963575044053,
-5.41611310490821)) ;
#163104=CARTESIAN_POINT('Ctrl Pts',(-5.80628621775607,-5.45053795385125,
-5.41000983135988)) ;
#163105=CARTESIAN_POINT('Ctrl Pts',(-5.9,-5.5295069829522,-5.48847029676528)) ;
#163106=CARTESIAN_POINT('Ctrl Pts',(-5.90000000000004,-5.48352164712825,
-5.41029821762256)) ;
#163107=CARTESIAN_POINT('Ctrl Pts',(-5.81258729511711,-5.47887520585225,
-5.39922629545968)) ;
#163108=CARTESIAN_POINT('Ctrl Pts',(-5.9,-5.60588533050919,-5.41437241570934)) ;
#163109=CARTESIAN_POINT('Ctrl Pts',(-5.89999999999995,-5.53371219741587,
-5.37246819784151)) ;
#163110=CARTESIAN_POINT('Ctrl Pts',(-5.82157770712951,-5.51930255765374,
-5.36217766736416)) ;
#163111=CARTESIAN_POINT('Ctrl Pts',(-5.9,-5.62810771557601,-5.36243656245292)) ;
#163112=CARTESIAN_POINT('Ctrl Pts',(-5.9,-5.54996909580657,-5.34142484145069)) ;
#163113=CARTESIAN_POINT('Ctrl Pts',(-5.8241936039171,-5.53106345572106,
-5.33621391054005)) ;
#163114=CARTESIAN_POINT('Ctrl Pts',(-5.9,-5.62807761009112,-5.30989335577685)) ;
#163115=CARTESIAN_POINT('Ctrl Pts',(-5.9,-5.54994729905278,-5.30993608021398)) ;
#163116=CARTESIAN_POINT('Ctrl Pts',(-5.82419006898362,-5.53104752404526,
-5.30994668678336)) ;
#163117=CARTESIAN_POINT('Origin',(-5.8,-5.62807764064044,-5.31)) ;
#163118=CARTESIAN_POINT('Origin',(-5.15068655017073,-5.25959399690224,-2.32059385290894)) ;
#163119=CARTESIAN_POINT('Origin',(-5.17275707706436,-5.26511162862565,-2.31)) ;
#163120=CARTESIAN_POINT('Origin',(-5.17275707706436,-5.05,-2.31)) ;
#163121=CARTESIAN_POINT('Origin',(-5.17275707706436,-5.26511162862565,-2.31)) ;
#163122=CARTESIAN_POINT('Origin',(-5.8,-5.05,-2.11)) ;
#163123=CARTESIAN_POINT('Origin',(-5.8,-5.42192235935956,-2.11)) ;
#163124=CARTESIAN_POINT('Origin',(-5.8,-5.62807764064044,-36.59)) ;
#163125=CARTESIAN_POINT('Origin',(-5.8,-5.62807764064044,-2.31)) ;
#163126=CARTESIAN_POINT('Origin',(-5.17275707706436,-5.26511162862565,-2.31)) ;
#163127=CARTESIAN_POINT('Origin',(-5.17275707706436,-5.26511162862565,-2.31)) ;
#163128=CARTESIAN_POINT('Ctrl Pts',(-5.9,-5.62807761009112,-2.31010664422313)) ;
#163129=CARTESIAN_POINT('Ctrl Pts',(-5.9,-5.54994729905279,-2.31006391978601)) ;
#163130=CARTESIAN_POINT('Ctrl Pts',(-5.82419006898363,-5.53104752404526,
-2.31005331321663)) ;
#163131=CARTESIAN_POINT('Ctrl Pts',(-5.9,-5.628107715576,-2.25756343754707)) ;
#163132=CARTESIAN_POINT('Ctrl Pts',(-5.9,-5.54996909580664,-2.27857515854929)) ;
#163133=CARTESIAN_POINT('Ctrl Pts',(-5.82419360391713,-5.53106345572106,
-2.28378608945993)) ;
#163134=CARTESIAN_POINT('Ctrl Pts',(-5.9,-5.6058853305092,-2.20562758429065)) ;
#163135=CARTESIAN_POINT('Ctrl Pts',(-5.89999999999998,-5.53371219741588,
-2.24753180215848)) ;
#163136=CARTESIAN_POINT('Ctrl Pts',(-5.82157770712952,-5.51930255765375,
-2.25782233263586)) ;
#163137=CARTESIAN_POINT('Ctrl Pts',(-5.9,-5.52950698295218,-2.13152970323473)) ;
#163138=CARTESIAN_POINT('Ctrl Pts',(-5.90000000000002,-5.48352164712826,
-2.20970178237743)) ;
#163139=CARTESIAN_POINT('Ctrl Pts',(-5.81258729511713,-5.47887520585223,
-2.22077370454031)) ;
#163140=CARTESIAN_POINT('Ctrl Pts',(-5.9,-5.47597273077139,-2.109970822884)) ;
#163141=CARTESIAN_POINT('Ctrl Pts',(-5.9,-5.44963575044054,-2.20388689509175)) ;
#163142=CARTESIAN_POINT('Ctrl Pts',(-5.80628621775611,-5.45053795385126,
-2.20999016864012)) ;
#163143=CARTESIAN_POINT('Ctrl Pts',(-5.9,-5.42181243301047,-2.11000002963748)) ;
#163144=CARTESIAN_POINT('Ctrl Pts',(-5.9,-5.42186418462488,-2.21008818447338)) ;
#163145=CARTESIAN_POINT('Ctrl Pts',(-5.79991187715166,-5.42186416305551,
-2.20999997682299)) ;
#163146=CARTESIAN_POINT('Origin',(-5.79999999999999,-5.42192235935953,-2.31000000000002)) ;
#163147=CARTESIAN_POINT('Origin',(-5.8066065036801,-5.42357398527959,-2.31)) ;
#163148=CARTESIAN_POINT('Origin',(-5.8,-5.05,-5.92)) ;
#163149=CARTESIAN_POINT('',(-5.87071067811865,-1.15,-5.99071067811865)) ;
#163150=CARTESIAN_POINT('Origin',(-5.81947611583159,-1.02473736077622,-5.92807935738799)) ;
#163151=CARTESIAN_POINT('Origin',(-5.80807935817055,-1.27526264085863,-5.93947611975157)) ;
#163152=CARTESIAN_POINT('',(-5.82425356250363,-5.43404914061138,-6.01701425001453)) ;
#163153=CARTESIAN_POINT('Origin',(-5.79999999999984,-5.42192235935956,-5.91999999998403)) ;
#163154=CARTESIAN_POINT('',(-5.87882054380159,-5.50499519875994,-5.98154122094028)) ;
#163155=CARTESIAN_POINT('Origin',(-5.79625409004975,-5.63940739348982,-5.91433454802145)) ;
#163156=CARTESIAN_POINT('Origin',(-5.80048106423751,-5.62703482768928,-5.92027064077534)) ;
#163157=CARTESIAN_POINT('Origin',(-5.8,-5.62807764064044,-36.59)) ;
#163158=CARTESIAN_POINT('',(-5.87882054380158,-5.56653641970014,-6.04308244188047)) ;
#163159=CARTESIAN_POINT('Origin',(-5.80050013342543,-5.62780271840948,-5.92105207279234)) ;
#163160=CARTESIAN_POINT('Origin',(-5.7962598489436,-5.63373078324888,-5.90869550130923)) ;
#163161=CARTESIAN_POINT('',(-5.87882054380156,-5.56653641970012,-9.19691755811957)) ;
#163162=CARTESIAN_POINT('Origin',(-5.79625409005666,-5.6337430926113,-9.33132975283448)) ;
#163163=CARTESIAN_POINT('Origin',(-5.80048106423679,-5.6278069998655,-9.31895718704807)) ;
#163164=CARTESIAN_POINT('Origin',(-5.8,-1.00857864376269,-36.59)) ;
#163165=CARTESIAN_POINT('Origin',(-5.81947611583159,-1.01665800115047,-5.93615871701256)) ;
#163166=CARTESIAN_POINT('Origin',(-5.81947611583101,-1.0166580011502,-9.30384128298823)) ;
#163167=CARTESIAN_POINT('Origin',(-5.8,-6.55,-9.32)) ;
#163168=CARTESIAN_POINT('',(-5.87882054380161,-5.50499519875992,-9.25845877905974)) ;
#163169=CARTESIAN_POINT('Origin',(-5.80050013341907,-5.62702556785333,-9.31972507777035)) ;
#163170=CARTESIAN_POINT('',(-5.82425356250363,-5.43404914061138,-9.22298574998547)) ;
#163171=CARTESIAN_POINT('Origin',(-5.79625984894763,-5.63938213931645,-9.3256531426013)) ;
#163172=CARTESIAN_POINT('Origin',(-5.79999999997662,-5.42192235934795,-9.32000000018081)) ;
#163173=CARTESIAN_POINT('',(-5.87071067811866,-1.14999999999999,-9.24928932188135)) ;
#163174=CARTESIAN_POINT('Origin',(-5.80807935817046,-1.27526264085876,-9.30052388024865)) ;
#163175=CARTESIAN_POINT('Origin',(-5.81947611583072,-1.02473736077575,-9.3119206426126)) ;
#163176=CARTESIAN_POINT('Origin',(-5.8,-5.05,-9.73)) ;
#163177=CARTESIAN_POINT('',(-5.87071067811865,-1.14999999999999,-9.80071067811865)) ;
#163178=CARTESIAN_POINT('Origin',(-5.81947611583089,-1.02473736077631,-9.73807935738754)) ;
#163179=CARTESIAN_POINT('Origin',(-5.80807935817105,-1.27526264085796,-9.74947611975234)) ;
#163180=CARTESIAN_POINT('',(-5.82425356250363,-5.43404914061138,-9.82701425001453)) ;
#163181=CARTESIAN_POINT('Origin',(-5.80000000000621,-5.42192235936274,-9.73000000003557)) ;
#163182=CARTESIAN_POINT('',(-5.87882054380157,-5.50499519875999,-9.79154122094031)) ;
#163183=CARTESIAN_POINT('Origin',(-5.79625409004102,-5.6394073935196,-9.72433454800673)) ;
#163184=CARTESIAN_POINT('Origin',(-5.80048106424258,-5.62703482768541,-9.73027064077687)) ;
#163185=CARTESIAN_POINT('Origin',(-5.8,-5.62807764064044,-36.59)) ;
#163186=CARTESIAN_POINT('',(-5.87882054380156,-5.56653641970012,-9.85308244188044)) ;
#163187=CARTESIAN_POINT('Origin',(-5.80050013342664,-5.62780271840903,-9.73105207279395)) ;
#163188=CARTESIAN_POINT('Origin',(-5.79625984896595,-5.63373078321645,-9.71869550137418)) ;
#163189=CARTESIAN_POINT('',(-5.87882054380156,-5.56653641970012,-13.0069175581196)) ;
#163190=CARTESIAN_POINT('Origin',(-5.79625409005982,-5.63374309260352,-13.1413297528191)) ;
#163191=CARTESIAN_POINT('Origin',(-5.80048106424012,-5.62780699986454,-13.1289571870464)) ;
#163192=CARTESIAN_POINT('Origin',(-5.8,-1.00857864376269,-36.59)) ;
#163193=CARTESIAN_POINT('Origin',(-5.81947611583026,-1.01665800114985,-9.7461587170121)) ;
#163194=CARTESIAN_POINT('Origin',(-5.81947611583107,-1.01665800115014,-13.1138412829883)) ;
#163195=CARTESIAN_POINT('Origin',(-5.8,-6.55,-13.13)) ;
#163196=CARTESIAN_POINT('',(-5.87882054380161,-5.50499519875992,-13.0684587790597)) ;
#163197=CARTESIAN_POINT('Origin',(-5.80050013342204,-5.62702556785267,-13.1297250777694)) ;
#163198=CARTESIAN_POINT('',(-5.82425356250363,-5.43404914061138,-13.0329857499855)) ;
#163199=CARTESIAN_POINT('Origin',(-5.79625984894408,-5.6393821393244,-13.135653142605)) ;
#163200=CARTESIAN_POINT('Origin',(-5.79999999997599,-5.42192235934763,-13.1300000002057)) ;
#163201=CARTESIAN_POINT('',(-5.87071067811866,-1.14999999999999,-13.0592893218813)) ;
#163202=CARTESIAN_POINT('Origin',(-5.80807935817108,-1.27526264085755,-13.1105238802474)) ;
#163203=CARTESIAN_POINT('Origin',(-5.81947611582975,-1.02473736077495,-13.121920642613)) ;
#163204=CARTESIAN_POINT('Origin',(-5.8,-5.05,-13.54)) ;
#163205=CARTESIAN_POINT('',(-5.87071067811865,-1.14999999999999,-13.6107106781187)) ;
#163206=CARTESIAN_POINT('Origin',(-5.8194761158307,-1.02473736077617,-13.5480793573875)) ;
#163207=CARTESIAN_POINT('Origin',(-5.80807935817103,-1.27526264085801,-13.5594761197523)) ;
#163208=CARTESIAN_POINT('',(-5.82425356250363,-5.43404914061138,-13.6370142500145)) ;
#163209=CARTESIAN_POINT('Origin',(-5.79999999999483,-5.42192235935705,-13.5399999999823)) ;
#163210=CARTESIAN_POINT('',(-5.87882054380157,-5.50499519875999,-13.6015412209403)) ;
#163211=CARTESIAN_POINT('Origin',(-5.79625409003451,-5.63940739354352,-13.5343345479947)) ;
#163212=CARTESIAN_POINT('Origin',(-5.80048106423289,-5.62703482768967,-13.5402706407743)) ;
#163213=CARTESIAN_POINT('Origin',(-5.8,-5.62807764064044,-36.59)) ;
#163214=CARTESIAN_POINT('',(-5.87882054380156,-5.56653641970012,-13.6630824418804)) ;
#163215=CARTESIAN_POINT('Origin',(-5.80050013342366,-5.62780271841002,-13.5410520727912)) ;
#163216=CARTESIAN_POINT('Origin',(-5.79625984897398,-5.63373078320201,-13.5286955014033)) ;
#163217=CARTESIAN_POINT('',(-5.8788205438016,-5.56653641970017,-16.8169175581195)) ;
#163218=CARTESIAN_POINT('Origin',(-5.79625409000273,-5.63374309268844,-16.9513297529886)) ;
#163219=CARTESIAN_POINT('Origin',(-5.80048106422758,-5.62780699986791,-16.9389571870545)) ;
#163220=CARTESIAN_POINT('Origin',(-5.8,-1.00857864376269,-36.59)) ;
#163221=CARTESIAN_POINT('Origin',(-5.81947611583107,-1.01665800115022,-13.5561587170129)) ;
#163222=CARTESIAN_POINT('Origin',(-5.81947611583164,-1.01665800115088,-16.9238412829861)) ;
#163223=CARTESIAN_POINT('Origin',(-5.8,-6.55,-16.94)) ;
#163224=CARTESIAN_POINT('',(-5.87882054380158,-5.50499519875998,-16.8784587790597)) ;
#163225=CARTESIAN_POINT('Origin',(-5.800500133426,-5.62702556784527,-16.9397250777684)) ;
#163226=CARTESIAN_POINT('',(-5.82425356250363,-5.43404914061138,-16.8429857499855)) ;
#163227=CARTESIAN_POINT('Origin',(-5.79625984893017,-5.63938213937326,-16.9456531426293)) ;
#163228=CARTESIAN_POINT('Origin',(-5.79999999994122,-5.42192235933025,-16.9400000004754)) ;
#163229=CARTESIAN_POINT('',(-5.87071067811866,-1.14999999999999,-16.8692893218814)) ;
#163230=CARTESIAN_POINT('Origin',(-5.80807935817212,-1.27526264085654,-16.9205238802451)) ;
#163231=CARTESIAN_POINT('Origin',(-5.81947611583181,-1.02473736077525,-16.9319206426127)) ;
#163232=CARTESIAN_POINT('Origin',(-5.8,-5.05,-17.35)) ;
#163233=CARTESIAN_POINT('',(-5.87071067811865,-1.14999999999999,-17.4207106781187)) ;
#163234=CARTESIAN_POINT('Origin',(-5.81947611583148,-1.02473736077474,-17.3580793573875)) ;
#163235=CARTESIAN_POINT('Origin',(-5.8080793581705,-1.27526264085864,-17.3694761197517)) ;
#163236=CARTESIAN_POINT('',(-5.82425356250363,-5.43404914061138,-17.4470142500145)) ;
#163237=CARTESIAN_POINT('Origin',(-5.79999999996682,-5.42192235934304,-17.3499999997148)) ;
#163238=CARTESIAN_POINT('',(-5.87882054380156,-5.50499519876001,-17.4115412209403)) ;
#163239=CARTESIAN_POINT('Origin',(-5.79625409003878,-5.63940739353005,-17.3443345480014)) ;
#163240=CARTESIAN_POINT('Origin',(-5.80048106423185,-5.62703482769178,-17.350270640774)) ;
#163241=CARTESIAN_POINT('Origin',(-5.8,-5.62807764064044,-36.59)) ;
#163242=CARTESIAN_POINT('',(-5.8788205438016,-5.56653641970017,-17.4730824418805)) ;
#163243=CARTESIAN_POINT('Origin',(-5.80050013342676,-5.6278027184087,-17.3510520727938)) ;
#163244=CARTESIAN_POINT('Origin',(-5.79625984893998,-5.63373078325259,-17.338695501302)) ;
#163245=CARTESIAN_POINT('',(-5.8788205438016,-5.56653641970017,-20.6269175581195)) ;
#163246=CARTESIAN_POINT('Origin',(-5.7962540900391,-5.63374309263502,-20.7613297528817)) ;
#163247=CARTESIAN_POINT('Origin',(-5.80048106423735,-5.62780699986498,-20.7489571870481)) ;
#163248=CARTESIAN_POINT('Origin',(-5.8,-1.00857864376269,-36.59)) ;
#163249=CARTESIAN_POINT('Origin',(-5.81947611583098,-1.0166580011507,-17.3661587170137)) ;
#163250=CARTESIAN_POINT('Origin',(-5.8194761158317,-1.01665800115097,-20.7338412829858)) ;
#163251=CARTESIAN_POINT('Origin',(-5.8,-6.55,-20.75)) ;
#163252=CARTESIAN_POINT('',(-5.87882054380158,-5.50499519875998,-20.6884587790597)) ;
#163253=CARTESIAN_POINT('Origin',(-5.80050013342497,-5.62702556784867,-20.7497250777695)) ;
#163254=CARTESIAN_POINT('',(-5.82425356250363,-5.43404914061138,-20.6529857499855)) ;
#163255=CARTESIAN_POINT('Origin',(-5.7962598489347,-5.63938213935898,-20.7556531426222)) ;
#163256=CARTESIAN_POINT('Origin',(-5.79999999987016,-5.42192235929471,-20.750000001076)) ;
#163257=CARTESIAN_POINT('',(-5.87071067811866,-1.14999999999999,-20.6792893218814)) ;
#163258=CARTESIAN_POINT('Origin',(-5.80807935817138,-1.27526264085804,-20.7305238802469)) ;
#163259=CARTESIAN_POINT('Origin',(-5.81947611583102,-1.02473736077477,-20.741920642613)) ;
#163260=CARTESIAN_POINT('Origin',(-5.8,-5.05,-21.16)) ;
#163261=CARTESIAN_POINT('',(-5.87071067811865,-1.14999999999999,-21.2307106781187)) ;
#163262=CARTESIAN_POINT('Origin',(-5.81947611583222,-1.02473736077531,-21.1680793573878)) ;
#163263=CARTESIAN_POINT('Origin',(-5.80807935817091,-1.27526264085785,-21.1794761197522)) ;
#163264=CARTESIAN_POINT('',(-5.82425356250363,-5.43404914061138,-21.2570142500145)) ;
#163265=CARTESIAN_POINT('Origin',(-5.7999999999067,-5.42192235931299,-21.1599999992661)) ;
#163266=CARTESIAN_POINT('',(-5.87882054380156,-5.50499519876001,-21.2215412209403)) ;
#163267=CARTESIAN_POINT('Origin',(-5.7962540900276,-5.63940739356463,-21.1543345479843)) ;
#163268=CARTESIAN_POINT('Origin',(-5.80048106422407,-5.62703482769801,-21.1602706407706)) ;
#163269=CARTESIAN_POINT('Origin',(-5.8,-5.62807764064044,-36.59)) ;
#163270=CARTESIAN_POINT('',(-5.8788205438016,-5.56653641970017,-21.2830824418805)) ;
#163271=CARTESIAN_POINT('Origin',(-5.80050013342682,-5.62780271840868,-21.1610520727937)) ;
#163272=CARTESIAN_POINT('Origin',(-5.79625984898204,-5.63373078318931,-21.1486955014297)) ;
#163273=CARTESIAN_POINT('',(-5.8788205438016,-5.56653641970017,-24.4369175581195)) ;
#163274=CARTESIAN_POINT('Origin',(-5.79625409005601,-5.63374309260924,-24.5713297528292)) ;
#163275=CARTESIAN_POINT('Origin',(-5.80048106422965,-5.62780699986711,-24.5589571870534)) ;
#163276=CARTESIAN_POINT('Origin',(-5.8,-1.00857864376269,-36.59)) ;
#163277=CARTESIAN_POINT('Origin',(-5.81947611583065,-1.01665800115061,-21.1761587170135)) ;
#163278=CARTESIAN_POINT('Origin',(-5.81947611583029,-1.01665800115036,-24.5438412829871)) ;
#163279=CARTESIAN_POINT('Origin',(-5.8,-6.55,-24.56)) ;
#163280=CARTESIAN_POINT('',(-5.87882054380158,-5.50499519875998,-24.4984587790597)) ;
#163281=CARTESIAN_POINT('Origin',(-5.80050013343402,-5.62702556784164,-24.5597250777665)) ;
#163282=CARTESIAN_POINT('',(-5.82425356250363,-5.43404914061138,-24.4629857499855)) ;
#163283=CARTESIAN_POINT('Origin',(-5.79625984894703,-5.63938213932085,-24.5656531426033)) ;
#163284=CARTESIAN_POINT('Origin',(-5.79999999991183,-5.42192235931555,-24.5600000007655)) ;
#163285=CARTESIAN_POINT('',(-5.87071067811866,-1.14999999999999,-24.4892893218814)) ;
#163286=CARTESIAN_POINT('Origin',(-5.80807935817052,-1.27526264085979,-24.5405238802492)) ;
#163287=CARTESIAN_POINT('Origin',(-5.81947611583105,-1.02473736077468,-24.551920642613)) ;
#163288=CARTESIAN_POINT('Origin',(-5.8,-5.05,-24.97)) ;
#163289=CARTESIAN_POINT('',(-5.87071067811865,-1.14999999999999,-25.0407106781187)) ;
#163290=CARTESIAN_POINT('Origin',(-5.8194761158313,-1.02473736077457,-24.9780793573874)) ;
#163291=CARTESIAN_POINT('Origin',(-5.8080793581727,-1.27526264085426,-24.9894761197567)) ;
#163292=CARTESIAN_POINT('',(-5.82425356250363,-5.43404914061138,-25.0670142500145)) ;
#163293=CARTESIAN_POINT('Origin',(-5.80000000000354,-5.4219223593614,-24.9699999999744)) ;
#163294=CARTESIAN_POINT('',(-5.87882054380156,-5.50499519876001,-25.0315412209403)) ;
#163295=CARTESIAN_POINT('Origin',(-5.79625409003997,-5.63940739352596,-24.9643345480035)) ;
#163296=CARTESIAN_POINT('Origin',(-5.80048106421586,-5.62703482770278,-24.9702706407684)) ;
#163297=CARTESIAN_POINT('Origin',(-5.8,-5.62807764064044,-36.59)) ;
#163298=CARTESIAN_POINT('',(-5.8788205438016,-5.56653641970017,-25.0930824418805)) ;
#163299=CARTESIAN_POINT('Origin',(-5.80050013342709,-5.62780271840868,-24.971052072793)) ;
#163300=CARTESIAN_POINT('Origin',(-5.79625984896229,-5.63373078321765,-24.9586955013721)) ;
#163301=CARTESIAN_POINT('',(-5.8788205438016,-5.56653641970017,-28.2469175581195)) ;
#163302=CARTESIAN_POINT('Origin',(-5.79625409004022,-5.63374309263231,-28.3813297528758)) ;
#163303=CARTESIAN_POINT('Origin',(-5.80048106423845,-5.62780699986491,-28.3689571870478)) ;
#163304=CARTESIAN_POINT('Origin',(-5.8,-1.00857864376269,-36.59)) ;
#163305=CARTESIAN_POINT('Origin',(-5.81947611583176,-1.01665800115109,-24.9861587170145)) ;
#163306=CARTESIAN_POINT('Origin',(-5.81947611583163,-1.01665800115093,-28.3538412829859)) ;
#163307=CARTESIAN_POINT('Origin',(-5.8,-6.55,-28.37)) ;
#163308=CARTESIAN_POINT('',(-5.87882054380158,-5.50499519875998,-28.3084587790597)) ;
#163309=CARTESIAN_POINT('Origin',(-5.80050013342543,-5.62702556784578,-28.3697250777687)) ;
#163310=CARTESIAN_POINT('',(-5.82425356250363,-5.43404914061138,-28.2729857499855)) ;
#163311=CARTESIAN_POINT('Origin',(-5.79625984893296,-5.63938213936453,-28.375653142625)) ;
#163312=CARTESIAN_POINT('Origin',(-5.79999999972037,-5.42192235921982,-28.3700000022139)) ;
#163313=CARTESIAN_POINT('',(-5.87071067811866,-1.14999999999999,-28.2992893218814)) ;
#163314=CARTESIAN_POINT('Origin',(-5.80807935817205,-1.2752626408567,-28.3505238802449)) ;
#163315=CARTESIAN_POINT('Origin',(-5.81947611583196,-1.02473736077544,-28.3619206426126)) ;
#163316=CARTESIAN_POINT('Origin',(-5.8,-5.05,-28.78)) ;
#163317=CARTESIAN_POINT('',(-5.87071067811865,-1.14999999999999,-28.8507106781187)) ;
#163318=CARTESIAN_POINT('Origin',(-5.81947611583263,-1.02473736077566,-28.788079357388)) ;
#163319=CARTESIAN_POINT('Origin',(-5.80807935817064,-1.27526264085834,-28.799476119752)) ;
#163320=CARTESIAN_POINT('',(-5.82425356250363,-5.43404914061138,-28.8770142500145)) ;
#163321=CARTESIAN_POINT('Origin',(-5.80000000005041,-5.42192235938484,-28.7800000004842)) ;
#163322=CARTESIAN_POINT('',(-5.87882054380157,-5.50499519876,-28.8415412209403)) ;
#163323=CARTESIAN_POINT('Origin',(-5.79625409004087,-5.63940739352319,-28.7743345480048)) ;
#163324=CARTESIAN_POINT('Origin',(-5.80048106422166,-5.62703482769908,-28.7802706407702)) ;
#163325=CARTESIAN_POINT('Origin',(-5.8,-5.62807764064044,-36.59)) ;
#163326=CARTESIAN_POINT('',(-5.8788205438016,-5.56653641970017,-28.9030824418805)) ;
#163327=CARTESIAN_POINT('Origin',(-5.80050013342867,-5.62780271840836,-28.7810520727939)) ;
#163328=CARTESIAN_POINT('Origin',(-5.79625984893701,-5.63373078325649,-28.7686955012943)) ;
#163329=CARTESIAN_POINT('',(-5.87882054380161,-5.56653641970018,-32.0569175581195)) ;
#163330=CARTESIAN_POINT('Origin',(-5.79625409009991,-5.63374309254529,-32.1913297527016)) ;
#163331=CARTESIAN_POINT('Origin',(-5.80048106422874,-5.62780699986764,-32.1789571870542)) ;
#163332=CARTESIAN_POINT('Origin',(-5.8,-1.00857864376269,-36.59)) ;
#163333=CARTESIAN_POINT('Origin',(-5.8194761158303,-1.01665800115047,-28.7961587170133)) ;
#163334=CARTESIAN_POINT('Origin',(-5.81947611583233,-1.01665800115071,-32.1638412829882)) ;
#163335=CARTESIAN_POINT('Origin',(-5.8,-6.55,-32.18)) ;
#163336=CARTESIAN_POINT('',(-5.87882054380161,-5.50499519875991,-32.1184587790597)) ;
#163337=CARTESIAN_POINT('Origin',(-5.80050013341193,-5.627025567861,-32.1797250777728)) ;
#163338=CARTESIAN_POINT('',(-5.82425356250363,-5.43404914061138,-32.0829857499855)) ;
#163339=CARTESIAN_POINT('Origin',(-5.79625984894212,-5.63938213933443,-32.1856531426101)) ;
#163340=CARTESIAN_POINT('Origin',(-5.79999999989758,-5.42192235930843,-32.1800000008904)) ;
#163341=CARTESIAN_POINT('',(-5.87071067811866,-1.14999999999999,-32.1092893218813)) ;
#163342=CARTESIAN_POINT('Origin',(-5.80807935817142,-1.27526264085807,-32.1605238802468)) ;
#163343=CARTESIAN_POINT('Origin',(-5.81947611582863,-1.02473736077885,-32.1719206426146)) ;
#163344=CARTESIAN_POINT('Origin',(-5.8,-5.05,-32.59)) ;
#163345=CARTESIAN_POINT('',(-5.87071067811865,-1.14999999999999,-32.6607106781187)) ;
#163346=CARTESIAN_POINT('Origin',(-5.81947611582916,-1.02473736077846,-32.5980793573863)) ;
#163347=CARTESIAN_POINT('Origin',(-5.80807935817332,-1.27526264085422,-32.6094761197577)) ;
#163348=CARTESIAN_POINT('',(-5.82425356250363,-5.43404914061138,-32.6870142500145)) ;
#163349=CARTESIAN_POINT('Origin',(-5.80000000004998,-5.42192235938451,-32.5900000003247)) ;
#163350=CARTESIAN_POINT('',(-5.87882054380129,-5.50499519876057,-32.6515412209407)) ;
#163351=CARTESIAN_POINT('Origin',(-5.79625409004923,-5.63940739351318,-32.5843345480113)) ;
#163352=CARTESIAN_POINT('Origin',(-5.80048106428436,-5.62703482765259,-32.5902706407885)) ;
#163353=CARTESIAN_POINT('Origin',(-5.8,-5.62807764064044,-36.59)) ;
#163354=CARTESIAN_POINT('',(-5.87882054380161,-5.56653641970018,-32.7130824418805)) ;
#163355=CARTESIAN_POINT('Origin',(-5.80050013340937,-5.62780271841368,-32.5910520727818)) ;
#163356=CARTESIAN_POINT('Origin',(-5.7962598489414,-5.6337307832541,-32.5786955012984)) ;
#163357=CARTESIAN_POINT('',(-5.87882054380161,-5.56653641970018,-35.8669175581195)) ;
#163358=CARTESIAN_POINT('Origin',(-5.79625409008121,-5.63374309257359,-36.0013297527579)) ;
#163359=CARTESIAN_POINT('Origin',(-5.80048106425034,-5.62780699986083,-35.9889571870404)) ;
#163360=CARTESIAN_POINT('Origin',(-5.8,-1.00857864376269,-36.59)) ;
#163361=CARTESIAN_POINT('Origin',(-5.81947611583112,-1.01665800115005,-32.60615871701)) ;
#163362=CARTESIAN_POINT('Origin',(-5.81947611583247,-1.01665800115081,-35.973841282988)) ;
#163363=CARTESIAN_POINT('Origin',(-5.8,-6.55,-35.99)) ;
#163364=CARTESIAN_POINT('',(-5.87882054380161,-5.50499519875991,-35.9284587790597)) ;
#163365=CARTESIAN_POINT('Origin',(-5.80050013341824,-5.62702556785893,-35.9897250777713)) ;
#163366=CARTESIAN_POINT('',(-5.82425356250363,-5.43404914061138,-35.8929857499855)) ;
#163367=CARTESIAN_POINT('Origin',(-5.79625984893577,-5.63938213935148,-35.9956531426186)) ;
#163368=CARTESIAN_POINT('Origin',(-5.80000000007751,-5.42192235939839,-35.9899999994296)) ;
#163369=CARTESIAN_POINT('',(-5.87071067811866,-1.14999999999999,-35.9192893218814)) ;
#163370=CARTESIAN_POINT('Origin',(-5.80807935817112,-1.2752626408587,-35.9705238802469)) ;
#163371=CARTESIAN_POINT('Origin',(-5.81947611582896,-1.02473736077925,-35.9819206426144)) ;
#163372=CARTESIAN_POINT('Origin',(-3.,4.45,-4.91)) ;
#163373=CARTESIAN_POINT('Origin',(-2.1,4.45,-4.91)) ;
#163374=CARTESIAN_POINT('Origin',(-2.9,4.45,-4.91)) ;
#163375=CARTESIAN_POINT('Origin',(-2.9,4.45,-4.71)) ;
#163376=CARTESIAN_POINT('Origin',(-3.1,4.45,-4.71)) ;
#163377=CARTESIAN_POINT('Origin',(-2.9,4.45,-4.71)) ;
#163378=CARTESIAN_POINT('Origin',(-2.1,4.45,-4.71)) ;
#163379=CARTESIAN_POINT('Origin',(-2.1,4.45,-4.71)) ;
#163380=CARTESIAN_POINT('Origin',(-1.9,4.45,-4.71)) ;
#163381=CARTESIAN_POINT('Origin',(-3.1,4.45,-4.81)) ;
#163382=CARTESIAN_POINT('Origin',(-3.1,4.45,-2.91)) ;
#163383=CARTESIAN_POINT('Origin',(-2.9,4.4,-4.71)) ;
#163384=CARTESIAN_POINT('Origin',(-2.9,4.35,-4.71)) ;
#163385=CARTESIAN_POINT('Origin',(-1.95156391047391E-16,4.35,-4.71)) ;
#163386=CARTESIAN_POINT('Origin',(-2.1,4.35,-4.71)) ;
#163387=CARTESIAN_POINT('Origin',(-2.9,4.35,-4.71)) ;
#163388=CARTESIAN_POINT('Origin',(-2.1,4.4,-4.71)) ;
#163389=CARTESIAN_POINT('Origin',(-2.1,4.35,-4.71)) ;
#163390=CARTESIAN_POINT('Origin',(-1.9,4.45,-4.81)) ;
#163391=CARTESIAN_POINT('Origin',(-1.9,4.45,-2.91)) ;
#163392=CARTESIAN_POINT('Origin',(-3.,4.45,-2.71)) ;
#163393=CARTESIAN_POINT('Origin',(-2.9,4.45,-2.71)) ;
#163394=CARTESIAN_POINT('Origin',(-2.1,4.45,-2.71)) ;
#163395=CARTESIAN_POINT('Origin',(-2.9,4.45,-2.91)) ;
#163396=CARTESIAN_POINT('Origin',(-2.9,4.45,-2.91)) ;
#163397=CARTESIAN_POINT('Origin',(-2.9,4.35,-4.71)) ;
#163398=CARTESIAN_POINT('Origin',(-2.9,4.35,-4.71)) ;
#163399=CARTESIAN_POINT('Origin',(-2.1,4.35,-4.71)) ;
#163400=CARTESIAN_POINT('Origin',(-2.1,4.35,-4.71)) ;
#163401=CARTESIAN_POINT('Origin',(-2.1,4.45,-2.91)) ;
#163402=CARTESIAN_POINT('Origin',(-2.1,4.45,-2.91)) ;
#163403=CARTESIAN_POINT('Origin',(-2.9,4.4,-2.91)) ;
#163404=CARTESIAN_POINT('Origin',(-2.9,4.35,-2.91)) ;
#163405=CARTESIAN_POINT('Origin',(-2.9,4.35,-3.81)) ;
#163406=CARTESIAN_POINT('Origin',(-2.9,4.35,-2.91)) ;
#163407=CARTESIAN_POINT('Origin',(-2.1,4.35,-3.81)) ;
#163408=CARTESIAN_POINT('Origin',(-2.1,4.35,-2.91)) ;
#163409=CARTESIAN_POINT('Origin',(-2.1,4.4,-2.91)) ;
#163410=CARTESIAN_POINT('Origin',(-2.1,4.35,-2.91)) ;
#163411=CARTESIAN_POINT('Origin',(-2.9,4.35,-2.91)) ;
#163412=CARTESIAN_POINT('Origin',(-2.9,4.35,-2.91)) ;
#163413=CARTESIAN_POINT('Origin',(-2.1,4.35,-2.91)) ;
#163414=CARTESIAN_POINT('Origin',(-2.1,4.35,-2.91)) ;
#163415=CARTESIAN_POINT('Origin',(-1.95156391047391E-16,4.35,-2.91)) ;
#163416=CARTESIAN_POINT('Origin',(-2.25,4.25,-4.56)) ;
#163417=CARTESIAN_POINT('Origin',(-2.25,4.3,-4.56)) ;
#163418=CARTESIAN_POINT('Origin',(-2.25,4.3,-3.81)) ;
#163419=CARTESIAN_POINT('Origin',(-2.25,4.3,-3.06)) ;
#163420=CARTESIAN_POINT('Origin',(-2.25,4.3,-4.56)) ;
#163421=CARTESIAN_POINT('Origin',(-2.25,4.25,-3.06)) ;
#163422=CARTESIAN_POINT('Origin',(-2.25,4.3,-3.06)) ;
#163423=CARTESIAN_POINT('Origin',(-2.25,4.3,-4.56)) ;
#163424=CARTESIAN_POINT('Origin',(-2.25,4.3,-4.56)) ;
#163425=CARTESIAN_POINT('Origin',(-2.25,4.3,-3.06)) ;
#163426=CARTESIAN_POINT('Origin',(-2.25,4.3,-3.06)) ;
#163427=CARTESIAN_POINT('Origin',(-2.75,4.25,-4.56)) ;
#163428=CARTESIAN_POINT('Origin',(-2.75,4.3,-4.56)) ;
#163429=CARTESIAN_POINT('Origin',(-1.97127667724637E-17,4.3,-4.56)) ;
#163430=CARTESIAN_POINT('Origin',(-2.75,4.3,-4.56)) ;
#163431=CARTESIAN_POINT('Origin',(-1.97127667724637E-17,4.3,-3.06)) ;
#163432=CARTESIAN_POINT('Origin',(-2.75,4.3,-3.06)) ;
#163433=CARTESIAN_POINT('Origin',(-2.75,4.25,-3.06)) ;
#163434=CARTESIAN_POINT('Origin',(-2.75,4.3,-3.06)) ;
#163435=CARTESIAN_POINT('Origin',(-2.75,4.3,-4.56)) ;
#163436=CARTESIAN_POINT('Origin',(-2.75,4.3,-4.56)) ;
#163437=CARTESIAN_POINT('Origin',(-2.75,4.3,-3.06)) ;
#163438=CARTESIAN_POINT('Origin',(-2.75,4.3,-3.06)) ;
#163439=CARTESIAN_POINT('Origin',(-2.75,4.3,-3.81)) ;
#163440=CARTESIAN_POINT('Origin',(7.8,2.9,-4.21)) ;
#163441=CARTESIAN_POINT('Origin',(7.8,2.9,-4.21)) ;
#163442=CARTESIAN_POINT('Origin',(7.8,2.9,-3.41)) ;
#163443=CARTESIAN_POINT('Origin',(7.8,2.9,-3.41)) ;
#163444=CARTESIAN_POINT('Origin',(7.8,2.9,-3.41)) ;
#163445=CARTESIAN_POINT('Origin',(7.8,2.9,-4.21)) ;
#163446=CARTESIAN_POINT('Origin',(7.8,2.9,-4.21)) ;
#163447=CARTESIAN_POINT('Origin',(9.6,2.9,-3.41)) ;
#163448=CARTESIAN_POINT('Origin',(9.6,2.9,-3.41)) ;
#163449=CARTESIAN_POINT('Origin',(9.6,2.9,-4.21)) ;
#163450=CARTESIAN_POINT('Origin',(9.6,2.9,-4.21)) ;
#163451=CARTESIAN_POINT('Origin',(9.6,2.9,-3.41)) ;
#163452=CARTESIAN_POINT('Origin',(9.6,2.9,-3.41)) ;
#163453=CARTESIAN_POINT('Origin',(9.6,2.9,-4.21)) ;
#163454=CARTESIAN_POINT('Origin',(9.6,2.9,-4.21)) ;
#163455=CARTESIAN_POINT('Origin',(9.6,2.9,-4.21)) ;
#163456=CARTESIAN_POINT('Origin',(-0.183301359729408,3.45,-2.29296321352403)) ;
#163457=CARTESIAN_POINT('Origin',(0.249234641435079,3.15,-3.69377997802131)) ;
#163458=CARTESIAN_POINT('Origin',(-0.249234641435079,3.15,-3.92622002197869)) ;
#163459=CARTESIAN_POINT('Origin',(-1.04429375741423,3.45,-2.69445056217769)) ;
#163460=CARTESIAN_POINT('Origin',(10.1,-2.15,-6.71688040659058)) ;
#163461=CARTESIAN_POINT('Origin',(10.1,-2.15,-6.71688040659058)) ;
#163462=CARTESIAN_POINT('Origin',(10.1,-2.15,-6.71688040659058)) ;
#163463=CARTESIAN_POINT('Origin',(10.1,-2.15,-6.71688040659058)) ;
#163464=CARTESIAN_POINT('Origin',(10.1,-2.15,-7.62)) ;
#163465=CARTESIAN_POINT('Origin',(10.1,-2.15,-6.315)) ;
#163466=CARTESIAN_POINT('Origin',(10.2,-2.15,-6.71688040659058)) ;
#163467=CARTESIAN_POINT('Origin',(3.7,-2.15,-6.71688040659058)) ;
#163468=CARTESIAN_POINT('Origin',(10.1,-3.65625,-7.62)) ;
#163469=CARTESIAN_POINT('Origin',(10.1,-2.15,-8.52311959340943)) ;
#163470=CARTESIAN_POINT('Origin',(10.1,-3.65625,-6.315)) ;
#163471=CARTESIAN_POINT('Origin',(10.1,1.9,-6.315)) ;
#163472=CARTESIAN_POINT('Origin',(10.1,-2.15,-6.315)) ;
#163473=CARTESIAN_POINT('Origin',(10.1,-2.15,-6.315)) ;
#163474=CARTESIAN_POINT('Origin',(10.1,-2.15,-6.315)) ;
#163475=CARTESIAN_POINT('Origin',(3.7,-2.15,-6.71688040659058)) ;
#163476=CARTESIAN_POINT('Origin',(3.7,-2.32153024911032,-6.8197267659824)) ;
#163477=CARTESIAN_POINT('Origin',(3.7,-2.35,-6.71688040659058)) ;
#163478=CARTESIAN_POINT('Origin',(10.1,-2.15,-8.52311959340942)) ;
#163479=CARTESIAN_POINT('Origin',(10.1,-2.15,-8.52311959340942)) ;
#163480=CARTESIAN_POINT('Origin',(10.1,-2.15,-8.52311959340942)) ;
#163481=CARTESIAN_POINT('Origin',(10.1,1.9,-7.62)) ;
#163482=CARTESIAN_POINT('Origin',(10.1,1.9,-8.925)) ;
#163483=CARTESIAN_POINT('Origin',(10.1,1.9,-6.315)) ;
#163484=CARTESIAN_POINT('Origin',(10.2,-2.15,-6.315)) ;
#163485=CARTESIAN_POINT('Origin',(3.7,-2.15,-6.315)) ;
#163486=CARTESIAN_POINT('Origin',(3.7,-2.35,-6.215)) ;
#163487=CARTESIAN_POINT('Origin',(3.7,-2.35,-6.315)) ;
#163488=CARTESIAN_POINT('Origin',(3.7,-3.65625,-7.62)) ;
#163489=CARTESIAN_POINT('Origin',(3.7,-2.32153024911032,-8.4202732340176)) ;
#163490=CARTESIAN_POINT('Origin',(10.2,-2.15,-8.52311959340942)) ;
#163491=CARTESIAN_POINT('Origin',(3.7,-2.15,-8.52311959340942)) ;
#163492=CARTESIAN_POINT('Origin',(10.1,-2.15,-7.62)) ;
#163493=CARTESIAN_POINT('Origin',(10.1,-2.15,-8.925)) ;
#163494=CARTESIAN_POINT('Origin',(10.1,-3.65625,-8.925)) ;
#163495=CARTESIAN_POINT('Origin',(10.1,1.9,-8.925)) ;
#163496=CARTESIAN_POINT('Origin',(10.1,-2.15,-8.925)) ;
#163497=CARTESIAN_POINT('Origin',(3.7,-2.35,-6.315)) ;
#163498=CARTESIAN_POINT('Origin',(3.5,-2.35,-6.315)) ;
#163499=CARTESIAN_POINT('Origin',(3.7,-2.15,-8.52311959340942)) ;
#163500=CARTESIAN_POINT('Origin',(3.7,-2.35,-8.52311959340942)) ;
#163501=CARTESIAN_POINT('Origin',(10.1,-2.15,-8.925)) ;
#163502=CARTESIAN_POINT('Origin',(10.1,-2.15,-8.925)) ;
#163503=CARTESIAN_POINT('Origin',(3.6,1.9,-6.115)) ;
#163504=CARTESIAN_POINT('Origin',(3.5,1.9,-6.115)) ;
#163505=CARTESIAN_POINT('Origin',(2.7,1.9,-6.115)) ;
#163506=CARTESIAN_POINT('Origin',(3.5,6.44767184226083E-16,-6.315)) ;
#163507=CARTESIAN_POINT('Origin',(3.5,-5.15,-6.315)) ;
#163508=CARTESIAN_POINT('Origin',(3.7,-2.35,-8.495)) ;
#163509=CARTESIAN_POINT('Origin',(3.7,-2.35,-8.925)) ;
#163510=CARTESIAN_POINT('Origin',(3.6,-2.15,-8.925)) ;
#163511=CARTESIAN_POINT('Origin',(3.7,-2.15,-8.925)) ;
#163512=CARTESIAN_POINT('Origin',(2.7,1.9,-6.115)) ;
#163513=CARTESIAN_POINT('Origin',(2.7,1.9,-6.115)) ;
#163514=CARTESIAN_POINT('Origin',(3.5,-5.15,-6.315)) ;
#163515=CARTESIAN_POINT('Origin',(3.5,-5.15,-6.315)) ;
#163516=CARTESIAN_POINT('Origin',(3.5,-5.15,-6.315)) ;
#163517=CARTESIAN_POINT('Origin',(3.7,-2.35,-8.925)) ;
#163518=CARTESIAN_POINT('Origin',(3.5,-2.35,-8.925)) ;
#163519=CARTESIAN_POINT('Origin',(2.7,2.,-6.115)) ;
#163520=CARTESIAN_POINT('Origin',(2.7,-5.15,-6.115)) ;
#163521=CARTESIAN_POINT('Origin',(3.6,-5.15,-6.315)) ;
#163522=CARTESIAN_POINT('Origin',(2.7,-5.15,-6.315)) ;
#163523=CARTESIAN_POINT('Origin',(3.5,-5.15,0.)) ;
#163524=CARTESIAN_POINT('Origin',(3.5,-5.15,-8.925)) ;
#163525=CARTESIAN_POINT('Origin',(3.5,-7.22673459250807E-16,-8.925)) ;
#163526=CARTESIAN_POINT('Origin',(3.5,-5.15,-8.925)) ;
#163527=CARTESIAN_POINT('Origin',(2.7,-5.15,-6.315)) ;
#163528=CARTESIAN_POINT('Origin',(2.7,-5.35,-6.315)) ;
#163529=CARTESIAN_POINT('Origin',(3.5,-5.15,-8.925)) ;
#163530=CARTESIAN_POINT('Origin',(3.5,-5.15,-8.925)) ;
#163531=CARTESIAN_POINT('Origin',(2.7,-5.35,-6.215)) ;
#163532=CARTESIAN_POINT('Origin',(2.7,-5.35,-8.925)) ;
#163533=CARTESIAN_POINT('Origin',(3.6,-5.15,-8.925)) ;
#163534=CARTESIAN_POINT('Origin',(2.7,-5.15,-8.925)) ;
#163535=CARTESIAN_POINT('Origin',(3.6,1.9,-9.125)) ;
#163536=CARTESIAN_POINT('Origin',(3.5,1.9,-9.125)) ;
#163537=CARTESIAN_POINT('Origin',(2.7,1.9,-9.125)) ;
#163538=CARTESIAN_POINT('Origin',(2.7,1.9,-9.025)) ;
#163539=CARTESIAN_POINT('Origin',(2.7,1.9,-9.925)) ;
#163540=CARTESIAN_POINT('Origin',(2.7,1.9,-9.125)) ;
#163541=CARTESIAN_POINT('Origin',(2.7,-5.15,-8.925)) ;
#163542=CARTESIAN_POINT('Origin',(2.7,-5.15,-9.125)) ;
#163543=CARTESIAN_POINT('Origin',(2.7,1.9,-9.125)) ;
#163544=CARTESIAN_POINT('Origin',(2.7,1.9,-9.125)) ;
#163545=CARTESIAN_POINT('Origin',(2.7,-5.25,-9.125)) ;
#163546=CARTESIAN_POINT('Ctrl Pts',(-3.8,-6.55,-6.52)) ;
#163547=CARTESIAN_POINT('Ctrl Pts',(-3.8,-6.55,-6.52)) ;
#163548=CARTESIAN_POINT('Ctrl Pts',(-3.8,-6.55,-6.52)) ;
#163549=CARTESIAN_POINT('Ctrl Pts',(-3.82625343282635,-6.55,-6.57250686565274)) ;
#163550=CARTESIAN_POINT('Ctrl Pts',(-3.83954133268481,-6.55,-6.55954133268496)) ;
#163551=CARTESIAN_POINT('Ctrl Pts',(-3.85250686565268,-6.55,-6.54625343282645)) ;
#163552=CARTESIAN_POINT('Ctrl Pts',(-3.85219871729854,-6.53922263893877,
-6.62439743459706)) ;
#163553=CARTESIAN_POINT('Ctrl Pts',(-3.87914655110981,-6.52362528614068,
-6.59914655110983)) ;
#163554=CARTESIAN_POINT('Ctrl Pts',(-3.90439743459708,-6.53922263893878,
-6.57219871729853)) ;
#163555=CARTESIAN_POINT('Ctrl Pts',(-3.87996665852871,-6.5114546977086,
-6.67993331705744)) ;
#163556=CARTESIAN_POINT('Ctrl Pts',(-3.9028838031416,-6.48208554016478,
-6.6228838031416)) ;
#163557=CARTESIAN_POINT('Ctrl Pts',(-3.95993331705742,-6.51145469770859,
-6.59996665852872)) ;
#163558=CARTESIAN_POINT('Ctrl Pts',(-3.88737865704135,-6.5003618540841,
-6.69475731408271)) ;
#163559=CARTESIAN_POINT('Ctrl Pts',(-3.90501307588292,-6.46792722356047,
-6.62501307588294)) ;
#163560=CARTESIAN_POINT('Ctrl Pts',(-3.9747573140827,-6.5003618540841,-6.60737865704135)) ;
#163561=CARTESIAN_POINT('Ctrl Pts',(-3.8973972494609,-6.47617483238892,
-6.71479449892181)) ;
#163562=CARTESIAN_POINT('Ctrl Pts',(-3.90329674356411,-6.4509405986842,
-6.6232967435641)) ;
#163563=CARTESIAN_POINT('Ctrl Pts',(-3.99479449892181,-6.47617483238892,
-6.61739724946091)) ;
#163564=CARTESIAN_POINT('Ctrl Pts',(-3.9,-6.46309229646328,-6.71999999918177)) ;
#163565=CARTESIAN_POINT('Ctrl Pts',(-3.90000730397382,-6.44945650155155,
-6.62000730395969)) ;
#163566=CARTESIAN_POINT('Ctrl Pts',(-3.99999999918173,-6.46309229646328,
-6.62)) ;
#163567=CARTESIAN_POINT('Ctrl Pts',(-3.9,-6.45,-6.72)) ;
#163568=CARTESIAN_POINT('Ctrl Pts',(-3.9,-6.45,-6.62)) ;
#163569=CARTESIAN_POINT('Ctrl Pts',(-4.,-6.45,-6.62)) ;
#163570=CARTESIAN_POINT('Origin',(-4.,-6.45,-6.72)) ;
#163571=CARTESIAN_POINT('Origin',(-4.,-6.4,-6.72)) ;
#163572=CARTESIAN_POINT('Origin',(-4.,-6.35,-6.72)) ;
#163573=CARTESIAN_POINT('Ctrl Pts',(-5.,-6.55,-6.52)) ;
#163574=CARTESIAN_POINT('Ctrl Pts',(-5.,-6.55,-6.52)) ;
#163575=CARTESIAN_POINT('Ctrl Pts',(-5.,-6.55,-6.52)) ;
#163576=CARTESIAN_POINT('Ctrl Pts',(-4.94749313434726,-6.55,-6.54625343282631)) ;
#163577=CARTESIAN_POINT('Ctrl Pts',(-4.96045866731611,-6.55,-6.55954133268376)) ;
#163578=CARTESIAN_POINT('Ctrl Pts',(-4.97374656717359,-6.55,-6.57250686565269)) ;
#163579=CARTESIAN_POINT('Ctrl Pts',(-4.89560256540291,-6.53922263893877,
-6.57219871729855)) ;
#163580=CARTESIAN_POINT('Ctrl Pts',(-4.9208534488902,-6.52362528614071,
-6.59914655110988)) ;
#163581=CARTESIAN_POINT('Ctrl Pts',(-4.94780128270146,-6.53922263893877,
-6.62439743459709)) ;
#163582=CARTESIAN_POINT('Ctrl Pts',(-4.84006668294258,-6.5114546977086,
-6.59996665852871)) ;
#163583=CARTESIAN_POINT('Ctrl Pts',(-4.89711619685839,-6.48208554016476,
-6.62288380314157)) ;
#163584=CARTESIAN_POINT('Ctrl Pts',(-4.92003334147129,-6.5114546977086,
-6.67993331705742)) ;
#163585=CARTESIAN_POINT('Ctrl Pts',(-4.82524268591729,-6.5003618540841,
-6.60737865704136)) ;
#163586=CARTESIAN_POINT('Ctrl Pts',(-4.89498692411706,-6.46792722356047,
-6.62501307588293)) ;
#163587=CARTESIAN_POINT('Ctrl Pts',(-4.91262134295865,-6.5003618540841,
-6.6947573140827)) ;
#163588=CARTESIAN_POINT('Ctrl Pts',(-4.80520550107819,-6.47617483238892,
-6.61739724946091)) ;
#163589=CARTESIAN_POINT('Ctrl Pts',(-4.8967032564359,-6.4509405986842,-6.62329674356412)) ;
#163590=CARTESIAN_POINT('Ctrl Pts',(-4.90260275053909,-6.47617483238892,
-6.71479449892182)) ;
#163591=CARTESIAN_POINT('Ctrl Pts',(-4.80000000081823,-6.46309229646328,
-6.62)) ;
#163592=CARTESIAN_POINT('Ctrl Pts',(-4.89999269600723,-6.44945650155945,
-6.62000730395977)) ;
#163593=CARTESIAN_POINT('Ctrl Pts',(-4.9,-6.46309229646328,-6.71999999918177)) ;
#163594=CARTESIAN_POINT('Ctrl Pts',(-4.8,-6.45,-6.62)) ;
#163595=CARTESIAN_POINT('Ctrl Pts',(-4.9,-6.45,-6.62)) ;
#163596=CARTESIAN_POINT('Ctrl Pts',(-4.9,-6.45,-6.72)) ;
#163597=CARTESIAN_POINT('Origin',(-4.8,-6.45,-6.72)) ;
#163598=CARTESIAN_POINT('Origin',(-4.,-6.35,-6.72)) ;
#163599=CARTESIAN_POINT('Origin',(-4.,-6.35,-6.72)) ;
#163600=CARTESIAN_POINT('Origin',(-4.,-6.35,-6.72)) ;
#163601=CARTESIAN_POINT('Ctrl Pts',(-3.8,-6.55,-8.72)) ;
#163602=CARTESIAN_POINT('Ctrl Pts',(-3.8,-6.55,-8.72)) ;
#163603=CARTESIAN_POINT('Ctrl Pts',(-3.8,-6.55,-8.72)) ;
#163604=CARTESIAN_POINT('Ctrl Pts',(-3.8525068656527,-6.55,-8.69374656717358)) ;
#163605=CARTESIAN_POINT('Ctrl Pts',(-3.83954133268498,-6.55,-8.68045866731507)) ;
#163606=CARTESIAN_POINT('Ctrl Pts',(-3.82625343282636,-6.55,-8.66749313434729)) ;
#163607=CARTESIAN_POINT('Ctrl Pts',(-3.90439743459706,-6.53922263893877,
-8.66780128270146)) ;
#163608=CARTESIAN_POINT('Ctrl Pts',(-3.8791465511098,-6.52362528614071,
-8.64085344889018)) ;
#163609=CARTESIAN_POINT('Ctrl Pts',(-3.85219871729855,-6.53922263893876,
-8.61560256540292)) ;
#163610=CARTESIAN_POINT('Ctrl Pts',(-3.95993331705743,-6.5114546977086,
-8.64003334147129)) ;
#163611=CARTESIAN_POINT('Ctrl Pts',(-3.90288380314161,-6.48208554016476,
-8.6171161968584)) ;
#163612=CARTESIAN_POINT('Ctrl Pts',(-3.8799666585287,-6.5114546977086,-8.56006668294258)) ;
#163613=CARTESIAN_POINT('Ctrl Pts',(-3.97475731408271,-6.5003618540841,
-8.63262134295865)) ;
#163614=CARTESIAN_POINT('Ctrl Pts',(-3.90501307588293,-6.46792722356048,
-8.61498692411705)) ;
#163615=CARTESIAN_POINT('Ctrl Pts',(-3.88737865704135,-6.5003618540841,
-8.54524268591729)) ;
#163616=CARTESIAN_POINT('Ctrl Pts',(-3.9947944989218,-6.47617483238892,
-8.6226027505391)) ;
#163617=CARTESIAN_POINT('Ctrl Pts',(-3.9032967435641,-6.45094059868419,
-8.61670325643593)) ;
#163618=CARTESIAN_POINT('Ctrl Pts',(-3.89739724946091,-6.47617483238892,
-8.5252055010782)) ;
#163619=CARTESIAN_POINT('Ctrl Pts',(-3.99999999918176,-6.46309229646328,
-8.62)) ;
#163620=CARTESIAN_POINT('Ctrl Pts',(-3.90000730395526,-6.44945650152442,
-8.61999269608717)) ;
#163621=CARTESIAN_POINT('Ctrl Pts',(-3.9,-6.46309229646328,-8.52000000081831)) ;
#163622=CARTESIAN_POINT('Ctrl Pts',(-4.,-6.45,-8.62)) ;
#163623=CARTESIAN_POINT('Ctrl Pts',(-3.9,-6.45,-8.62)) ;
#163624=CARTESIAN_POINT('Ctrl Pts',(-3.9,-6.45,-8.52)) ;
#163625=CARTESIAN_POINT('Origin',(-4.,-6.45,-8.52)) ;
#163626=CARTESIAN_POINT('Origin',(-4.8,-6.4,-6.72)) ;
#163627=CARTESIAN_POINT('Origin',(-4.8,-6.35,-6.72)) ;
#163628=CARTESIAN_POINT('Origin',(1.9515639104739E-16,-6.35,-6.72000000000001)) ;
#163629=CARTESIAN_POINT('Origin',(-4.8,-6.35,-6.72)) ;
#163630=CARTESIAN_POINT('Origin',(-4.,-6.35,-7.62)) ;
#163631=CARTESIAN_POINT('Origin',(-4.,-6.35,-8.52)) ;
#163632=CARTESIAN_POINT('Origin',(-4.,-6.4,-8.52)) ;
#163633=CARTESIAN_POINT('Origin',(-4.,-6.35,-8.52)) ;
#163634=CARTESIAN_POINT('Origin',(-4.8,-6.35,-6.72)) ;
#163635=CARTESIAN_POINT('Origin',(-4.8,-6.35,-6.72)) ;
#163636=CARTESIAN_POINT('Origin',(-4.,-6.35,-8.52)) ;
#163637=CARTESIAN_POINT('Origin',(-4.,-6.35,-8.52)) ;
#163638=CARTESIAN_POINT('Origin',(-4.8,-6.35,-7.62)) ;
#163639=CARTESIAN_POINT('Origin',(-4.8,-6.35,-8.52)) ;
#163640=CARTESIAN_POINT('Origin',(1.95156391047391E-16,-6.35,-8.52)) ;
#163641=CARTESIAN_POINT('Origin',(-4.8,-6.35,-8.52)) ;
#163642=CARTESIAN_POINT('Origin',(-4.8,-6.35,-8.52)) ;
#163643=CARTESIAN_POINT('Origin',(-4.8,-6.35,-8.52)) ;
#163644=CARTESIAN_POINT('Origin',(-4.8,-6.4,-8.52)) ;
#163645=CARTESIAN_POINT('Origin',(-4.8,-6.45,-8.52)) ;
#163646=CARTESIAN_POINT('Ctrl Pts',(-5.,-6.55,-8.72)) ;
#163647=CARTESIAN_POINT('Ctrl Pts',(-5.,-6.55,-8.72)) ;
#163648=CARTESIAN_POINT('Ctrl Pts',(-5.,-6.55,-8.72)) ;
#163649=CARTESIAN_POINT('Ctrl Pts',(-4.97374656717352,-6.55,-8.66749313434731)) ;
#163650=CARTESIAN_POINT('Ctrl Pts',(-4.96045866731608,-6.55,-8.68045866731609)) ;
#163651=CARTESIAN_POINT('Ctrl Pts',(-4.94749313434721,-6.55,-8.69374656717377)) ;
#163652=CARTESIAN_POINT('Ctrl Pts',(-4.94780128270146,-6.53922263893877,
-8.61560256540297)) ;
#163653=CARTESIAN_POINT('Ctrl Pts',(-4.92085344889017,-6.52362528614071,
-8.64085344889023)) ;
#163654=CARTESIAN_POINT('Ctrl Pts',(-4.89560256540291,-6.53922263893879,
-8.66780128270149)) ;
#163655=CARTESIAN_POINT('Ctrl Pts',(-4.92003334147129,-6.5114546977086,
-8.56006668294255)) ;
#163656=CARTESIAN_POINT('Ctrl Pts',(-4.8971161968584,-6.48208554016476,
-8.61711619685837)) ;
#163657=CARTESIAN_POINT('Ctrl Pts',(-4.84006668294258,-6.51145469770858,
-8.64003334147128)) ;
#163658=CARTESIAN_POINT('Ctrl Pts',(-4.91262134295865,-6.5003618540841,
-8.54524268591729)) ;
#163659=CARTESIAN_POINT('Ctrl Pts',(-4.89498692411706,-6.46792722356048,
-8.61498692411705)) ;
#163660=CARTESIAN_POINT('Ctrl Pts',(-4.82524268591729,-6.5003618540841,
-8.63262134295865)) ;
#163661=CARTESIAN_POINT('Ctrl Pts',(-4.90260275053909,-6.47617483238892,
-8.5252055010782)) ;
#163662=CARTESIAN_POINT('Ctrl Pts',(-4.8967032564359,-6.45094059868419,
-8.61670325643593)) ;
#163663=CARTESIAN_POINT('Ctrl Pts',(-4.80520550107819,-6.47617483238892,
-8.6226027505391)) ;
#163664=CARTESIAN_POINT('Ctrl Pts',(-4.9,-6.46309229646328,-8.52000000081831)) ;
#163665=CARTESIAN_POINT('Ctrl Pts',(-4.89999269604004,-6.44945650152635,
-8.6199926960872)) ;
#163666=CARTESIAN_POINT('Ctrl Pts',(-4.80000000081823,-6.46309229646328,
-8.62)) ;
#163667=CARTESIAN_POINT('Ctrl Pts',(-4.9,-6.45,-8.52)) ;
#163668=CARTESIAN_POINT('Ctrl Pts',(-4.9,-6.45,-8.62)) ;
#163669=CARTESIAN_POINT('Ctrl Pts',(-4.8,-6.45,-8.62)) ;
#163670=CARTESIAN_POINT('Ctrl Pts',(-5.82426676739355,-5.43399303700595,
-6.01701096596876)) ;
#163671=CARTESIAN_POINT('Ctrl Pts',(-5.8026698877831,-5.52572360682934,
-6.02235401735037)) ;
#163672=CARTESIAN_POINT('Ctrl Pts',(-5.82426676352017,-5.53106667371342,
-6.11408458718272)) ;
#163673=CARTESIAN_POINT('Ctrl Pts',(-5.83498671931123,-5.43935351191891,
-6.01432945819615)) ;
#163674=CARTESIAN_POINT('Ctrl Pts',(-5.80595263122263,-5.52411753147702,
-6.02396009354016)) ;
#163675=CARTESIAN_POINT('Ctrl Pts',(-5.83498671397627,-5.53374818067469,
-6.10872411314632)) ;
#163676=CARTESIAN_POINT('Ctrl Pts',(-5.8452610584572,-5.44830326289477,
-6.00985284019614)) ;
#163677=CARTESIAN_POINT('Ctrl Pts',(-5.81370932746129,-5.52260132030851,
-6.02547630599891)) ;
#163678=CARTESIAN_POINT('Ctrl Pts',(-5.84526105243721,-5.53822479746339,
-6.0997743635698)) ;
#163679=CARTESIAN_POINT('Ctrl Pts',(-5.86378685403706,-5.47240020430389,
-5.99780325130861)) ;
#163680=CARTESIAN_POINT('Ctrl Pts',(-5.83531854275282,-5.52733067404477,
-6.02074695511457)) ;
#163681=CARTESIAN_POINT('Ctrl Pts',(-5.86378684816461,-5.550274384599,-6.07567742500549)) ;
#163682=CARTESIAN_POINT('Ctrl Pts',(-5.87203852631583,-5.48754495134725,
-5.99023155289433)) ;
#163683=CARTESIAN_POINT('Ctrl Pts',(-5.84834787930679,-5.53310199490444,
-6.01497563577601)) ;
#163684=CARTESIAN_POINT('Ctrl Pts',(-5.8720385212304,-5.55784608243457,
-6.06053267951394)) ;
#163685=CARTESIAN_POINT('Ctrl Pts',(-5.892427473048,-5.53981202333449,-5.96410565113754)) ;
#163686=CARTESIAN_POINT('Ctrl Pts',(-5.88223383300418,-5.56084219179273,
-5.9872354431742)) ;
#163687=CARTESIAN_POINT('Ctrl Pts',(-5.89242747063502,-5.58397198402774,
-6.00826561232782)) ;
#163688=CARTESIAN_POINT('Ctrl Pts',(-5.9,-5.58381083947293,-5.94211940014292)) ;
#163689=CARTESIAN_POINT('Ctrl Pts',(-5.9,-5.59485304502627,-5.95322459288698)) ;
#163690=CARTESIAN_POINT('Ctrl Pts',(-5.9,-5.60595823775499,-5.96426679844055)) ;
#163691=CARTESIAN_POINT('Ctrl Pts',(-5.9,-5.62807764064044,-5.92)) ;
#163692=CARTESIAN_POINT('Ctrl Pts',(-5.9,-5.62807764064044,-5.92)) ;
#163693=CARTESIAN_POINT('Ctrl Pts',(-5.9,-5.62807764064044,-5.92)) ;
#163694=CARTESIAN_POINT('Origin',(-5.84850712500726,-5.43404914061138,-6.11402850002907)) ;
#163695=CARTESIAN_POINT('Ctrl Pts',(-5.82425356250363,-5.53106339062591,
-6.11402850002907)) ;
#163696=CARTESIAN_POINT('Ctrl Pts',(-5.80269484027818,-5.52567371006955,
-6.0224039305709)) ;
#163697=CARTESIAN_POINT('Ctrl Pts',(-5.82425356250363,-5.43404914061138,
-6.01701425001453)) ;
#163698=CARTESIAN_POINT('Ctrl Pts',(-5.80840777707093,-5.52710194426774,
-6.11798994590434)) ;
#163699=CARTESIAN_POINT('Ctrl Pts',(-5.79341417645228,-5.52335354411309,
-6.0228358498184)) ;
#163700=CARTESIAN_POINT('Ctrl Pts',(-5.81633079157288,-5.43008775511759,
-6.01899494274722)) ;
#163701=CARTESIAN_POINT('Ctrl Pts',(-5.79207992677991,-5.52301998169498,
-6.11999999953396)) ;
#163702=CARTESIAN_POINT('Ctrl Pts',(-5.78430903206645,-5.52107725801661,
-6.02196139543286)) ;
#163703=CARTESIAN_POINT('Ctrl Pts',(-5.808166653183,-5.42600568595106,-6.02)) ;
#163704=CARTESIAN_POINT('Ctrl Pts',(-5.77574643749636,-5.51893660937409,
-6.12)) ;
#163705=CARTESIAN_POINT('Ctrl Pts',(-5.77574643749636,-5.51893660937409,
-6.02)) ;
#163706=CARTESIAN_POINT('Ctrl Pts',(-5.8,-5.42192235935956,-6.02)) ;
#163707=CARTESIAN_POINT('Origin',(-5.8,-5.42192235935956,-6.12)) ;
#163708=CARTESIAN_POINT('Origin',(-5.8066065036801,-5.42357398527959,-6.12)) ;
#163709=CARTESIAN_POINT('Origin',(-5.17275707706436,-5.26511162862565,-6.12)) ;
#163710=CARTESIAN_POINT('Origin',(-5.15068655017073,-5.25959399690224,-6.13059385290895)) ;
#163711=CARTESIAN_POINT('Origin',(-5.17275707706436,-5.26511162862565,-6.12)) ;
#163712=CARTESIAN_POINT('Origin',(-5.17275707706436,-5.26511162862565,-6.12)) ;
#163713=CARTESIAN_POINT('Origin',(-5.17275707706436,-5.26511162862565,-6.12)) ;
#163714=CARTESIAN_POINT('Origin',(-5.17275707706436,-5.05,-6.12)) ;
#163715=CARTESIAN_POINT('Origin',(-5.17275707706436,-1.91866427917294,-6.12)) ;
#163716=CARTESIAN_POINT('Origin',(-3.78014014831103,-3.31128120792626,-6.7884561258016)) ;
#163717=CARTESIAN_POINT('Origin',(-5.17275707706436,-1.91866427917294,-6.12)) ;
#163718=CARTESIAN_POINT('Origin',(-5.17275707706436,-1.91866427917293,-6.12)) ;
#163719=CARTESIAN_POINT('Origin',(-5.17275707706436,-1.91866427917294,-6.12)) ;
#163720=CARTESIAN_POINT('Origin',(-3.97071067811865,-3.12071067811865,-6.12)) ;
#163721=CARTESIAN_POINT('Origin',(-5.8,-1.2914213562373,-6.12)) ;
#163722=CARTESIAN_POINT('Ctrl Pts',(-5.87071067811865,-1.14999999999999,
-5.99071067811865)) ;
#163723=CARTESIAN_POINT('Ctrl Pts',(-5.8471404520791,-1.10285954792089,
-6.01428090415821)) ;
#163724=CARTESIAN_POINT('Ctrl Pts',(-5.87071067811865,-1.07928932188134,
-6.06142135623731)) ;
#163725=CARTESIAN_POINT('Ctrl Pts',(-5.85217562795663,-1.18707010095462,
-6.00924572828067)) ;
#163726=CARTESIAN_POINT('Ctrl Pts',(-5.81261165662048,-1.13738834337934,
-6.03586147194932)) ;
#163727=CARTESIAN_POINT('Ctrl Pts',(-5.83353949671043,-1.11646050328957,
-6.09859253638095)) ;
#163728=CARTESIAN_POINT('Ctrl Pts',(-5.82627077431954,-1.23887980759834,
-6.02)) ;
#163729=CARTESIAN_POINT('Ctrl Pts',(-5.76566787907959,-1.18433212092047,
-6.037148943713)) ;
#163730=CARTESIAN_POINT('Ctrl Pts',(-5.78190678732234,-1.16809321267766,
-6.11999999941873)) ;
#163731=CARTESIAN_POINT('Ctrl Pts',(-5.8,-1.2914213562373,-6.02)) ;
#163732=CARTESIAN_POINT('Ctrl Pts',(-5.72928932188134,-1.22071067811865,
-6.02)) ;
#163733=CARTESIAN_POINT('Ctrl Pts',(-5.72928932188134,-1.22071067811865,
-6.12)) ;
#163734=CARTESIAN_POINT('Origin',(-5.94142135623731,-1.15,-6.06142135623731)) ;
#163735=CARTESIAN_POINT('Ctrl Pts',(-5.9,-1.00857864376269,-5.92)) ;
#163736=CARTESIAN_POINT('Ctrl Pts',(-5.9,-1.00857864376269,-5.92)) ;
#163737=CARTESIAN_POINT('Ctrl Pts',(-5.9,-1.00857864376269,-5.92)) ;
#163738=CARTESIAN_POINT('Ctrl Pts',(-5.9,-1.0611201924017,-5.94627077431948)) ;
#163739=CARTESIAN_POINT('Ctrl Pts',(-5.9,-1.04860238143826,-5.9600237376757)) ;
#163740=CARTESIAN_POINT('Ctrl Pts',(-5.9,-1.03484941808215,-5.97254154863899)) ;
#163741=CARTESIAN_POINT('Ctrl Pts',(-5.88924572828065,-1.11292989904533,
-5.97217562795666)) ;
#163742=CARTESIAN_POINT('Ctrl Pts',(-5.8745170062455,-1.08721613124893,
-5.99863748748648)) ;
#163743=CARTESIAN_POINT('Ctrl Pts',(-5.88924572828069,-1.0607542717193,
-6.02435125528271)) ;
#163744=CARTESIAN_POINT('Ctrl Pts',(-5.87071067811865,-1.14999999999999,
-5.99071067811865)) ;
#163745=CARTESIAN_POINT('Ctrl Pts',(-5.8471404520791,-1.10285954792089,
-6.01428090415821)) ;
#163746=CARTESIAN_POINT('Ctrl Pts',(-5.87071067811865,-1.07928932188134,
-6.06142135623731)) ;
#163747=CARTESIAN_POINT('Ctrl Pts',(-5.87071067811866,-1.14999999999999,
-9.24928932188135)) ;
#163748=CARTESIAN_POINT('Ctrl Pts',(-5.84714045207911,-1.10285954792089,
-9.2257190958418)) ;
#163749=CARTESIAN_POINT('Ctrl Pts',(-5.87071067811866,-1.07928932188134,
-9.1785786437627)) ;
#163750=CARTESIAN_POINT('Ctrl Pts',(-5.88924572828065,-1.11292989904533,
-9.26782437204335)) ;
#163751=CARTESIAN_POINT('Ctrl Pts',(-5.87451700627504,-1.08721613123207,
-9.24136251253051)) ;
#163752=CARTESIAN_POINT('Ctrl Pts',(-5.8892457282807,-1.06075427171929,
-9.21564874471729)) ;
#163753=CARTESIAN_POINT('Ctrl Pts',(-5.9,-1.06112019240166,-9.29372922568044)) ;
#163754=CARTESIAN_POINT('Ctrl Pts',(-5.9,-1.04860238145159,-9.27997626231091)) ;
#163755=CARTESIAN_POINT('Ctrl Pts',(-5.9,-1.03484941808214,-9.26745845136102)) ;
#163756=CARTESIAN_POINT('Ctrl Pts',(-5.9,-1.00857864376269,-9.32)) ;
#163757=CARTESIAN_POINT('Ctrl Pts',(-5.9,-1.00857864376269,-9.32)) ;
#163758=CARTESIAN_POINT('Ctrl Pts',(-5.9,-1.00857864376269,-9.32)) ;
#163759=CARTESIAN_POINT('Origin',(-5.94142135623734,-1.14999999999996,-9.17857864376272)) ;
#163760=CARTESIAN_POINT('Ctrl Pts',(-5.8,-1.2914213562373,-9.22)) ;
#163761=CARTESIAN_POINT('Ctrl Pts',(-5.72928932188134,-1.22071067811865,
-9.22)) ;
#163762=CARTESIAN_POINT('Ctrl Pts',(-5.72928932188134,-1.22071067811865,
-9.12)) ;
#163763=CARTESIAN_POINT('Ctrl Pts',(-5.82627077431945,-1.23887980759835,
-9.22)) ;
#163764=CARTESIAN_POINT('Ctrl Pts',(-5.76566787907942,-1.18433212092059,
-9.2028510562869)) ;
#163765=CARTESIAN_POINT('Ctrl Pts',(-5.78190678732237,-1.16809321267762,
-9.1200000005814)) ;
#163766=CARTESIAN_POINT('Ctrl Pts',(-5.85217562795658,-1.18707010095451,
-9.23075427171927)) ;
#163767=CARTESIAN_POINT('Ctrl Pts',(-5.81261165662068,-1.13738834337918,
-9.20413852805062)) ;
#163768=CARTESIAN_POINT('Ctrl Pts',(-5.83353949671039,-1.1164605032896,
-9.141407463619)) ;
#163769=CARTESIAN_POINT('Ctrl Pts',(-5.87071067811866,-1.14999999999999,
-9.24928932188135)) ;
#163770=CARTESIAN_POINT('Ctrl Pts',(-5.84714045207911,-1.10285954792089,
-9.2257190958418)) ;
#163771=CARTESIAN_POINT('Ctrl Pts',(-5.87071067811866,-1.07928932188133,
-9.1785786437627)) ;
#163772=CARTESIAN_POINT('Origin',(-5.8,-1.29142135623731,-9.12)) ;
#163773=CARTESIAN_POINT('Origin',(-3.59571067811865,-3.49571067811865,-9.12)) ;
#163774=CARTESIAN_POINT('Origin',(-5.17275707706437,-1.91866427917293,-9.12)) ;
#163775=CARTESIAN_POINT('Origin',(-3.09057773798104,-4.00084361825625,-8.12055391724001)) ;
#163776=CARTESIAN_POINT('Origin',(-5.17275707706437,-1.91866427917293,-9.12)) ;
#163777=CARTESIAN_POINT('Origin',(-5.17275707706437,-1.91866427917293,-9.12)) ;
#163778=CARTESIAN_POINT('Origin',(-5.17275707706437,-1.91866427917293,-9.12)) ;
#163779=CARTESIAN_POINT('Origin',(-5.17275707706437,-5.05,-9.12)) ;
#163780=CARTESIAN_POINT('Origin',(-5.17275707706437,-5.26511162862565,-9.12)) ;
#163781=CARTESIAN_POINT('Origin',(-3.96111272388873,-4.96220054033175,-8.53841071047569)) ;
#163782=CARTESIAN_POINT('Origin',(-5.17275707706437,-5.26511162862565,-9.12)) ;
#163783=CARTESIAN_POINT('Origin',(-5.17275707706437,-5.26511162862565,-9.12)) ;
#163784=CARTESIAN_POINT('Origin',(-5.17275707706437,-5.26511162862565,-9.12)) ;
#163785=CARTESIAN_POINT('Origin',(-5.10072415073893,-5.24710339704429,-9.12)) ;
#163786=CARTESIAN_POINT('Origin',(-5.8,-5.42192235935956,-9.12)) ;
#163787=CARTESIAN_POINT('Ctrl Pts',(-5.77574643749636,-5.51893660937409,
-9.12)) ;
#163788=CARTESIAN_POINT('Ctrl Pts',(-5.77574643749636,-5.51893660937409,
-9.22)) ;
#163789=CARTESIAN_POINT('Ctrl Pts',(-5.8,-5.42192235935956,-9.22)) ;
#163790=CARTESIAN_POINT('Ctrl Pts',(-5.79207992677989,-5.52301998169497,
-9.12000000046604)) ;
#163791=CARTESIAN_POINT('Ctrl Pts',(-5.78430903206643,-5.5210772580166,
-9.21803860456717)) ;
#163792=CARTESIAN_POINT('Ctrl Pts',(-5.808166653183,-5.42600568595104,-9.22)) ;
#163793=CARTESIAN_POINT('Ctrl Pts',(-5.80840777707096,-5.52710194426774,
-9.12201005409562)) ;
#163794=CARTESIAN_POINT('Ctrl Pts',(-5.79341417645231,-5.52335354411309,
-9.21716415018153)) ;
#163795=CARTESIAN_POINT('Ctrl Pts',(-5.81633079157287,-5.4300877551176,
-9.22100505725278)) ;
#163796=CARTESIAN_POINT('Ctrl Pts',(-5.82425356250363,-5.53106339062591,
-9.12597149997094)) ;
#163797=CARTESIAN_POINT('Ctrl Pts',(-5.80269484027818,-5.52567371006955,
-9.21759606942911)) ;
#163798=CARTESIAN_POINT('Ctrl Pts',(-5.82425356250363,-5.43404914061138,
-9.22298574998547)) ;
#163799=CARTESIAN_POINT('Origin',(-5.84850712500726,-5.43404914061138,-9.12597149997094)) ;
#163800=CARTESIAN_POINT('Ctrl Pts',(-5.82426676739349,-5.53106667467168,
-9.1259153963657)) ;
#163801=CARTESIAN_POINT('Ctrl Pts',(-5.80266988778307,-5.52572362328987,
-9.21764596618925)) ;
#163802=CARTESIAN_POINT('Ctrl Pts',(-5.82426676352025,-5.43399305345737,
-9.222989033073)) ;
#163803=CARTESIAN_POINT('Ctrl Pts',(-5.83498671931119,-5.53374818244428,
-9.1312758712786)) ;
#163804=CARTESIAN_POINT('Ctrl Pts',(-5.80595263122257,-5.5241175471001,
-9.21603989083685)) ;
#163805=CARTESIAN_POINT('Ctrl Pts',(-5.83498671397637,-5.4393535274938,
-9.22567054003428)) ;
#163806=CARTESIAN_POINT('Ctrl Pts',(-5.84526105845713,-5.53822480044428,
-9.14022562225452)) ;
#163807=CARTESIAN_POINT('Ctrl Pts',(-5.81370932746126,-5.52260133464133,
-9.21452367966838)) ;
#163808=CARTESIAN_POINT('Ctrl Pts',(-5.84526105243735,-5.44830327707035,
-9.23014715682302)) ;
#163809=CARTESIAN_POINT('Ctrl Pts',(-5.86378685403698,-5.55027438933176,
-9.16432256366359)) ;
#163810=CARTESIAN_POINT('Ctrl Pts',(-5.83531854275277,-5.5273306855257,
-9.21925303340452)) ;
#163811=CARTESIAN_POINT('Ctrl Pts',(-5.86378684816472,-5.47240021563471,
-9.24219674395865)) ;
#163812=CARTESIAN_POINT('Ctrl Pts',(-5.87203852631577,-5.55784608774606,
-9.17946731070693)) ;
#163813=CARTESIAN_POINT('Ctrl Pts',(-5.84834787930678,-5.5331020048643,
-9.22502435426416)) ;
#163814=CARTESIAN_POINT('Ctrl Pts',(-5.87203852123051,-5.48754496112629,
-9.24976844179423)) ;
#163815=CARTESIAN_POINT('Ctrl Pts',(-5.89242747304796,-5.58397198950281,
-9.23173438269412)) ;
#163816=CARTESIAN_POINT('Ctrl Pts',(-5.88223383300416,-5.56084219746612,
-9.25276455115244)) ;
#163817=CARTESIAN_POINT('Ctrl Pts',(-5.89242747063508,-5.53981202831252,
-9.27589434338744)) ;
#163818=CARTESIAN_POINT('Ctrl Pts',(-5.9,-5.60595824049742,-9.27573319883257)) ;
#163819=CARTESIAN_POINT('Ctrl Pts',(-5.9,-5.59485304775401,-9.28677540438623)) ;
#163820=CARTESIAN_POINT('Ctrl Pts',(-5.9,-5.58381084219975,-9.29788059711478)) ;
#163821=CARTESIAN_POINT('Ctrl Pts',(-5.9,-5.62807764064044,-9.32)) ;
#163822=CARTESIAN_POINT('Ctrl Pts',(-5.9,-5.62807764064044,-9.32)) ;
#163823=CARTESIAN_POINT('Ctrl Pts',(-5.9,-5.62807764064044,-9.32)) ;
#163824=CARTESIAN_POINT('Origin',(7.8,2.1,-8.02)) ;
#163825=CARTESIAN_POINT('Origin',(7.8,2.1,-8.22)) ;
#163826=CARTESIAN_POINT('Origin',(7.6,2.1,-8.02)) ;
#163827=CARTESIAN_POINT('Origin',(7.6,2.1,-8.02)) ;
#163828=CARTESIAN_POINT('Origin',(7.6,2.1,-7.22)) ;
#163829=CARTESIAN_POINT('Origin',(7.8,2.1,-8.22)) ;
#163830=CARTESIAN_POINT('Origin',(9.6,2.1,-8.22)) ;
#163831=CARTESIAN_POINT('Origin',(7.8,2.1,-7.22)) ;
#163832=CARTESIAN_POINT('Origin',(7.8,2.1,-7.02)) ;
#163833=CARTESIAN_POINT('Origin',(9.6,2.1,-8.02)) ;
#163834=CARTESIAN_POINT('Origin',(9.8,2.1,-8.02)) ;
#163835=CARTESIAN_POINT('Origin',(7.8,2.1,-7.02)) ;
#163836=CARTESIAN_POINT('Origin',(9.6,2.1,-7.02)) ;
#163837=CARTESIAN_POINT('Origin',(9.8,2.1,-8.02)) ;
#163838=CARTESIAN_POINT('Origin',(9.8,2.1,-7.22)) ;
#163839=CARTESIAN_POINT('Origin',(9.6,2.1,-7.22)) ;
#163840=CARTESIAN_POINT('Origin',(-4.15,-6.25,-6.87)) ;
#163841=CARTESIAN_POINT('Origin',(-4.15,-6.3,-6.87)) ;
#163842=CARTESIAN_POINT('Origin',(-4.15,-6.3,-7.62)) ;
#163843=CARTESIAN_POINT('Origin',(-4.15,-6.3,-8.37)) ;
#163844=CARTESIAN_POINT('Origin',(-4.15,-6.3,-6.87)) ;
#163845=CARTESIAN_POINT('Origin',(-4.15,-6.25,-8.37)) ;
#163846=CARTESIAN_POINT('Origin',(-4.15,-6.3,-8.37)) ;
#163847=CARTESIAN_POINT('Origin',(-4.15,-6.3,-6.87)) ;
#163848=CARTESIAN_POINT('Origin',(-4.15,-6.3,-6.87)) ;
#163849=CARTESIAN_POINT('Origin',(-4.15,-6.3,-8.37)) ;
#163850=CARTESIAN_POINT('Origin',(-4.15,-6.3,-8.37)) ;
#163851=CARTESIAN_POINT('Origin',(-4.65,-6.25,-6.87)) ;
#163852=CARTESIAN_POINT('Origin',(-4.65,-6.3,-6.87)) ;
#163853=CARTESIAN_POINT('Origin',(0.,-6.3,-6.87)) ;
#163854=CARTESIAN_POINT('Origin',(-4.65,-6.3,-6.87)) ;
#163855=CARTESIAN_POINT('Origin',(0.,-6.3,-8.37)) ;
#163856=CARTESIAN_POINT('Origin',(-4.65,-6.3,-8.37)) ;
#163857=CARTESIAN_POINT('Origin',(-4.65,-6.25,-8.37)) ;
#163858=CARTESIAN_POINT('Origin',(-4.65,-6.3,-8.37)) ;
#163859=CARTESIAN_POINT('Origin',(-4.65,-6.3,-6.87)) ;
#163860=CARTESIAN_POINT('Origin',(-4.65,-6.3,-6.87)) ;
#163861=CARTESIAN_POINT('Origin',(-4.65,-6.3,-8.37)) ;
#163862=CARTESIAN_POINT('Origin',(-4.65,-6.3,-8.37)) ;
#163863=CARTESIAN_POINT('Origin',(-4.65,-6.3,-7.62)) ;
#163864=CARTESIAN_POINT('Origin',(-3.,4.45,-8.72)) ;
#163865=CARTESIAN_POINT('Origin',(-2.1,4.45,-8.72)) ;
#163866=CARTESIAN_POINT('Origin',(-2.9,4.45,-8.72)) ;
#163867=CARTESIAN_POINT('Origin',(-2.9,4.45,-8.52)) ;
#163868=CARTESIAN_POINT('Origin',(-3.1,4.45,-8.52)) ;
#163869=CARTESIAN_POINT('Origin',(-2.9,4.45,-8.52)) ;
#163870=CARTESIAN_POINT('Origin',(-2.1,4.45,-8.52)) ;
#163871=CARTESIAN_POINT('Origin',(-2.1,4.45,-8.52)) ;
#163872=CARTESIAN_POINT('Origin',(-1.9,4.45,-8.52)) ;
#163873=CARTESIAN_POINT('Origin',(-3.1,4.45,-8.62)) ;
#163874=CARTESIAN_POINT('Origin',(-3.1,4.45,-6.72)) ;
#163875=CARTESIAN_POINT('Origin',(-2.9,4.4,-8.52)) ;
#163876=CARTESIAN_POINT('Origin',(-2.9,4.35,-8.52)) ;
#163877=CARTESIAN_POINT('Origin',(-1.95156391047391E-16,4.35,-8.52)) ;
#163878=CARTESIAN_POINT('Origin',(-2.1,4.35,-8.52)) ;
#163879=CARTESIAN_POINT('Origin',(-2.9,4.35,-8.52)) ;
#163880=CARTESIAN_POINT('Origin',(-2.1,4.4,-8.52)) ;
#163881=CARTESIAN_POINT('Origin',(-2.1,4.35,-8.52)) ;
#163882=CARTESIAN_POINT('Origin',(-1.9,4.45,-8.62)) ;
#163883=CARTESIAN_POINT('Origin',(-1.9,4.45,-6.72)) ;
#163884=CARTESIAN_POINT('Origin',(-3.,4.45,-6.52)) ;
#163885=CARTESIAN_POINT('Origin',(-2.9,4.45,-6.52)) ;
#163886=CARTESIAN_POINT('Origin',(-2.1,4.45,-6.52)) ;
#163887=CARTESIAN_POINT('Origin',(-2.9,4.45,-6.72)) ;
#163888=CARTESIAN_POINT('Origin',(-2.9,4.45,-6.72)) ;
#163889=CARTESIAN_POINT('Origin',(-2.9,4.35,-8.52)) ;
#163890=CARTESIAN_POINT('Origin',(-2.9,4.35,-8.52)) ;
#163891=CARTESIAN_POINT('Origin',(-2.1,4.35,-8.52)) ;
#163892=CARTESIAN_POINT('Origin',(-2.1,4.35,-8.52)) ;
#163893=CARTESIAN_POINT('Origin',(-2.1,4.45,-6.72)) ;
#163894=CARTESIAN_POINT('Origin',(-2.1,4.45,-6.72)) ;
#163895=CARTESIAN_POINT('Origin',(-2.9,4.4,-6.72)) ;
#163896=CARTESIAN_POINT('Origin',(-2.9,4.35,-6.72)) ;
#163897=CARTESIAN_POINT('Origin',(-2.9,4.35,-7.62)) ;
#163898=CARTESIAN_POINT('Origin',(-2.9,4.35,-6.72)) ;
#163899=CARTESIAN_POINT('Origin',(-2.1,4.35,-7.62)) ;
#163900=CARTESIAN_POINT('Origin',(-2.1,4.35,-6.72)) ;
#163901=CARTESIAN_POINT('Origin',(-2.1,4.4,-6.72)) ;
#163902=CARTESIAN_POINT('Origin',(-2.1,4.35,-6.72)) ;
#163903=CARTESIAN_POINT('Origin',(-2.9,4.35,-6.72)) ;
#163904=CARTESIAN_POINT('Origin',(-2.9,4.35,-6.72)) ;
#163905=CARTESIAN_POINT('Origin',(-2.1,4.35,-6.72)) ;
#163906=CARTESIAN_POINT('Origin',(-2.1,4.35,-6.72)) ;
#163907=CARTESIAN_POINT('Origin',(-1.95156391047391E-16,4.35,-6.72)) ;
#163908=CARTESIAN_POINT('Origin',(-2.25,4.25,-8.37)) ;
#163909=CARTESIAN_POINT('Origin',(-2.25,4.3,-8.37)) ;
#163910=CARTESIAN_POINT('Origin',(-2.25,4.3,-7.62)) ;
#163911=CARTESIAN_POINT('Origin',(-2.25,4.3,-6.87)) ;
#163912=CARTESIAN_POINT('Origin',(-2.25,4.3,-8.37)) ;
#163913=CARTESIAN_POINT('Origin',(-2.25,4.25,-6.87)) ;
#163914=CARTESIAN_POINT('Origin',(-2.25,4.3,-6.87)) ;
#163915=CARTESIAN_POINT('Origin',(-2.25,4.3,-8.37)) ;
#163916=CARTESIAN_POINT('Origin',(-2.25,4.3,-8.37)) ;
#163917=CARTESIAN_POINT('Origin',(-2.25,4.3,-6.87)) ;
#163918=CARTESIAN_POINT('Origin',(-2.25,4.3,-6.87)) ;
#163919=CARTESIAN_POINT('Origin',(-2.75,4.25,-8.37)) ;
#163920=CARTESIAN_POINT('Origin',(-2.75,4.3,-8.37)) ;
#163921=CARTESIAN_POINT('Origin',(-1.97127667724637E-17,4.3,-8.37)) ;
#163922=CARTESIAN_POINT('Origin',(-2.75,4.3,-8.37)) ;
#163923=CARTESIAN_POINT('Origin',(-1.97127667724637E-17,4.3,-6.87)) ;
#163924=CARTESIAN_POINT('Origin',(-2.75,4.3,-6.87)) ;
#163925=CARTESIAN_POINT('Origin',(-2.75,4.25,-6.87)) ;
#163926=CARTESIAN_POINT('Origin',(-2.75,4.3,-6.87)) ;
#163927=CARTESIAN_POINT('Origin',(-2.75,4.3,-8.37)) ;
#163928=CARTESIAN_POINT('Origin',(-2.75,4.3,-8.37)) ;
#163929=CARTESIAN_POINT('Origin',(-2.75,4.3,-6.87)) ;
#163930=CARTESIAN_POINT('Origin',(-2.75,4.3,-6.87)) ;
#163931=CARTESIAN_POINT('Origin',(-2.75,4.3,-7.62)) ;
#163932=CARTESIAN_POINT('Origin',(7.8,2.9,-8.02)) ;
#163933=CARTESIAN_POINT('Origin',(7.8,2.9,-8.02)) ;
#163934=CARTESIAN_POINT('Origin',(7.8,2.9,-7.22)) ;
#163935=CARTESIAN_POINT('Origin',(7.8,2.9,-7.22)) ;
#163936=CARTESIAN_POINT('Origin',(7.8,2.9,-7.22)) ;
#163937=CARTESIAN_POINT('Origin',(7.8,2.9,-8.02)) ;
#163938=CARTESIAN_POINT('Origin',(7.8,2.9,-8.02)) ;
#163939=CARTESIAN_POINT('Origin',(9.6,2.9,-7.22)) ;
#163940=CARTESIAN_POINT('Origin',(9.6,2.9,-7.22)) ;
#163941=CARTESIAN_POINT('Origin',(9.6,2.9,-8.02)) ;
#163942=CARTESIAN_POINT('Origin',(9.6,2.9,-8.02)) ;
#163943=CARTESIAN_POINT('Origin',(9.6,2.9,-7.22)) ;
#163944=CARTESIAN_POINT('Origin',(9.6,2.9,-7.22)) ;
#163945=CARTESIAN_POINT('Origin',(9.6,2.9,-8.02)) ;
#163946=CARTESIAN_POINT('Origin',(9.6,2.9,-8.02)) ;
#163947=CARTESIAN_POINT('Origin',(9.6,2.9,-8.02)) ;
#163948=CARTESIAN_POINT('Origin',(-0.183301359729408,3.45,-6.10296321352403)) ;
#163949=CARTESIAN_POINT('Origin',(0.249234641435079,3.15,-7.50377997802131)) ;
#163950=CARTESIAN_POINT('Origin',(-0.249234641435079,3.15,-7.73622002197869)) ;
#163951=CARTESIAN_POINT('Origin',(-1.04429375741423,3.45,-6.50445056217769)) ;
#163952=CARTESIAN_POINT('Origin',(10.1,-2.15,-10.5268804065906)) ;
#163953=CARTESIAN_POINT('Origin',(10.1,-2.15,-10.5268804065906)) ;
#163954=CARTESIAN_POINT('Origin',(10.1,-2.15,-10.5268804065906)) ;
#163955=CARTESIAN_POINT('Origin',(10.1,-2.15,-10.5268804065906)) ;
#163956=CARTESIAN_POINT('Origin',(10.1,-2.15,-11.43)) ;
#163957=CARTESIAN_POINT('Origin',(10.1,-2.15,-10.125)) ;
#163958=CARTESIAN_POINT('Origin',(10.2,-2.15,-10.5268804065906)) ;
#163959=CARTESIAN_POINT('Origin',(3.7,-2.15,-10.5268804065906)) ;
#163960=CARTESIAN_POINT('Origin',(10.1,-3.65625,-11.43)) ;
#163961=CARTESIAN_POINT('Origin',(10.1,-2.15,-12.3331195934094)) ;
#163962=CARTESIAN_POINT('Origin',(10.1,-3.65625,-10.125)) ;
#163963=CARTESIAN_POINT('Origin',(10.1,1.9,-10.125)) ;
#163964=CARTESIAN_POINT('Origin',(10.1,-2.15,-10.125)) ;
#163965=CARTESIAN_POINT('Origin',(10.1,-2.15,-10.125)) ;
#163966=CARTESIAN_POINT('Origin',(10.1,-2.15,-10.125)) ;
#163967=CARTESIAN_POINT('Origin',(3.7,-2.15,-10.5268804065906)) ;
#163968=CARTESIAN_POINT('Origin',(3.7,-2.32153024911032,-10.6297267659824)) ;
#163969=CARTESIAN_POINT('Origin',(3.7,-2.35,-10.5268804065906)) ;
#163970=CARTESIAN_POINT('Origin',(10.1,-2.15,-12.3331195934094)) ;
#163971=CARTESIAN_POINT('Origin',(10.1,-2.15,-12.3331195934094)) ;
#163972=CARTESIAN_POINT('Origin',(10.1,-2.15,-12.3331195934094)) ;
#163973=CARTESIAN_POINT('Origin',(10.1,1.9,-11.43)) ;
#163974=CARTESIAN_POINT('Origin',(10.1,1.9,-12.735)) ;
#163975=CARTESIAN_POINT('Origin',(10.1,1.9,-10.125)) ;
#163976=CARTESIAN_POINT('Origin',(10.2,-2.15,-10.125)) ;
#163977=CARTESIAN_POINT('Origin',(3.7,-2.15,-10.125)) ;
#163978=CARTESIAN_POINT('Origin',(3.7,-2.35,-10.025)) ;
#163979=CARTESIAN_POINT('Origin',(3.7,-2.35,-10.125)) ;
#163980=CARTESIAN_POINT('Origin',(3.7,-3.65625,-11.43)) ;
#163981=CARTESIAN_POINT('Origin',(3.7,-2.32153024911032,-12.2302732340176)) ;
#163982=CARTESIAN_POINT('Origin',(10.2,-2.15,-12.3331195934094)) ;
#163983=CARTESIAN_POINT('Origin',(3.7,-2.15,-12.3331195934094)) ;
#163984=CARTESIAN_POINT('Origin',(10.1,-2.15,-11.43)) ;
#163985=CARTESIAN_POINT('Origin',(10.1,-2.15,-12.735)) ;
#163986=CARTESIAN_POINT('Origin',(10.1,-3.65625,-12.735)) ;
#163987=CARTESIAN_POINT('Origin',(10.1,1.9,-12.735)) ;
#163988=CARTESIAN_POINT('Origin',(10.1,-2.15,-12.735)) ;
#163989=CARTESIAN_POINT('Origin',(3.7,-2.35,-10.125)) ;
#163990=CARTESIAN_POINT('Origin',(3.5,-2.35,-10.125)) ;
#163991=CARTESIAN_POINT('Origin',(3.7,-2.15,-12.3331195934094)) ;
#163992=CARTESIAN_POINT('Origin',(3.7,-2.35,-12.3331195934094)) ;
#163993=CARTESIAN_POINT('Origin',(10.1,-2.15,-12.735)) ;
#163994=CARTESIAN_POINT('Origin',(10.1,-2.15,-12.735)) ;
#163995=CARTESIAN_POINT('Origin',(3.6,1.9,-9.925)) ;
#163996=CARTESIAN_POINT('Origin',(3.5,1.9,-9.925)) ;
#163997=CARTESIAN_POINT('Origin',(2.7,1.9,-9.925)) ;
#163998=CARTESIAN_POINT('Origin',(3.5,9.86627345095305E-16,-10.125)) ;
#163999=CARTESIAN_POINT('Origin',(3.5,-5.15,-10.125)) ;
#164000=CARTESIAN_POINT('Origin',(3.7,-2.35,-12.305)) ;
#164001=CARTESIAN_POINT('Origin',(3.7,-2.35,-12.735)) ;
#164002=CARTESIAN_POINT('Origin',(3.6,-2.15,-12.735)) ;
#164003=CARTESIAN_POINT('Origin',(3.7,-2.15,-12.735)) ;
#164004=CARTESIAN_POINT('Origin',(2.7,1.9,-9.925)) ;
#164005=CARTESIAN_POINT('Origin',(2.7,1.9,-9.925)) ;
#164006=CARTESIAN_POINT('Origin',(3.5,-5.15,-10.125)) ;
#164007=CARTESIAN_POINT('Origin',(3.5,-5.15,-10.125)) ;
#164008=CARTESIAN_POINT('Origin',(3.5,-5.15,-10.125)) ;
#164009=CARTESIAN_POINT('Origin',(3.7,-2.35,-12.735)) ;
#164010=CARTESIAN_POINT('Origin',(3.5,-2.35,-12.735)) ;
#164011=CARTESIAN_POINT('Origin',(2.7,2.,-9.925)) ;
#164012=CARTESIAN_POINT('Origin',(2.7,-5.15,-9.925)) ;
#164013=CARTESIAN_POINT('Origin',(3.6,-5.15,-10.125)) ;
#164014=CARTESIAN_POINT('Origin',(2.7,-5.15,-10.125)) ;
#164015=CARTESIAN_POINT('Origin',(3.5,-5.15,0.)) ;
#164016=CARTESIAN_POINT('Origin',(3.5,-5.15,-12.735)) ;
#164017=CARTESIAN_POINT('Origin',(3.5,-1.06453362012003E-15,-12.735)) ;
#164018=CARTESIAN_POINT('Origin',(3.5,-5.15,-12.735)) ;
#164019=CARTESIAN_POINT('Origin',(2.7,-5.15,-10.125)) ;
#164020=CARTESIAN_POINT('Origin',(2.7,-5.35,-10.125)) ;
#164021=CARTESIAN_POINT('Origin',(3.5,-5.15,-12.735)) ;
#164022=CARTESIAN_POINT('Origin',(3.5,-5.15,-12.735)) ;
#164023=CARTESIAN_POINT('Origin',(2.7,-5.35,-10.025)) ;
#164024=CARTESIAN_POINT('Origin',(2.7,-5.35,-12.735)) ;
#164025=CARTESIAN_POINT('Origin',(3.6,-5.15,-12.735)) ;
#164026=CARTESIAN_POINT('Origin',(2.7,-5.15,-12.735)) ;
#164027=CARTESIAN_POINT('Origin',(3.6,1.9,-12.935)) ;
#164028=CARTESIAN_POINT('Origin',(3.5,1.9,-12.935)) ;
#164029=CARTESIAN_POINT('Origin',(2.7,1.9,-12.935)) ;
#164030=CARTESIAN_POINT('Origin',(2.7,1.9,-12.835)) ;
#164031=CARTESIAN_POINT('Origin',(2.7,1.9,-13.735)) ;
#164032=CARTESIAN_POINT('Origin',(2.7,1.9,-12.935)) ;
#164033=CARTESIAN_POINT('Origin',(2.7,-5.15,-12.735)) ;
#164034=CARTESIAN_POINT('Origin',(2.7,-5.15,-12.935)) ;
#164035=CARTESIAN_POINT('Origin',(2.7,1.9,-12.935)) ;
#164036=CARTESIAN_POINT('Origin',(2.7,1.9,-12.935)) ;
#164037=CARTESIAN_POINT('Origin',(2.7,-5.25,-12.935)) ;
#164038=CARTESIAN_POINT('Ctrl Pts',(-3.8,-6.55,-10.33)) ;
#164039=CARTESIAN_POINT('Ctrl Pts',(-3.8,-6.55,-10.33)) ;
#164040=CARTESIAN_POINT('Ctrl Pts',(-3.8,-6.55,-10.33)) ;
#164041=CARTESIAN_POINT('Ctrl Pts',(-3.82625343282639,-6.55,-10.3825068656527)) ;
#164042=CARTESIAN_POINT('Ctrl Pts',(-3.83954133268484,-6.55,-10.3695413326849)) ;
#164043=CARTESIAN_POINT('Ctrl Pts',(-3.85250686565269,-6.55,-10.3562534328264)) ;
#164044=CARTESIAN_POINT('Ctrl Pts',(-3.85219871729854,-6.53922263893877,
-10.4343974345971)) ;
#164045=CARTESIAN_POINT('Ctrl Pts',(-3.87914655110982,-6.52362528614073,
-10.4091465511098)) ;
#164046=CARTESIAN_POINT('Ctrl Pts',(-3.90439743459708,-6.53922263893877,
-10.3821987172985)) ;
#164047=CARTESIAN_POINT('Ctrl Pts',(-3.87996665852871,-6.5114546977086,
-10.4899333170574)) ;
#164048=CARTESIAN_POINT('Ctrl Pts',(-3.9028838031416,-6.48208554016475,
-10.4328838031416)) ;
#164049=CARTESIAN_POINT('Ctrl Pts',(-3.95993331705742,-6.5114546977086,
-10.4099666585287)) ;
#164050=CARTESIAN_POINT('Ctrl Pts',(-3.88737865704135,-6.5003618540841,
-10.5047573140827)) ;
#164051=CARTESIAN_POINT('Ctrl Pts',(-3.9050130758829,-6.46792722356045,
-10.435013075883)) ;
#164052=CARTESIAN_POINT('Ctrl Pts',(-3.9747573140827,-6.5003618540841,-10.4173786570414)) ;
#164053=CARTESIAN_POINT('Ctrl Pts',(-3.8973972494609,-6.47617483238892,
-10.5247944989218)) ;
#164054=CARTESIAN_POINT('Ctrl Pts',(-3.90329674356413,-6.45094059868423,
-10.4332967435641)) ;
#164055=CARTESIAN_POINT('Ctrl Pts',(-3.99479449892181,-6.47617483238892,
-10.4273972494609)) ;
#164056=CARTESIAN_POINT('Ctrl Pts',(-3.9,-6.46309229646327,-10.5299999991817)) ;
#164057=CARTESIAN_POINT('Ctrl Pts',(-3.90000730395039,-6.4494565015223,
-10.4300073039127)) ;
#164058=CARTESIAN_POINT('Ctrl Pts',(-3.99999999918173,-6.46309229646328,
-10.43)) ;
#164059=CARTESIAN_POINT('Ctrl Pts',(-3.9,-6.45,-10.53)) ;
#164060=CARTESIAN_POINT('Ctrl Pts',(-3.9,-6.45,-10.43)) ;
#164061=CARTESIAN_POINT('Ctrl Pts',(-4.,-6.45,-10.43)) ;
#164062=CARTESIAN_POINT('Origin',(-4.,-6.45,-10.53)) ;
#164063=CARTESIAN_POINT('Origin',(-4.,-6.4,-10.53)) ;
#164064=CARTESIAN_POINT('Origin',(-4.,-6.35,-10.53)) ;
#164065=CARTESIAN_POINT('Ctrl Pts',(-5.,-6.55,-10.33)) ;
#164066=CARTESIAN_POINT('Ctrl Pts',(-5.,-6.55,-10.33)) ;
#164067=CARTESIAN_POINT('Ctrl Pts',(-5.,-6.55,-10.33)) ;
#164068=CARTESIAN_POINT('Ctrl Pts',(-4.94749313434721,-6.55,-10.3562534328262)) ;
#164069=CARTESIAN_POINT('Ctrl Pts',(-4.96045866731606,-6.55,-10.3695413326839)) ;
#164070=CARTESIAN_POINT('Ctrl Pts',(-4.97374656717352,-6.55,-10.3825068656527)) ;
#164071=CARTESIAN_POINT('Ctrl Pts',(-4.89560256540291,-6.53922263893879,
-10.3821987172985)) ;
#164072=CARTESIAN_POINT('Ctrl Pts',(-4.92085344889017,-6.52362528614073,
-10.4091465511097)) ;
#164073=CARTESIAN_POINT('Ctrl Pts',(-4.94780128270146,-6.53922263893877,
-10.434397434597)) ;
#164074=CARTESIAN_POINT('Ctrl Pts',(-4.84006668294258,-6.51145469770858,
-10.4099666585287)) ;
#164075=CARTESIAN_POINT('Ctrl Pts',(-4.8971161968584,-6.48208554016475,
-10.4328838031417)) ;
#164076=CARTESIAN_POINT('Ctrl Pts',(-4.92003334147129,-6.5114546977086,
-10.4899333170575)) ;
#164077=CARTESIAN_POINT('Ctrl Pts',(-4.82524268591729,-6.5003618540841,
-10.4173786570414)) ;
#164078=CARTESIAN_POINT('Ctrl Pts',(-4.89498692411708,-6.46792722356046,
-10.435013075883)) ;
#164079=CARTESIAN_POINT('Ctrl Pts',(-4.91262134295865,-6.5003618540841,
-10.5047573140827)) ;
#164080=CARTESIAN_POINT('Ctrl Pts',(-4.80520550107819,-6.47617483238892,
-10.4273972494609)) ;
#164081=CARTESIAN_POINT('Ctrl Pts',(-4.89670325643589,-6.45094059868422,
-10.4332967435641)) ;
#164082=CARTESIAN_POINT('Ctrl Pts',(-4.90260275053909,-6.47617483238892,
-10.5247944989218)) ;
#164083=CARTESIAN_POINT('Ctrl Pts',(-4.80000000081823,-6.46309229646328,
-10.43)) ;
#164084=CARTESIAN_POINT('Ctrl Pts',(-4.89999269603066,-6.4494565015302,
-10.4300073039128)) ;
#164085=CARTESIAN_POINT('Ctrl Pts',(-4.9,-6.46309229646328,-10.5299999991817)) ;
#164086=CARTESIAN_POINT('Ctrl Pts',(-4.8,-6.45,-10.43)) ;
#164087=CARTESIAN_POINT('Ctrl Pts',(-4.9,-6.45,-10.43)) ;
#164088=CARTESIAN_POINT('Ctrl Pts',(-4.9,-6.45,-10.53)) ;
#164089=CARTESIAN_POINT('Origin',(-4.8,-6.45,-10.53)) ;
#164090=CARTESIAN_POINT('Origin',(-4.,-6.35,-10.53)) ;
#164091=CARTESIAN_POINT('Origin',(-4.,-6.35,-10.53)) ;
#164092=CARTESIAN_POINT('Origin',(-4.,-6.35,-10.53)) ;
#164093=CARTESIAN_POINT('Ctrl Pts',(-3.8,-6.55,-12.53)) ;
#164094=CARTESIAN_POINT('Ctrl Pts',(-3.8,-6.55,-12.53)) ;
#164095=CARTESIAN_POINT('Ctrl Pts',(-3.8,-6.55,-12.53)) ;
#164096=CARTESIAN_POINT('Ctrl Pts',(-3.8525068656527,-6.55,-12.5037465671736)) ;
#164097=CARTESIAN_POINT('Ctrl Pts',(-3.83954133268456,-6.55,-12.4904586673157)) ;
#164098=CARTESIAN_POINT('Ctrl Pts',(-3.82625343282636,-6.55,-12.4774931343473)) ;
#164099=CARTESIAN_POINT('Ctrl Pts',(-3.90439743459706,-6.53922263893877,
-12.4778012827015)) ;
#164100=CARTESIAN_POINT('Ctrl Pts',(-3.87914655110982,-6.52362528614073,
-12.4508534488902)) ;
#164101=CARTESIAN_POINT('Ctrl Pts',(-3.85219871729855,-6.53922263893876,
-12.4256025654029)) ;
#164102=CARTESIAN_POINT('Ctrl Pts',(-3.95993331705743,-6.5114546977086,
-12.4500333414713)) ;
#164103=CARTESIAN_POINT('Ctrl Pts',(-3.9028838031416,-6.48208554016474,
-12.4271161968584)) ;
#164104=CARTESIAN_POINT('Ctrl Pts',(-3.8799666585287,-6.5114546977086,-12.3700666829426)) ;
#164105=CARTESIAN_POINT('Ctrl Pts',(-3.97475731408271,-6.5003618540841,
-12.4426213429587)) ;
#164106=CARTESIAN_POINT('Ctrl Pts',(-3.90501307588293,-6.46792722356048,
-12.424986924117)) ;
#164107=CARTESIAN_POINT('Ctrl Pts',(-3.88737865704135,-6.5003618540841,
-12.3552426859173)) ;
#164108=CARTESIAN_POINT('Ctrl Pts',(-3.9947944989218,-6.47617483238892,
-12.4326027505391)) ;
#164109=CARTESIAN_POINT('Ctrl Pts',(-3.9032967435641,-6.45094059868419,
-12.4267032564359)) ;
#164110=CARTESIAN_POINT('Ctrl Pts',(-3.89739724946091,-6.47617483238892,
-12.3352055010782)) ;
#164111=CARTESIAN_POINT('Ctrl Pts',(-3.99999999918176,-6.46309229646328,
-12.43)) ;
#164112=CARTESIAN_POINT('Ctrl Pts',(-3.90000730395526,-6.44945650152442,
-12.4299926960872)) ;
#164113=CARTESIAN_POINT('Ctrl Pts',(-3.9,-6.46309229646328,-12.3300000008183)) ;
#164114=CARTESIAN_POINT('Ctrl Pts',(-4.,-6.45,-12.43)) ;
#164115=CARTESIAN_POINT('Ctrl Pts',(-3.9,-6.45,-12.43)) ;
#164116=CARTESIAN_POINT('Ctrl Pts',(-3.9,-6.45,-12.33)) ;
#164117=CARTESIAN_POINT('Origin',(-4.,-6.45,-12.33)) ;
#164118=CARTESIAN_POINT('Origin',(-4.8,-6.4,-10.53)) ;
#164119=CARTESIAN_POINT('Origin',(-4.8,-6.35,-10.53)) ;
#164120=CARTESIAN_POINT('Origin',(1.9515639104739E-16,-6.35,-10.53)) ;
#164121=CARTESIAN_POINT('Origin',(-4.8,-6.35,-10.53)) ;
#164122=CARTESIAN_POINT('Origin',(-4.,-6.35,-11.43)) ;
#164123=CARTESIAN_POINT('Origin',(-4.,-6.35,-12.33)) ;
#164124=CARTESIAN_POINT('Origin',(-4.,-6.4,-12.33)) ;
#164125=CARTESIAN_POINT('Origin',(-4.,-6.35,-12.33)) ;
#164126=CARTESIAN_POINT('Origin',(-4.8,-6.35,-10.53)) ;
#164127=CARTESIAN_POINT('Origin',(-4.8,-6.35,-10.53)) ;
#164128=CARTESIAN_POINT('Origin',(-4.,-6.35,-12.33)) ;
#164129=CARTESIAN_POINT('Origin',(-4.,-6.35,-12.33)) ;
#164130=CARTESIAN_POINT('Origin',(-4.8,-6.35,-11.43)) ;
#164131=CARTESIAN_POINT('Origin',(-4.8,-6.35,-12.33)) ;
#164132=CARTESIAN_POINT('Origin',(1.95156391047391E-16,-6.35,-12.33)) ;
#164133=CARTESIAN_POINT('Origin',(-4.8,-6.35,-12.33)) ;
#164134=CARTESIAN_POINT('Origin',(-4.8,-6.35,-12.33)) ;
#164135=CARTESIAN_POINT('Origin',(-4.8,-6.35,-12.33)) ;
#164136=CARTESIAN_POINT('Origin',(-4.8,-6.4,-12.33)) ;
#164137=CARTESIAN_POINT('Origin',(-4.8,-6.45,-12.33)) ;
#164138=CARTESIAN_POINT('Ctrl Pts',(-5.,-6.55,-12.53)) ;
#164139=CARTESIAN_POINT('Ctrl Pts',(-5.,-6.55,-12.53)) ;
#164140=CARTESIAN_POINT('Ctrl Pts',(-5.,-6.55,-12.53)) ;
#164141=CARTESIAN_POINT('Ctrl Pts',(-4.97374656717353,-6.55,-12.4774931343473)) ;
#164142=CARTESIAN_POINT('Ctrl Pts',(-4.96045866731541,-6.55,-12.4904586673157)) ;
#164143=CARTESIAN_POINT('Ctrl Pts',(-4.94749313434721,-6.55,-12.5037465671738)) ;
#164144=CARTESIAN_POINT('Ctrl Pts',(-4.94780128270146,-6.53922263893877,
-12.425602565403)) ;
#164145=CARTESIAN_POINT('Ctrl Pts',(-4.92085344889015,-6.52362528614073,
-12.4508534488903)) ;
#164146=CARTESIAN_POINT('Ctrl Pts',(-4.89560256540291,-6.53922263893879,
-12.4778012827015)) ;
#164147=CARTESIAN_POINT('Ctrl Pts',(-4.92003334147129,-6.5114546977086,
-12.3700666829426)) ;
#164148=CARTESIAN_POINT('Ctrl Pts',(-4.89711619685841,-6.48208554016475,
-12.4271161968583)) ;
#164149=CARTESIAN_POINT('Ctrl Pts',(-4.84006668294258,-6.51145469770858,
-12.4500333414713)) ;
#164150=CARTESIAN_POINT('Ctrl Pts',(-4.91262134295865,-6.5003618540841,
-12.3552426859173)) ;
#164151=CARTESIAN_POINT('Ctrl Pts',(-4.89498692411706,-6.46792722356048,
-12.424986924117)) ;
#164152=CARTESIAN_POINT('Ctrl Pts',(-4.82524268591729,-6.5003618540841,
-12.4426213429587)) ;
#164153=CARTESIAN_POINT('Ctrl Pts',(-4.90260275053909,-6.47617483238892,
-12.3352055010782)) ;
#164154=CARTESIAN_POINT('Ctrl Pts',(-4.8967032564359,-6.45094059868419,
-12.4267032564359)) ;
#164155=CARTESIAN_POINT('Ctrl Pts',(-4.80520550107819,-6.47617483238892,
-12.4326027505391)) ;
#164156=CARTESIAN_POINT('Ctrl Pts',(-4.9,-6.46309229646328,-12.3300000008183)) ;
#164157=CARTESIAN_POINT('Ctrl Pts',(-4.89999269604004,-6.44945650152635,
-12.4299926960872)) ;
#164158=CARTESIAN_POINT('Ctrl Pts',(-4.80000000081823,-6.46309229646328,
-12.43)) ;
#164159=CARTESIAN_POINT('Ctrl Pts',(-4.9,-6.45,-12.33)) ;
#164160=CARTESIAN_POINT('Ctrl Pts',(-4.9,-6.45,-12.43)) ;
#164161=CARTESIAN_POINT('Ctrl Pts',(-4.8,-6.45,-12.43)) ;
#164162=CARTESIAN_POINT('Ctrl Pts',(-5.82426676739351,-5.4339930370061,
-9.82701096596875)) ;
#164163=CARTESIAN_POINT('Ctrl Pts',(-5.80266988778316,-5.52572360682928,
-9.83235401735051)) ;
#164164=CARTESIAN_POINT('Ctrl Pts',(-5.82426676352015,-5.53106667371341,
-9.92408458718265)) ;
#164165=CARTESIAN_POINT('Ctrl Pts',(-5.83498671931116,-5.43935351191906,
-9.82432945819617)) ;
#164166=CARTESIAN_POINT('Ctrl Pts',(-5.80595263122268,-5.52411753147701,
-9.83396009354034)) ;
#164167=CARTESIAN_POINT('Ctrl Pts',(-5.83498671397627,-5.53374818067468,
-9.9187241131463)) ;
#164168=CARTESIAN_POINT('Ctrl Pts',(-5.84526105845716,-5.44830326289491,
-9.81985284019616)) ;
#164169=CARTESIAN_POINT('Ctrl Pts',(-5.81370932746138,-5.52260132030847,
-9.83547630599898)) ;
#164170=CARTESIAN_POINT('Ctrl Pts',(-5.84526105243718,-5.53822479746337,
-9.90977436356971)) ;
#164171=CARTESIAN_POINT('Ctrl Pts',(-5.86378685403699,-5.47240020430401,
-9.80780325130868)) ;
#164172=CARTESIAN_POINT('Ctrl Pts',(-5.83531854275287,-5.52733067404477,
-9.83074695511466)) ;
#164173=CARTESIAN_POINT('Ctrl Pts',(-5.86378684816458,-5.55027438459897,
-9.88567742500545)) ;
#164174=CARTESIAN_POINT('Ctrl Pts',(-5.87203852631578,-5.48754495134734,
-9.80023155289438)) ;
#164175=CARTESIAN_POINT('Ctrl Pts',(-5.84834787930686,-5.53310199490447,
-9.82497563577609)) ;
#164176=CARTESIAN_POINT('Ctrl Pts',(-5.87203852123038,-5.55784608243454,
-9.8705326795139)) ;
#164177=CARTESIAN_POINT('Ctrl Pts',(-5.89242747304797,-5.53981202333454,
-9.7741056511376)) ;
#164178=CARTESIAN_POINT('Ctrl Pts',(-5.88223383300419,-5.56084219179272,
-9.79723544317417)) ;
#164179=CARTESIAN_POINT('Ctrl Pts',(-5.892427470635,-5.58397198402772,-9.81826561232779)) ;
#164180=CARTESIAN_POINT('Ctrl Pts',(-5.9,-5.58381083947299,-9.752119400143)) ;
#164181=CARTESIAN_POINT('Ctrl Pts',(-5.9,-5.59485304502621,-9.76322459288697)) ;
#164182=CARTESIAN_POINT('Ctrl Pts',(-5.9,-5.60595823775496,-9.77426679844052)) ;
#164183=CARTESIAN_POINT('Ctrl Pts',(-5.9,-5.62807764064044,-9.73)) ;
#164184=CARTESIAN_POINT('Ctrl Pts',(-5.9,-5.62807764064044,-9.73)) ;
#164185=CARTESIAN_POINT('Ctrl Pts',(-5.9,-5.62807764064044,-9.73)) ;
#164186=CARTESIAN_POINT('Origin',(-5.84850712500726,-5.43404914061138,-9.92402850002907)) ;
#164187=CARTESIAN_POINT('Ctrl Pts',(-5.82425356250363,-5.53106339062591,
-9.92402850002907)) ;
#164188=CARTESIAN_POINT('Ctrl Pts',(-5.80269484027818,-5.52567371006955,
-9.83240393057089)) ;
#164189=CARTESIAN_POINT('Ctrl Pts',(-5.82425356250363,-5.43404914061138,
-9.82701425001453)) ;
#164190=CARTESIAN_POINT('Ctrl Pts',(-5.80840777707097,-5.52710194426774,
-9.92798994590438)) ;
#164191=CARTESIAN_POINT('Ctrl Pts',(-5.7934141764523,-5.52335354411309,
-9.83283584981848)) ;
#164192=CARTESIAN_POINT('Ctrl Pts',(-5.81633079157287,-5.4300877551176,
-9.82899494274722)) ;
#164193=CARTESIAN_POINT('Ctrl Pts',(-5.79207992677988,-5.52301998169497,
-9.92999999953396)) ;
#164194=CARTESIAN_POINT('Ctrl Pts',(-5.78430903206643,-5.52107725801661,
-9.83196139543284)) ;
#164195=CARTESIAN_POINT('Ctrl Pts',(-5.808166653183,-5.42600568595106,-9.83)) ;
#164196=CARTESIAN_POINT('Ctrl Pts',(-5.77574643749636,-5.51893660937409,
-9.93)) ;
#164197=CARTESIAN_POINT('Ctrl Pts',(-5.77574643749636,-5.51893660937409,
-9.83)) ;
#164198=CARTESIAN_POINT('Ctrl Pts',(-5.8,-5.42192235935956,-9.83)) ;
#164199=CARTESIAN_POINT('Origin',(-5.8,-5.42192235935956,-9.93)) ;
#164200=CARTESIAN_POINT('Origin',(-5.8066065036801,-5.42357398527959,-9.93)) ;
#164201=CARTESIAN_POINT('Origin',(-5.17275707706436,-5.26511162862565,-9.93)) ;
#164202=CARTESIAN_POINT('Origin',(-5.15068655017073,-5.25959399690224,-9.94059385290894)) ;
#164203=CARTESIAN_POINT('Origin',(-5.17275707706436,-5.26511162862565,-9.93)) ;
#164204=CARTESIAN_POINT('Origin',(-5.17275707706436,-5.26511162862565,-9.93)) ;
#164205=CARTESIAN_POINT('Origin',(-5.17275707706436,-5.26511162862565,-9.93)) ;
#164206=CARTESIAN_POINT('Origin',(-5.17275707706436,-5.05,-9.93)) ;
#164207=CARTESIAN_POINT('Origin',(-5.17275707706436,-1.91866427917294,-9.93)) ;
#164208=CARTESIAN_POINT('Origin',(-3.78014014831103,-3.31128120792626,-10.5984561258016)) ;
#164209=CARTESIAN_POINT('Origin',(-5.17275707706437,-1.91866427917293,-9.93)) ;
#164210=CARTESIAN_POINT('Origin',(-5.17275707706436,-1.91866427917293,-9.93)) ;
#164211=CARTESIAN_POINT('Origin',(-5.17275707706436,-1.91866427917294,-9.93)) ;
#164212=CARTESIAN_POINT('Origin',(-3.97071067811865,-3.12071067811865,-9.93)) ;
#164213=CARTESIAN_POINT('Origin',(-5.8,-1.2914213562373,-9.93)) ;
#164214=CARTESIAN_POINT('Ctrl Pts',(-5.87071067811865,-1.14999999999999,
-9.80071067811865)) ;
#164215=CARTESIAN_POINT('Ctrl Pts',(-5.8471404520791,-1.10285954792089,
-9.8242809041582)) ;
#164216=CARTESIAN_POINT('Ctrl Pts',(-5.87071067811865,-1.07928932188134,
-9.87142135623731)) ;
#164217=CARTESIAN_POINT('Ctrl Pts',(-5.85217562795664,-1.18707010095463,
-9.81924572828067)) ;
#164218=CARTESIAN_POINT('Ctrl Pts',(-5.81261165662074,-1.13738834337929,
-9.84586147194964)) ;
#164219=CARTESIAN_POINT('Ctrl Pts',(-5.83353949671041,-1.11646050328958,
-9.90859253638103)) ;
#164220=CARTESIAN_POINT('Ctrl Pts',(-5.82627077431947,-1.23887980759831,
-9.83)) ;
#164221=CARTESIAN_POINT('Ctrl Pts',(-5.76566787907945,-1.18433212092055,
-9.84714894371283)) ;
#164222=CARTESIAN_POINT('Ctrl Pts',(-5.78190678732235,-1.16809321267764,
-9.9299999994186)) ;
#164223=CARTESIAN_POINT('Ctrl Pts',(-5.8,-1.2914213562373,-9.83)) ;
#164224=CARTESIAN_POINT('Ctrl Pts',(-5.72928932188134,-1.22071067811865,
-9.83)) ;
#164225=CARTESIAN_POINT('Ctrl Pts',(-5.72928932188134,-1.22071067811865,
-9.93)) ;
#164226=CARTESIAN_POINT('Origin',(-5.94142135623731,-1.14999999999999,-9.87142135623731)) ;
#164227=CARTESIAN_POINT('Ctrl Pts',(-5.9,-1.00857864376269,-9.73)) ;
#164228=CARTESIAN_POINT('Ctrl Pts',(-5.9,-1.00857864376269,-9.73)) ;
#164229=CARTESIAN_POINT('Ctrl Pts',(-5.9,-1.00857864376269,-9.73)) ;
#164230=CARTESIAN_POINT('Ctrl Pts',(-5.9,-1.06112019240168,-9.75627077431956)) ;
#164231=CARTESIAN_POINT('Ctrl Pts',(-5.9,-1.04860238143836,-9.77002373767573)) ;
#164232=CARTESIAN_POINT('Ctrl Pts',(-5.9,-1.03484941808221,-9.78254154863898)) ;
#164233=CARTESIAN_POINT('Ctrl Pts',(-5.88924572828063,-1.11292989904529,
-9.78217562795668)) ;
#164234=CARTESIAN_POINT('Ctrl Pts',(-5.87451700624548,-1.08721613124892,
-9.80863748748634)) ;
#164235=CARTESIAN_POINT('Ctrl Pts',(-5.88924572828066,-1.06075427171933,
-9.83435125528267)) ;
#164236=CARTESIAN_POINT('Ctrl Pts',(-5.87071067811865,-1.14999999999999,
-9.80071067811865)) ;
#164237=CARTESIAN_POINT('Ctrl Pts',(-5.8471404520791,-1.10285954792089,
-9.82428090415821)) ;
#164238=CARTESIAN_POINT('Ctrl Pts',(-5.87071067811865,-1.07928932188134,
-9.87142135623731)) ;
#164239=CARTESIAN_POINT('Ctrl Pts',(-5.87071067811866,-1.14999999999999,
-13.0592893218813)) ;
#164240=CARTESIAN_POINT('Ctrl Pts',(-5.84714045207911,-1.10285954792089,
-13.0357190958418)) ;
#164241=CARTESIAN_POINT('Ctrl Pts',(-5.87071067811866,-1.07928932188134,
-12.9885786437627)) ;
#164242=CARTESIAN_POINT('Ctrl Pts',(-5.88924572828065,-1.11292989904533,
-13.0778243720433)) ;
#164243=CARTESIAN_POINT('Ctrl Pts',(-5.87451700625929,-1.08721613124107,
-13.0513625125215)) ;
#164244=CARTESIAN_POINT('Ctrl Pts',(-5.8892457282807,-1.06075427171929,
-13.0256487447173)) ;
#164245=CARTESIAN_POINT('Ctrl Pts',(-5.9,-1.06112019240165,-13.1037292256804)) ;
#164246=CARTESIAN_POINT('Ctrl Pts',(-5.9,-1.04860238144452,-13.0899762623181)) ;
#164247=CARTESIAN_POINT('Ctrl Pts',(-5.9,-1.03484941808214,-13.077458451361)) ;
#164248=CARTESIAN_POINT('Ctrl Pts',(-5.9,-1.00857864376269,-13.13)) ;
#164249=CARTESIAN_POINT('Ctrl Pts',(-5.9,-1.00857864376269,-13.13)) ;
#164250=CARTESIAN_POINT('Ctrl Pts',(-5.9,-1.00857864376269,-13.13)) ;
#164251=CARTESIAN_POINT('Origin',(-5.94142135623734,-1.14999999999996,-12.9885786437627)) ;
#164252=CARTESIAN_POINT('Ctrl Pts',(-5.8,-1.2914213562373,-13.03)) ;
#164253=CARTESIAN_POINT('Ctrl Pts',(-5.72928932188134,-1.22071067811865,
-13.03)) ;
#164254=CARTESIAN_POINT('Ctrl Pts',(-5.72928932188134,-1.22071067811865,
-12.93)) ;
#164255=CARTESIAN_POINT('Ctrl Pts',(-5.82627077431945,-1.23887980759835,
-13.03)) ;
#164256=CARTESIAN_POINT('Ctrl Pts',(-5.76566787907943,-1.18433212092059,
-13.0128510562869)) ;
#164257=CARTESIAN_POINT('Ctrl Pts',(-5.78190678732238,-1.16809321267762,
-12.9300000005814)) ;
#164258=CARTESIAN_POINT('Ctrl Pts',(-5.85217562795658,-1.18707010095451,
-13.0407542717193)) ;
#164259=CARTESIAN_POINT('Ctrl Pts',(-5.81261165662068,-1.13738834337918,
-13.0141385280506)) ;
#164260=CARTESIAN_POINT('Ctrl Pts',(-5.83353949671039,-1.11646050328961,
-12.951407463619)) ;
#164261=CARTESIAN_POINT('Ctrl Pts',(-5.87071067811866,-1.14999999999999,
-13.0592893218813)) ;
#164262=CARTESIAN_POINT('Ctrl Pts',(-5.84714045207911,-1.10285954792089,
-13.0357190958418)) ;
#164263=CARTESIAN_POINT('Ctrl Pts',(-5.87071067811866,-1.07928932188133,
-12.9885786437627)) ;
#164264=CARTESIAN_POINT('Origin',(-5.8,-1.29142135623731,-12.93)) ;
#164265=CARTESIAN_POINT('Origin',(-3.59571067811865,-3.49571067811865,-12.93)) ;
#164266=CARTESIAN_POINT('Origin',(-5.17275707706436,-1.91866427917293,-12.93)) ;
#164267=CARTESIAN_POINT('Origin',(-3.09057773798104,-4.00084361825625,-11.93055391724)) ;
#164268=CARTESIAN_POINT('Origin',(-5.17275707706436,-1.91866427917294,-12.93)) ;
#164269=CARTESIAN_POINT('Origin',(-5.17275707706436,-1.91866427917293,-12.93)) ;
#164270=CARTESIAN_POINT('Origin',(-5.17275707706436,-1.91866427917293,-12.93)) ;
#164271=CARTESIAN_POINT('Origin',(-5.17275707706436,-5.05,-12.93)) ;
#164272=CARTESIAN_POINT('Origin',(-5.17275707706436,-5.26511162862565,-12.93)) ;
#164273=CARTESIAN_POINT('Origin',(-3.96111272388873,-4.96220054033175,-12.3484107104757)) ;
#164274=CARTESIAN_POINT('Origin',(-5.17275707706437,-5.26511162862565,-12.93)) ;
#164275=CARTESIAN_POINT('Origin',(-5.17275707706436,-5.26511162862565,-12.93)) ;
#164276=CARTESIAN_POINT('Origin',(-5.17275707706436,-5.26511162862565,-12.93)) ;
#164277=CARTESIAN_POINT('Origin',(-5.10072415073893,-5.24710339704429,-12.93)) ;
#164278=CARTESIAN_POINT('Origin',(-5.8,-5.42192235935956,-12.93)) ;
#164279=CARTESIAN_POINT('Ctrl Pts',(-5.77574643749636,-5.51893660937409,
-12.93)) ;
#164280=CARTESIAN_POINT('Ctrl Pts',(-5.77574643749636,-5.51893660937409,
-13.03)) ;
#164281=CARTESIAN_POINT('Ctrl Pts',(-5.8,-5.42192235935956,-13.03)) ;
#164282=CARTESIAN_POINT('Ctrl Pts',(-5.79207992677988,-5.52301998169497,
-12.930000000466)) ;
#164283=CARTESIAN_POINT('Ctrl Pts',(-5.78430903206646,-5.52107725801655,
-13.0280386045672)) ;
#164284=CARTESIAN_POINT('Ctrl Pts',(-5.808166653183,-5.42600568595104,-13.03)) ;
#164285=CARTESIAN_POINT('Ctrl Pts',(-5.80840777707096,-5.52710194426774,
-12.9320100540956)) ;
#164286=CARTESIAN_POINT('Ctrl Pts',(-5.7934141764523,-5.52335354411304,
-13.0271641501816)) ;
#164287=CARTESIAN_POINT('Ctrl Pts',(-5.81633079157287,-5.4300877551176,
-13.0310050572528)) ;
#164288=CARTESIAN_POINT('Ctrl Pts',(-5.82425356250363,-5.53106339062591,
-12.9359714999709)) ;
#164289=CARTESIAN_POINT('Ctrl Pts',(-5.80269484027818,-5.52567371006955,
-13.0275960694291)) ;
#164290=CARTESIAN_POINT('Ctrl Pts',(-5.82425356250363,-5.43404914061138,
-13.0329857499855)) ;
#164291=CARTESIAN_POINT('Origin',(-5.84850712500726,-5.43404914061138,-12.9359714999709)) ;
#164292=CARTESIAN_POINT('Ctrl Pts',(-5.82426676739353,-5.53106667467168,
-12.9359153963655)) ;
#164293=CARTESIAN_POINT('Ctrl Pts',(-5.80266988778304,-5.52572362328999,
-13.0276459661892)) ;
#164294=CARTESIAN_POINT('Ctrl Pts',(-5.82426676352026,-5.43399305345736,
-13.0329890330731)) ;
#164295=CARTESIAN_POINT('Ctrl Pts',(-5.83498671931122,-5.53374818244429,
-12.9412758712785)) ;
#164296=CARTESIAN_POINT('Ctrl Pts',(-5.80595263122252,-5.52411754710016,
-13.0260398908369)) ;
#164297=CARTESIAN_POINT('Ctrl Pts',(-5.83498671397638,-5.4393535274938,
-13.0356705400343)) ;
#164298=CARTESIAN_POINT('Ctrl Pts',(-5.84526105845717,-5.53822480044429,
-12.9502256222545)) ;
#164299=CARTESIAN_POINT('Ctrl Pts',(-5.81370932746123,-5.52260133464142,
-13.0245236796683)) ;
#164300=CARTESIAN_POINT('Ctrl Pts',(-5.84526105243736,-5.44830327707034,
-13.0401471568231)) ;
#164301=CARTESIAN_POINT('Ctrl Pts',(-5.86378685403702,-5.5502743893318,
-12.9743225636635)) ;
#164302=CARTESIAN_POINT('Ctrl Pts',(-5.83531854275273,-5.52733068552576,
-13.0292530334046)) ;
#164303=CARTESIAN_POINT('Ctrl Pts',(-5.86378684816473,-5.47240021563469,
-13.0521967439587)) ;
#164304=CARTESIAN_POINT('Ctrl Pts',(-5.87203852631581,-5.5578460877461,
-12.9894673107069)) ;
#164305=CARTESIAN_POINT('Ctrl Pts',(-5.84834787930675,-5.53310200486434,
-13.0350243542641)) ;
#164306=CARTESIAN_POINT('Ctrl Pts',(-5.87203852123052,-5.48754496112629,
-13.0597684417942)) ;
#164307=CARTESIAN_POINT('Ctrl Pts',(-5.89242747304798,-5.58397198950286,
-13.0417343826941)) ;
#164308=CARTESIAN_POINT('Ctrl Pts',(-5.88223383300414,-5.56084219746614,
-13.0627645511524)) ;
#164309=CARTESIAN_POINT('Ctrl Pts',(-5.89242747063508,-5.53981202831252,
-13.0858943433875)) ;
#164310=CARTESIAN_POINT('Ctrl Pts',(-5.9,-5.60595824049745,-13.0857331988325)) ;
#164311=CARTESIAN_POINT('Ctrl Pts',(-5.9,-5.59485304775402,-13.0967754043861)) ;
#164312=CARTESIAN_POINT('Ctrl Pts',(-5.9,-5.58381084219975,-13.1078805971148)) ;
#164313=CARTESIAN_POINT('Ctrl Pts',(-5.9,-5.62807764064044,-13.13)) ;
#164314=CARTESIAN_POINT('Ctrl Pts',(-5.9,-5.62807764064044,-13.13)) ;
#164315=CARTESIAN_POINT('Ctrl Pts',(-5.9,-5.62807764064044,-13.13)) ;
#164316=CARTESIAN_POINT('Origin',(7.8,2.1,-11.83)) ;
#164317=CARTESIAN_POINT('Origin',(7.8,2.1,-12.03)) ;
#164318=CARTESIAN_POINT('Origin',(7.6,2.1,-11.83)) ;
#164319=CARTESIAN_POINT('Origin',(7.6,2.1,-11.83)) ;
#164320=CARTESIAN_POINT('Origin',(7.6,2.1,-11.03)) ;
#164321=CARTESIAN_POINT('Origin',(7.8,2.1,-12.03)) ;
#164322=CARTESIAN_POINT('Origin',(9.6,2.1,-12.03)) ;
#164323=CARTESIAN_POINT('Origin',(7.8,2.1,-11.03)) ;
#164324=CARTESIAN_POINT('Origin',(7.8,2.1,-10.83)) ;
#164325=CARTESIAN_POINT('Origin',(9.6,2.1,-11.83)) ;
#164326=CARTESIAN_POINT('Origin',(9.8,2.1,-11.83)) ;
#164327=CARTESIAN_POINT('Origin',(7.8,2.1,-10.83)) ;
#164328=CARTESIAN_POINT('Origin',(9.6,2.1,-10.83)) ;
#164329=CARTESIAN_POINT('Origin',(9.8,2.1,-11.83)) ;
#164330=CARTESIAN_POINT('Origin',(9.8,2.1,-11.03)) ;
#164331=CARTESIAN_POINT('Origin',(9.6,2.1,-11.03)) ;
#164332=CARTESIAN_POINT('Origin',(-4.15,-6.25,-10.68)) ;
#164333=CARTESIAN_POINT('Origin',(-4.15,-6.3,-10.68)) ;
#164334=CARTESIAN_POINT('Origin',(-4.15,-6.3,-11.43)) ;
#164335=CARTESIAN_POINT('Origin',(-4.15,-6.3,-12.18)) ;
#164336=CARTESIAN_POINT('Origin',(-4.15,-6.3,-10.68)) ;
#164337=CARTESIAN_POINT('Origin',(-4.15,-6.25,-12.18)) ;
#164338=CARTESIAN_POINT('Origin',(-4.15,-6.3,-12.18)) ;
#164339=CARTESIAN_POINT('Origin',(-4.15,-6.3,-10.68)) ;
#164340=CARTESIAN_POINT('Origin',(-4.15,-6.3,-10.68)) ;
#164341=CARTESIAN_POINT('Origin',(-4.15,-6.3,-12.18)) ;
#164342=CARTESIAN_POINT('Origin',(-4.15,-6.3,-12.18)) ;
#164343=CARTESIAN_POINT('Origin',(-4.65,-6.25,-10.68)) ;
#164344=CARTESIAN_POINT('Origin',(-4.65,-6.3,-10.68)) ;
#164345=CARTESIAN_POINT('Origin',(0.,-6.3,-10.68)) ;
#164346=CARTESIAN_POINT('Origin',(-4.65,-6.3,-10.68)) ;
#164347=CARTESIAN_POINT('Origin',(0.,-6.3,-12.18)) ;
#164348=CARTESIAN_POINT('Origin',(-4.65,-6.3,-12.18)) ;
#164349=CARTESIAN_POINT('Origin',(-4.65,-6.25,-12.18)) ;
#164350=CARTESIAN_POINT('Origin',(-4.65,-6.3,-12.18)) ;
#164351=CARTESIAN_POINT('Origin',(-4.65,-6.3,-10.68)) ;
#164352=CARTESIAN_POINT('Origin',(-4.65,-6.3,-10.68)) ;
#164353=CARTESIAN_POINT('Origin',(-4.65,-6.3,-12.18)) ;
#164354=CARTESIAN_POINT('Origin',(-4.65,-6.3,-12.18)) ;
#164355=CARTESIAN_POINT('Origin',(-4.65,-6.3,-11.43)) ;
#164356=CARTESIAN_POINT('Origin',(-3.,4.45,-12.53)) ;
#164357=CARTESIAN_POINT('Origin',(-2.1,4.45,-12.53)) ;
#164358=CARTESIAN_POINT('Origin',(-2.9,4.45,-12.53)) ;
#164359=CARTESIAN_POINT('Origin',(-2.9,4.45,-12.33)) ;
#164360=CARTESIAN_POINT('Origin',(-3.1,4.45,-12.33)) ;
#164361=CARTESIAN_POINT('Origin',(-2.9,4.45,-12.33)) ;
#164362=CARTESIAN_POINT('Origin',(-2.1,4.45,-12.33)) ;
#164363=CARTESIAN_POINT('Origin',(-2.1,4.45,-12.33)) ;
#164364=CARTESIAN_POINT('Origin',(-1.9,4.45,-12.33)) ;
#164365=CARTESIAN_POINT('Origin',(-3.1,4.45,-12.43)) ;
#164366=CARTESIAN_POINT('Origin',(-3.1,4.45,-10.53)) ;
#164367=CARTESIAN_POINT('Origin',(-2.9,4.4,-12.33)) ;
#164368=CARTESIAN_POINT('Origin',(-2.9,4.35,-12.33)) ;
#164369=CARTESIAN_POINT('Origin',(-1.95156391047391E-16,4.35,-12.33)) ;
#164370=CARTESIAN_POINT('Origin',(-2.1,4.35,-12.33)) ;
#164371=CARTESIAN_POINT('Origin',(-2.9,4.35,-12.33)) ;
#164372=CARTESIAN_POINT('Origin',(-2.1,4.4,-12.33)) ;
#164373=CARTESIAN_POINT('Origin',(-2.1,4.35,-12.33)) ;
#164374=CARTESIAN_POINT('Origin',(-1.9,4.45,-12.43)) ;
#164375=CARTESIAN_POINT('Origin',(-1.9,4.45,-10.53)) ;
#164376=CARTESIAN_POINT('Origin',(-3.,4.45,-10.33)) ;
#164377=CARTESIAN_POINT('Origin',(-2.9,4.45,-10.33)) ;
#164378=CARTESIAN_POINT('Origin',(-2.1,4.45,-10.33)) ;
#164379=CARTESIAN_POINT('Origin',(-2.9,4.45,-10.53)) ;
#164380=CARTESIAN_POINT('Origin',(-2.9,4.45,-10.53)) ;
#164381=CARTESIAN_POINT('Origin',(-2.9,4.35,-12.33)) ;
#164382=CARTESIAN_POINT('Origin',(-2.9,4.35,-12.33)) ;
#164383=CARTESIAN_POINT('Origin',(-2.1,4.35,-12.33)) ;
#164384=CARTESIAN_POINT('Origin',(-2.1,4.35,-12.33)) ;
#164385=CARTESIAN_POINT('Origin',(-2.1,4.45,-10.53)) ;
#164386=CARTESIAN_POINT('Origin',(-2.1,4.45,-10.53)) ;
#164387=CARTESIAN_POINT('Origin',(-2.9,4.4,-10.53)) ;
#164388=CARTESIAN_POINT('Origin',(-2.9,4.35,-10.53)) ;
#164389=CARTESIAN_POINT('Origin',(-2.9,4.35,-11.43)) ;
#164390=CARTESIAN_POINT('Origin',(-2.9,4.35,-10.53)) ;
#164391=CARTESIAN_POINT('Origin',(-2.1,4.35,-11.43)) ;
#164392=CARTESIAN_POINT('Origin',(-2.1,4.35,-10.53)) ;
#164393=CARTESIAN_POINT('Origin',(-2.1,4.4,-10.53)) ;
#164394=CARTESIAN_POINT('Origin',(-2.1,4.35,-10.53)) ;
#164395=CARTESIAN_POINT('Origin',(-2.9,4.35,-10.53)) ;
#164396=CARTESIAN_POINT('Origin',(-2.9,4.35,-10.53)) ;
#164397=CARTESIAN_POINT('Origin',(-2.1,4.35,-10.53)) ;
#164398=CARTESIAN_POINT('Origin',(-2.1,4.35,-10.53)) ;
#164399=CARTESIAN_POINT('Origin',(-1.95156391047391E-16,4.35,-10.53)) ;
#164400=CARTESIAN_POINT('Origin',(-2.25,4.25,-12.18)) ;
#164401=CARTESIAN_POINT('Origin',(-2.25,4.3,-12.18)) ;
#164402=CARTESIAN_POINT('Origin',(-2.25,4.3,-11.43)) ;
#164403=CARTESIAN_POINT('Origin',(-2.25,4.3,-10.68)) ;
#164404=CARTESIAN_POINT('Origin',(-2.25,4.3,-12.18)) ;
#164405=CARTESIAN_POINT('Origin',(-2.25,4.25,-10.68)) ;
#164406=CARTESIAN_POINT('Origin',(-2.25,4.3,-10.68)) ;
#164407=CARTESIAN_POINT('Origin',(-2.25,4.3,-12.18)) ;
#164408=CARTESIAN_POINT('Origin',(-2.25,4.3,-12.18)) ;
#164409=CARTESIAN_POINT('Origin',(-2.25,4.3,-10.68)) ;
#164410=CARTESIAN_POINT('Origin',(-2.25,4.3,-10.68)) ;
#164411=CARTESIAN_POINT('Origin',(-2.75,4.25,-12.18)) ;
#164412=CARTESIAN_POINT('Origin',(-2.75,4.3,-12.18)) ;
#164413=CARTESIAN_POINT('Origin',(-1.97127667724637E-17,4.3,-12.18)) ;
#164414=CARTESIAN_POINT('Origin',(-2.75,4.3,-12.18)) ;
#164415=CARTESIAN_POINT('Origin',(-1.97127667724637E-17,4.3,-10.68)) ;
#164416=CARTESIAN_POINT('Origin',(-2.75,4.3,-10.68)) ;
#164417=CARTESIAN_POINT('Origin',(-2.75,4.25,-10.68)) ;
#164418=CARTESIAN_POINT('Origin',(-2.75,4.3,-10.68)) ;
#164419=CARTESIAN_POINT('Origin',(-2.75,4.3,-12.18)) ;
#164420=CARTESIAN_POINT('Origin',(-2.75,4.3,-12.18)) ;
#164421=CARTESIAN_POINT('Origin',(-2.75,4.3,-10.68)) ;
#164422=CARTESIAN_POINT('Origin',(-2.75,4.3,-10.68)) ;
#164423=CARTESIAN_POINT('Origin',(-2.75,4.3,-11.43)) ;
#164424=CARTESIAN_POINT('Origin',(7.8,2.9,-11.83)) ;
#164425=CARTESIAN_POINT('Origin',(7.8,2.9,-11.83)) ;
#164426=CARTESIAN_POINT('Origin',(7.8,2.9,-11.03)) ;
#164427=CARTESIAN_POINT('Origin',(7.8,2.9,-11.03)) ;
#164428=CARTESIAN_POINT('Origin',(7.8,2.9,-11.03)) ;
#164429=CARTESIAN_POINT('Origin',(7.8,2.9,-11.83)) ;
#164430=CARTESIAN_POINT('Origin',(7.8,2.9,-11.83)) ;
#164431=CARTESIAN_POINT('Origin',(9.6,2.9,-11.03)) ;
#164432=CARTESIAN_POINT('Origin',(9.6,2.9,-11.03)) ;
#164433=CARTESIAN_POINT('Origin',(9.6,2.9,-11.83)) ;
#164434=CARTESIAN_POINT('Origin',(9.6,2.9,-11.83)) ;
#164435=CARTESIAN_POINT('Origin',(9.6,2.9,-11.03)) ;
#164436=CARTESIAN_POINT('Origin',(9.6,2.9,-11.03)) ;
#164437=CARTESIAN_POINT('Origin',(9.6,2.9,-11.83)) ;
#164438=CARTESIAN_POINT('Origin',(9.6,2.9,-11.83)) ;
#164439=CARTESIAN_POINT('Origin',(9.6,2.9,-11.83)) ;
#164440=CARTESIAN_POINT('Origin',(-0.183301359729408,3.45,-9.91296321352402)) ;
#164441=CARTESIAN_POINT('Origin',(0.249234641435079,3.15,-11.3137799780213)) ;
#164442=CARTESIAN_POINT('Origin',(-0.249234641435079,3.15,-11.5462200219787)) ;
#164443=CARTESIAN_POINT('Origin',(-1.04429375741423,3.45,-10.3144505621777)) ;
#164444=CARTESIAN_POINT('Origin',(10.1,-2.15,-14.3368804065906)) ;
#164445=CARTESIAN_POINT('Origin',(10.1,-2.15,-14.3368804065906)) ;
#164446=CARTESIAN_POINT('Origin',(10.1,-2.15,-14.3368804065906)) ;
#164447=CARTESIAN_POINT('Origin',(10.1,-2.15,-14.3368804065906)) ;
#164448=CARTESIAN_POINT('Origin',(10.1,-2.15,-15.24)) ;
#164449=CARTESIAN_POINT('Origin',(10.1,-2.15,-13.935)) ;
#164450=CARTESIAN_POINT('Origin',(10.2,-2.15,-14.3368804065906)) ;
#164451=CARTESIAN_POINT('Origin',(3.7,-2.15,-14.3368804065906)) ;
#164452=CARTESIAN_POINT('Origin',(10.1,-3.65625,-15.24)) ;
#164453=CARTESIAN_POINT('Origin',(10.1,-2.15,-16.1431195934094)) ;
#164454=CARTESIAN_POINT('Origin',(10.1,-3.65625,-13.935)) ;
#164455=CARTESIAN_POINT('Origin',(10.1,1.9,-13.935)) ;
#164456=CARTESIAN_POINT('Origin',(10.1,-2.15,-13.935)) ;
#164457=CARTESIAN_POINT('Origin',(10.1,-2.15,-13.935)) ;
#164458=CARTESIAN_POINT('Origin',(10.1,-2.15,-13.935)) ;
#164459=CARTESIAN_POINT('Origin',(3.7,-2.15,-14.3368804065906)) ;
#164460=CARTESIAN_POINT('Origin',(3.7,-2.32153024911032,-14.4397267659824)) ;
#164461=CARTESIAN_POINT('Origin',(3.7,-2.35,-14.3368804065906)) ;
#164462=CARTESIAN_POINT('Origin',(10.1,-2.15,-16.1431195934094)) ;
#164463=CARTESIAN_POINT('Origin',(10.1,-2.15,-16.1431195934094)) ;
#164464=CARTESIAN_POINT('Origin',(10.1,-2.15,-16.1431195934094)) ;
#164465=CARTESIAN_POINT('Origin',(10.1,1.9,-15.24)) ;
#164466=CARTESIAN_POINT('Origin',(10.1,1.9,-16.545)) ;
#164467=CARTESIAN_POINT('Origin',(10.1,1.9,-13.935)) ;
#164468=CARTESIAN_POINT('Origin',(10.2,-2.15,-13.935)) ;
#164469=CARTESIAN_POINT('Origin',(3.7,-2.15,-13.935)) ;
#164470=CARTESIAN_POINT('Origin',(3.7,-2.35,-13.835)) ;
#164471=CARTESIAN_POINT('Origin',(3.7,-2.35,-13.935)) ;
#164472=CARTESIAN_POINT('Origin',(3.7,-3.65625,-15.24)) ;
#164473=CARTESIAN_POINT('Origin',(3.7,-2.32153024911032,-16.0402732340176)) ;
#164474=CARTESIAN_POINT('Origin',(10.2,-2.15,-16.1431195934094)) ;
#164475=CARTESIAN_POINT('Origin',(3.7,-2.15,-16.1431195934094)) ;
#164476=CARTESIAN_POINT('Origin',(10.1,-2.15,-15.24)) ;
#164477=CARTESIAN_POINT('Origin',(10.1,-2.15,-16.545)) ;
#164478=CARTESIAN_POINT('Origin',(10.1,-3.65625,-16.545)) ;
#164479=CARTESIAN_POINT('Origin',(10.1,1.9,-16.545)) ;
#164480=CARTESIAN_POINT('Origin',(10.1,-2.15,-16.545)) ;
#164481=CARTESIAN_POINT('Origin',(3.7,-2.35,-13.935)) ;
#164482=CARTESIAN_POINT('Origin',(3.5,-2.35,-13.935)) ;
#164483=CARTESIAN_POINT('Origin',(3.7,-2.15,-16.1431195934094)) ;
#164484=CARTESIAN_POINT('Origin',(3.7,-2.35,-16.1431195934094)) ;
#164485=CARTESIAN_POINT('Origin',(10.1,-2.15,-16.545)) ;
#164486=CARTESIAN_POINT('Origin',(10.1,-2.15,-16.545)) ;
#164487=CARTESIAN_POINT('Origin',(3.6,1.9,-13.735)) ;
#164488=CARTESIAN_POINT('Origin',(3.5,1.9,-13.735)) ;
#164489=CARTESIAN_POINT('Origin',(2.7,1.9,-13.735)) ;
#164490=CARTESIAN_POINT('Origin',(3.5,1.32848750596453E-15,-13.935)) ;
#164491=CARTESIAN_POINT('Origin',(3.5,-5.15,-13.935)) ;
#164492=CARTESIAN_POINT('Origin',(3.7,-2.35,-16.115)) ;
#164493=CARTESIAN_POINT('Origin',(3.7,-2.35,-16.545)) ;
#164494=CARTESIAN_POINT('Origin',(3.6,-2.15,-16.545)) ;
#164495=CARTESIAN_POINT('Origin',(3.7,-2.15,-16.545)) ;
#164496=CARTESIAN_POINT('Origin',(2.7,1.9,-13.735)) ;
#164497=CARTESIAN_POINT('Origin',(2.7,1.9,-13.735)) ;
#164498=CARTESIAN_POINT('Origin',(3.5,-5.15,-13.935)) ;
#164499=CARTESIAN_POINT('Origin',(3.5,-5.15,-13.935)) ;
#164500=CARTESIAN_POINT('Origin',(3.5,-5.15,-13.935)) ;
#164501=CARTESIAN_POINT('Origin',(3.7,-2.35,-16.545)) ;
#164502=CARTESIAN_POINT('Origin',(3.5,-2.35,-16.545)) ;
#164503=CARTESIAN_POINT('Origin',(2.7,2.,-13.735)) ;
#164504=CARTESIAN_POINT('Origin',(2.7,-5.15,-13.735)) ;
#164505=CARTESIAN_POINT('Origin',(3.6,-5.15,-13.935)) ;
#164506=CARTESIAN_POINT('Origin',(2.7,-5.15,-13.935)) ;
#164507=CARTESIAN_POINT('Origin',(3.5,-5.15,0.)) ;
#164508=CARTESIAN_POINT('Origin',(3.5,-5.15,-16.545)) ;
#164509=CARTESIAN_POINT('Origin',(3.5,-1.40639378098925E-15,-16.545)) ;
#164510=CARTESIAN_POINT('Origin',(3.5,-5.15,-16.545)) ;
#164511=CARTESIAN_POINT('Origin',(2.7,-5.15,-13.935)) ;
#164512=CARTESIAN_POINT('Origin',(2.7,-5.35,-13.935)) ;
#164513=CARTESIAN_POINT('Origin',(3.5,-5.15,-16.545)) ;
#164514=CARTESIAN_POINT('Origin',(3.5,-5.15,-16.545)) ;
#164515=CARTESIAN_POINT('Origin',(2.7,-5.35,-13.835)) ;
#164516=CARTESIAN_POINT('Origin',(2.7,-5.35,-16.545)) ;
#164517=CARTESIAN_POINT('Origin',(3.6,-5.15,-16.545)) ;
#164518=CARTESIAN_POINT('Origin',(2.7,-5.15,-16.545)) ;
#164519=CARTESIAN_POINT('Origin',(3.6,1.9,-16.745)) ;
#164520=CARTESIAN_POINT('Origin',(3.5,1.9,-16.745)) ;
#164521=CARTESIAN_POINT('Origin',(2.7,1.9,-16.745)) ;
#164522=CARTESIAN_POINT('Origin',(2.7,1.9,-16.645)) ;
#164523=CARTESIAN_POINT('Origin',(2.7,1.9,-17.545)) ;
#164524=CARTESIAN_POINT('Origin',(2.7,1.9,-16.745)) ;
#164525=CARTESIAN_POINT('Origin',(2.7,-5.15,-16.545)) ;
#164526=CARTESIAN_POINT('Origin',(2.7,-5.15,-16.745)) ;
#164527=CARTESIAN_POINT('Origin',(2.7,1.9,-16.745)) ;
#164528=CARTESIAN_POINT('Origin',(2.7,1.9,-16.745)) ;
#164529=CARTESIAN_POINT('Origin',(2.7,-5.25,-16.745)) ;
#164530=CARTESIAN_POINT('Ctrl Pts',(-3.8,-6.55,-14.14)) ;
#164531=CARTESIAN_POINT('Ctrl Pts',(-3.8,-6.55,-14.14)) ;
#164532=CARTESIAN_POINT('Ctrl Pts',(-3.8,-6.55,-14.14)) ;
#164533=CARTESIAN_POINT('Ctrl Pts',(-3.8262534328264,-6.55,-14.1925068656527)) ;
#164534=CARTESIAN_POINT('Ctrl Pts',(-3.83954133268484,-6.55,-14.1795413326849)) ;
#164535=CARTESIAN_POINT('Ctrl Pts',(-3.85250686565269,-6.55,-14.1662534328264)) ;
#164536=CARTESIAN_POINT('Ctrl Pts',(-3.85219871729854,-6.53922263893877,
-14.2443974345971)) ;
#164537=CARTESIAN_POINT('Ctrl Pts',(-3.87914655110982,-6.52362528614073,
-14.2191465511098)) ;
#164538=CARTESIAN_POINT('Ctrl Pts',(-3.90439743459708,-6.53922263893877,
-14.1921987172985)) ;
#164539=CARTESIAN_POINT('Ctrl Pts',(-3.87996665852871,-6.5114546977086,
-14.2999333170574)) ;
#164540=CARTESIAN_POINT('Ctrl Pts',(-3.9028838031416,-6.48208554016475,
-14.2428838031416)) ;
#164541=CARTESIAN_POINT('Ctrl Pts',(-3.95993331705742,-6.5114546977086,
-14.2199666585287)) ;
#164542=CARTESIAN_POINT('Ctrl Pts',(-3.88737865704135,-6.5003618540841,
-14.3147573140827)) ;
#164543=CARTESIAN_POINT('Ctrl Pts',(-3.90501307588294,-6.46792722356047,
-14.2450130758829)) ;
#164544=CARTESIAN_POINT('Ctrl Pts',(-3.9747573140827,-6.5003618540841,-14.2273786570414)) ;
#164545=CARTESIAN_POINT('Ctrl Pts',(-3.8973972494609,-6.47617483238892,
-14.3347944989218)) ;
#164546=CARTESIAN_POINT('Ctrl Pts',(-3.90329674356409,-6.4509405986842,
-14.2432967435641)) ;
#164547=CARTESIAN_POINT('Ctrl Pts',(-3.99479449892181,-6.47617483238892,
-14.2373972494609)) ;
#164548=CARTESIAN_POINT('Ctrl Pts',(-3.9,-6.46309229646327,-14.3399999991817)) ;
#164549=CARTESIAN_POINT('Ctrl Pts',(-3.90000730393163,-6.44945650151458,
-14.2400073039128)) ;
#164550=CARTESIAN_POINT('Ctrl Pts',(-3.99999999918173,-6.46309229646328,
-14.24)) ;
#164551=CARTESIAN_POINT('Ctrl Pts',(-3.9,-6.45,-14.34)) ;
#164552=CARTESIAN_POINT('Ctrl Pts',(-3.9,-6.45,-14.24)) ;
#164553=CARTESIAN_POINT('Ctrl Pts',(-4.,-6.45,-14.24)) ;
#164554=CARTESIAN_POINT('Origin',(-4.,-6.45,-14.34)) ;
#164555=CARTESIAN_POINT('Origin',(-4.,-6.4,-14.34)) ;
#164556=CARTESIAN_POINT('Origin',(-4.,-6.35,-14.34)) ;
#164557=CARTESIAN_POINT('Ctrl Pts',(-5.,-6.55,-14.14)) ;
#164558=CARTESIAN_POINT('Ctrl Pts',(-5.,-6.55,-14.14)) ;
#164559=CARTESIAN_POINT('Ctrl Pts',(-5.,-6.55,-14.14)) ;
#164560=CARTESIAN_POINT('Ctrl Pts',(-4.94749313434721,-6.55,-14.1662534328262)) ;
#164561=CARTESIAN_POINT('Ctrl Pts',(-4.96045866731609,-6.55,-14.1795413326839)) ;
#164562=CARTESIAN_POINT('Ctrl Pts',(-4.97374656717352,-6.55,-14.1925068656527)) ;
#164563=CARTESIAN_POINT('Ctrl Pts',(-4.89560256540291,-6.53922263893879,
-14.1921987172985)) ;
#164564=CARTESIAN_POINT('Ctrl Pts',(-4.9208534488902,-6.52362528614071,
-14.2191465511098)) ;
#164565=CARTESIAN_POINT('Ctrl Pts',(-4.94780128270146,-6.53922263893877,
-14.244397434597)) ;
#164566=CARTESIAN_POINT('Ctrl Pts',(-4.84006668294258,-6.51145469770858,
-14.2199666585287)) ;
#164567=CARTESIAN_POINT('Ctrl Pts',(-4.89711619685838,-6.48208554016476,
-14.2428838031416)) ;
#164568=CARTESIAN_POINT('Ctrl Pts',(-4.92003334147129,-6.5114546977086,
-14.2999333170575)) ;
#164569=CARTESIAN_POINT('Ctrl Pts',(-4.82524268591729,-6.5003618540841,
-14.2273786570414)) ;
#164570=CARTESIAN_POINT('Ctrl Pts',(-4.89498692411705,-6.46792722356049,
-14.2450130758829)) ;
#164571=CARTESIAN_POINT('Ctrl Pts',(-4.91262134295865,-6.5003618540841,
-14.3147573140827)) ;
#164572=CARTESIAN_POINT('Ctrl Pts',(-4.80520550107819,-6.47617483238892,
-14.2373972494609)) ;
#164573=CARTESIAN_POINT('Ctrl Pts',(-4.89670325643591,-6.45094059868419,
-14.2432967435641)) ;
#164574=CARTESIAN_POINT('Ctrl Pts',(-4.90260275053909,-6.47617483238892,
-14.3347944989218)) ;
#164575=CARTESIAN_POINT('Ctrl Pts',(-4.80000000081823,-6.46309229646328,
-14.24)) ;
#164576=CARTESIAN_POINT('Ctrl Pts',(-4.89999269604942,-6.44945650152248,
-14.2400073039129)) ;
#164577=CARTESIAN_POINT('Ctrl Pts',(-4.9,-6.46309229646328,-14.3399999991817)) ;
#164578=CARTESIAN_POINT('Ctrl Pts',(-4.8,-6.45,-14.24)) ;
#164579=CARTESIAN_POINT('Ctrl Pts',(-4.9,-6.45,-14.24)) ;
#164580=CARTESIAN_POINT('Ctrl Pts',(-4.9,-6.45,-14.34)) ;
#164581=CARTESIAN_POINT('Origin',(-4.8,-6.45,-14.34)) ;
#164582=CARTESIAN_POINT('Origin',(-4.,-6.35,-14.34)) ;
#164583=CARTESIAN_POINT('Origin',(-4.,-6.35,-14.34)) ;
#164584=CARTESIAN_POINT('Origin',(-4.,-6.35,-14.34)) ;
#164585=CARTESIAN_POINT('Ctrl Pts',(-3.8,-6.55,-16.34)) ;
#164586=CARTESIAN_POINT('Ctrl Pts',(-3.8,-6.55,-16.34)) ;
#164587=CARTESIAN_POINT('Ctrl Pts',(-3.8,-6.55,-16.34)) ;
#164588=CARTESIAN_POINT('Ctrl Pts',(-3.85250686565272,-6.55,-16.3137465671736)) ;
#164589=CARTESIAN_POINT('Ctrl Pts',(-3.83954133268385,-6.55,-16.3004586673161)) ;
#164590=CARTESIAN_POINT('Ctrl Pts',(-3.82625343282628,-6.55,-16.2874931343472)) ;
#164591=CARTESIAN_POINT('Ctrl Pts',(-3.90439743459706,-6.53922263893874,
-16.2878012827014)) ;
#164592=CARTESIAN_POINT('Ctrl Pts',(-3.87914655110978,-6.52362528614071,
-16.2608534488901)) ;
#164593=CARTESIAN_POINT('Ctrl Pts',(-3.85219871729855,-6.53922263893876,
-16.2356025654029)) ;
#164594=CARTESIAN_POINT('Ctrl Pts',(-3.95993331705743,-6.51145469770861,
-16.2600333414713)) ;
#164595=CARTESIAN_POINT('Ctrl Pts',(-3.90288380314162,-6.48208554016476,
-16.2371161968584)) ;
#164596=CARTESIAN_POINT('Ctrl Pts',(-3.8799666585287,-6.5114546977086,-16.1800666829426)) ;
#164597=CARTESIAN_POINT('Ctrl Pts',(-3.97475731408271,-6.5003618540841,
-16.2526213429587)) ;
#164598=CARTESIAN_POINT('Ctrl Pts',(-3.90501307588293,-6.46792722356047,
-16.2349869241171)) ;
#164599=CARTESIAN_POINT('Ctrl Pts',(-3.88737865704135,-6.5003618540841,
-16.1652426859173)) ;
#164600=CARTESIAN_POINT('Ctrl Pts',(-3.9947944989218,-6.47617483238891,
-16.2426027505391)) ;
#164601=CARTESIAN_POINT('Ctrl Pts',(-3.9032967435641,-6.4509405986842,-16.2367032564358)) ;
#164602=CARTESIAN_POINT('Ctrl Pts',(-3.89739724946091,-6.47617483238892,
-16.1452055010782)) ;
#164603=CARTESIAN_POINT('Ctrl Pts',(-3.99999999918176,-6.46309229646328,
-16.24)) ;
#164604=CARTESIAN_POINT('Ctrl Pts',(-3.90000730395532,-6.44945650152054,
-16.2399926960966)) ;
#164605=CARTESIAN_POINT('Ctrl Pts',(-3.9,-6.46309229646328,-16.1400000008182)) ;
#164606=CARTESIAN_POINT('Ctrl Pts',(-4.,-6.45,-16.24)) ;
#164607=CARTESIAN_POINT('Ctrl Pts',(-3.9,-6.45,-16.24)) ;
#164608=CARTESIAN_POINT('Ctrl Pts',(-3.9,-6.45,-16.14)) ;
#164609=CARTESIAN_POINT('Origin',(-4.,-6.45,-16.14)) ;
#164610=CARTESIAN_POINT('Origin',(-4.8,-6.4,-14.34)) ;
#164611=CARTESIAN_POINT('Origin',(-4.8,-6.35,-14.34)) ;
#164612=CARTESIAN_POINT('Origin',(1.9515639104739E-16,-6.35,-14.34)) ;
#164613=CARTESIAN_POINT('Origin',(-4.8,-6.35,-14.34)) ;
#164614=CARTESIAN_POINT('Origin',(-4.,-6.35,-15.24)) ;
#164615=CARTESIAN_POINT('Origin',(-4.,-6.35,-16.14)) ;
#164616=CARTESIAN_POINT('Origin',(-4.,-6.4,-16.14)) ;
#164617=CARTESIAN_POINT('Origin',(-4.,-6.35,-16.14)) ;
#164618=CARTESIAN_POINT('Origin',(-4.8,-6.35,-14.34)) ;
#164619=CARTESIAN_POINT('Origin',(-4.8,-6.35,-14.34)) ;
#164620=CARTESIAN_POINT('Origin',(-4.,-6.35,-16.14)) ;
#164621=CARTESIAN_POINT('Origin',(-4.,-6.35,-16.14)) ;
#164622=CARTESIAN_POINT('Origin',(-4.8,-6.35,-15.24)) ;
#164623=CARTESIAN_POINT('Origin',(-4.8,-6.35,-16.14)) ;
#164624=CARTESIAN_POINT('Origin',(1.95156391047391E-16,-6.35,-16.14)) ;
#164625=CARTESIAN_POINT('Origin',(-4.8,-6.35,-16.14)) ;
#164626=CARTESIAN_POINT('Origin',(-4.8,-6.35,-16.14)) ;
#164627=CARTESIAN_POINT('Origin',(-4.8,-6.35,-16.14)) ;
#164628=CARTESIAN_POINT('Origin',(-4.8,-6.4,-16.14)) ;
#164629=CARTESIAN_POINT('Origin',(-4.8,-6.45,-16.14)) ;
#164630=CARTESIAN_POINT('Ctrl Pts',(-5.,-6.55,-16.34)) ;
#164631=CARTESIAN_POINT('Ctrl Pts',(-5.,-6.55,-16.34)) ;
#164632=CARTESIAN_POINT('Ctrl Pts',(-5.,-6.55,-16.34)) ;
#164633=CARTESIAN_POINT('Ctrl Pts',(-4.97374656717361,-6.55,-16.2874931343473)) ;
#164634=CARTESIAN_POINT('Ctrl Pts',(-4.96045866731621,-6.55,-16.300458667316)) ;
#164635=CARTESIAN_POINT('Ctrl Pts',(-4.94749313434733,-6.55,-16.3137465671736)) ;
#164636=CARTESIAN_POINT('Ctrl Pts',(-4.94780128270146,-6.53922263893877,
-16.2356025654029)) ;
#164637=CARTESIAN_POINT('Ctrl Pts',(-4.92085344889017,-6.52362528614074,
-16.2608534488901)) ;
#164638=CARTESIAN_POINT('Ctrl Pts',(-4.89560256540291,-6.53922263893874,
-16.2878012827014)) ;
#164639=CARTESIAN_POINT('Ctrl Pts',(-4.92003334147129,-6.5114546977086,
-16.1800666829426)) ;
#164640=CARTESIAN_POINT('Ctrl Pts',(-4.8971161968584,-6.48208554016475,
-16.2371161968584)) ;
#164641=CARTESIAN_POINT('Ctrl Pts',(-4.84006668294258,-6.51145469770861,
-16.2600333414713)) ;
#164642=CARTESIAN_POINT('Ctrl Pts',(-4.91262134295865,-6.5003618540841,
-16.1652426859173)) ;
#164643=CARTESIAN_POINT('Ctrl Pts',(-4.89498692411706,-6.46792722356047,
-16.2349869241171)) ;
#164644=CARTESIAN_POINT('Ctrl Pts',(-4.82524268591729,-6.5003618540841,
-16.2526213429587)) ;
#164645=CARTESIAN_POINT('Ctrl Pts',(-4.90260275053909,-6.47617483238892,
-16.1452055010782)) ;
#164646=CARTESIAN_POINT('Ctrl Pts',(-4.8967032564359,-6.4509405986842,-16.2367032564358)) ;
#164647=CARTESIAN_POINT('Ctrl Pts',(-4.80520550107819,-6.47617483238891,
-16.2426027505391)) ;
#164648=CARTESIAN_POINT('Ctrl Pts',(-4.9,-6.46309229646328,-16.1400000008182)) ;
#164649=CARTESIAN_POINT('Ctrl Pts',(-4.89999269603999,-6.44945650152247,
-16.2399926960966)) ;
#164650=CARTESIAN_POINT('Ctrl Pts',(-4.80000000081823,-6.46309229646328,
-16.24)) ;
#164651=CARTESIAN_POINT('Ctrl Pts',(-4.9,-6.45,-16.14)) ;
#164652=CARTESIAN_POINT('Ctrl Pts',(-4.9,-6.45,-16.24)) ;
#164653=CARTESIAN_POINT('Ctrl Pts',(-4.8,-6.45,-16.24)) ;
#164654=CARTESIAN_POINT('Ctrl Pts',(-5.8242667673935,-5.43399303700614,
-13.6370109659688)) ;
#164655=CARTESIAN_POINT('Ctrl Pts',(-5.80266988778317,-5.52572360682923,
-13.6423540173506)) ;
#164656=CARTESIAN_POINT('Ctrl Pts',(-5.82426676352013,-5.53106667371341,
-13.7340845871826)) ;
#164657=CARTESIAN_POINT('Ctrl Pts',(-5.83498671931115,-5.4393535119191,
-13.6343294581962)) ;
#164658=CARTESIAN_POINT('Ctrl Pts',(-5.8059526312227,-5.52411753147693,
-13.6439600935404)) ;
#164659=CARTESIAN_POINT('Ctrl Pts',(-5.83498671397625,-5.53374818067468,
-13.7287241131462)) ;
#164660=CARTESIAN_POINT('Ctrl Pts',(-5.84526105845714,-5.44830326289495,
-13.6298528401961)) ;
#164661=CARTESIAN_POINT('Ctrl Pts',(-5.81370932746142,-5.52260132030844,
-13.6454763059991)) ;
#164662=CARTESIAN_POINT('Ctrl Pts',(-5.84526105243717,-5.53822479746337,
-13.7197743635697)) ;
#164663=CARTESIAN_POINT('Ctrl Pts',(-5.86378685403697,-5.47240020430403,
-13.6178032513087)) ;
#164664=CARTESIAN_POINT('Ctrl Pts',(-5.83531854275289,-5.52733067404475,
-13.6407469551147)) ;
#164665=CARTESIAN_POINT('Ctrl Pts',(-5.86378684816457,-5.55027438459895,
-13.6956774250055)) ;
#164666=CARTESIAN_POINT('Ctrl Pts',(-5.87203852631577,-5.48754495134736,
-13.6102315528944)) ;
#164667=CARTESIAN_POINT('Ctrl Pts',(-5.84834787930687,-5.53310199490446,
-13.6349756357761)) ;
#164668=CARTESIAN_POINT('Ctrl Pts',(-5.87203852123036,-5.55784608243453,
-13.6805326795138)) ;
#164669=CARTESIAN_POINT('Ctrl Pts',(-5.89242747304797,-5.53981202333455,
-13.5841056511376)) ;
#164670=CARTESIAN_POINT('Ctrl Pts',(-5.88223383300419,-5.56084219179272,
-13.6072354431742)) ;
#164671=CARTESIAN_POINT('Ctrl Pts',(-5.89242747063499,-5.5839719840277,
-13.6282656123278)) ;
#164672=CARTESIAN_POINT('Ctrl Pts',(-5.9,-5.58381083947298,-13.562119400143)) ;
#164673=CARTESIAN_POINT('Ctrl Pts',(-5.9,-5.5948530450262,-13.5732245928869)) ;
#164674=CARTESIAN_POINT('Ctrl Pts',(-5.9,-5.60595823775494,-13.5842667984405)) ;
#164675=CARTESIAN_POINT('Ctrl Pts',(-5.9,-5.62807764064044,-13.54)) ;
#164676=CARTESIAN_POINT('Ctrl Pts',(-5.9,-5.62807764064044,-13.54)) ;
#164677=CARTESIAN_POINT('Ctrl Pts',(-5.9,-5.62807764064044,-13.54)) ;
#164678=CARTESIAN_POINT('Origin',(-5.84850712500726,-5.43404914061138,-13.7340285000291)) ;
#164679=CARTESIAN_POINT('Ctrl Pts',(-5.82425356250363,-5.53106339062591,
-13.7340285000291)) ;
#164680=CARTESIAN_POINT('Ctrl Pts',(-5.80269484027818,-5.52567371006955,
-13.6424039305709)) ;
#164681=CARTESIAN_POINT('Ctrl Pts',(-5.82425356250363,-5.43404914061138,
-13.6370142500145)) ;
#164682=CARTESIAN_POINT('Ctrl Pts',(-5.80840777707097,-5.52710194426774,
-13.7379899459044)) ;
#164683=CARTESIAN_POINT('Ctrl Pts',(-5.79341417645231,-5.52335354411303,
-13.6428358498184)) ;
#164684=CARTESIAN_POINT('Ctrl Pts',(-5.81633079157288,-5.4300877551176,
-13.6389949427472)) ;
#164685=CARTESIAN_POINT('Ctrl Pts',(-5.79207992677989,-5.52301998169497,
-13.739999999534)) ;
#164686=CARTESIAN_POINT('Ctrl Pts',(-5.78430903206645,-5.52107725801655,
-13.6419613954328)) ;
#164687=CARTESIAN_POINT('Ctrl Pts',(-5.80816665318298,-5.42600568595105,
-13.64)) ;
#164688=CARTESIAN_POINT('Ctrl Pts',(-5.77574643749636,-5.51893660937409,
-13.74)) ;
#164689=CARTESIAN_POINT('Ctrl Pts',(-5.77574643749636,-5.51893660937409,
-13.64)) ;
#164690=CARTESIAN_POINT('Ctrl Pts',(-5.8,-5.42192235935956,-13.64)) ;
#164691=CARTESIAN_POINT('Origin',(-5.8,-5.42192235935956,-13.74)) ;
#164692=CARTESIAN_POINT('Origin',(-5.8066065036801,-5.42357398527959,-13.74)) ;
#164693=CARTESIAN_POINT('Origin',(-5.17275707706436,-5.26511162862565,-13.74)) ;
#164694=CARTESIAN_POINT('Origin',(-5.15068655017073,-5.25959399690224,-13.7505938529089)) ;
#164695=CARTESIAN_POINT('Origin',(-5.17275707706436,-5.26511162862565,-13.74)) ;
#164696=CARTESIAN_POINT('Origin',(-5.17275707706436,-5.26511162862565,-13.74)) ;
#164697=CARTESIAN_POINT('Origin',(-5.17275707706436,-5.26511162862565,-13.74)) ;
#164698=CARTESIAN_POINT('Origin',(-5.17275707706436,-5.05,-13.74)) ;
#164699=CARTESIAN_POINT('Origin',(-5.17275707706436,-1.91866427917294,-13.74)) ;
#164700=CARTESIAN_POINT('Origin',(-3.78014014831103,-3.31128120792626,-14.4084561258016)) ;
#164701=CARTESIAN_POINT('Origin',(-5.17275707706437,-1.91866427917293,-13.74)) ;
#164702=CARTESIAN_POINT('Origin',(-5.17275707706436,-1.91866427917293,-13.74)) ;
#164703=CARTESIAN_POINT('Origin',(-5.17275707706436,-1.91866427917294,-13.74)) ;
#164704=CARTESIAN_POINT('Origin',(-3.97071067811865,-3.12071067811865,-13.74)) ;
#164705=CARTESIAN_POINT('Origin',(-5.8,-1.2914213562373,-13.74)) ;
#164706=CARTESIAN_POINT('Ctrl Pts',(-5.87071067811865,-1.14999999999999,
-13.6107106781187)) ;
#164707=CARTESIAN_POINT('Ctrl Pts',(-5.8471404520791,-1.10285954792089,
-13.6342809041582)) ;
#164708=CARTESIAN_POINT('Ctrl Pts',(-5.87071067811865,-1.07928932188134,
-13.6814213562373)) ;
#164709=CARTESIAN_POINT('Ctrl Pts',(-5.85217562795664,-1.18707010095462,
-13.6292457282807)) ;
#164710=CARTESIAN_POINT('Ctrl Pts',(-5.81261165662076,-1.13738834337924,
-13.6558614719497)) ;
#164711=CARTESIAN_POINT('Ctrl Pts',(-5.83353949671041,-1.11646050328959,
-13.718592536381)) ;
#164712=CARTESIAN_POINT('Ctrl Pts',(-5.82627077431947,-1.23887980759831,
-13.64)) ;
#164713=CARTESIAN_POINT('Ctrl Pts',(-5.76566787907943,-1.18433212092057,
-13.6571489437128)) ;
#164714=CARTESIAN_POINT('Ctrl Pts',(-5.78190678732235,-1.16809321267764,
-13.7399999994186)) ;
#164715=CARTESIAN_POINT('Ctrl Pts',(-5.8,-1.2914213562373,-13.64)) ;
#164716=CARTESIAN_POINT('Ctrl Pts',(-5.72928932188134,-1.22071067811865,
-13.64)) ;
#164717=CARTESIAN_POINT('Ctrl Pts',(-5.72928932188134,-1.22071067811865,
-13.74)) ;
#164718=CARTESIAN_POINT('Origin',(-5.94142135623731,-1.14999999999999,-13.6814213562373)) ;
#164719=CARTESIAN_POINT('Ctrl Pts',(-5.9,-1.00857864376269,-13.54)) ;
#164720=CARTESIAN_POINT('Ctrl Pts',(-5.9,-1.00857864376269,-13.54)) ;
#164721=CARTESIAN_POINT('Ctrl Pts',(-5.9,-1.00857864376269,-13.54)) ;
#164722=CARTESIAN_POINT('Ctrl Pts',(-5.9,-1.06112019240168,-13.5662707743196)) ;
#164723=CARTESIAN_POINT('Ctrl Pts',(-5.9,-1.04860238143836,-13.5800237376757)) ;
#164724=CARTESIAN_POINT('Ctrl Pts',(-5.9,-1.03484941808221,-13.592541548639)) ;
#164725=CARTESIAN_POINT('Ctrl Pts',(-5.88924572828063,-1.11292989904529,
-13.5921756279567)) ;
#164726=CARTESIAN_POINT('Ctrl Pts',(-5.87451700624548,-1.08721613124892,
-13.6186374874863)) ;
#164727=CARTESIAN_POINT('Ctrl Pts',(-5.88924572828066,-1.06075427171933,
-13.6443512552827)) ;
#164728=CARTESIAN_POINT('Ctrl Pts',(-5.87071067811865,-1.14999999999999,
-13.6107106781187)) ;
#164729=CARTESIAN_POINT('Ctrl Pts',(-5.8471404520791,-1.10285954792089,
-13.6342809041582)) ;
#164730=CARTESIAN_POINT('Ctrl Pts',(-5.87071067811865,-1.07928932188134,
-13.6814213562373)) ;
#164731=CARTESIAN_POINT('Ctrl Pts',(-5.87071067811866,-1.14999999999999,
-16.8692893218813)) ;
#164732=CARTESIAN_POINT('Ctrl Pts',(-5.84714045207911,-1.10285954792089,
-16.8457190958418)) ;
#164733=CARTESIAN_POINT('Ctrl Pts',(-5.87071067811866,-1.07928932188134,
-16.7985786437627)) ;
#164734=CARTESIAN_POINT('Ctrl Pts',(-5.88924572828071,-1.11292989904541,
-16.8878243720434)) ;
#164735=CARTESIAN_POINT('Ctrl Pts',(-5.87451700627498,-1.08721613123208,
-16.8613625125308)) ;
#164736=CARTESIAN_POINT('Ctrl Pts',(-5.88924572828061,-1.06075427171938,
-16.8356487447174)) ;
#164737=CARTESIAN_POINT('Ctrl Pts',(-5.9,-1.06112019240159,-16.9137292256804)) ;
#164738=CARTESIAN_POINT('Ctrl Pts',(-5.9,-1.04860238145164,-16.8999762623108)) ;
#164739=CARTESIAN_POINT('Ctrl Pts',(-5.9,-1.03484941808214,-16.887458451361)) ;
#164740=CARTESIAN_POINT('Ctrl Pts',(-5.9,-1.00857864376269,-16.94)) ;
#164741=CARTESIAN_POINT('Ctrl Pts',(-5.9,-1.00857864376269,-16.94)) ;
#164742=CARTESIAN_POINT('Ctrl Pts',(-5.9,-1.00857864376269,-16.94)) ;
#164743=CARTESIAN_POINT('Origin',(-5.94142135623734,-1.14999999999996,-16.7985786437627)) ;
#164744=CARTESIAN_POINT('Ctrl Pts',(-5.8,-1.2914213562373,-16.84)) ;
#164745=CARTESIAN_POINT('Ctrl Pts',(-5.72928932188134,-1.22071067811865,
-16.84)) ;
#164746=CARTESIAN_POINT('Ctrl Pts',(-5.72928932188134,-1.22071067811865,
-16.74)) ;
#164747=CARTESIAN_POINT('Ctrl Pts',(-5.82627077431952,-1.23887980759821,
-16.84)) ;
#164748=CARTESIAN_POINT('Ctrl Pts',(-5.76566787907979,-1.18433212092022,
-16.8228510562871)) ;
#164749=CARTESIAN_POINT('Ctrl Pts',(-5.78190678732242,-1.16809321267757,
-16.7400000005814)) ;
#164750=CARTESIAN_POINT('Ctrl Pts',(-5.85217562795678,-1.18707010095484,
-16.8507542717195)) ;
#164751=CARTESIAN_POINT('Ctrl Pts',(-5.81261165662032,-1.13738834337968,
-16.8241385280508)) ;
#164752=CARTESIAN_POINT('Ctrl Pts',(-5.83353949671032,-1.11646050328967,
-16.7614074636191)) ;
#164753=CARTESIAN_POINT('Ctrl Pts',(-5.87071067811866,-1.14999999999999,
-16.8692893218813)) ;
#164754=CARTESIAN_POINT('Ctrl Pts',(-5.84714045207911,-1.10285954792088,
-16.8457190958418)) ;
#164755=CARTESIAN_POINT('Ctrl Pts',(-5.87071067811866,-1.07928932188133,
-16.7985786437627)) ;
#164756=CARTESIAN_POINT('Origin',(-5.8,-1.29142135623731,-16.74)) ;
#164757=CARTESIAN_POINT('Origin',(-3.59571067811865,-3.49571067811865,-16.74)) ;
#164758=CARTESIAN_POINT('Origin',(-5.17275707706437,-1.91866427917293,-16.74)) ;
#164759=CARTESIAN_POINT('Origin',(-3.09057773798104,-4.00084361825625,-15.74055391724)) ;
#164760=CARTESIAN_POINT('Origin',(-5.17275707706436,-1.91866427917293,-16.74)) ;
#164761=CARTESIAN_POINT('Origin',(-5.17275707706436,-1.91866427917293,-16.74)) ;
#164762=CARTESIAN_POINT('Origin',(-5.17275707706436,-1.91866427917293,-16.74)) ;
#164763=CARTESIAN_POINT('Origin',(-5.17275707706436,-5.05,-16.74)) ;
#164764=CARTESIAN_POINT('Origin',(-5.17275707706436,-5.26511162862565,-16.74)) ;
#164765=CARTESIAN_POINT('Origin',(-3.96111272388873,-4.96220054033175,-16.1584107104757)) ;
#164766=CARTESIAN_POINT('Origin',(-5.17275707706436,-5.26511162862565,-16.74)) ;
#164767=CARTESIAN_POINT('Origin',(-5.17275707706436,-5.26511162862565,-16.74)) ;
#164768=CARTESIAN_POINT('Origin',(-5.17275707706436,-5.26511162862565,-16.74)) ;
#164769=CARTESIAN_POINT('Origin',(-5.10072415073893,-5.24710339704429,-16.74)) ;
#164770=CARTESIAN_POINT('Origin',(-5.8,-5.42192235935956,-16.74)) ;
#164771=CARTESIAN_POINT('Ctrl Pts',(-5.77574643749636,-5.51893660937409,
-16.74)) ;
#164772=CARTESIAN_POINT('Ctrl Pts',(-5.77574643749636,-5.51893660937409,
-16.84)) ;
#164773=CARTESIAN_POINT('Ctrl Pts',(-5.8,-5.42192235935956,-16.84)) ;
#164774=CARTESIAN_POINT('Ctrl Pts',(-5.7920799267799,-5.52301998169498,
-16.740000000466)) ;
#164775=CARTESIAN_POINT('Ctrl Pts',(-5.78430903206643,-5.5210772580166,
-16.8380386045671)) ;
#164776=CARTESIAN_POINT('Ctrl Pts',(-5.808166653183,-5.42600568595105,-16.84)) ;
#164777=CARTESIAN_POINT('Ctrl Pts',(-5.80840777707094,-5.52710194426774,
-16.7420100540957)) ;
#164778=CARTESIAN_POINT('Ctrl Pts',(-5.7934141764523,-5.52335354411309,
-16.8371641501816)) ;
#164779=CARTESIAN_POINT('Ctrl Pts',(-5.81633079157288,-5.43008775511759,
-16.8410050572528)) ;
#164780=CARTESIAN_POINT('Ctrl Pts',(-5.82425356250363,-5.53106339062591,
-16.7459714999709)) ;
#164781=CARTESIAN_POINT('Ctrl Pts',(-5.80269484027818,-5.52567371006955,
-16.8375960694291)) ;
#164782=CARTESIAN_POINT('Ctrl Pts',(-5.82425356250363,-5.43404914061138,
-16.8429857499855)) ;
#164783=CARTESIAN_POINT('Origin',(-5.84850712500726,-5.43404914061138,-16.7459714999709)) ;
#164784=CARTESIAN_POINT('Ctrl Pts',(-5.82426676739356,-5.5310666746717,
-16.7459153963654)) ;
#164785=CARTESIAN_POINT('Ctrl Pts',(-5.80266988778307,-5.52572362329014,
-16.8376459661889)) ;
#164786=CARTESIAN_POINT('Ctrl Pts',(-5.82426676352019,-5.43399305345765,
-16.842989033073)) ;
#164787=CARTESIAN_POINT('Ctrl Pts',(-5.83498671931125,-5.53374818244431,
-16.7512758712784)) ;
#164788=CARTESIAN_POINT('Ctrl Pts',(-5.80595263122257,-5.52411754710035,
-16.8360398908367)) ;
#164789=CARTESIAN_POINT('Ctrl Pts',(-5.8349867139763,-5.43935352749406,
-16.8456705400343)) ;
#164790=CARTESIAN_POINT('Ctrl Pts',(-5.84526105845723,-5.53822480044432,
-16.7602256222542)) ;
#164791=CARTESIAN_POINT('Ctrl Pts',(-5.81370932746128,-5.52260133464156,
-16.8345236796681)) ;
#164792=CARTESIAN_POINT('Ctrl Pts',(-5.84526105243723,-5.44830327707059,
-16.850147156823)) ;
#164793=CARTESIAN_POINT('Ctrl Pts',(-5.86378685403707,-5.55027438933184,
-16.7843225636634)) ;
#164794=CARTESIAN_POINT('Ctrl Pts',(-5.83531854275277,-5.52733068552589,
-16.8392530334044)) ;
#164795=CARTESIAN_POINT('Ctrl Pts',(-5.86378684816465,-5.4724002156349,
-16.8621967439586)) ;
#164796=CARTESIAN_POINT('Ctrl Pts',(-5.87203852631585,-5.55784608774615,
-16.7994673107067)) ;
#164797=CARTESIAN_POINT('Ctrl Pts',(-5.84834787930678,-5.53310200486445,
-16.845024354264)) ;
#164798=CARTESIAN_POINT('Ctrl Pts',(-5.87203852123043,-5.48754496112646,
-16.8697684417941)) ;
#164799=CARTESIAN_POINT('Ctrl Pts',(-5.892427473048,-5.58397198950291,-16.851734382694)) ;
#164800=CARTESIAN_POINT('Ctrl Pts',(-5.88223383300415,-5.56084219746622,
-16.8727645511521)) ;
#164801=CARTESIAN_POINT('Ctrl Pts',(-5.89242747063501,-5.5398120283126,
-16.8958943433873)) ;
#164802=CARTESIAN_POINT('Ctrl Pts',(-5.9,-5.60595824049753,-16.8957331988325)) ;
#164803=CARTESIAN_POINT('Ctrl Pts',(-5.9,-5.59485304775418,-16.9067754043861)) ;
#164804=CARTESIAN_POINT('Ctrl Pts',(-5.9,-5.58381084219989,-16.9178805971146)) ;
#164805=CARTESIAN_POINT('Ctrl Pts',(-5.9,-5.62807764064044,-16.94)) ;
#164806=CARTESIAN_POINT('Ctrl Pts',(-5.9,-5.62807764064044,-16.94)) ;
#164807=CARTESIAN_POINT('Ctrl Pts',(-5.9,-5.62807764064044,-16.94)) ;
#164808=CARTESIAN_POINT('Origin',(7.8,2.1,-15.64)) ;
#164809=CARTESIAN_POINT('Origin',(7.8,2.1,-15.84)) ;
#164810=CARTESIAN_POINT('Origin',(7.6,2.1,-15.64)) ;
#164811=CARTESIAN_POINT('Origin',(7.6,2.1,-15.64)) ;
#164812=CARTESIAN_POINT('Origin',(7.6,2.1,-14.84)) ;
#164813=CARTESIAN_POINT('Origin',(7.8,2.1,-15.84)) ;
#164814=CARTESIAN_POINT('Origin',(9.6,2.1,-15.84)) ;
#164815=CARTESIAN_POINT('Origin',(7.8,2.1,-14.84)) ;
#164816=CARTESIAN_POINT('Origin',(7.8,2.1,-14.64)) ;
#164817=CARTESIAN_POINT('Origin',(9.6,2.1,-15.64)) ;
#164818=CARTESIAN_POINT('Origin',(9.8,2.1,-15.64)) ;
#164819=CARTESIAN_POINT('Origin',(7.8,2.1,-14.64)) ;
#164820=CARTESIAN_POINT('Origin',(9.6,2.1,-14.64)) ;
#164821=CARTESIAN_POINT('Origin',(9.8,2.1,-15.64)) ;
#164822=CARTESIAN_POINT('Origin',(9.8,2.1,-14.84)) ;
#164823=CARTESIAN_POINT('Origin',(9.6,2.1,-14.84)) ;
#164824=CARTESIAN_POINT('Origin',(-4.15,-6.25,-14.49)) ;
#164825=CARTESIAN_POINT('Origin',(-4.15,-6.3,-14.49)) ;
#164826=CARTESIAN_POINT('Origin',(-4.15,-6.3,-15.24)) ;
#164827=CARTESIAN_POINT('Origin',(-4.15,-6.3,-15.99)) ;
#164828=CARTESIAN_POINT('Origin',(-4.15,-6.3,-14.49)) ;
#164829=CARTESIAN_POINT('Origin',(-4.15,-6.25,-15.99)) ;
#164830=CARTESIAN_POINT('Origin',(-4.15,-6.3,-15.99)) ;
#164831=CARTESIAN_POINT('Origin',(-4.15,-6.3,-14.49)) ;
#164832=CARTESIAN_POINT('Origin',(-4.15,-6.3,-14.49)) ;
#164833=CARTESIAN_POINT('Origin',(-4.15,-6.3,-15.99)) ;
#164834=CARTESIAN_POINT('Origin',(-4.15,-6.3,-15.99)) ;
#164835=CARTESIAN_POINT('Origin',(-4.65,-6.25,-14.49)) ;
#164836=CARTESIAN_POINT('Origin',(-4.65,-6.3,-14.49)) ;
#164837=CARTESIAN_POINT('Origin',(0.,-6.3,-14.49)) ;
#164838=CARTESIAN_POINT('Origin',(-4.65,-6.3,-14.49)) ;
#164839=CARTESIAN_POINT('Origin',(0.,-6.3,-15.99)) ;
#164840=CARTESIAN_POINT('Origin',(-4.65,-6.3,-15.99)) ;
#164841=CARTESIAN_POINT('Origin',(-4.65,-6.25,-15.99)) ;
#164842=CARTESIAN_POINT('Origin',(-4.65,-6.3,-15.99)) ;
#164843=CARTESIAN_POINT('Origin',(-4.65,-6.3,-14.49)) ;
#164844=CARTESIAN_POINT('Origin',(-4.65,-6.3,-14.49)) ;
#164845=CARTESIAN_POINT('Origin',(-4.65,-6.3,-15.99)) ;
#164846=CARTESIAN_POINT('Origin',(-4.65,-6.3,-15.99)) ;
#164847=CARTESIAN_POINT('Origin',(-4.65,-6.3,-15.24)) ;
#164848=CARTESIAN_POINT('Origin',(-3.,4.45,-16.34)) ;
#164849=CARTESIAN_POINT('Origin',(-2.1,4.45,-16.34)) ;
#164850=CARTESIAN_POINT('Origin',(-2.9,4.45,-16.34)) ;
#164851=CARTESIAN_POINT('Origin',(-2.9,4.45,-16.14)) ;
#164852=CARTESIAN_POINT('Origin',(-3.1,4.45,-16.14)) ;
#164853=CARTESIAN_POINT('Origin',(-2.9,4.45,-16.14)) ;
#164854=CARTESIAN_POINT('Origin',(-2.1,4.45,-16.14)) ;
#164855=CARTESIAN_POINT('Origin',(-2.1,4.45,-16.14)) ;
#164856=CARTESIAN_POINT('Origin',(-1.9,4.45,-16.14)) ;
#164857=CARTESIAN_POINT('Origin',(-3.1,4.45,-16.24)) ;
#164858=CARTESIAN_POINT('Origin',(-3.1,4.45,-14.34)) ;
#164859=CARTESIAN_POINT('Origin',(-2.9,4.4,-16.14)) ;
#164860=CARTESIAN_POINT('Origin',(-2.9,4.35,-16.14)) ;
#164861=CARTESIAN_POINT('Origin',(-1.95156391047391E-16,4.35,-16.14)) ;
#164862=CARTESIAN_POINT('Origin',(-2.1,4.35,-16.14)) ;
#164863=CARTESIAN_POINT('Origin',(-2.9,4.35,-16.14)) ;
#164864=CARTESIAN_POINT('Origin',(-2.1,4.4,-16.14)) ;
#164865=CARTESIAN_POINT('Origin',(-2.1,4.35,-16.14)) ;
#164866=CARTESIAN_POINT('Origin',(-1.9,4.45,-16.24)) ;
#164867=CARTESIAN_POINT('Origin',(-1.9,4.45,-14.34)) ;
#164868=CARTESIAN_POINT('Origin',(-3.,4.45,-14.14)) ;
#164869=CARTESIAN_POINT('Origin',(-2.9,4.45,-14.14)) ;
#164870=CARTESIAN_POINT('Origin',(-2.1,4.45,-14.14)) ;
#164871=CARTESIAN_POINT('Origin',(-2.9,4.45,-14.34)) ;
#164872=CARTESIAN_POINT('Origin',(-2.9,4.45,-14.34)) ;
#164873=CARTESIAN_POINT('Origin',(-2.9,4.35,-16.14)) ;
#164874=CARTESIAN_POINT('Origin',(-2.9,4.35,-16.14)) ;
#164875=CARTESIAN_POINT('Origin',(-2.1,4.35,-16.14)) ;
#164876=CARTESIAN_POINT('Origin',(-2.1,4.35,-16.14)) ;
#164877=CARTESIAN_POINT('Origin',(-2.1,4.45,-14.34)) ;
#164878=CARTESIAN_POINT('Origin',(-2.1,4.45,-14.34)) ;
#164879=CARTESIAN_POINT('Origin',(-2.9,4.4,-14.34)) ;
#164880=CARTESIAN_POINT('Origin',(-2.9,4.35,-14.34)) ;
#164881=CARTESIAN_POINT('Origin',(-2.9,4.35,-15.24)) ;
#164882=CARTESIAN_POINT('Origin',(-2.9,4.35,-14.34)) ;
#164883=CARTESIAN_POINT('Origin',(-2.1,4.35,-15.24)) ;
#164884=CARTESIAN_POINT('Origin',(-2.1,4.35,-14.34)) ;
#164885=CARTESIAN_POINT('Origin',(-2.1,4.4,-14.34)) ;
#164886=CARTESIAN_POINT('Origin',(-2.1,4.35,-14.34)) ;
#164887=CARTESIAN_POINT('Origin',(-2.9,4.35,-14.34)) ;
#164888=CARTESIAN_POINT('Origin',(-2.9,4.35,-14.34)) ;
#164889=CARTESIAN_POINT('Origin',(-2.1,4.35,-14.34)) ;
#164890=CARTESIAN_POINT('Origin',(-2.1,4.35,-14.34)) ;
#164891=CARTESIAN_POINT('Origin',(-1.95156391047391E-16,4.35,-14.34)) ;
#164892=CARTESIAN_POINT('Origin',(-2.25,4.25,-15.99)) ;
#164893=CARTESIAN_POINT('Origin',(-2.25,4.3,-15.99)) ;
#164894=CARTESIAN_POINT('Origin',(-2.25,4.3,-15.24)) ;
#164895=CARTESIAN_POINT('Origin',(-2.25,4.3,-14.49)) ;
#164896=CARTESIAN_POINT('Origin',(-2.25,4.3,-15.99)) ;
#164897=CARTESIAN_POINT('Origin',(-2.25,4.25,-14.49)) ;
#164898=CARTESIAN_POINT('Origin',(-2.25,4.3,-14.49)) ;
#164899=CARTESIAN_POINT('Origin',(-2.25,4.3,-15.99)) ;
#164900=CARTESIAN_POINT('Origin',(-2.25,4.3,-15.99)) ;
#164901=CARTESIAN_POINT('Origin',(-2.25,4.3,-14.49)) ;
#164902=CARTESIAN_POINT('Origin',(-2.25,4.3,-14.49)) ;
#164903=CARTESIAN_POINT('Origin',(-2.75,4.25,-15.99)) ;
#164904=CARTESIAN_POINT('Origin',(-2.75,4.3,-15.99)) ;
#164905=CARTESIAN_POINT('Origin',(-1.97127667724637E-17,4.3,-15.99)) ;
#164906=CARTESIAN_POINT('Origin',(-2.75,4.3,-15.99)) ;
#164907=CARTESIAN_POINT('Origin',(-1.97127667724637E-17,4.3,-14.49)) ;
#164908=CARTESIAN_POINT('Origin',(-2.75,4.3,-14.49)) ;
#164909=CARTESIAN_POINT('Origin',(-2.75,4.25,-14.49)) ;
#164910=CARTESIAN_POINT('Origin',(-2.75,4.3,-14.49)) ;
#164911=CARTESIAN_POINT('Origin',(-2.75,4.3,-15.99)) ;
#164912=CARTESIAN_POINT('Origin',(-2.75,4.3,-15.99)) ;
#164913=CARTESIAN_POINT('Origin',(-2.75,4.3,-14.49)) ;
#164914=CARTESIAN_POINT('Origin',(-2.75,4.3,-14.49)) ;
#164915=CARTESIAN_POINT('Origin',(-2.75,4.3,-15.24)) ;
#164916=CARTESIAN_POINT('Origin',(7.8,2.9,-15.64)) ;
#164917=CARTESIAN_POINT('Origin',(7.8,2.9,-15.64)) ;
#164918=CARTESIAN_POINT('Origin',(7.8,2.9,-14.84)) ;
#164919=CARTESIAN_POINT('Origin',(7.8,2.9,-14.84)) ;
#164920=CARTESIAN_POINT('Origin',(7.8,2.9,-14.84)) ;
#164921=CARTESIAN_POINT('Origin',(7.8,2.9,-15.64)) ;
#164922=CARTESIAN_POINT('Origin',(7.8,2.9,-15.64)) ;
#164923=CARTESIAN_POINT('Origin',(9.6,2.9,-14.84)) ;
#164924=CARTESIAN_POINT('Origin',(9.6,2.9,-14.84)) ;
#164925=CARTESIAN_POINT('Origin',(9.6,2.9,-15.64)) ;
#164926=CARTESIAN_POINT('Origin',(9.6,2.9,-15.64)) ;
#164927=CARTESIAN_POINT('Origin',(9.6,2.9,-14.84)) ;
#164928=CARTESIAN_POINT('Origin',(9.6,2.9,-14.84)) ;
#164929=CARTESIAN_POINT('Origin',(9.6,2.9,-15.64)) ;
#164930=CARTESIAN_POINT('Origin',(9.6,2.9,-15.64)) ;
#164931=CARTESIAN_POINT('Origin',(9.6,2.9,-15.64)) ;
#164932=CARTESIAN_POINT('Origin',(-0.183301359729408,3.45,-13.722963213524)) ;
#164933=CARTESIAN_POINT('Origin',(0.249234641435079,3.15,-15.1237799780213)) ;
#164934=CARTESIAN_POINT('Origin',(-0.249234641435079,3.15,-15.3562200219787)) ;
#164935=CARTESIAN_POINT('Origin',(-1.04429375741423,3.45,-14.1244505621777)) ;
#164936=CARTESIAN_POINT('Origin',(10.1,-2.15,-18.1468804065906)) ;
#164937=CARTESIAN_POINT('Origin',(10.1,-2.15,-18.1468804065906)) ;
#164938=CARTESIAN_POINT('Origin',(10.1,-2.15,-18.1468804065906)) ;
#164939=CARTESIAN_POINT('Origin',(10.1,-2.15,-18.1468804065906)) ;
#164940=CARTESIAN_POINT('Origin',(10.1,-2.15,-19.05)) ;
#164941=CARTESIAN_POINT('Origin',(10.1,-2.15,-17.745)) ;
#164942=CARTESIAN_POINT('Origin',(10.2,-2.15,-18.1468804065906)) ;
#164943=CARTESIAN_POINT('Origin',(3.7,-2.15,-18.1468804065906)) ;
#164944=CARTESIAN_POINT('Origin',(10.1,-3.65625,-19.05)) ;
#164945=CARTESIAN_POINT('Origin',(10.1,-2.15,-19.9531195934094)) ;
#164946=CARTESIAN_POINT('Origin',(10.1,-3.65625,-17.745)) ;
#164947=CARTESIAN_POINT('Origin',(10.1,1.9,-17.745)) ;
#164948=CARTESIAN_POINT('Origin',(10.1,-2.15,-17.745)) ;
#164949=CARTESIAN_POINT('Origin',(10.1,-2.15,-17.745)) ;
#164950=CARTESIAN_POINT('Origin',(10.1,-2.15,-17.745)) ;
#164951=CARTESIAN_POINT('Origin',(3.7,-2.15,-18.1468804065906)) ;
#164952=CARTESIAN_POINT('Origin',(3.7,-2.32153024911032,-18.2497267659824)) ;
#164953=CARTESIAN_POINT('Origin',(3.7,-2.35,-18.1468804065906)) ;
#164954=CARTESIAN_POINT('Origin',(10.1,-2.15,-19.9531195934094)) ;
#164955=CARTESIAN_POINT('Origin',(10.1,-2.15,-19.9531195934094)) ;
#164956=CARTESIAN_POINT('Origin',(10.1,-2.15,-19.9531195934094)) ;
#164957=CARTESIAN_POINT('Origin',(10.1,1.9,-19.05)) ;
#164958=CARTESIAN_POINT('Origin',(10.1,1.9,-20.355)) ;
#164959=CARTESIAN_POINT('Origin',(10.1,1.9,-17.745)) ;
#164960=CARTESIAN_POINT('Origin',(10.2,-2.15,-17.745)) ;
#164961=CARTESIAN_POINT('Origin',(3.7,-2.15,-17.745)) ;
#164962=CARTESIAN_POINT('Origin',(3.7,-2.35,-17.645)) ;
#164963=CARTESIAN_POINT('Origin',(3.7,-2.35,-17.745)) ;
#164964=CARTESIAN_POINT('Origin',(3.7,-3.65625,-19.05)) ;
#164965=CARTESIAN_POINT('Origin',(3.7,-2.32153024911032,-19.8502732340176)) ;
#164966=CARTESIAN_POINT('Origin',(10.2,-2.15,-19.9531195934094)) ;
#164967=CARTESIAN_POINT('Origin',(3.7,-2.15,-19.9531195934094)) ;
#164968=CARTESIAN_POINT('Origin',(10.1,-2.15,-19.05)) ;
#164969=CARTESIAN_POINT('Origin',(10.1,-2.15,-20.355)) ;
#164970=CARTESIAN_POINT('Origin',(10.1,-3.65625,-20.355)) ;
#164971=CARTESIAN_POINT('Origin',(10.1,1.9,-20.355)) ;
#164972=CARTESIAN_POINT('Origin',(10.1,-2.15,-20.355)) ;
#164973=CARTESIAN_POINT('Origin',(3.7,-2.35,-17.745)) ;
#164974=CARTESIAN_POINT('Origin',(3.5,-2.35,-17.745)) ;
#164975=CARTESIAN_POINT('Origin',(3.7,-2.15,-19.9531195934094)) ;
#164976=CARTESIAN_POINT('Origin',(3.7,-2.35,-19.9531195934094)) ;
#164977=CARTESIAN_POINT('Origin',(10.1,-2.15,-20.355)) ;
#164978=CARTESIAN_POINT('Origin',(10.1,-2.15,-20.355)) ;
#164979=CARTESIAN_POINT('Origin',(3.6,1.9,-17.545)) ;
#164980=CARTESIAN_POINT('Origin',(3.5,1.9,-17.545)) ;
#164981=CARTESIAN_POINT('Origin',(2.7,1.9,-17.545)) ;
#164982=CARTESIAN_POINT('Origin',(3.5,1.67034766683375E-15,-17.745)) ;
#164983=CARTESIAN_POINT('Origin',(3.5,-5.15,-17.745)) ;
#164984=CARTESIAN_POINT('Origin',(3.7,-2.35,-19.925)) ;
#164985=CARTESIAN_POINT('Origin',(3.7,-2.35,-20.355)) ;
#164986=CARTESIAN_POINT('Origin',(3.6,-2.15,-20.355)) ;
#164987=CARTESIAN_POINT('Origin',(3.7,-2.15,-20.355)) ;
#164988=CARTESIAN_POINT('Origin',(2.7,1.9,-17.545)) ;
#164989=CARTESIAN_POINT('Origin',(2.7,1.9,-17.545)) ;
#164990=CARTESIAN_POINT('Origin',(3.5,-5.15,-17.745)) ;
#164991=CARTESIAN_POINT('Origin',(3.5,-5.15,-17.745)) ;
#164992=CARTESIAN_POINT('Origin',(3.5,-5.15,-17.745)) ;
#164993=CARTESIAN_POINT('Origin',(3.7,-2.35,-20.355)) ;
#164994=CARTESIAN_POINT('Origin',(3.5,-2.35,-20.355)) ;
#164995=CARTESIAN_POINT('Origin',(2.7,2.,-17.545)) ;
#164996=CARTESIAN_POINT('Origin',(2.7,-5.15,-17.545)) ;
#164997=CARTESIAN_POINT('Origin',(3.6,-5.15,-17.745)) ;
#164998=CARTESIAN_POINT('Origin',(2.7,-5.15,-17.745)) ;
#164999=CARTESIAN_POINT('Origin',(3.5,-5.15,0.)) ;
#165000=CARTESIAN_POINT('Origin',(3.5,-5.15,-20.355)) ;
#165001=CARTESIAN_POINT('Origin',(3.5,-1.74825394185847E-15,-20.355)) ;
#165002=CARTESIAN_POINT('Origin',(3.5,-5.15,-20.355)) ;
#165003=CARTESIAN_POINT('Origin',(2.7,-5.15,-17.745)) ;
#165004=CARTESIAN_POINT('Origin',(2.7,-5.35,-17.745)) ;
#165005=CARTESIAN_POINT('Origin',(3.5,-5.15,-20.355)) ;
#165006=CARTESIAN_POINT('Origin',(3.5,-5.15,-20.355)) ;
#165007=CARTESIAN_POINT('Origin',(2.7,-5.35,-17.645)) ;
#165008=CARTESIAN_POINT('Origin',(2.7,-5.35,-20.355)) ;
#165009=CARTESIAN_POINT('Origin',(3.6,-5.15,-20.355)) ;
#165010=CARTESIAN_POINT('Origin',(2.7,-5.15,-20.355)) ;
#165011=CARTESIAN_POINT('Origin',(3.6,1.9,-20.555)) ;
#165012=CARTESIAN_POINT('Origin',(3.5,1.9,-20.555)) ;
#165013=CARTESIAN_POINT('Origin',(2.7,1.9,-20.555)) ;
#165014=CARTESIAN_POINT('Origin',(2.7,1.9,-20.455)) ;
#165015=CARTESIAN_POINT('Origin',(2.7,1.9,-21.355)) ;
#165016=CARTESIAN_POINT('Origin',(2.7,1.9,-20.555)) ;
#165017=CARTESIAN_POINT('Origin',(2.7,-5.15,-20.355)) ;
#165018=CARTESIAN_POINT('Origin',(2.7,-5.15,-20.555)) ;
#165019=CARTESIAN_POINT('Origin',(2.7,1.9,-20.555)) ;
#165020=CARTESIAN_POINT('Origin',(2.7,1.9,-20.555)) ;
#165021=CARTESIAN_POINT('Origin',(2.7,-5.25,-20.555)) ;
#165022=CARTESIAN_POINT('Ctrl Pts',(-3.8,-6.55,-17.95)) ;
#165023=CARTESIAN_POINT('Ctrl Pts',(-3.8,-6.55,-17.95)) ;
#165024=CARTESIAN_POINT('Ctrl Pts',(-3.8,-6.55,-17.95)) ;
#165025=CARTESIAN_POINT('Ctrl Pts',(-3.82625343282631,-6.55,-18.0025068656527)) ;
#165026=CARTESIAN_POINT('Ctrl Pts',(-3.83954133268377,-6.55,-17.9895413326839)) ;
#165027=CARTESIAN_POINT('Ctrl Pts',(-3.8525068656527,-6.55,-17.9762534328264)) ;
#165028=CARTESIAN_POINT('Ctrl Pts',(-3.85219871729854,-6.53922263893877,
-18.0543974345971)) ;
#165029=CARTESIAN_POINT('Ctrl Pts',(-3.87914655110981,-6.52362528614074,
-18.0291465511099)) ;
#165030=CARTESIAN_POINT('Ctrl Pts',(-3.90439743459708,-6.53922263893874,
-18.0021987172986)) ;
#165031=CARTESIAN_POINT('Ctrl Pts',(-3.87996665852871,-6.5114546977086,
-18.1099333170574)) ;
#165032=CARTESIAN_POINT('Ctrl Pts',(-3.90288380314161,-6.48208554016475,
-18.0528838031416)) ;
#165033=CARTESIAN_POINT('Ctrl Pts',(-3.95993331705742,-6.51145469770861,
-18.0299666585287)) ;
#165034=CARTESIAN_POINT('Ctrl Pts',(-3.88737865704135,-6.5003618540841,
-18.1247573140827)) ;
#165035=CARTESIAN_POINT('Ctrl Pts',(-3.90501307588293,-6.46792722356046,
-18.0550130758829)) ;
#165036=CARTESIAN_POINT('Ctrl Pts',(-3.9747573140827,-6.5003618540841,-18.0373786570414)) ;
#165037=CARTESIAN_POINT('Ctrl Pts',(-3.8973972494609,-6.47617483238892,
-18.1447944989218)) ;
#165038=CARTESIAN_POINT('Ctrl Pts',(-3.9032967435641,-6.45094059868421,
-18.0532967435641)) ;
#165039=CARTESIAN_POINT('Ctrl Pts',(-3.99479449892181,-6.47617483238891,
-18.0473972494609)) ;
#165040=CARTESIAN_POINT('Ctrl Pts',(-3.9,-6.46309229646327,-18.1499999991818)) ;
#165041=CARTESIAN_POINT('Ctrl Pts',(-3.90000730394106,-6.44945650151457,
-18.0500073039033)) ;
#165042=CARTESIAN_POINT('Ctrl Pts',(-3.99999999918173,-6.46309229646329,
-18.05)) ;
#165043=CARTESIAN_POINT('Ctrl Pts',(-3.9,-6.45,-18.15)) ;
#165044=CARTESIAN_POINT('Ctrl Pts',(-3.9,-6.45,-18.05)) ;
#165045=CARTESIAN_POINT('Ctrl Pts',(-4.,-6.45,-18.05)) ;
#165046=CARTESIAN_POINT('Origin',(-4.,-6.45,-18.15)) ;
#165047=CARTESIAN_POINT('Origin',(-4.,-6.4,-18.15)) ;
#165048=CARTESIAN_POINT('Origin',(-4.,-6.35,-18.15)) ;
#165049=CARTESIAN_POINT('Ctrl Pts',(-5.,-6.55,-17.95)) ;
#165050=CARTESIAN_POINT('Ctrl Pts',(-5.,-6.55,-17.95)) ;
#165051=CARTESIAN_POINT('Ctrl Pts',(-5.,-6.55,-17.95)) ;
#165052=CARTESIAN_POINT('Ctrl Pts',(-4.94749313434733,-6.55,-17.9762534328264)) ;
#165053=CARTESIAN_POINT('Ctrl Pts',(-4.96045866731622,-6.55,-17.989541332684)) ;
#165054=CARTESIAN_POINT('Ctrl Pts',(-4.97374656717362,-6.55,-18.0025068656527)) ;
#165055=CARTESIAN_POINT('Ctrl Pts',(-4.89560256540291,-6.53922263893874,
-18.0021987172986)) ;
#165056=CARTESIAN_POINT('Ctrl Pts',(-4.92085344889017,-6.52362528614074,
-18.0291465511099)) ;
#165057=CARTESIAN_POINT('Ctrl Pts',(-4.94780128270146,-6.53922263893877,
-18.0543974345971)) ;
#165058=CARTESIAN_POINT('Ctrl Pts',(-4.84006668294258,-6.51145469770861,
-18.0299666585287)) ;
#165059=CARTESIAN_POINT('Ctrl Pts',(-4.8971161968584,-6.48208554016475,
-18.0528838031416)) ;
#165060=CARTESIAN_POINT('Ctrl Pts',(-4.92003334147129,-6.5114546977086,
-18.1099333170574)) ;
#165061=CARTESIAN_POINT('Ctrl Pts',(-4.82524268591729,-6.5003618540841,
-18.0373786570414)) ;
#165062=CARTESIAN_POINT('Ctrl Pts',(-4.89498692411706,-6.46792722356047,
-18.0550130758829)) ;
#165063=CARTESIAN_POINT('Ctrl Pts',(-4.91262134295865,-6.5003618540841,
-18.1247573140827)) ;
#165064=CARTESIAN_POINT('Ctrl Pts',(-4.80520550107819,-6.47617483238891,
-18.0473972494609)) ;
#165065=CARTESIAN_POINT('Ctrl Pts',(-4.8967032564359,-6.4509405986842,-18.0532967435642)) ;
#165066=CARTESIAN_POINT('Ctrl Pts',(-4.90260275053909,-6.47617483238892,
-18.1447944989218)) ;
#165067=CARTESIAN_POINT('Ctrl Pts',(-4.80000000081823,-6.46309229646328,
-18.05)) ;
#165068=CARTESIAN_POINT('Ctrl Pts',(-4.89999269603999,-6.44945650152247,
-18.0500073039034)) ;
#165069=CARTESIAN_POINT('Ctrl Pts',(-4.9,-6.46309229646329,-18.1499999991818)) ;
#165070=CARTESIAN_POINT('Ctrl Pts',(-4.8,-6.45,-18.05)) ;
#165071=CARTESIAN_POINT('Ctrl Pts',(-4.9,-6.45,-18.05)) ;
#165072=CARTESIAN_POINT('Ctrl Pts',(-4.9,-6.45,-18.15)) ;
#165073=CARTESIAN_POINT('Origin',(-4.8,-6.45,-18.15)) ;
#165074=CARTESIAN_POINT('Origin',(-4.,-6.35,-18.15)) ;
#165075=CARTESIAN_POINT('Origin',(-4.,-6.35,-18.15)) ;
#165076=CARTESIAN_POINT('Origin',(-4.,-6.35,-18.15)) ;
#165077=CARTESIAN_POINT('Ctrl Pts',(-3.8,-6.55,-20.15)) ;
#165078=CARTESIAN_POINT('Ctrl Pts',(-3.8,-6.55,-20.15)) ;
#165079=CARTESIAN_POINT('Ctrl Pts',(-3.8,-6.55,-20.15)) ;
#165080=CARTESIAN_POINT('Ctrl Pts',(-3.85250686565272,-6.55,-20.1237465671736)) ;
#165081=CARTESIAN_POINT('Ctrl Pts',(-3.83954133268385,-6.55,-20.1104586673161)) ;
#165082=CARTESIAN_POINT('Ctrl Pts',(-3.82625343282627,-6.55,-20.0974931343473)) ;
#165083=CARTESIAN_POINT('Ctrl Pts',(-3.90439743459706,-6.53922263893874,
-20.0978012827014)) ;
#165084=CARTESIAN_POINT('Ctrl Pts',(-3.87914655110978,-6.52362528614071,
-20.0708534488901)) ;
#165085=CARTESIAN_POINT('Ctrl Pts',(-3.85219871729855,-6.53922263893876,
-20.0456025654029)) ;
#165086=CARTESIAN_POINT('Ctrl Pts',(-3.95993331705743,-6.51145469770861,
-20.0700333414713)) ;
#165087=CARTESIAN_POINT('Ctrl Pts',(-3.90288380314162,-6.48208554016476,
-20.0471161968584)) ;
#165088=CARTESIAN_POINT('Ctrl Pts',(-3.8799666585287,-6.5114546977086,-19.9900666829426)) ;
#165089=CARTESIAN_POINT('Ctrl Pts',(-3.97475731408271,-6.5003618540841,
-20.0626213429587)) ;
#165090=CARTESIAN_POINT('Ctrl Pts',(-3.90501307588293,-6.46792722356047,
-20.0449869241171)) ;
#165091=CARTESIAN_POINT('Ctrl Pts',(-3.88737865704135,-6.5003618540841,
-19.9752426859173)) ;
#165092=CARTESIAN_POINT('Ctrl Pts',(-3.9947944989218,-6.47617483238891,
-20.0526027505391)) ;
#165093=CARTESIAN_POINT('Ctrl Pts',(-3.9032967435641,-6.4509405986842,-20.0467032564358)) ;
#165094=CARTESIAN_POINT('Ctrl Pts',(-3.89739724946091,-6.47617483238892,
-19.9552055010782)) ;
#165095=CARTESIAN_POINT('Ctrl Pts',(-3.99999999918176,-6.46309229646328,
-20.05)) ;
#165096=CARTESIAN_POINT('Ctrl Pts',(-3.90000730395532,-6.44945650152054,
-20.0499926960966)) ;
#165097=CARTESIAN_POINT('Ctrl Pts',(-3.9,-6.46309229646328,-19.9500000008182)) ;
#165098=CARTESIAN_POINT('Ctrl Pts',(-4.,-6.45,-20.05)) ;
#165099=CARTESIAN_POINT('Ctrl Pts',(-3.9,-6.45,-20.05)) ;
#165100=CARTESIAN_POINT('Ctrl Pts',(-3.9,-6.45,-19.95)) ;
#165101=CARTESIAN_POINT('Origin',(-4.,-6.45,-19.95)) ;
#165102=CARTESIAN_POINT('Origin',(-4.8,-6.4,-18.15)) ;
#165103=CARTESIAN_POINT('Origin',(-4.8,-6.35,-18.15)) ;
#165104=CARTESIAN_POINT('Origin',(1.9515639104739E-16,-6.35,-18.15)) ;
#165105=CARTESIAN_POINT('Origin',(-4.8,-6.35,-18.15)) ;
#165106=CARTESIAN_POINT('Origin',(-4.,-6.35,-19.05)) ;
#165107=CARTESIAN_POINT('Origin',(-4.,-6.35,-19.95)) ;
#165108=CARTESIAN_POINT('Origin',(-4.,-6.4,-19.95)) ;
#165109=CARTESIAN_POINT('Origin',(-4.,-6.35,-19.95)) ;
#165110=CARTESIAN_POINT('Origin',(-4.8,-6.35,-18.15)) ;
#165111=CARTESIAN_POINT('Origin',(-4.8,-6.35,-18.15)) ;
#165112=CARTESIAN_POINT('Origin',(-4.,-6.35,-19.95)) ;
#165113=CARTESIAN_POINT('Origin',(-4.,-6.35,-19.95)) ;
#165114=CARTESIAN_POINT('Origin',(-4.8,-6.35,-19.05)) ;
#165115=CARTESIAN_POINT('Origin',(-4.8,-6.35,-19.95)) ;
#165116=CARTESIAN_POINT('Origin',(1.95156391047391E-16,-6.35,-19.95)) ;
#165117=CARTESIAN_POINT('Origin',(-4.8,-6.35,-19.95)) ;
#165118=CARTESIAN_POINT('Origin',(-4.8,-6.35,-19.95)) ;
#165119=CARTESIAN_POINT('Origin',(-4.8,-6.35,-19.95)) ;
#165120=CARTESIAN_POINT('Origin',(-4.8,-6.4,-19.95)) ;
#165121=CARTESIAN_POINT('Origin',(-4.8,-6.45,-19.95)) ;
#165122=CARTESIAN_POINT('Ctrl Pts',(-5.,-6.55,-20.15)) ;
#165123=CARTESIAN_POINT('Ctrl Pts',(-5.,-6.55,-20.15)) ;
#165124=CARTESIAN_POINT('Ctrl Pts',(-5.,-6.55,-20.15)) ;
#165125=CARTESIAN_POINT('Ctrl Pts',(-4.97374656717362,-6.55,-20.0974931343473)) ;
#165126=CARTESIAN_POINT('Ctrl Pts',(-4.96045866731623,-6.55,-20.110458667316)) ;
#165127=CARTESIAN_POINT('Ctrl Pts',(-4.94749313434733,-6.55,-20.1237465671736)) ;
#165128=CARTESIAN_POINT('Ctrl Pts',(-4.94780128270146,-6.53922263893877,
-20.0456025654029)) ;
#165129=CARTESIAN_POINT('Ctrl Pts',(-4.92085344889017,-6.52362528614074,
-20.0708534488901)) ;
#165130=CARTESIAN_POINT('Ctrl Pts',(-4.89560256540291,-6.53922263893874,
-20.0978012827014)) ;
#165131=CARTESIAN_POINT('Ctrl Pts',(-4.92003334147129,-6.5114546977086,
-19.9900666829426)) ;
#165132=CARTESIAN_POINT('Ctrl Pts',(-4.8971161968584,-6.48208554016475,
-20.0471161968584)) ;
#165133=CARTESIAN_POINT('Ctrl Pts',(-4.84006668294258,-6.51145469770861,
-20.0700333414713)) ;
#165134=CARTESIAN_POINT('Ctrl Pts',(-4.91262134295865,-6.5003618540841,
-19.9752426859173)) ;
#165135=CARTESIAN_POINT('Ctrl Pts',(-4.89498692411706,-6.46792722356047,
-20.0449869241171)) ;
#165136=CARTESIAN_POINT('Ctrl Pts',(-4.82524268591729,-6.5003618540841,
-20.0626213429587)) ;
#165137=CARTESIAN_POINT('Ctrl Pts',(-4.90260275053909,-6.47617483238892,
-19.9552055010782)) ;
#165138=CARTESIAN_POINT('Ctrl Pts',(-4.8967032564359,-6.4509405986842,-20.0467032564358)) ;
#165139=CARTESIAN_POINT('Ctrl Pts',(-4.80520550107819,-6.47617483238891,
-20.0526027505391)) ;
#165140=CARTESIAN_POINT('Ctrl Pts',(-4.9,-6.46309229646328,-19.9500000008182)) ;
#165141=CARTESIAN_POINT('Ctrl Pts',(-4.89999269603999,-6.44945650152247,
-20.0499926960966)) ;
#165142=CARTESIAN_POINT('Ctrl Pts',(-4.80000000081823,-6.46309229646328,
-20.05)) ;
#165143=CARTESIAN_POINT('Ctrl Pts',(-4.9,-6.45,-19.95)) ;
#165144=CARTESIAN_POINT('Ctrl Pts',(-4.9,-6.45,-20.05)) ;
#165145=CARTESIAN_POINT('Ctrl Pts',(-4.8,-6.45,-20.05)) ;
#165146=CARTESIAN_POINT('Ctrl Pts',(-5.82426676739348,-5.43399303700626,
-17.4470109659688)) ;
#165147=CARTESIAN_POINT('Ctrl Pts',(-5.80266988778314,-5.52572360682945,
-17.4523540173507)) ;
#165148=CARTESIAN_POINT('Ctrl Pts',(-5.82426676352019,-5.53106667371342,
-17.5440845871829)) ;
#165149=CARTESIAN_POINT('Ctrl Pts',(-5.83498671931113,-5.43935351191921,
-17.4443294581962)) ;
#165150=CARTESIAN_POINT('Ctrl Pts',(-5.80595263122268,-5.52411753147717,
-17.4539600935404)) ;
#165151=CARTESIAN_POINT('Ctrl Pts',(-5.8349867139763,-5.5337481806747,-17.5387241131464)) ;
#165152=CARTESIAN_POINT('Ctrl Pts',(-5.84526105845708,-5.44830326289504,
-17.4398528401961)) ;
#165153=CARTESIAN_POINT('Ctrl Pts',(-5.8137093274614,-5.52260132030862,
-17.4554763059992)) ;
#165154=CARTESIAN_POINT('Ctrl Pts',(-5.84526105243725,-5.53822479746341,
-17.5297743635699)) ;
#165155=CARTESIAN_POINT('Ctrl Pts',(-5.86378685403694,-5.47240020430411,
-17.4278032513088)) ;
#165156=CARTESIAN_POINT('Ctrl Pts',(-5.83531854275286,-5.52733067404489,
-17.4507469551147)) ;
#165157=CARTESIAN_POINT('Ctrl Pts',(-5.86378684816464,-5.55027438459902,
-17.5056774250056)) ;
#165158=CARTESIAN_POINT('Ctrl Pts',(-5.87203852631572,-5.48754495134743,
-17.4202315528944)) ;
#165159=CARTESIAN_POINT('Ctrl Pts',(-5.84834787930686,-5.53310199490459,
-17.4449756357761)) ;
#165160=CARTESIAN_POINT('Ctrl Pts',(-5.87203852123043,-5.5578460824346,
-17.490532679514)) ;
#165161=CARTESIAN_POINT('Ctrl Pts',(-5.89242747304799,-5.53981202333459,
-17.3941056511376)) ;
#165162=CARTESIAN_POINT('Ctrl Pts',(-5.88223383300419,-5.56084219179275,
-17.4172354431742)) ;
#165163=CARTESIAN_POINT('Ctrl Pts',(-5.89242747063503,-5.58397198402777,
-17.4382656123278)) ;
#165164=CARTESIAN_POINT('Ctrl Pts',(-5.9,-5.58381083947301,-17.3721194001431)) ;
#165165=CARTESIAN_POINT('Ctrl Pts',(-5.9,-5.59485304502678,-17.3832245928864)) ;
#165166=CARTESIAN_POINT('Ctrl Pts',(-5.9,-5.60595823775504,-17.3942667984405)) ;
#165167=CARTESIAN_POINT('Ctrl Pts',(-5.9,-5.62807764064044,-17.35)) ;
#165168=CARTESIAN_POINT('Ctrl Pts',(-5.9,-5.62807764064044,-17.35)) ;
#165169=CARTESIAN_POINT('Ctrl Pts',(-5.9,-5.62807764064044,-17.35)) ;
#165170=CARTESIAN_POINT('Origin',(-5.84850712500726,-5.43404914061138,-17.5440285000291)) ;
#165171=CARTESIAN_POINT('Ctrl Pts',(-5.82425356250363,-5.53106339062591,
-17.5440285000291)) ;
#165172=CARTESIAN_POINT('Ctrl Pts',(-5.80269484027818,-5.52567371006955,
-17.4524039305709)) ;
#165173=CARTESIAN_POINT('Ctrl Pts',(-5.82425356250363,-5.43404914061138,
-17.4470142500145)) ;
#165174=CARTESIAN_POINT('Ctrl Pts',(-5.80840777707096,-5.52710194426774,
-17.5479899459043)) ;
#165175=CARTESIAN_POINT('Ctrl Pts',(-5.7934141764523,-5.52335354411309,
-17.4528358498184)) ;
#165176=CARTESIAN_POINT('Ctrl Pts',(-5.81633079157288,-5.43008775511759,
-17.4489949427472)) ;
#165177=CARTESIAN_POINT('Ctrl Pts',(-5.79207992677989,-5.52301998169497,
-17.549999999534)) ;
#165178=CARTESIAN_POINT('Ctrl Pts',(-5.78430903206643,-5.52107725801661,
-17.4519613954329)) ;
#165179=CARTESIAN_POINT('Ctrl Pts',(-5.80816665318299,-5.42600568595106,
-17.45)) ;
#165180=CARTESIAN_POINT('Ctrl Pts',(-5.77574643749636,-5.51893660937409,
-17.55)) ;
#165181=CARTESIAN_POINT('Ctrl Pts',(-5.77574643749636,-5.51893660937409,
-17.45)) ;
#165182=CARTESIAN_POINT('Ctrl Pts',(-5.8,-5.42192235935956,-17.45)) ;
#165183=CARTESIAN_POINT('Origin',(-5.8,-5.42192235935956,-17.55)) ;
#165184=CARTESIAN_POINT('Origin',(-5.8066065036801,-5.42357398527959,-17.55)) ;
#165185=CARTESIAN_POINT('Origin',(-5.17275707706437,-5.26511162862565,-17.55)) ;
#165186=CARTESIAN_POINT('Origin',(-5.15068655017073,-5.25959399690224,-17.5605938529089)) ;
#165187=CARTESIAN_POINT('Origin',(-5.17275707706436,-5.26511162862565,-17.55)) ;
#165188=CARTESIAN_POINT('Origin',(-5.17275707706436,-5.26511162862565,-17.55)) ;
#165189=CARTESIAN_POINT('Origin',(-5.17275707706436,-5.26511162862565,-17.55)) ;
#165190=CARTESIAN_POINT('Origin',(-5.17275707706436,-5.05,-17.55)) ;
#165191=CARTESIAN_POINT('Origin',(-5.17275707706436,-1.91866427917294,-17.55)) ;
#165192=CARTESIAN_POINT('Origin',(-3.78014014831103,-3.31128120792626,-18.2184561258016)) ;
#165193=CARTESIAN_POINT('Origin',(-5.17275707706436,-1.91866427917294,-17.55)) ;
#165194=CARTESIAN_POINT('Origin',(-5.17275707706436,-1.91866427917293,-17.55)) ;
#165195=CARTESIAN_POINT('Origin',(-5.17275707706436,-1.91866427917294,-17.55)) ;
#165196=CARTESIAN_POINT('Origin',(-3.97071067811865,-3.12071067811865,-17.55)) ;
#165197=CARTESIAN_POINT('Origin',(-5.8,-1.2914213562373,-17.55)) ;
#165198=CARTESIAN_POINT('Ctrl Pts',(-5.87071067811865,-1.14999999999999,
-17.4207106781187)) ;
#165199=CARTESIAN_POINT('Ctrl Pts',(-5.8471404520791,-1.10285954792089,
-17.4442809041582)) ;
#165200=CARTESIAN_POINT('Ctrl Pts',(-5.87071067811865,-1.07928932188134,
-17.4914213562373)) ;
#165201=CARTESIAN_POINT('Ctrl Pts',(-5.85217562795657,-1.18707010095452,
-17.4392457282807)) ;
#165202=CARTESIAN_POINT('Ctrl Pts',(-5.81261165662082,-1.1373883433793,
-17.4658614719499)) ;
#165203=CARTESIAN_POINT('Ctrl Pts',(-5.8335394967105,-1.1164605032895,-17.5285925363811)) ;
#165204=CARTESIAN_POINT('Ctrl Pts',(-5.82627077431945,-1.23887980759835,
-17.45)) ;
#165205=CARTESIAN_POINT('Ctrl Pts',(-5.76566787907942,-1.18433212092055,
-17.4671489437127)) ;
#165206=CARTESIAN_POINT('Ctrl Pts',(-5.78190678732229,-1.16809321267771,
-17.5499999994186)) ;
#165207=CARTESIAN_POINT('Ctrl Pts',(-5.8,-1.2914213562373,-17.45)) ;
#165208=CARTESIAN_POINT('Ctrl Pts',(-5.72928932188134,-1.22071067811865,
-17.45)) ;
#165209=CARTESIAN_POINT('Ctrl Pts',(-5.72928932188134,-1.22071067811865,
-17.55)) ;
#165210=CARTESIAN_POINT('Origin',(-5.94142135623731,-1.15,-17.4914213562373)) ;
#165211=CARTESIAN_POINT('Ctrl Pts',(-5.9,-1.00857864376269,-17.35)) ;
#165212=CARTESIAN_POINT('Ctrl Pts',(-5.9,-1.00857864376269,-17.35)) ;
#165213=CARTESIAN_POINT('Ctrl Pts',(-5.9,-1.00857864376269,-17.35)) ;
#165214=CARTESIAN_POINT('Ctrl Pts',(-5.9,-1.06112019240164,-17.3762707743195)) ;
#165215=CARTESIAN_POINT('Ctrl Pts',(-5.9,-1.04860238145267,-17.3900237376901)) ;
#165216=CARTESIAN_POINT('Ctrl Pts',(-5.9,-1.03484941808214,-17.402541548639)) ;
#165217=CARTESIAN_POINT('Ctrl Pts',(-5.88924572828071,-1.11292989904543,
-17.4021756279566)) ;
#165218=CARTESIAN_POINT('Ctrl Pts',(-5.87451700627693,-1.08721613123091,
-17.4286374874681)) ;
#165219=CARTESIAN_POINT('Ctrl Pts',(-5.88924572828062,-1.06075427171938,
-17.4543512552826)) ;
#165220=CARTESIAN_POINT('Ctrl Pts',(-5.87071067811865,-1.14999999999999,
-17.4207106781187)) ;
#165221=CARTESIAN_POINT('Ctrl Pts',(-5.8471404520791,-1.10285954792089,
-17.4442809041582)) ;
#165222=CARTESIAN_POINT('Ctrl Pts',(-5.87071067811865,-1.07928932188134,
-17.4914213562373)) ;
#165223=CARTESIAN_POINT('Ctrl Pts',(-5.87071067811866,-1.14999999999999,
-20.6792893218813)) ;
#165224=CARTESIAN_POINT('Ctrl Pts',(-5.84714045207911,-1.10285954792089,
-20.6557190958418)) ;
#165225=CARTESIAN_POINT('Ctrl Pts',(-5.87071067811866,-1.07928932188134,
-20.6085786437627)) ;
#165226=CARTESIAN_POINT('Ctrl Pts',(-5.8892457282807,-1.11292989904542,
-20.6978243720434)) ;
#165227=CARTESIAN_POINT('Ctrl Pts',(-5.87451700627498,-1.08721613123207,
-20.6713625125308)) ;
#165228=CARTESIAN_POINT('Ctrl Pts',(-5.88924572828062,-1.06075427171937,
-20.6456487447174)) ;
#165229=CARTESIAN_POINT('Ctrl Pts',(-5.9,-1.06112019240159,-20.7237292256804)) ;
#165230=CARTESIAN_POINT('Ctrl Pts',(-5.9,-1.04860238145164,-20.7099762623107)) ;
#165231=CARTESIAN_POINT('Ctrl Pts',(-5.9,-1.03484941808214,-20.697458451361)) ;
#165232=CARTESIAN_POINT('Ctrl Pts',(-5.9,-1.00857864376269,-20.75)) ;
#165233=CARTESIAN_POINT('Ctrl Pts',(-5.9,-1.00857864376269,-20.75)) ;
#165234=CARTESIAN_POINT('Ctrl Pts',(-5.9,-1.00857864376269,-20.75)) ;
#165235=CARTESIAN_POINT('Origin',(-5.94142135623734,-1.14999999999996,-20.6085786437627)) ;
#165236=CARTESIAN_POINT('Ctrl Pts',(-5.8,-1.2914213562373,-20.65)) ;
#165237=CARTESIAN_POINT('Ctrl Pts',(-5.72928932188134,-1.22071067811865,
-20.65)) ;
#165238=CARTESIAN_POINT('Ctrl Pts',(-5.72928932188134,-1.22071067811865,
-20.55)) ;
#165239=CARTESIAN_POINT('Ctrl Pts',(-5.82627077431951,-1.23887980759822,
-20.65)) ;
#165240=CARTESIAN_POINT('Ctrl Pts',(-5.76566787907979,-1.18433212092022,
-20.6328510562872)) ;
#165241=CARTESIAN_POINT('Ctrl Pts',(-5.78190678732243,-1.16809321267756,
-20.5500000005814)) ;
#165242=CARTESIAN_POINT('Ctrl Pts',(-5.85217562795678,-1.18707010095483,
-20.6607542717195)) ;
#165243=CARTESIAN_POINT('Ctrl Pts',(-5.81261165662032,-1.13738834337969,
-20.6341385280508)) ;
#165244=CARTESIAN_POINT('Ctrl Pts',(-5.83353949671031,-1.11646050328968,
-20.571407463619)) ;
#165245=CARTESIAN_POINT('Ctrl Pts',(-5.87071067811866,-1.14999999999999,
-20.6792893218813)) ;
#165246=CARTESIAN_POINT('Ctrl Pts',(-5.84714045207911,-1.10285954792088,
-20.6557190958418)) ;
#165247=CARTESIAN_POINT('Ctrl Pts',(-5.87071067811866,-1.07928932188133,
-20.6085786437627)) ;
#165248=CARTESIAN_POINT('Origin',(-5.8,-1.29142135623731,-20.55)) ;
#165249=CARTESIAN_POINT('Origin',(-3.59571067811865,-3.49571067811865,-20.55)) ;
#165250=CARTESIAN_POINT('Origin',(-5.17275707706437,-1.91866427917293,-20.55)) ;
#165251=CARTESIAN_POINT('Origin',(-3.09057773798104,-4.00084361825625,-19.55055391724)) ;
#165252=CARTESIAN_POINT('Origin',(-5.17275707706436,-1.91866427917293,-20.55)) ;
#165253=CARTESIAN_POINT('Origin',(-5.17275707706436,-1.91866427917293,-20.55)) ;
#165254=CARTESIAN_POINT('Origin',(-5.17275707706436,-1.91866427917293,-20.55)) ;
#165255=CARTESIAN_POINT('Origin',(-5.17275707706436,-5.05,-20.55)) ;
#165256=CARTESIAN_POINT('Origin',(-5.17275707706436,-5.26511162862565,-20.55)) ;
#165257=CARTESIAN_POINT('Origin',(-3.96111272388873,-4.96220054033175,-19.9684107104757)) ;
#165258=CARTESIAN_POINT('Origin',(-5.17275707706436,-5.26511162862565,-20.55)) ;
#165259=CARTESIAN_POINT('Origin',(-5.17275707706436,-5.26511162862565,-20.55)) ;
#165260=CARTESIAN_POINT('Origin',(-5.17275707706436,-5.26511162862565,-20.55)) ;
#165261=CARTESIAN_POINT('Origin',(-5.10072415073893,-5.24710339704429,-20.55)) ;
#165262=CARTESIAN_POINT('Origin',(-5.8,-5.42192235935956,-20.55)) ;
#165263=CARTESIAN_POINT('Ctrl Pts',(-5.77574643749636,-5.51893660937409,
-20.55)) ;
#165264=CARTESIAN_POINT('Ctrl Pts',(-5.77574643749636,-5.51893660937409,
-20.65)) ;
#165265=CARTESIAN_POINT('Ctrl Pts',(-5.8,-5.42192235935956,-20.65)) ;
#165266=CARTESIAN_POINT('Ctrl Pts',(-5.79207992677989,-5.52301998169497,
-20.550000000466)) ;
#165267=CARTESIAN_POINT('Ctrl Pts',(-5.78430903206644,-5.5210772580166,
-20.6480386045671)) ;
#165268=CARTESIAN_POINT('Ctrl Pts',(-5.80816665318301,-5.42600568595105,
-20.65)) ;
#165269=CARTESIAN_POINT('Ctrl Pts',(-5.80840777707096,-5.52710194426774,
-20.5520100540957)) ;
#165270=CARTESIAN_POINT('Ctrl Pts',(-5.7934141764523,-5.52335354411309,
-20.6471641501816)) ;
#165271=CARTESIAN_POINT('Ctrl Pts',(-5.81633079157287,-5.43008775511759,
-20.6510050572528)) ;
#165272=CARTESIAN_POINT('Ctrl Pts',(-5.82425356250363,-5.53106339062591,
-20.5559714999709)) ;
#165273=CARTESIAN_POINT('Ctrl Pts',(-5.80269484027818,-5.52567371006955,
-20.6475960694291)) ;
#165274=CARTESIAN_POINT('Ctrl Pts',(-5.82425356250363,-5.43404914061138,
-20.6529857499855)) ;
#165275=CARTESIAN_POINT('Origin',(-5.84850712500726,-5.43404914061138,-20.5559714999709)) ;
#165276=CARTESIAN_POINT('Ctrl Pts',(-5.82426676739356,-5.5310666746717,
-20.5559153963654)) ;
#165277=CARTESIAN_POINT('Ctrl Pts',(-5.80266988778305,-5.52572362329012,
-20.647645966189)) ;
#165278=CARTESIAN_POINT('Ctrl Pts',(-5.82426676352021,-5.43399305345753,
-20.652989033073)) ;
#165279=CARTESIAN_POINT('Ctrl Pts',(-5.83498671931124,-5.53374818244431,
-20.5612758712785)) ;
#165280=CARTESIAN_POINT('Ctrl Pts',(-5.80595263122255,-5.52411754710033,
-20.6460398908368)) ;
#165281=CARTESIAN_POINT('Ctrl Pts',(-5.83498671397632,-5.43935352749395,
-20.6556705400343)) ;
#165282=CARTESIAN_POINT('Ctrl Pts',(-5.84526105845722,-5.53822480044432,
-20.5702256222543)) ;
#165283=CARTESIAN_POINT('Ctrl Pts',(-5.81370932746126,-5.52260133464154,
-20.6445236796681)) ;
#165284=CARTESIAN_POINT('Ctrl Pts',(-5.84526105243727,-5.4483032770705,
-20.660147156823)) ;
#165285=CARTESIAN_POINT('Ctrl Pts',(-5.86378685403706,-5.55027438933182,
-20.5943225636634)) ;
#165286=CARTESIAN_POINT('Ctrl Pts',(-5.83531854275274,-5.52733068552585,
-20.6492530334044)) ;
#165287=CARTESIAN_POINT('Ctrl Pts',(-5.86378684816468,-5.47240021563482,
-20.6721967439586)) ;
#165288=CARTESIAN_POINT('Ctrl Pts',(-5.87203852631585,-5.55784608774614,
-20.6094673107067)) ;
#165289=CARTESIAN_POINT('Ctrl Pts',(-5.84834787930676,-5.53310200486442,
-20.6550243542642)) ;
#165290=CARTESIAN_POINT('Ctrl Pts',(-5.87203852123047,-5.4875449611264,
-20.6797684417942)) ;
#165291=CARTESIAN_POINT('Ctrl Pts',(-5.892427473048,-5.5839719895029,-20.661734382694)) ;
#165292=CARTESIAN_POINT('Ctrl Pts',(-5.88223383300415,-5.56084219746619,
-20.6827645511522)) ;
#165293=CARTESIAN_POINT('Ctrl Pts',(-5.89242747063503,-5.53981202831257,
-20.7058943433874)) ;
#165294=CARTESIAN_POINT('Ctrl Pts',(-5.9,-5.60595824049752,-20.7057331988325)) ;
#165295=CARTESIAN_POINT('Ctrl Pts',(-5.9,-5.59485304775417,-20.7167754043861)) ;
#165296=CARTESIAN_POINT('Ctrl Pts',(-5.9,-5.58381084219988,-20.7278805971145)) ;
#165297=CARTESIAN_POINT('Ctrl Pts',(-5.9,-5.62807764064044,-20.75)) ;
#165298=CARTESIAN_POINT('Ctrl Pts',(-5.9,-5.62807764064044,-20.75)) ;
#165299=CARTESIAN_POINT('Ctrl Pts',(-5.9,-5.62807764064044,-20.75)) ;
#165300=CARTESIAN_POINT('Origin',(7.8,2.1,-19.45)) ;
#165301=CARTESIAN_POINT('Origin',(7.8,2.1,-19.65)) ;
#165302=CARTESIAN_POINT('Origin',(7.6,2.1,-19.45)) ;
#165303=CARTESIAN_POINT('Origin',(7.6,2.1,-19.45)) ;
#165304=CARTESIAN_POINT('Origin',(7.6,2.1,-18.65)) ;
#165305=CARTESIAN_POINT('Origin',(7.8,2.1,-19.65)) ;
#165306=CARTESIAN_POINT('Origin',(9.6,2.1,-19.65)) ;
#165307=CARTESIAN_POINT('Origin',(7.8,2.1,-18.65)) ;
#165308=CARTESIAN_POINT('Origin',(7.8,2.1,-18.45)) ;
#165309=CARTESIAN_POINT('Origin',(9.6,2.1,-19.45)) ;
#165310=CARTESIAN_POINT('Origin',(9.8,2.1,-19.45)) ;
#165311=CARTESIAN_POINT('Origin',(7.8,2.1,-18.45)) ;
#165312=CARTESIAN_POINT('Origin',(9.6,2.1,-18.45)) ;
#165313=CARTESIAN_POINT('Origin',(9.8,2.1,-19.45)) ;
#165314=CARTESIAN_POINT('Origin',(9.8,2.1,-18.65)) ;
#165315=CARTESIAN_POINT('Origin',(9.6,2.1,-18.65)) ;
#165316=CARTESIAN_POINT('Origin',(-4.15,-6.25,-18.3)) ;
#165317=CARTESIAN_POINT('Origin',(-4.15,-6.3,-18.3)) ;
#165318=CARTESIAN_POINT('Origin',(-4.15,-6.3,-19.05)) ;
#165319=CARTESIAN_POINT('Origin',(-4.15,-6.3,-19.8)) ;
#165320=CARTESIAN_POINT('Origin',(-4.15,-6.3,-18.3)) ;
#165321=CARTESIAN_POINT('Origin',(-4.15,-6.25,-19.8)) ;
#165322=CARTESIAN_POINT('Origin',(-4.15,-6.3,-19.8)) ;
#165323=CARTESIAN_POINT('Origin',(-4.15,-6.3,-18.3)) ;
#165324=CARTESIAN_POINT('Origin',(-4.15,-6.3,-18.3)) ;
#165325=CARTESIAN_POINT('Origin',(-4.15,-6.3,-19.8)) ;
#165326=CARTESIAN_POINT('Origin',(-4.15,-6.3,-19.8)) ;
#165327=CARTESIAN_POINT('Origin',(-4.65,-6.25,-18.3)) ;
#165328=CARTESIAN_POINT('Origin',(-4.65,-6.3,-18.3)) ;
#165329=CARTESIAN_POINT('Origin',(0.,-6.3,-18.3)) ;
#165330=CARTESIAN_POINT('Origin',(-4.65,-6.3,-18.3)) ;
#165331=CARTESIAN_POINT('Origin',(0.,-6.3,-19.8)) ;
#165332=CARTESIAN_POINT('Origin',(-4.65,-6.3,-19.8)) ;
#165333=CARTESIAN_POINT('Origin',(-4.65,-6.25,-19.8)) ;
#165334=CARTESIAN_POINT('Origin',(-4.65,-6.3,-19.8)) ;
#165335=CARTESIAN_POINT('Origin',(-4.65,-6.3,-18.3)) ;
#165336=CARTESIAN_POINT('Origin',(-4.65,-6.3,-18.3)) ;
#165337=CARTESIAN_POINT('Origin',(-4.65,-6.3,-19.8)) ;
#165338=CARTESIAN_POINT('Origin',(-4.65,-6.3,-19.8)) ;
#165339=CARTESIAN_POINT('Origin',(-4.65,-6.3,-19.05)) ;
#165340=CARTESIAN_POINT('Origin',(-3.,4.45,-20.15)) ;
#165341=CARTESIAN_POINT('Origin',(-2.1,4.45,-20.15)) ;
#165342=CARTESIAN_POINT('Origin',(-2.9,4.45,-20.15)) ;
#165343=CARTESIAN_POINT('Origin',(-2.9,4.45,-19.95)) ;
#165344=CARTESIAN_POINT('Origin',(-3.1,4.45,-19.95)) ;
#165345=CARTESIAN_POINT('Origin',(-2.9,4.45,-19.95)) ;
#165346=CARTESIAN_POINT('Origin',(-2.1,4.45,-19.95)) ;
#165347=CARTESIAN_POINT('Origin',(-2.1,4.45,-19.95)) ;
#165348=CARTESIAN_POINT('Origin',(-1.9,4.45,-19.95)) ;
#165349=CARTESIAN_POINT('Origin',(-3.1,4.45,-20.05)) ;
#165350=CARTESIAN_POINT('Origin',(-3.1,4.45,-18.15)) ;
#165351=CARTESIAN_POINT('Origin',(-2.9,4.4,-19.95)) ;
#165352=CARTESIAN_POINT('Origin',(-2.9,4.35,-19.95)) ;
#165353=CARTESIAN_POINT('Origin',(-1.95156391047391E-16,4.35,-19.95)) ;
#165354=CARTESIAN_POINT('Origin',(-2.1,4.35,-19.95)) ;
#165355=CARTESIAN_POINT('Origin',(-2.9,4.35,-19.95)) ;
#165356=CARTESIAN_POINT('Origin',(-2.1,4.4,-19.95)) ;
#165357=CARTESIAN_POINT('Origin',(-2.1,4.35,-19.95)) ;
#165358=CARTESIAN_POINT('Origin',(-1.9,4.45,-20.05)) ;
#165359=CARTESIAN_POINT('Origin',(-1.9,4.45,-18.15)) ;
#165360=CARTESIAN_POINT('Origin',(-3.,4.45,-17.95)) ;
#165361=CARTESIAN_POINT('Origin',(-2.9,4.45,-17.95)) ;
#165362=CARTESIAN_POINT('Origin',(-2.1,4.45,-17.95)) ;
#165363=CARTESIAN_POINT('Origin',(-2.9,4.45,-18.15)) ;
#165364=CARTESIAN_POINT('Origin',(-2.9,4.45,-18.15)) ;
#165365=CARTESIAN_POINT('Origin',(-2.9,4.35,-19.95)) ;
#165366=CARTESIAN_POINT('Origin',(-2.9,4.35,-19.95)) ;
#165367=CARTESIAN_POINT('Origin',(-2.1,4.35,-19.95)) ;
#165368=CARTESIAN_POINT('Origin',(-2.1,4.35,-19.95)) ;
#165369=CARTESIAN_POINT('Origin',(-2.1,4.45,-18.15)) ;
#165370=CARTESIAN_POINT('Origin',(-2.1,4.45,-18.15)) ;
#165371=CARTESIAN_POINT('Origin',(-2.9,4.4,-18.15)) ;
#165372=CARTESIAN_POINT('Origin',(-2.9,4.35,-18.15)) ;
#165373=CARTESIAN_POINT('Origin',(-2.9,4.35,-19.05)) ;
#165374=CARTESIAN_POINT('Origin',(-2.9,4.35,-18.15)) ;
#165375=CARTESIAN_POINT('Origin',(-2.1,4.35,-19.05)) ;
#165376=CARTESIAN_POINT('Origin',(-2.1,4.35,-18.15)) ;
#165377=CARTESIAN_POINT('Origin',(-2.1,4.4,-18.15)) ;
#165378=CARTESIAN_POINT('Origin',(-2.1,4.35,-18.15)) ;
#165379=CARTESIAN_POINT('Origin',(-2.9,4.35,-18.15)) ;
#165380=CARTESIAN_POINT('Origin',(-2.9,4.35,-18.15)) ;
#165381=CARTESIAN_POINT('Origin',(-2.1,4.35,-18.15)) ;
#165382=CARTESIAN_POINT('Origin',(-2.1,4.35,-18.15)) ;
#165383=CARTESIAN_POINT('Origin',(-1.95156391047391E-16,4.35,-18.15)) ;
#165384=CARTESIAN_POINT('Origin',(-2.25,4.25,-19.8)) ;
#165385=CARTESIAN_POINT('Origin',(-2.25,4.3,-19.8)) ;
#165386=CARTESIAN_POINT('Origin',(-2.25,4.3,-19.05)) ;
#165387=CARTESIAN_POINT('Origin',(-2.25,4.3,-18.3)) ;
#165388=CARTESIAN_POINT('Origin',(-2.25,4.3,-19.8)) ;
#165389=CARTESIAN_POINT('Origin',(-2.25,4.25,-18.3)) ;
#165390=CARTESIAN_POINT('Origin',(-2.25,4.3,-18.3)) ;
#165391=CARTESIAN_POINT('Origin',(-2.25,4.3,-19.8)) ;
#165392=CARTESIAN_POINT('Origin',(-2.25,4.3,-19.8)) ;
#165393=CARTESIAN_POINT('Origin',(-2.25,4.3,-18.3)) ;
#165394=CARTESIAN_POINT('Origin',(-2.25,4.3,-18.3)) ;
#165395=CARTESIAN_POINT('Origin',(-2.75,4.25,-19.8)) ;
#165396=CARTESIAN_POINT('Origin',(-2.75,4.3,-19.8)) ;
#165397=CARTESIAN_POINT('Origin',(-1.97127667724637E-17,4.3,-19.8)) ;
#165398=CARTESIAN_POINT('Origin',(-2.75,4.3,-19.8)) ;
#165399=CARTESIAN_POINT('Origin',(-1.97127667724637E-17,4.3,-18.3)) ;
#165400=CARTESIAN_POINT('Origin',(-2.75,4.3,-18.3)) ;
#165401=CARTESIAN_POINT('Origin',(-2.75,4.25,-18.3)) ;
#165402=CARTESIAN_POINT('Origin',(-2.75,4.3,-18.3)) ;
#165403=CARTESIAN_POINT('Origin',(-2.75,4.3,-19.8)) ;
#165404=CARTESIAN_POINT('Origin',(-2.75,4.3,-19.8)) ;
#165405=CARTESIAN_POINT('Origin',(-2.75,4.3,-18.3)) ;
#165406=CARTESIAN_POINT('Origin',(-2.75,4.3,-18.3)) ;
#165407=CARTESIAN_POINT('Origin',(-2.75,4.3,-19.05)) ;
#165408=CARTESIAN_POINT('Origin',(7.8,2.9,-19.45)) ;
#165409=CARTESIAN_POINT('Origin',(7.8,2.9,-19.45)) ;
#165410=CARTESIAN_POINT('Origin',(7.8,2.9,-18.65)) ;
#165411=CARTESIAN_POINT('Origin',(7.8,2.9,-18.65)) ;
#165412=CARTESIAN_POINT('Origin',(7.8,2.9,-18.65)) ;
#165413=CARTESIAN_POINT('Origin',(7.8,2.9,-19.45)) ;
#165414=CARTESIAN_POINT('Origin',(7.8,2.9,-19.45)) ;
#165415=CARTESIAN_POINT('Origin',(9.6,2.9,-18.65)) ;
#165416=CARTESIAN_POINT('Origin',(9.6,2.9,-18.65)) ;
#165417=CARTESIAN_POINT('Origin',(9.6,2.9,-19.45)) ;
#165418=CARTESIAN_POINT('Origin',(9.6,2.9,-19.45)) ;
#165419=CARTESIAN_POINT('Origin',(9.6,2.9,-18.65)) ;
#165420=CARTESIAN_POINT('Origin',(9.6,2.9,-18.65)) ;
#165421=CARTESIAN_POINT('Origin',(9.6,2.9,-19.45)) ;
#165422=CARTESIAN_POINT('Origin',(9.6,2.9,-19.45)) ;
#165423=CARTESIAN_POINT('Origin',(9.6,2.9,-19.45)) ;
#165424=CARTESIAN_POINT('Origin',(-0.183301359729408,3.45,-17.532963213524)) ;
#165425=CARTESIAN_POINT('Origin',(0.24923464143508,3.15,-18.9337799780213)) ;
#165426=CARTESIAN_POINT('Origin',(-0.249234641435079,3.15,-19.1662200219787)) ;
#165427=CARTESIAN_POINT('Origin',(-1.04429375741423,3.45,-17.9344505621777)) ;
#165428=CARTESIAN_POINT('Origin',(10.1,-2.15,-21.9568804065906)) ;
#165429=CARTESIAN_POINT('Origin',(10.1,-2.15,-21.9568804065906)) ;
#165430=CARTESIAN_POINT('Origin',(10.1,-2.15,-21.9568804065906)) ;
#165431=CARTESIAN_POINT('Origin',(10.1,-2.15,-21.9568804065906)) ;
#165432=CARTESIAN_POINT('Origin',(10.1,-2.15,-22.86)) ;
#165433=CARTESIAN_POINT('Origin',(10.1,-2.15,-21.555)) ;
#165434=CARTESIAN_POINT('Origin',(10.2,-2.15,-21.9568804065906)) ;
#165435=CARTESIAN_POINT('Origin',(3.7,-2.15,-21.9568804065906)) ;
#165436=CARTESIAN_POINT('Origin',(10.1,-3.65625,-22.86)) ;
#165437=CARTESIAN_POINT('Origin',(10.1,-2.15,-23.7631195934094)) ;
#165438=CARTESIAN_POINT('Origin',(10.1,-3.65625,-21.555)) ;
#165439=CARTESIAN_POINT('Origin',(10.1,1.9,-21.555)) ;
#165440=CARTESIAN_POINT('Origin',(10.1,-2.15,-21.555)) ;
#165441=CARTESIAN_POINT('Origin',(10.1,-2.15,-21.555)) ;
#165442=CARTESIAN_POINT('Origin',(10.1,-2.15,-21.555)) ;
#165443=CARTESIAN_POINT('Origin',(3.7,-2.15,-21.9568804065906)) ;
#165444=CARTESIAN_POINT('Origin',(3.7,-2.32153024911032,-22.0597267659824)) ;
#165445=CARTESIAN_POINT('Origin',(3.7,-2.35,-21.9568804065906)) ;
#165446=CARTESIAN_POINT('Origin',(10.1,-2.15,-23.7631195934094)) ;
#165447=CARTESIAN_POINT('Origin',(10.1,-2.15,-23.7631195934094)) ;
#165448=CARTESIAN_POINT('Origin',(10.1,-2.15,-23.7631195934094)) ;
#165449=CARTESIAN_POINT('Origin',(10.1,1.9,-22.86)) ;
#165450=CARTESIAN_POINT('Origin',(10.1,1.9,-24.165)) ;
#165451=CARTESIAN_POINT('Origin',(10.1,1.9,-21.555)) ;
#165452=CARTESIAN_POINT('Origin',(10.2,-2.15,-21.555)) ;
#165453=CARTESIAN_POINT('Origin',(3.7,-2.15,-21.555)) ;
#165454=CARTESIAN_POINT('Origin',(3.7,-2.35,-21.455)) ;
#165455=CARTESIAN_POINT('Origin',(3.7,-2.35,-21.555)) ;
#165456=CARTESIAN_POINT('Origin',(3.7,-3.65625,-22.86)) ;
#165457=CARTESIAN_POINT('Origin',(3.7,-2.32153024911032,-23.6602732340176)) ;
#165458=CARTESIAN_POINT('Origin',(10.2,-2.15,-23.7631195934094)) ;
#165459=CARTESIAN_POINT('Origin',(3.7,-2.15,-23.7631195934094)) ;
#165460=CARTESIAN_POINT('Origin',(10.1,-2.15,-22.86)) ;
#165461=CARTESIAN_POINT('Origin',(10.1,-2.15,-24.165)) ;
#165462=CARTESIAN_POINT('Origin',(10.1,-3.65625,-24.165)) ;
#165463=CARTESIAN_POINT('Origin',(10.1,1.9,-24.165)) ;
#165464=CARTESIAN_POINT('Origin',(10.1,-2.15,-24.165)) ;
#165465=CARTESIAN_POINT('Origin',(3.7,-2.35,-21.555)) ;
#165466=CARTESIAN_POINT('Origin',(3.5,-2.35,-21.555)) ;
#165467=CARTESIAN_POINT('Origin',(3.7,-2.15,-23.7631195934094)) ;
#165468=CARTESIAN_POINT('Origin',(3.7,-2.35,-23.7631195934094)) ;
#165469=CARTESIAN_POINT('Origin',(10.1,-2.15,-24.165)) ;
#165470=CARTESIAN_POINT('Origin',(10.1,-2.15,-24.165)) ;
#165471=CARTESIAN_POINT('Origin',(3.6,1.9,-21.355)) ;
#165472=CARTESIAN_POINT('Origin',(3.5,1.9,-21.355)) ;
#165473=CARTESIAN_POINT('Origin',(2.7,1.9,-21.355)) ;
#165474=CARTESIAN_POINT('Origin',(3.5,2.01220782770297E-15,-21.555)) ;
#165475=CARTESIAN_POINT('Origin',(3.5,-5.15,-21.555)) ;
#165476=CARTESIAN_POINT('Origin',(3.7,-2.35,-23.735)) ;
#165477=CARTESIAN_POINT('Origin',(3.7,-2.35,-24.165)) ;
#165478=CARTESIAN_POINT('Origin',(3.6,-2.15,-24.165)) ;
#165479=CARTESIAN_POINT('Origin',(3.7,-2.15,-24.165)) ;
#165480=CARTESIAN_POINT('Origin',(2.7,1.9,-21.355)) ;
#165481=CARTESIAN_POINT('Origin',(2.7,1.9,-21.355)) ;
#165482=CARTESIAN_POINT('Origin',(3.5,-5.15,-21.555)) ;
#165483=CARTESIAN_POINT('Origin',(3.5,-5.15,-21.555)) ;
#165484=CARTESIAN_POINT('Origin',(3.5,-5.15,-21.555)) ;
#165485=CARTESIAN_POINT('Origin',(3.7,-2.35,-24.165)) ;
#165486=CARTESIAN_POINT('Origin',(3.5,-2.35,-24.165)) ;
#165487=CARTESIAN_POINT('Origin',(2.7,2.,-21.355)) ;
#165488=CARTESIAN_POINT('Origin',(2.7,-5.15,-21.355)) ;
#165489=CARTESIAN_POINT('Origin',(3.6,-5.15,-21.555)) ;
#165490=CARTESIAN_POINT('Origin',(2.7,-5.15,-21.555)) ;
#165491=CARTESIAN_POINT('Origin',(3.5,-5.15,0.)) ;
#165492=CARTESIAN_POINT('Origin',(3.5,-5.15,-24.165)) ;
#165493=CARTESIAN_POINT('Origin',(3.5,-2.0901141027277E-15,-24.165)) ;
#165494=CARTESIAN_POINT('Origin',(3.5,-5.15,-24.165)) ;
#165495=CARTESIAN_POINT('Origin',(2.7,-5.15,-21.555)) ;
#165496=CARTESIAN_POINT('Origin',(2.7,-5.35,-21.555)) ;
#165497=CARTESIAN_POINT('Origin',(3.5,-5.15,-24.165)) ;
#165498=CARTESIAN_POINT('Origin',(3.5,-5.15,-24.165)) ;
#165499=CARTESIAN_POINT('Origin',(2.7,-5.35,-21.455)) ;
#165500=CARTESIAN_POINT('Origin',(2.7,-5.35,-24.165)) ;
#165501=CARTESIAN_POINT('Origin',(3.6,-5.15,-24.165)) ;
#165502=CARTESIAN_POINT('Origin',(2.7,-5.15,-24.165)) ;
#165503=CARTESIAN_POINT('Origin',(3.6,1.9,-24.365)) ;
#165504=CARTESIAN_POINT('Origin',(3.5,1.9,-24.365)) ;
#165505=CARTESIAN_POINT('Origin',(2.7,1.9,-24.365)) ;
#165506=CARTESIAN_POINT('Origin',(2.7,1.9,-24.265)) ;
#165507=CARTESIAN_POINT('Origin',(2.7,1.9,-25.165)) ;
#165508=CARTESIAN_POINT('Origin',(2.7,1.9,-24.365)) ;
#165509=CARTESIAN_POINT('Origin',(2.7,-5.15,-24.165)) ;
#165510=CARTESIAN_POINT('Origin',(2.7,-5.15,-24.365)) ;
#165511=CARTESIAN_POINT('Origin',(2.7,1.9,-24.365)) ;
#165512=CARTESIAN_POINT('Origin',(2.7,1.9,-24.365)) ;
#165513=CARTESIAN_POINT('Origin',(2.7,-5.25,-24.365)) ;
#165514=CARTESIAN_POINT('Ctrl Pts',(-3.8,-6.55,-21.76)) ;
#165515=CARTESIAN_POINT('Ctrl Pts',(-3.8,-6.55,-21.76)) ;
#165516=CARTESIAN_POINT('Ctrl Pts',(-3.8,-6.55,-21.76)) ;
#165517=CARTESIAN_POINT('Ctrl Pts',(-3.82625343282631,-6.55,-21.8125068656527)) ;
#165518=CARTESIAN_POINT('Ctrl Pts',(-3.83954133268389,-6.55,-21.7995413326847)) ;
#165519=CARTESIAN_POINT('Ctrl Pts',(-3.8525068656527,-6.55,-21.7862534328264)) ;
#165520=CARTESIAN_POINT('Ctrl Pts',(-3.85219871729854,-6.53922263893877,
-21.8643974345971)) ;
#165521=CARTESIAN_POINT('Ctrl Pts',(-3.87914655110976,-6.52362528614071,
-21.83914655111)) ;
#165522=CARTESIAN_POINT('Ctrl Pts',(-3.90439743459708,-6.53922263893874,
-21.8121987172986)) ;
#165523=CARTESIAN_POINT('Ctrl Pts',(-3.87996665852871,-6.5114546977086,
-21.9199333170574)) ;
#165524=CARTESIAN_POINT('Ctrl Pts',(-3.90288380314163,-6.48208554016476,
-21.8628838031415)) ;
#165525=CARTESIAN_POINT('Ctrl Pts',(-3.95993331705742,-6.51145469770861,
-21.8399666585287)) ;
#165526=CARTESIAN_POINT('Ctrl Pts',(-3.88737865704135,-6.5003618540841,
-21.9347573140827)) ;
#165527=CARTESIAN_POINT('Ctrl Pts',(-3.90501307588293,-6.46792722356046,
-21.8650130758829)) ;
#165528=CARTESIAN_POINT('Ctrl Pts',(-3.9747573140827,-6.5003618540841,-21.8473786570414)) ;
#165529=CARTESIAN_POINT('Ctrl Pts',(-3.8973972494609,-6.47617483238892,
-21.9547944989218)) ;
#165530=CARTESIAN_POINT('Ctrl Pts',(-3.9032967435641,-6.45094059868421,
-21.8632967435641)) ;
#165531=CARTESIAN_POINT('Ctrl Pts',(-3.99479449892181,-6.47617483238891,
-21.8573972494609)) ;
#165532=CARTESIAN_POINT('Ctrl Pts',(-3.9,-6.46309229646327,-21.9599999991818)) ;
#165533=CARTESIAN_POINT('Ctrl Pts',(-3.90000730399733,-6.44945650153778,
-21.860007303903)) ;
#165534=CARTESIAN_POINT('Ctrl Pts',(-3.99999999918173,-6.46309229646329,
-21.86)) ;
#165535=CARTESIAN_POINT('Ctrl Pts',(-3.9,-6.45,-21.96)) ;
#165536=CARTESIAN_POINT('Ctrl Pts',(-3.89999999999999,-6.45,-21.86)) ;
#165537=CARTESIAN_POINT('Ctrl Pts',(-4.,-6.45,-21.86)) ;
#165538=CARTESIAN_POINT('Origin',(-4.,-6.45,-21.96)) ;
#165539=CARTESIAN_POINT('Origin',(-4.,-6.4,-21.96)) ;
#165540=CARTESIAN_POINT('Origin',(-4.,-6.35,-21.96)) ;
#165541=CARTESIAN_POINT('Ctrl Pts',(-5.,-6.55,-21.76)) ;
#165542=CARTESIAN_POINT('Ctrl Pts',(-5.,-6.55,-21.76)) ;
#165543=CARTESIAN_POINT('Ctrl Pts',(-5.,-6.55,-21.76)) ;
#165544=CARTESIAN_POINT('Ctrl Pts',(-4.94749313434733,-6.55,-21.7862534328264)) ;
#165545=CARTESIAN_POINT('Ctrl Pts',(-4.9604586673161,-6.55,-21.7995413326849)) ;
#165546=CARTESIAN_POINT('Ctrl Pts',(-4.97374656717362,-6.55,-21.8125068656527)) ;
#165547=CARTESIAN_POINT('Ctrl Pts',(-4.89560256540291,-6.53922263893874,
-21.8121987172986)) ;
#165548=CARTESIAN_POINT('Ctrl Pts',(-4.92085344889023,-6.52362528614071,
-21.83914655111)) ;
#165549=CARTESIAN_POINT('Ctrl Pts',(-4.94780128270146,-6.53922263893877,
-21.8643974345971)) ;
#165550=CARTESIAN_POINT('Ctrl Pts',(-4.84006668294258,-6.51145469770861,
-21.8399666585287)) ;
#165551=CARTESIAN_POINT('Ctrl Pts',(-4.89711619685837,-6.48208554016477,
-21.8628838031415)) ;
#165552=CARTESIAN_POINT('Ctrl Pts',(-4.92003334147129,-6.5114546977086,
-21.9199333170574)) ;
#165553=CARTESIAN_POINT('Ctrl Pts',(-4.82524268591729,-6.5003618540841,
-21.8473786570414)) ;
#165554=CARTESIAN_POINT('Ctrl Pts',(-4.89498692411706,-6.46792722356047,
-21.8650130758829)) ;
#165555=CARTESIAN_POINT('Ctrl Pts',(-4.91262134295865,-6.5003618540841,
-21.9347573140827)) ;
#165556=CARTESIAN_POINT('Ctrl Pts',(-4.80520550107819,-6.47617483238891,
-21.8573972494609)) ;
#165557=CARTESIAN_POINT('Ctrl Pts',(-4.8967032564359,-6.4509405986842,-21.8632967435642)) ;
#165558=CARTESIAN_POINT('Ctrl Pts',(-4.90260275053909,-6.47617483238892,
-21.9547944989218)) ;
#165559=CARTESIAN_POINT('Ctrl Pts',(-4.80000000081823,-6.46309229646328,
-21.86)) ;
#165560=CARTESIAN_POINT('Ctrl Pts',(-4.89999269598372,-6.4494565015457,
-21.8600073039031)) ;
#165561=CARTESIAN_POINT('Ctrl Pts',(-4.9,-6.46309229646328,-21.9599999991818)) ;
#165562=CARTESIAN_POINT('Ctrl Pts',(-4.8,-6.45,-21.86)) ;
#165563=CARTESIAN_POINT('Ctrl Pts',(-4.9,-6.45,-21.86)) ;
#165564=CARTESIAN_POINT('Ctrl Pts',(-4.9,-6.45,-21.96)) ;
#165565=CARTESIAN_POINT('Origin',(-4.8,-6.45,-21.96)) ;
#165566=CARTESIAN_POINT('Origin',(-4.,-6.35,-21.96)) ;
#165567=CARTESIAN_POINT('Origin',(-4.,-6.35,-21.96)) ;
#165568=CARTESIAN_POINT('Origin',(-4.,-6.35,-21.96)) ;
#165569=CARTESIAN_POINT('Ctrl Pts',(-3.8,-6.55,-23.96)) ;
#165570=CARTESIAN_POINT('Ctrl Pts',(-3.8,-6.55,-23.96)) ;
#165571=CARTESIAN_POINT('Ctrl Pts',(-3.8,-6.55,-23.96)) ;
#165572=CARTESIAN_POINT('Ctrl Pts',(-3.85250686565272,-6.55,-23.9337465671736)) ;
#165573=CARTESIAN_POINT('Ctrl Pts',(-3.83954133268377,-6.55,-23.9204586673159)) ;
#165574=CARTESIAN_POINT('Ctrl Pts',(-3.82625343282628,-6.55,-23.9074931343472)) ;
#165575=CARTESIAN_POINT('Ctrl Pts',(-3.90439743459706,-6.53922263893874,
-23.9078012827014)) ;
#165576=CARTESIAN_POINT('Ctrl Pts',(-3.87914655110984,-6.52362528614073,
-23.8808534488902)) ;
#165577=CARTESIAN_POINT('Ctrl Pts',(-3.85219871729855,-6.53922263893876,
-23.8556025654029)) ;
#165578=CARTESIAN_POINT('Ctrl Pts',(-3.95993331705743,-6.51145469770861,
-23.8800333414713)) ;
#165579=CARTESIAN_POINT('Ctrl Pts',(-3.90288380314159,-6.48208554016475,
-23.8571161968584)) ;
#165580=CARTESIAN_POINT('Ctrl Pts',(-3.8799666585287,-6.5114546977086,-23.8000666829426)) ;
#165581=CARTESIAN_POINT('Ctrl Pts',(-3.97475731408271,-6.5003618540841,
-23.8726213429587)) ;
#165582=CARTESIAN_POINT('Ctrl Pts',(-3.90501307588293,-6.46792722356048,
-23.8549869241171)) ;
#165583=CARTESIAN_POINT('Ctrl Pts',(-3.88737865704135,-6.5003618540841,
-23.7852426859173)) ;
#165584=CARTESIAN_POINT('Ctrl Pts',(-3.9947944989218,-6.47617483238891,
-23.8626027505391)) ;
#165585=CARTESIAN_POINT('Ctrl Pts',(-3.9032967435641,-6.4509405986842,-23.8567032564358)) ;
#165586=CARTESIAN_POINT('Ctrl Pts',(-3.89739724946091,-6.47617483238892,
-23.7652055010782)) ;
#165587=CARTESIAN_POINT('Ctrl Pts',(-3.99999999918176,-6.46309229646328,
-23.86)) ;
#165588=CARTESIAN_POINT('Ctrl Pts',(-3.90000730403035,-6.4494565015515,
-23.859992696097)) ;
#165589=CARTESIAN_POINT('Ctrl Pts',(-3.9,-6.46309229646329,-23.7600000008182)) ;
#165590=CARTESIAN_POINT('Ctrl Pts',(-4.,-6.45,-23.86)) ;
#165591=CARTESIAN_POINT('Ctrl Pts',(-3.9,-6.45,-23.86)) ;
#165592=CARTESIAN_POINT('Ctrl Pts',(-3.9,-6.45,-23.76)) ;
#165593=CARTESIAN_POINT('Origin',(-4.,-6.45,-23.76)) ;
#165594=CARTESIAN_POINT('Origin',(-4.8,-6.4,-21.96)) ;
#165595=CARTESIAN_POINT('Origin',(-4.8,-6.35,-21.96)) ;
#165596=CARTESIAN_POINT('Origin',(1.9515639104739E-16,-6.35,-21.96)) ;
#165597=CARTESIAN_POINT('Origin',(-4.8,-6.35,-21.96)) ;
#165598=CARTESIAN_POINT('Origin',(-4.,-6.35,-22.86)) ;
#165599=CARTESIAN_POINT('Origin',(-4.,-6.35,-23.76)) ;
#165600=CARTESIAN_POINT('Origin',(-4.,-6.4,-23.76)) ;
#165601=CARTESIAN_POINT('Origin',(-4.,-6.35,-23.76)) ;
#165602=CARTESIAN_POINT('Origin',(-4.8,-6.35,-21.96)) ;
#165603=CARTESIAN_POINT('Origin',(-4.8,-6.35,-21.96)) ;
#165604=CARTESIAN_POINT('Origin',(-4.,-6.35,-23.76)) ;
#165605=CARTESIAN_POINT('Origin',(-4.,-6.35,-23.76)) ;
#165606=CARTESIAN_POINT('Origin',(-4.8,-6.35,-22.86)) ;
#165607=CARTESIAN_POINT('Origin',(-4.8,-6.35,-23.76)) ;
#165608=CARTESIAN_POINT('Origin',(1.95156391047391E-16,-6.35,-23.76)) ;
#165609=CARTESIAN_POINT('Origin',(-4.8,-6.35,-23.76)) ;
#165610=CARTESIAN_POINT('Origin',(-4.8,-6.35,-23.76)) ;
#165611=CARTESIAN_POINT('Origin',(-4.8,-6.35,-23.76)) ;
#165612=CARTESIAN_POINT('Origin',(-4.8,-6.4,-23.76)) ;
#165613=CARTESIAN_POINT('Origin',(-4.8,-6.45,-23.76)) ;
#165614=CARTESIAN_POINT('Ctrl Pts',(-5.,-6.55,-23.96)) ;
#165615=CARTESIAN_POINT('Ctrl Pts',(-5.,-6.55,-23.96)) ;
#165616=CARTESIAN_POINT('Ctrl Pts',(-5.,-6.55,-23.96)) ;
#165617=CARTESIAN_POINT('Ctrl Pts',(-4.97374656717362,-6.55,-23.9074931343473)) ;
#165618=CARTESIAN_POINT('Ctrl Pts',(-4.96045866731629,-6.55,-23.9204586673159)) ;
#165619=CARTESIAN_POINT('Ctrl Pts',(-4.94749313434732,-6.55,-23.9337465671736)) ;
#165620=CARTESIAN_POINT('Ctrl Pts',(-4.94780128270146,-6.53922263893877,
-23.8556025654029)) ;
#165621=CARTESIAN_POINT('Ctrl Pts',(-4.92085344889012,-6.52362528614073,
-23.8808534488902)) ;
#165622=CARTESIAN_POINT('Ctrl Pts',(-4.89560256540291,-6.53922263893874,
-23.9078012827014)) ;
#165623=CARTESIAN_POINT('Ctrl Pts',(-4.92003334147129,-6.5114546977086,
-23.8000666829426)) ;
#165624=CARTESIAN_POINT('Ctrl Pts',(-4.89711619685843,-6.48208554016475,
-23.8571161968584)) ;
#165625=CARTESIAN_POINT('Ctrl Pts',(-4.84006668294258,-6.51145469770861,
-23.8800333414713)) ;
#165626=CARTESIAN_POINT('Ctrl Pts',(-4.91262134295865,-6.5003618540841,
-23.7852426859173)) ;
#165627=CARTESIAN_POINT('Ctrl Pts',(-4.89498692411706,-6.46792722356048,
-23.8549869241171)) ;
#165628=CARTESIAN_POINT('Ctrl Pts',(-4.82524268591729,-6.5003618540841,
-23.8726213429587)) ;
#165629=CARTESIAN_POINT('Ctrl Pts',(-4.90260275053909,-6.47617483238892,
-23.7652055010782)) ;
#165630=CARTESIAN_POINT('Ctrl Pts',(-4.8967032564359,-6.4509405986842,-23.8567032564358)) ;
#165631=CARTESIAN_POINT('Ctrl Pts',(-4.80520550107819,-6.47617483238891,
-23.8626027505391)) ;
#165632=CARTESIAN_POINT('Ctrl Pts',(-4.9,-6.46309229646329,-23.7600000008182)) ;
#165633=CARTESIAN_POINT('Ctrl Pts',(-4.89999269596496,-6.44945650155343,
-23.859992696097)) ;
#165634=CARTESIAN_POINT('Ctrl Pts',(-4.80000000081823,-6.46309229646328,
-23.86)) ;
#165635=CARTESIAN_POINT('Ctrl Pts',(-4.9,-6.45,-23.76)) ;
#165636=CARTESIAN_POINT('Ctrl Pts',(-4.9,-6.45,-23.86)) ;
#165637=CARTESIAN_POINT('Ctrl Pts',(-4.8,-6.45,-23.86)) ;
#165638=CARTESIAN_POINT('Ctrl Pts',(-5.82426676739348,-5.43399303700622,
-21.2570109659688)) ;
#165639=CARTESIAN_POINT('Ctrl Pts',(-5.80266988778317,-5.52572360682937,
-21.2623540173507)) ;
#165640=CARTESIAN_POINT('Ctrl Pts',(-5.82426676352017,-5.53106667371342,
-21.3540845871828)) ;
#165641=CARTESIAN_POINT('Ctrl Pts',(-5.83498671931114,-5.43935351191918,
-21.2543294581962)) ;
#165642=CARTESIAN_POINT('Ctrl Pts',(-5.80595263122269,-5.52411753147702,
-21.2639600935403)) ;
#165643=CARTESIAN_POINT('Ctrl Pts',(-5.83498671397627,-5.53374818067469,
-21.3487241131463)) ;
#165644=CARTESIAN_POINT('Ctrl Pts',(-5.84526105845709,-5.44830326289501,
-21.2498528401961)) ;
#165645=CARTESIAN_POINT('Ctrl Pts',(-5.81370932746141,-5.52260132030856,
-21.2654763059991)) ;
#165646=CARTESIAN_POINT('Ctrl Pts',(-5.84526105243722,-5.5382247974634,
-21.3397743635698)) ;
#165647=CARTESIAN_POINT('Ctrl Pts',(-5.86378685403696,-5.47240020430408,
-21.2378032513087)) ;
#165648=CARTESIAN_POINT('Ctrl Pts',(-5.83531854275287,-5.52733067404484,
-21.2607469551147)) ;
#165649=CARTESIAN_POINT('Ctrl Pts',(-5.86378684816461,-5.550274384599,-21.3156774250055)) ;
#165650=CARTESIAN_POINT('Ctrl Pts',(-5.87203852631573,-5.48754495134741,
-21.2302315528944)) ;
#165651=CARTESIAN_POINT('Ctrl Pts',(-5.84834787930687,-5.53310199490454,
-21.2549756357761)) ;
#165652=CARTESIAN_POINT('Ctrl Pts',(-5.87203852123041,-5.55784608243458,
-21.300532679514)) ;
#165653=CARTESIAN_POINT('Ctrl Pts',(-5.89242747304799,-5.53981202333458,
-21.2041056511376)) ;
#165654=CARTESIAN_POINT('Ctrl Pts',(-5.88223383300419,-5.56084219179274,
-21.2272354431742)) ;
#165655=CARTESIAN_POINT('Ctrl Pts',(-5.89242747063502,-5.58397198402775,
-21.2482656123278)) ;
#165656=CARTESIAN_POINT('Ctrl Pts',(-5.9,-5.58381083947299,-21.182119400143)) ;
#165657=CARTESIAN_POINT('Ctrl Pts',(-5.9,-5.59485304502619,-21.1932245928863)) ;
#165658=CARTESIAN_POINT('Ctrl Pts',(-5.9,-5.60595823775503,-21.2042667984405)) ;
#165659=CARTESIAN_POINT('Ctrl Pts',(-5.9,-5.62807764064044,-21.16)) ;
#165660=CARTESIAN_POINT('Ctrl Pts',(-5.9,-5.62807764064044,-21.16)) ;
#165661=CARTESIAN_POINT('Ctrl Pts',(-5.9,-5.62807764064044,-21.16)) ;
#165662=CARTESIAN_POINT('Origin',(-5.84850712500726,-5.43404914061138,-21.3540285000291)) ;
#165663=CARTESIAN_POINT('Ctrl Pts',(-5.82425356250363,-5.53106339062591,
-21.3540285000291)) ;
#165664=CARTESIAN_POINT('Ctrl Pts',(-5.80269484027818,-5.52567371006955,
-21.2624039305709)) ;
#165665=CARTESIAN_POINT('Ctrl Pts',(-5.82425356250363,-5.43404914061138,
-21.2570142500145)) ;
#165666=CARTESIAN_POINT('Ctrl Pts',(-5.80840777707096,-5.52710194426774,
-21.3579899459043)) ;
#165667=CARTESIAN_POINT('Ctrl Pts',(-5.79341417645232,-5.52335354411302,
-21.2628358498184)) ;
#165668=CARTESIAN_POINT('Ctrl Pts',(-5.81633079157288,-5.43008775511759,
-21.2589949427472)) ;
#165669=CARTESIAN_POINT('Ctrl Pts',(-5.79207992677988,-5.52301998169497,
-21.359999999534)) ;
#165670=CARTESIAN_POINT('Ctrl Pts',(-5.78430903206641,-5.52107725801669,
-21.2619613954329)) ;
#165671=CARTESIAN_POINT('Ctrl Pts',(-5.808166653183,-5.42600568595106,-21.26)) ;
#165672=CARTESIAN_POINT('Ctrl Pts',(-5.77574643749636,-5.51893660937409,
-21.36)) ;
#165673=CARTESIAN_POINT('Ctrl Pts',(-5.77574643749636,-5.51893660937409,
-21.26)) ;
#165674=CARTESIAN_POINT('Ctrl Pts',(-5.8,-5.42192235935956,-21.26)) ;
#165675=CARTESIAN_POINT('Origin',(-5.8,-5.42192235935956,-21.36)) ;
#165676=CARTESIAN_POINT('Origin',(-5.8066065036801,-5.42357398527959,-21.36)) ;
#165677=CARTESIAN_POINT('Origin',(-5.17275707706437,-5.26511162862565,-21.36)) ;
#165678=CARTESIAN_POINT('Origin',(-5.15068655017073,-5.25959399690224,-21.3705938529089)) ;
#165679=CARTESIAN_POINT('Origin',(-5.17275707706436,-5.26511162862565,-21.36)) ;
#165680=CARTESIAN_POINT('Origin',(-5.17275707706436,-5.26511162862565,-21.36)) ;
#165681=CARTESIAN_POINT('Origin',(-5.17275707706436,-5.26511162862565,-21.36)) ;
#165682=CARTESIAN_POINT('Origin',(-5.17275707706436,-5.05,-21.36)) ;
#165683=CARTESIAN_POINT('Origin',(-5.17275707706436,-1.91866427917294,-21.36)) ;
#165684=CARTESIAN_POINT('Origin',(-3.78014014831103,-3.31128120792626,-22.0284561258016)) ;
#165685=CARTESIAN_POINT('Origin',(-5.17275707706436,-1.91866427917294,-21.36)) ;
#165686=CARTESIAN_POINT('Origin',(-5.17275707706436,-1.91866427917293,-21.36)) ;
#165687=CARTESIAN_POINT('Origin',(-5.17275707706436,-1.91866427917294,-21.36)) ;
#165688=CARTESIAN_POINT('Origin',(-3.97071067811865,-3.12071067811865,-21.36)) ;
#165689=CARTESIAN_POINT('Origin',(-5.8,-1.2914213562373,-21.36)) ;
#165690=CARTESIAN_POINT('Ctrl Pts',(-5.87071067811865,-1.14999999999999,
-21.2307106781187)) ;
#165691=CARTESIAN_POINT('Ctrl Pts',(-5.8471404520791,-1.10285954792089,
-21.2542809041582)) ;
#165692=CARTESIAN_POINT('Ctrl Pts',(-5.87071067811865,-1.07928932188134,
-21.3014213562373)) ;
#165693=CARTESIAN_POINT('Ctrl Pts',(-5.85217562795657,-1.18707010095452,
-21.2492457282807)) ;
#165694=CARTESIAN_POINT('Ctrl Pts',(-5.81261165662081,-1.13738834337931,
-21.2758614719499)) ;
#165695=CARTESIAN_POINT('Ctrl Pts',(-5.83353949671049,-1.1164605032895,
-21.3385925363811)) ;
#165696=CARTESIAN_POINT('Ctrl Pts',(-5.82627077431945,-1.23887980759835,
-21.26)) ;
#165697=CARTESIAN_POINT('Ctrl Pts',(-5.7656678790793,-1.18433212092041,
-21.2771489437127)) ;
#165698=CARTESIAN_POINT('Ctrl Pts',(-5.78190678732229,-1.1680932126777,
-21.3599999994186)) ;
#165699=CARTESIAN_POINT('Ctrl Pts',(-5.8,-1.2914213562373,-21.26)) ;
#165700=CARTESIAN_POINT('Ctrl Pts',(-5.72928932188135,-1.22071067811865,
-21.26)) ;
#165701=CARTESIAN_POINT('Ctrl Pts',(-5.72928932188134,-1.22071067811865,
-21.36)) ;
#165702=CARTESIAN_POINT('Origin',(-5.94142135623731,-1.15,-21.3014213562373)) ;
#165703=CARTESIAN_POINT('Ctrl Pts',(-5.9,-1.00857864376269,-21.16)) ;
#165704=CARTESIAN_POINT('Ctrl Pts',(-5.9,-1.00857864376269,-21.16)) ;
#165705=CARTESIAN_POINT('Ctrl Pts',(-5.9,-1.00857864376269,-21.16)) ;
#165706=CARTESIAN_POINT('Ctrl Pts',(-5.9,-1.06112019240165,-21.1862707743195)) ;
#165707=CARTESIAN_POINT('Ctrl Pts',(-5.9,-1.04860238144602,-21.2000237376826)) ;
#165708=CARTESIAN_POINT('Ctrl Pts',(-5.9,-1.03484941808214,-21.212541548639)) ;
#165709=CARTESIAN_POINT('Ctrl Pts',(-5.88924572828071,-1.11292989904543,
-21.2121756279566)) ;
#165710=CARTESIAN_POINT('Ctrl Pts',(-5.87451700626115,-1.08721613124018,
-21.2386374874767)) ;
#165711=CARTESIAN_POINT('Ctrl Pts',(-5.88924572828062,-1.06075427171937,
-21.2643512552826)) ;
#165712=CARTESIAN_POINT('Ctrl Pts',(-5.87071067811865,-1.14999999999999,
-21.2307106781187)) ;
#165713=CARTESIAN_POINT('Ctrl Pts',(-5.8471404520791,-1.10285954792089,
-21.2542809041582)) ;
#165714=CARTESIAN_POINT('Ctrl Pts',(-5.87071067811865,-1.07928932188134,
-21.3014213562373)) ;
#165715=CARTESIAN_POINT('Ctrl Pts',(-5.87071067811866,-1.14999999999999,
-24.4892893218813)) ;
#165716=CARTESIAN_POINT('Ctrl Pts',(-5.84714045207911,-1.10285954792089,
-24.4657190958418)) ;
#165717=CARTESIAN_POINT('Ctrl Pts',(-5.87071067811866,-1.07928932188134,
-24.4185786437627)) ;
#165718=CARTESIAN_POINT('Ctrl Pts',(-5.8892457282807,-1.11292989904542,
-24.5078243720434)) ;
#165719=CARTESIAN_POINT('Ctrl Pts',(-5.87451700625923,-1.08721613124108,
-24.4813625125218)) ;
#165720=CARTESIAN_POINT('Ctrl Pts',(-5.88924572828062,-1.06075427171937,
-24.4556487447174)) ;
#165721=CARTESIAN_POINT('Ctrl Pts',(-5.9,-1.06112019240159,-24.5337292256804)) ;
#165722=CARTESIAN_POINT('Ctrl Pts',(-5.9,-1.04860238144416,-24.5199762623175)) ;
#165723=CARTESIAN_POINT('Ctrl Pts',(-5.9,-1.03484941808214,-24.507458451361)) ;
#165724=CARTESIAN_POINT('Ctrl Pts',(-5.9,-1.00857864376269,-24.56)) ;
#165725=CARTESIAN_POINT('Ctrl Pts',(-5.9,-1.00857864376269,-24.56)) ;
#165726=CARTESIAN_POINT('Ctrl Pts',(-5.9,-1.00857864376269,-24.56)) ;
#165727=CARTESIAN_POINT('Origin',(-5.94142135623734,-1.14999999999996,-24.4185786437627)) ;
#165728=CARTESIAN_POINT('Ctrl Pts',(-5.8,-1.2914213562373,-24.46)) ;
#165729=CARTESIAN_POINT('Ctrl Pts',(-5.72928932188134,-1.22071067811865,
-24.46)) ;
#165730=CARTESIAN_POINT('Ctrl Pts',(-5.72928932188134,-1.22071067811865,
-24.36)) ;
#165731=CARTESIAN_POINT('Ctrl Pts',(-5.82627077431951,-1.23887980759822,
-24.46)) ;
#165732=CARTESIAN_POINT('Ctrl Pts',(-5.76566787908001,-1.18433212092034,
-24.4428510562871)) ;
#165733=CARTESIAN_POINT('Ctrl Pts',(-5.78190678732243,-1.16809321267757,
-24.3600000005814)) ;
#165734=CARTESIAN_POINT('Ctrl Pts',(-5.85217562795678,-1.18707010095483,
-24.4707542717195)) ;
#165735=CARTESIAN_POINT('Ctrl Pts',(-5.81261165662028,-1.13738834337977,
-24.4441385280509)) ;
#165736=CARTESIAN_POINT('Ctrl Pts',(-5.83353949671032,-1.11646050328967,
-24.3814074636191)) ;
#165737=CARTESIAN_POINT('Ctrl Pts',(-5.87071067811866,-1.14999999999999,
-24.4892893218813)) ;
#165738=CARTESIAN_POINT('Ctrl Pts',(-5.84714045207911,-1.10285954792088,
-24.4657190958418)) ;
#165739=CARTESIAN_POINT('Ctrl Pts',(-5.87071067811866,-1.07928932188133,
-24.4185786437627)) ;
#165740=CARTESIAN_POINT('Origin',(-5.8,-1.29142135623731,-24.36)) ;
#165741=CARTESIAN_POINT('Origin',(-3.59571067811865,-3.49571067811865,-24.36)) ;
#165742=CARTESIAN_POINT('Origin',(-5.17275707706437,-1.91866427917293,-24.36)) ;
#165743=CARTESIAN_POINT('Origin',(-3.09057773798104,-4.00084361825625,-23.36055391724)) ;
#165744=CARTESIAN_POINT('Origin',(-5.17275707706436,-1.91866427917293,-24.36)) ;
#165745=CARTESIAN_POINT('Origin',(-5.17275707706436,-1.91866427917293,-24.36)) ;
#165746=CARTESIAN_POINT('Origin',(-5.17275707706436,-1.91866427917293,-24.36)) ;
#165747=CARTESIAN_POINT('Origin',(-5.17275707706436,-5.05,-24.36)) ;
#165748=CARTESIAN_POINT('Origin',(-5.17275707706436,-5.26511162862565,-24.36)) ;
#165749=CARTESIAN_POINT('Origin',(-3.96111272388873,-4.96220054033175,-23.7784107104757)) ;
#165750=CARTESIAN_POINT('Origin',(-5.17275707706436,-5.26511162862565,-24.36)) ;
#165751=CARTESIAN_POINT('Origin',(-5.17275707706436,-5.26511162862565,-24.36)) ;
#165752=CARTESIAN_POINT('Origin',(-5.17275707706436,-5.26511162862565,-24.36)) ;
#165753=CARTESIAN_POINT('Origin',(-5.10072415073893,-5.24710339704429,-24.36)) ;
#165754=CARTESIAN_POINT('Origin',(-5.8,-5.42192235935956,-24.36)) ;
#165755=CARTESIAN_POINT('Ctrl Pts',(-5.77574643749636,-5.51893660937409,
-24.36)) ;
#165756=CARTESIAN_POINT('Ctrl Pts',(-5.77574643749636,-5.5189366093741,
-24.46)) ;
#165757=CARTESIAN_POINT('Ctrl Pts',(-5.8,-5.42192235935956,-24.46)) ;
#165758=CARTESIAN_POINT('Ctrl Pts',(-5.7920799267799,-5.52301998169498,
-24.360000000466)) ;
#165759=CARTESIAN_POINT('Ctrl Pts',(-5.78430903206646,-5.52107725801652,
-24.4580386045671)) ;
#165760=CARTESIAN_POINT('Ctrl Pts',(-5.80816665318299,-5.42600568595104,
-24.46)) ;
#165761=CARTESIAN_POINT('Ctrl Pts',(-5.80840777707095,-5.52710194426774,
-24.3620100540957)) ;
#165762=CARTESIAN_POINT('Ctrl Pts',(-5.79341417645228,-5.52335354411315,
-24.4571641501816)) ;
#165763=CARTESIAN_POINT('Ctrl Pts',(-5.81633079157289,-5.4300877551176,
-24.4610050572528)) ;
#165764=CARTESIAN_POINT('Ctrl Pts',(-5.82425356250363,-5.53106339062591,
-24.3659714999709)) ;
#165765=CARTESIAN_POINT('Ctrl Pts',(-5.80269484027818,-5.52567371006954,
-24.4575960694291)) ;
#165766=CARTESIAN_POINT('Ctrl Pts',(-5.82425356250363,-5.43404914061138,
-24.4629857499855)) ;
#165767=CARTESIAN_POINT('Origin',(-5.84850712500726,-5.43404914061138,-24.3659714999709)) ;
#165768=CARTESIAN_POINT('Ctrl Pts',(-5.82426676739355,-5.53106667467169,
-24.3659153963654)) ;
#165769=CARTESIAN_POINT('Ctrl Pts',(-5.80266988778311,-5.52572362329009,
-24.4576459661888)) ;
#165770=CARTESIAN_POINT('Ctrl Pts',(-5.82426676352016,-5.43399305345777,
-24.462989033073)) ;
#165771=CARTESIAN_POINT('Ctrl Pts',(-5.83498671931122,-5.5337481824443,
-24.3712758712785)) ;
#165772=CARTESIAN_POINT('Ctrl Pts',(-5.80595263122263,-5.52411754710037,
-24.4560398908365)) ;
#165773=CARTESIAN_POINT('Ctrl Pts',(-5.83498671397625,-5.43935352749418,
-24.4656705400343)) ;
#165774=CARTESIAN_POINT('Ctrl Pts',(-5.8452610584572,-5.53822480044432,
-24.3802256222543)) ;
#165775=CARTESIAN_POINT('Ctrl Pts',(-5.81370932746134,-5.52260133464154,
-24.454523679668)) ;
#165776=CARTESIAN_POINT('Ctrl Pts',(-5.84526105243719,-5.4483032770707,
-24.4701471568229)) ;
#165777=CARTESIAN_POINT('Ctrl Pts',(-5.86378685403706,-5.55027438933182,
-24.4043225636634)) ;
#165778=CARTESIAN_POINT('Ctrl Pts',(-5.83531854275281,-5.52733068552588,
-24.4592530334043)) ;
#165779=CARTESIAN_POINT('Ctrl Pts',(-5.86378684816461,-5.47240021563498,
-24.4821967439585)) ;
#165780=CARTESIAN_POINT('Ctrl Pts',(-5.87203852631583,-5.55784608774613,
-24.4194673107067)) ;
#165781=CARTESIAN_POINT('Ctrl Pts',(-5.84834787930681,-5.53310200486445,
-24.465024354264)) ;
#165782=CARTESIAN_POINT('Ctrl Pts',(-5.87203852123039,-5.48754496112653,
-24.4897684417941)) ;
#165783=CARTESIAN_POINT('Ctrl Pts',(-5.892427473048,-5.58397198950289,-24.471734382694)) ;
#165784=CARTESIAN_POINT('Ctrl Pts',(-5.88223383300416,-5.56084219746623,
-24.4927645511521)) ;
#165785=CARTESIAN_POINT('Ctrl Pts',(-5.892427470635,-5.53981202831264,-24.5158943433873)) ;
#165786=CARTESIAN_POINT('Ctrl Pts',(-5.9,-5.60595824049751,-24.5157331988325)) ;
#165787=CARTESIAN_POINT('Ctrl Pts',(-5.9,-5.59485304775425,-24.5267754043855)) ;
#165788=CARTESIAN_POINT('Ctrl Pts',(-5.9,-5.5838108421999,-24.5378805971145)) ;
#165789=CARTESIAN_POINT('Ctrl Pts',(-5.9,-5.62807764064044,-24.56)) ;
#165790=CARTESIAN_POINT('Ctrl Pts',(-5.9,-5.62807764064044,-24.56)) ;
#165791=CARTESIAN_POINT('Ctrl Pts',(-5.9,-5.62807764064044,-24.56)) ;
#165792=CARTESIAN_POINT('Origin',(7.8,2.1,-23.26)) ;
#165793=CARTESIAN_POINT('Origin',(7.8,2.1,-23.46)) ;
#165794=CARTESIAN_POINT('Origin',(7.6,2.1,-23.26)) ;
#165795=CARTESIAN_POINT('Origin',(7.6,2.1,-23.26)) ;
#165796=CARTESIAN_POINT('Origin',(7.6,2.1,-22.46)) ;
#165797=CARTESIAN_POINT('Origin',(7.8,2.1,-23.46)) ;
#165798=CARTESIAN_POINT('Origin',(9.6,2.1,-23.46)) ;
#165799=CARTESIAN_POINT('Origin',(7.8,2.1,-22.46)) ;
#165800=CARTESIAN_POINT('Origin',(7.8,2.1,-22.26)) ;
#165801=CARTESIAN_POINT('Origin',(9.6,2.1,-23.26)) ;
#165802=CARTESIAN_POINT('Origin',(9.8,2.1,-23.26)) ;
#165803=CARTESIAN_POINT('Origin',(7.8,2.1,-22.26)) ;
#165804=CARTESIAN_POINT('Origin',(9.6,2.1,-22.26)) ;
#165805=CARTESIAN_POINT('Origin',(9.8,2.1,-23.26)) ;
#165806=CARTESIAN_POINT('Origin',(9.8,2.1,-22.46)) ;
#165807=CARTESIAN_POINT('Origin',(9.6,2.1,-22.46)) ;
#165808=CARTESIAN_POINT('Origin',(-4.15,-6.25,-22.11)) ;
#165809=CARTESIAN_POINT('Origin',(-4.15,-6.3,-22.11)) ;
#165810=CARTESIAN_POINT('Origin',(-4.15,-6.3,-22.86)) ;
#165811=CARTESIAN_POINT('Origin',(-4.15,-6.3,-23.61)) ;
#165812=CARTESIAN_POINT('Origin',(-4.15,-6.3,-22.11)) ;
#165813=CARTESIAN_POINT('Origin',(-4.15,-6.25,-23.61)) ;
#165814=CARTESIAN_POINT('Origin',(-4.15,-6.3,-23.61)) ;
#165815=CARTESIAN_POINT('Origin',(-4.15,-6.3,-22.11)) ;
#165816=CARTESIAN_POINT('Origin',(-4.15,-6.3,-22.11)) ;
#165817=CARTESIAN_POINT('Origin',(-4.15,-6.3,-23.61)) ;
#165818=CARTESIAN_POINT('Origin',(-4.15,-6.3,-23.61)) ;
#165819=CARTESIAN_POINT('Origin',(-4.65,-6.25,-22.11)) ;
#165820=CARTESIAN_POINT('Origin',(-4.65,-6.3,-22.11)) ;
#165821=CARTESIAN_POINT('Origin',(0.,-6.3,-22.11)) ;
#165822=CARTESIAN_POINT('Origin',(-4.65,-6.3,-22.11)) ;
#165823=CARTESIAN_POINT('Origin',(0.,-6.3,-23.61)) ;
#165824=CARTESIAN_POINT('Origin',(-4.65,-6.3,-23.61)) ;
#165825=CARTESIAN_POINT('Origin',(-4.65,-6.25,-23.61)) ;
#165826=CARTESIAN_POINT('Origin',(-4.65,-6.3,-23.61)) ;
#165827=CARTESIAN_POINT('Origin',(-4.65,-6.3,-22.11)) ;
#165828=CARTESIAN_POINT('Origin',(-4.65,-6.3,-22.11)) ;
#165829=CARTESIAN_POINT('Origin',(-4.65,-6.3,-23.61)) ;
#165830=CARTESIAN_POINT('Origin',(-4.65,-6.3,-23.61)) ;
#165831=CARTESIAN_POINT('Origin',(-4.65,-6.3,-22.86)) ;
#165832=CARTESIAN_POINT('Origin',(-3.,4.45,-23.96)) ;
#165833=CARTESIAN_POINT('Origin',(-2.1,4.45,-23.96)) ;
#165834=CARTESIAN_POINT('Origin',(-2.9,4.45,-23.96)) ;
#165835=CARTESIAN_POINT('Origin',(-2.9,4.45,-23.76)) ;
#165836=CARTESIAN_POINT('Origin',(-3.1,4.45,-23.76)) ;
#165837=CARTESIAN_POINT('Origin',(-2.9,4.45,-23.76)) ;
#165838=CARTESIAN_POINT('Origin',(-2.1,4.45,-23.76)) ;
#165839=CARTESIAN_POINT('Origin',(-2.1,4.45,-23.76)) ;
#165840=CARTESIAN_POINT('Origin',(-1.9,4.45,-23.76)) ;
#165841=CARTESIAN_POINT('Origin',(-3.1,4.45,-23.86)) ;
#165842=CARTESIAN_POINT('Origin',(-3.1,4.45,-21.96)) ;
#165843=CARTESIAN_POINT('Origin',(-2.9,4.4,-23.76)) ;
#165844=CARTESIAN_POINT('Origin',(-2.9,4.35,-23.76)) ;
#165845=CARTESIAN_POINT('Origin',(-1.95156391047391E-16,4.35,-23.76)) ;
#165846=CARTESIAN_POINT('Origin',(-2.1,4.35,-23.76)) ;
#165847=CARTESIAN_POINT('Origin',(-2.9,4.35,-23.76)) ;
#165848=CARTESIAN_POINT('Origin',(-2.1,4.4,-23.76)) ;
#165849=CARTESIAN_POINT('Origin',(-2.1,4.35,-23.76)) ;
#165850=CARTESIAN_POINT('Origin',(-1.9,4.45,-23.86)) ;
#165851=CARTESIAN_POINT('Origin',(-1.9,4.45,-21.96)) ;
#165852=CARTESIAN_POINT('Origin',(-3.,4.45,-21.76)) ;
#165853=CARTESIAN_POINT('Origin',(-2.9,4.45,-21.76)) ;
#165854=CARTESIAN_POINT('Origin',(-2.1,4.45,-21.76)) ;
#165855=CARTESIAN_POINT('Origin',(-2.9,4.45,-21.96)) ;
#165856=CARTESIAN_POINT('Origin',(-2.9,4.45,-21.96)) ;
#165857=CARTESIAN_POINT('Origin',(-2.9,4.35,-23.76)) ;
#165858=CARTESIAN_POINT('Origin',(-2.9,4.35,-23.76)) ;
#165859=CARTESIAN_POINT('Origin',(-2.1,4.35,-23.76)) ;
#165860=CARTESIAN_POINT('Origin',(-2.1,4.35,-23.76)) ;
#165861=CARTESIAN_POINT('Origin',(-2.1,4.45,-21.96)) ;
#165862=CARTESIAN_POINT('Origin',(-2.1,4.45,-21.96)) ;
#165863=CARTESIAN_POINT('Origin',(-2.9,4.4,-21.96)) ;
#165864=CARTESIAN_POINT('Origin',(-2.9,4.35,-21.96)) ;
#165865=CARTESIAN_POINT('Origin',(-2.9,4.35,-22.86)) ;
#165866=CARTESIAN_POINT('Origin',(-2.9,4.35,-21.96)) ;
#165867=CARTESIAN_POINT('Origin',(-2.1,4.35,-22.86)) ;
#165868=CARTESIAN_POINT('Origin',(-2.1,4.35,-21.96)) ;
#165869=CARTESIAN_POINT('Origin',(-2.1,4.4,-21.96)) ;
#165870=CARTESIAN_POINT('Origin',(-2.1,4.35,-21.96)) ;
#165871=CARTESIAN_POINT('Origin',(-2.9,4.35,-21.96)) ;
#165872=CARTESIAN_POINT('Origin',(-2.9,4.35,-21.96)) ;
#165873=CARTESIAN_POINT('Origin',(-2.1,4.35,-21.96)) ;
#165874=CARTESIAN_POINT('Origin',(-2.1,4.35,-21.96)) ;
#165875=CARTESIAN_POINT('Origin',(-1.95156391047391E-16,4.35,-21.96)) ;
#165876=CARTESIAN_POINT('Origin',(-2.25,4.25,-23.61)) ;
#165877=CARTESIAN_POINT('Origin',(-2.25,4.3,-23.61)) ;
#165878=CARTESIAN_POINT('Origin',(-2.25,4.3,-22.86)) ;
#165879=CARTESIAN_POINT('Origin',(-2.25,4.3,-22.11)) ;
#165880=CARTESIAN_POINT('Origin',(-2.25,4.3,-23.61)) ;
#165881=CARTESIAN_POINT('Origin',(-2.25,4.25,-22.11)) ;
#165882=CARTESIAN_POINT('Origin',(-2.25,4.3,-22.11)) ;
#165883=CARTESIAN_POINT('Origin',(-2.25,4.3,-23.61)) ;
#165884=CARTESIAN_POINT('Origin',(-2.25,4.3,-23.61)) ;
#165885=CARTESIAN_POINT('Origin',(-2.25,4.3,-22.11)) ;
#165886=CARTESIAN_POINT('Origin',(-2.25,4.3,-22.11)) ;
#165887=CARTESIAN_POINT('Origin',(-2.75,4.25,-23.61)) ;
#165888=CARTESIAN_POINT('Origin',(-2.75,4.3,-23.61)) ;
#165889=CARTESIAN_POINT('Origin',(-1.97127667724637E-17,4.3,-23.61)) ;
#165890=CARTESIAN_POINT('Origin',(-2.75,4.3,-23.61)) ;
#165891=CARTESIAN_POINT('Origin',(-1.97127667724637E-17,4.3,-22.11)) ;
#165892=CARTESIAN_POINT('Origin',(-2.75,4.3,-22.11)) ;
#165893=CARTESIAN_POINT('Origin',(-2.75,4.25,-22.11)) ;
#165894=CARTESIAN_POINT('Origin',(-2.75,4.3,-22.11)) ;
#165895=CARTESIAN_POINT('Origin',(-2.75,4.3,-23.61)) ;
#165896=CARTESIAN_POINT('Origin',(-2.75,4.3,-23.61)) ;
#165897=CARTESIAN_POINT('Origin',(-2.75,4.3,-22.11)) ;
#165898=CARTESIAN_POINT('Origin',(-2.75,4.3,-22.11)) ;
#165899=CARTESIAN_POINT('Origin',(-2.75,4.3,-22.86)) ;
#165900=CARTESIAN_POINT('Origin',(7.8,2.9,-23.26)) ;
#165901=CARTESIAN_POINT('Origin',(7.8,2.9,-23.26)) ;
#165902=CARTESIAN_POINT('Origin',(7.8,2.9,-22.46)) ;
#165903=CARTESIAN_POINT('Origin',(7.8,2.9,-22.46)) ;
#165904=CARTESIAN_POINT('Origin',(7.8,2.9,-22.46)) ;
#165905=CARTESIAN_POINT('Origin',(7.8,2.9,-23.26)) ;
#165906=CARTESIAN_POINT('Origin',(7.8,2.9,-23.26)) ;
#165907=CARTESIAN_POINT('Origin',(9.6,2.9,-22.46)) ;
#165908=CARTESIAN_POINT('Origin',(9.6,2.9,-22.46)) ;
#165909=CARTESIAN_POINT('Origin',(9.6,2.9,-23.26)) ;
#165910=CARTESIAN_POINT('Origin',(9.6,2.9,-23.26)) ;
#165911=CARTESIAN_POINT('Origin',(9.6,2.9,-22.46)) ;
#165912=CARTESIAN_POINT('Origin',(9.6,2.9,-22.46)) ;
#165913=CARTESIAN_POINT('Origin',(9.6,2.9,-23.26)) ;
#165914=CARTESIAN_POINT('Origin',(9.6,2.9,-23.26)) ;
#165915=CARTESIAN_POINT('Origin',(9.6,2.9,-23.26)) ;
#165916=CARTESIAN_POINT('Origin',(-0.183301359729408,3.45,-21.342963213524)) ;
#165917=CARTESIAN_POINT('Origin',(0.24923464143508,3.15,-22.7437799780213)) ;
#165918=CARTESIAN_POINT('Origin',(-0.249234641435079,3.15,-22.9762200219787)) ;
#165919=CARTESIAN_POINT('Origin',(-1.04429375741423,3.45,-21.7444505621777)) ;
#165920=CARTESIAN_POINT('Origin',(10.1,-2.15,-25.7668804065906)) ;
#165921=CARTESIAN_POINT('Origin',(10.1,-2.15,-25.7668804065906)) ;
#165922=CARTESIAN_POINT('Origin',(10.1,-2.15,-25.7668804065906)) ;
#165923=CARTESIAN_POINT('Origin',(10.1,-2.15,-25.7668804065906)) ;
#165924=CARTESIAN_POINT('Origin',(10.1,-2.15,-26.67)) ;
#165925=CARTESIAN_POINT('Origin',(10.1,-2.15,-25.365)) ;
#165926=CARTESIAN_POINT('Origin',(10.2,-2.15,-25.7668804065906)) ;
#165927=CARTESIAN_POINT('Origin',(3.7,-2.15,-25.7668804065906)) ;
#165928=CARTESIAN_POINT('Origin',(10.1,-3.65625,-26.67)) ;
#165929=CARTESIAN_POINT('Origin',(10.1,-2.15,-27.5731195934094)) ;
#165930=CARTESIAN_POINT('Origin',(10.1,-3.65625,-25.365)) ;
#165931=CARTESIAN_POINT('Origin',(10.1,1.9,-25.365)) ;
#165932=CARTESIAN_POINT('Origin',(10.1,-2.15,-25.365)) ;
#165933=CARTESIAN_POINT('Origin',(10.1,-2.15,-25.365)) ;
#165934=CARTESIAN_POINT('Origin',(10.1,-2.15,-25.365)) ;
#165935=CARTESIAN_POINT('Origin',(3.7,-2.15,-25.7668804065906)) ;
#165936=CARTESIAN_POINT('Origin',(3.7,-2.32153024911032,-25.8697267659824)) ;
#165937=CARTESIAN_POINT('Origin',(3.7,-2.35,-25.7668804065906)) ;
#165938=CARTESIAN_POINT('Origin',(10.1,-2.15,-27.5731195934094)) ;
#165939=CARTESIAN_POINT('Origin',(10.1,-2.15,-27.5731195934094)) ;
#165940=CARTESIAN_POINT('Origin',(10.1,-2.15,-27.5731195934094)) ;
#165941=CARTESIAN_POINT('Origin',(10.1,1.9,-26.67)) ;
#165942=CARTESIAN_POINT('Origin',(10.1,1.9,-27.975)) ;
#165943=CARTESIAN_POINT('Origin',(10.1,1.9,-25.365)) ;
#165944=CARTESIAN_POINT('Origin',(10.2,-2.15,-25.365)) ;
#165945=CARTESIAN_POINT('Origin',(3.7,-2.15,-25.365)) ;
#165946=CARTESIAN_POINT('Origin',(3.7,-2.35,-25.265)) ;
#165947=CARTESIAN_POINT('Origin',(3.7,-2.35,-25.365)) ;
#165948=CARTESIAN_POINT('Origin',(3.7,-3.65625,-26.67)) ;
#165949=CARTESIAN_POINT('Origin',(3.7,-2.32153024911032,-27.4702732340176)) ;
#165950=CARTESIAN_POINT('Origin',(10.2,-2.15,-27.5731195934094)) ;
#165951=CARTESIAN_POINT('Origin',(3.7,-2.15,-27.5731195934094)) ;
#165952=CARTESIAN_POINT('Origin',(10.1,-2.15,-26.67)) ;
#165953=CARTESIAN_POINT('Origin',(10.1,-2.15,-27.975)) ;
#165954=CARTESIAN_POINT('Origin',(10.1,-3.65625,-27.975)) ;
#165955=CARTESIAN_POINT('Origin',(10.1,1.9,-27.975)) ;
#165956=CARTESIAN_POINT('Origin',(10.1,-2.15,-27.975)) ;
#165957=CARTESIAN_POINT('Origin',(3.7,-2.35,-25.365)) ;
#165958=CARTESIAN_POINT('Origin',(3.5,-2.35,-25.365)) ;
#165959=CARTESIAN_POINT('Origin',(3.7,-2.15,-27.5731195934094)) ;
#165960=CARTESIAN_POINT('Origin',(3.7,-2.35,-27.5731195934094)) ;
#165961=CARTESIAN_POINT('Origin',(10.1,-2.15,-27.975)) ;
#165962=CARTESIAN_POINT('Origin',(10.1,-2.15,-27.975)) ;
#165963=CARTESIAN_POINT('Origin',(3.6,1.9,-25.165)) ;
#165964=CARTESIAN_POINT('Origin',(3.5,1.9,-25.165)) ;
#165965=CARTESIAN_POINT('Origin',(2.7,1.9,-25.165)) ;
#165966=CARTESIAN_POINT('Origin',(3.5,2.3540679885722E-15,-25.365)) ;
#165967=CARTESIAN_POINT('Origin',(3.5,-5.15,-25.365)) ;
#165968=CARTESIAN_POINT('Origin',(3.7,-2.35,-27.545)) ;
#165969=CARTESIAN_POINT('Origin',(3.7,-2.35,-27.975)) ;
#165970=CARTESIAN_POINT('Origin',(3.6,-2.15,-27.975)) ;
#165971=CARTESIAN_POINT('Origin',(3.7,-2.15,-27.975)) ;
#165972=CARTESIAN_POINT('Origin',(2.7,1.9,-25.165)) ;
#165973=CARTESIAN_POINT('Origin',(2.7,1.9,-25.165)) ;
#165974=CARTESIAN_POINT('Origin',(3.5,-5.15,-25.365)) ;
#165975=CARTESIAN_POINT('Origin',(3.5,-5.15,-25.365)) ;
#165976=CARTESIAN_POINT('Origin',(3.5,-5.15,-25.365)) ;
#165977=CARTESIAN_POINT('Origin',(3.7,-2.35,-27.975)) ;
#165978=CARTESIAN_POINT('Origin',(3.5,-2.35,-27.975)) ;
#165979=CARTESIAN_POINT('Origin',(2.7,2.,-25.165)) ;
#165980=CARTESIAN_POINT('Origin',(2.7,-5.15,-25.165)) ;
#165981=CARTESIAN_POINT('Origin',(3.6,-5.15,-25.365)) ;
#165982=CARTESIAN_POINT('Origin',(2.7,-5.15,-25.365)) ;
#165983=CARTESIAN_POINT('Origin',(3.5,-5.15,0.)) ;
#165984=CARTESIAN_POINT('Origin',(3.5,-5.15,-27.975)) ;
#165985=CARTESIAN_POINT('Origin',(3.5,-2.43197426359692E-15,-27.975)) ;
#165986=CARTESIAN_POINT('Origin',(3.5,-5.15,-27.975)) ;
#165987=CARTESIAN_POINT('Origin',(2.7,-5.15,-25.365)) ;
#165988=CARTESIAN_POINT('Origin',(2.7,-5.35,-25.365)) ;
#165989=CARTESIAN_POINT('Origin',(3.5,-5.15,-27.975)) ;
#165990=CARTESIAN_POINT('Origin',(3.5,-5.15,-27.975)) ;
#165991=CARTESIAN_POINT('Origin',(2.7,-5.35,-25.265)) ;
#165992=CARTESIAN_POINT('Origin',(2.7,-5.35,-27.975)) ;
#165993=CARTESIAN_POINT('Origin',(3.6,-5.15,-27.975)) ;
#165994=CARTESIAN_POINT('Origin',(2.7,-5.15,-27.975)) ;
#165995=CARTESIAN_POINT('Origin',(3.6,1.9,-28.175)) ;
#165996=CARTESIAN_POINT('Origin',(3.5,1.9,-28.175)) ;
#165997=CARTESIAN_POINT('Origin',(2.7,1.9,-28.175)) ;
#165998=CARTESIAN_POINT('Origin',(2.7,1.9,-28.075)) ;
#165999=CARTESIAN_POINT('Origin',(2.7,1.9,-28.975)) ;
#166000=CARTESIAN_POINT('Origin',(2.7,1.9,-28.175)) ;
#166001=CARTESIAN_POINT('Origin',(2.7,-5.15,-27.975)) ;
#166002=CARTESIAN_POINT('Origin',(2.7,-5.15,-28.175)) ;
#166003=CARTESIAN_POINT('Origin',(2.7,1.9,-28.175)) ;
#166004=CARTESIAN_POINT('Origin',(2.7,1.9,-28.175)) ;
#166005=CARTESIAN_POINT('Origin',(2.7,-5.25,-28.175)) ;
#166006=CARTESIAN_POINT('Ctrl Pts',(-3.8,-6.55,-25.57)) ;
#166007=CARTESIAN_POINT('Ctrl Pts',(-3.8,-6.55,-25.57)) ;
#166008=CARTESIAN_POINT('Ctrl Pts',(-3.8,-6.55,-25.57)) ;
#166009=CARTESIAN_POINT('Ctrl Pts',(-3.82625343282631,-6.55,-25.6225068656527)) ;
#166010=CARTESIAN_POINT('Ctrl Pts',(-3.83954133268378,-6.55,-25.6095413326839)) ;
#166011=CARTESIAN_POINT('Ctrl Pts',(-3.85250686565271,-6.55,-25.5962534328264)) ;
#166012=CARTESIAN_POINT('Ctrl Pts',(-3.85219871729854,-6.53922263893877,
-25.6743974345971)) ;
#166013=CARTESIAN_POINT('Ctrl Pts',(-3.87914655110981,-6.52362528614074,
-25.6491465511099)) ;
#166014=CARTESIAN_POINT('Ctrl Pts',(-3.90439743459708,-6.53922263893874,
-25.6221987172986)) ;
#166015=CARTESIAN_POINT('Ctrl Pts',(-3.87996665852871,-6.5114546977086,
-25.7299333170574)) ;
#166016=CARTESIAN_POINT('Ctrl Pts',(-3.90288380314161,-6.48208554016475,
-25.6728838031416)) ;
#166017=CARTESIAN_POINT('Ctrl Pts',(-3.95993331705742,-6.51145469770861,
-25.6499666585287)) ;
#166018=CARTESIAN_POINT('Ctrl Pts',(-3.88737865704135,-6.5003618540841,
-25.7447573140827)) ;
#166019=CARTESIAN_POINT('Ctrl Pts',(-3.90501307588296,-6.46792722356047,
-25.6750130758829)) ;
#166020=CARTESIAN_POINT('Ctrl Pts',(-3.9747573140827,-6.5003618540841,-25.6573786570413)) ;
#166021=CARTESIAN_POINT('Ctrl Pts',(-3.8973972494609,-6.47617483238892,
-25.7647944989218)) ;
#166022=CARTESIAN_POINT('Ctrl Pts',(-3.90329674356407,-6.4509405986842,
-25.6732967435641)) ;
#166023=CARTESIAN_POINT('Ctrl Pts',(-3.99479449892181,-6.47617483238891,
-25.6673972494609)) ;
#166024=CARTESIAN_POINT('Ctrl Pts',(-3.9,-6.46309229646327,-25.7699999991818)) ;
#166025=CARTESIAN_POINT('Ctrl Pts',(-3.90000730395982,-6.44945650152231,
-25.6700073039032)) ;
#166026=CARTESIAN_POINT('Ctrl Pts',(-3.99999999918173,-6.46309229646329,
-25.67)) ;
#166027=CARTESIAN_POINT('Ctrl Pts',(-3.9,-6.45,-25.77)) ;
#166028=CARTESIAN_POINT('Ctrl Pts',(-3.9,-6.45,-25.67)) ;
#166029=CARTESIAN_POINT('Ctrl Pts',(-4.,-6.45,-25.67)) ;
#166030=CARTESIAN_POINT('Origin',(-4.,-6.45,-25.77)) ;
#166031=CARTESIAN_POINT('Origin',(-4.,-6.4,-25.77)) ;
#166032=CARTESIAN_POINT('Origin',(-4.,-6.35,-25.77)) ;
#166033=CARTESIAN_POINT('Ctrl Pts',(-5.,-6.55,-25.57)) ;
#166034=CARTESIAN_POINT('Ctrl Pts',(-5.,-6.55,-25.57)) ;
#166035=CARTESIAN_POINT('Ctrl Pts',(-5.,-6.55,-25.57)) ;
#166036=CARTESIAN_POINT('Ctrl Pts',(-4.94749313434733,-6.55,-25.5962534328264)) ;
#166037=CARTESIAN_POINT('Ctrl Pts',(-4.96045866731621,-6.55,-25.609541332684)) ;
#166038=CARTESIAN_POINT('Ctrl Pts',(-4.97374656717362,-6.55,-25.6225068656527)) ;
#166039=CARTESIAN_POINT('Ctrl Pts',(-4.89560256540291,-6.53922263893874,
-25.6221987172986)) ;
#166040=CARTESIAN_POINT('Ctrl Pts',(-4.92085344889017,-6.52362528614074,
-25.6491465511099)) ;
#166041=CARTESIAN_POINT('Ctrl Pts',(-4.94780128270146,-6.53922263893877,
-25.6743974345971)) ;
#166042=CARTESIAN_POINT('Ctrl Pts',(-4.84006668294258,-6.51145469770861,
-25.6499666585287)) ;
#166043=CARTESIAN_POINT('Ctrl Pts',(-4.8971161968584,-6.48208554016475,
-25.6728838031416)) ;
#166044=CARTESIAN_POINT('Ctrl Pts',(-4.92003334147129,-6.5114546977086,
-25.7299333170574)) ;
#166045=CARTESIAN_POINT('Ctrl Pts',(-4.82524268591729,-6.5003618540841,
-25.6573786570413)) ;
#166046=CARTESIAN_POINT('Ctrl Pts',(-4.89498692411703,-6.46792722356048,
-25.6750130758829)) ;
#166047=CARTESIAN_POINT('Ctrl Pts',(-4.91262134295865,-6.5003618540841,
-25.7447573140827)) ;
#166048=CARTESIAN_POINT('Ctrl Pts',(-4.80520550107819,-6.47617483238891,
-25.6673972494609)) ;
#166049=CARTESIAN_POINT('Ctrl Pts',(-4.89670325643594,-6.45094059868419,
-25.6732967435642)) ;
#166050=CARTESIAN_POINT('Ctrl Pts',(-4.90260275053909,-6.47617483238892,
-25.7647944989218)) ;
#166051=CARTESIAN_POINT('Ctrl Pts',(-4.80000000081823,-6.46309229646328,
-25.67)) ;
#166052=CARTESIAN_POINT('Ctrl Pts',(-4.89999269602123,-6.44945650153022,
-25.6700073039033)) ;
#166053=CARTESIAN_POINT('Ctrl Pts',(-4.9,-6.46309229646329,-25.7699999991818)) ;
#166054=CARTESIAN_POINT('Ctrl Pts',(-4.8,-6.45,-25.67)) ;
#166055=CARTESIAN_POINT('Ctrl Pts',(-4.9,-6.45,-25.67)) ;
#166056=CARTESIAN_POINT('Ctrl Pts',(-4.9,-6.45,-25.77)) ;
#166057=CARTESIAN_POINT('Origin',(-4.8,-6.45,-25.77)) ;
#166058=CARTESIAN_POINT('Origin',(-4.,-6.35,-25.77)) ;
#166059=CARTESIAN_POINT('Origin',(-4.,-6.35,-25.77)) ;
#166060=CARTESIAN_POINT('Origin',(-4.,-6.35,-25.77)) ;
#166061=CARTESIAN_POINT('Ctrl Pts',(-3.8,-6.55,-27.77)) ;
#166062=CARTESIAN_POINT('Ctrl Pts',(-3.8,-6.55,-27.77)) ;
#166063=CARTESIAN_POINT('Ctrl Pts',(-3.8,-6.55,-27.77)) ;
#166064=CARTESIAN_POINT('Ctrl Pts',(-3.85250686565272,-6.55,-27.7437465671736)) ;
#166065=CARTESIAN_POINT('Ctrl Pts',(-3.83954133268385,-6.55,-27.7304586673161)) ;
#166066=CARTESIAN_POINT('Ctrl Pts',(-3.82625343282628,-6.55,-27.7174931343473)) ;
#166067=CARTESIAN_POINT('Ctrl Pts',(-3.90439743459706,-6.53922263893874,
-27.7178012827014)) ;
#166068=CARTESIAN_POINT('Ctrl Pts',(-3.87914655110978,-6.52362528614071,
-27.6908534488901)) ;
#166069=CARTESIAN_POINT('Ctrl Pts',(-3.85219871729855,-6.53922263893876,
-27.6656025654029)) ;
#166070=CARTESIAN_POINT('Ctrl Pts',(-3.95993331705743,-6.51145469770861,
-27.6900333414713)) ;
#166071=CARTESIAN_POINT('Ctrl Pts',(-3.90288380314162,-6.48208554016476,
-27.6671161968584)) ;
#166072=CARTESIAN_POINT('Ctrl Pts',(-3.8799666585287,-6.5114546977086,-27.6100666829426)) ;
#166073=CARTESIAN_POINT('Ctrl Pts',(-3.97475731408271,-6.5003618540841,
-27.6826213429587)) ;
#166074=CARTESIAN_POINT('Ctrl Pts',(-3.90501307588297,-6.46792722356048,
-27.6649869241171)) ;
#166075=CARTESIAN_POINT('Ctrl Pts',(-3.88737865704135,-6.5003618540841,
-27.5952426859173)) ;
#166076=CARTESIAN_POINT('Ctrl Pts',(-3.9947944989218,-6.47617483238891,
-27.6726027505391)) ;
#166077=CARTESIAN_POINT('Ctrl Pts',(-3.90329674356406,-6.45094059868419,
-27.6667032564358)) ;
#166078=CARTESIAN_POINT('Ctrl Pts',(-3.89739724946091,-6.47617483238892,
-27.5752055010782)) ;
#166079=CARTESIAN_POINT('Ctrl Pts',(-3.99999999918176,-6.46309229646328,
-27.67)) ;
#166080=CARTESIAN_POINT('Ctrl Pts',(-3.90000730395532,-6.44945650152054,
-27.6699926960965)) ;
#166081=CARTESIAN_POINT('Ctrl Pts',(-3.9,-6.46309229646329,-27.5700000008182)) ;
#166082=CARTESIAN_POINT('Ctrl Pts',(-4.,-6.45,-27.67)) ;
#166083=CARTESIAN_POINT('Ctrl Pts',(-3.9,-6.45,-27.67)) ;
#166084=CARTESIAN_POINT('Ctrl Pts',(-3.9,-6.45,-27.57)) ;
#166085=CARTESIAN_POINT('Origin',(-4.,-6.45,-27.57)) ;
#166086=CARTESIAN_POINT('Origin',(-4.8,-6.4,-25.77)) ;
#166087=CARTESIAN_POINT('Origin',(-4.8,-6.35,-25.77)) ;
#166088=CARTESIAN_POINT('Origin',(1.9515639104739E-16,-6.35,-25.77)) ;
#166089=CARTESIAN_POINT('Origin',(-4.8,-6.35,-25.77)) ;
#166090=CARTESIAN_POINT('Origin',(-4.,-6.35,-26.67)) ;
#166091=CARTESIAN_POINT('Origin',(-4.,-6.35,-27.57)) ;
#166092=CARTESIAN_POINT('Origin',(-4.,-6.4,-27.57)) ;
#166093=CARTESIAN_POINT('Origin',(-4.,-6.35,-27.57)) ;
#166094=CARTESIAN_POINT('Origin',(-4.8,-6.35,-25.77)) ;
#166095=CARTESIAN_POINT('Origin',(-4.8,-6.35,-25.77)) ;
#166096=CARTESIAN_POINT('Origin',(-4.,-6.35,-27.57)) ;
#166097=CARTESIAN_POINT('Origin',(-4.,-6.35,-27.57)) ;
#166098=CARTESIAN_POINT('Origin',(-4.8,-6.35,-26.67)) ;
#166099=CARTESIAN_POINT('Origin',(-4.8,-6.35,-27.57)) ;
#166100=CARTESIAN_POINT('Origin',(1.95156391047391E-16,-6.35,-27.57)) ;
#166101=CARTESIAN_POINT('Origin',(-4.8,-6.35,-27.57)) ;
#166102=CARTESIAN_POINT('Origin',(-4.8,-6.35,-27.57)) ;
#166103=CARTESIAN_POINT('Origin',(-4.8,-6.35,-27.57)) ;
#166104=CARTESIAN_POINT('Origin',(-4.8,-6.4,-27.57)) ;
#166105=CARTESIAN_POINT('Origin',(-4.8,-6.45,-27.57)) ;
#166106=CARTESIAN_POINT('Ctrl Pts',(-5.,-6.55,-27.77)) ;
#166107=CARTESIAN_POINT('Ctrl Pts',(-5.,-6.55,-27.77)) ;
#166108=CARTESIAN_POINT('Ctrl Pts',(-5.,-6.55,-27.77)) ;
#166109=CARTESIAN_POINT('Ctrl Pts',(-4.97374656717361,-6.55,-27.7174931343473)) ;
#166110=CARTESIAN_POINT('Ctrl Pts',(-4.96045866731622,-6.55,-27.730458667316)) ;
#166111=CARTESIAN_POINT('Ctrl Pts',(-4.94749313434733,-6.55,-27.7437465671736)) ;
#166112=CARTESIAN_POINT('Ctrl Pts',(-4.94780128270146,-6.53922263893877,
-27.6656025654029)) ;
#166113=CARTESIAN_POINT('Ctrl Pts',(-4.92085344889017,-6.52362528614073,
-27.6908534488901)) ;
#166114=CARTESIAN_POINT('Ctrl Pts',(-4.89560256540291,-6.53922263893874,
-27.7178012827014)) ;
#166115=CARTESIAN_POINT('Ctrl Pts',(-4.92003334147129,-6.5114546977086,
-27.6100666829426)) ;
#166116=CARTESIAN_POINT('Ctrl Pts',(-4.8971161968584,-6.48208554016475,
-27.6671161968584)) ;
#166117=CARTESIAN_POINT('Ctrl Pts',(-4.84006668294258,-6.51145469770861,
-27.6900333414713)) ;
#166118=CARTESIAN_POINT('Ctrl Pts',(-4.91262134295865,-6.5003618540841,
-27.5952426859173)) ;
#166119=CARTESIAN_POINT('Ctrl Pts',(-4.89498692411703,-6.46792722356048,
-27.6649869241171)) ;
#166120=CARTESIAN_POINT('Ctrl Pts',(-4.82524268591729,-6.5003618540841,
-27.6826213429587)) ;
#166121=CARTESIAN_POINT('Ctrl Pts',(-4.90260275053909,-6.47617483238892,
-27.5752055010782)) ;
#166122=CARTESIAN_POINT('Ctrl Pts',(-4.89670325643594,-6.45094059868419,
-27.6667032564358)) ;
#166123=CARTESIAN_POINT('Ctrl Pts',(-4.80520550107819,-6.47617483238891,
-27.6726027505391)) ;
#166124=CARTESIAN_POINT('Ctrl Pts',(-4.9,-6.46309229646329,-27.5700000008182)) ;
#166125=CARTESIAN_POINT('Ctrl Pts',(-4.89999269603999,-6.44945650152248,
-27.6699926960966)) ;
#166126=CARTESIAN_POINT('Ctrl Pts',(-4.80000000081823,-6.46309229646328,
-27.67)) ;
#166127=CARTESIAN_POINT('Ctrl Pts',(-4.9,-6.45,-27.57)) ;
#166128=CARTESIAN_POINT('Ctrl Pts',(-4.9,-6.45,-27.67)) ;
#166129=CARTESIAN_POINT('Ctrl Pts',(-4.8,-6.45,-27.67)) ;
#166130=CARTESIAN_POINT('Ctrl Pts',(-5.82426676739349,-5.43399303700618,
-25.0670109659688)) ;
#166131=CARTESIAN_POINT('Ctrl Pts',(-5.80266988778314,-5.5257236068294,
-25.0723540173506)) ;
#166132=CARTESIAN_POINT('Ctrl Pts',(-5.82426676352018,-5.53106667371342,
-25.1640845871828)) ;
#166133=CARTESIAN_POINT('Ctrl Pts',(-5.83498671931115,-5.43935351191914,
-25.0643294581962)) ;
#166134=CARTESIAN_POINT('Ctrl Pts',(-5.80595263122267,-5.52411753147712,
-25.0739600935403)) ;
#166135=CARTESIAN_POINT('Ctrl Pts',(-5.83498671397629,-5.53374818067469,
-25.1587241131463)) ;
#166136=CARTESIAN_POINT('Ctrl Pts',(-5.84526105845711,-5.44830326289498,
-25.0598528401962)) ;
#166137=CARTESIAN_POINT('Ctrl Pts',(-5.8137093274614,-5.52260132030856,
-25.0754763059991)) ;
#166138=CARTESIAN_POINT('Ctrl Pts',(-5.84526105243723,-5.5382247974634,
-25.1497743635698)) ;
#166139=CARTESIAN_POINT('Ctrl Pts',(-5.86378685403698,-5.47240020430406,
-25.0478032513087)) ;
#166140=CARTESIAN_POINT('Ctrl Pts',(-5.83531854275285,-5.52733067404486,
-25.0707469551147)) ;
#166141=CARTESIAN_POINT('Ctrl Pts',(-5.86378684816463,-5.55027438459901,
-25.1256774250056)) ;
#166142=CARTESIAN_POINT('Ctrl Pts',(-5.87203852631574,-5.4875449513474,
-25.0402315528944)) ;
#166143=CARTESIAN_POINT('Ctrl Pts',(-5.84834787930682,-5.53310199490455,
-25.0649756357762)) ;
#166144=CARTESIAN_POINT('Ctrl Pts',(-5.87203852123042,-5.55784608243458,
-25.110532679514)) ;
#166145=CARTESIAN_POINT('Ctrl Pts',(-5.89242747304799,-5.53981202333456,
-25.0141056511376)) ;
#166146=CARTESIAN_POINT('Ctrl Pts',(-5.88223383300423,-5.56084219179271,
-25.0372354431741)) ;
#166147=CARTESIAN_POINT('Ctrl Pts',(-5.89242747063502,-5.58397198402776,
-25.0582656123278)) ;
#166148=CARTESIAN_POINT('Ctrl Pts',(-5.9,-5.58381083947299,-24.992119400143)) ;
#166149=CARTESIAN_POINT('Ctrl Pts',(-5.9,-5.59485304502672,-25.0032245928865)) ;
#166150=CARTESIAN_POINT('Ctrl Pts',(-5.9,-5.60595823775503,-25.0142667984405)) ;
#166151=CARTESIAN_POINT('Ctrl Pts',(-5.9,-5.62807764064044,-24.97)) ;
#166152=CARTESIAN_POINT('Ctrl Pts',(-5.9,-5.62807764064044,-24.97)) ;
#166153=CARTESIAN_POINT('Ctrl Pts',(-5.9,-5.62807764064044,-24.97)) ;
#166154=CARTESIAN_POINT('Origin',(-5.84850712500726,-5.43404914061138,-25.1640285000291)) ;
#166155=CARTESIAN_POINT('Ctrl Pts',(-5.82425356250363,-5.53106339062591,
-25.1640285000291)) ;
#166156=CARTESIAN_POINT('Ctrl Pts',(-5.80269484027818,-5.52567371006955,
-25.0724039305709)) ;
#166157=CARTESIAN_POINT('Ctrl Pts',(-5.82425356250363,-5.43404914061138,
-25.0670142500145)) ;
#166158=CARTESIAN_POINT('Ctrl Pts',(-5.80840777707096,-5.52710194426774,
-25.1679899459043)) ;
#166159=CARTESIAN_POINT('Ctrl Pts',(-5.79341417645231,-5.52335354411309,
-25.0728358498184)) ;
#166160=CARTESIAN_POINT('Ctrl Pts',(-5.81633079157288,-5.43008775511759,
-25.0689949427472)) ;
#166161=CARTESIAN_POINT('Ctrl Pts',(-5.79207992677989,-5.52301998169497,
-25.169999999534)) ;
#166162=CARTESIAN_POINT('Ctrl Pts',(-5.78430903206645,-5.52107725801649,
-25.0719613954329)) ;
#166163=CARTESIAN_POINT('Ctrl Pts',(-5.80816665318299,-5.42600568595106,
-25.07)) ;
#166164=CARTESIAN_POINT('Ctrl Pts',(-5.77574643749636,-5.51893660937409,
-25.17)) ;
#166165=CARTESIAN_POINT('Ctrl Pts',(-5.77574643749636,-5.51893660937409,
-25.07)) ;
#166166=CARTESIAN_POINT('Ctrl Pts',(-5.8,-5.42192235935956,-25.07)) ;
#166167=CARTESIAN_POINT('Origin',(-5.8,-5.42192235935956,-25.17)) ;
#166168=CARTESIAN_POINT('Origin',(-5.8066065036801,-5.42357398527959,-25.17)) ;
#166169=CARTESIAN_POINT('Origin',(-5.17275707706437,-5.26511162862565,-25.17)) ;
#166170=CARTESIAN_POINT('Origin',(-5.15068655017073,-5.25959399690224,-25.1805938529089)) ;
#166171=CARTESIAN_POINT('Origin',(-5.17275707706436,-5.26511162862565,-25.17)) ;
#166172=CARTESIAN_POINT('Origin',(-5.17275707706436,-5.26511162862565,-25.17)) ;
#166173=CARTESIAN_POINT('Origin',(-5.17275707706436,-5.26511162862565,-25.17)) ;
#166174=CARTESIAN_POINT('Origin',(-5.17275707706436,-5.05,-25.17)) ;
#166175=CARTESIAN_POINT('Origin',(-5.17275707706436,-1.91866427917294,-25.17)) ;
#166176=CARTESIAN_POINT('Origin',(-3.78014014831103,-3.31128120792626,-25.8384561258016)) ;
#166177=CARTESIAN_POINT('Origin',(-5.17275707706436,-1.91866427917294,-25.17)) ;
#166178=CARTESIAN_POINT('Origin',(-5.17275707706436,-1.91866427917293,-25.17)) ;
#166179=CARTESIAN_POINT('Origin',(-5.17275707706436,-1.91866427917294,-25.17)) ;
#166180=CARTESIAN_POINT('Origin',(-3.97071067811865,-3.12071067811865,-25.17)) ;
#166181=CARTESIAN_POINT('Origin',(-5.8,-1.2914213562373,-25.17)) ;
#166182=CARTESIAN_POINT('Ctrl Pts',(-5.87071067811865,-1.14999999999999,
-25.0407106781187)) ;
#166183=CARTESIAN_POINT('Ctrl Pts',(-5.8471404520791,-1.10285954792089,
-25.0642809041582)) ;
#166184=CARTESIAN_POINT('Ctrl Pts',(-5.87071067811865,-1.07928932188134,
-25.1114213562373)) ;
#166185=CARTESIAN_POINT('Ctrl Pts',(-5.85217562795657,-1.18707010095451,
-25.0592457282807)) ;
#166186=CARTESIAN_POINT('Ctrl Pts',(-5.81261165662078,-1.13738834337949,
-25.0858614719497)) ;
#166187=CARTESIAN_POINT('Ctrl Pts',(-5.83353949671049,-1.1164605032895,
-25.1485925363811)) ;
#166188=CARTESIAN_POINT('Ctrl Pts',(-5.82627077431945,-1.23887980759835,
-25.07)) ;
#166189=CARTESIAN_POINT('Ctrl Pts',(-5.76566787907951,-1.18433212092046,
-25.0871489437127)) ;
#166190=CARTESIAN_POINT('Ctrl Pts',(-5.78190678732229,-1.1680932126777,
-25.1699999994186)) ;
#166191=CARTESIAN_POINT('Ctrl Pts',(-5.8,-1.2914213562373,-25.07)) ;
#166192=CARTESIAN_POINT('Ctrl Pts',(-5.72928932188134,-1.22071067811865,
-25.07)) ;
#166193=CARTESIAN_POINT('Ctrl Pts',(-5.72928932188134,-1.22071067811865,
-25.17)) ;
#166194=CARTESIAN_POINT('Origin',(-5.94142135623731,-1.15,-25.1114213562373)) ;
#166195=CARTESIAN_POINT('Ctrl Pts',(-5.9,-1.00857864376269,-24.97)) ;
#166196=CARTESIAN_POINT('Ctrl Pts',(-5.9,-1.00857864376269,-24.97)) ;
#166197=CARTESIAN_POINT('Ctrl Pts',(-5.9,-1.00857864376269,-24.97)) ;
#166198=CARTESIAN_POINT('Ctrl Pts',(-5.9,-1.06112019240164,-24.9962707743195)) ;
#166199=CARTESIAN_POINT('Ctrl Pts',(-5.9,-1.04860238145267,-25.0100237376901)) ;
#166200=CARTESIAN_POINT('Ctrl Pts',(-5.9,-1.03484941808214,-25.022541548639)) ;
#166201=CARTESIAN_POINT('Ctrl Pts',(-5.88924572828071,-1.11292989904543,
-25.0221756279566)) ;
#166202=CARTESIAN_POINT('Ctrl Pts',(-5.87451700627693,-1.08721613123091,
-25.0486374874681)) ;
#166203=CARTESIAN_POINT('Ctrl Pts',(-5.88924572828062,-1.06075427171937,
-25.0743512552826)) ;
#166204=CARTESIAN_POINT('Ctrl Pts',(-5.87071067811865,-1.14999999999999,
-25.0407106781187)) ;
#166205=CARTESIAN_POINT('Ctrl Pts',(-5.8471404520791,-1.10285954792089,
-25.0642809041582)) ;
#166206=CARTESIAN_POINT('Ctrl Pts',(-5.87071067811865,-1.07928932188134,
-25.1114213562373)) ;
#166207=CARTESIAN_POINT('Ctrl Pts',(-5.87071067811866,-1.14999999999999,
-28.2992893218813)) ;
#166208=CARTESIAN_POINT('Ctrl Pts',(-5.84714045207911,-1.10285954792089,
-28.2757190958418)) ;
#166209=CARTESIAN_POINT('Ctrl Pts',(-5.87071067811866,-1.07928932188134,
-28.2285786437627)) ;
#166210=CARTESIAN_POINT('Ctrl Pts',(-5.8892457282807,-1.11292989904542,
-28.3178243720434)) ;
#166211=CARTESIAN_POINT('Ctrl Pts',(-5.87451700627501,-1.08721613123182,
-28.2913625125304)) ;
#166212=CARTESIAN_POINT('Ctrl Pts',(-5.88924572828062,-1.06075427171937,
-28.2656487447174)) ;
#166213=CARTESIAN_POINT('Ctrl Pts',(-5.9,-1.06112019240159,-28.3437292256804)) ;
#166214=CARTESIAN_POINT('Ctrl Pts',(-5.9,-1.0486023814516,-28.3299762623108)) ;
#166215=CARTESIAN_POINT('Ctrl Pts',(-5.9,-1.03484941808214,-28.317458451361)) ;
#166216=CARTESIAN_POINT('Ctrl Pts',(-5.9,-1.00857864376269,-28.37)) ;
#166217=CARTESIAN_POINT('Ctrl Pts',(-5.9,-1.00857864376269,-28.37)) ;
#166218=CARTESIAN_POINT('Ctrl Pts',(-5.9,-1.00857864376269,-28.37)) ;
#166219=CARTESIAN_POINT('Origin',(-5.94142135623734,-1.14999999999996,-28.2285786437627)) ;
#166220=CARTESIAN_POINT('Ctrl Pts',(-5.8,-1.2914213562373,-28.27)) ;
#166221=CARTESIAN_POINT('Ctrl Pts',(-5.72928932188134,-1.22071067811865,
-28.27)) ;
#166222=CARTESIAN_POINT('Ctrl Pts',(-5.72928932188134,-1.22071067811865,
-28.17)) ;
#166223=CARTESIAN_POINT('Ctrl Pts',(-5.82627077431951,-1.23887980759822,
-28.27)) ;
#166224=CARTESIAN_POINT('Ctrl Pts',(-5.76566787907979,-1.18433212092023,
-28.2528510562872)) ;
#166225=CARTESIAN_POINT('Ctrl Pts',(-5.78190678732242,-1.16809321267757,
-28.1700000005814)) ;
#166226=CARTESIAN_POINT('Ctrl Pts',(-5.85217562795678,-1.18707010095483,
-28.2807542717195)) ;
#166227=CARTESIAN_POINT('Ctrl Pts',(-5.81261165662033,-1.13738834337968,
-28.2541385280508)) ;
#166228=CARTESIAN_POINT('Ctrl Pts',(-5.83353949671033,-1.11646050328967,
-28.1914074636191)) ;
#166229=CARTESIAN_POINT('Ctrl Pts',(-5.87071067811866,-1.14999999999999,
-28.2992893218813)) ;
#166230=CARTESIAN_POINT('Ctrl Pts',(-5.84714045207911,-1.10285954792088,
-28.2757190958418)) ;
#166231=CARTESIAN_POINT('Ctrl Pts',(-5.87071067811866,-1.07928932188133,
-28.2285786437627)) ;
#166232=CARTESIAN_POINT('Origin',(-5.8,-1.29142135623731,-28.17)) ;
#166233=CARTESIAN_POINT('Origin',(-3.59571067811865,-3.49571067811865,-28.17)) ;
#166234=CARTESIAN_POINT('Origin',(-5.17275707706437,-1.91866427917293,-28.17)) ;
#166235=CARTESIAN_POINT('Origin',(-3.09057773798104,-4.00084361825625,-27.17055391724)) ;
#166236=CARTESIAN_POINT('Origin',(-5.17275707706436,-1.91866427917293,-28.17)) ;
#166237=CARTESIAN_POINT('Origin',(-5.17275707706436,-1.91866427917293,-28.17)) ;
#166238=CARTESIAN_POINT('Origin',(-5.17275707706436,-1.91866427917293,-28.17)) ;
#166239=CARTESIAN_POINT('Origin',(-5.17275707706436,-5.05,-28.17)) ;
#166240=CARTESIAN_POINT('Origin',(-5.17275707706436,-5.26511162862565,-28.17)) ;
#166241=CARTESIAN_POINT('Origin',(-3.96111272388873,-4.96220054033175,-27.5884107104757)) ;
#166242=CARTESIAN_POINT('Origin',(-5.17275707706436,-5.26511162862565,-28.17)) ;
#166243=CARTESIAN_POINT('Origin',(-5.17275707706436,-5.26511162862565,-28.17)) ;
#166244=CARTESIAN_POINT('Origin',(-5.17275707706436,-5.26511162862565,-28.17)) ;
#166245=CARTESIAN_POINT('Origin',(-5.10072415073893,-5.24710339704429,-28.17)) ;
#166246=CARTESIAN_POINT('Origin',(-5.8,-5.42192235935956,-28.17)) ;
#166247=CARTESIAN_POINT('Ctrl Pts',(-5.77574643749636,-5.51893660937409,
-28.17)) ;
#166248=CARTESIAN_POINT('Ctrl Pts',(-5.77574643749636,-5.51893660937409,
-28.27)) ;
#166249=CARTESIAN_POINT('Ctrl Pts',(-5.8,-5.42192235935956,-28.27)) ;
#166250=CARTESIAN_POINT('Ctrl Pts',(-5.7920799267799,-5.52301998169498,
-28.170000000466)) ;
#166251=CARTESIAN_POINT('Ctrl Pts',(-5.78430903206646,-5.52107725801649,
-28.2680386045671)) ;
#166252=CARTESIAN_POINT('Ctrl Pts',(-5.80816665318301,-5.42600568595105,
-28.27)) ;
#166253=CARTESIAN_POINT('Ctrl Pts',(-5.80840777707094,-5.52710194426774,
-28.1720100540957)) ;
#166254=CARTESIAN_POINT('Ctrl Pts',(-5.7934141764523,-5.52335354411309,
-28.2671641501816)) ;
#166255=CARTESIAN_POINT('Ctrl Pts',(-5.81633079157287,-5.43008775511759,
-28.2710050572528)) ;
#166256=CARTESIAN_POINT('Ctrl Pts',(-5.82425356250363,-5.53106339062591,
-28.1759714999709)) ;
#166257=CARTESIAN_POINT('Ctrl Pts',(-5.80269484027818,-5.52567371006955,
-28.2675960694291)) ;
#166258=CARTESIAN_POINT('Ctrl Pts',(-5.82425356250363,-5.43404914061138,
-28.2729857499855)) ;
#166259=CARTESIAN_POINT('Origin',(-5.84850712500726,-5.43404914061138,-28.1759714999709)) ;
#166260=CARTESIAN_POINT('Ctrl Pts',(-5.82426676739352,-5.53106667467169,
-28.1759153963656)) ;
#166261=CARTESIAN_POINT('Ctrl Pts',(-5.80266988778309,-5.52572362328995,
-28.267645966189)) ;
#166262=CARTESIAN_POINT('Ctrl Pts',(-5.82426676352022,-5.43399305345751,
-28.272989033073)) ;
#166263=CARTESIAN_POINT('Ctrl Pts',(-5.83498671931118,-5.53374818244429,
-28.1812758712786)) ;
#166264=CARTESIAN_POINT('Ctrl Pts',(-5.80595263122259,-5.52411754710017,
-28.2660398908368)) ;
#166265=CARTESIAN_POINT('Ctrl Pts',(-5.83498671397633,-5.43935352749393,
-28.2756705400343)) ;
#166266=CARTESIAN_POINT('Ctrl Pts',(-5.84526105845716,-5.53822480044429,
-28.1902256222544)) ;
#166267=CARTESIAN_POINT('Ctrl Pts',(-5.81370932746132,-5.52260133464138,
-28.2645236796683)) ;
#166268=CARTESIAN_POINT('Ctrl Pts',(-5.84526105243728,-5.44830327707048,
-28.280147156823)) ;
#166269=CARTESIAN_POINT('Ctrl Pts',(-5.863786854037,-5.55027438933178,-28.2143225636635)) ;
#166270=CARTESIAN_POINT('Ctrl Pts',(-5.83531854275277,-5.52733068552579,
-28.2692530334044)) ;
#166271=CARTESIAN_POINT('Ctrl Pts',(-5.86378684816469,-5.47240021563481,
-28.2921967439586)) ;
#166272=CARTESIAN_POINT('Ctrl Pts',(-5.87203852631579,-5.55784608774608,
-28.2294673107068)) ;
#166273=CARTESIAN_POINT('Ctrl Pts',(-5.84834787930676,-5.53310200486437,
-28.2750243542641)) ;
#166274=CARTESIAN_POINT('Ctrl Pts',(-5.87203852123048,-5.48754496112639,
-28.2997684417942)) ;
#166275=CARTESIAN_POINT('Ctrl Pts',(-5.89242747304797,-5.58397198950285,
-28.2817343826941)) ;
#166276=CARTESIAN_POINT('Ctrl Pts',(-5.8822338330042,-5.56084219746613,
-28.3027645511524)) ;
#166277=CARTESIAN_POINT('Ctrl Pts',(-5.89242747063504,-5.53981202831257,
-28.3258943433874)) ;
#166278=CARTESIAN_POINT('Ctrl Pts',(-5.9,-5.60595824049749,-28.3257331988326)) ;
#166279=CARTESIAN_POINT('Ctrl Pts',(-5.9,-5.59485304775411,-28.3367754043862)) ;
#166280=CARTESIAN_POINT('Ctrl Pts',(-5.9,-5.58381084219986,-28.3478805971146)) ;
#166281=CARTESIAN_POINT('Ctrl Pts',(-5.9,-5.62807764064044,-28.37)) ;
#166282=CARTESIAN_POINT('Ctrl Pts',(-5.9,-5.62807764064044,-28.37)) ;
#166283=CARTESIAN_POINT('Ctrl Pts',(-5.9,-5.62807764064044,-28.37)) ;
#166284=CARTESIAN_POINT('Origin',(7.8,2.1,-27.07)) ;
#166285=CARTESIAN_POINT('Origin',(7.8,2.1,-27.27)) ;
#166286=CARTESIAN_POINT('Origin',(7.6,2.1,-27.07)) ;
#166287=CARTESIAN_POINT('Origin',(7.6,2.1,-27.07)) ;
#166288=CARTESIAN_POINT('Origin',(7.6,2.1,-26.27)) ;
#166289=CARTESIAN_POINT('Origin',(7.8,2.1,-27.27)) ;
#166290=CARTESIAN_POINT('Origin',(9.6,2.1,-27.27)) ;
#166291=CARTESIAN_POINT('Origin',(7.8,2.1,-26.27)) ;
#166292=CARTESIAN_POINT('Origin',(7.8,2.1,-26.07)) ;
#166293=CARTESIAN_POINT('Origin',(9.6,2.1,-27.07)) ;
#166294=CARTESIAN_POINT('Origin',(9.8,2.1,-27.07)) ;
#166295=CARTESIAN_POINT('Origin',(7.8,2.1,-26.07)) ;
#166296=CARTESIAN_POINT('Origin',(9.6,2.1,-26.07)) ;
#166297=CARTESIAN_POINT('Origin',(9.8,2.1,-27.07)) ;
#166298=CARTESIAN_POINT('Origin',(9.8,2.1,-26.27)) ;
#166299=CARTESIAN_POINT('Origin',(9.6,2.1,-26.27)) ;
#166300=CARTESIAN_POINT('Origin',(-4.15,-6.25,-25.92)) ;
#166301=CARTESIAN_POINT('Origin',(-4.15,-6.3,-25.92)) ;
#166302=CARTESIAN_POINT('Origin',(-4.15,-6.3,-26.67)) ;
#166303=CARTESIAN_POINT('Origin',(-4.15,-6.3,-27.42)) ;
#166304=CARTESIAN_POINT('Origin',(-4.15,-6.3,-25.92)) ;
#166305=CARTESIAN_POINT('Origin',(-4.15,-6.25,-27.42)) ;
#166306=CARTESIAN_POINT('Origin',(-4.15,-6.3,-27.42)) ;
#166307=CARTESIAN_POINT('Origin',(-4.15,-6.3,-25.92)) ;
#166308=CARTESIAN_POINT('Origin',(-4.15,-6.3,-25.92)) ;
#166309=CARTESIAN_POINT('Origin',(-4.15,-6.3,-27.42)) ;
#166310=CARTESIAN_POINT('Origin',(-4.15,-6.3,-27.42)) ;
#166311=CARTESIAN_POINT('Origin',(-4.65,-6.25,-25.92)) ;
#166312=CARTESIAN_POINT('Origin',(-4.65,-6.3,-25.92)) ;
#166313=CARTESIAN_POINT('Origin',(0.,-6.3,-25.92)) ;
#166314=CARTESIAN_POINT('Origin',(-4.65,-6.3,-25.92)) ;
#166315=CARTESIAN_POINT('Origin',(0.,-6.3,-27.42)) ;
#166316=CARTESIAN_POINT('Origin',(-4.65,-6.3,-27.42)) ;
#166317=CARTESIAN_POINT('Origin',(-4.65,-6.25,-27.42)) ;
#166318=CARTESIAN_POINT('Origin',(-4.65,-6.3,-27.42)) ;
#166319=CARTESIAN_POINT('Origin',(-4.65,-6.3,-25.92)) ;
#166320=CARTESIAN_POINT('Origin',(-4.65,-6.3,-25.92)) ;
#166321=CARTESIAN_POINT('Origin',(-4.65,-6.3,-27.42)) ;
#166322=CARTESIAN_POINT('Origin',(-4.65,-6.3,-27.42)) ;
#166323=CARTESIAN_POINT('Origin',(-4.65,-6.3,-26.67)) ;
#166324=CARTESIAN_POINT('Origin',(-3.,4.45,-27.77)) ;
#166325=CARTESIAN_POINT('Origin',(-2.1,4.45,-27.77)) ;
#166326=CARTESIAN_POINT('Origin',(-2.9,4.45,-27.77)) ;
#166327=CARTESIAN_POINT('Origin',(-2.9,4.45,-27.57)) ;
#166328=CARTESIAN_POINT('Origin',(-3.1,4.45,-27.57)) ;
#166329=CARTESIAN_POINT('Origin',(-2.9,4.45,-27.57)) ;
#166330=CARTESIAN_POINT('Origin',(-2.1,4.45,-27.57)) ;
#166331=CARTESIAN_POINT('Origin',(-2.1,4.45,-27.57)) ;
#166332=CARTESIAN_POINT('Origin',(-1.9,4.45,-27.57)) ;
#166333=CARTESIAN_POINT('Origin',(-3.1,4.45,-27.67)) ;
#166334=CARTESIAN_POINT('Origin',(-3.1,4.45,-25.77)) ;
#166335=CARTESIAN_POINT('Origin',(-2.9,4.4,-27.57)) ;
#166336=CARTESIAN_POINT('Origin',(-2.9,4.35,-27.57)) ;
#166337=CARTESIAN_POINT('Origin',(-1.95156391047391E-16,4.35,-27.57)) ;
#166338=CARTESIAN_POINT('Origin',(-2.1,4.35,-27.57)) ;
#166339=CARTESIAN_POINT('Origin',(-2.9,4.35,-27.57)) ;
#166340=CARTESIAN_POINT('Origin',(-2.1,4.4,-27.57)) ;
#166341=CARTESIAN_POINT('Origin',(-2.1,4.35,-27.57)) ;
#166342=CARTESIAN_POINT('Origin',(-1.9,4.45,-27.67)) ;
#166343=CARTESIAN_POINT('Origin',(-1.9,4.45,-25.77)) ;
#166344=CARTESIAN_POINT('Origin',(-3.,4.45,-25.57)) ;
#166345=CARTESIAN_POINT('Origin',(-2.9,4.45,-25.57)) ;
#166346=CARTESIAN_POINT('Origin',(-2.1,4.45,-25.57)) ;
#166347=CARTESIAN_POINT('Origin',(-2.9,4.45,-25.77)) ;
#166348=CARTESIAN_POINT('Origin',(-2.9,4.45,-25.77)) ;
#166349=CARTESIAN_POINT('Origin',(-2.9,4.35,-27.57)) ;
#166350=CARTESIAN_POINT('Origin',(-2.9,4.35,-27.57)) ;
#166351=CARTESIAN_POINT('Origin',(-2.1,4.35,-27.57)) ;
#166352=CARTESIAN_POINT('Origin',(-2.1,4.35,-27.57)) ;
#166353=CARTESIAN_POINT('Origin',(-2.1,4.45,-25.77)) ;
#166354=CARTESIAN_POINT('Origin',(-2.1,4.45,-25.77)) ;
#166355=CARTESIAN_POINT('Origin',(-2.9,4.4,-25.77)) ;
#166356=CARTESIAN_POINT('Origin',(-2.9,4.35,-25.77)) ;
#166357=CARTESIAN_POINT('Origin',(-2.9,4.35,-26.67)) ;
#166358=CARTESIAN_POINT('Origin',(-2.9,4.35,-25.77)) ;
#166359=CARTESIAN_POINT('Origin',(-2.1,4.35,-26.67)) ;
#166360=CARTESIAN_POINT('Origin',(-2.1,4.35,-25.77)) ;
#166361=CARTESIAN_POINT('Origin',(-2.1,4.4,-25.77)) ;
#166362=CARTESIAN_POINT('Origin',(-2.1,4.35,-25.77)) ;
#166363=CARTESIAN_POINT('Origin',(-2.9,4.35,-25.77)) ;
#166364=CARTESIAN_POINT('Origin',(-2.9,4.35,-25.77)) ;
#166365=CARTESIAN_POINT('Origin',(-2.1,4.35,-25.77)) ;
#166366=CARTESIAN_POINT('Origin',(-2.1,4.35,-25.77)) ;
#166367=CARTESIAN_POINT('Origin',(-1.95156391047391E-16,4.35,-25.77)) ;
#166368=CARTESIAN_POINT('Origin',(-2.25,4.25,-27.42)) ;
#166369=CARTESIAN_POINT('Origin',(-2.25,4.3,-27.42)) ;
#166370=CARTESIAN_POINT('Origin',(-2.25,4.3,-26.67)) ;
#166371=CARTESIAN_POINT('Origin',(-2.25,4.3,-25.92)) ;
#166372=CARTESIAN_POINT('Origin',(-2.25,4.3,-27.42)) ;
#166373=CARTESIAN_POINT('Origin',(-2.25,4.25,-25.92)) ;
#166374=CARTESIAN_POINT('Origin',(-2.25,4.3,-25.92)) ;
#166375=CARTESIAN_POINT('Origin',(-2.25,4.3,-27.42)) ;
#166376=CARTESIAN_POINT('Origin',(-2.25,4.3,-27.42)) ;
#166377=CARTESIAN_POINT('Origin',(-2.25,4.3,-25.92)) ;
#166378=CARTESIAN_POINT('Origin',(-2.25,4.3,-25.92)) ;
#166379=CARTESIAN_POINT('Origin',(-2.75,4.25,-27.42)) ;
#166380=CARTESIAN_POINT('Origin',(-2.75,4.3,-27.42)) ;
#166381=CARTESIAN_POINT('Origin',(-1.97127667724637E-17,4.3,-27.42)) ;
#166382=CARTESIAN_POINT('Origin',(-2.75,4.3,-27.42)) ;
#166383=CARTESIAN_POINT('Origin',(-1.97127667724637E-17,4.3,-25.92)) ;
#166384=CARTESIAN_POINT('Origin',(-2.75,4.3,-25.92)) ;
#166385=CARTESIAN_POINT('Origin',(-2.75,4.25,-25.92)) ;
#166386=CARTESIAN_POINT('Origin',(-2.75,4.3,-25.92)) ;
#166387=CARTESIAN_POINT('Origin',(-2.75,4.3,-27.42)) ;
#166388=CARTESIAN_POINT('Origin',(-2.75,4.3,-27.42)) ;
#166389=CARTESIAN_POINT('Origin',(-2.75,4.3,-25.92)) ;
#166390=CARTESIAN_POINT('Origin',(-2.75,4.3,-25.92)) ;
#166391=CARTESIAN_POINT('Origin',(-2.75,4.3,-26.67)) ;
#166392=CARTESIAN_POINT('Origin',(7.8,2.9,-27.07)) ;
#166393=CARTESIAN_POINT('Origin',(7.8,2.9,-27.07)) ;
#166394=CARTESIAN_POINT('Origin',(7.8,2.9,-26.27)) ;
#166395=CARTESIAN_POINT('Origin',(7.8,2.9,-26.27)) ;
#166396=CARTESIAN_POINT('Origin',(7.8,2.9,-26.27)) ;
#166397=CARTESIAN_POINT('Origin',(7.8,2.9,-27.07)) ;
#166398=CARTESIAN_POINT('Origin',(7.8,2.9,-27.07)) ;
#166399=CARTESIAN_POINT('Origin',(9.6,2.9,-26.27)) ;
#166400=CARTESIAN_POINT('Origin',(9.6,2.9,-26.27)) ;
#166401=CARTESIAN_POINT('Origin',(9.6,2.9,-27.07)) ;
#166402=CARTESIAN_POINT('Origin',(9.6,2.9,-27.07)) ;
#166403=CARTESIAN_POINT('Origin',(9.6,2.9,-26.27)) ;
#166404=CARTESIAN_POINT('Origin',(9.6,2.9,-26.27)) ;
#166405=CARTESIAN_POINT('Origin',(9.6,2.9,-27.07)) ;
#166406=CARTESIAN_POINT('Origin',(9.6,2.9,-27.07)) ;
#166407=CARTESIAN_POINT('Origin',(9.6,2.9,-27.07)) ;
#166408=CARTESIAN_POINT('Origin',(-0.183301359729408,3.45,-25.152963213524)) ;
#166409=CARTESIAN_POINT('Origin',(0.24923464143508,3.15,-26.5537799780213)) ;
#166410=CARTESIAN_POINT('Origin',(-0.249234641435079,3.15,-26.7862200219787)) ;
#166411=CARTESIAN_POINT('Origin',(-1.04429375741423,3.45,-25.5544505621777)) ;
#166412=CARTESIAN_POINT('Origin',(10.1,-2.15,-29.5768804065906)) ;
#166413=CARTESIAN_POINT('Origin',(10.1,-2.15,-29.5768804065906)) ;
#166414=CARTESIAN_POINT('Origin',(10.1,-2.15,-29.5768804065906)) ;
#166415=CARTESIAN_POINT('Origin',(10.1,-2.15,-29.5768804065906)) ;
#166416=CARTESIAN_POINT('Origin',(10.1,-2.15,-30.48)) ;
#166417=CARTESIAN_POINT('Origin',(10.1,-2.15,-29.175)) ;
#166418=CARTESIAN_POINT('Origin',(10.2,-2.15,-29.5768804065906)) ;
#166419=CARTESIAN_POINT('Origin',(3.7,-2.15,-29.5768804065906)) ;
#166420=CARTESIAN_POINT('Origin',(10.1,-3.65625,-30.48)) ;
#166421=CARTESIAN_POINT('Origin',(10.1,-2.15,-31.3831195934094)) ;
#166422=CARTESIAN_POINT('Origin',(10.1,-3.65625,-29.175)) ;
#166423=CARTESIAN_POINT('Origin',(10.1,1.9,-29.175)) ;
#166424=CARTESIAN_POINT('Origin',(10.1,-2.15,-29.175)) ;
#166425=CARTESIAN_POINT('Origin',(10.1,-2.15,-29.175)) ;
#166426=CARTESIAN_POINT('Origin',(10.1,-2.15,-29.175)) ;
#166427=CARTESIAN_POINT('Origin',(3.7,-2.15,-29.5768804065906)) ;
#166428=CARTESIAN_POINT('Origin',(3.7,-2.32153024911032,-29.6797267659824)) ;
#166429=CARTESIAN_POINT('Origin',(3.7,-2.35,-29.5768804065906)) ;
#166430=CARTESIAN_POINT('Origin',(10.1,-2.15,-31.3831195934094)) ;
#166431=CARTESIAN_POINT('Origin',(10.1,-2.15,-31.3831195934094)) ;
#166432=CARTESIAN_POINT('Origin',(10.1,-2.15,-31.3831195934094)) ;
#166433=CARTESIAN_POINT('Origin',(10.1,1.9,-30.48)) ;
#166434=CARTESIAN_POINT('Origin',(10.1,1.9,-31.785)) ;
#166435=CARTESIAN_POINT('Origin',(10.1,1.9,-29.175)) ;
#166436=CARTESIAN_POINT('Origin',(10.2,-2.15,-29.175)) ;
#166437=CARTESIAN_POINT('Origin',(3.7,-2.15,-29.175)) ;
#166438=CARTESIAN_POINT('Origin',(3.7,-2.35,-29.075)) ;
#166439=CARTESIAN_POINT('Origin',(3.7,-2.35,-29.175)) ;
#166440=CARTESIAN_POINT('Origin',(3.7,-3.65625,-30.48)) ;
#166441=CARTESIAN_POINT('Origin',(3.7,-2.32153024911032,-31.2802732340176)) ;
#166442=CARTESIAN_POINT('Origin',(10.2,-2.15,-31.3831195934094)) ;
#166443=CARTESIAN_POINT('Origin',(3.7,-2.15,-31.3831195934094)) ;
#166444=CARTESIAN_POINT('Origin',(10.1,-2.15,-30.48)) ;
#166445=CARTESIAN_POINT('Origin',(10.1,-2.15,-31.785)) ;
#166446=CARTESIAN_POINT('Origin',(10.1,-3.65625,-31.785)) ;
#166447=CARTESIAN_POINT('Origin',(10.1,1.9,-31.785)) ;
#166448=CARTESIAN_POINT('Origin',(10.1,-2.15,-31.785)) ;
#166449=CARTESIAN_POINT('Origin',(3.7,-2.35,-29.175)) ;
#166450=CARTESIAN_POINT('Origin',(3.5,-2.35,-29.175)) ;
#166451=CARTESIAN_POINT('Origin',(3.7,-2.15,-31.3831195934094)) ;
#166452=CARTESIAN_POINT('Origin',(3.7,-2.35,-31.3831195934094)) ;
#166453=CARTESIAN_POINT('Origin',(10.1,-2.15,-31.785)) ;
#166454=CARTESIAN_POINT('Origin',(10.1,-2.15,-31.785)) ;
#166455=CARTESIAN_POINT('Origin',(3.6,1.9,-28.975)) ;
#166456=CARTESIAN_POINT('Origin',(3.5,1.9,-28.975)) ;
#166457=CARTESIAN_POINT('Origin',(2.7,1.9,-28.975)) ;
#166458=CARTESIAN_POINT('Origin',(3.5,2.69592814944142E-15,-29.175)) ;
#166459=CARTESIAN_POINT('Origin',(3.5,-5.15,-29.175)) ;
#166460=CARTESIAN_POINT('Origin',(3.7,-2.35,-31.355)) ;
#166461=CARTESIAN_POINT('Origin',(3.7,-2.35,-31.785)) ;
#166462=CARTESIAN_POINT('Origin',(3.6,-2.15,-31.785)) ;
#166463=CARTESIAN_POINT('Origin',(3.7,-2.15,-31.785)) ;
#166464=CARTESIAN_POINT('Origin',(2.7,1.9,-28.975)) ;
#166465=CARTESIAN_POINT('Origin',(2.7,1.9,-28.975)) ;
#166466=CARTESIAN_POINT('Origin',(3.5,-5.15,-29.175)) ;
#166467=CARTESIAN_POINT('Origin',(3.5,-5.15,-29.175)) ;
#166468=CARTESIAN_POINT('Origin',(3.5,-5.15,-29.175)) ;
#166469=CARTESIAN_POINT('Origin',(3.7,-2.35,-31.785)) ;
#166470=CARTESIAN_POINT('Origin',(3.5,-2.35,-31.785)) ;
#166471=CARTESIAN_POINT('Origin',(2.7,2.,-28.975)) ;
#166472=CARTESIAN_POINT('Origin',(2.7,-5.15,-28.975)) ;
#166473=CARTESIAN_POINT('Origin',(3.6,-5.15,-29.175)) ;
#166474=CARTESIAN_POINT('Origin',(2.7,-5.15,-29.175)) ;
#166475=CARTESIAN_POINT('Origin',(3.5,-5.15,0.)) ;
#166476=CARTESIAN_POINT('Origin',(3.5,-5.15,-31.785)) ;
#166477=CARTESIAN_POINT('Origin',(3.5,-2.77383442446614E-15,-31.785)) ;
#166478=CARTESIAN_POINT('Origin',(3.5,-5.15,-31.785)) ;
#166479=CARTESIAN_POINT('Origin',(2.7,-5.15,-29.175)) ;
#166480=CARTESIAN_POINT('Origin',(2.7,-5.35,-29.175)) ;
#166481=CARTESIAN_POINT('Origin',(3.5,-5.15,-31.785)) ;
#166482=CARTESIAN_POINT('Origin',(3.5,-5.15,-31.785)) ;
#166483=CARTESIAN_POINT('Origin',(2.7,-5.35,-29.075)) ;
#166484=CARTESIAN_POINT('Origin',(2.7,-5.35,-31.785)) ;
#166485=CARTESIAN_POINT('Origin',(3.6,-5.15,-31.785)) ;
#166486=CARTESIAN_POINT('Origin',(2.7,-5.15,-31.785)) ;
#166487=CARTESIAN_POINT('Origin',(3.6,1.9,-31.985)) ;
#166488=CARTESIAN_POINT('Origin',(3.5,1.9,-31.985)) ;
#166489=CARTESIAN_POINT('Origin',(2.7,1.9,-31.985)) ;
#166490=CARTESIAN_POINT('Origin',(2.7,1.9,-31.885)) ;
#166491=CARTESIAN_POINT('Origin',(2.7,1.9,-32.785)) ;
#166492=CARTESIAN_POINT('Origin',(2.7,1.9,-31.985)) ;
#166493=CARTESIAN_POINT('Origin',(2.7,-5.15,-31.785)) ;
#166494=CARTESIAN_POINT('Origin',(2.7,-5.15,-31.985)) ;
#166495=CARTESIAN_POINT('Origin',(2.7,1.9,-31.985)) ;
#166496=CARTESIAN_POINT('Origin',(2.7,1.9,-31.985)) ;
#166497=CARTESIAN_POINT('Origin',(2.7,-5.25,-31.985)) ;
#166498=CARTESIAN_POINT('Ctrl Pts',(-3.8,-6.55,-29.38)) ;
#166499=CARTESIAN_POINT('Ctrl Pts',(-3.8,-6.55,-29.38)) ;
#166500=CARTESIAN_POINT('Ctrl Pts',(-3.8,-6.55,-29.38)) ;
#166501=CARTESIAN_POINT('Ctrl Pts',(-3.82625343282633,-6.55,-29.4325068656528)) ;
#166502=CARTESIAN_POINT('Ctrl Pts',(-3.83954133268475,-6.55,-29.419541332684)) ;
#166503=CARTESIAN_POINT('Ctrl Pts',(-3.8525068656527,-6.55,-29.4062534328264)) ;
#166504=CARTESIAN_POINT('Ctrl Pts',(-3.85219871729854,-6.53922263893877,
-29.4843974345971)) ;
#166505=CARTESIAN_POINT('Ctrl Pts',(-3.87914655110986,-6.52362528614073,
-29.4591465511098)) ;
#166506=CARTESIAN_POINT('Ctrl Pts',(-3.90439743459708,-6.53922263893874,
-29.4321987172986)) ;
#166507=CARTESIAN_POINT('Ctrl Pts',(-3.87996665852871,-6.5114546977086,
-29.5399333170574)) ;
#166508=CARTESIAN_POINT('Ctrl Pts',(-3.90288380314158,-6.48208554016475,
-29.4828838031416)) ;
#166509=CARTESIAN_POINT('Ctrl Pts',(-3.95993331705742,-6.51145469770861,
-29.4599666585287)) ;
#166510=CARTESIAN_POINT('Ctrl Pts',(-3.88737865704135,-6.5003618540841,
-29.5547573140827)) ;
#166511=CARTESIAN_POINT('Ctrl Pts',(-3.90501307588293,-6.46792722356046,
-29.4850130758829)) ;
#166512=CARTESIAN_POINT('Ctrl Pts',(-3.9747573140827,-6.5003618540841,-29.4673786570414)) ;
#166513=CARTESIAN_POINT('Ctrl Pts',(-3.8973972494609,-6.47617483238892,
-29.5747944989218)) ;
#166514=CARTESIAN_POINT('Ctrl Pts',(-3.9032967435641,-6.45094059868421,
-29.4832967435641)) ;
#166515=CARTESIAN_POINT('Ctrl Pts',(-3.99479449892181,-6.47617483238891,
-29.4773972494609)) ;
#166516=CARTESIAN_POINT('Ctrl Pts',(-3.9,-6.46309229646327,-29.5799999991818)) ;
#166517=CARTESIAN_POINT('Ctrl Pts',(-3.90000730388479,-6.44945650149135,
-29.4800073039037)) ;
#166518=CARTESIAN_POINT('Ctrl Pts',(-3.99999999918173,-6.46309229646329,
-29.48)) ;
#166519=CARTESIAN_POINT('Ctrl Pts',(-3.9,-6.45,-29.58)) ;
#166520=CARTESIAN_POINT('Ctrl Pts',(-3.9,-6.45,-29.48)) ;
#166521=CARTESIAN_POINT('Ctrl Pts',(-4.,-6.45,-29.48)) ;
#166522=CARTESIAN_POINT('Origin',(-4.,-6.45,-29.58)) ;
#166523=CARTESIAN_POINT('Origin',(-4.,-6.4,-29.58)) ;
#166524=CARTESIAN_POINT('Origin',(-4.,-6.35,-29.58)) ;
#166525=CARTESIAN_POINT('Ctrl Pts',(-5.,-6.55,-29.38)) ;
#166526=CARTESIAN_POINT('Ctrl Pts',(-5.,-6.55,-29.38)) ;
#166527=CARTESIAN_POINT('Ctrl Pts',(-5.,-6.55,-29.38)) ;
#166528=CARTESIAN_POINT('Ctrl Pts',(-4.94749313434733,-6.55,-29.4062534328264)) ;
#166529=CARTESIAN_POINT('Ctrl Pts',(-4.96045866731527,-6.55,-29.4195413326841)) ;
#166530=CARTESIAN_POINT('Ctrl Pts',(-4.97374656717361,-6.55,-29.4325068656527)) ;
#166531=CARTESIAN_POINT('Ctrl Pts',(-4.89560256540291,-6.53922263893874,
-29.4321987172986)) ;
#166532=CARTESIAN_POINT('Ctrl Pts',(-4.92085344889015,-6.52362528614075,
-29.4591465511098)) ;
#166533=CARTESIAN_POINT('Ctrl Pts',(-4.94780128270146,-6.53922263893877,
-29.4843974345971)) ;
#166534=CARTESIAN_POINT('Ctrl Pts',(-4.84006668294258,-6.51145469770861,
-29.4599666585287)) ;
#166535=CARTESIAN_POINT('Ctrl Pts',(-4.89711619685841,-6.48208554016473,
-29.4828838031416)) ;
#166536=CARTESIAN_POINT('Ctrl Pts',(-4.92003334147129,-6.5114546977086,
-29.5399333170574)) ;
#166537=CARTESIAN_POINT('Ctrl Pts',(-4.82524268591729,-6.5003618540841,
-29.4673786570414)) ;
#166538=CARTESIAN_POINT('Ctrl Pts',(-4.89498692411706,-6.46792722356047,
-29.4850130758829)) ;
#166539=CARTESIAN_POINT('Ctrl Pts',(-4.91262134295865,-6.5003618540841,
-29.5547573140827)) ;
#166540=CARTESIAN_POINT('Ctrl Pts',(-4.80520550107819,-6.47617483238891,
-29.4773972494609)) ;
#166541=CARTESIAN_POINT('Ctrl Pts',(-4.8967032564359,-6.4509405986842,-29.4832967435642)) ;
#166542=CARTESIAN_POINT('Ctrl Pts',(-4.90260275053909,-6.47617483238892,
-29.5747944989218)) ;
#166543=CARTESIAN_POINT('Ctrl Pts',(-4.80000000081823,-6.46309229646328,
-29.48)) ;
#166544=CARTESIAN_POINT('Ctrl Pts',(-4.89999269609626,-6.44945650149925,
-29.4800073039037)) ;
#166545=CARTESIAN_POINT('Ctrl Pts',(-4.9,-6.46309229646329,-29.5799999991818)) ;
#166546=CARTESIAN_POINT('Ctrl Pts',(-4.8,-6.45,-29.48)) ;
#166547=CARTESIAN_POINT('Ctrl Pts',(-4.9,-6.45,-29.48)) ;
#166548=CARTESIAN_POINT('Ctrl Pts',(-4.9,-6.45,-29.58)) ;
#166549=CARTESIAN_POINT('Origin',(-4.8,-6.45,-29.58)) ;
#166550=CARTESIAN_POINT('Origin',(-4.,-6.35,-29.58)) ;
#166551=CARTESIAN_POINT('Origin',(-4.,-6.35,-29.58)) ;
#166552=CARTESIAN_POINT('Origin',(-4.,-6.35,-29.58)) ;
#166553=CARTESIAN_POINT('Ctrl Pts',(-3.8,-6.55,-31.58)) ;
#166554=CARTESIAN_POINT('Ctrl Pts',(-3.8,-6.55,-31.58)) ;
#166555=CARTESIAN_POINT('Ctrl Pts',(-3.8,-6.55,-31.58)) ;
#166556=CARTESIAN_POINT('Ctrl Pts',(-3.85250686565254,-6.55,-31.5537465671732)) ;
#166557=CARTESIAN_POINT('Ctrl Pts',(-3.83954133268437,-6.55,-31.5404586673145)) ;
#166558=CARTESIAN_POINT('Ctrl Pts',(-3.82625343282625,-6.55,-31.5274931343472)) ;
#166559=CARTESIAN_POINT('Ctrl Pts',(-3.90439743459706,-6.53922263893883,
-31.5278012827015)) ;
#166560=CARTESIAN_POINT('Ctrl Pts',(-3.87914655110982,-6.52362528614068,
-31.5008534488903)) ;
#166561=CARTESIAN_POINT('Ctrl Pts',(-3.85219871729855,-6.53922263893876,
-31.475602565403)) ;
#166562=CARTESIAN_POINT('Ctrl Pts',(-3.95993331705743,-6.51145469770856,
-31.5000333414713)) ;
#166563=CARTESIAN_POINT('Ctrl Pts',(-3.9028838031416,-6.48208554016478,
-31.4771161968583)) ;
#166564=CARTESIAN_POINT('Ctrl Pts',(-3.8799666585287,-6.5114546977086,-31.4200666829425)) ;
#166565=CARTESIAN_POINT('Ctrl Pts',(-3.97475731408271,-6.5003618540841,
-31.4926213429587)) ;
#166566=CARTESIAN_POINT('Ctrl Pts',(-3.90501307588293,-6.46792722356049,
-31.4749869241171)) ;
#166567=CARTESIAN_POINT('Ctrl Pts',(-3.88737865704135,-6.5003618540841,
-31.4052426859173)) ;
#166568=CARTESIAN_POINT('Ctrl Pts',(-3.9947944989218,-6.47617483238892,
-31.4826027505391)) ;
#166569=CARTESIAN_POINT('Ctrl Pts',(-3.9032967435641,-6.45094059868419,
-31.4767032564359)) ;
#166570=CARTESIAN_POINT('Ctrl Pts',(-3.89739724946091,-6.47617483238892,
-31.3852055010782)) ;
#166571=CARTESIAN_POINT('Ctrl Pts',(-3.99999999918176,-6.46309229646328,
-31.48)) ;
#166572=CARTESIAN_POINT('Ctrl Pts',(-3.90000730395432,-6.44945650161364,
-31.4799926958712)) ;
#166573=CARTESIAN_POINT('Ctrl Pts',(-3.9,-6.46309229646328,-31.3800000008181)) ;
#166574=CARTESIAN_POINT('Ctrl Pts',(-4.,-6.45,-31.48)) ;
#166575=CARTESIAN_POINT('Ctrl Pts',(-3.9,-6.45,-31.48)) ;
#166576=CARTESIAN_POINT('Ctrl Pts',(-3.9,-6.45,-31.38)) ;
#166577=CARTESIAN_POINT('Origin',(-4.,-6.45,-31.38)) ;
#166578=CARTESIAN_POINT('Origin',(-4.8,-6.4,-29.58)) ;
#166579=CARTESIAN_POINT('Origin',(-4.8,-6.35,-29.58)) ;
#166580=CARTESIAN_POINT('Origin',(1.9515639104739E-16,-6.35,-29.58)) ;
#166581=CARTESIAN_POINT('Origin',(-4.8,-6.35,-29.58)) ;
#166582=CARTESIAN_POINT('Origin',(-4.,-6.35,-30.48)) ;
#166583=CARTESIAN_POINT('Origin',(-4.,-6.35,-31.38)) ;
#166584=CARTESIAN_POINT('Origin',(-4.,-6.4,-31.38)) ;
#166585=CARTESIAN_POINT('Origin',(-4.,-6.35,-31.38)) ;
#166586=CARTESIAN_POINT('Origin',(-4.8,-6.35,-29.58)) ;
#166587=CARTESIAN_POINT('Origin',(-4.8,-6.35,-29.58)) ;
#166588=CARTESIAN_POINT('Origin',(-4.,-6.35,-31.38)) ;
#166589=CARTESIAN_POINT('Origin',(-4.,-6.35,-31.38)) ;
#166590=CARTESIAN_POINT('Origin',(-4.8,-6.35,-30.48)) ;
#166591=CARTESIAN_POINT('Origin',(-4.8,-6.35,-31.38)) ;
#166592=CARTESIAN_POINT('Origin',(1.9515639104739E-16,-6.35,-31.38)) ;
#166593=CARTESIAN_POINT('Origin',(-4.8,-6.35,-31.38)) ;
#166594=CARTESIAN_POINT('Origin',(-4.8,-6.35,-31.38)) ;
#166595=CARTESIAN_POINT('Origin',(-4.8,-6.35,-31.38)) ;
#166596=CARTESIAN_POINT('Origin',(-4.8,-6.4,-31.38)) ;
#166597=CARTESIAN_POINT('Origin',(-4.8,-6.45,-31.38)) ;
#166598=CARTESIAN_POINT('Ctrl Pts',(-5.,-6.55,-31.58)) ;
#166599=CARTESIAN_POINT('Ctrl Pts',(-5.,-6.55,-31.58)) ;
#166600=CARTESIAN_POINT('Ctrl Pts',(-5.,-6.55,-31.58)) ;
#166601=CARTESIAN_POINT('Ctrl Pts',(-4.97374656717363,-6.55,-31.5274931343472)) ;
#166602=CARTESIAN_POINT('Ctrl Pts',(-4.96045866731563,-6.55,-31.5404586673165)) ;
#166603=CARTESIAN_POINT('Ctrl Pts',(-4.94749313434715,-6.55,-31.5537465671739)) ;
#166604=CARTESIAN_POINT('Ctrl Pts',(-4.94780128270146,-6.53922263893877,
-31.475602565403)) ;
#166605=CARTESIAN_POINT('Ctrl Pts',(-4.92085344889015,-6.52362528614069,
-31.5008534488903)) ;
#166606=CARTESIAN_POINT('Ctrl Pts',(-4.89560256540291,-6.53922263893883,
-31.5278012827015)) ;
#166607=CARTESIAN_POINT('Ctrl Pts',(-4.92003334147129,-6.5114546977086,
-31.4200666829425)) ;
#166608=CARTESIAN_POINT('Ctrl Pts',(-4.89711619685841,-6.48208554016478,
-31.4771161968583)) ;
#166609=CARTESIAN_POINT('Ctrl Pts',(-4.84006668294258,-6.51145469770856,
-31.5000333414713)) ;
#166610=CARTESIAN_POINT('Ctrl Pts',(-4.91262134295865,-6.5003618540841,
-31.4052426859173)) ;
#166611=CARTESIAN_POINT('Ctrl Pts',(-4.89498692411706,-6.46792722356049,
-31.4749869241171)) ;
#166612=CARTESIAN_POINT('Ctrl Pts',(-4.82524268591729,-6.5003618540841,
-31.4926213429587)) ;
#166613=CARTESIAN_POINT('Ctrl Pts',(-4.90260275053909,-6.47617483238892,
-31.3852055010782)) ;
#166614=CARTESIAN_POINT('Ctrl Pts',(-4.8967032564359,-6.45094059868419,
-31.4767032564359)) ;
#166615=CARTESIAN_POINT('Ctrl Pts',(-4.80520550107819,-6.47617483238892,
-31.4826027505391)) ;
#166616=CARTESIAN_POINT('Ctrl Pts',(-4.9,-6.46309229646328,-31.3800000008181)) ;
#166617=CARTESIAN_POINT('Ctrl Pts',(-4.89999269604099,-6.44945650161557,
-31.4799926958712)) ;
#166618=CARTESIAN_POINT('Ctrl Pts',(-4.80000000081823,-6.46309229646328,
-31.48)) ;
#166619=CARTESIAN_POINT('Ctrl Pts',(-4.9,-6.45,-31.38)) ;
#166620=CARTESIAN_POINT('Ctrl Pts',(-4.9,-6.45,-31.48)) ;
#166621=CARTESIAN_POINT('Ctrl Pts',(-4.8,-6.45,-31.48)) ;
#166622=CARTESIAN_POINT('Ctrl Pts',(-5.82426676739353,-5.43399303700601,
-28.8770109659688)) ;
#166623=CARTESIAN_POINT('Ctrl Pts',(-5.80266988778306,-5.52572360682955,
-28.8823540173505)) ;
#166624=CARTESIAN_POINT('Ctrl Pts',(-5.82426676352022,-5.53106667371343,
-28.974084587183)) ;
#166625=CARTESIAN_POINT('Ctrl Pts',(-5.83498671931121,-5.43935351191898,
-28.8743294581962)) ;
#166626=CARTESIAN_POINT('Ctrl Pts',(-5.80595263122257,-5.52411753147731,
-28.8839600935403)) ;
#166627=CARTESIAN_POINT('Ctrl Pts',(-5.83498671397634,-5.53374818067472,
-28.9687241131465)) ;
#166628=CARTESIAN_POINT('Ctrl Pts',(-5.84526105845717,-5.44830326289483,
-28.8698528401961)) ;
#166629=CARTESIAN_POINT('Ctrl Pts',(-5.81370932746127,-5.52260132030868,
-28.885476305999)) ;
#166630=CARTESIAN_POINT('Ctrl Pts',(-5.8452610524373,-5.53822479746343,
-28.95977436357)) ;
#166631=CARTESIAN_POINT('Ctrl Pts',(-5.86378685403704,-5.47240020430394,
-28.8578032513087)) ;
#166632=CARTESIAN_POINT('Ctrl Pts',(-5.83531854275276,-5.5273306740449,
-28.8807469551146)) ;
#166633=CARTESIAN_POINT('Ctrl Pts',(-5.8637868481647,-5.55027438459906,
-28.9356774250057)) ;
#166634=CARTESIAN_POINT('Ctrl Pts',(-5.8720385263158,-5.48754495134729,
-28.8502315528944)) ;
#166635=CARTESIAN_POINT('Ctrl Pts',(-5.84834787930678,-5.53310199490458,
-28.8749756357761)) ;
#166636=CARTESIAN_POINT('Ctrl Pts',(-5.87203852123047,-5.55784608243464,
-28.9205326795141)) ;
#166637=CARTESIAN_POINT('Ctrl Pts',(-5.89242747304802,-5.53981202333451,
-28.8241056511375)) ;
#166638=CARTESIAN_POINT('Ctrl Pts',(-5.88223383300416,-5.56084219179273,
-28.8472354431742)) ;
#166639=CARTESIAN_POINT('Ctrl Pts',(-5.89242747063505,-5.58397198402782,
-28.8682656123278)) ;
#166640=CARTESIAN_POINT('Ctrl Pts',(-5.9,-5.58381083947297,-28.802119400143)) ;
#166641=CARTESIAN_POINT('Ctrl Pts',(-5.9,-5.59485304502685,-28.813224592887)) ;
#166642=CARTESIAN_POINT('Ctrl Pts',(-5.9,-5.60595823775506,-28.8242667984406)) ;
#166643=CARTESIAN_POINT('Ctrl Pts',(-5.9,-5.62807764064044,-28.78)) ;
#166644=CARTESIAN_POINT('Ctrl Pts',(-5.9,-5.62807764064044,-28.78)) ;
#166645=CARTESIAN_POINT('Ctrl Pts',(-5.9,-5.62807764064044,-28.78)) ;
#166646=CARTESIAN_POINT('Origin',(-5.84850712500726,-5.43404914061138,-28.9740285000291)) ;
#166647=CARTESIAN_POINT('Ctrl Pts',(-5.82425356250363,-5.53106339062591,
-28.9740285000291)) ;
#166648=CARTESIAN_POINT('Ctrl Pts',(-5.80269484027818,-5.52567371006954,
-28.8824039305709)) ;
#166649=CARTESIAN_POINT('Ctrl Pts',(-5.82425356250363,-5.43404914061138,
-28.8770142500145)) ;
#166650=CARTESIAN_POINT('Ctrl Pts',(-5.80840777707096,-5.52710194426774,
-28.9779899459043)) ;
#166651=CARTESIAN_POINT('Ctrl Pts',(-5.79341417645228,-5.52335354411315,
-28.8828358498184)) ;
#166652=CARTESIAN_POINT('Ctrl Pts',(-5.81633079157288,-5.43008775511759,
-28.8789949427472)) ;
#166653=CARTESIAN_POINT('Ctrl Pts',(-5.79207992677989,-5.52301998169497,
-28.979999999534)) ;
#166654=CARTESIAN_POINT('Ctrl Pts',(-5.78430903206646,-5.52107725801653,
-28.8819613954329)) ;
#166655=CARTESIAN_POINT('Ctrl Pts',(-5.80816665318299,-5.42600568595106,
-28.88)) ;
#166656=CARTESIAN_POINT('Ctrl Pts',(-5.77574643749636,-5.51893660937409,
-28.98)) ;
#166657=CARTESIAN_POINT('Ctrl Pts',(-5.77574643749636,-5.5189366093741,
-28.88)) ;
#166658=CARTESIAN_POINT('Ctrl Pts',(-5.8,-5.42192235935956,-28.88)) ;
#166659=CARTESIAN_POINT('Origin',(-5.8,-5.42192235935956,-28.98)) ;
#166660=CARTESIAN_POINT('Origin',(-5.8066065036801,-5.42357398527959,-28.98)) ;
#166661=CARTESIAN_POINT('Origin',(-5.17275707706437,-5.26511162862565,-28.98)) ;
#166662=CARTESIAN_POINT('Origin',(-5.15068655017073,-5.25959399690224,-28.9905938529089)) ;
#166663=CARTESIAN_POINT('Origin',(-5.17275707706436,-5.26511162862565,-28.98)) ;
#166664=CARTESIAN_POINT('Origin',(-5.17275707706436,-5.26511162862565,-28.98)) ;
#166665=CARTESIAN_POINT('Origin',(-5.17275707706436,-5.26511162862565,-28.98)) ;
#166666=CARTESIAN_POINT('Origin',(-5.17275707706436,-5.05,-28.98)) ;
#166667=CARTESIAN_POINT('Origin',(-5.17275707706436,-1.91866427917294,-28.98)) ;
#166668=CARTESIAN_POINT('Origin',(-3.78014014831103,-3.31128120792626,-29.6484561258016)) ;
#166669=CARTESIAN_POINT('Origin',(-5.17275707706436,-1.91866427917294,-28.98)) ;
#166670=CARTESIAN_POINT('Origin',(-5.17275707706436,-1.91866427917293,-28.98)) ;
#166671=CARTESIAN_POINT('Origin',(-5.17275707706436,-1.91866427917294,-28.98)) ;
#166672=CARTESIAN_POINT('Origin',(-3.97071067811865,-3.12071067811865,-28.98)) ;
#166673=CARTESIAN_POINT('Origin',(-5.8,-1.2914213562373,-28.98)) ;
#166674=CARTESIAN_POINT('Ctrl Pts',(-5.87071067811865,-1.14999999999999,
-28.8507106781187)) ;
#166675=CARTESIAN_POINT('Ctrl Pts',(-5.8471404520791,-1.10285954792089,
-28.8742809041582)) ;
#166676=CARTESIAN_POINT('Ctrl Pts',(-5.87071067811865,-1.07928932188134,
-28.9214213562373)) ;
#166677=CARTESIAN_POINT('Ctrl Pts',(-5.85217562795658,-1.18707010095451,
-28.8692457282807)) ;
#166678=CARTESIAN_POINT('Ctrl Pts',(-5.81261165662082,-1.1373883433793,
-28.8958614719498)) ;
#166679=CARTESIAN_POINT('Ctrl Pts',(-5.8335394967105,-1.11646050328949,
-28.9585925363811)) ;
#166680=CARTESIAN_POINT('Ctrl Pts',(-5.82627077431945,-1.23887980759835,
-28.88)) ;
#166681=CARTESIAN_POINT('Ctrl Pts',(-5.76566787907959,-1.18433212092071,
-28.8971489437127)) ;
#166682=CARTESIAN_POINT('Ctrl Pts',(-5.78190678732228,-1.16809321267771,
-28.9799999994186)) ;
#166683=CARTESIAN_POINT('Ctrl Pts',(-5.8,-1.2914213562373,-28.88)) ;
#166684=CARTESIAN_POINT('Ctrl Pts',(-5.72928932188134,-1.22071067811865,
-28.88)) ;
#166685=CARTESIAN_POINT('Ctrl Pts',(-5.72928932188134,-1.22071067811865,
-28.98)) ;
#166686=CARTESIAN_POINT('Origin',(-5.94142135623731,-1.15,-28.9214213562373)) ;
#166687=CARTESIAN_POINT('Ctrl Pts',(-5.9,-1.00857864376269,-28.78)) ;
#166688=CARTESIAN_POINT('Ctrl Pts',(-5.9,-1.00857864376269,-28.78)) ;
#166689=CARTESIAN_POINT('Ctrl Pts',(-5.9,-1.00857864376269,-28.78)) ;
#166690=CARTESIAN_POINT('Ctrl Pts',(-5.9,-1.06112019240163,-28.8062707743195)) ;
#166691=CARTESIAN_POINT('Ctrl Pts',(-5.9,-1.04860238144513,-28.8200237376833)) ;
#166692=CARTESIAN_POINT('Ctrl Pts',(-5.9,-1.03484941808214,-28.832541548639)) ;
#166693=CARTESIAN_POINT('Ctrl Pts',(-5.8892457282807,-1.11292989904544,
-28.8321756279566)) ;
#166694=CARTESIAN_POINT('Ctrl Pts',(-5.8745170062612,-1.08721613123966,
-28.8586374874774)) ;
#166695=CARTESIAN_POINT('Ctrl Pts',(-5.88924572828062,-1.06075427171937,
-28.8843512552826)) ;
#166696=CARTESIAN_POINT('Ctrl Pts',(-5.87071067811865,-1.14999999999999,
-28.8507106781187)) ;
#166697=CARTESIAN_POINT('Ctrl Pts',(-5.8471404520791,-1.10285954792089,
-28.8742809041582)) ;
#166698=CARTESIAN_POINT('Ctrl Pts',(-5.87071067811865,-1.07928932188134,
-28.9214213562373)) ;
#166699=CARTESIAN_POINT('Ctrl Pts',(-5.87071067811866,-1.14999999999999,
-32.1092893218813)) ;
#166700=CARTESIAN_POINT('Ctrl Pts',(-5.8471404520791,-1.10285954792089,
-32.0857190958418)) ;
#166701=CARTESIAN_POINT('Ctrl Pts',(-5.87071067811866,-1.07928932188134,
-32.0385786437627)) ;
#166702=CARTESIAN_POINT('Ctrl Pts',(-5.88924572828049,-1.11292989904507,
-32.1278243720432)) ;
#166703=CARTESIAN_POINT('Ctrl Pts',(-5.87451700624374,-1.08721613124994,
-32.1013625125115)) ;
#166704=CARTESIAN_POINT('Ctrl Pts',(-5.88924572828073,-1.06075427171926,
-32.0756487447172)) ;
#166705=CARTESIAN_POINT('Ctrl Pts',(-5.9,-1.06112019240149,-32.1537292256798)) ;
#166706=CARTESIAN_POINT('Ctrl Pts',(-5.9,-1.04860238143642,-32.1399762623248)) ;
#166707=CARTESIAN_POINT('Ctrl Pts',(-5.9,-1.03484941808206,-32.127458451361)) ;
#166708=CARTESIAN_POINT('Ctrl Pts',(-5.9,-1.00857864376269,-32.18)) ;
#166709=CARTESIAN_POINT('Ctrl Pts',(-5.9,-1.00857864376269,-32.18)) ;
#166710=CARTESIAN_POINT('Ctrl Pts',(-5.9,-1.00857864376269,-32.18)) ;
#166711=CARTESIAN_POINT('Origin',(-5.94142135623734,-1.14999999999996,-32.0385786437627)) ;
#166712=CARTESIAN_POINT('Ctrl Pts',(-5.8,-1.2914213562373,-32.08)) ;
#166713=CARTESIAN_POINT('Ctrl Pts',(-5.72928932188134,-1.22071067811865,
-32.08)) ;
#166714=CARTESIAN_POINT('Ctrl Pts',(-5.72928932188134,-1.22071067811865,
-31.98)) ;
#166715=CARTESIAN_POINT('Ctrl Pts',(-5.82627077431952,-1.2388798075982,
-32.08)) ;
#166716=CARTESIAN_POINT('Ctrl Pts',(-5.76566787907932,-1.18433212092069,
-32.0628510562865)) ;
#166717=CARTESIAN_POINT('Ctrl Pts',(-5.7819067873223,-1.16809321267769,
-31.9800000005809)) ;
#166718=CARTESIAN_POINT('Ctrl Pts',(-5.8521756279568,-1.18707010095488,
-32.0907542717195)) ;
#166719=CARTESIAN_POINT('Ctrl Pts',(-5.81261165662085,-1.13738834337918,
-32.0641385280509)) ;
#166720=CARTESIAN_POINT('Ctrl Pts',(-5.83353949671049,-1.11646050328951,
-32.0014074636193)) ;
#166721=CARTESIAN_POINT('Ctrl Pts',(-5.87071067811865,-1.14999999999999,
-32.1092893218813)) ;
#166722=CARTESIAN_POINT('Ctrl Pts',(-5.8471404520791,-1.10285954792089,
-32.0857190958418)) ;
#166723=CARTESIAN_POINT('Ctrl Pts',(-5.87071067811866,-1.07928932188134,
-32.0385786437627)) ;
#166724=CARTESIAN_POINT('Origin',(-5.8,-1.29142135623731,-31.98)) ;
#166725=CARTESIAN_POINT('Origin',(-3.59571067811865,-3.49571067811865,-31.98)) ;
#166726=CARTESIAN_POINT('Origin',(-5.17275707706436,-1.91866427917294,-31.98)) ;
#166727=CARTESIAN_POINT('Origin',(-3.09057773798104,-4.00084361825625,-30.98055391724)) ;
#166728=CARTESIAN_POINT('Origin',(-5.17275707706435,-1.91866427917295,-31.98)) ;
#166729=CARTESIAN_POINT('Origin',(-5.17275707706435,-1.91866427917295,-31.98)) ;
#166730=CARTESIAN_POINT('Origin',(-5.17275707706435,-1.91866427917295,-31.98)) ;
#166731=CARTESIAN_POINT('Origin',(-5.17275707706435,-5.05,-31.98)) ;
#166732=CARTESIAN_POINT('Origin',(-5.17275707706435,-5.26511162862565,-31.98)) ;
#166733=CARTESIAN_POINT('Origin',(-3.96111272388873,-4.96220054033175,-31.3984107104757)) ;
#166734=CARTESIAN_POINT('Origin',(-5.17275707706435,-5.26511162862565,-31.98)) ;
#166735=CARTESIAN_POINT('Origin',(-5.17275707706435,-5.26511162862565,-31.98)) ;
#166736=CARTESIAN_POINT('Origin',(-5.17275707706435,-5.26511162862565,-31.98)) ;
#166737=CARTESIAN_POINT('Origin',(-5.10072415073893,-5.24710339704429,-31.98)) ;
#166738=CARTESIAN_POINT('Origin',(-5.8,-5.42192235935956,-31.98)) ;
#166739=CARTESIAN_POINT('Ctrl Pts',(-5.77574643749636,-5.51893660937409,
-31.98)) ;
#166740=CARTESIAN_POINT('Ctrl Pts',(-5.77574643749636,-5.51893660937409,
-32.08)) ;
#166741=CARTESIAN_POINT('Ctrl Pts',(-5.8,-5.42192235935956,-32.08)) ;
#166742=CARTESIAN_POINT('Ctrl Pts',(-5.79207992677987,-5.52301998169497,
-31.980000000466)) ;
#166743=CARTESIAN_POINT('Ctrl Pts',(-5.78430903206628,-5.52107725801656,
-32.078038604567)) ;
#166744=CARTESIAN_POINT('Ctrl Pts',(-5.80816665318301,-5.42600568595105,
-32.08)) ;
#166745=CARTESIAN_POINT('Ctrl Pts',(-5.80840777707098,-5.52710194426775,
-31.9820100540956)) ;
#166746=CARTESIAN_POINT('Ctrl Pts',(-5.79341417645243,-5.52335354411312,
-32.0771641501814)) ;
#166747=CARTESIAN_POINT('Ctrl Pts',(-5.81633079157286,-5.43008775511761,
-32.0810050572528)) ;
#166748=CARTESIAN_POINT('Ctrl Pts',(-5.82425356250363,-5.53106339062591,
-31.9859714999709)) ;
#166749=CARTESIAN_POINT('Ctrl Pts',(-5.80269484027818,-5.52567371006955,
-32.0775960694291)) ;
#166750=CARTESIAN_POINT('Ctrl Pts',(-5.82425356250363,-5.43404914061138,
-32.0829857499855)) ;
#166751=CARTESIAN_POINT('Origin',(-5.84850712500726,-5.43404914061138,-31.9859714999709)) ;
#166752=CARTESIAN_POINT('Ctrl Pts',(-5.82426676739357,-5.5310666746717,
-31.9859153963653)) ;
#166753=CARTESIAN_POINT('Ctrl Pts',(-5.80266988778296,-5.52572362329017,
-32.0776459661893)) ;
#166754=CARTESIAN_POINT('Ctrl Pts',(-5.82426676352028,-5.43399305345725,
-32.0829890330731)) ;
#166755=CARTESIAN_POINT('Ctrl Pts',(-5.83498671931132,-5.53374818244432,
-31.9912758712783)) ;
#166756=CARTESIAN_POINT('Ctrl Pts',(-5.80595263122238,-5.5241175471004,
-32.0760398908369)) ;
#166757=CARTESIAN_POINT('Ctrl Pts',(-5.83498671397641,-5.4393535274937,
-32.0856705400343)) ;
#166758=CARTESIAN_POINT('Ctrl Pts',(-5.84526105845724,-5.53822480044432,
-32.0002256222542)) ;
#166759=CARTESIAN_POINT('Ctrl Pts',(-5.81370932746113,-5.52260133464156,
-32.0745236796683)) ;
#166760=CARTESIAN_POINT('Ctrl Pts',(-5.84526105243737,-5.44830327707024,
-32.0901471568231)) ;
#166761=CARTESIAN_POINT('Ctrl Pts',(-5.86378685403709,-5.55027438933185,
-32.0243225636634)) ;
#166762=CARTESIAN_POINT('Ctrl Pts',(-5.83531854275266,-5.52733068552581,
-32.0792530334047)) ;
#166763=CARTESIAN_POINT('Ctrl Pts',(-5.86378684816477,-5.47240021563463,
-32.1021967439587)) ;
#166764=CARTESIAN_POINT('Ctrl Pts',(-5.87203852631586,-5.55784608774616,
-32.0394673107066)) ;
#166765=CARTESIAN_POINT('Ctrl Pts',(-5.84834787930667,-5.53310200486441,
-32.085024354264)) ;
#166766=CARTESIAN_POINT('Ctrl Pts',(-5.8720385212305,-5.48754496112624,
-32.1097684417943)) ;
#166767=CARTESIAN_POINT('Ctrl Pts',(-5.89242747304801,-5.58397198950293,
-32.0917343826941)) ;
#166768=CARTESIAN_POINT('Ctrl Pts',(-5.88223383300416,-5.56084219746613,
-32.1127645511526)) ;
#166769=CARTESIAN_POINT('Ctrl Pts',(-5.89242747063516,-5.53981202831248,
-32.1358943433876)) ;
#166770=CARTESIAN_POINT('Ctrl Pts',(-5.9,-5.60595824049754,-32.1357331988324)) ;
#166771=CARTESIAN_POINT('Ctrl Pts',(-5.9,-5.59485304775361,-32.1467754043864)) ;
#166772=CARTESIAN_POINT('Ctrl Pts',(-5.9,-5.58381084219965,-32.1578805971149)) ;
#166773=CARTESIAN_POINT('Ctrl Pts',(-5.9,-5.62807764064044,-32.18)) ;
#166774=CARTESIAN_POINT('Ctrl Pts',(-5.9,-5.62807764064044,-32.18)) ;
#166775=CARTESIAN_POINT('Ctrl Pts',(-5.9,-5.62807764064044,-32.18)) ;
#166776=CARTESIAN_POINT('Origin',(7.8,2.1,-30.88)) ;
#166777=CARTESIAN_POINT('Origin',(7.8,2.1,-31.08)) ;
#166778=CARTESIAN_POINT('Origin',(7.6,2.1,-30.88)) ;
#166779=CARTESIAN_POINT('Origin',(7.6,2.1,-30.88)) ;
#166780=CARTESIAN_POINT('Origin',(7.6,2.1,-30.08)) ;
#166781=CARTESIAN_POINT('Origin',(7.8,2.1,-31.08)) ;
#166782=CARTESIAN_POINT('Origin',(9.6,2.1,-31.08)) ;
#166783=CARTESIAN_POINT('Origin',(7.8,2.1,-30.08)) ;
#166784=CARTESIAN_POINT('Origin',(7.8,2.1,-29.88)) ;
#166785=CARTESIAN_POINT('Origin',(9.6,2.1,-30.88)) ;
#166786=CARTESIAN_POINT('Origin',(9.8,2.1,-30.88)) ;
#166787=CARTESIAN_POINT('Origin',(7.8,2.1,-29.88)) ;
#166788=CARTESIAN_POINT('Origin',(9.6,2.1,-29.88)) ;
#166789=CARTESIAN_POINT('Origin',(9.8,2.1,-30.88)) ;
#166790=CARTESIAN_POINT('Origin',(9.8,2.1,-30.08)) ;
#166791=CARTESIAN_POINT('Origin',(9.6,2.1,-30.08)) ;
#166792=CARTESIAN_POINT('Origin',(-4.15,-6.25,-29.73)) ;
#166793=CARTESIAN_POINT('Origin',(-4.15,-6.3,-29.73)) ;
#166794=CARTESIAN_POINT('Origin',(-4.15,-6.3,-30.48)) ;
#166795=CARTESIAN_POINT('Origin',(-4.15,-6.3,-31.23)) ;
#166796=CARTESIAN_POINT('Origin',(-4.15,-6.3,-29.73)) ;
#166797=CARTESIAN_POINT('Origin',(-4.15,-6.25,-31.23)) ;
#166798=CARTESIAN_POINT('Origin',(-4.15,-6.3,-31.23)) ;
#166799=CARTESIAN_POINT('Origin',(-4.15,-6.3,-29.73)) ;
#166800=CARTESIAN_POINT('Origin',(-4.15,-6.3,-29.73)) ;
#166801=CARTESIAN_POINT('Origin',(-4.15,-6.3,-31.23)) ;
#166802=CARTESIAN_POINT('Origin',(-4.15,-6.3,-31.23)) ;
#166803=CARTESIAN_POINT('Origin',(-4.65,-6.25,-29.73)) ;
#166804=CARTESIAN_POINT('Origin',(-4.65,-6.3,-29.73)) ;
#166805=CARTESIAN_POINT('Origin',(0.,-6.3,-29.73)) ;
#166806=CARTESIAN_POINT('Origin',(-4.65,-6.3,-29.73)) ;
#166807=CARTESIAN_POINT('Origin',(0.,-6.3,-31.23)) ;
#166808=CARTESIAN_POINT('Origin',(-4.65,-6.3,-31.23)) ;
#166809=CARTESIAN_POINT('Origin',(-4.65,-6.25,-31.23)) ;
#166810=CARTESIAN_POINT('Origin',(-4.65,-6.3,-31.23)) ;
#166811=CARTESIAN_POINT('Origin',(-4.65,-6.3,-29.73)) ;
#166812=CARTESIAN_POINT('Origin',(-4.65,-6.3,-29.73)) ;
#166813=CARTESIAN_POINT('Origin',(-4.65,-6.3,-31.23)) ;
#166814=CARTESIAN_POINT('Origin',(-4.65,-6.3,-31.23)) ;
#166815=CARTESIAN_POINT('Origin',(-4.65,-6.3,-30.48)) ;
#166816=CARTESIAN_POINT('Origin',(-3.,4.45,-31.58)) ;
#166817=CARTESIAN_POINT('Origin',(-2.1,4.45,-31.58)) ;
#166818=CARTESIAN_POINT('Origin',(-2.9,4.45,-31.58)) ;
#166819=CARTESIAN_POINT('Origin',(-2.9,4.45,-31.38)) ;
#166820=CARTESIAN_POINT('Origin',(-3.1,4.45,-31.38)) ;
#166821=CARTESIAN_POINT('Origin',(-2.9,4.45,-31.38)) ;
#166822=CARTESIAN_POINT('Origin',(-2.1,4.45,-31.38)) ;
#166823=CARTESIAN_POINT('Origin',(-2.1,4.45,-31.38)) ;
#166824=CARTESIAN_POINT('Origin',(-1.9,4.45,-31.38)) ;
#166825=CARTESIAN_POINT('Origin',(-3.1,4.45,-31.48)) ;
#166826=CARTESIAN_POINT('Origin',(-3.1,4.45,-29.58)) ;
#166827=CARTESIAN_POINT('Origin',(-2.9,4.4,-31.38)) ;
#166828=CARTESIAN_POINT('Origin',(-2.9,4.35,-31.38)) ;
#166829=CARTESIAN_POINT('Origin',(-1.95156391047391E-16,4.35,-31.38)) ;
#166830=CARTESIAN_POINT('Origin',(-2.1,4.35,-31.38)) ;
#166831=CARTESIAN_POINT('Origin',(-2.9,4.35,-31.38)) ;
#166832=CARTESIAN_POINT('Origin',(-2.1,4.4,-31.38)) ;
#166833=CARTESIAN_POINT('Origin',(-2.1,4.35,-31.38)) ;
#166834=CARTESIAN_POINT('Origin',(-1.9,4.45,-31.48)) ;
#166835=CARTESIAN_POINT('Origin',(-1.9,4.45,-29.58)) ;
#166836=CARTESIAN_POINT('Origin',(-3.,4.45,-29.38)) ;
#166837=CARTESIAN_POINT('Origin',(-2.9,4.45,-29.38)) ;
#166838=CARTESIAN_POINT('Origin',(-2.1,4.45,-29.38)) ;
#166839=CARTESIAN_POINT('Origin',(-2.9,4.45,-29.58)) ;
#166840=CARTESIAN_POINT('Origin',(-2.9,4.45,-29.58)) ;
#166841=CARTESIAN_POINT('Origin',(-2.9,4.35,-31.38)) ;
#166842=CARTESIAN_POINT('Origin',(-2.9,4.35,-31.38)) ;
#166843=CARTESIAN_POINT('Origin',(-2.1,4.35,-31.38)) ;
#166844=CARTESIAN_POINT('Origin',(-2.1,4.35,-31.38)) ;
#166845=CARTESIAN_POINT('Origin',(-2.1,4.45,-29.58)) ;
#166846=CARTESIAN_POINT('Origin',(-2.1,4.45,-29.58)) ;
#166847=CARTESIAN_POINT('Origin',(-2.9,4.4,-29.58)) ;
#166848=CARTESIAN_POINT('Origin',(-2.9,4.35,-29.58)) ;
#166849=CARTESIAN_POINT('Origin',(-2.9,4.35,-30.48)) ;
#166850=CARTESIAN_POINT('Origin',(-2.9,4.35,-29.58)) ;
#166851=CARTESIAN_POINT('Origin',(-2.1,4.35,-30.48)) ;
#166852=CARTESIAN_POINT('Origin',(-2.1,4.35,-29.58)) ;
#166853=CARTESIAN_POINT('Origin',(-2.1,4.4,-29.58)) ;
#166854=CARTESIAN_POINT('Origin',(-2.1,4.35,-29.58)) ;
#166855=CARTESIAN_POINT('Origin',(-2.9,4.35,-29.58)) ;
#166856=CARTESIAN_POINT('Origin',(-2.9,4.35,-29.58)) ;
#166857=CARTESIAN_POINT('Origin',(-2.1,4.35,-29.58)) ;
#166858=CARTESIAN_POINT('Origin',(-2.1,4.35,-29.58)) ;
#166859=CARTESIAN_POINT('Origin',(-1.95156391047391E-16,4.35,-29.58)) ;
#166860=CARTESIAN_POINT('Origin',(-2.25,4.25,-31.23)) ;
#166861=CARTESIAN_POINT('Origin',(-2.25,4.3,-31.23)) ;
#166862=CARTESIAN_POINT('Origin',(-2.25,4.3,-30.48)) ;
#166863=CARTESIAN_POINT('Origin',(-2.25,4.3,-29.73)) ;
#166864=CARTESIAN_POINT('Origin',(-2.25,4.3,-31.23)) ;
#166865=CARTESIAN_POINT('Origin',(-2.25,4.25,-29.73)) ;
#166866=CARTESIAN_POINT('Origin',(-2.25,4.3,-29.73)) ;
#166867=CARTESIAN_POINT('Origin',(-2.25,4.3,-31.23)) ;
#166868=CARTESIAN_POINT('Origin',(-2.25,4.3,-31.23)) ;
#166869=CARTESIAN_POINT('Origin',(-2.25,4.3,-29.73)) ;
#166870=CARTESIAN_POINT('Origin',(-2.25,4.3,-29.73)) ;
#166871=CARTESIAN_POINT('Origin',(-2.75,4.25,-31.23)) ;
#166872=CARTESIAN_POINT('Origin',(-2.75,4.3,-31.23)) ;
#166873=CARTESIAN_POINT('Origin',(-1.97127667724637E-17,4.3,-31.23)) ;
#166874=CARTESIAN_POINT('Origin',(-2.75,4.3,-31.23)) ;
#166875=CARTESIAN_POINT('Origin',(-1.97127667724637E-17,4.3,-29.73)) ;
#166876=CARTESIAN_POINT('Origin',(-2.75,4.3,-29.73)) ;
#166877=CARTESIAN_POINT('Origin',(-2.75,4.25,-29.73)) ;
#166878=CARTESIAN_POINT('Origin',(-2.75,4.3,-29.73)) ;
#166879=CARTESIAN_POINT('Origin',(-2.75,4.3,-31.23)) ;
#166880=CARTESIAN_POINT('Origin',(-2.75,4.3,-31.23)) ;
#166881=CARTESIAN_POINT('Origin',(-2.75,4.3,-29.73)) ;
#166882=CARTESIAN_POINT('Origin',(-2.75,4.3,-29.73)) ;
#166883=CARTESIAN_POINT('Origin',(-2.75,4.3,-30.48)) ;
#166884=CARTESIAN_POINT('Origin',(7.8,2.9,-30.88)) ;
#166885=CARTESIAN_POINT('Origin',(7.8,2.9,-30.88)) ;
#166886=CARTESIAN_POINT('Origin',(7.8,2.9,-30.08)) ;
#166887=CARTESIAN_POINT('Origin',(7.8,2.9,-30.08)) ;
#166888=CARTESIAN_POINT('Origin',(7.8,2.9,-30.08)) ;
#166889=CARTESIAN_POINT('Origin',(7.8,2.9,-30.88)) ;
#166890=CARTESIAN_POINT('Origin',(7.8,2.9,-30.88)) ;
#166891=CARTESIAN_POINT('Origin',(9.6,2.9,-30.08)) ;
#166892=CARTESIAN_POINT('Origin',(9.6,2.9,-30.08)) ;
#166893=CARTESIAN_POINT('Origin',(9.6,2.9,-30.88)) ;
#166894=CARTESIAN_POINT('Origin',(9.6,2.9,-30.88)) ;
#166895=CARTESIAN_POINT('Origin',(9.6,2.9,-30.08)) ;
#166896=CARTESIAN_POINT('Origin',(9.6,2.9,-30.08)) ;
#166897=CARTESIAN_POINT('Origin',(9.6,2.9,-30.88)) ;
#166898=CARTESIAN_POINT('Origin',(9.6,2.9,-30.88)) ;
#166899=CARTESIAN_POINT('Origin',(9.6,2.9,-30.88)) ;
#166900=CARTESIAN_POINT('Origin',(-0.183301359729408,3.45,-28.962963213524)) ;
#166901=CARTESIAN_POINT('Origin',(0.24923464143508,3.15,-30.3637799780213)) ;
#166902=CARTESIAN_POINT('Origin',(-0.249234641435079,3.15,-30.5962200219787)) ;
#166903=CARTESIAN_POINT('Origin',(-1.04429375741423,3.45,-29.3644505621777)) ;
#166904=CARTESIAN_POINT('Origin',(10.1,-2.15,-33.3868804065906)) ;
#166905=CARTESIAN_POINT('Origin',(10.1,-2.15,-33.3868804065906)) ;
#166906=CARTESIAN_POINT('Origin',(10.1,-2.15,-33.3868804065906)) ;
#166907=CARTESIAN_POINT('Origin',(10.1,-2.15,-33.3868804065906)) ;
#166908=CARTESIAN_POINT('Origin',(10.1,-2.15,-34.29)) ;
#166909=CARTESIAN_POINT('Origin',(10.1,-2.15,-32.985)) ;
#166910=CARTESIAN_POINT('Origin',(10.2,-2.15,-33.3868804065906)) ;
#166911=CARTESIAN_POINT('Origin',(3.7,-2.15,-33.3868804065906)) ;
#166912=CARTESIAN_POINT('Origin',(10.1,-3.65625,-34.29)) ;
#166913=CARTESIAN_POINT('Origin',(10.1,-2.15,-35.1931195934094)) ;
#166914=CARTESIAN_POINT('Origin',(10.1,-3.65625,-32.985)) ;
#166915=CARTESIAN_POINT('Origin',(10.1,1.9,-32.985)) ;
#166916=CARTESIAN_POINT('Origin',(10.1,-2.15,-32.985)) ;
#166917=CARTESIAN_POINT('Origin',(10.1,-2.15,-32.985)) ;
#166918=CARTESIAN_POINT('Origin',(10.1,-2.15,-32.985)) ;
#166919=CARTESIAN_POINT('Origin',(3.7,-2.15,-33.3868804065906)) ;
#166920=CARTESIAN_POINT('Origin',(3.7,-2.32153024911032,-33.4897267659824)) ;
#166921=CARTESIAN_POINT('Origin',(3.7,-2.35,-33.3868804065906)) ;
#166922=CARTESIAN_POINT('Origin',(10.1,-2.15,-35.1931195934094)) ;
#166923=CARTESIAN_POINT('Origin',(10.1,-2.15,-35.1931195934094)) ;
#166924=CARTESIAN_POINT('Origin',(10.1,-2.15,-35.1931195934094)) ;
#166925=CARTESIAN_POINT('Origin',(10.1,1.9,-34.29)) ;
#166926=CARTESIAN_POINT('Origin',(10.1,1.9,-35.595)) ;
#166927=CARTESIAN_POINT('Origin',(10.1,1.9,-32.985)) ;
#166928=CARTESIAN_POINT('Origin',(10.2,-2.15,-32.985)) ;
#166929=CARTESIAN_POINT('Origin',(3.7,-2.15,-32.985)) ;
#166930=CARTESIAN_POINT('Origin',(3.7,-2.35,-32.885)) ;
#166931=CARTESIAN_POINT('Origin',(3.7,-2.35,-32.985)) ;
#166932=CARTESIAN_POINT('Origin',(3.7,-3.65625,-34.29)) ;
#166933=CARTESIAN_POINT('Origin',(3.7,-2.32153024911032,-35.0902732340176)) ;
#166934=CARTESIAN_POINT('Origin',(10.2,-2.15,-35.1931195934094)) ;
#166935=CARTESIAN_POINT('Origin',(3.7,-2.15,-35.1931195934094)) ;
#166936=CARTESIAN_POINT('Origin',(10.1,-2.15,-34.29)) ;
#166937=CARTESIAN_POINT('Origin',(10.1,-2.15,-35.595)) ;
#166938=CARTESIAN_POINT('Origin',(10.1,-3.65625,-35.595)) ;
#166939=CARTESIAN_POINT('Origin',(10.1,1.9,-35.595)) ;
#166940=CARTESIAN_POINT('Origin',(10.1,-2.15,-35.595)) ;
#166941=CARTESIAN_POINT('Origin',(3.7,-2.35,-32.985)) ;
#166942=CARTESIAN_POINT('Origin',(3.5,-2.35,-32.985)) ;
#166943=CARTESIAN_POINT('Origin',(3.7,-2.15,-35.1931195934094)) ;
#166944=CARTESIAN_POINT('Origin',(3.7,-2.35,-35.1931195934094)) ;
#166945=CARTESIAN_POINT('Origin',(10.1,-2.15,-35.595)) ;
#166946=CARTESIAN_POINT('Origin',(10.1,-2.15,-35.595)) ;
#166947=CARTESIAN_POINT('Origin',(3.6,1.9,-32.785)) ;
#166948=CARTESIAN_POINT('Origin',(3.5,1.9,-32.785)) ;
#166949=CARTESIAN_POINT('Origin',(2.7,1.9,-32.785)) ;
#166950=CARTESIAN_POINT('Origin',(3.5,3.03778831031064E-15,-32.985)) ;
#166951=CARTESIAN_POINT('Origin',(3.5,-5.15,-32.985)) ;
#166952=CARTESIAN_POINT('Origin',(3.7,-2.35,-35.165)) ;
#166953=CARTESIAN_POINT('Origin',(3.7,-2.35,-35.595)) ;
#166954=CARTESIAN_POINT('Origin',(3.6,-2.15,-35.595)) ;
#166955=CARTESIAN_POINT('Origin',(3.7,-2.15,-35.595)) ;
#166956=CARTESIAN_POINT('Origin',(2.7,1.9,-32.785)) ;
#166957=CARTESIAN_POINT('Origin',(2.7,1.9,-32.785)) ;
#166958=CARTESIAN_POINT('Origin',(3.5,-5.15,-32.985)) ;
#166959=CARTESIAN_POINT('Origin',(3.5,-5.15,-32.985)) ;
#166960=CARTESIAN_POINT('Origin',(3.5,-5.15,-32.985)) ;
#166961=CARTESIAN_POINT('Origin',(3.7,-2.35,-35.595)) ;
#166962=CARTESIAN_POINT('Origin',(3.5,-2.35,-35.595)) ;
#166963=CARTESIAN_POINT('Origin',(2.7,2.,-32.785)) ;
#166964=CARTESIAN_POINT('Origin',(2.7,-5.15,-32.785)) ;
#166965=CARTESIAN_POINT('Origin',(3.6,-5.15,-32.985)) ;
#166966=CARTESIAN_POINT('Origin',(2.7,-5.15,-32.985)) ;
#166967=CARTESIAN_POINT('Origin',(3.5,-5.15,0.)) ;
#166968=CARTESIAN_POINT('Origin',(3.5,-5.15,-35.595)) ;
#166969=CARTESIAN_POINT('Origin',(3.5,-3.11569458533536E-15,-35.595)) ;
#166970=CARTESIAN_POINT('Origin',(3.5,-5.15,-35.595)) ;
#166971=CARTESIAN_POINT('Origin',(2.7,-5.15,-32.985)) ;
#166972=CARTESIAN_POINT('Origin',(2.7,-5.35,-32.985)) ;
#166973=CARTESIAN_POINT('Origin',(3.5,-5.15,-35.595)) ;
#166974=CARTESIAN_POINT('Origin',(3.5,-5.15,-35.595)) ;
#166975=CARTESIAN_POINT('Origin',(2.7,-5.35,-32.885)) ;
#166976=CARTESIAN_POINT('Origin',(2.7,-5.35,-35.595)) ;
#166977=CARTESIAN_POINT('Origin',(3.6,-5.15,-35.595)) ;
#166978=CARTESIAN_POINT('Origin',(2.7,-5.15,-35.595)) ;
#166979=CARTESIAN_POINT('Origin',(3.6,1.9,-35.795)) ;
#166980=CARTESIAN_POINT('Origin',(3.5,1.9,-35.795)) ;
#166981=CARTESIAN_POINT('Origin',(2.7,1.9,-35.795)) ;
#166982=CARTESIAN_POINT('Origin',(2.7,1.9,-35.695)) ;
#166983=CARTESIAN_POINT('Origin',(2.7,1.9,-36.49)) ;
#166984=CARTESIAN_POINT('Origin',(2.7,1.9,-35.795)) ;
#166985=CARTESIAN_POINT('Origin',(2.7,-5.15,-35.595)) ;
#166986=CARTESIAN_POINT('Origin',(2.7,-5.15,-35.795)) ;
#166987=CARTESIAN_POINT('Origin',(2.7,1.9,-35.795)) ;
#166988=CARTESIAN_POINT('Origin',(2.7,1.9,-35.795)) ;
#166989=CARTESIAN_POINT('Origin',(2.7,-5.25,-35.795)) ;
#166990=CARTESIAN_POINT('Ctrl Pts',(-3.8,-6.55,-33.19)) ;
#166991=CARTESIAN_POINT('Ctrl Pts',(-3.8,-6.55,-33.19)) ;
#166992=CARTESIAN_POINT('Ctrl Pts',(-3.8,-6.55,-33.19)) ;
#166993=CARTESIAN_POINT('Ctrl Pts',(-3.8262534328263,-6.55,-33.2425068656528)) ;
#166994=CARTESIAN_POINT('Ctrl Pts',(-3.83954133268437,-6.55,-33.2295413326857)) ;
#166995=CARTESIAN_POINT('Ctrl Pts',(-3.85250686565253,-6.55,-33.2162534328268)) ;
#166996=CARTESIAN_POINT('Ctrl Pts',(-3.85219871729854,-6.53922263893877,
-33.294397434597)) ;
#166997=CARTESIAN_POINT('Ctrl Pts',(-3.87914655110985,-6.52362528614074,
-33.2691465511097)) ;
#166998=CARTESIAN_POINT('Ctrl Pts',(-3.90439743459708,-6.53922263893883,
-33.2421987172985)) ;
#166999=CARTESIAN_POINT('Ctrl Pts',(-3.87996665852871,-6.5114546977086,
-33.3499333170575)) ;
#167000=CARTESIAN_POINT('Ctrl Pts',(-3.90288380314158,-6.48208554016475,
-33.2928838031417)) ;
#167001=CARTESIAN_POINT('Ctrl Pts',(-3.95993331705742,-6.51145469770856,
-33.2699666585287)) ;
#167002=CARTESIAN_POINT('Ctrl Pts',(-3.88737865704135,-6.5003618540841,
-33.3647573140827)) ;
#167003=CARTESIAN_POINT('Ctrl Pts',(-3.90501307588292,-6.46792722356047,
-33.295013075883)) ;
#167004=CARTESIAN_POINT('Ctrl Pts',(-3.9747573140827,-6.5003618540841,-33.2773786570414)) ;
#167005=CARTESIAN_POINT('Ctrl Pts',(-3.8973972494609,-6.47617483238892,
-33.3847944989218)) ;
#167006=CARTESIAN_POINT('Ctrl Pts',(-3.90329674356411,-6.4509405986842,
-33.2932967435641)) ;
#167007=CARTESIAN_POINT('Ctrl Pts',(-3.99479449892181,-6.47617483238892,
-33.2873972494609)) ;
#167008=CARTESIAN_POINT('Ctrl Pts',(-3.9,-6.46309229646328,-33.3899999991819)) ;
#167009=CARTESIAN_POINT('Ctrl Pts',(-3.90000730394006,-6.44945650160767,
-33.2900073041287)) ;
#167010=CARTESIAN_POINT('Ctrl Pts',(-3.99999999918173,-6.46309229646328,
-33.29)) ;
#167011=CARTESIAN_POINT('Ctrl Pts',(-3.9,-6.45,-33.39)) ;
#167012=CARTESIAN_POINT('Ctrl Pts',(-3.9,-6.45,-33.29)) ;
#167013=CARTESIAN_POINT('Ctrl Pts',(-4.,-6.45,-33.29)) ;
#167014=CARTESIAN_POINT('Origin',(-4.,-6.45,-33.39)) ;
#167015=CARTESIAN_POINT('Origin',(-4.,-6.4,-33.39)) ;
#167016=CARTESIAN_POINT('Origin',(-4.,-6.35,-33.39)) ;
#167017=CARTESIAN_POINT('Ctrl Pts',(-5.,-6.55,-33.19)) ;
#167018=CARTESIAN_POINT('Ctrl Pts',(-5.,-6.55,-33.19)) ;
#167019=CARTESIAN_POINT('Ctrl Pts',(-5.,-6.55,-33.19)) ;
#167020=CARTESIAN_POINT('Ctrl Pts',(-4.94749313434715,-6.55,-33.2162534328261)) ;
#167021=CARTESIAN_POINT('Ctrl Pts',(-4.96045866731563,-6.55,-33.2295413326835)) ;
#167022=CARTESIAN_POINT('Ctrl Pts',(-4.97374656717363,-6.55,-33.2425068656528)) ;
#167023=CARTESIAN_POINT('Ctrl Pts',(-4.89560256540291,-6.53922263893883,
-33.2421987172985)) ;
#167024=CARTESIAN_POINT('Ctrl Pts',(-4.92085344889015,-6.52362528614069,
-33.2691465511097)) ;
#167025=CARTESIAN_POINT('Ctrl Pts',(-4.94780128270146,-6.53922263893877,
-33.294397434597)) ;
#167026=CARTESIAN_POINT('Ctrl Pts',(-4.84006668294258,-6.51145469770856,
-33.2699666585287)) ;
#167027=CARTESIAN_POINT('Ctrl Pts',(-4.89711619685841,-6.48208554016478,
-33.2928838031417)) ;
#167028=CARTESIAN_POINT('Ctrl Pts',(-4.92003334147129,-6.5114546977086,
-33.3499333170575)) ;
#167029=CARTESIAN_POINT('Ctrl Pts',(-4.82524268591729,-6.5003618540841,
-33.2773786570414)) ;
#167030=CARTESIAN_POINT('Ctrl Pts',(-4.89498692411706,-6.46792722356049,
-33.2950130758829)) ;
#167031=CARTESIAN_POINT('Ctrl Pts',(-4.91262134295865,-6.5003618540841,
-33.3647573140827)) ;
#167032=CARTESIAN_POINT('Ctrl Pts',(-4.80520550107819,-6.47617483238892,
-33.2873972494609)) ;
#167033=CARTESIAN_POINT('Ctrl Pts',(-4.8967032564359,-6.45094059868419,
-33.2932967435641)) ;
#167034=CARTESIAN_POINT('Ctrl Pts',(-4.90260275053909,-6.47617483238892,
-33.3847944989218)) ;
#167035=CARTESIAN_POINT('Ctrl Pts',(-4.80000000081823,-6.46309229646328,
-33.29)) ;
#167036=CARTESIAN_POINT('Ctrl Pts',(-4.89999269604099,-6.44945650161557,
-33.2900073041287)) ;
#167037=CARTESIAN_POINT('Ctrl Pts',(-4.9,-6.46309229646328,-33.3899999991819)) ;
#167038=CARTESIAN_POINT('Ctrl Pts',(-4.8,-6.45,-33.29)) ;
#167039=CARTESIAN_POINT('Ctrl Pts',(-4.9,-6.45,-33.29)) ;
#167040=CARTESIAN_POINT('Ctrl Pts',(-4.9,-6.45,-33.39)) ;
#167041=CARTESIAN_POINT('Origin',(-4.8,-6.45,-33.39)) ;
#167042=CARTESIAN_POINT('Origin',(-4.,-6.35,-33.39)) ;
#167043=CARTESIAN_POINT('Origin',(-4.,-6.35,-33.39)) ;
#167044=CARTESIAN_POINT('Origin',(-4.,-6.35,-33.39)) ;
#167045=CARTESIAN_POINT('Ctrl Pts',(-3.8,-6.55,-35.39)) ;
#167046=CARTESIAN_POINT('Ctrl Pts',(-3.8,-6.55,-35.39)) ;
#167047=CARTESIAN_POINT('Ctrl Pts',(-3.8,-6.55,-35.39)) ;
#167048=CARTESIAN_POINT('Ctrl Pts',(-3.85250686565255,-6.55,-35.3637465671732)) ;
#167049=CARTESIAN_POINT('Ctrl Pts',(-3.83954133268437,-6.55,-35.3504586673145)) ;
#167050=CARTESIAN_POINT('Ctrl Pts',(-3.82625343282626,-6.55,-35.3374931343472)) ;
#167051=CARTESIAN_POINT('Ctrl Pts',(-3.90439743459706,-6.53922263893883,
-35.3378012827015)) ;
#167052=CARTESIAN_POINT('Ctrl Pts',(-3.87914655110982,-6.52362528614068,
-35.3108534488903)) ;
#167053=CARTESIAN_POINT('Ctrl Pts',(-3.85219871729855,-6.53922263893876,
-35.285602565403)) ;
#167054=CARTESIAN_POINT('Ctrl Pts',(-3.95993331705743,-6.51145469770856,
-35.3100333414713)) ;
#167055=CARTESIAN_POINT('Ctrl Pts',(-3.9028838031416,-6.48208554016478,
-35.2871161968583)) ;
#167056=CARTESIAN_POINT('Ctrl Pts',(-3.8799666585287,-6.5114546977086,-35.2300666829425)) ;
#167057=CARTESIAN_POINT('Ctrl Pts',(-3.97475731408271,-6.5003618540841,
-35.3026213429587)) ;
#167058=CARTESIAN_POINT('Ctrl Pts',(-3.90501307588293,-6.46792722356049,
-35.284986924117)) ;
#167059=CARTESIAN_POINT('Ctrl Pts',(-3.88737865704135,-6.5003618540841,
-35.2152426859173)) ;
#167060=CARTESIAN_POINT('Ctrl Pts',(-3.9947944989218,-6.47617483238892,
-35.2926027505391)) ;
#167061=CARTESIAN_POINT('Ctrl Pts',(-3.9032967435641,-6.45094059868419,
-35.2867032564359)) ;
#167062=CARTESIAN_POINT('Ctrl Pts',(-3.89739724946091,-6.47617483238892,
-35.1952055010782)) ;
#167063=CARTESIAN_POINT('Ctrl Pts',(-3.99999999918176,-6.46309229646328,
-35.29)) ;
#167064=CARTESIAN_POINT('Ctrl Pts',(-3.90000730395432,-6.44945650161364,
-35.2899926958712)) ;
#167065=CARTESIAN_POINT('Ctrl Pts',(-3.9,-6.46309229646328,-35.1900000008181)) ;
#167066=CARTESIAN_POINT('Ctrl Pts',(-4.,-6.45,-35.29)) ;
#167067=CARTESIAN_POINT('Ctrl Pts',(-3.9,-6.45,-35.29)) ;
#167068=CARTESIAN_POINT('Ctrl Pts',(-3.9,-6.45,-35.19)) ;
#167069=CARTESIAN_POINT('Origin',(-4.,-6.45,-35.19)) ;
#167070=CARTESIAN_POINT('Origin',(-4.8,-6.4,-33.39)) ;
#167071=CARTESIAN_POINT('Origin',(-4.8,-6.35,-33.39)) ;
#167072=CARTESIAN_POINT('Origin',(1.9515639104739E-16,-6.35,-33.39)) ;
#167073=CARTESIAN_POINT('Origin',(-4.8,-6.35,-33.39)) ;
#167074=CARTESIAN_POINT('Origin',(-4.,-6.35,-34.29)) ;
#167075=CARTESIAN_POINT('Origin',(-4.,-6.35,-35.19)) ;
#167076=CARTESIAN_POINT('Origin',(-4.,-6.4,-35.19)) ;
#167077=CARTESIAN_POINT('Origin',(-4.,-6.35,-35.19)) ;
#167078=CARTESIAN_POINT('Origin',(-4.8,-6.35,-33.39)) ;
#167079=CARTESIAN_POINT('Origin',(-4.8,-6.35,-33.39)) ;
#167080=CARTESIAN_POINT('Origin',(-4.,-6.35,-35.19)) ;
#167081=CARTESIAN_POINT('Origin',(-4.,-6.35,-35.19)) ;
#167082=CARTESIAN_POINT('Origin',(-4.8,-6.35,-34.29)) ;
#167083=CARTESIAN_POINT('Origin',(-4.8,-6.35,-35.19)) ;
#167084=CARTESIAN_POINT('Origin',(1.9515639104739E-16,-6.35,-35.19)) ;
#167085=CARTESIAN_POINT('Origin',(-4.8,-6.35,-35.19)) ;
#167086=CARTESIAN_POINT('Origin',(-4.8,-6.35,-35.19)) ;
#167087=CARTESIAN_POINT('Origin',(-4.8,-6.35,-35.19)) ;
#167088=CARTESIAN_POINT('Origin',(-4.8,-6.4,-35.19)) ;
#167089=CARTESIAN_POINT('Origin',(-4.8,-6.45,-35.19)) ;
#167090=CARTESIAN_POINT('Ctrl Pts',(-5.,-6.55,-35.39)) ;
#167091=CARTESIAN_POINT('Ctrl Pts',(-5.,-6.55,-35.39)) ;
#167092=CARTESIAN_POINT('Ctrl Pts',(-5.,-6.55,-35.39)) ;
#167093=CARTESIAN_POINT('Ctrl Pts',(-4.97374656717363,-6.55,-35.3374931343472)) ;
#167094=CARTESIAN_POINT('Ctrl Pts',(-4.96045866731564,-6.55,-35.3504586673165)) ;
#167095=CARTESIAN_POINT('Ctrl Pts',(-4.94749313434714,-6.55,-35.3637465671739)) ;
#167096=CARTESIAN_POINT('Ctrl Pts',(-4.94780128270146,-6.53922263893877,
-35.285602565403)) ;
#167097=CARTESIAN_POINT('Ctrl Pts',(-4.92085344889015,-6.52362528614069,
-35.3108534488903)) ;
#167098=CARTESIAN_POINT('Ctrl Pts',(-4.89560256540291,-6.53922263893883,
-35.3378012827015)) ;
#167099=CARTESIAN_POINT('Ctrl Pts',(-4.92003334147129,-6.5114546977086,
-35.2300666829425)) ;
#167100=CARTESIAN_POINT('Ctrl Pts',(-4.89711619685841,-6.48208554016478,
-35.2871161968583)) ;
#167101=CARTESIAN_POINT('Ctrl Pts',(-4.84006668294258,-6.51145469770856,
-35.3100333414713)) ;
#167102=CARTESIAN_POINT('Ctrl Pts',(-4.91262134295865,-6.5003618540841,
-35.2152426859173)) ;
#167103=CARTESIAN_POINT('Ctrl Pts',(-4.89498692411706,-6.46792722356049,
-35.284986924117)) ;
#167104=CARTESIAN_POINT('Ctrl Pts',(-4.82524268591729,-6.5003618540841,
-35.3026213429587)) ;
#167105=CARTESIAN_POINT('Ctrl Pts',(-4.90260275053909,-6.47617483238892,
-35.1952055010782)) ;
#167106=CARTESIAN_POINT('Ctrl Pts',(-4.8967032564359,-6.45094059868419,
-35.2867032564359)) ;
#167107=CARTESIAN_POINT('Ctrl Pts',(-4.80520550107819,-6.47617483238892,
-35.2926027505391)) ;
#167108=CARTESIAN_POINT('Ctrl Pts',(-4.9,-6.46309229646328,-35.1900000008181)) ;
#167109=CARTESIAN_POINT('Ctrl Pts',(-4.89999269604099,-6.44945650161557,
-35.2899926958712)) ;
#167110=CARTESIAN_POINT('Ctrl Pts',(-4.80000000081823,-6.46309229646328,
-35.29)) ;
#167111=CARTESIAN_POINT('Ctrl Pts',(-4.9,-6.45,-35.19)) ;
#167112=CARTESIAN_POINT('Ctrl Pts',(-4.9,-6.45,-35.29)) ;
#167113=CARTESIAN_POINT('Ctrl Pts',(-4.8,-6.45,-35.29)) ;
#167114=CARTESIAN_POINT('Ctrl Pts',(-5.82426676739305,-5.43399303700803,
-32.6870109659689)) ;
#167115=CARTESIAN_POINT('Ctrl Pts',(-5.80266988778346,-5.5257236068299,
-32.6923540173524)) ;
#167116=CARTESIAN_POINT('Ctrl Pts',(-5.82426676352028,-5.53106667371345,
-32.7840845871832)) ;
#167117=CARTESIAN_POINT('Ctrl Pts',(-5.83498671931055,-5.43935351192089,
-32.6843294581964)) ;
#167118=CARTESIAN_POINT('Ctrl Pts',(-5.80595263122304,-5.52411753147769,
-32.6939600935421)) ;
#167119=CARTESIAN_POINT('Ctrl Pts',(-5.83498671397647,-5.53374818067475,
-32.7787241131469)) ;
#167120=CARTESIAN_POINT('Ctrl Pts',(-5.84526105845644,-5.44830326289658,
-32.6798528401965)) ;
#167121=CARTESIAN_POINT('Ctrl Pts',(-5.81370932746181,-5.52260132030917,
-32.6954763060005)) ;
#167122=CARTESIAN_POINT('Ctrl Pts',(-5.84526105243738,-5.53822479746348,
-32.7697743635703)) ;
#167123=CARTESIAN_POINT('Ctrl Pts',(-5.8637868540363,-5.47240020430534,
-32.6678032513093)) ;
#167124=CARTESIAN_POINT('Ctrl Pts',(-5.83531854275321,-5.52733067404543,
-32.6907469551157)) ;
#167125=CARTESIAN_POINT('Ctrl Pts',(-5.86378684816478,-5.55027438459912,
-32.7456774250058)) ;
#167126=CARTESIAN_POINT('Ctrl Pts',(-5.87203852631515,-5.48754495134849,
-32.660231552895)) ;
#167127=CARTESIAN_POINT('Ctrl Pts',(-5.84834787930713,-5.53310199490509,
-32.6849756357771)) ;
#167128=CARTESIAN_POINT('Ctrl Pts',(-5.87203852123054,-5.55784608243472,
-32.7305326795143)) ;
#167129=CARTESIAN_POINT('Ctrl Pts',(-5.89242747304776,-5.53981202333512,
-32.6341056511382)) ;
#167130=CARTESIAN_POINT('Ctrl Pts',(-5.88223383300432,-5.56084219179316,
-32.6572354431745)) ;
#167131=CARTESIAN_POINT('Ctrl Pts',(-5.8924274706351,-5.58397198402791,
-32.6782656123278)) ;
#167132=CARTESIAN_POINT('Ctrl Pts',(-5.9,-5.58381083947351,-32.6121194001439)) ;
#167133=CARTESIAN_POINT('Ctrl Pts',(-5.9,-5.59485304502719,-32.6232245928871)) ;
#167134=CARTESIAN_POINT('Ctrl Pts',(-5.9,-5.60595823775519,-32.6342667984408)) ;
#167135=CARTESIAN_POINT('Ctrl Pts',(-5.9,-5.62807764064044,-32.59)) ;
#167136=CARTESIAN_POINT('Ctrl Pts',(-5.9,-5.62807764064044,-32.59)) ;
#167137=CARTESIAN_POINT('Ctrl Pts',(-5.9,-5.62807764064044,-32.59)) ;
#167138=CARTESIAN_POINT('Origin',(-5.84850712500726,-5.43404914061138,-32.7840285000291)) ;
#167139=CARTESIAN_POINT('Ctrl Pts',(-5.82425356250363,-5.53106339062591,
-32.7840285000291)) ;
#167140=CARTESIAN_POINT('Ctrl Pts',(-5.80269484027818,-5.52567371006955,
-32.6924039305709)) ;
#167141=CARTESIAN_POINT('Ctrl Pts',(-5.82425356250363,-5.43404914061138,
-32.6870142500145)) ;
#167142=CARTESIAN_POINT('Ctrl Pts',(-5.80840777707099,-5.52710194426775,
-32.7879899459044)) ;
#167143=CARTESIAN_POINT('Ctrl Pts',(-5.79341417645244,-5.52335354411312,
-32.6928358498186)) ;
#167144=CARTESIAN_POINT('Ctrl Pts',(-5.81633079157287,-5.43008775511762,
-32.6889949427472)) ;
#167145=CARTESIAN_POINT('Ctrl Pts',(-5.79207992677986,-5.52301998169497,
-32.789999999534)) ;
#167146=CARTESIAN_POINT('Ctrl Pts',(-5.78430903206626,-5.52107725801657,
-32.691961395433)) ;
#167147=CARTESIAN_POINT('Ctrl Pts',(-5.80816665318299,-5.42600568595105,
-32.69)) ;
#167148=CARTESIAN_POINT('Ctrl Pts',(-5.77574643749636,-5.51893660937409,
-32.79)) ;
#167149=CARTESIAN_POINT('Ctrl Pts',(-5.77574643749636,-5.51893660937409,
-32.69)) ;
#167150=CARTESIAN_POINT('Ctrl Pts',(-5.8,-5.42192235935956,-32.69)) ;
#167151=CARTESIAN_POINT('Origin',(-5.8,-5.42192235935956,-32.79)) ;
#167152=CARTESIAN_POINT('Origin',(-5.8066065036801,-5.42357398527959,-32.79)) ;
#167153=CARTESIAN_POINT('Origin',(-5.17275707706435,-5.26511162862565,-32.79)) ;
#167154=CARTESIAN_POINT('Origin',(-5.15068655017073,-5.25959399690224,-32.8005938529089)) ;
#167155=CARTESIAN_POINT('Origin',(-5.17275707706436,-5.26511162862565,-32.79)) ;
#167156=CARTESIAN_POINT('Origin',(-5.17275707706436,-5.26511162862565,-32.79)) ;
#167157=CARTESIAN_POINT('Origin',(-5.17275707706436,-5.26511162862565,-32.79)) ;
#167158=CARTESIAN_POINT('Origin',(-5.17275707706436,-5.05,-32.79)) ;
#167159=CARTESIAN_POINT('Origin',(-5.17275707706436,-1.91866427917294,-32.79)) ;
#167160=CARTESIAN_POINT('Origin',(-3.78014014831103,-3.31128120792626,-33.4584561258016)) ;
#167161=CARTESIAN_POINT('Origin',(-5.17275707706436,-1.91866427917294,-32.79)) ;
#167162=CARTESIAN_POINT('Origin',(-5.17275707706436,-1.91866427917294,-32.79)) ;
#167163=CARTESIAN_POINT('Origin',(-5.17275707706436,-1.91866427917294,-32.79)) ;
#167164=CARTESIAN_POINT('Origin',(-3.97071067811865,-3.12071067811865,-32.79)) ;
#167165=CARTESIAN_POINT('Origin',(-5.8,-1.2914213562373,-32.79)) ;
#167166=CARTESIAN_POINT('Ctrl Pts',(-5.87071067811865,-1.14999999999999,
-32.6607106781187)) ;
#167167=CARTESIAN_POINT('Ctrl Pts',(-5.8471404520791,-1.10285954792089,
-32.6842809041582)) ;
#167168=CARTESIAN_POINT('Ctrl Pts',(-5.87071067811865,-1.07928932188134,
-32.7314213562373)) ;
#167169=CARTESIAN_POINT('Ctrl Pts',(-5.85217562795678,-1.18707010095486,
-32.6792457282805)) ;
#167170=CARTESIAN_POINT('Ctrl Pts',(-5.81261165662092,-1.1373883433792,
-32.7058614719491)) ;
#167171=CARTESIAN_POINT('Ctrl Pts',(-5.83353949671048,-1.11646050328952,
-32.7685925363807)) ;
#167172=CARTESIAN_POINT('Ctrl Pts',(-5.82627077431952,-1.2388798075982,
-32.69)) ;
#167173=CARTESIAN_POINT('Ctrl Pts',(-5.76566787907928,-1.18433212092069,
-32.7071489437134)) ;
#167174=CARTESIAN_POINT('Ctrl Pts',(-5.7819067873223,-1.16809321267769,
-32.7899999994191)) ;
#167175=CARTESIAN_POINT('Ctrl Pts',(-5.8,-1.2914213562373,-32.69)) ;
#167176=CARTESIAN_POINT('Ctrl Pts',(-5.72928932188134,-1.22071067811865,
-32.69)) ;
#167177=CARTESIAN_POINT('Ctrl Pts',(-5.72928932188134,-1.22071067811865,
-32.79)) ;
#167178=CARTESIAN_POINT('Origin',(-5.94142135623731,-1.14999999999999,-32.7314213562373)) ;
#167179=CARTESIAN_POINT('Ctrl Pts',(-5.9,-1.00857864376269,-32.59)) ;
#167180=CARTESIAN_POINT('Ctrl Pts',(-5.9,-1.00857864376269,-32.59)) ;
#167181=CARTESIAN_POINT('Ctrl Pts',(-5.9,-1.00857864376269,-32.59)) ;
#167182=CARTESIAN_POINT('Ctrl Pts',(-5.9,-1.06112019240157,-32.61627077432)) ;
#167183=CARTESIAN_POINT('Ctrl Pts',(-5.9,-1.04860238143819,-32.6300237376769)) ;
#167184=CARTESIAN_POINT('Ctrl Pts',(-5.9,-1.03484941808205,-32.642541548639)) ;
#167185=CARTESIAN_POINT('Ctrl Pts',(-5.88924572828051,-1.11292989904511,
-32.6421756279568)) ;
#167186=CARTESIAN_POINT('Ctrl Pts',(-5.87451700624767,-1.08721613124767,
-32.6686374874862)) ;
#167187=CARTESIAN_POINT('Ctrl Pts',(-5.88924572828078,-1.06075427171922,
-32.6943512552828)) ;
#167188=CARTESIAN_POINT('Ctrl Pts',(-5.87071067811865,-1.14999999999999,
-32.6607106781187)) ;
#167189=CARTESIAN_POINT('Ctrl Pts',(-5.8471404520791,-1.10285954792089,
-32.6842809041582)) ;
#167190=CARTESIAN_POINT('Ctrl Pts',(-5.87071067811865,-1.07928932188134,
-32.7314213562373)) ;
#167191=CARTESIAN_POINT('Ctrl Pts',(-5.87071067811866,-1.14999999999999,
-35.9192893218814)) ;
#167192=CARTESIAN_POINT('Ctrl Pts',(-5.8471404520791,-1.10285954792089,
-35.8957190958418)) ;
#167193=CARTESIAN_POINT('Ctrl Pts',(-5.87071067811866,-1.07928932188134,
-35.8485786437627)) ;
#167194=CARTESIAN_POINT('Ctrl Pts',(-5.88924572828049,-1.11292989904506,
-35.9378243720432)) ;
#167195=CARTESIAN_POINT('Ctrl Pts',(-5.87451700624375,-1.08721613124993,
-35.9113625125116)) ;
#167196=CARTESIAN_POINT('Ctrl Pts',(-5.88924572828075,-1.06075427171925,
-35.8856487447172)) ;
#167197=CARTESIAN_POINT('Ctrl Pts',(-5.9,-1.0611201924015,-35.9637292256798)) ;
#167198=CARTESIAN_POINT('Ctrl Pts',(-5.9,-1.04860238143643,-35.9499762623248)) ;
#167199=CARTESIAN_POINT('Ctrl Pts',(-5.9,-1.03484941808207,-35.937458451361)) ;
#167200=CARTESIAN_POINT('Ctrl Pts',(-5.9,-1.00857864376269,-35.99)) ;
#167201=CARTESIAN_POINT('Ctrl Pts',(-5.9,-1.00857864376269,-35.99)) ;
#167202=CARTESIAN_POINT('Ctrl Pts',(-5.9,-1.00857864376269,-35.99)) ;
#167203=CARTESIAN_POINT('Origin',(-5.94142135623734,-1.14999999999996,-35.8485786437627)) ;
#167204=CARTESIAN_POINT('Ctrl Pts',(-5.8,-1.2914213562373,-35.89)) ;
#167205=CARTESIAN_POINT('Ctrl Pts',(-5.72928932188134,-1.22071067811865,
-35.89)) ;
#167206=CARTESIAN_POINT('Ctrl Pts',(-5.72928932188134,-1.22071067811865,
-35.79)) ;
#167207=CARTESIAN_POINT('Ctrl Pts',(-5.82627077431952,-1.2388798075982,
-35.89)) ;
#167208=CARTESIAN_POINT('Ctrl Pts',(-5.76566787907933,-1.18433212092069,
-35.8728510562865)) ;
#167209=CARTESIAN_POINT('Ctrl Pts',(-5.78190678732231,-1.16809321267768,
-35.7900000005809)) ;
#167210=CARTESIAN_POINT('Ctrl Pts',(-5.8521756279568,-1.18707010095487,
-35.9007542717195)) ;
#167211=CARTESIAN_POINT('Ctrl Pts',(-5.81261165662085,-1.13738834337918,
-35.8741385280509)) ;
#167212=CARTESIAN_POINT('Ctrl Pts',(-5.83353949671047,-1.11646050328952,
-35.8114074636193)) ;
#167213=CARTESIAN_POINT('Ctrl Pts',(-5.87071067811865,-1.14999999999999,
-35.9192893218814)) ;
#167214=CARTESIAN_POINT('Ctrl Pts',(-5.8471404520791,-1.10285954792089,
-35.8957190958418)) ;
#167215=CARTESIAN_POINT('Ctrl Pts',(-5.87071067811866,-1.07928932188134,
-35.8485786437627)) ;
#167216=CARTESIAN_POINT('Origin',(-5.8,-1.29142135623731,-35.79)) ;
#167217=CARTESIAN_POINT('Origin',(-3.59571067811865,-3.49571067811865,-35.79)) ;
#167218=CARTESIAN_POINT('Origin',(-5.17275707706436,-1.91866427917294,-35.79)) ;
#167219=CARTESIAN_POINT('Origin',(-3.09057773798104,-4.00084361825625,-34.79055391724)) ;
#167220=CARTESIAN_POINT('Origin',(-5.17275707706435,-1.91866427917295,-35.79)) ;
#167221=CARTESIAN_POINT('Origin',(-5.17275707706435,-1.91866427917295,-35.79)) ;
#167222=CARTESIAN_POINT('Origin',(-5.17275707706435,-1.91866427917295,-35.79)) ;
#167223=CARTESIAN_POINT('Origin',(-5.17275707706435,-5.05,-35.79)) ;
#167224=CARTESIAN_POINT('Origin',(-5.17275707706435,-5.26511162862565,-35.79)) ;
#167225=CARTESIAN_POINT('Origin',(-3.96111272388873,-4.96220054033175,-35.2084107104757)) ;
#167226=CARTESIAN_POINT('Origin',(-5.17275707706435,-5.26511162862565,-35.79)) ;
#167227=CARTESIAN_POINT('Origin',(-5.17275707706435,-5.26511162862565,-35.79)) ;
#167228=CARTESIAN_POINT('Origin',(-5.17275707706435,-5.26511162862565,-35.79)) ;
#167229=CARTESIAN_POINT('Origin',(-5.10072415073893,-5.24710339704429,-35.79)) ;
#167230=CARTESIAN_POINT('Origin',(-5.8,-5.42192235935956,-35.79)) ;
#167231=CARTESIAN_POINT('Ctrl Pts',(-5.77574643749636,-5.51893660937409,
-35.79)) ;
#167232=CARTESIAN_POINT('Ctrl Pts',(-5.77574643749636,-5.51893660937409,
-35.89)) ;
#167233=CARTESIAN_POINT('Ctrl Pts',(-5.8,-5.42192235935956,-35.89)) ;
#167234=CARTESIAN_POINT('Ctrl Pts',(-5.79207992677986,-5.52301998169497,
-35.790000000466)) ;
#167235=CARTESIAN_POINT('Ctrl Pts',(-5.78430903206628,-5.52107725801656,
-35.888038604567)) ;
#167236=CARTESIAN_POINT('Ctrl Pts',(-5.808166653183,-5.42600568595104,-35.89)) ;
#167237=CARTESIAN_POINT('Ctrl Pts',(-5.808407777071,-5.52710194426775,-35.7920100540956)) ;
#167238=CARTESIAN_POINT('Ctrl Pts',(-5.79341417645243,-5.52335354411312,
-35.8871641501814)) ;
#167239=CARTESIAN_POINT('Ctrl Pts',(-5.81633079157287,-5.43008775511762,
-35.8910050572528)) ;
#167240=CARTESIAN_POINT('Ctrl Pts',(-5.82425356250363,-5.53106339062591,
-35.7959714999709)) ;
#167241=CARTESIAN_POINT('Ctrl Pts',(-5.80269484027818,-5.52567371006955,
-35.8875960694291)) ;
#167242=CARTESIAN_POINT('Ctrl Pts',(-5.82425356250363,-5.43404914061138,
-35.8929857499855)) ;
#167243=CARTESIAN_POINT('Origin',(-5.84850712500726,-5.43404914061138,-35.7959714999709)) ;
#167244=CARTESIAN_POINT('Ctrl Pts',(-5.82426676739358,-5.5310666746717,
-35.7959153963653)) ;
#167245=CARTESIAN_POINT('Ctrl Pts',(-5.80266988778302,-5.52572362329019,
-35.8876459661891)) ;
#167246=CARTESIAN_POINT('Ctrl Pts',(-5.82426676352022,-5.4339930534575,
-35.8929890330731)) ;
#167247=CARTESIAN_POINT('Ctrl Pts',(-5.83498671931134,-5.53374818244432,
-35.8012758712783)) ;
#167248=CARTESIAN_POINT('Ctrl Pts',(-5.80595263122244,-5.52411754710043,
-35.8860398908366)) ;
#167249=CARTESIAN_POINT('Ctrl Pts',(-5.83498671397634,-5.43935352749392,
-35.8956705400343)) ;
#167250=CARTESIAN_POINT('Ctrl Pts',(-5.84526105845725,-5.53822480044432,
-35.8102256222542)) ;
#167251=CARTESIAN_POINT('Ctrl Pts',(-5.8137093274612,-5.5226013346416,-35.8845236796681)) ;
#167252=CARTESIAN_POINT('Ctrl Pts',(-5.84526105243728,-5.44830327707045,
-35.900147156823)) ;
#167253=CARTESIAN_POINT('Ctrl Pts',(-5.86378685403709,-5.55027438933186,
-35.8343225636634)) ;
#167254=CARTESIAN_POINT('Ctrl Pts',(-5.83531854275271,-5.52733068552586,
-35.8892530334045)) ;
#167255=CARTESIAN_POINT('Ctrl Pts',(-5.86378684816469,-5.4724002156348,
-35.9121967439586)) ;
#167256=CARTESIAN_POINT('Ctrl Pts',(-5.87203852631588,-5.55784608774616,
-35.8494673107066)) ;
#167257=CARTESIAN_POINT('Ctrl Pts',(-5.84834787930671,-5.53310200486446,
-35.895024354264)) ;
#167258=CARTESIAN_POINT('Ctrl Pts',(-5.87203852123043,-5.48754496112637,
-35.9197684417942)) ;
#167259=CARTESIAN_POINT('Ctrl Pts',(-5.89242747304801,-5.58397198950293,
-35.9017343826941)) ;
#167260=CARTESIAN_POINT('Ctrl Pts',(-5.88223383300418,-5.56084219746617,
-35.9227645511525)) ;
#167261=CARTESIAN_POINT('Ctrl Pts',(-5.89242747063512,-5.53981202831256,
-35.9458943433875)) ;
#167262=CARTESIAN_POINT('Ctrl Pts',(-5.9,-5.60595824049755,-35.9457331988324)) ;
#167263=CARTESIAN_POINT('Ctrl Pts',(-5.9,-5.59485304775362,-35.9567754043864)) ;
#167264=CARTESIAN_POINT('Ctrl Pts',(-5.9,-5.58381084219971,-35.9678805971148)) ;
#167265=CARTESIAN_POINT('Ctrl Pts',(-5.9,-5.62807764064044,-35.99)) ;
#167266=CARTESIAN_POINT('Ctrl Pts',(-5.9,-5.62807764064044,-35.99)) ;
#167267=CARTESIAN_POINT('Ctrl Pts',(-5.9,-5.62807764064044,-35.99)) ;
#167268=CARTESIAN_POINT('Origin',(7.8,2.1,-34.69)) ;
#167269=CARTESIAN_POINT('Origin',(7.8,2.1,-34.89)) ;
#167270=CARTESIAN_POINT('Origin',(7.6,2.1,-34.69)) ;
#167271=CARTESIAN_POINT('Origin',(7.6,2.1,-34.69)) ;
#167272=CARTESIAN_POINT('Origin',(7.6,2.1,-33.89)) ;
#167273=CARTESIAN_POINT('Origin',(7.8,2.1,-34.89)) ;
#167274=CARTESIAN_POINT('Origin',(9.6,2.1,-34.89)) ;
#167275=CARTESIAN_POINT('Origin',(7.8,2.1,-33.89)) ;
#167276=CARTESIAN_POINT('Origin',(7.8,2.1,-33.69)) ;
#167277=CARTESIAN_POINT('Origin',(9.6,2.1,-34.69)) ;
#167278=CARTESIAN_POINT('Origin',(9.8,2.1,-34.69)) ;
#167279=CARTESIAN_POINT('Origin',(7.8,2.1,-33.69)) ;
#167280=CARTESIAN_POINT('Origin',(9.6,2.1,-33.69)) ;
#167281=CARTESIAN_POINT('Origin',(9.8,2.1,-34.69)) ;
#167282=CARTESIAN_POINT('Origin',(9.8,2.1,-33.89)) ;
#167283=CARTESIAN_POINT('Origin',(9.6,2.1,-33.89)) ;
#167284=CARTESIAN_POINT('Origin',(-4.15,-6.25,-33.54)) ;
#167285=CARTESIAN_POINT('Origin',(-4.15,-6.3,-33.54)) ;
#167286=CARTESIAN_POINT('Origin',(-4.15,-6.3,-34.29)) ;
#167287=CARTESIAN_POINT('Origin',(-4.15,-6.3,-35.04)) ;
#167288=CARTESIAN_POINT('Origin',(-4.15,-6.3,-33.54)) ;
#167289=CARTESIAN_POINT('Origin',(-4.15,-6.25,-35.04)) ;
#167290=CARTESIAN_POINT('Origin',(-4.15,-6.3,-35.04)) ;
#167291=CARTESIAN_POINT('Origin',(-4.15,-6.3,-33.54)) ;
#167292=CARTESIAN_POINT('Origin',(-4.15,-6.3,-33.54)) ;
#167293=CARTESIAN_POINT('Origin',(-4.15,-6.3,-35.04)) ;
#167294=CARTESIAN_POINT('Origin',(-4.15,-6.3,-35.04)) ;
#167295=CARTESIAN_POINT('Origin',(-4.65,-6.25,-33.54)) ;
#167296=CARTESIAN_POINT('Origin',(-4.65,-6.3,-33.54)) ;
#167297=CARTESIAN_POINT('Origin',(0.,-6.3,-33.54)) ;
#167298=CARTESIAN_POINT('Origin',(-4.65,-6.3,-33.54)) ;
#167299=CARTESIAN_POINT('Origin',(0.,-6.3,-35.04)) ;
#167300=CARTESIAN_POINT('Origin',(-4.65,-6.3,-35.04)) ;
#167301=CARTESIAN_POINT('Origin',(-4.65,-6.25,-35.04)) ;
#167302=CARTESIAN_POINT('Origin',(-4.65,-6.3,-35.04)) ;
#167303=CARTESIAN_POINT('Origin',(-4.65,-6.3,-33.54)) ;
#167304=CARTESIAN_POINT('Origin',(-4.65,-6.3,-33.54)) ;
#167305=CARTESIAN_POINT('Origin',(-4.65,-6.3,-35.04)) ;
#167306=CARTESIAN_POINT('Origin',(-4.65,-6.3,-35.04)) ;
#167307=CARTESIAN_POINT('Origin',(-4.65,-6.3,-34.29)) ;
#167308=CARTESIAN_POINT('Origin',(-3.,4.45,-35.39)) ;
#167309=CARTESIAN_POINT('Origin',(-2.1,4.45,-35.39)) ;
#167310=CARTESIAN_POINT('Origin',(-2.9,4.45,-35.39)) ;
#167311=CARTESIAN_POINT('Origin',(-2.9,4.45,-35.19)) ;
#167312=CARTESIAN_POINT('Origin',(-3.1,4.45,-35.19)) ;
#167313=CARTESIAN_POINT('Origin',(-2.9,4.45,-35.19)) ;
#167314=CARTESIAN_POINT('Origin',(-2.1,4.45,-35.19)) ;
#167315=CARTESIAN_POINT('Origin',(-2.1,4.45,-35.19)) ;
#167316=CARTESIAN_POINT('Origin',(-1.9,4.45,-35.19)) ;
#167317=CARTESIAN_POINT('Origin',(-3.1,4.45,-35.29)) ;
#167318=CARTESIAN_POINT('Origin',(-3.1,4.45,-33.39)) ;
#167319=CARTESIAN_POINT('Origin',(-2.9,4.4,-35.19)) ;
#167320=CARTESIAN_POINT('Origin',(-2.9,4.35,-35.19)) ;
#167321=CARTESIAN_POINT('Origin',(-1.95156391047391E-16,4.35,-35.19)) ;
#167322=CARTESIAN_POINT('Origin',(-2.1,4.35,-35.19)) ;
#167323=CARTESIAN_POINT('Origin',(-2.9,4.35,-35.19)) ;
#167324=CARTESIAN_POINT('Origin',(-2.1,4.4,-35.19)) ;
#167325=CARTESIAN_POINT('Origin',(-2.1,4.35,-35.19)) ;
#167326=CARTESIAN_POINT('Origin',(-1.9,4.45,-35.29)) ;
#167327=CARTESIAN_POINT('Origin',(-1.9,4.45,-33.39)) ;
#167328=CARTESIAN_POINT('Origin',(-3.,4.45,-33.19)) ;
#167329=CARTESIAN_POINT('Origin',(-2.9,4.45,-33.19)) ;
#167330=CARTESIAN_POINT('Origin',(-2.1,4.45,-33.19)) ;
#167331=CARTESIAN_POINT('Origin',(-2.9,4.45,-33.39)) ;
#167332=CARTESIAN_POINT('Origin',(-2.9,4.45,-33.39)) ;
#167333=CARTESIAN_POINT('Origin',(-2.9,4.35,-35.19)) ;
#167334=CARTESIAN_POINT('Origin',(-2.9,4.35,-35.19)) ;
#167335=CARTESIAN_POINT('Origin',(-2.1,4.35,-35.19)) ;
#167336=CARTESIAN_POINT('Origin',(-2.1,4.35,-35.19)) ;
#167337=CARTESIAN_POINT('Origin',(-2.1,4.45,-33.39)) ;
#167338=CARTESIAN_POINT('Origin',(-2.1,4.45,-33.39)) ;
#167339=CARTESIAN_POINT('Origin',(-2.9,4.4,-33.39)) ;
#167340=CARTESIAN_POINT('Origin',(-2.9,4.35,-33.39)) ;
#167341=CARTESIAN_POINT('Origin',(-2.9,4.35,-34.29)) ;
#167342=CARTESIAN_POINT('Origin',(-2.9,4.35,-33.39)) ;
#167343=CARTESIAN_POINT('Origin',(-2.1,4.35,-34.29)) ;
#167344=CARTESIAN_POINT('Origin',(-2.1,4.35,-33.39)) ;
#167345=CARTESIAN_POINT('Origin',(-2.1,4.4,-33.39)) ;
#167346=CARTESIAN_POINT('Origin',(-2.1,4.35,-33.39)) ;
#167347=CARTESIAN_POINT('Origin',(-2.9,4.35,-33.39)) ;
#167348=CARTESIAN_POINT('Origin',(-2.9,4.35,-33.39)) ;
#167349=CARTESIAN_POINT('Origin',(-2.1,4.35,-33.39)) ;
#167350=CARTESIAN_POINT('Origin',(-2.1,4.35,-33.39)) ;
#167351=CARTESIAN_POINT('Origin',(-1.95156391047391E-16,4.35,-33.39)) ;
#167352=CARTESIAN_POINT('Origin',(-2.25,4.25,-35.04)) ;
#167353=CARTESIAN_POINT('Origin',(-2.25,4.3,-35.04)) ;
#167354=CARTESIAN_POINT('Origin',(-2.25,4.3,-34.29)) ;
#167355=CARTESIAN_POINT('Origin',(-2.25,4.3,-33.54)) ;
#167356=CARTESIAN_POINT('Origin',(-2.25,4.3,-35.04)) ;
#167357=CARTESIAN_POINT('Origin',(-2.25,4.25,-33.54)) ;
#167358=CARTESIAN_POINT('Origin',(-2.25,4.3,-33.54)) ;
#167359=CARTESIAN_POINT('Origin',(-2.25,4.3,-35.04)) ;
#167360=CARTESIAN_POINT('Origin',(-2.25,4.3,-35.04)) ;
#167361=CARTESIAN_POINT('Origin',(-2.25,4.3,-33.54)) ;
#167362=CARTESIAN_POINT('Origin',(-2.25,4.3,-33.54)) ;
#167363=CARTESIAN_POINT('Origin',(-2.75,4.25,-35.04)) ;
#167364=CARTESIAN_POINT('Origin',(-2.75,4.3,-35.04)) ;
#167365=CARTESIAN_POINT('Origin',(-1.97127667724637E-17,4.3,-35.04)) ;
#167366=CARTESIAN_POINT('Origin',(-2.75,4.3,-35.04)) ;
#167367=CARTESIAN_POINT('Origin',(-1.97127667724637E-17,4.3,-33.54)) ;
#167368=CARTESIAN_POINT('Origin',(-2.75,4.3,-33.54)) ;
#167369=CARTESIAN_POINT('Origin',(-2.75,4.25,-33.54)) ;
#167370=CARTESIAN_POINT('Origin',(-2.75,4.3,-33.54)) ;
#167371=CARTESIAN_POINT('Origin',(-2.75,4.3,-35.04)) ;
#167372=CARTESIAN_POINT('Origin',(-2.75,4.3,-35.04)) ;
#167373=CARTESIAN_POINT('Origin',(-2.75,4.3,-33.54)) ;
#167374=CARTESIAN_POINT('Origin',(-2.75,4.3,-33.54)) ;
#167375=CARTESIAN_POINT('Origin',(-2.75,4.3,-34.29)) ;
#167376=CARTESIAN_POINT('Origin',(7.8,2.9,-34.69)) ;
#167377=CARTESIAN_POINT('Origin',(7.8,2.9,-34.69)) ;
#167378=CARTESIAN_POINT('Origin',(7.8,2.9,-33.89)) ;
#167379=CARTESIAN_POINT('Origin',(7.8,2.9,-33.89)) ;
#167380=CARTESIAN_POINT('Origin',(7.8,2.9,-33.89)) ;
#167381=CARTESIAN_POINT('Origin',(7.8,2.9,-34.69)) ;
#167382=CARTESIAN_POINT('Origin',(7.8,2.9,-34.69)) ;
#167383=CARTESIAN_POINT('Origin',(9.6,2.9,-33.89)) ;
#167384=CARTESIAN_POINT('Origin',(9.6,2.9,-33.89)) ;
#167385=CARTESIAN_POINT('Origin',(9.6,2.9,-34.69)) ;
#167386=CARTESIAN_POINT('Origin',(9.6,2.9,-34.69)) ;
#167387=CARTESIAN_POINT('Origin',(9.6,2.9,-33.89)) ;
#167388=CARTESIAN_POINT('Origin',(9.6,2.9,-33.89)) ;
#167389=CARTESIAN_POINT('Origin',(9.6,2.9,-34.69)) ;
#167390=CARTESIAN_POINT('Origin',(9.6,2.9,-34.69)) ;
#167391=CARTESIAN_POINT('Origin',(9.6,2.9,-34.69)) ;
#167392=CARTESIAN_POINT('Origin',(-0.183301359729408,3.45,-32.772963213524)) ;
#167393=CARTESIAN_POINT('Origin',(0.24923464143508,3.15,-34.1737799780213)) ;
#167394=CARTESIAN_POINT('Origin',(-0.249234641435079,3.15,-34.4062200219787)) ;
#167395=CARTESIAN_POINT('Origin',(-1.04429375741423,3.45,-33.1744505621777)) ;
#167396=CARTESIAN_POINT('Origin',(3.7,2.1,-2.405)) ;
#167397=CARTESIAN_POINT('Origin',(3.7,2.1,-5.115)) ;
#167398=CARTESIAN_POINT('Origin',(3.7,2.1,-2.505)) ;
#167399=CARTESIAN_POINT('Origin',(3.7,2.1,-6.215)) ;
#167400=CARTESIAN_POINT('Origin',(3.7,2.1,-8.925)) ;
#167401=CARTESIAN_POINT('Origin',(3.7,2.1,-6.315)) ;
#167402=CARTESIAN_POINT('Origin',(3.7,2.1,-10.025)) ;
#167403=CARTESIAN_POINT('Origin',(3.7,2.1,-12.735)) ;
#167404=CARTESIAN_POINT('Origin',(3.7,2.1,-10.125)) ;
#167405=CARTESIAN_POINT('Origin',(3.7,2.1,-13.835)) ;
#167406=CARTESIAN_POINT('Origin',(3.7,2.1,-16.545)) ;
#167407=CARTESIAN_POINT('Origin',(3.7,2.1,-13.935)) ;
#167408=CARTESIAN_POINT('Origin',(3.7,2.1,-17.645)) ;
#167409=CARTESIAN_POINT('Origin',(3.7,2.1,-20.355)) ;
#167410=CARTESIAN_POINT('Origin',(3.7,2.1,-17.745)) ;
#167411=CARTESIAN_POINT('Origin',(3.7,2.1,-21.455)) ;
#167412=CARTESIAN_POINT('Origin',(3.7,2.1,-24.165)) ;
#167413=CARTESIAN_POINT('Origin',(3.7,2.1,-21.555)) ;
#167414=CARTESIAN_POINT('Origin',(3.7,2.1,-25.265)) ;
#167415=CARTESIAN_POINT('Origin',(3.7,2.1,-27.975)) ;
#167416=CARTESIAN_POINT('Origin',(3.7,2.1,-25.365)) ;
#167417=CARTESIAN_POINT('Origin',(3.7,2.1,-29.075)) ;
#167418=CARTESIAN_POINT('Origin',(3.7,2.1,-31.785)) ;
#167419=CARTESIAN_POINT('Origin',(3.7,2.1,-29.175)) ;
#167420=CARTESIAN_POINT('Origin',(3.7,2.1,-32.885)) ;
#167421=CARTESIAN_POINT('Origin',(3.7,2.1,-35.595)) ;
#167422=CARTESIAN_POINT('Origin',(3.7,2.1,-32.985)) ;
#167423=CARTESIAN_POINT('Origin',(3.5,1.9,-6.115)) ;
#167424=CARTESIAN_POINT('',(3.55,2.01339745962156,-6.115)) ;
#167425=CARTESIAN_POINT('Origin',(3.5,2.1,-6.115)) ;
#167426=CARTESIAN_POINT('Ctrl Pts',(3.55,2.01339745962156,-6.115)) ;
#167427=CARTESIAN_POINT('Ctrl Pts',(3.55164546205118,2.01434746757975,-6.115)) ;
#167428=CARTESIAN_POINT('Ctrl Pts',(3.55326668047441,2.01534654795451,-6.1153329780303)) ;
#167429=CARTESIAN_POINT('Ctrl Pts',(3.55550702654634,2.01680421826673,-6.11609826168305)) ;
#167430=CARTESIAN_POINT('Ctrl Pts',(3.55618577699068,2.01725684095079,-6.11637359606383)) ;
#167431=CARTESIAN_POINT('Ctrl Pts',(3.55727967686454,2.01800266699454,-6.1168678300958)) ;
#167432=CARTESIAN_POINT('Ctrl Pts',(3.55771141786834,2.01830156212325,-6.11707831894258)) ;
#167433=CARTESIAN_POINT('Ctrl Pts',(3.56202821818157,2.02133211263481,-6.1191706910972)) ;
#167434=CARTESIAN_POINT('Ctrl Pts',(3.56570108751477,2.02427663140637,-6.12224393162826)) ;
#167435=CARTESIAN_POINT('Ctrl Pts',(3.5699034772656,2.02797441535145,-6.12640200473845)) ;
#167436=CARTESIAN_POINT('Ctrl Pts',(3.57072473561126,2.02871480216321,-6.12724959773093)) ;
#167437=CARTESIAN_POINT('Ctrl Pts',(3.5738286330762,2.03157464832067,-6.13054171893286)) ;
#167438=CARTESIAN_POINT('Ctrl Pts',(3.5759706937612,2.03369481096682,-6.13313773435733)) ;
#167439=CARTESIAN_POINT('Ctrl Pts',(3.58156103639368,2.03956384830232,-6.14075811677975)) ;
#167440=CARTESIAN_POINT('Ctrl Pts',(3.58475859790495,2.04336775308648,-6.14615483852158)) ;
#167441=CARTESIAN_POINT('Ctrl Pts',(3.58897725231935,2.0490105592432,-6.15495483430059)) ;
#167442=CARTESIAN_POINT('Ctrl Pts',(3.59034871903171,2.05099358132072,-6.15822253384318)) ;
#167443=CARTESIAN_POINT('Ctrl Pts',(3.59365488292729,2.05613355260445,-6.16724922860835)) ;
#167444=CARTESIAN_POINT('Ctrl Pts',(3.59534780095525,2.05919518104045,-6.17324371161029)) ;
#167445=CARTESIAN_POINT('Ctrl Pts',(3.59674625886212,2.06216860863464,-6.17996044662966)) ;
#167446=CARTESIAN_POINT('Ctrl Pts',(3.59685725281059,2.06240883133061,-6.18051031510962)) ;
#167447=CARTESIAN_POINT('Ctrl Pts',(3.59768573690243,2.06423460359408,-6.18474653762001)) ;
#167448=CARTESIAN_POINT('Ctrl Pts',(3.59826864191792,2.06571343564803,-6.18852399715655)) ;
#167449=CARTESIAN_POINT('Ctrl Pts',(3.59959273712775,2.06963221119414,-6.19968301436906)) ;
#167450=CARTESIAN_POINT('Ctrl Pts',(3.6,2.07172309150643,-6.2072993579658)) ;
#167451=CARTESIAN_POINT('Ctrl Pts',(3.6,2.07320508075689,-6.215)) ;
#167452=CARTESIAN_POINT('Origin',(3.5,2.1,-1.01757522333835E-15)) ;
#167453=CARTESIAN_POINT('Origin',(3.5,2.1,-6.115)) ;
#167454=CARTESIAN_POINT('',(3.55,2.01339745962156,-5.315)) ;
#167455=CARTESIAN_POINT('Origin',(3.5,2.1,-5.315)) ;
#167456=CARTESIAN_POINT('Origin',(3.5,2.1,-5.315)) ;
#167457=CARTESIAN_POINT('Origin',(3.5,1.9,-5.315)) ;
#167458=CARTESIAN_POINT('Ctrl Pts',(3.6,2.07320508075689,-5.215)) ;
#167459=CARTESIAN_POINT('Ctrl Pts',(3.6,2.07265589924994,-5.21785357667012)) ;
#167460=CARTESIAN_POINT('Ctrl Pts',(3.59994554076638,2.07202433860048,-5.22069358004935)) ;
#167461=CARTESIAN_POINT('Ctrl Pts',(3.59971739924421,2.07059366100571,-5.22637921497773)) ;
#167462=CARTESIAN_POINT('Ctrl Pts',(3.59954156373427,2.06979274847054,-5.22921873634714)) ;
#167463=CARTESIAN_POINT('Ctrl Pts',(3.59880783141185,2.06712577191658,-5.23778089072537)) ;
#167464=CARTESIAN_POINT('Ctrl Pts',(3.59804129495587,2.0650190276639,-5.24341713644386)) ;
#167465=CARTESIAN_POINT('Ctrl Pts',(3.59624340061598,2.06105248659392,-5.25263353946359)) ;
#167466=CARTESIAN_POINT('Ctrl Pts',(3.59536494855695,2.05931170891995,-5.25632347138735)) ;
#167467=CARTESIAN_POINT('Ctrl Pts',(3.5928372720244,2.05479606436794,-5.26519943205902)) ;
#167468=CARTESIAN_POINT('Ctrl Pts',(3.59099650883092,2.05188276467123,-5.27034424200709)) ;
#167469=CARTESIAN_POINT('Ctrl Pts',(3.58838944624308,2.04823719194672,-5.27622737667942)) ;
#167470=CARTESIAN_POINT('Ctrl Pts',(3.58794537962075,2.04762948672743,-5.27719091385135)) ;
#167471=CARTESIAN_POINT('Ctrl Pts',(3.58597371492279,2.04498948329048,-5.28130665172963)) ;
#167472=CARTESIAN_POINT('Ctrl Pts',(3.58430396743904,2.04289920268562,-5.28439316248021)) ;
#167473=CARTESIAN_POINT('Ctrl Pts',(3.58008903321353,2.03798436571141,-5.29128092067904)) ;
#167474=CARTESIAN_POINT('Ctrl Pts',(3.57743593401578,2.0351394536771,-5.29500157292073)) ;
#167475=CARTESIAN_POINT('Ctrl Pts',(3.57357563759658,2.03136250950841,-5.29958640159694)) ;
#167476=CARTESIAN_POINT('Ctrl Pts',(3.57257888733672,2.03041544381399,-5.30070656893144)) ;
#167477=CARTESIAN_POINT('Ctrl Pts',(3.56956839719841,2.02764175140691,-5.30390390778882)) ;
#167478=CARTESIAN_POINT('Ctrl Pts',(3.56746189551952,2.02581554544786,-5.30598430067898)) ;
#167479=CARTESIAN_POINT('Ctrl Pts',(3.56503628433188,2.02384076964147,-5.30802226003855)) ;
#167480=CARTESIAN_POINT('Ctrl Pts',(3.56481411023493,2.02366103014357,-5.30820583968785)) ;
#167481=CARTESIAN_POINT('Ctrl Pts',(3.56285239425759,2.02208416924062,-5.30979838212049)) ;
#167482=CARTESIAN_POINT('Ctrl Pts',(3.56093641846881,2.02061618613973,-5.31118717775178)) ;
#167483=CARTESIAN_POINT('Ctrl Pts',(3.5587973662077,2.01908299720839,-5.31237714025465)) ;
#167484=CARTESIAN_POINT('Ctrl Pts',(3.55867935922409,2.01899873301461,-5.31244171035243)) ;
#167485=CARTESIAN_POINT('Ctrl Pts',(3.5578895339955,2.01843691186419,-5.31286648337378)) ;
#167486=CARTESIAN_POINT('Ctrl Pts',(3.55720723474254,2.01796200020269,-5.313197549106)) ;
#167487=CARTESIAN_POINT('Ctrl Pts',(3.55509125643152,2.01652382826846,-5.31409794445157)) ;
#167488=CARTESIAN_POINT('Ctrl Pts',(3.55356547969792,2.01553571874065,-5.31460356135168)) ;
#167489=CARTESIAN_POINT('Ctrl Pts',(3.55133342567605,2.01417771500982,-5.31494476439962)) ;
#167490=CARTESIAN_POINT('Ctrl Pts',(3.55066861961529,2.01378348733643,-5.31499963178873)) ;
#167491=CARTESIAN_POINT('Ctrl Pts',(3.55,2.01339745962156,-5.315)) ;
#167492=CARTESIAN_POINT('Origin',(3.5,1.9,-2.305)) ;
#167493=CARTESIAN_POINT('Ctrl Pts',(3.55000000000001,2.01339745962156,-2.305)) ;
#167494=CARTESIAN_POINT('Ctrl Pts',(3.55164546205119,2.01434746757975,-2.305)) ;
#167495=CARTESIAN_POINT('Ctrl Pts',(3.55326668047441,2.01534654795451,-2.30533297803029)) ;
#167496=CARTESIAN_POINT('Ctrl Pts',(3.55550702654634,2.01680421826673,-2.30609826168304)) ;
#167497=CARTESIAN_POINT('Ctrl Pts',(3.55618577699068,2.01725684095079,-2.30637359606382)) ;
#167498=CARTESIAN_POINT('Ctrl Pts',(3.55727967686454,2.01800266699453,-2.3068678300958)) ;
#167499=CARTESIAN_POINT('Ctrl Pts',(3.55771141786834,2.01830156212325,-2.30707831894258)) ;
#167500=CARTESIAN_POINT('Ctrl Pts',(3.56202821818163,2.02133211263485,-2.30917069109723)) ;
#167501=CARTESIAN_POINT('Ctrl Pts',(3.56570108751487,2.02427663140646,-2.31224393162834)) ;
#167502=CARTESIAN_POINT('Ctrl Pts',(3.5699034772657,2.02797441535154,-2.31640200473853)) ;
#167503=CARTESIAN_POINT('Ctrl Pts',(3.5707247356113,2.02871480216325,-2.31724959773097)) ;
#167504=CARTESIAN_POINT('Ctrl Pts',(3.5738286330762,2.03157464832067,-2.32054171893286)) ;
#167505=CARTESIAN_POINT('Ctrl Pts',(3.5759706937612,2.03369481096682,-2.32313773435733)) ;
#167506=CARTESIAN_POINT('Ctrl Pts',(3.58156103639367,2.03956384830232,-2.33075811677975)) ;
#167507=CARTESIAN_POINT('Ctrl Pts',(3.58475859790494,2.04336775308648,-2.33615483852158)) ;
#167508=CARTESIAN_POINT('Ctrl Pts',(3.58897725231935,2.04901055924319,-2.34495483430059)) ;
#167509=CARTESIAN_POINT('Ctrl Pts',(3.59034871903171,2.05099358132072,-2.34822253384318)) ;
#167510=CARTESIAN_POINT('Ctrl Pts',(3.59365488292729,2.05613355260444,-2.35724922860834)) ;
#167511=CARTESIAN_POINT('Ctrl Pts',(3.59534780095525,2.05919518104044,-2.36324371161028)) ;
#167512=CARTESIAN_POINT('Ctrl Pts',(3.59674625886211,2.06216860863463,-2.36996044662965)) ;
#167513=CARTESIAN_POINT('Ctrl Pts',(3.59685725281059,2.0624088313306,-2.37051031510962)) ;
#167514=CARTESIAN_POINT('Ctrl Pts',(3.59768573690243,2.06423460359408,-2.37474653762001)) ;
#167515=CARTESIAN_POINT('Ctrl Pts',(3.59826864191792,2.06571343564803,-2.37852399715655)) ;
#167516=CARTESIAN_POINT('Ctrl Pts',(3.59959273712775,2.06963221119414,-2.38968301436905)) ;
#167517=CARTESIAN_POINT('Ctrl Pts',(3.6,2.07172309150643,-2.3972993579658)) ;
#167518=CARTESIAN_POINT('Ctrl Pts',(3.6,2.07320508075689,-2.405)) ;
#167519=CARTESIAN_POINT('Origin',(3.5,1.9,-9.925)) ;
#167520=CARTESIAN_POINT('',(3.55,2.01339745962156,-9.925)) ;
#167521=CARTESIAN_POINT('Origin',(3.5,2.1,-9.925)) ;
#167522=CARTESIAN_POINT('Ctrl Pts',(3.55,2.01339745962156,-9.925)) ;
#167523=CARTESIAN_POINT('Ctrl Pts',(3.55164546205119,2.01434746757975,-9.925)) ;
#167524=CARTESIAN_POINT('Ctrl Pts',(3.55326668047443,2.01534654795452,-9.92533297803029)) ;
#167525=CARTESIAN_POINT('Ctrl Pts',(3.55550702654635,2.01680421826674,-9.92609826168304)) ;
#167526=CARTESIAN_POINT('Ctrl Pts',(3.55618577699069,2.0172568409508,-9.92637359606382)) ;
#167527=CARTESIAN_POINT('Ctrl Pts',(3.55727967686454,2.01800266699454,-9.92686783009579)) ;
#167528=CARTESIAN_POINT('Ctrl Pts',(3.55771141786834,2.01830156212325,-9.92707831894258)) ;
#167529=CARTESIAN_POINT('Ctrl Pts',(3.56202821818162,2.02133211263484,-9.92917069109722)) ;
#167530=CARTESIAN_POINT('Ctrl Pts',(3.56570108751486,2.02427663140645,-9.93224393162833)) ;
#167531=CARTESIAN_POINT('Ctrl Pts',(3.56990347726569,2.02797441535153,-9.93640200473853)) ;
#167532=CARTESIAN_POINT('Ctrl Pts',(3.5707247356113,2.02871480216325,-9.93724959773096)) ;
#167533=CARTESIAN_POINT('Ctrl Pts',(3.57382863307621,2.03157464832067,-9.94054171893286)) ;
#167534=CARTESIAN_POINT('Ctrl Pts',(3.5759706937612,2.03369481096682,-9.94313773435733)) ;
#167535=CARTESIAN_POINT('Ctrl Pts',(3.58156103639368,2.03956384830232,-9.95075811677975)) ;
#167536=CARTESIAN_POINT('Ctrl Pts',(3.58475859790494,2.04336775308648,-9.95615483852156)) ;
#167537=CARTESIAN_POINT('Ctrl Pts',(3.58897725231935,2.0490105592432,-9.96495483430059)) ;
#167538=CARTESIAN_POINT('Ctrl Pts',(3.59034871903171,2.05099358132072,-9.96822253384318)) ;
#167539=CARTESIAN_POINT('Ctrl Pts',(3.59365488292729,2.05613355260445,-9.97724922860834)) ;
#167540=CARTESIAN_POINT('Ctrl Pts',(3.59534780095525,2.05919518104045,-9.98324371161027)) ;
#167541=CARTESIAN_POINT('Ctrl Pts',(3.59674625886211,2.06216860863464,-9.98996044662965)) ;
#167542=CARTESIAN_POINT('Ctrl Pts',(3.59685725281059,2.06240883133061,-9.99051031510962)) ;
#167543=CARTESIAN_POINT('Ctrl Pts',(3.59768573690243,2.06423460359409,-9.99474653762001)) ;
#167544=CARTESIAN_POINT('Ctrl Pts',(3.59826864191792,2.06571343564803,-9.99852399715655)) ;
#167545=CARTESIAN_POINT('Ctrl Pts',(3.59959273712775,2.06963221119414,-10.0096830143691)) ;
#167546=CARTESIAN_POINT('Ctrl Pts',(3.6,2.07172309150643,-10.0172993579658)) ;
#167547=CARTESIAN_POINT('Ctrl Pts',(3.6,2.07320508075689,-10.025)) ;
#167548=CARTESIAN_POINT('Origin',(3.5,2.1,-1.01757522333835E-15)) ;
#167549=CARTESIAN_POINT('Origin',(3.5,2.1,-9.925)) ;
#167550=CARTESIAN_POINT('',(3.55,2.01339745962156,-9.125)) ;
#167551=CARTESIAN_POINT('Origin',(3.5,2.1,-9.125)) ;
#167552=CARTESIAN_POINT('Origin',(3.5,2.1,-9.125)) ;
#167553=CARTESIAN_POINT('Origin',(3.5,1.9,-9.125)) ;
#167554=CARTESIAN_POINT('Ctrl Pts',(3.6,2.07320508075689,-9.025)) ;
#167555=CARTESIAN_POINT('Ctrl Pts',(3.6,2.07265589924992,-9.02785357667023)) ;
#167556=CARTESIAN_POINT('Ctrl Pts',(3.59994554076637,2.07202433860043,-9.03069358004957)) ;
#167557=CARTESIAN_POINT('Ctrl Pts',(3.59971739924419,2.0705936610056,-9.03637921497813)) ;
#167558=CARTESIAN_POINT('Ctrl Pts',(3.59954156373424,2.06979274847041,-9.03921873634762)) ;
#167559=CARTESIAN_POINT('Ctrl Pts',(3.5988078314118,2.06712577191644,-9.04778089072574)) ;
#167560=CARTESIAN_POINT('Ctrl Pts',(3.59804129495583,2.06501902766383,-9.05341713644404)) ;
#167561=CARTESIAN_POINT('Ctrl Pts',(3.59624340061598,2.06105248659392,-9.06263353946358)) ;
#167562=CARTESIAN_POINT('Ctrl Pts',(3.59536494855695,2.05931170891995,-9.06632347138735)) ;
#167563=CARTESIAN_POINT('Ctrl Pts',(3.5928372720244,2.05479606436796,-9.075199432059)) ;
#167564=CARTESIAN_POINT('Ctrl Pts',(3.59099650883094,2.05188276467126,-9.08034424200704)) ;
#167565=CARTESIAN_POINT('Ctrl Pts',(3.58838944624311,2.04823719194676,-9.08622737667937)) ;
#167566=CARTESIAN_POINT('Ctrl Pts',(3.58794537962076,2.04762948672745,-9.08719091385132)) ;
#167567=CARTESIAN_POINT('Ctrl Pts',(3.58597371492279,2.04498948329048,-9.09130665172963)) ;
#167568=CARTESIAN_POINT('Ctrl Pts',(3.58430396743904,2.04289920268562,-9.09439316248022)) ;
#167569=CARTESIAN_POINT('Ctrl Pts',(3.58008903321355,2.03798436571145,-9.10128092067901)) ;
#167570=CARTESIAN_POINT('Ctrl Pts',(3.57743593401584,2.03513945367717,-9.10500157292067)) ;
#167571=CARTESIAN_POINT('Ctrl Pts',(3.57357563759665,2.03136250950848,-9.1095864015969)) ;
#167572=CARTESIAN_POINT('Ctrl Pts',(3.57257888733676,2.03041544381403,-9.11070656893144)) ;
#167573=CARTESIAN_POINT('Ctrl Pts',(3.56956839719839,2.0276417514069,-9.11390390778888)) ;
#167574=CARTESIAN_POINT('Ctrl Pts',(3.56746189551947,2.02581554544782,-9.11598430067906)) ;
#167575=CARTESIAN_POINT('Ctrl Pts',(3.56503628433183,2.02384076964143,-9.11802226003861)) ;
#167576=CARTESIAN_POINT('Ctrl Pts',(3.56481411023491,2.02366103014355,-9.11820583968789)) ;
#167577=CARTESIAN_POINT('Ctrl Pts',(3.56285239425755,2.02208416924059,-9.11979838212054)) ;
#167578=CARTESIAN_POINT('Ctrl Pts',(3.56093641846873,2.02061618613967,-9.12118717775184)) ;
#167579=CARTESIAN_POINT('Ctrl Pts',(3.55879736620764,2.01908299720835,-9.12237714025469)) ;
#167580=CARTESIAN_POINT('Ctrl Pts',(3.5586793592241,2.01899873301461,-9.12244171035242)) ;
#167581=CARTESIAN_POINT('Ctrl Pts',(3.55788953399554,2.01843691186422,-9.12286648337376)) ;
#167582=CARTESIAN_POINT('Ctrl Pts',(3.55720723474255,2.0179620002027,-9.123197549106)) ;
#167583=CARTESIAN_POINT('Ctrl Pts',(3.55509125643146,2.01652382826842,-9.12409794445161)) ;
#167584=CARTESIAN_POINT('Ctrl Pts',(3.5535654796978,2.01553571874058,-9.12460356135171)) ;
#167585=CARTESIAN_POINT('Ctrl Pts',(3.55133342567592,2.01417771500975,-9.12494476439961)) ;
#167586=CARTESIAN_POINT('Ctrl Pts',(3.55066861961523,2.01378348733639,-9.12499963178872)) ;
#167587=CARTESIAN_POINT('Ctrl Pts',(3.55,2.01339745962156,-9.125)) ;
#167588=CARTESIAN_POINT('Origin',(3.5,1.9,-13.735)) ;
#167589=CARTESIAN_POINT('',(3.55,2.01339745962156,-13.735)) ;
#167590=CARTESIAN_POINT('Origin',(3.5,2.1,-13.735)) ;
#167591=CARTESIAN_POINT('Ctrl Pts',(3.55,2.01339745962156,-13.735)) ;
#167592=CARTESIAN_POINT('Ctrl Pts',(3.55164546205119,2.01434746757975,-13.735)) ;
#167593=CARTESIAN_POINT('Ctrl Pts',(3.55326668047442,2.01534654795452,-13.7353329780303)) ;
#167594=CARTESIAN_POINT('Ctrl Pts',(3.55550702654635,2.01680421826673,-13.736098261683)) ;
#167595=CARTESIAN_POINT('Ctrl Pts',(3.55618577699069,2.0172568409508,-13.7363735960638)) ;
#167596=CARTESIAN_POINT('Ctrl Pts',(3.55727967686454,2.01800266699454,-13.7368678300958)) ;
#167597=CARTESIAN_POINT('Ctrl Pts',(3.55771141786834,2.01830156212325,-13.7370783189426)) ;
#167598=CARTESIAN_POINT('Ctrl Pts',(3.56202821818163,2.02133211263485,-13.7391706910972)) ;
#167599=CARTESIAN_POINT('Ctrl Pts',(3.56570108751487,2.02427663140646,-13.7422439316283)) ;
#167600=CARTESIAN_POINT('Ctrl Pts',(3.5699034772657,2.02797441535153,-13.7464020047385)) ;
#167601=CARTESIAN_POINT('Ctrl Pts',(3.57072473561131,2.02871480216325,-13.747249597731)) ;
#167602=CARTESIAN_POINT('Ctrl Pts',(3.57382863307621,2.03157464832067,-13.7505417189329)) ;
#167603=CARTESIAN_POINT('Ctrl Pts',(3.57597069376121,2.03369481096682,-13.7531377343573)) ;
#167604=CARTESIAN_POINT('Ctrl Pts',(3.58156103639367,2.03956384830232,-13.7607581167797)) ;
#167605=CARTESIAN_POINT('Ctrl Pts',(3.58475859790494,2.04336775308648,-13.7661548385216)) ;
#167606=CARTESIAN_POINT('Ctrl Pts',(3.58897725231935,2.0490105592432,-13.7749548343006)) ;
#167607=CARTESIAN_POINT('Ctrl Pts',(3.59034871903171,2.05099358132072,-13.7782225338432)) ;
#167608=CARTESIAN_POINT('Ctrl Pts',(3.5936548829273,2.05613355260447,-13.7872492286084)) ;
#167609=CARTESIAN_POINT('Ctrl Pts',(3.59534780095527,2.05919518104048,-13.7932437116103)) ;
#167610=CARTESIAN_POINT('Ctrl Pts',(3.59674625886213,2.06216860863467,-13.7999604466297)) ;
#167611=CARTESIAN_POINT('Ctrl Pts',(3.5968572528106,2.06240883133063,-13.8005103151097)) ;
#167612=CARTESIAN_POINT('Ctrl Pts',(3.59768573690243,2.06423460359409,-13.80474653762)) ;
#167613=CARTESIAN_POINT('Ctrl Pts',(3.59826864191792,2.06571343564803,-13.8085239971566)) ;
#167614=CARTESIAN_POINT('Ctrl Pts',(3.59959273712776,2.06963221119414,-13.8196830143691)) ;
#167615=CARTESIAN_POINT('Ctrl Pts',(3.6,2.07172309150643,-13.8272993579658)) ;
#167616=CARTESIAN_POINT('Ctrl Pts',(3.6,2.07320508075689,-13.835)) ;
#167617=CARTESIAN_POINT('Origin',(3.5,2.10000000000001,-1.01757522333835E-15)) ;
#167618=CARTESIAN_POINT('Origin',(3.5,2.1,-13.735)) ;
#167619=CARTESIAN_POINT('',(3.55,2.01339745962156,-12.935)) ;
#167620=CARTESIAN_POINT('Origin',(3.5,2.1,-12.935)) ;
#167621=CARTESIAN_POINT('Origin',(3.5,2.1,-12.935)) ;
#167622=CARTESIAN_POINT('Origin',(3.5,1.9,-12.935)) ;
#167623=CARTESIAN_POINT('Ctrl Pts',(3.6,2.07320508075689,-12.835)) ;
#167624=CARTESIAN_POINT('Ctrl Pts',(3.6,2.07265589924993,-12.8378535766702)) ;
#167625=CARTESIAN_POINT('Ctrl Pts',(3.59994554076638,2.07202433860046,-12.8406935800495)) ;
#167626=CARTESIAN_POINT('Ctrl Pts',(3.59971739924421,2.07059366100576,-12.8463792149776)) ;
#167627=CARTESIAN_POINT('Ctrl Pts',(3.5995415637343,2.0697927484707,-12.8492187363466)) ;
#167628=CARTESIAN_POINT('Ctrl Pts',(3.59880783141193,2.06712577191679,-12.8577808907248)) ;
#167629=CARTESIAN_POINT('Ctrl Pts',(3.59804129495592,2.06501902766401,-12.8634171364436)) ;
#167630=CARTESIAN_POINT('Ctrl Pts',(3.59624340061598,2.06105248659392,-12.8726335394636)) ;
#167631=CARTESIAN_POINT('Ctrl Pts',(3.59536494855695,2.05931170891995,-12.8763234713874)) ;
#167632=CARTESIAN_POINT('Ctrl Pts',(3.59283727202456,2.05479606436822,-12.8851994320584)) ;
#167633=CARTESIAN_POINT('Ctrl Pts',(3.5909965088313,2.05188276467182,-12.890344242006)) ;
#167634=CARTESIAN_POINT('Ctrl Pts',(3.58838944624354,2.04823719194735,-12.8962273766784)) ;
#167635=CARTESIAN_POINT('Ctrl Pts',(3.58794537962099,2.04762948672774,-12.8971909138509)) ;
#167636=CARTESIAN_POINT('Ctrl Pts',(3.58597371492279,2.04498948329048,-12.9013066517297)) ;
#167637=CARTESIAN_POINT('Ctrl Pts',(3.58430396743904,2.04289920268562,-12.9043931624803)) ;
#167638=CARTESIAN_POINT('Ctrl Pts',(3.58008903321359,2.03798436571149,-12.9112809206789)) ;
#167639=CARTESIAN_POINT('Ctrl Pts',(3.57743593401593,2.03513945367727,-12.9150015729205)) ;
#167640=CARTESIAN_POINT('Ctrl Pts',(3.57357563759675,2.03136250950857,-12.9195864015968)) ;
#167641=CARTESIAN_POINT('Ctrl Pts',(3.57257888733681,2.03041544381408,-12.9207065689314)) ;
#167642=CARTESIAN_POINT('Ctrl Pts',(3.56956839719853,2.02764175140703,-12.9239039077887)) ;
#167643=CARTESIAN_POINT('Ctrl Pts',(3.56746189551978,2.02581554544809,-12.9259843006788)) ;
#167644=CARTESIAN_POINT('Ctrl Pts',(3.56503628433215,2.02384076964169,-12.9280222600383)) ;
#167645=CARTESIAN_POINT('Ctrl Pts',(3.56481411023507,2.02366103014368,-12.9282058396877)) ;
#167646=CARTESIAN_POINT('Ctrl Pts',(3.56285239425758,2.02208416924061,-12.9297983821205)) ;
#167647=CARTESIAN_POINT('Ctrl Pts',(3.56093641846878,2.02061618613971,-12.9311871777518)) ;
#167648=CARTESIAN_POINT('Ctrl Pts',(3.55879736620769,2.01908299720838,-12.9323771402546)) ;
#167649=CARTESIAN_POINT('Ctrl Pts',(3.55867935922412,2.01899873301463,-12.9324417103524)) ;
#167650=CARTESIAN_POINT('Ctrl Pts',(3.55788953399555,2.01843691186422,-12.9328664833737)) ;
#167651=CARTESIAN_POINT('Ctrl Pts',(3.55720723474256,2.0179620002027,-12.933197549106)) ;
#167652=CARTESIAN_POINT('Ctrl Pts',(3.55509125643146,2.01652382826842,-12.9340979444515)) ;
#167653=CARTESIAN_POINT('Ctrl Pts',(3.55356547969779,2.01553571874057,-12.9346035613517)) ;
#167654=CARTESIAN_POINT('Ctrl Pts',(3.55133342567592,2.01417771500975,-12.9349447643996)) ;
#167655=CARTESIAN_POINT('Ctrl Pts',(3.55066861961523,2.01378348733639,-12.9349996317887)) ;
#167656=CARTESIAN_POINT('Ctrl Pts',(3.55,2.01339745962156,-12.935)) ;
#167657=CARTESIAN_POINT('Origin',(3.5,1.9,-17.545)) ;
#167658=CARTESIAN_POINT('',(3.55,2.01339745962156,-17.545)) ;
#167659=CARTESIAN_POINT('Origin',(3.5,2.1,-17.545)) ;
#167660=CARTESIAN_POINT('Ctrl Pts',(3.55,2.01339745962156,-17.545)) ;
#167661=CARTESIAN_POINT('Ctrl Pts',(3.55164546205118,2.01434746757975,-17.545)) ;
#167662=CARTESIAN_POINT('Ctrl Pts',(3.55326668047441,2.01534654795451,-17.5453329780303)) ;
#167663=CARTESIAN_POINT('Ctrl Pts',(3.55550702654633,2.01680421826672,-17.546098261683)) ;
#167664=CARTESIAN_POINT('Ctrl Pts',(3.55618577699068,2.01725684095079,-17.5463735960638)) ;
#167665=CARTESIAN_POINT('Ctrl Pts',(3.55727967686454,2.01800266699453,-17.5468678300958)) ;
#167666=CARTESIAN_POINT('Ctrl Pts',(3.55771141786834,2.01830156212325,-17.5470783189426)) ;
#167667=CARTESIAN_POINT('Ctrl Pts',(3.56202821818158,2.02133211263482,-17.5491706910972)) ;
#167668=CARTESIAN_POINT('Ctrl Pts',(3.56570108751479,2.02427663140639,-17.5522439316283)) ;
#167669=CARTESIAN_POINT('Ctrl Pts',(3.56990347726563,2.02797441535147,-17.5564020047385)) ;
#167670=CARTESIAN_POINT('Ctrl Pts',(3.57072473561127,2.02871480216322,-17.5572495977309)) ;
#167671=CARTESIAN_POINT('Ctrl Pts',(3.5738286330762,2.03157464832067,-17.5605417189329)) ;
#167672=CARTESIAN_POINT('Ctrl Pts',(3.5759706937612,2.03369481096682,-17.5631377343573)) ;
#167673=CARTESIAN_POINT('Ctrl Pts',(3.58156103639368,2.03956384830232,-17.5707581167797)) ;
#167674=CARTESIAN_POINT('Ctrl Pts',(3.58475859790495,2.04336775308648,-17.5761548385216)) ;
#167675=CARTESIAN_POINT('Ctrl Pts',(3.58897725231935,2.0490105592432,-17.5849548343006)) ;
#167676=CARTESIAN_POINT('Ctrl Pts',(3.59034871903171,2.05099358132072,-17.5882225338432)) ;
#167677=CARTESIAN_POINT('Ctrl Pts',(3.59365488292715,2.05613355260423,-17.597249228608)) ;
#167678=CARTESIAN_POINT('Ctrl Pts',(3.59534780095503,2.05919518104004,-17.6032437116095)) ;
#167679=CARTESIAN_POINT('Ctrl Pts',(3.59674625886195,2.06216860863428,-17.6099604466289)) ;
#167680=CARTESIAN_POINT('Ctrl Pts',(3.59685725281051,2.06240883133043,-17.6105103151092)) ;
#167681=CARTESIAN_POINT('Ctrl Pts',(3.59768573690243,2.06423460359408,-17.61474653762)) ;
#167682=CARTESIAN_POINT('Ctrl Pts',(3.59826864191792,2.06571343564803,-17.6185239971566)) ;
#167683=CARTESIAN_POINT('Ctrl Pts',(3.59959273712775,2.06963221119414,-17.6296830143691)) ;
#167684=CARTESIAN_POINT('Ctrl Pts',(3.6,2.07172309150643,-17.6372993579658)) ;
#167685=CARTESIAN_POINT('Ctrl Pts',(3.6,2.07320508075689,-17.645)) ;
#167686=CARTESIAN_POINT('Origin',(3.5,2.10000000000001,-1.01757522333836E-15)) ;
#167687=CARTESIAN_POINT('Origin',(3.5,2.1,-17.545)) ;
#167688=CARTESIAN_POINT('',(3.55,2.01339745962156,-16.745)) ;
#167689=CARTESIAN_POINT('Origin',(3.5,2.1,-16.745)) ;
#167690=CARTESIAN_POINT('Origin',(3.5,2.1,-16.745)) ;
#167691=CARTESIAN_POINT('Origin',(3.5,1.9,-16.745)) ;
#167692=CARTESIAN_POINT('Ctrl Pts',(3.6,2.07320508075689,-16.645)) ;
#167693=CARTESIAN_POINT('Ctrl Pts',(3.6,2.0724036454051,-16.6491643012255)) ;
#167694=CARTESIAN_POINT('Ctrl Pts',(3.59988358031788,2.07142604615684,-16.6532993264777)) ;
#167695=CARTESIAN_POINT('Ctrl Pts',(3.5992764543265,2.06860573724892,-16.6634232053159)) ;
#167696=CARTESIAN_POINT('Ctrl Pts',(3.59862250828209,2.06654864780065,-16.6694017962796)) ;
#167697=CARTESIAN_POINT('Ctrl Pts',(3.5974369582727,2.06370626825461,-16.6764308805049)) ;
#167698=CARTESIAN_POINT('Ctrl Pts',(3.59721441711742,2.06319475755342,-16.6776558946613)) ;
#167699=CARTESIAN_POINT('Ctrl Pts',(3.59624340061598,2.06105248659392,-16.6826335394636)) ;
#167700=CARTESIAN_POINT('Ctrl Pts',(3.59536494855695,2.05931170891994,-16.6863234713874)) ;
#167701=CARTESIAN_POINT('Ctrl Pts',(3.59283727202454,2.05479606436819,-16.6951994320585)) ;
#167702=CARTESIAN_POINT('Ctrl Pts',(3.59099650883127,2.05188276467178,-16.7003442420061)) ;
#167703=CARTESIAN_POINT('Ctrl Pts',(3.58838944624351,2.0482371919473,-16.7062273766785)) ;
#167704=CARTESIAN_POINT('Ctrl Pts',(3.58794537962097,2.04762948672772,-16.7071909138509)) ;
#167705=CARTESIAN_POINT('Ctrl Pts',(3.58597371492279,2.04498948329048,-16.7113066517297)) ;
#167706=CARTESIAN_POINT('Ctrl Pts',(3.58430396743904,2.04289920268562,-16.7143931624803)) ;
#167707=CARTESIAN_POINT('Ctrl Pts',(3.58008903321369,2.0379843657116,-16.7212809206788)) ;
#167708=CARTESIAN_POINT('Ctrl Pts',(3.57743593401614,2.03513945367749,-16.7250015729202)) ;
#167709=CARTESIAN_POINT('Ctrl Pts',(3.57357563759699,2.03136250950879,-16.7295864015965)) ;
#167710=CARTESIAN_POINT('Ctrl Pts',(3.57257888733693,2.03041544381418,-16.7307065689312)) ;
#167711=CARTESIAN_POINT('Ctrl Pts',(3.56956839719843,2.02764175140693,-16.7339039077887)) ;
#167712=CARTESIAN_POINT('Ctrl Pts',(3.56746189551956,2.0258155454479,-16.7359843006789)) ;
#167713=CARTESIAN_POINT('Ctrl Pts',(3.56503628433193,2.02384076964151,-16.7380222600385)) ;
#167714=CARTESIAN_POINT('Ctrl Pts',(3.56481411023496,2.02366103014359,-16.7382058396878)) ;
#167715=CARTESIAN_POINT('Ctrl Pts',(3.56285239425741,2.02208416924048,-16.7397983821207)) ;
#167716=CARTESIAN_POINT('Ctrl Pts',(3.56093641846842,2.02061618613943,-16.7411871777521)) ;
#167717=CARTESIAN_POINT('Ctrl Pts',(3.55879736620727,2.01908299720808,-16.7423771402549)) ;
#167718=CARTESIAN_POINT('Ctrl Pts',(3.55867935922384,2.01899873301443,-16.7424417103526)) ;
#167719=CARTESIAN_POINT('Ctrl Pts',(3.55788953399545,2.01843691186415,-16.7428664833738)) ;
#167720=CARTESIAN_POINT('Ctrl Pts',(3.55720723474251,2.01796200020267,-16.743197549106)) ;
#167721=CARTESIAN_POINT('Ctrl Pts',(3.55509125643154,2.01652382826847,-16.7440979444515)) ;
#167722=CARTESIAN_POINT('Ctrl Pts',(3.55356547969798,2.01553571874069,-16.7446035613516)) ;
#167723=CARTESIAN_POINT('Ctrl Pts',(3.55133342567611,2.01417771500986,-16.7449447643996)) ;
#167724=CARTESIAN_POINT('Ctrl Pts',(3.55066861961532,2.01378348733645,-16.7449996317888)) ;
#167725=CARTESIAN_POINT('Ctrl Pts',(3.55,2.01339745962156,-16.745)) ;
#167726=CARTESIAN_POINT('Origin',(3.5,1.9,-21.355)) ;
#167727=CARTESIAN_POINT('',(3.55,2.01339745962156,-21.355)) ;
#167728=CARTESIAN_POINT('Origin',(3.5,2.1,-21.355)) ;
#167729=CARTESIAN_POINT('Ctrl Pts',(3.55,2.01339745962156,-21.355)) ;
#167730=CARTESIAN_POINT('Ctrl Pts',(3.55164546205118,2.01434746757974,-21.355)) ;
#167731=CARTESIAN_POINT('Ctrl Pts',(3.5532666804744,2.01534654795451,-21.3553329780303)) ;
#167732=CARTESIAN_POINT('Ctrl Pts',(3.55550702654633,2.01680421826672,-21.356098261683)) ;
#167733=CARTESIAN_POINT('Ctrl Pts',(3.55618577699068,2.01725684095079,-21.3563735960638)) ;
#167734=CARTESIAN_POINT('Ctrl Pts',(3.55727967686454,2.01800266699453,-21.3568678300958)) ;
#167735=CARTESIAN_POINT('Ctrl Pts',(3.55771141786834,2.01830156212325,-21.3570783189426)) ;
#167736=CARTESIAN_POINT('Ctrl Pts',(3.56202821818158,2.02133211263481,-21.3591706910972)) ;
#167737=CARTESIAN_POINT('Ctrl Pts',(3.56570108751478,2.02427663140639,-21.3622439316283)) ;
#167738=CARTESIAN_POINT('Ctrl Pts',(3.56990347726562,2.02797441535147,-21.3664020047385)) ;
#167739=CARTESIAN_POINT('Ctrl Pts',(3.57072473561127,2.02871480216322,-21.3672495977309)) ;
#167740=CARTESIAN_POINT('Ctrl Pts',(3.5738286330762,2.03157464832067,-21.3705417189329)) ;
#167741=CARTESIAN_POINT('Ctrl Pts',(3.5759706937612,2.03369481096682,-21.3731377343573)) ;
#167742=CARTESIAN_POINT('Ctrl Pts',(3.58156103639368,2.03956384830231,-21.3807581167797)) ;
#167743=CARTESIAN_POINT('Ctrl Pts',(3.58475859790495,2.04336775308647,-21.3861548385216)) ;
#167744=CARTESIAN_POINT('Ctrl Pts',(3.58897725231935,2.04901055924319,-21.3949548343006)) ;
#167745=CARTESIAN_POINT('Ctrl Pts',(3.59034871903171,2.05099358132072,-21.3982225338432)) ;
#167746=CARTESIAN_POINT('Ctrl Pts',(3.59365488292718,2.05613355260427,-21.407249228608)) ;
#167747=CARTESIAN_POINT('Ctrl Pts',(3.59534780095507,2.05919518104011,-21.4132437116097)) ;
#167748=CARTESIAN_POINT('Ctrl Pts',(3.59674625886198,2.06216860863434,-21.419960446629)) ;
#167749=CARTESIAN_POINT('Ctrl Pts',(3.59685725281052,2.06240883133046,-21.4205103151093)) ;
#167750=CARTESIAN_POINT('Ctrl Pts',(3.59768573690243,2.06423460359408,-21.42474653762)) ;
#167751=CARTESIAN_POINT('Ctrl Pts',(3.59826864191791,2.06571343564803,-21.4285239971566)) ;
#167752=CARTESIAN_POINT('Ctrl Pts',(3.59959273712775,2.06963221119414,-21.4396830143691)) ;
#167753=CARTESIAN_POINT('Ctrl Pts',(3.6,2.07172309150643,-21.4472993579658)) ;
#167754=CARTESIAN_POINT('Ctrl Pts',(3.6,2.07320508075689,-21.455)) ;
#167755=CARTESIAN_POINT('Origin',(3.5,2.10000000000001,-1.01757522333836E-15)) ;
#167756=CARTESIAN_POINT('Origin',(3.5,2.1,-21.355)) ;
#167757=CARTESIAN_POINT('',(3.55,2.01339745962156,-20.555)) ;
#167758=CARTESIAN_POINT('Origin',(3.5,2.1,-20.555)) ;
#167759=CARTESIAN_POINT('Origin',(3.5,2.1,-20.555)) ;
#167760=CARTESIAN_POINT('Origin',(3.5,1.9,-20.555)) ;
#167761=CARTESIAN_POINT('Ctrl Pts',(3.6,2.07320508075689,-20.455)) ;
#167762=CARTESIAN_POINT('Ctrl Pts',(3.6,2.07265589924995,-20.45785357667)) ;
#167763=CARTESIAN_POINT('Ctrl Pts',(3.59994554076638,2.07202433860051,-20.4606935800491)) ;
#167764=CARTESIAN_POINT('Ctrl Pts',(3.59971739924421,2.07059366100571,-20.4663792149777)) ;
#167765=CARTESIAN_POINT('Ctrl Pts',(3.59954156373426,2.06979274847046,-20.4692187363474)) ;
#167766=CARTESIAN_POINT('Ctrl Pts',(3.5988078314118,2.06712577191645,-20.4777808907258)) ;
#167767=CARTESIAN_POINT('Ctrl Pts',(3.59804129495583,2.06501902766384,-20.4834171364441)) ;
#167768=CARTESIAN_POINT('Ctrl Pts',(3.59624340061598,2.06105248659392,-20.4926335394636)) ;
#167769=CARTESIAN_POINT('Ctrl Pts',(3.59536494855695,2.05931170891995,-20.4963234713874)) ;
#167770=CARTESIAN_POINT('Ctrl Pts',(3.59283727202454,2.05479606436819,-20.5051994320585)) ;
#167771=CARTESIAN_POINT('Ctrl Pts',(3.59099650883126,2.05188276467176,-20.5103442420061)) ;
#167772=CARTESIAN_POINT('Ctrl Pts',(3.58838944624349,2.04823719194729,-20.5162273766785)) ;
#167773=CARTESIAN_POINT('Ctrl Pts',(3.58794537962096,2.04762948672771,-20.5171909138509)) ;
#167774=CARTESIAN_POINT('Ctrl Pts',(3.58597371492279,2.04498948329048,-20.5213066517297)) ;
#167775=CARTESIAN_POINT('Ctrl Pts',(3.58430396743904,2.04289920268562,-20.5243931624803)) ;
#167776=CARTESIAN_POINT('Ctrl Pts',(3.58008903321371,2.03798436571163,-20.5312809206787)) ;
#167777=CARTESIAN_POINT('Ctrl Pts',(3.5774359340162,2.03513945367755,-20.5350015729202)) ;
#167778=CARTESIAN_POINT('Ctrl Pts',(3.57357563759705,2.03136250950885,-20.5395864015964)) ;
#167779=CARTESIAN_POINT('Ctrl Pts',(3.57257888733696,2.03041544381421,-20.5407065689312)) ;
#167780=CARTESIAN_POINT('Ctrl Pts',(3.56956839719839,2.0276417514069,-20.5439039077888)) ;
#167781=CARTESIAN_POINT('Ctrl Pts',(3.56746189551949,2.02581554544783,-20.545984300679)) ;
#167782=CARTESIAN_POINT('Ctrl Pts',(3.56503628433185,2.02384076964144,-20.5480222600386)) ;
#167783=CARTESIAN_POINT('Ctrl Pts',(3.56481411023492,2.02366103014355,-20.5482058396879)) ;
#167784=CARTESIAN_POINT('Ctrl Pts',(3.56285239425741,2.02208416924048,-20.5497983821207)) ;
#167785=CARTESIAN_POINT('Ctrl Pts',(3.56093641846842,2.02061618613943,-20.5511871777521)) ;
#167786=CARTESIAN_POINT('Ctrl Pts',(3.55879736620726,2.01908299720807,-20.5523771402549)) ;
#167787=CARTESIAN_POINT('Ctrl Pts',(3.55867935922383,2.01899873301443,-20.5524417103526)) ;
#167788=CARTESIAN_POINT('Ctrl Pts',(3.55788953399544,2.01843691186415,-20.5528664833738)) ;
#167789=CARTESIAN_POINT('Ctrl Pts',(3.55720723474251,2.01796200020267,-20.553197549106)) ;
#167790=CARTESIAN_POINT('Ctrl Pts',(3.55509125643154,2.01652382826847,-20.5540979444516)) ;
#167791=CARTESIAN_POINT('Ctrl Pts',(3.55356547969797,2.01553571874069,-20.5546035613518)) ;
#167792=CARTESIAN_POINT('Ctrl Pts',(3.55133342567611,2.01417771500986,-20.5549447643997)) ;
#167793=CARTESIAN_POINT('Ctrl Pts',(3.55066861961532,2.01378348733645,-20.5549996317888)) ;
#167794=CARTESIAN_POINT('Ctrl Pts',(3.55,2.01339745962156,-20.555)) ;
#167795=CARTESIAN_POINT('Origin',(3.5,1.9,-25.165)) ;
#167796=CARTESIAN_POINT('',(3.55,2.01339745962156,-25.165)) ;
#167797=CARTESIAN_POINT('Origin',(3.5,2.1,-25.165)) ;
#167798=CARTESIAN_POINT('Ctrl Pts',(3.55,2.01339745962156,-25.165)) ;
#167799=CARTESIAN_POINT('Ctrl Pts',(3.55164546205118,2.01434746757975,-25.165)) ;
#167800=CARTESIAN_POINT('Ctrl Pts',(3.55326668047441,2.01534654795451,-25.1653329780303)) ;
#167801=CARTESIAN_POINT('Ctrl Pts',(3.55550702654633,2.01680421826672,-25.166098261683)) ;
#167802=CARTESIAN_POINT('Ctrl Pts',(3.55618577699068,2.01725684095079,-25.1663735960638)) ;
#167803=CARTESIAN_POINT('Ctrl Pts',(3.55727967686454,2.01800266699453,-25.1668678300958)) ;
#167804=CARTESIAN_POINT('Ctrl Pts',(3.55771141786834,2.01830156212325,-25.1670783189426)) ;
#167805=CARTESIAN_POINT('Ctrl Pts',(3.56202821818159,2.02133211263482,-25.1691706910972)) ;
#167806=CARTESIAN_POINT('Ctrl Pts',(3.56570108751481,2.02427663140641,-25.1722439316283)) ;
#167807=CARTESIAN_POINT('Ctrl Pts',(3.56990347726564,2.02797441535149,-25.1764020047385)) ;
#167808=CARTESIAN_POINT('Ctrl Pts',(3.57072473561128,2.02871480216323,-25.1772495977309)) ;
#167809=CARTESIAN_POINT('Ctrl Pts',(3.57382863307621,2.03157464832067,-25.1805417189329)) ;
#167810=CARTESIAN_POINT('Ctrl Pts',(3.5759706937612,2.03369481096682,-25.1831377343573)) ;
#167811=CARTESIAN_POINT('Ctrl Pts',(3.58156103639368,2.03956384830231,-25.1907581167797)) ;
#167812=CARTESIAN_POINT('Ctrl Pts',(3.58475859790494,2.04336775308647,-25.1961548385216)) ;
#167813=CARTESIAN_POINT('Ctrl Pts',(3.58897725231935,2.04901055924319,-25.2049548343006)) ;
#167814=CARTESIAN_POINT('Ctrl Pts',(3.59034871903171,2.05099358132072,-25.2082225338432)) ;
#167815=CARTESIAN_POINT('Ctrl Pts',(3.5936548829272,2.0561335526043,-25.2172492286081)) ;
#167816=CARTESIAN_POINT('Ctrl Pts',(3.5953478009551,2.05919518104017,-25.2232437116098)) ;
#167817=CARTESIAN_POINT('Ctrl Pts',(3.596746258862,2.06216860863439,-25.2299604466291)) ;
#167818=CARTESIAN_POINT('Ctrl Pts',(3.59685725281053,2.06240883133048,-25.2305103151093)) ;
#167819=CARTESIAN_POINT('Ctrl Pts',(3.59768573690243,2.06423460359408,-25.23474653762)) ;
#167820=CARTESIAN_POINT('Ctrl Pts',(3.59826864191792,2.06571343564803,-25.2385239971565)) ;
#167821=CARTESIAN_POINT('Ctrl Pts',(3.59959273712775,2.06963221119414,-25.2496830143691)) ;
#167822=CARTESIAN_POINT('Ctrl Pts',(3.6,2.07172309150643,-25.2572993579658)) ;
#167823=CARTESIAN_POINT('Ctrl Pts',(3.6,2.07320508075689,-25.265)) ;
#167824=CARTESIAN_POINT('Origin',(3.5,2.10000000000001,-1.01757522333836E-15)) ;
#167825=CARTESIAN_POINT('Origin',(3.5,2.1,-25.165)) ;
#167826=CARTESIAN_POINT('',(3.55,2.01339745962156,-24.365)) ;
#167827=CARTESIAN_POINT('Origin',(3.5,2.1,-24.365)) ;
#167828=CARTESIAN_POINT('Origin',(3.5,2.1,-24.365)) ;
#167829=CARTESIAN_POINT('Origin',(3.5,1.9,-24.365)) ;
#167830=CARTESIAN_POINT('Ctrl Pts',(3.6,2.07320508075689,-24.265)) ;
#167831=CARTESIAN_POINT('Ctrl Pts',(3.6,2.07265589924987,-24.2678535766704)) ;
#167832=CARTESIAN_POINT('Ctrl Pts',(3.59994554076637,2.07202433860034,-24.27069358005)) ;
#167833=CARTESIAN_POINT('Ctrl Pts',(3.59971739924417,2.0705936610055,-24.2763792149785)) ;
#167834=CARTESIAN_POINT('Ctrl Pts',(3.59954156373423,2.06979274847036,-24.2792187363477)) ;
#167835=CARTESIAN_POINT('Ctrl Pts',(3.59880783141181,2.06712577191647,-24.2877808907257)) ;
#167836=CARTESIAN_POINT('Ctrl Pts',(3.59804129495584,2.06501902766384,-24.293417136444)) ;
#167837=CARTESIAN_POINT('Ctrl Pts',(3.59624340061598,2.06105248659392,-24.3026335394636)) ;
#167838=CARTESIAN_POINT('Ctrl Pts',(3.59536494855695,2.05931170891994,-24.3063234713874)) ;
#167839=CARTESIAN_POINT('Ctrl Pts',(3.59283727202457,2.05479606436824,-24.3151994320584)) ;
#167840=CARTESIAN_POINT('Ctrl Pts',(3.59099650883134,2.05188276467188,-24.3203442420059)) ;
#167841=CARTESIAN_POINT('Ctrl Pts',(3.58838944624358,2.04823719194741,-24.3262273766783)) ;
#167842=CARTESIAN_POINT('Ctrl Pts',(3.58794537962101,2.04762948672777,-24.3271909138508)) ;
#167843=CARTESIAN_POINT('Ctrl Pts',(3.58597371492279,2.04498948329048,-24.3313066517297)) ;
#167844=CARTESIAN_POINT('Ctrl Pts',(3.58430396743904,2.04289920268562,-24.3343931624803)) ;
#167845=CARTESIAN_POINT('Ctrl Pts',(3.58008903321372,2.03798436571164,-24.3412809206787)) ;
#167846=CARTESIAN_POINT('Ctrl Pts',(3.57743593401622,2.03513945367757,-24.3450015729201)) ;
#167847=CARTESIAN_POINT('Ctrl Pts',(3.57357563759708,2.03136250950888,-24.3495864015964)) ;
#167848=CARTESIAN_POINT('Ctrl Pts',(3.57257888733697,2.03041544381422,-24.3507065689311)) ;
#167849=CARTESIAN_POINT('Ctrl Pts',(3.56956839719845,2.02764175140695,-24.3539039077887)) ;
#167850=CARTESIAN_POINT('Ctrl Pts',(3.5674618955196,2.02581554544793,-24.3559843006788)) ;
#167851=CARTESIAN_POINT('Ctrl Pts',(3.56503628433197,2.02384076964154,-24.3580222600385)) ;
#167852=CARTESIAN_POINT('Ctrl Pts',(3.56481411023498,2.0236610301436,-24.3582058396878)) ;
#167853=CARTESIAN_POINT('Ctrl Pts',(3.5628523942574,2.02208416924047,-24.3597983821207)) ;
#167854=CARTESIAN_POINT('Ctrl Pts',(3.56093641846841,2.02061618613942,-24.3611871777521)) ;
#167855=CARTESIAN_POINT('Ctrl Pts',(3.55879736620725,2.01908299720807,-24.3623771402549)) ;
#167856=CARTESIAN_POINT('Ctrl Pts',(3.55867935922383,2.01899873301442,-24.3624417103526)) ;
#167857=CARTESIAN_POINT('Ctrl Pts',(3.55788953399544,2.01843691186415,-24.3628664833738)) ;
#167858=CARTESIAN_POINT('Ctrl Pts',(3.55720723474251,2.01796200020267,-24.363197549106)) ;
#167859=CARTESIAN_POINT('Ctrl Pts',(3.55509125643155,2.01652382826848,-24.3640979444516)) ;
#167860=CARTESIAN_POINT('Ctrl Pts',(3.55356547969799,2.0155357187407,-24.3646035613517)) ;
#167861=CARTESIAN_POINT('Ctrl Pts',(3.55133342567613,2.01417771500987,-24.3649447643996)) ;
#167862=CARTESIAN_POINT('Ctrl Pts',(3.55066861961533,2.01378348733645,-24.3649996317888)) ;
#167863=CARTESIAN_POINT('Ctrl Pts',(3.55,2.01339745962156,-24.365)) ;
#167864=CARTESIAN_POINT('Origin',(3.5,1.9,-28.975)) ;
#167865=CARTESIAN_POINT('',(3.55,2.01339745962156,-28.975)) ;
#167866=CARTESIAN_POINT('Origin',(3.5,2.1,-28.975)) ;
#167867=CARTESIAN_POINT('Ctrl Pts',(3.55,2.01339745962156,-28.975)) ;
#167868=CARTESIAN_POINT('Ctrl Pts',(3.55164546205118,2.01434746757975,-28.975)) ;
#167869=CARTESIAN_POINT('Ctrl Pts',(3.55326668047441,2.01534654795451,-28.9753329780303)) ;
#167870=CARTESIAN_POINT('Ctrl Pts',(3.55550702654633,2.01680421826672,-28.976098261683)) ;
#167871=CARTESIAN_POINT('Ctrl Pts',(3.55618577699068,2.01725684095079,-28.9763735960638)) ;
#167872=CARTESIAN_POINT('Ctrl Pts',(3.55727967686454,2.01800266699453,-28.9768678300958)) ;
#167873=CARTESIAN_POINT('Ctrl Pts',(3.55771141786834,2.01830156212325,-28.9770783189426)) ;
#167874=CARTESIAN_POINT('Ctrl Pts',(3.56202821818157,2.02133211263481,-28.9791706910972)) ;
#167875=CARTESIAN_POINT('Ctrl Pts',(3.56570108751476,2.02427663140637,-28.9822439316283)) ;
#167876=CARTESIAN_POINT('Ctrl Pts',(3.5699034772656,2.02797441535145,-28.9864020047384)) ;
#167877=CARTESIAN_POINT('Ctrl Pts',(3.57072473561126,2.02871480216321,-28.9872495977309)) ;
#167878=CARTESIAN_POINT('Ctrl Pts',(3.5738286330762,2.03157464832067,-28.9905417189329)) ;
#167879=CARTESIAN_POINT('Ctrl Pts',(3.5759706937612,2.03369481096682,-28.9931377343573)) ;
#167880=CARTESIAN_POINT('Ctrl Pts',(3.58156103639367,2.03956384830231,-29.0007581167797)) ;
#167881=CARTESIAN_POINT('Ctrl Pts',(3.58475859790494,2.04336775308647,-29.0061548385216)) ;
#167882=CARTESIAN_POINT('Ctrl Pts',(3.58897725231935,2.04901055924319,-29.0149548343006)) ;
#167883=CARTESIAN_POINT('Ctrl Pts',(3.59034871903171,2.05099358132072,-29.0182225338432)) ;
#167884=CARTESIAN_POINT('Ctrl Pts',(3.59365488292715,2.05613355260422,-29.0272492286079)) ;
#167885=CARTESIAN_POINT('Ctrl Pts',(3.59534780095502,2.05919518104002,-29.0332437116095)) ;
#167886=CARTESIAN_POINT('Ctrl Pts',(3.59674625886194,2.06216860863426,-29.0399604466288)) ;
#167887=CARTESIAN_POINT('Ctrl Pts',(3.5968572528105,2.06240883133042,-29.0405103151092)) ;
#167888=CARTESIAN_POINT('Ctrl Pts',(3.59768573690243,2.06423460359408,-29.04474653762)) ;
#167889=CARTESIAN_POINT('Ctrl Pts',(3.59826864191791,2.06571343564803,-29.0485239971566)) ;
#167890=CARTESIAN_POINT('Ctrl Pts',(3.59959273712775,2.06963221119414,-29.0596830143691)) ;
#167891=CARTESIAN_POINT('Ctrl Pts',(3.6,2.07172309150643,-29.0672993579658)) ;
#167892=CARTESIAN_POINT('Ctrl Pts',(3.6,2.07320508075689,-29.075)) ;
#167893=CARTESIAN_POINT('Origin',(3.5,2.10000000000001,-1.01757522333836E-15)) ;
#167894=CARTESIAN_POINT('Origin',(3.5,2.1,-28.975)) ;
#167895=CARTESIAN_POINT('',(3.55,2.01339745962156,-28.175)) ;
#167896=CARTESIAN_POINT('Origin',(3.5,2.1,-28.175)) ;
#167897=CARTESIAN_POINT('Origin',(3.5,2.1,-28.175)) ;
#167898=CARTESIAN_POINT('Origin',(3.5,1.9,-28.175)) ;
#167899=CARTESIAN_POINT('Ctrl Pts',(3.6,2.07320508075689,-28.075)) ;
#167900=CARTESIAN_POINT('Ctrl Pts',(3.6,2.0724036454051,-28.0791643012255)) ;
#167901=CARTESIAN_POINT('Ctrl Pts',(3.59988358031788,2.07142604615684,-28.0832993264777)) ;
#167902=CARTESIAN_POINT('Ctrl Pts',(3.5992764543265,2.06860573724893,-28.0934232053159)) ;
#167903=CARTESIAN_POINT('Ctrl Pts',(3.59862250828209,2.06654864780066,-28.0994017962796)) ;
#167904=CARTESIAN_POINT('Ctrl Pts',(3.5974369582727,2.06370626825463,-28.1064308805049)) ;
#167905=CARTESIAN_POINT('Ctrl Pts',(3.59721441711742,2.06319475755343,-28.1076558946613)) ;
#167906=CARTESIAN_POINT('Ctrl Pts',(3.59624340061598,2.06105248659392,-28.1126335394636)) ;
#167907=CARTESIAN_POINT('Ctrl Pts',(3.59536494855695,2.05931170891995,-28.1163234713874)) ;
#167908=CARTESIAN_POINT('Ctrl Pts',(3.59283727202455,2.0547960643682,-28.1251994320585)) ;
#167909=CARTESIAN_POINT('Ctrl Pts',(3.59099650883128,2.05188276467179,-28.1303442420061)) ;
#167910=CARTESIAN_POINT('Ctrl Pts',(3.58838944624352,2.04823719194732,-28.1362273766785)) ;
#167911=CARTESIAN_POINT('Ctrl Pts',(3.58794537962097,2.04762948672773,-28.1371909138509)) ;
#167912=CARTESIAN_POINT('Ctrl Pts',(3.58597371492279,2.04498948329048,-28.1413066517297)) ;
#167913=CARTESIAN_POINT('Ctrl Pts',(3.58430396743904,2.04289920268562,-28.1443931624803)) ;
#167914=CARTESIAN_POINT('Ctrl Pts',(3.58008903321371,2.03798436571163,-28.1512809206787)) ;
#167915=CARTESIAN_POINT('Ctrl Pts',(3.5774359340162,2.03513945367755,-28.1550015729202)) ;
#167916=CARTESIAN_POINT('Ctrl Pts',(3.57357563759705,2.03136250950885,-28.1595864015964)) ;
#167917=CARTESIAN_POINT('Ctrl Pts',(3.57257888733696,2.03041544381421,-28.1607065689312)) ;
#167918=CARTESIAN_POINT('Ctrl Pts',(3.5695683971984,2.0276417514069,-28.1639039077888)) ;
#167919=CARTESIAN_POINT('Ctrl Pts',(3.5674618955195,2.02581554544784,-28.1659843006789)) ;
#167920=CARTESIAN_POINT('Ctrl Pts',(3.56503628433186,2.02384076964145,-28.1680222600386)) ;
#167921=CARTESIAN_POINT('Ctrl Pts',(3.56481411023493,2.02366103014356,-28.1682058396879)) ;
#167922=CARTESIAN_POINT('Ctrl Pts',(3.56285239425745,2.02208416924051,-28.1697983821206)) ;
#167923=CARTESIAN_POINT('Ctrl Pts',(3.5609364184685,2.02061618613949,-28.171187177752)) ;
#167924=CARTESIAN_POINT('Ctrl Pts',(3.55879736620735,2.01908299720814,-28.1723771402548)) ;
#167925=CARTESIAN_POINT('Ctrl Pts',(3.55867935922389,2.01899873301446,-28.1724417103525)) ;
#167926=CARTESIAN_POINT('Ctrl Pts',(3.55788953399546,2.01843691186416,-28.1728664833738)) ;
#167927=CARTESIAN_POINT('Ctrl Pts',(3.55720723474251,2.01796200020267,-28.173197549106)) ;
#167928=CARTESIAN_POINT('Ctrl Pts',(3.55509125643154,2.01652382826847,-28.1740979444515)) ;
#167929=CARTESIAN_POINT('Ctrl Pts',(3.55356547969798,2.01553571874069,-28.1746035613518)) ;
#167930=CARTESIAN_POINT('Ctrl Pts',(3.55133342567612,2.01417771500986,-28.1749447643997)) ;
#167931=CARTESIAN_POINT('Ctrl Pts',(3.55066861961533,2.01378348733645,-28.1749996317888)) ;
#167932=CARTESIAN_POINT('Ctrl Pts',(3.55,2.01339745962156,-28.175)) ;
#167933=CARTESIAN_POINT('Origin',(3.5,1.9,-32.785)) ;
#167934=CARTESIAN_POINT('',(3.55,2.01339745962156,-32.785)) ;
#167935=CARTESIAN_POINT('Origin',(3.5,2.1,-32.785)) ;
#167936=CARTESIAN_POINT('Ctrl Pts',(3.55,2.01339745962156,-32.785)) ;
#167937=CARTESIAN_POINT('Ctrl Pts',(3.5516454620512,2.01434746757976,-32.7850000000001)) ;
#167938=CARTESIAN_POINT('Ctrl Pts',(3.55326668047444,2.01534654795453,-32.7853329780303)) ;
#167939=CARTESIAN_POINT('Ctrl Pts',(3.55550702654636,2.01680421826674,-32.7860982616831)) ;
#167940=CARTESIAN_POINT('Ctrl Pts',(3.55618577699069,2.0172568409508,-32.7863735960638)) ;
#167941=CARTESIAN_POINT('Ctrl Pts',(3.55727967686453,2.01800266699453,-32.7868678300958)) ;
#167942=CARTESIAN_POINT('Ctrl Pts',(3.55771141786833,2.01830156212324,-32.7870783189426)) ;
#167943=CARTESIAN_POINT('Ctrl Pts',(3.56202821818145,2.02133211263472,-32.7891706910972)) ;
#167944=CARTESIAN_POINT('Ctrl Pts',(3.56570108751455,2.02427663140619,-32.7922439316281)) ;
#167945=CARTESIAN_POINT('Ctrl Pts',(3.56990347726541,2.02797441535127,-32.7964020047383)) ;
#167946=CARTESIAN_POINT('Ctrl Pts',(3.57072473561116,2.02871480216311,-32.7972495977309)) ;
#167947=CARTESIAN_POINT('Ctrl Pts',(3.5738286330762,2.03157464832066,-32.8005417189329)) ;
#167948=CARTESIAN_POINT('Ctrl Pts',(3.5759706937612,2.03369481096681,-32.8031377343573)) ;
#167949=CARTESIAN_POINT('Ctrl Pts',(3.58156103639367,2.03956384830231,-32.8107581167798)) ;
#167950=CARTESIAN_POINT('Ctrl Pts',(3.58475859790494,2.04336775308647,-32.8161548385216)) ;
#167951=CARTESIAN_POINT('Ctrl Pts',(3.58897725231935,2.04901055924319,-32.8249548343006)) ;
#167952=CARTESIAN_POINT('Ctrl Pts',(3.59034871903171,2.05099358132071,-32.8282225338432)) ;
#167953=CARTESIAN_POINT('Ctrl Pts',(3.59365488292739,2.0561335526046,-32.8372492286086)) ;
#167954=CARTESIAN_POINT('Ctrl Pts',(3.59534780095541,2.05919518104073,-32.8432437116108)) ;
#167955=CARTESIAN_POINT('Ctrl Pts',(3.59674625886223,2.06216860863489,-32.8499604466302)) ;
#167956=CARTESIAN_POINT('Ctrl Pts',(3.59685725281065,2.06240883133073,-32.8505103151099)) ;
#167957=CARTESIAN_POINT('Ctrl Pts',(3.59768573690243,2.06423460359408,-32.85474653762)) ;
#167958=CARTESIAN_POINT('Ctrl Pts',(3.59826864191792,2.06571343564803,-32.8585239971566)) ;
#167959=CARTESIAN_POINT('Ctrl Pts',(3.59959273712776,2.06963221119414,-32.8696830143691)) ;
#167960=CARTESIAN_POINT('Ctrl Pts',(3.6,2.07172309150643,-32.8772993579658)) ;
#167961=CARTESIAN_POINT('Ctrl Pts',(3.6,2.07320508075689,-32.885)) ;
#167962=CARTESIAN_POINT('Origin',(3.5,2.10000000000002,-1.01757522333836E-15)) ;
#167963=CARTESIAN_POINT('Origin',(3.5,2.1,-32.785)) ;
#167964=CARTESIAN_POINT('',(3.55,2.01339745962156,-31.985)) ;
#167965=CARTESIAN_POINT('Origin',(3.5,2.1,-31.985)) ;
#167966=CARTESIAN_POINT('Origin',(3.5,2.1,-31.985)) ;
#167967=CARTESIAN_POINT('Origin',(3.5,1.9,-31.985)) ;
#167968=CARTESIAN_POINT('Ctrl Pts',(3.6,2.07320508075689,-31.885)) ;
#167969=CARTESIAN_POINT('Ctrl Pts',(3.6,2.07240364540511,-31.8891643012255)) ;
#167970=CARTESIAN_POINT('Ctrl Pts',(3.59988358031788,2.07142604615685,-31.8932993264777)) ;
#167971=CARTESIAN_POINT('Ctrl Pts',(3.59927645432651,2.06860573724896,-31.9034232053158)) ;
#167972=CARTESIAN_POINT('Ctrl Pts',(3.59862250828212,2.06654864780071,-31.9094017962794)) ;
#167973=CARTESIAN_POINT('Ctrl Pts',(3.59743695827272,2.06370626825467,-31.9164308805048)) ;
#167974=CARTESIAN_POINT('Ctrl Pts',(3.59721441711744,2.06319475755345,-31.9176558946612)) ;
#167975=CARTESIAN_POINT('Ctrl Pts',(3.59624340061598,2.06105248659392,-31.9226335394636)) ;
#167976=CARTESIAN_POINT('Ctrl Pts',(3.59536494855695,2.05931170891994,-31.9263234713874)) ;
#167977=CARTESIAN_POINT('Ctrl Pts',(3.59283727202455,2.0547960643682,-31.9351994320585)) ;
#167978=CARTESIAN_POINT('Ctrl Pts',(3.59099650883129,2.0518827646718,-31.940344242006)) ;
#167979=CARTESIAN_POINT('Ctrl Pts',(3.58838944624353,2.04823719194733,-31.9462273766785)) ;
#167980=CARTESIAN_POINT('Ctrl Pts',(3.58794537962098,2.04762948672773,-31.9471909138509)) ;
#167981=CARTESIAN_POINT('Ctrl Pts',(3.58597371492279,2.04498948329048,-31.9513066517297)) ;
#167982=CARTESIAN_POINT('Ctrl Pts',(3.58430396743904,2.04289920268562,-31.9543931624802)) ;
#167983=CARTESIAN_POINT('Ctrl Pts',(3.58008903321372,2.03798436571164,-31.9612809206787)) ;
#167984=CARTESIAN_POINT('Ctrl Pts',(3.57743593401621,2.03513945367757,-31.9650015729201)) ;
#167985=CARTESIAN_POINT('Ctrl Pts',(3.57357563759707,2.03136250950887,-31.9695864015964)) ;
#167986=CARTESIAN_POINT('Ctrl Pts',(3.57257888733696,2.03041544381421,-31.9707065689311)) ;
#167987=CARTESIAN_POINT('Ctrl Pts',(3.56956839719855,2.02764175140704,-31.9739039077886)) ;
#167988=CARTESIAN_POINT('Ctrl Pts',(3.56746189551982,2.02581554544812,-31.9759843006786)) ;
#167989=CARTESIAN_POINT('Ctrl Pts',(3.5650362843322,2.02384076964172,-31.9780222600382)) ;
#167990=CARTESIAN_POINT('Ctrl Pts',(3.5648141102351,2.02366103014369,-31.9782058396877)) ;
#167991=CARTESIAN_POINT('Ctrl Pts',(3.56285239425763,2.02208416924065,-31.9797983821204)) ;
#167992=CARTESIAN_POINT('Ctrl Pts',(3.56093641846891,2.0206161861398,-31.9811871777517)) ;
#167993=CARTESIAN_POINT('Ctrl Pts',(3.55879736620774,2.01908299720842,-31.9823771402546)) ;
#167994=CARTESIAN_POINT('Ctrl Pts',(3.55867935922403,2.01899873301456,-31.9824417103524)) ;
#167995=CARTESIAN_POINT('Ctrl Pts',(3.55788953399539,2.01843691186411,-31.9828664833738)) ;
#167996=CARTESIAN_POINT('Ctrl Pts',(3.55720723474248,2.01796200020265,-31.983197549106)) ;
#167997=CARTESIAN_POINT('Ctrl Pts',(3.55509125643159,2.01652382826851,-31.9840979444515)) ;
#167998=CARTESIAN_POINT('Ctrl Pts',(3.55356547969806,2.01553571874074,-31.9846035613517)) ;
#167999=CARTESIAN_POINT('Ctrl Pts',(3.55133342567619,2.01417771500991,-31.9849447643996)) ;
#168000=CARTESIAN_POINT('Ctrl Pts',(3.55066861961536,2.01378348733647,-31.9849996317887)) ;
#168001=CARTESIAN_POINT('Ctrl Pts',(3.55,2.01339745962156,-31.985)) ;
#168002=CARTESIAN_POINT('Origin',(3.5,2.10000000000002,-1.01757522333836E-15)) ;
#168003=CARTESIAN_POINT('Origin',(3.5,2.1,-36.49)) ;
#168004=CARTESIAN_POINT('',(3.55,2.01339745962156,-35.795)) ;
#168005=CARTESIAN_POINT('Origin',(3.5,2.1,-35.795)) ;
#168006=CARTESIAN_POINT('Origin',(3.5,2.1,-35.795)) ;
#168007=CARTESIAN_POINT('Origin',(3.5,1.9,-35.795)) ;
#168008=CARTESIAN_POINT('Ctrl Pts',(3.6,2.07320508075689,-35.695)) ;
#168009=CARTESIAN_POINT('Ctrl Pts',(3.6,2.07240364540511,-35.6991643012256)) ;
#168010=CARTESIAN_POINT('Ctrl Pts',(3.59988358031788,2.07142604615685,-35.7032993264777)) ;
#168011=CARTESIAN_POINT('Ctrl Pts',(3.59927645432651,2.06860573724896,-35.7134232053158)) ;
#168012=CARTESIAN_POINT('Ctrl Pts',(3.59862250828211,2.0665486478007,-35.7194017962795)) ;
#168013=CARTESIAN_POINT('Ctrl Pts',(3.59743695827272,2.06370626825466,-35.7264308805048)) ;
#168014=CARTESIAN_POINT('Ctrl Pts',(3.59721441711743,2.06319475755345,-35.7276558946612)) ;
#168015=CARTESIAN_POINT('Ctrl Pts',(3.59624340061598,2.06105248659392,-35.7326335394636)) ;
#168016=CARTESIAN_POINT('Ctrl Pts',(3.59536494855695,2.05931170891994,-35.7363234713874)) ;
#168017=CARTESIAN_POINT('Ctrl Pts',(3.59283727202456,2.05479606436823,-35.7451994320584)) ;
#168018=CARTESIAN_POINT('Ctrl Pts',(3.59099650883132,2.05188276467186,-35.7503442420059)) ;
#168019=CARTESIAN_POINT('Ctrl Pts',(3.58838944624357,2.04823719194739,-35.7562273766784)) ;
#168020=CARTESIAN_POINT('Ctrl Pts',(3.587945379621,2.04762948672776,-35.7571909138508)) ;
#168021=CARTESIAN_POINT('Ctrl Pts',(3.58597371492279,2.04498948329048,-35.7613066517297)) ;
#168022=CARTESIAN_POINT('Ctrl Pts',(3.58430396743904,2.04289920268562,-35.7643931624803)) ;
#168023=CARTESIAN_POINT('Ctrl Pts',(3.58008903321367,2.03798436571158,-35.7712809206788)) ;
#168024=CARTESIAN_POINT('Ctrl Pts',(3.57743593401611,2.03513945367745,-35.7750015729203)) ;
#168025=CARTESIAN_POINT('Ctrl Pts',(3.57357563759695,2.03136250950875,-35.7795864015965)) ;
#168026=CARTESIAN_POINT('Ctrl Pts',(3.5725788873369,2.03041544381416,-35.7807065689312)) ;
#168027=CARTESIAN_POINT('Ctrl Pts',(3.56956839719846,2.02764175140696,-35.7839039077887)) ;
#168028=CARTESIAN_POINT('Ctrl Pts',(3.56746189551964,2.02581554544796,-35.7859843006788)) ;
#168029=CARTESIAN_POINT('Ctrl Pts',(3.565036284332,2.02384076964157,-35.7880222600384)) ;
#168030=CARTESIAN_POINT('Ctrl Pts',(3.564814110235,2.02366103014362,-35.7882058396878)) ;
#168031=CARTESIAN_POINT('Ctrl Pts',(3.56285239425736,2.02208416924043,-35.7897983821207)) ;
#168032=CARTESIAN_POINT('Ctrl Pts',(3.5609364184683,2.02061618613934,-35.7911871777521)) ;
#168033=CARTESIAN_POINT('Ctrl Pts',(3.55879736620711,2.01908299720796,-35.7923771402549)) ;
#168034=CARTESIAN_POINT('Ctrl Pts',(3.55867935922371,2.01899873301434,-35.7924417103526)) ;
#168035=CARTESIAN_POINT('Ctrl Pts',(3.55788953399539,2.01843691186411,-35.7928664833738)) ;
#168036=CARTESIAN_POINT('Ctrl Pts',(3.55720723474248,2.01796200020265,-35.793197549106)) ;
#168037=CARTESIAN_POINT('Ctrl Pts',(3.55509125643159,2.01652382826851,-35.7940979444515)) ;
#168038=CARTESIAN_POINT('Ctrl Pts',(3.55356547969807,2.01553571874075,-35.7946035613517)) ;
#168039=CARTESIAN_POINT('Ctrl Pts',(3.55133342567621,2.01417771500992,-35.7949447643996)) ;
#168040=CARTESIAN_POINT('Ctrl Pts',(3.55066861961537,2.01378348733647,-35.7949996317887)) ;
#168041=CARTESIAN_POINT('Ctrl Pts',(3.55,2.01339745962156,-35.795)) ;
#168042=CARTESIAN_POINT('Origin',(3.7,2.1,-5.115)) ;
#168043=CARTESIAN_POINT('',(3.7,1.98660254037844,-5.165)) ;
#168044=CARTESIAN_POINT('Ctrl Pts',(3.60000000000001,1.92679491924311,-5.215)) ;
#168045=CARTESIAN_POINT('Ctrl Pts',(3.60642117639485,1.92803067521647,-5.215)) ;
#168046=CARTESIAN_POINT('Ctrl Pts',(3.61278477806504,1.92968896670924,-5.21472281361407)) ;
#168047=CARTESIAN_POINT('Ctrl Pts',(3.61897283239529,1.93170032347262,-5.21412352491366)) ;
#168048=CARTESIAN_POINT('Ctrl Pts',(3.62020584678442,1.93210110079269,-5.21400411232427)) ;
#168049=CARTESIAN_POINT('Ctrl Pts',(3.62143195421093,1.93251577262755,-5.21387200280826)) ;
#168050=CARTESIAN_POINT('Ctrl Pts',(3.62265032708637,1.93294361409314,-5.21372698243403)) ;
#168051=CARTESIAN_POINT('Ctrl Pts',(3.62647624625549,1.9342871164786,-5.21327159128008)) ;
#168052=CARTESIAN_POINT('Ctrl Pts',(3.63025346237246,1.93576539638805,-5.21268573681767)) ;
#168053=CARTESIAN_POINT('Ctrl Pts',(3.6339385638818,1.93735364065939,-5.21196503626974)) ;
#168054=CARTESIAN_POINT('Ctrl Pts',(3.63907793749079,1.93956866259898,-5.21095992165713)) ;
#168055=CARTESIAN_POINT('Ctrl Pts',(3.64410916187594,1.9420207691991,-5.20967872244963)) ;
#168056=CARTESIAN_POINT('Ctrl Pts',(3.64894317395081,1.94461872744766,-5.20812217773586)) ;
#168057=CARTESIAN_POINT('Ctrl Pts',(3.64993855309172,1.94515367717669,-5.20780166712976)) ;
#168058=CARTESIAN_POINT('Ctrl Pts',(3.65092568100078,1.94569474416707,-5.20746960315685)) ;
#168059=CARTESIAN_POINT('Ctrl Pts',(3.65190395907094,1.94624104404949,-5.20712618093672)) ;
#168060=CARTESIAN_POINT('Ctrl Pts',(3.6524134286835,1.94652554719632,-5.20694733282516)) ;
#168061=CARTESIAN_POINT('Ctrl Pts',(3.65292046817499,1.94681147780209,-5.20676540574)) ;
#168062=CARTESIAN_POINT('Ctrl Pts',(3.65342498214111,1.94709871486665,-5.20658043363331)) ;
#168063=CARTESIAN_POINT('Ctrl Pts',(3.65677402871197,1.94900544167845,-5.20535255840841)) ;
#168064=CARTESIAN_POINT('Ctrl Pts',(3.66003813592315,1.95098496635821,-5.20398063668092)) ;
#168065=CARTESIAN_POINT('Ctrl Pts',(3.66320312645638,1.95301617633166,-5.20246240139399)) ;
#168066=CARTESIAN_POINT('Ctrl Pts',(3.66757373088823,1.95582111846932,-5.20036583718505)) ;
#168067=CARTESIAN_POINT('Ctrl Pts',(3.67181875309394,1.95875330073085,-5.19796612617077)) ;
#168068=CARTESIAN_POINT('Ctrl Pts',(3.67584388612554,1.96174615985082,-5.19526003578551)) ;
#168069=CARTESIAN_POINT('Ctrl Pts',(3.67661208162804,1.96231734616877,-5.1947435791996)) ;
#168070=CARTESIAN_POINT('Ctrl Pts',(3.6773723784937,1.96289065080929,-5.19421601587661)) ;
#168071=CARTESIAN_POINT('Ctrl Pts',(3.67812428214755,1.96346549105991,-5.1936773988359)) ;
#168072=CARTESIAN_POINT('Ctrl Pts',(3.6785349394885,1.96377944400799,-5.19338322944252)) ;
#168073=CARTESIAN_POINT('Ctrl Pts',(3.67894301851534,1.96409388168819,-5.19308575174331)) ;
#168074=CARTESIAN_POINT('Ctrl Pts',(3.67934840022277,1.96440871854257,-5.19278496939811)) ;
#168075=CARTESIAN_POINT('Ctrl Pts',(3.68198440184427,1.96645595067818,-5.19082912695353)) ;
#168076=CARTESIAN_POINT('Ctrl Pts',(3.68449751351864,1.96851545671307,-5.18873828347164)) ;
#168077=CARTESIAN_POINT('Ctrl Pts',(3.68685379133723,1.97055696562013,-5.18652085039877)) ;
#168078=CARTESIAN_POINT('Ctrl Pts',(3.68896164651385,1.97238323800785,-5.18453720155032)) ;
#168079=CARTESIAN_POINT('Ctrl Pts',(3.69104797813205,1.97419718002547,-5.18244243877983)) ;
#168080=CARTESIAN_POINT('Ctrl Pts',(3.69290978292493,1.97598569412168,-5.18024500103231)) ;
#168081=CARTESIAN_POINT('Ctrl Pts',(3.69362192319645,1.97666980070416,-5.17940448116676)) ;
#168082=CARTESIAN_POINT('Ctrl Pts',(3.69430163271861,1.97734979318971,-5.17854897561523)) ;
#168083=CARTESIAN_POINT('Ctrl Pts',(3.69493905694205,1.97802369895108,-5.17767908836304)) ;
#168084=CARTESIAN_POINT('Ctrl Pts',(3.69605143900785,1.9791997456958,-5.17616103030527)) ;
#168085=CARTESIAN_POINT('Ctrl Pts',(3.69703421735413,1.98035885502255,-5.1745986233173)) ;
#168086=CARTESIAN_POINT('Ctrl Pts',(3.6978475066491,1.98151165953424,-5.17295719153115)) ;
#168087=CARTESIAN_POINT('Ctrl Pts',(3.69841279947843,1.98231293913807,-5.17181628186435)) ;
#168088=CARTESIAN_POINT('Ctrl Pts',(3.69890310384953,1.98311438470598,-5.17063324801215)) ;
#168089=CARTESIAN_POINT('Ctrl Pts',(3.69929098301994,1.98393783265455,-5.1693581070746)) ;
#168090=CARTESIAN_POINT('Ctrl Pts',(3.69936193271525,1.98408845528529,-5.16912486211612)) ;
#168091=CARTESIAN_POINT('Ctrl Pts',(3.69942931950317,1.98423979370566,-5.16888851468591)) ;
#168092=CARTESIAN_POINT('Ctrl Pts',(3.69949277412724,1.98439195189924,-5.16864873028523)) ;
#168093=CARTESIAN_POINT('Ctrl Pts',(3.69967702385849,1.98483376534755,-5.16795248139832)) ;
#168094=CARTESIAN_POINT('Ctrl Pts',(3.69981936684305,1.98527475083258,-5.16723933425853)) ;
#168095=CARTESIAN_POINT('Ctrl Pts',(3.69990669142684,1.98570953653121,-5.16651584102814)) ;
#168096=CARTESIAN_POINT('Ctrl Pts',(3.69996666908332,1.98600816294479,-5.16601891992581)) ;
#168097=CARTESIAN_POINT('Ctrl Pts',(3.7,1.98630780592128,-5.16551049505454)) ;
#168098=CARTESIAN_POINT('Ctrl Pts',(3.7,1.98660254037844,-5.165)) ;
#168099=CARTESIAN_POINT('Origin',(3.7,1.9,-5.115)) ;
#168100=CARTESIAN_POINT('Origin',(10.2,1.9,-5.115)) ;
#168101=CARTESIAN_POINT('Origin',(3.7,1.9,-5.115)) ;
#168102=CARTESIAN_POINT('Origin',(10.1,1.9,-5.115)) ;
#168103=CARTESIAN_POINT('Origin',(10.1,1.9,-5.115)) ;
#168104=CARTESIAN_POINT('Origin',(3.7,2.1,-2.505)) ;
#168105=CARTESIAN_POINT('',(3.7,1.98660254037844,-2.455)) ;
#168106=CARTESIAN_POINT('Origin',(3.7,1.9,-2.505)) ;
#168107=CARTESIAN_POINT('Ctrl Pts',(3.7,1.98660254037844,-2.455)) ;
#168108=CARTESIAN_POINT('Ctrl Pts',(3.69999911718144,1.98567700534182,-2.45339692629239)) ;
#168109=CARTESIAN_POINT('Ctrl Pts',(3.69968163901485,1.984703699336,-2.45181800228455)) ;
#168110=CARTESIAN_POINT('Ctrl Pts',(3.69895427931585,1.98325895404995,-2.44959445604081)) ;
#168111=CARTESIAN_POINT('Ctrl Pts',(3.69867650892745,1.98278649590681,-2.44888609842392)) ;
#168112=CARTESIAN_POINT('Ctrl Pts',(3.69717970712967,1.9804354328423,-2.44544091878433)) ;
#168113=CARTESIAN_POINT('Ctrl Pts',(3.69541014605544,1.97847095301992,-2.44282412084427)) ;
#168114=CARTESIAN_POINT('Ctrl Pts',(3.69146029518774,1.97457001268155,-2.43797344350903)) ;
#168115=CARTESIAN_POINT('Ctrl Pts',(3.68915436790411,1.97254004967205,-2.43563220687652)) ;
#168116=CARTESIAN_POINT('Ctrl Pts',(3.68263623161792,1.9668885044718,-2.42949991845677)) ;
#168117=CARTESIAN_POINT('Ctrl Pts',(3.67796661383159,1.96321337091313,-2.42597925228307)) ;
#168118=CARTESIAN_POINT('Ctrl Pts',(3.67279117399678,1.95950210067477,-2.42276234339455)) ;
#168119=CARTESIAN_POINT('Ctrl Pts',(3.67252519027994,1.95931231248683,-2.42259880905816)) ;
#168120=CARTESIAN_POINT('Ctrl Pts',(3.6693311210617,1.95704457126181,-2.42065620430678)) ;
#168121=CARTESIAN_POINT('Ctrl Pts',(3.66628216680076,1.95498580453519,-2.41900961223909)) ;
#168122=CARTESIAN_POINT('Ctrl Pts',(3.65739884032377,1.94929644648107,-2.41475902421228)) ;
#168123=CARTESIAN_POINT('Ctrl Pts',(3.65126071410426,1.94574201114262,-2.41247113326881)) ;
#168124=CARTESIAN_POINT('Ctrl Pts',(3.64132315686417,1.94068746317945,-2.40963796590125)) ;
#168125=CARTESIAN_POINT('Ctrl Pts',(3.63763353946351,1.93894751340588,-2.40875659938477)) ;
#168126=CARTESIAN_POINT('Ctrl Pts',(3.62813871250319,1.93486114467728,-2.40690439135811)) ;
#168127=CARTESIAN_POINT('Ctrl Pts',(3.62220485293009,1.93266004719381,-2.40611534404151)) ;
#168128=CARTESIAN_POINT('Ctrl Pts',(3.6135954374234,1.9300316723429,-2.40542021745114)) ;
#168129=CARTESIAN_POINT('Ctrl Pts',(3.61101642177029,1.92931331154719,-2.40526698255319)) ;
#168130=CARTESIAN_POINT('Ctrl Pts',(3.60562851963663,1.92796119665949,-2.40505325677268)) ;
#168131=CARTESIAN_POINT('Ctrl Pts',(3.60282089026148,1.92733781012842,-2.405)) ;
#168132=CARTESIAN_POINT('Ctrl Pts',(3.6,1.92679491924311,-2.405)) ;
#168133=CARTESIAN_POINT('Origin',(3.6,1.9,-2.505)) ;
#168134=CARTESIAN_POINT('Origin',(3.7,1.9,-2.505)) ;
#168135=CARTESIAN_POINT('Origin',(10.1,1.9,-2.505)) ;
#168136=CARTESIAN_POINT('Origin',(10.1,1.9,-2.505)) ;
#168137=CARTESIAN_POINT('Origin',(3.7,2.1,-8.925)) ;
#168138=CARTESIAN_POINT('',(3.7,1.98660254037844,-8.975)) ;
#168139=CARTESIAN_POINT('Ctrl Pts',(3.60000000000001,1.92679491924311,-9.025)) ;
#168140=CARTESIAN_POINT('Ctrl Pts',(3.60642117639486,1.92803067521647,-9.025)) ;
#168141=CARTESIAN_POINT('Ctrl Pts',(3.61278477806504,1.92968896670924,-9.02472281361407)) ;
#168142=CARTESIAN_POINT('Ctrl Pts',(3.6189728323953,1.93170032347262,-9.02412352491366)) ;
#168143=CARTESIAN_POINT('Ctrl Pts',(3.62020584678443,1.93210110079269,-9.02400411232427)) ;
#168144=CARTESIAN_POINT('Ctrl Pts',(3.62143195421094,1.93251577262755,-9.02387200280826)) ;
#168145=CARTESIAN_POINT('Ctrl Pts',(3.62265032708637,1.93294361409314,-9.02372698243403)) ;
#168146=CARTESIAN_POINT('Ctrl Pts',(3.62647624625549,1.9342871164786,-9.02327159128008)) ;
#168147=CARTESIAN_POINT('Ctrl Pts',(3.63025346237246,1.93576539638805,-9.02268573681767)) ;
#168148=CARTESIAN_POINT('Ctrl Pts',(3.6339385638818,1.9373536406594,-9.02196503626974)) ;
#168149=CARTESIAN_POINT('Ctrl Pts',(3.63907793749079,1.93956866259898,-9.02095992165713)) ;
#168150=CARTESIAN_POINT('Ctrl Pts',(3.64410916187594,1.9420207691991,-9.01967872244964)) ;
#168151=CARTESIAN_POINT('Ctrl Pts',(3.6489431739508,1.94461872744765,-9.01812217773586)) ;
#168152=CARTESIAN_POINT('Ctrl Pts',(3.64993855309173,1.94515367717669,-9.01780166712976)) ;
#168153=CARTESIAN_POINT('Ctrl Pts',(3.65092568100081,1.94569474416709,-9.01746960315684)) ;
#168154=CARTESIAN_POINT('Ctrl Pts',(3.65190395907098,1.94624104404951,-9.01712618093671)) ;
#168155=CARTESIAN_POINT('Ctrl Pts',(3.65241342868353,1.94652554719634,-9.01694733282515)) ;
#168156=CARTESIAN_POINT('Ctrl Pts',(3.652920468175,1.94681147780209,-9.01676540573999)) ;
#168157=CARTESIAN_POINT('Ctrl Pts',(3.6534249821411,1.94709871486665,-9.01658043363331)) ;
#168158=CARTESIAN_POINT('Ctrl Pts',(3.65677402871197,1.94900544167845,-9.01535255840841)) ;
#168159=CARTESIAN_POINT('Ctrl Pts',(3.66003813592315,1.95098496635821,-9.01398063668092)) ;
#168160=CARTESIAN_POINT('Ctrl Pts',(3.66320312645637,1.95301617633166,-9.01246240139399)) ;
#168161=CARTESIAN_POINT('Ctrl Pts',(3.66757373088828,1.95582111846936,-9.01036583718502)) ;
#168162=CARTESIAN_POINT('Ctrl Pts',(3.67181875309405,1.95875330073093,-9.0079661261707)) ;
#168163=CARTESIAN_POINT('Ctrl Pts',(3.6758438861257,1.96174615985095,-9.00526003578539)) ;
#168164=CARTESIAN_POINT('Ctrl Pts',(3.67661208162813,1.96231734616885,-9.00474357919953)) ;
#168165=CARTESIAN_POINT('Ctrl Pts',(3.67737237849372,1.96289065080932,-9.00421601587659)) ;
#168166=CARTESIAN_POINT('Ctrl Pts',(3.6781242821475,1.96346549105988,-9.00367739883592)) ;
#168167=CARTESIAN_POINT('Ctrl Pts',(3.67853493948847,1.96377944400797,-9.00338322944253)) ;
#168168=CARTESIAN_POINT('Ctrl Pts',(3.67894301851532,1.96409388168817,-9.00308575174333)) ;
#168169=CARTESIAN_POINT('Ctrl Pts',(3.67934840022276,1.96440871854256,-9.00278496939812)) ;
#168170=CARTESIAN_POINT('Ctrl Pts',(3.68198440184425,1.96645595067819,-9.00082912695352)) ;
#168171=CARTESIAN_POINT('Ctrl Pts',(3.68449751351864,1.96851545671307,-8.99873828347164)) ;
#168172=CARTESIAN_POINT('Ctrl Pts',(3.68685379133723,1.97055696562013,-8.99652085039877)) ;
#168173=CARTESIAN_POINT('Ctrl Pts',(3.68896164651385,1.97238323800784,-8.99453720155032)) ;
#168174=CARTESIAN_POINT('Ctrl Pts',(3.69104797813205,1.97419718002547,-8.99244243877983)) ;
#168175=CARTESIAN_POINT('Ctrl Pts',(3.69290978292493,1.97598569412168,-8.9902450010323)) ;
#168176=CARTESIAN_POINT('Ctrl Pts',(3.69362192319645,1.97666980070416,-8.98940448116676)) ;
#168177=CARTESIAN_POINT('Ctrl Pts',(3.69430163271861,1.97734979318971,-8.98854897561523)) ;
#168178=CARTESIAN_POINT('Ctrl Pts',(3.69493905694205,1.97802369895108,-8.98767908836304)) ;
#168179=CARTESIAN_POINT('Ctrl Pts',(3.69605143900784,1.9791997456958,-8.98616103030527)) ;
#168180=CARTESIAN_POINT('Ctrl Pts',(3.69703421735413,1.98035885502255,-8.9845986233173)) ;
#168181=CARTESIAN_POINT('Ctrl Pts',(3.6978475066491,1.98151165953424,-8.98295719153115)) ;
#168182=CARTESIAN_POINT('Ctrl Pts',(3.69841279947843,1.98231293913807,-8.98181628186435)) ;
#168183=CARTESIAN_POINT('Ctrl Pts',(3.69890310384954,1.98311438470598,-8.98063324801215)) ;
#168184=CARTESIAN_POINT('Ctrl Pts',(3.69929098301995,1.98393783265455,-8.97935810707461)) ;
#168185=CARTESIAN_POINT('Ctrl Pts',(3.69936193271525,1.98408845528529,-8.97912486211613)) ;
#168186=CARTESIAN_POINT('Ctrl Pts',(3.69942931950317,1.98423979370565,-8.97888851468592)) ;
#168187=CARTESIAN_POINT('Ctrl Pts',(3.69949277412724,1.98439195189923,-8.97864873028525)) ;
#168188=CARTESIAN_POINT('Ctrl Pts',(3.69967702385849,1.98483376534754,-8.97795248139834)) ;
#168189=CARTESIAN_POINT('Ctrl Pts',(3.69981936684304,1.98527475083258,-8.97723933425854)) ;
#168190=CARTESIAN_POINT('Ctrl Pts',(3.69990669142683,1.98570953653121,-8.97651584102814)) ;
#168191=CARTESIAN_POINT('Ctrl Pts',(3.69996666908332,1.98600816294479,-8.97601891992581)) ;
#168192=CARTESIAN_POINT('Ctrl Pts',(3.7,1.98630780592129,-8.97551049505454)) ;
#168193=CARTESIAN_POINT('Ctrl Pts',(3.7,1.98660254037844,-8.975)) ;
#168194=CARTESIAN_POINT('Origin',(3.7,1.9,-8.925)) ;
#168195=CARTESIAN_POINT('Origin',(10.2,1.9,-8.925)) ;
#168196=CARTESIAN_POINT('Origin',(3.7,1.9,-8.925)) ;
#168197=CARTESIAN_POINT('Origin',(10.1,1.9,-8.925)) ;
#168198=CARTESIAN_POINT('Origin',(10.1,1.9,-8.925)) ;
#168199=CARTESIAN_POINT('Origin',(3.7,2.1,-6.315)) ;
#168200=CARTESIAN_POINT('',(3.7,1.98660254037844,-6.265)) ;
#168201=CARTESIAN_POINT('Origin',(3.7,1.9,-6.315)) ;
#168202=CARTESIAN_POINT('Ctrl Pts',(3.7,1.98660254037844,-6.265)) ;
#168203=CARTESIAN_POINT('Ctrl Pts',(3.69999911718144,1.98567700534183,-6.26339692629239)) ;
#168204=CARTESIAN_POINT('Ctrl Pts',(3.69968163901485,1.984703699336,-6.26181800228456)) ;
#168205=CARTESIAN_POINT('Ctrl Pts',(3.69895427931586,1.98325895404995,-6.25959445604082)) ;
#168206=CARTESIAN_POINT('Ctrl Pts',(3.69867650892745,1.98278649590681,-6.25888609842392)) ;
#168207=CARTESIAN_POINT('Ctrl Pts',(3.69717970712967,1.9804354328423,-6.25544091878433)) ;
#168208=CARTESIAN_POINT('Ctrl Pts',(3.69541014605544,1.97847095301992,-6.25282412084426)) ;
#168209=CARTESIAN_POINT('Ctrl Pts',(3.69146029518774,1.97457001268155,-6.24797344350903)) ;
#168210=CARTESIAN_POINT('Ctrl Pts',(3.68915436790411,1.97254004967205,-6.24563220687652)) ;
#168211=CARTESIAN_POINT('Ctrl Pts',(3.6826362316179,1.96688850447178,-6.23949991845675)) ;
#168212=CARTESIAN_POINT('Ctrl Pts',(3.67796661383154,1.96321337091309,-6.23597925228304)) ;
#168213=CARTESIAN_POINT('Ctrl Pts',(3.67279117399673,1.95950210067473,-6.23276234339452)) ;
#168214=CARTESIAN_POINT('Ctrl Pts',(3.67252519027992,1.95931231248681,-6.23259880905815)) ;
#168215=CARTESIAN_POINT('Ctrl Pts',(3.6693311210617,1.95704457126181,-6.23065620430679)) ;
#168216=CARTESIAN_POINT('Ctrl Pts',(3.66628216680076,1.95498580453519,-6.22900961223909)) ;
#168217=CARTESIAN_POINT('Ctrl Pts',(3.65739884032377,1.94929644648107,-6.22475902421228)) ;
#168218=CARTESIAN_POINT('Ctrl Pts',(3.65126071410426,1.94574201114262,-6.22247113326881)) ;
#168219=CARTESIAN_POINT('Ctrl Pts',(3.64132315686417,1.94068746317945,-6.21963796590125)) ;
#168220=CARTESIAN_POINT('Ctrl Pts',(3.63763353946351,1.93894751340588,-6.21875659938478)) ;
#168221=CARTESIAN_POINT('Ctrl Pts',(3.62813871250319,1.93486114467728,-6.21690439135811)) ;
#168222=CARTESIAN_POINT('Ctrl Pts',(3.62220485293009,1.93266004719381,-6.21611534404151)) ;
#168223=CARTESIAN_POINT('Ctrl Pts',(3.61359543742331,1.93003167234287,-6.21542021745113)) ;
#168224=CARTESIAN_POINT('Ctrl Pts',(3.61101642177012,1.92931331154715,-6.21526698255318)) ;
#168225=CARTESIAN_POINT('Ctrl Pts',(3.60562851963646,1.92796119665945,-6.21505325677268)) ;
#168226=CARTESIAN_POINT('Ctrl Pts',(3.60282089026139,1.92733781012841,-6.215)) ;
#168227=CARTESIAN_POINT('Ctrl Pts',(3.6,1.92679491924311,-6.215)) ;
#168228=CARTESIAN_POINT('Origin',(3.6,1.9,-6.315)) ;
#168229=CARTESIAN_POINT('Origin',(3.7,1.9,-6.315)) ;
#168230=CARTESIAN_POINT('Origin',(10.1,1.9,-6.315)) ;
#168231=CARTESIAN_POINT('Origin',(10.1,1.9,-6.315)) ;
#168232=CARTESIAN_POINT('Origin',(3.7,2.1,-12.735)) ;
#168233=CARTESIAN_POINT('',(3.7,1.98660254037844,-12.785)) ;
#168234=CARTESIAN_POINT('Ctrl Pts',(3.60000000000001,1.92679491924311,-12.835)) ;
#168235=CARTESIAN_POINT('Ctrl Pts',(3.60642117639459,1.92803067521642,-12.835)) ;
#168236=CARTESIAN_POINT('Ctrl Pts',(3.61278477806451,1.92968896670911,-12.8347228136141)) ;
#168237=CARTESIAN_POINT('Ctrl Pts',(3.61897283239452,1.93170032347238,-12.8341235249137)) ;
#168238=CARTESIAN_POINT('Ctrl Pts',(3.62020584678391,1.93210110079252,-12.8340041123243)) ;
#168239=CARTESIAN_POINT('Ctrl Pts',(3.62143195421068,1.93251577262747,-12.8338720028083)) ;
#168240=CARTESIAN_POINT('Ctrl Pts',(3.62265032708637,1.93294361409315,-12.833726982434)) ;
#168241=CARTESIAN_POINT('Ctrl Pts',(3.62647624625549,1.9342871164786,-12.8332715912801)) ;
#168242=CARTESIAN_POINT('Ctrl Pts',(3.63025346237246,1.93576539638805,-12.8326857368177)) ;
#168243=CARTESIAN_POINT('Ctrl Pts',(3.6339385638818,1.93735364065939,-12.8319650362697)) ;
#168244=CARTESIAN_POINT('Ctrl Pts',(3.63907793749009,1.93956866259867,-12.8309599216573)) ;
#168245=CARTESIAN_POINT('Ctrl Pts',(3.64410916187458,1.94202076919845,-12.82967872245)) ;
#168246=CARTESIAN_POINT('Ctrl Pts',(3.64894317394883,1.94461872744659,-12.8281221777365)) ;
#168247=CARTESIAN_POINT('Ctrl Pts',(3.64993855309046,1.94515367717599,-12.8278016671302)) ;
#168248=CARTESIAN_POINT('Ctrl Pts',(3.65092568100022,1.94569474416675,-12.8274696031571)) ;
#168249=CARTESIAN_POINT('Ctrl Pts',(3.65190395907107,1.94624104404954,-12.8271261809367)) ;
#168250=CARTESIAN_POINT('Ctrl Pts',(3.65241342868358,1.94652554719635,-12.8269473328251)) ;
#168251=CARTESIAN_POINT('Ctrl Pts',(3.65292046817503,1.94681147780212,-12.82676540574)) ;
#168252=CARTESIAN_POINT('Ctrl Pts',(3.65342498214111,1.94709871486667,-12.8265804336333)) ;
#168253=CARTESIAN_POINT('Ctrl Pts',(3.65677402871197,1.94900544167846,-12.8253525584084)) ;
#168254=CARTESIAN_POINT('Ctrl Pts',(3.66003813592314,1.95098496635819,-12.8239806366809)) ;
#168255=CARTESIAN_POINT('Ctrl Pts',(3.66320312645637,1.95301617633164,-12.822462401394)) ;
#168256=CARTESIAN_POINT('Ctrl Pts',(3.6675737308879,1.9558211184691,-12.8203658371852)) ;
#168257=CARTESIAN_POINT('Ctrl Pts',(3.67181875309331,1.95875330073043,-12.8179661261711)) ;
#168258=CARTESIAN_POINT('Ctrl Pts',(3.67584388612464,1.96174615985015,-12.8152600357861)) ;
#168259=CARTESIAN_POINT('Ctrl Pts',(3.67661208162745,1.96231734616832,-12.8147435792)) ;
#168260=CARTESIAN_POINT('Ctrl Pts',(3.67737237849342,1.96289065080907,-12.8142160158768)) ;
#168261=CARTESIAN_POINT('Ctrl Pts',(3.67812428214757,1.96346549105991,-12.8136773988359)) ;
#168262=CARTESIAN_POINT('Ctrl Pts',(3.67853493948852,1.96377944400797,-12.8133832294425)) ;
#168263=CARTESIAN_POINT('Ctrl Pts',(3.67894301851535,1.96409388168821,-12.8130857517433)) ;
#168264=CARTESIAN_POINT('Ctrl Pts',(3.67934840022277,1.96440871854258,-12.8127849693981)) ;
#168265=CARTESIAN_POINT('Ctrl Pts',(3.68198440184426,1.96645595067818,-12.8108291269535)) ;
#168266=CARTESIAN_POINT('Ctrl Pts',(3.68449751351864,1.96851545671311,-12.8087382834716)) ;
#168267=CARTESIAN_POINT('Ctrl Pts',(3.68685379133723,1.97055696562016,-12.8065208503987)) ;
#168268=CARTESIAN_POINT('Ctrl Pts',(3.68896164651378,1.97238323800782,-12.8045372015504)) ;
#168269=CARTESIAN_POINT('Ctrl Pts',(3.69104797813192,1.97419718002535,-12.80244243878)) ;
#168270=CARTESIAN_POINT('Ctrl Pts',(3.69290978292475,1.9759856941215,-12.8002450010325)) ;
#168271=CARTESIAN_POINT('Ctrl Pts',(3.69362192319634,1.97666980070403,-12.7994044811669)) ;
#168272=CARTESIAN_POINT('Ctrl Pts',(3.69430163271856,1.97734979318964,-12.7985489756153)) ;
#168273=CARTESIAN_POINT('Ctrl Pts',(3.69493905694205,1.97802369895107,-12.797679088363)) ;
#168274=CARTESIAN_POINT('Ctrl Pts',(3.69605143900784,1.9791997456958,-12.7961610303053)) ;
#168275=CARTESIAN_POINT('Ctrl Pts',(3.69703421735413,1.98035885502254,-12.7945986233173)) ;
#168276=CARTESIAN_POINT('Ctrl Pts',(3.6978475066491,1.98151165953422,-12.7929571915312)) ;
#168277=CARTESIAN_POINT('Ctrl Pts',(3.69841279947841,1.98231293913801,-12.7918162818644)) ;
#168278=CARTESIAN_POINT('Ctrl Pts',(3.69890310384951,1.98311438470592,-12.7906332480122)) ;
#168279=CARTESIAN_POINT('Ctrl Pts',(3.6992909830199,1.98393783265445,-12.7893581070748)) ;
#168280=CARTESIAN_POINT('Ctrl Pts',(3.69936193271523,1.98408845528522,-12.7891248621162)) ;
#168281=CARTESIAN_POINT('Ctrl Pts',(3.69942931950317,1.98423979370565,-12.7888885146859)) ;
#168282=CARTESIAN_POINT('Ctrl Pts',(3.69949277412725,1.98439195189925,-12.7886487302852)) ;
#168283=CARTESIAN_POINT('Ctrl Pts',(3.69967702385849,1.98483376534754,-12.7879524813983)) ;
#168284=CARTESIAN_POINT('Ctrl Pts',(3.69981936684304,1.98527475083261,-12.7872393342585)) ;
#168285=CARTESIAN_POINT('Ctrl Pts',(3.69990669142683,1.98570953653124,-12.7865158410281)) ;
#168286=CARTESIAN_POINT('Ctrl Pts',(3.69996666908332,1.98600816294482,-12.7860189199258)) ;
#168287=CARTESIAN_POINT('Ctrl Pts',(3.7,1.9863078059213,-12.7855104950545)) ;
#168288=CARTESIAN_POINT('Ctrl Pts',(3.7,1.98660254037844,-12.785)) ;
#168289=CARTESIAN_POINT('Origin',(3.7,1.9,-12.735)) ;
#168290=CARTESIAN_POINT('Origin',(10.2,1.9,-12.735)) ;
#168291=CARTESIAN_POINT('Origin',(3.7,1.9,-12.735)) ;
#168292=CARTESIAN_POINT('Origin',(10.1,1.9,-12.735)) ;
#168293=CARTESIAN_POINT('Origin',(10.1,1.9,-12.735)) ;
#168294=CARTESIAN_POINT('Origin',(3.7,2.1,-10.125)) ;
#168295=CARTESIAN_POINT('',(3.7,1.98660254037844,-10.075)) ;
#168296=CARTESIAN_POINT('Origin',(3.7,1.9,-10.125)) ;
#168297=CARTESIAN_POINT('Ctrl Pts',(3.7,1.98660254037844,-10.075)) ;
#168298=CARTESIAN_POINT('Ctrl Pts',(3.69999911718144,1.98567700534183,-10.0733969262924)) ;
#168299=CARTESIAN_POINT('Ctrl Pts',(3.69968163901485,1.98470369933601,-10.0718180022846)) ;
#168300=CARTESIAN_POINT('Ctrl Pts',(3.69895427931586,1.98325895404995,-10.0695944560408)) ;
#168301=CARTESIAN_POINT('Ctrl Pts',(3.69867650892745,1.98278649590681,-10.0688860984239)) ;
#168302=CARTESIAN_POINT('Ctrl Pts',(3.69717970712967,1.9804354328423,-10.0654409187843)) ;
#168303=CARTESIAN_POINT('Ctrl Pts',(3.69541014605544,1.97847095301992,-10.0628241208443)) ;
#168304=CARTESIAN_POINT('Ctrl Pts',(3.69146029518774,1.97457001268155,-10.057973443509)) ;
#168305=CARTESIAN_POINT('Ctrl Pts',(3.68915436790411,1.97254004967205,-10.0556322068765)) ;
#168306=CARTESIAN_POINT('Ctrl Pts',(3.68263623161784,1.96688850447173,-10.0494999184567)) ;
#168307=CARTESIAN_POINT('Ctrl Pts',(3.67796661383141,1.96321337091298,-10.0459792522829)) ;
#168308=CARTESIAN_POINT('Ctrl Pts',(3.67279117399659,1.95950210067463,-10.0427623433944)) ;
#168309=CARTESIAN_POINT('Ctrl Pts',(3.67252519027985,1.95931231248676,-10.0425988090581)) ;
#168310=CARTESIAN_POINT('Ctrl Pts',(3.6693311210617,1.95704457126181,-10.0406562043068)) ;
#168311=CARTESIAN_POINT('Ctrl Pts',(3.66628216680076,1.95498580453519,-10.0390096122391)) ;
#168312=CARTESIAN_POINT('Ctrl Pts',(3.65739884032376,1.94929644648107,-10.0347590242123)) ;
#168313=CARTESIAN_POINT('Ctrl Pts',(3.65126071410427,1.94574201114262,-10.0324711332688)) ;
#168314=CARTESIAN_POINT('Ctrl Pts',(3.64132315686418,1.94068746317945,-10.0296379659012)) ;
#168315=CARTESIAN_POINT('Ctrl Pts',(3.63763353946351,1.93894751340588,-10.0287565993848)) ;
#168316=CARTESIAN_POINT('Ctrl Pts',(3.62813871250319,1.93486114467728,-10.0269043913581)) ;
#168317=CARTESIAN_POINT('Ctrl Pts',(3.62220485293008,1.9326600471938,-10.0261153440415)) ;
#168318=CARTESIAN_POINT('Ctrl Pts',(3.61359543742328,1.93003167234287,-10.0254202174511)) ;
#168319=CARTESIAN_POINT('Ctrl Pts',(3.61101642177007,1.92931331154713,-10.0252669825532)) ;
#168320=CARTESIAN_POINT('Ctrl Pts',(3.60562851963641,1.92796119665944,-10.0250532567727)) ;
#168321=CARTESIAN_POINT('Ctrl Pts',(3.60282089026137,1.92733781012841,-10.025)) ;
#168322=CARTESIAN_POINT('Ctrl Pts',(3.6,1.92679491924311,-10.025)) ;
#168323=CARTESIAN_POINT('Origin',(3.6,1.9,-10.125)) ;
#168324=CARTESIAN_POINT('Origin',(3.7,1.9,-10.125)) ;
#168325=CARTESIAN_POINT('Origin',(10.1,1.9,-10.125)) ;
#168326=CARTESIAN_POINT('Origin',(10.1,1.9,-10.125)) ;
#168327=CARTESIAN_POINT('Origin',(3.7,2.1,-16.545)) ;
#168328=CARTESIAN_POINT('',(3.7,1.98660254037845,-16.595)) ;
#168329=CARTESIAN_POINT('Ctrl Pts',(3.60000000000001,1.92679491924311,-16.645)) ;
#168330=CARTESIAN_POINT('Ctrl Pts',(3.60642117639496,1.92803067521649,-16.645)) ;
#168331=CARTESIAN_POINT('Ctrl Pts',(3.61278477806524,1.92968896670929,-16.6447228136141)) ;
#168332=CARTESIAN_POINT('Ctrl Pts',(3.61897283239559,1.93170032347272,-16.6441235249136)) ;
#168333=CARTESIAN_POINT('Ctrl Pts',(3.62020584678462,1.93210110079276,-16.6440041123243)) ;
#168334=CARTESIAN_POINT('Ctrl Pts',(3.62143195421103,1.93251577262759,-16.6438720028083)) ;
#168335=CARTESIAN_POINT('Ctrl Pts',(3.62265032708637,1.93294361409314,-16.643726982434)) ;
#168336=CARTESIAN_POINT('Ctrl Pts',(3.62647624625549,1.9342871164786,-16.6432715912801)) ;
#168337=CARTESIAN_POINT('Ctrl Pts',(3.63025346237246,1.93576539638807,-16.6426857368177)) ;
#168338=CARTESIAN_POINT('Ctrl Pts',(3.6339385638818,1.9373536406594,-16.6419650362697)) ;
#168339=CARTESIAN_POINT('Ctrl Pts',(3.6390779374911,1.93956866259911,-16.6409599216571)) ;
#168340=CARTESIAN_POINT('Ctrl Pts',(3.64410916187654,1.94202076919938,-16.6396787224495)) ;
#168341=CARTESIAN_POINT('Ctrl Pts',(3.64894317395167,1.94461872744812,-16.6381221777356)) ;
#168342=CARTESIAN_POINT('Ctrl Pts',(3.64993855309228,1.945153677177,-16.6378016671296)) ;
#168343=CARTESIAN_POINT('Ctrl Pts',(3.65092568100105,1.94569474416723,-16.6374696031568)) ;
#168344=CARTESIAN_POINT('Ctrl Pts',(3.65190395907092,1.94624104404949,-16.6371261809367)) ;
#168345=CARTESIAN_POINT('Ctrl Pts',(3.65241342868349,1.94652554719633,-16.6369473328252)) ;
#168346=CARTESIAN_POINT('Ctrl Pts',(3.65292046817498,1.94681147780208,-16.63676540574)) ;
#168347=CARTESIAN_POINT('Ctrl Pts',(3.6534249821411,1.94709871486665,-16.6365804336333)) ;
#168348=CARTESIAN_POINT('Ctrl Pts',(3.65677402871197,1.94900544167846,-16.6353525584084)) ;
#168349=CARTESIAN_POINT('Ctrl Pts',(3.66003813592314,1.95098496635819,-16.6339806366809)) ;
#168350=CARTESIAN_POINT('Ctrl Pts',(3.66320312645638,1.95301617633166,-16.632462401394)) ;
#168351=CARTESIAN_POINT('Ctrl Pts',(3.66757373088829,1.95582111846938,-16.630365837185)) ;
#168352=CARTESIAN_POINT('Ctrl Pts',(3.67181875309404,1.95875330073095,-16.6279661261707)) ;
#168353=CARTESIAN_POINT('Ctrl Pts',(3.67584388612568,1.96174615985092,-16.6252600357854)) ;
#168354=CARTESIAN_POINT('Ctrl Pts',(3.67661208162821,1.96231734616889,-16.6247435791995)) ;
#168355=CARTESIAN_POINT('Ctrl Pts',(3.6773723784939,1.96289065080943,-16.6242160158765)) ;
#168356=CARTESIAN_POINT('Ctrl Pts',(3.67812428214779,1.96346549106007,-16.6236773988357)) ;
#168357=CARTESIAN_POINT('Ctrl Pts',(3.67853493948866,1.96377944400807,-16.6233832294424)) ;
#168358=CARTESIAN_POINT('Ctrl Pts',(3.67894301851542,1.96409388168823,-16.6230857517433)) ;
#168359=CARTESIAN_POINT('Ctrl Pts',(3.67934840022277,1.96440871854255,-16.6227849693981)) ;
#168360=CARTESIAN_POINT('Ctrl Pts',(3.68198440184425,1.96645595067818,-16.6208291269535)) ;
#168361=CARTESIAN_POINT('Ctrl Pts',(3.68449751351864,1.96851545671311,-16.6187382834716)) ;
#168362=CARTESIAN_POINT('Ctrl Pts',(3.68685379133723,1.97055696562017,-16.6165208503987)) ;
#168363=CARTESIAN_POINT('Ctrl Pts',(3.68896164651388,1.9723832380079,-16.6145372015503)) ;
#168364=CARTESIAN_POINT('Ctrl Pts',(3.6910479781321,1.97419718002554,-16.6124424387798)) ;
#168365=CARTESIAN_POINT('Ctrl Pts',(3.69290978292499,1.97598569412176,-16.6102450010322)) ;
#168366=CARTESIAN_POINT('Ctrl Pts',(3.6936219231965,1.97666980070422,-16.6094044811667)) ;
#168367=CARTESIAN_POINT('Ctrl Pts',(3.69430163271864,1.97734979318976,-16.6085489756152)) ;
#168368=CARTESIAN_POINT('Ctrl Pts',(3.69493905694207,1.9780236989511,-16.607679088363)) ;
#168369=CARTESIAN_POINT('Ctrl Pts',(3.69605143900786,1.9791997456958,-16.6061610303053)) ;
#168370=CARTESIAN_POINT('Ctrl Pts',(3.69703421735413,1.98035885502256,-16.6045986233173)) ;
#168371=CARTESIAN_POINT('Ctrl Pts',(3.6978475066491,1.98151165953425,-16.6029571915311)) ;
#168372=CARTESIAN_POINT('Ctrl Pts',(3.69841279947847,1.98231293913814,-16.6018162818643)) ;
#168373=CARTESIAN_POINT('Ctrl Pts',(3.6989031038496,1.98311438470612,-16.6006332480119)) ;
#168374=CARTESIAN_POINT('Ctrl Pts',(3.69929098302002,1.98393783265472,-16.5993581070744)) ;
#168375=CARTESIAN_POINT('Ctrl Pts',(3.6993619327153,1.98408845528541,-16.5991248621159)) ;
#168376=CARTESIAN_POINT('Ctrl Pts',(3.69942931950321,1.98423979370578,-16.5988885146857)) ;
#168377=CARTESIAN_POINT('Ctrl Pts',(3.69949277412727,1.98439195189931,-16.5986487302851)) ;
#168378=CARTESIAN_POINT('Ctrl Pts',(3.6996770238585,1.98483376534759,-16.5979524813983)) ;
#168379=CARTESIAN_POINT('Ctrl Pts',(3.69981936684305,1.98527475083261,-16.5972393342585)) ;
#168380=CARTESIAN_POINT('Ctrl Pts',(3.69990669142684,1.9857095365312,-16.5965158410282)) ;
#168381=CARTESIAN_POINT('Ctrl Pts',(3.69996666908332,1.98600816294476,-16.5960189199259)) ;
#168382=CARTESIAN_POINT('Ctrl Pts',(3.7,1.9863078059213,-16.5955104950545)) ;
#168383=CARTESIAN_POINT('Ctrl Pts',(3.7,1.98660254037844,-16.595)) ;
#168384=CARTESIAN_POINT('Origin',(3.7,1.9,-16.545)) ;
#168385=CARTESIAN_POINT('Origin',(10.2,1.9,-16.545)) ;
#168386=CARTESIAN_POINT('Origin',(3.7,1.9,-16.545)) ;
#168387=CARTESIAN_POINT('Origin',(10.1,1.9,-16.545)) ;
#168388=CARTESIAN_POINT('Origin',(10.1,1.9,-16.545)) ;
#168389=CARTESIAN_POINT('Origin',(3.7,2.1,-13.935)) ;
#168390=CARTESIAN_POINT('',(3.7,1.98660254037844,-13.885)) ;
#168391=CARTESIAN_POINT('Origin',(3.7,1.9,-13.935)) ;
#168392=CARTESIAN_POINT('Ctrl Pts',(3.7,1.98660254037844,-13.885)) ;
#168393=CARTESIAN_POINT('Ctrl Pts',(3.69999911718144,1.98567700534183,-13.8833969262924)) ;
#168394=CARTESIAN_POINT('Ctrl Pts',(3.69968163901485,1.984703699336,-13.8818180022846)) ;
#168395=CARTESIAN_POINT('Ctrl Pts',(3.69895427931585,1.98325895404995,-13.8795944560408)) ;
#168396=CARTESIAN_POINT('Ctrl Pts',(3.69867650892745,1.98278649590681,-13.8788860984239)) ;
#168397=CARTESIAN_POINT('Ctrl Pts',(3.69717970712967,1.9804354328423,-13.8754409187843)) ;
#168398=CARTESIAN_POINT('Ctrl Pts',(3.69541014605544,1.97847095301992,-13.8728241208443)) ;
#168399=CARTESIAN_POINT('Ctrl Pts',(3.69146029518774,1.97457001268155,-13.867973443509)) ;
#168400=CARTESIAN_POINT('Ctrl Pts',(3.68915436790411,1.97254004967205,-13.8656322068765)) ;
#168401=CARTESIAN_POINT('Ctrl Pts',(3.68263623161783,1.96688850447172,-13.8594999184567)) ;
#168402=CARTESIAN_POINT('Ctrl Pts',(3.67796661383139,1.96321337091296,-13.8559792522829)) ;
#168403=CARTESIAN_POINT('Ctrl Pts',(3.67279117399656,1.95950210067461,-13.8527623433944)) ;
#168404=CARTESIAN_POINT('Ctrl Pts',(3.67252519027983,1.95931231248676,-13.8525988090581)) ;
#168405=CARTESIAN_POINT('Ctrl Pts',(3.6693311210617,1.95704457126181,-13.8506562043068)) ;
#168406=CARTESIAN_POINT('Ctrl Pts',(3.66628216680076,1.95498580453519,-13.8490096122391)) ;
#168407=CARTESIAN_POINT('Ctrl Pts',(3.65739884032376,1.94929644648107,-13.8447590242123)) ;
#168408=CARTESIAN_POINT('Ctrl Pts',(3.65126071410427,1.94574201114262,-13.8424711332688)) ;
#168409=CARTESIAN_POINT('Ctrl Pts',(3.64132315686417,1.94068746317945,-13.8396379659013)) ;
#168410=CARTESIAN_POINT('Ctrl Pts',(3.63763353946351,1.93894751340588,-13.8387565993848)) ;
#168411=CARTESIAN_POINT('Ctrl Pts',(3.62813871250318,1.93486114467727,-13.8369043913581)) ;
#168412=CARTESIAN_POINT('Ctrl Pts',(3.62220485293007,1.9326600471938,-13.8361153440415)) ;
#168413=CARTESIAN_POINT('Ctrl Pts',(3.61359543742316,1.93003167234283,-13.8354202174511)) ;
#168414=CARTESIAN_POINT('Ctrl Pts',(3.61101642176982,1.92931331154706,-13.8352669825532)) ;
#168415=CARTESIAN_POINT('Ctrl Pts',(3.60562851963616,1.92796119665938,-13.8350532567727)) ;
#168416=CARTESIAN_POINT('Ctrl Pts',(3.60282089026124,1.92733781012838,-13.835)) ;
#168417=CARTESIAN_POINT('Ctrl Pts',(3.6,1.92679491924311,-13.835)) ;
#168418=CARTESIAN_POINT('Origin',(3.6,1.9,-13.935)) ;
#168419=CARTESIAN_POINT('Origin',(3.7,1.9,-13.935)) ;
#168420=CARTESIAN_POINT('Origin',(10.1,1.9,-13.935)) ;
#168421=CARTESIAN_POINT('Origin',(10.1,1.9,-13.935)) ;
#168422=CARTESIAN_POINT('Origin',(3.7,2.1,-20.355)) ;
#168423=CARTESIAN_POINT('',(3.7,1.98660254037845,-20.405)) ;
#168424=CARTESIAN_POINT('Ctrl Pts',(3.60000000000001,1.92679491924311,-20.455)) ;
#168425=CARTESIAN_POINT('Ctrl Pts',(3.60642117639513,1.92803067521652,-20.455)) ;
#168426=CARTESIAN_POINT('Ctrl Pts',(3.61278477806557,1.92968896670937,-20.4547228136141)) ;
#168427=CARTESIAN_POINT('Ctrl Pts',(3.61897283239609,1.93170032347287,-20.4541235249136)) ;
#168428=CARTESIAN_POINT('Ctrl Pts',(3.62020584678495,1.93210110079286,-20.4540041123242)) ;
#168429=CARTESIAN_POINT('Ctrl Pts',(3.62143195421119,1.93251577262764,-20.4538720028082)) ;
#168430=CARTESIAN_POINT('Ctrl Pts',(3.62265032708637,1.93294361409314,-20.453726982434)) ;
#168431=CARTESIAN_POINT('Ctrl Pts',(3.62647624625549,1.9342871164786,-20.4532715912801)) ;
#168432=CARTESIAN_POINT('Ctrl Pts',(3.63025346237246,1.93576539638807,-20.4526857368177)) ;
#168433=CARTESIAN_POINT('Ctrl Pts',(3.6339385638818,1.9373536406594,-20.4519650362697)) ;
#168434=CARTESIAN_POINT('Ctrl Pts',(3.63907793749117,1.93956866259914,-20.4509599216571)) ;
#168435=CARTESIAN_POINT('Ctrl Pts',(3.64410916187667,1.94202076919945,-20.4496787224495)) ;
#168436=CARTESIAN_POINT('Ctrl Pts',(3.64894317395187,1.94461872744823,-20.4481221777355)) ;
#168437=CARTESIAN_POINT('Ctrl Pts',(3.64993855309242,1.94515367717707,-20.4478016671295)) ;
#168438=CARTESIAN_POINT('Ctrl Pts',(3.65092568100113,1.94569474416727,-20.4474696031567)) ;
#168439=CARTESIAN_POINT('Ctrl Pts',(3.65190395907093,1.94624104404949,-20.4471261809367)) ;
#168440=CARTESIAN_POINT('Ctrl Pts',(3.6524134286835,1.94652554719633,-20.4469473328252)) ;
#168441=CARTESIAN_POINT('Ctrl Pts',(3.65292046817498,1.94681147780208,-20.44676540574)) ;
#168442=CARTESIAN_POINT('Ctrl Pts',(3.6534249821411,1.94709871486665,-20.4465804336333)) ;
#168443=CARTESIAN_POINT('Ctrl Pts',(3.65677402871197,1.94900544167847,-20.4453525584084)) ;
#168444=CARTESIAN_POINT('Ctrl Pts',(3.66003813592314,1.9509849663582,-20.4439806366809)) ;
#168445=CARTESIAN_POINT('Ctrl Pts',(3.66320312645638,1.95301617633166,-20.442462401394)) ;
#168446=CARTESIAN_POINT('Ctrl Pts',(3.66757373088817,1.9558211184693,-20.4403658371851)) ;
#168447=CARTESIAN_POINT('Ctrl Pts',(3.67181875309382,1.9587533007308,-20.4379661261708)) ;
#168448=CARTESIAN_POINT('Ctrl Pts',(3.67584388612536,1.96174615985069,-20.4352600357856)) ;
#168449=CARTESIAN_POINT('Ctrl Pts',(3.676612081628,1.96231734616874,-20.4347435791996)) ;
#168450=CARTESIAN_POINT('Ctrl Pts',(3.67737237849379,1.96289065080935,-20.4342160158766)) ;
#168451=CARTESIAN_POINT('Ctrl Pts',(3.67812428214777,1.96346549106006,-20.4336773988358)) ;
#168452=CARTESIAN_POINT('Ctrl Pts',(3.67853493948865,1.96377944400807,-20.4333832294424)) ;
#168453=CARTESIAN_POINT('Ctrl Pts',(3.67894301851541,1.96409388168823,-20.4330857517433)) ;
#168454=CARTESIAN_POINT('Ctrl Pts',(3.67934840022277,1.96440871854255,-20.4327849693981)) ;
#168455=CARTESIAN_POINT('Ctrl Pts',(3.68198440184425,1.96645595067818,-20.4308291269535)) ;
#168456=CARTESIAN_POINT('Ctrl Pts',(3.68449751351864,1.96851545671311,-20.4287382834716)) ;
#168457=CARTESIAN_POINT('Ctrl Pts',(3.68685379133723,1.97055696562016,-20.4265208503987)) ;
#168458=CARTESIAN_POINT('Ctrl Pts',(3.68896164651387,1.97238323800789,-20.4245372015503)) ;
#168459=CARTESIAN_POINT('Ctrl Pts',(3.69104797813208,1.97419718002552,-20.4224424387798)) ;
#168460=CARTESIAN_POINT('Ctrl Pts',(3.69290978292497,1.97598569412173,-20.4202450010322)) ;
#168461=CARTESIAN_POINT('Ctrl Pts',(3.69362192319649,1.97666980070421,-20.4194044811667)) ;
#168462=CARTESIAN_POINT('Ctrl Pts',(3.69430163271864,1.97734979318975,-20.4185489756152)) ;
#168463=CARTESIAN_POINT('Ctrl Pts',(3.69493905694207,1.9780236989511,-20.417679088363)) ;
#168464=CARTESIAN_POINT('Ctrl Pts',(3.69605143900786,1.9791997456958,-20.4161610303053)) ;
#168465=CARTESIAN_POINT('Ctrl Pts',(3.69703421735413,1.98035885502256,-20.4145986233173)) ;
#168466=CARTESIAN_POINT('Ctrl Pts',(3.69784750664911,1.98151165953425,-20.4129571915311)) ;
#168467=CARTESIAN_POINT('Ctrl Pts',(3.69841279947848,1.98231293913814,-20.4118162818643)) ;
#168468=CARTESIAN_POINT('Ctrl Pts',(3.69890310384961,1.98311438470612,-20.4106332480119)) ;
#168469=CARTESIAN_POINT('Ctrl Pts',(3.69929098302003,1.98393783265478,-20.4093581070743)) ;
#168470=CARTESIAN_POINT('Ctrl Pts',(3.69936193271531,1.98408845528547,-20.4091248621159)) ;
#168471=CARTESIAN_POINT('Ctrl Pts',(3.69942931950321,1.98423979370578,-20.4088885146857)) ;
#168472=CARTESIAN_POINT('Ctrl Pts',(3.69949277412726,1.9843919518993,-20.4086487302851)) ;
#168473=CARTESIAN_POINT('Ctrl Pts',(3.6996770238585,1.98483376534759,-20.4079524813983)) ;
#168474=CARTESIAN_POINT('Ctrl Pts',(3.69981936684305,1.98527475083261,-20.4072393342585)) ;
#168475=CARTESIAN_POINT('Ctrl Pts',(3.69990669142684,1.9857095365312,-20.4065158410282)) ;
#168476=CARTESIAN_POINT('Ctrl Pts',(3.69996666908332,1.98600816294476,-20.4060189199259)) ;
#168477=CARTESIAN_POINT('Ctrl Pts',(3.7,1.98630780592131,-20.4055104950545)) ;
#168478=CARTESIAN_POINT('Ctrl Pts',(3.7,1.98660254037844,-20.405)) ;
#168479=CARTESIAN_POINT('Origin',(3.7,1.9,-20.355)) ;
#168480=CARTESIAN_POINT('Origin',(10.2,1.9,-20.355)) ;
#168481=CARTESIAN_POINT('Origin',(3.7,1.9,-20.355)) ;
#168482=CARTESIAN_POINT('Origin',(10.1,1.9,-20.355)) ;
#168483=CARTESIAN_POINT('Origin',(10.1,1.9,-20.355)) ;
#168484=CARTESIAN_POINT('Origin',(3.7,2.1,-17.745)) ;
#168485=CARTESIAN_POINT('',(3.7,1.98660254037844,-17.695)) ;
#168486=CARTESIAN_POINT('Origin',(3.7,1.9,-17.745)) ;
#168487=CARTESIAN_POINT('Ctrl Pts',(3.7,1.98660254037844,-17.695)) ;
#168488=CARTESIAN_POINT('Ctrl Pts',(3.69999911718144,1.98567700534182,-17.6933969262924)) ;
#168489=CARTESIAN_POINT('Ctrl Pts',(3.69968163901485,1.98470369933599,-17.6918180022845)) ;
#168490=CARTESIAN_POINT('Ctrl Pts',(3.69895427931585,1.98325895404994,-17.6895944560408)) ;
#168491=CARTESIAN_POINT('Ctrl Pts',(3.69867650892745,1.9827864959068,-17.6888860984239)) ;
#168492=CARTESIAN_POINT('Ctrl Pts',(3.69717970712967,1.9804354328423,-17.6854409187843)) ;
#168493=CARTESIAN_POINT('Ctrl Pts',(3.69541014605544,1.97847095301992,-17.6828241208443)) ;
#168494=CARTESIAN_POINT('Ctrl Pts',(3.69146029518774,1.97457001268155,-17.677973443509)) ;
#168495=CARTESIAN_POINT('Ctrl Pts',(3.68915436790411,1.97254004967205,-17.6756322068765)) ;
#168496=CARTESIAN_POINT('Ctrl Pts',(3.68263623161792,1.9668885044718,-17.6694999184568)) ;
#168497=CARTESIAN_POINT('Ctrl Pts',(3.67796661383158,1.96321337091312,-17.6659792522831)) ;
#168498=CARTESIAN_POINT('Ctrl Pts',(3.67279117399677,1.95950210067476,-17.6627623433945)) ;
#168499=CARTESIAN_POINT('Ctrl Pts',(3.67252519027994,1.95931231248683,-17.6625988090582)) ;
#168500=CARTESIAN_POINT('Ctrl Pts',(3.6693311210617,1.95704457126181,-17.6606562043068)) ;
#168501=CARTESIAN_POINT('Ctrl Pts',(3.66628216680076,1.95498580453519,-17.6590096122391)) ;
#168502=CARTESIAN_POINT('Ctrl Pts',(3.65739884032376,1.94929644648107,-17.6547590242123)) ;
#168503=CARTESIAN_POINT('Ctrl Pts',(3.65126071410426,1.94574201114262,-17.6524711332688)) ;
#168504=CARTESIAN_POINT('Ctrl Pts',(3.64132315686417,1.94068746317945,-17.6496379659013)) ;
#168505=CARTESIAN_POINT('Ctrl Pts',(3.63763353946351,1.93894751340588,-17.6487565993848)) ;
#168506=CARTESIAN_POINT('Ctrl Pts',(3.62813871250313,1.93486114467725,-17.6469043913581)) ;
#168507=CARTESIAN_POINT('Ctrl Pts',(3.62220485292998,1.93266004719376,-17.6461153440415)) ;
#168508=CARTESIAN_POINT('Ctrl Pts',(3.61359543742287,1.93003167234274,-17.6454202174511)) ;
#168509=CARTESIAN_POINT('Ctrl Pts',(3.61101642176938,1.92931331154694,-17.6452669825531)) ;
#168510=CARTESIAN_POINT('Ctrl Pts',(3.60562851963576,1.92796119665929,-17.6450532567727)) ;
#168511=CARTESIAN_POINT('Ctrl Pts',(3.60282089026104,1.92733781012834,-17.645)) ;
#168512=CARTESIAN_POINT('Ctrl Pts',(3.6,1.92679491924311,-17.645)) ;
#168513=CARTESIAN_POINT('Origin',(3.6,1.9,-17.745)) ;
#168514=CARTESIAN_POINT('Origin',(3.7,1.9,-17.745)) ;
#168515=CARTESIAN_POINT('Origin',(10.1,1.9,-17.745)) ;
#168516=CARTESIAN_POINT('Origin',(10.1,1.9,-17.745)) ;
#168517=CARTESIAN_POINT('Origin',(3.7,2.1,-24.165)) ;
#168518=CARTESIAN_POINT('',(3.7,1.98660254037845,-24.215)) ;
#168519=CARTESIAN_POINT('Ctrl Pts',(3.60000000000001,1.92679491924311,-24.265)) ;
#168520=CARTESIAN_POINT('Ctrl Pts',(3.60642117639458,1.92803067521642,-24.265)) ;
#168521=CARTESIAN_POINT('Ctrl Pts',(3.61278477806449,1.9296889667091,-24.2647228136141)) ;
#168522=CARTESIAN_POINT('Ctrl Pts',(3.6189728323945,1.93170032347237,-24.2641235249137)) ;
#168523=CARTESIAN_POINT('Ctrl Pts',(3.62020584678389,1.93210110079252,-24.2640041123243)) ;
#168524=CARTESIAN_POINT('Ctrl Pts',(3.62143195421067,1.93251577262747,-24.2638720028083)) ;
#168525=CARTESIAN_POINT('Ctrl Pts',(3.62265032708637,1.93294361409315,-24.263726982434)) ;
#168526=CARTESIAN_POINT('Ctrl Pts',(3.62647624625549,1.9342871164786,-24.2632715912801)) ;
#168527=CARTESIAN_POINT('Ctrl Pts',(3.63025346237246,1.93576539638805,-24.2626857368177)) ;
#168528=CARTESIAN_POINT('Ctrl Pts',(3.6339385638818,1.9373536406594,-24.2619650362697)) ;
#168529=CARTESIAN_POINT('Ctrl Pts',(3.63907793749079,1.93956866259898,-24.2609599216571)) ;
#168530=CARTESIAN_POINT('Ctrl Pts',(3.64410916187594,1.94202076919911,-24.2596787224496)) ;
#168531=CARTESIAN_POINT('Ctrl Pts',(3.64894317395081,1.94461872744766,-24.2581221777359)) ;
#168532=CARTESIAN_POINT('Ctrl Pts',(3.64993855309173,1.94515367717669,-24.2578016671298)) ;
#168533=CARTESIAN_POINT('Ctrl Pts',(3.65092568100079,1.94569474416708,-24.2574696031568)) ;
#168534=CARTESIAN_POINT('Ctrl Pts',(3.65190395907095,1.9462410440495,-24.2571261809367)) ;
#168535=CARTESIAN_POINT('Ctrl Pts',(3.65241342868351,1.94652554719632,-24.2569473328252)) ;
#168536=CARTESIAN_POINT('Ctrl Pts',(3.65292046817499,1.9468114778021,-24.25676540574)) ;
#168537=CARTESIAN_POINT('Ctrl Pts',(3.65342498214111,1.94709871486667,-24.2565804336333)) ;
#168538=CARTESIAN_POINT('Ctrl Pts',(3.65677402871197,1.94900544167846,-24.2553525584084)) ;
#168539=CARTESIAN_POINT('Ctrl Pts',(3.66003813592314,1.95098496635819,-24.2539806366809)) ;
#168540=CARTESIAN_POINT('Ctrl Pts',(3.66320312645637,1.95301617633163,-24.252462401394)) ;
#168541=CARTESIAN_POINT('Ctrl Pts',(3.66757373088834,1.95582111846937,-24.250365837185)) ;
#168542=CARTESIAN_POINT('Ctrl Pts',(3.67181875309416,1.95875330073098,-24.2479661261707)) ;
#168543=CARTESIAN_POINT('Ctrl Pts',(3.67584388612586,1.96174615985107,-24.2452600357853)) ;
#168544=CARTESIAN_POINT('Ctrl Pts',(3.67661208162847,1.96231734616911,-24.2447435791993)) ;
#168545=CARTESIAN_POINT('Ctrl Pts',(3.67737237849424,1.96289065080973,-24.2442160158762)) ;
#168546=CARTESIAN_POINT('Ctrl Pts',(3.6781242821482,1.96346549106044,-24.2436773988354)) ;
#168547=CARTESIAN_POINT('Ctrl Pts',(3.67853493948893,1.96377944400835,-24.2433832294422)) ;
#168548=CARTESIAN_POINT('Ctrl Pts',(3.67894301851555,1.96409388168833,-24.2430857517432)) ;
#168549=CARTESIAN_POINT('Ctrl Pts',(3.67934840022277,1.96440871854255,-24.2427849693981)) ;
#168550=CARTESIAN_POINT('Ctrl Pts',(3.68198440184425,1.96645595067817,-24.2408291269535)) ;
#168551=CARTESIAN_POINT('Ctrl Pts',(3.68449751351863,1.96851545671311,-24.2387382834716)) ;
#168552=CARTESIAN_POINT('Ctrl Pts',(3.68685379133722,1.97055696562016,-24.2365208503987)) ;
#168553=CARTESIAN_POINT('Ctrl Pts',(3.68896164651379,1.97238323800783,-24.2345372015503)) ;
#168554=CARTESIAN_POINT('Ctrl Pts',(3.69104797813193,1.97419718002536,-24.23244243878)) ;
#168555=CARTESIAN_POINT('Ctrl Pts',(3.69290978292477,1.97598569412151,-24.2302450010325)) ;
#168556=CARTESIAN_POINT('Ctrl Pts',(3.69362192319636,1.97666980070404,-24.2294044811669)) ;
#168557=CARTESIAN_POINT('Ctrl Pts',(3.69430163271857,1.97734979318965,-24.2285489756153)) ;
#168558=CARTESIAN_POINT('Ctrl Pts',(3.69493905694206,1.97802369895107,-24.227679088363)) ;
#168559=CARTESIAN_POINT('Ctrl Pts',(3.69605143900786,1.9791997456958,-24.2261610303053)) ;
#168560=CARTESIAN_POINT('Ctrl Pts',(3.69703421735413,1.98035885502255,-24.2245986233173)) ;
#168561=CARTESIAN_POINT('Ctrl Pts',(3.69784750664911,1.98151165953424,-24.2229571915312)) ;
#168562=CARTESIAN_POINT('Ctrl Pts',(3.69841279947844,1.98231293913807,-24.2218162818643)) ;
#168563=CARTESIAN_POINT('Ctrl Pts',(3.69890310384955,1.98311438470599,-24.2206332480121)) ;
#168564=CARTESIAN_POINT('Ctrl Pts',(3.69929098301996,1.98393783265456,-24.2193581070746)) ;
#168565=CARTESIAN_POINT('Ctrl Pts',(3.69936193271526,1.98408845528528,-24.2191248621161)) ;
#168566=CARTESIAN_POINT('Ctrl Pts',(3.69942931950317,1.98423979370565,-24.2188885146859)) ;
#168567=CARTESIAN_POINT('Ctrl Pts',(3.69949277412723,1.98439195189921,-24.2186487302853)) ;
#168568=CARTESIAN_POINT('Ctrl Pts',(3.69967702385848,1.98483376534753,-24.2179524813984)) ;
#168569=CARTESIAN_POINT('Ctrl Pts',(3.69981936684304,1.98527475083255,-24.2172393342586)) ;
#168570=CARTESIAN_POINT('Ctrl Pts',(3.69990669142684,1.98570953653118,-24.2165158410282)) ;
#168571=CARTESIAN_POINT('Ctrl Pts',(3.69996666908332,1.98600816294476,-24.2160189199259)) ;
#168572=CARTESIAN_POINT('Ctrl Pts',(3.7,1.98630780592131,-24.2155104950545)) ;
#168573=CARTESIAN_POINT('Ctrl Pts',(3.7,1.98660254037844,-24.215)) ;
#168574=CARTESIAN_POINT('Origin',(3.7,1.9,-24.165)) ;
#168575=CARTESIAN_POINT('Origin',(10.2,1.9,-24.165)) ;
#168576=CARTESIAN_POINT('Origin',(3.7,1.9,-24.165)) ;
#168577=CARTESIAN_POINT('Origin',(10.1,1.9,-24.165)) ;
#168578=CARTESIAN_POINT('Origin',(10.1,1.9,-24.165)) ;
#168579=CARTESIAN_POINT('Origin',(3.7,2.1,-21.555)) ;
#168580=CARTESIAN_POINT('',(3.7,1.98660254037844,-21.505)) ;
#168581=CARTESIAN_POINT('Origin',(3.7,1.9,-21.555)) ;
#168582=CARTESIAN_POINT('Ctrl Pts',(3.7,1.98660254037844,-21.505)) ;
#168583=CARTESIAN_POINT('Ctrl Pts',(3.69999911718144,1.98567700534182,-21.5033969262924)) ;
#168584=CARTESIAN_POINT('Ctrl Pts',(3.69968163901484,1.98470369933599,-21.5018180022845)) ;
#168585=CARTESIAN_POINT('Ctrl Pts',(3.69895427931585,1.98325895404993,-21.4995944560408)) ;
#168586=CARTESIAN_POINT('Ctrl Pts',(3.69867650892744,1.9827864959068,-21.4988860984239)) ;
#168587=CARTESIAN_POINT('Ctrl Pts',(3.69717970712967,1.98043543284229,-21.4954409187843)) ;
#168588=CARTESIAN_POINT('Ctrl Pts',(3.69541014605544,1.97847095301991,-21.4928241208443)) ;
#168589=CARTESIAN_POINT('Ctrl Pts',(3.69146029518774,1.97457001268155,-21.487973443509)) ;
#168590=CARTESIAN_POINT('Ctrl Pts',(3.68915436790411,1.97254004967205,-21.4856322068765)) ;
#168591=CARTESIAN_POINT('Ctrl Pts',(3.68263623161789,1.96688850447178,-21.4794999184567)) ;
#168592=CARTESIAN_POINT('Ctrl Pts',(3.67796661383153,1.96321337091308,-21.475979252283)) ;
#168593=CARTESIAN_POINT('Ctrl Pts',(3.67279117399672,1.95950210067472,-21.4727623433945)) ;
#168594=CARTESIAN_POINT('Ctrl Pts',(3.67252519027991,1.95931231248681,-21.4725988090581)) ;
#168595=CARTESIAN_POINT('Ctrl Pts',(3.6693311210617,1.95704457126181,-21.4706562043068)) ;
#168596=CARTESIAN_POINT('Ctrl Pts',(3.66628216680076,1.95498580453519,-21.4690096122391)) ;
#168597=CARTESIAN_POINT('Ctrl Pts',(3.65739884032377,1.94929644648107,-21.4647590242123)) ;
#168598=CARTESIAN_POINT('Ctrl Pts',(3.65126071410427,1.94574201114262,-21.4624711332688)) ;
#168599=CARTESIAN_POINT('Ctrl Pts',(3.64132315686418,1.94068746317945,-21.4596379659013)) ;
#168600=CARTESIAN_POINT('Ctrl Pts',(3.63763353946351,1.93894751340588,-21.4587565993848)) ;
#168601=CARTESIAN_POINT('Ctrl Pts',(3.62813871250314,1.93486114467726,-21.4569043913581)) ;
#168602=CARTESIAN_POINT('Ctrl Pts',(3.62220485292999,1.93266004719377,-21.4561153440415)) ;
#168603=CARTESIAN_POINT('Ctrl Pts',(3.61359543742306,1.9300316723428,-21.4554202174511)) ;
#168604=CARTESIAN_POINT('Ctrl Pts',(3.61101642176975,1.92931331154704,-21.4552669825532)) ;
#168605=CARTESIAN_POINT('Ctrl Pts',(3.60562851963613,1.92796119665937,-21.4550532567727)) ;
#168606=CARTESIAN_POINT('Ctrl Pts',(3.60282089026123,1.92733781012838,-21.455)) ;
#168607=CARTESIAN_POINT('Ctrl Pts',(3.6,1.92679491924311,-21.455)) ;
#168608=CARTESIAN_POINT('Origin',(3.6,1.9,-21.555)) ;
#168609=CARTESIAN_POINT('Origin',(3.7,1.9,-21.555)) ;
#168610=CARTESIAN_POINT('Origin',(10.1,1.9,-21.555)) ;
#168611=CARTESIAN_POINT('Origin',(10.1,1.9,-21.555)) ;
#168612=CARTESIAN_POINT('Origin',(3.7,2.1,-27.975)) ;
#168613=CARTESIAN_POINT('',(3.7,1.98660254037845,-28.025)) ;
#168614=CARTESIAN_POINT('Ctrl Pts',(3.60000000000001,1.92679491924311,-28.075)) ;
#168615=CARTESIAN_POINT('Ctrl Pts',(3.60642117639513,1.92803067521652,-28.075)) ;
#168616=CARTESIAN_POINT('Ctrl Pts',(3.61278477806557,1.92968896670937,-28.074722813614)) ;
#168617=CARTESIAN_POINT('Ctrl Pts',(3.61897283239608,1.93170032347287,-28.0741235249136)) ;
#168618=CARTESIAN_POINT('Ctrl Pts',(3.62020584678494,1.93210110079286,-28.0740041123242)) ;
#168619=CARTESIAN_POINT('Ctrl Pts',(3.62143195421119,1.93251577262764,-28.0738720028082)) ;
#168620=CARTESIAN_POINT('Ctrl Pts',(3.62265032708637,1.93294361409314,-28.073726982434)) ;
#168621=CARTESIAN_POINT('Ctrl Pts',(3.62647624625549,1.9342871164786,-28.0732715912801)) ;
#168622=CARTESIAN_POINT('Ctrl Pts',(3.63025346237246,1.93576539638806,-28.0726857368177)) ;
#168623=CARTESIAN_POINT('Ctrl Pts',(3.6339385638818,1.9373536406594,-28.0719650362697)) ;
#168624=CARTESIAN_POINT('Ctrl Pts',(3.63907793749119,1.93956866259915,-28.0709599216571)) ;
#168625=CARTESIAN_POINT('Ctrl Pts',(3.64410916187671,1.94202076919947,-28.0696787224494)) ;
#168626=CARTESIAN_POINT('Ctrl Pts',(3.64894317395192,1.94461872744825,-28.0681221777355)) ;
#168627=CARTESIAN_POINT('Ctrl Pts',(3.64993855309245,1.94515367717709,-28.0678016671295)) ;
#168628=CARTESIAN_POINT('Ctrl Pts',(3.65092568100114,1.94569474416728,-28.0674696031567)) ;
#168629=CARTESIAN_POINT('Ctrl Pts',(3.65190395907093,1.94624104404949,-28.0671261809367)) ;
#168630=CARTESIAN_POINT('Ctrl Pts',(3.6524134286835,1.94652554719633,-28.0669473328252)) ;
#168631=CARTESIAN_POINT('Ctrl Pts',(3.65292046817498,1.94681147780211,-28.06676540574)) ;
#168632=CARTESIAN_POINT('Ctrl Pts',(3.6534249821411,1.94709871486668,-28.0665804336333)) ;
#168633=CARTESIAN_POINT('Ctrl Pts',(3.65677402871197,1.94900544167846,-28.0653525584084)) ;
#168634=CARTESIAN_POINT('Ctrl Pts',(3.66003813592314,1.95098496635819,-28.0639806366809)) ;
#168635=CARTESIAN_POINT('Ctrl Pts',(3.66320312645637,1.95301617633164,-28.062462401394)) ;
#168636=CARTESIAN_POINT('Ctrl Pts',(3.66757373088807,1.95582111846921,-28.0603658371851)) ;
#168637=CARTESIAN_POINT('Ctrl Pts',(3.67181875309364,1.95875330073064,-28.0579661261709)) ;
#168638=CARTESIAN_POINT('Ctrl Pts',(3.67584388612511,1.96174615985051,-28.0552600357858)) ;
#168639=CARTESIAN_POINT('Ctrl Pts',(3.67661208162794,1.9623173461687,-28.0547435791997)) ;
#168640=CARTESIAN_POINT('Ctrl Pts',(3.67737237849392,1.96289065080947,-28.0542160158765)) ;
#168641=CARTESIAN_POINT('Ctrl Pts',(3.67812428214809,1.96346549106034,-28.0536773988355)) ;
#168642=CARTESIAN_POINT('Ctrl Pts',(3.67853493948886,1.96377944400827,-28.0533832294423)) ;
#168643=CARTESIAN_POINT('Ctrl Pts',(3.67894301851552,1.96409388168833,-28.0530857517432)) ;
#168644=CARTESIAN_POINT('Ctrl Pts',(3.67934840022277,1.96440871854257,-28.0527849693981)) ;
#168645=CARTESIAN_POINT('Ctrl Pts',(3.68198440184425,1.96645595067818,-28.0508291269535)) ;
#168646=CARTESIAN_POINT('Ctrl Pts',(3.68449751351863,1.96851545671303,-28.0487382834717)) ;
#168647=CARTESIAN_POINT('Ctrl Pts',(3.68685379133722,1.97055696562012,-28.0465208503988)) ;
#168648=CARTESIAN_POINT('Ctrl Pts',(3.68896164651378,1.97238323800781,-28.0445372015504)) ;
#168649=CARTESIAN_POINT('Ctrl Pts',(3.69104797813191,1.97419718002534,-28.04244243878)) ;
#168650=CARTESIAN_POINT('Ctrl Pts',(3.69290978292473,1.97598569412148,-28.0402450010326)) ;
#168651=CARTESIAN_POINT('Ctrl Pts',(3.69362192319633,1.97666980070402,-28.0394044811669)) ;
#168652=CARTESIAN_POINT('Ctrl Pts',(3.69430163271855,1.97734979318964,-28.0385489756153)) ;
#168653=CARTESIAN_POINT('Ctrl Pts',(3.69493905694205,1.97802369895107,-28.037679088363)) ;
#168654=CARTESIAN_POINT('Ctrl Pts',(3.69605143900785,1.9791997456958,-28.0361610303053)) ;
#168655=CARTESIAN_POINT('Ctrl Pts',(3.69703421735413,1.98035885502255,-28.0345986233173)) ;
#168656=CARTESIAN_POINT('Ctrl Pts',(3.69784750664911,1.98151165953425,-28.0329571915311)) ;
#168657=CARTESIAN_POINT('Ctrl Pts',(3.69841279947842,1.98231293913806,-28.0318162818644)) ;
#168658=CARTESIAN_POINT('Ctrl Pts',(3.69890310384951,1.98311438470593,-28.0306332480122)) ;
#168659=CARTESIAN_POINT('Ctrl Pts',(3.69929098301991,1.98393783265451,-28.0293581070747)) ;
#168660=CARTESIAN_POINT('Ctrl Pts',(3.69936193271523,1.98408845528527,-28.0291248621162)) ;
#168661=CARTESIAN_POINT('Ctrl Pts',(3.69942931950316,1.98423979370561,-28.028888514686)) ;
#168662=CARTESIAN_POINT('Ctrl Pts',(3.69949277412724,1.9843919518992,-28.0286487302853)) ;
#168663=CARTESIAN_POINT('Ctrl Pts',(3.69967702385849,1.98483376534753,-28.0279524813983)) ;
#168664=CARTESIAN_POINT('Ctrl Pts',(3.69981936684304,1.98527475083255,-28.0272393342586)) ;
#168665=CARTESIAN_POINT('Ctrl Pts',(3.69990669142683,1.98570953653118,-28.0265158410282)) ;
#168666=CARTESIAN_POINT('Ctrl Pts',(3.69996666908332,1.98600816294476,-28.0260189199259)) ;
#168667=CARTESIAN_POINT('Ctrl Pts',(3.7,1.98630780592131,-28.0255104950545)) ;
#168668=CARTESIAN_POINT('Ctrl Pts',(3.7,1.98660254037844,-28.025)) ;
#168669=CARTESIAN_POINT('Origin',(3.7,1.9,-27.975)) ;
#168670=CARTESIAN_POINT('Origin',(10.2,1.9,-27.975)) ;
#168671=CARTESIAN_POINT('Origin',(3.7,1.9,-27.975)) ;
#168672=CARTESIAN_POINT('Origin',(10.1,1.9,-27.975)) ;
#168673=CARTESIAN_POINT('Origin',(10.1,1.9,-27.975)) ;
#168674=CARTESIAN_POINT('Origin',(3.7,2.1,-25.365)) ;
#168675=CARTESIAN_POINT('',(3.7,1.98660254037844,-25.315)) ;
#168676=CARTESIAN_POINT('Origin',(3.7,1.9,-25.365)) ;
#168677=CARTESIAN_POINT('Ctrl Pts',(3.7,1.98660254037844,-25.315)) ;
#168678=CARTESIAN_POINT('Ctrl Pts',(3.69999911718144,1.98567700534182,-25.3133969262924)) ;
#168679=CARTESIAN_POINT('Ctrl Pts',(3.69968163901484,1.98470369933599,-25.3118180022845)) ;
#168680=CARTESIAN_POINT('Ctrl Pts',(3.69895427931585,1.98325895404993,-25.3095944560408)) ;
#168681=CARTESIAN_POINT('Ctrl Pts',(3.69867650892744,1.9827864959068,-25.3088860984239)) ;
#168682=CARTESIAN_POINT('Ctrl Pts',(3.69717970712967,1.98043543284229,-25.3054409187843)) ;
#168683=CARTESIAN_POINT('Ctrl Pts',(3.69541014605544,1.97847095301992,-25.3028241208443)) ;
#168684=CARTESIAN_POINT('Ctrl Pts',(3.69146029518774,1.97457001268155,-25.297973443509)) ;
#168685=CARTESIAN_POINT('Ctrl Pts',(3.68915436790411,1.97254004967205,-25.2956322068765)) ;
#168686=CARTESIAN_POINT('Ctrl Pts',(3.68263623161792,1.96688850447181,-25.2894999184568)) ;
#168687=CARTESIAN_POINT('Ctrl Pts',(3.6779666138316,1.96321337091313,-25.2859792522831)) ;
#168688=CARTESIAN_POINT('Ctrl Pts',(3.67279117399679,1.95950210067478,-25.2827623433946)) ;
#168689=CARTESIAN_POINT('Ctrl Pts',(3.67252519027995,1.95931231248684,-25.2825988090582)) ;
#168690=CARTESIAN_POINT('Ctrl Pts',(3.6693311210617,1.95704457126181,-25.2806562043068)) ;
#168691=CARTESIAN_POINT('Ctrl Pts',(3.66628216680076,1.95498580453519,-25.2790096122391)) ;
#168692=CARTESIAN_POINT('Ctrl Pts',(3.65739884032376,1.94929644648107,-25.2747590242123)) ;
#168693=CARTESIAN_POINT('Ctrl Pts',(3.65126071410426,1.94574201114262,-25.2724711332688)) ;
#168694=CARTESIAN_POINT('Ctrl Pts',(3.64132315686417,1.94068746317945,-25.2696379659012)) ;
#168695=CARTESIAN_POINT('Ctrl Pts',(3.63763353946351,1.93894751340588,-25.2687565993848)) ;
#168696=CARTESIAN_POINT('Ctrl Pts',(3.62813871250315,1.93486114467726,-25.2669043913581)) ;
#168697=CARTESIAN_POINT('Ctrl Pts',(3.62220485293001,1.93266004719377,-25.2661153440415)) ;
#168698=CARTESIAN_POINT('Ctrl Pts',(3.61359543742302,1.93003167234278,-25.2654202174511)) ;
#168699=CARTESIAN_POINT('Ctrl Pts',(3.61101642176965,1.92931331154701,-25.2652669825532)) ;
#168700=CARTESIAN_POINT('Ctrl Pts',(3.60562851963602,1.92796119665935,-25.2650532567727)) ;
#168701=CARTESIAN_POINT('Ctrl Pts',(3.60282089026117,1.92733781012837,-25.265)) ;
#168702=CARTESIAN_POINT('Ctrl Pts',(3.6,1.92679491924311,-25.265)) ;
#168703=CARTESIAN_POINT('Origin',(3.6,1.9,-25.365)) ;
#168704=CARTESIAN_POINT('Origin',(3.7,1.9,-25.365)) ;
#168705=CARTESIAN_POINT('Origin',(10.1,1.9,-25.365)) ;
#168706=CARTESIAN_POINT('Origin',(10.1,1.9,-25.365)) ;
#168707=CARTESIAN_POINT('Origin',(3.7,2.1,-31.785)) ;
#168708=CARTESIAN_POINT('',(3.7,1.98660254037844,-31.835)) ;
#168709=CARTESIAN_POINT('Ctrl Pts',(3.6,1.92679491924311,-31.885)) ;
#168710=CARTESIAN_POINT('Ctrl Pts',(3.6064211763948,1.92803067521646,-31.885)) ;
#168711=CARTESIAN_POINT('Ctrl Pts',(3.61278477806494,1.92968896670921,-31.8847228136141)) ;
#168712=CARTESIAN_POINT('Ctrl Pts',(3.61897283239515,1.93170032347258,-31.8841235249137)) ;
#168713=CARTESIAN_POINT('Ctrl Pts',(3.62020584678433,1.93210110079266,-31.8840041123243)) ;
#168714=CARTESIAN_POINT('Ctrl Pts',(3.62143195421089,1.93251577262754,-31.8838720028083)) ;
#168715=CARTESIAN_POINT('Ctrl Pts',(3.62265032708637,1.93294361409314,-31.883726982434)) ;
#168716=CARTESIAN_POINT('Ctrl Pts',(3.62647624625549,1.9342871164786,-31.8832715912801)) ;
#168717=CARTESIAN_POINT('Ctrl Pts',(3.63025346237246,1.93576539638805,-31.8826857368177)) ;
#168718=CARTESIAN_POINT('Ctrl Pts',(3.6339385638818,1.9373536406594,-31.8819650362697)) ;
#168719=CARTESIAN_POINT('Ctrl Pts',(3.6390779374906,1.9395686625989,-31.8809599216572)) ;
#168720=CARTESIAN_POINT('Ctrl Pts',(3.64410916187556,1.94202076919892,-31.8796787224497)) ;
#168721=CARTESIAN_POINT('Ctrl Pts',(3.64894317395025,1.94461872744736,-31.878122177736)) ;
#168722=CARTESIAN_POINT('Ctrl Pts',(3.6499385530912,1.94515367717641,-31.8778016671299)) ;
#168723=CARTESIAN_POINT('Ctrl Pts',(3.6509256810003,1.9456947441668,-31.877469603157)) ;
#168724=CARTESIAN_POINT('Ctrl Pts',(3.65190395907048,1.94624104404923,-31.8771261809369)) ;
#168725=CARTESIAN_POINT('Ctrl Pts',(3.6524134286832,1.94652554719615,-31.8769473328253)) ;
#168726=CARTESIAN_POINT('Ctrl Pts',(3.65292046817483,1.94681147780198,-31.8767654057401)) ;
#168727=CARTESIAN_POINT('Ctrl Pts',(3.6534249821411,1.94709871486664,-31.8765804336333)) ;
#168728=CARTESIAN_POINT('Ctrl Pts',(3.65677402871197,1.94900544167845,-31.8753525584084)) ;
#168729=CARTESIAN_POINT('Ctrl Pts',(3.66003813592314,1.95098496635819,-31.8739806366809)) ;
#168730=CARTESIAN_POINT('Ctrl Pts',(3.66320312645637,1.95301617633165,-31.872462401394)) ;
#168731=CARTESIAN_POINT('Ctrl Pts',(3.66757373088845,1.95582111846949,-31.8703658371849)) ;
#168732=CARTESIAN_POINT('Ctrl Pts',(3.67181875309438,1.95875330073117,-31.8679661261705)) ;
#168733=CARTESIAN_POINT('Ctrl Pts',(3.67584388612618,1.96174615985132,-31.8652600357851)) ;
#168734=CARTESIAN_POINT('Ctrl Pts',(3.6766120816284,1.96231734616908,-31.8647435791993)) ;
#168735=CARTESIAN_POINT('Ctrl Pts',(3.67737237849379,1.9628906508094,-31.8642160158765)) ;
#168736=CARTESIAN_POINT('Ctrl Pts',(3.67812428214738,1.96346549105982,-31.863677398836)) ;
#168737=CARTESIAN_POINT('Ctrl Pts',(3.67853493948839,1.96377944400794,-31.8633832294426)) ;
#168738=CARTESIAN_POINT('Ctrl Pts',(3.67894301851528,1.96409388168812,-31.8630857517434)) ;
#168739=CARTESIAN_POINT('Ctrl Pts',(3.67934840022277,1.96440871854255,-31.8627849693981)) ;
#168740=CARTESIAN_POINT('Ctrl Pts',(3.68198440184425,1.96645595067817,-31.8608291269535)) ;
#168741=CARTESIAN_POINT('Ctrl Pts',(3.68449751351863,1.96851545671311,-31.8587382834716)) ;
#168742=CARTESIAN_POINT('Ctrl Pts',(3.68685379133723,1.97055696562017,-31.8565208503987)) ;
#168743=CARTESIAN_POINT('Ctrl Pts',(3.68896164651388,1.9723832380079,-31.8545372015503)) ;
#168744=CARTESIAN_POINT('Ctrl Pts',(3.69104797813211,1.97419718002555,-31.8524424387797)) ;
#168745=CARTESIAN_POINT('Ctrl Pts',(3.692909782925,1.97598569412177,-31.8502450010322)) ;
#168746=CARTESIAN_POINT('Ctrl Pts',(3.6936219231965,1.97666980070423,-31.8494044811667)) ;
#168747=CARTESIAN_POINT('Ctrl Pts',(3.69430163271863,1.97734979318975,-31.8485489756152)) ;
#168748=CARTESIAN_POINT('Ctrl Pts',(3.69493905694205,1.97802369895109,-31.847679088363)) ;
#168749=CARTESIAN_POINT('Ctrl Pts',(3.69605143900784,1.9791997456958,-31.8461610303053)) ;
#168750=CARTESIAN_POINT('Ctrl Pts',(3.69703421735413,1.98035885502255,-31.8445986233173)) ;
#168751=CARTESIAN_POINT('Ctrl Pts',(3.6978475066491,1.98151165953424,-31.8429571915312)) ;
#168752=CARTESIAN_POINT('Ctrl Pts',(3.69841279947843,1.98231293913806,-31.8418162818644)) ;
#168753=CARTESIAN_POINT('Ctrl Pts',(3.69890310384954,1.98311438470598,-31.8406332480121)) ;
#168754=CARTESIAN_POINT('Ctrl Pts',(3.69929098301994,1.98393783265454,-31.8393581070746)) ;
#168755=CARTESIAN_POINT('Ctrl Pts',(3.69936193271525,1.98408845528528,-31.8391248621161)) ;
#168756=CARTESIAN_POINT('Ctrl Pts',(3.69942931950318,1.98423979370566,-31.8388885146859)) ;
#168757=CARTESIAN_POINT('Ctrl Pts',(3.69949277412726,1.98439195189924,-31.8386487302852)) ;
#168758=CARTESIAN_POINT('Ctrl Pts',(3.6996770238585,1.98483376534753,-31.8379524813983)) ;
#168759=CARTESIAN_POINT('Ctrl Pts',(3.69981936684305,1.98527475083261,-31.8372393342585)) ;
#168760=CARTESIAN_POINT('Ctrl Pts',(3.69990669142684,1.98570953653123,-31.8365158410281)) ;
#168761=CARTESIAN_POINT('Ctrl Pts',(3.69996666908332,1.98600816294481,-31.8360189199258)) ;
#168762=CARTESIAN_POINT('Ctrl Pts',(3.7,1.98630780592131,-31.8355104950545)) ;
#168763=CARTESIAN_POINT('Ctrl Pts',(3.7,1.98660254037844,-31.835)) ;
#168764=CARTESIAN_POINT('Origin',(3.7,1.9,-31.785)) ;
#168765=CARTESIAN_POINT('Origin',(10.2,1.9,-31.785)) ;
#168766=CARTESIAN_POINT('Origin',(3.7,1.9,-31.785)) ;
#168767=CARTESIAN_POINT('Origin',(10.1,1.9,-31.785)) ;
#168768=CARTESIAN_POINT('Origin',(10.1,1.9,-31.785)) ;
#168769=CARTESIAN_POINT('Origin',(3.7,2.1,-29.175)) ;
#168770=CARTESIAN_POINT('',(3.7,1.98660254037844,-29.125)) ;
#168771=CARTESIAN_POINT('Origin',(3.7,1.9,-29.175)) ;
#168772=CARTESIAN_POINT('Ctrl Pts',(3.7,1.98660254037844,-29.125)) ;
#168773=CARTESIAN_POINT('Ctrl Pts',(3.69999911718144,1.98567700534183,-29.1233969262924)) ;
#168774=CARTESIAN_POINT('Ctrl Pts',(3.69968163901485,1.984703699336,-29.1218180022846)) ;
#168775=CARTESIAN_POINT('Ctrl Pts',(3.69895427931585,1.98325895404995,-29.1195944560408)) ;
#168776=CARTESIAN_POINT('Ctrl Pts',(3.69867650892745,1.98278649590681,-29.1188860984239)) ;
#168777=CARTESIAN_POINT('Ctrl Pts',(3.69717970712967,1.9804354328423,-29.1154409187843)) ;
#168778=CARTESIAN_POINT('Ctrl Pts',(3.69541014605544,1.97847095301992,-29.1128241208443)) ;
#168779=CARTESIAN_POINT('Ctrl Pts',(3.69146029518774,1.97457001268155,-29.107973443509)) ;
#168780=CARTESIAN_POINT('Ctrl Pts',(3.68915436790411,1.97254004967204,-29.1056322068765)) ;
#168781=CARTESIAN_POINT('Ctrl Pts',(3.68263623161792,1.9668885044718,-29.0994999184568)) ;
#168782=CARTESIAN_POINT('Ctrl Pts',(3.67796661383159,1.96321337091313,-29.0959792522831)) ;
#168783=CARTESIAN_POINT('Ctrl Pts',(3.67279117399678,1.95950210067477,-29.0927623433945)) ;
#168784=CARTESIAN_POINT('Ctrl Pts',(3.67252519027994,1.95931231248683,-29.0925988090582)) ;
#168785=CARTESIAN_POINT('Ctrl Pts',(3.6693311210617,1.95704457126181,-29.0906562043068)) ;
#168786=CARTESIAN_POINT('Ctrl Pts',(3.66628216680077,1.95498580453519,-29.0890096122391)) ;
#168787=CARTESIAN_POINT('Ctrl Pts',(3.65739884032376,1.94929644648107,-29.0847590242123)) ;
#168788=CARTESIAN_POINT('Ctrl Pts',(3.65126071410426,1.94574201114262,-29.0824711332688)) ;
#168789=CARTESIAN_POINT('Ctrl Pts',(3.64132315686417,1.94068746317945,-29.0796379659012)) ;
#168790=CARTESIAN_POINT('Ctrl Pts',(3.63763353946351,1.93894751340588,-29.0787565993848)) ;
#168791=CARTESIAN_POINT('Ctrl Pts',(3.62813871250316,1.93486114467726,-29.0769043913581)) ;
#168792=CARTESIAN_POINT('Ctrl Pts',(3.62220485293003,1.93266004719378,-29.0761153440415)) ;
#168793=CARTESIAN_POINT('Ctrl Pts',(3.61359543742317,1.93003167234283,-29.0754202174511)) ;
#168794=CARTESIAN_POINT('Ctrl Pts',(3.61101642176993,1.92931331154709,-29.0752669825532)) ;
#168795=CARTESIAN_POINT('Ctrl Pts',(3.60562851963629,1.92796119665941,-29.0750532567727)) ;
#168796=CARTESIAN_POINT('Ctrl Pts',(3.60282089026131,1.92733781012839,-29.075)) ;
#168797=CARTESIAN_POINT('Ctrl Pts',(3.6,1.92679491924311,-29.075)) ;
#168798=CARTESIAN_POINT('Origin',(3.6,1.9,-29.175)) ;
#168799=CARTESIAN_POINT('Origin',(3.7,1.9,-29.175)) ;
#168800=CARTESIAN_POINT('Origin',(10.1,1.9,-29.175)) ;
#168801=CARTESIAN_POINT('Origin',(10.1,1.9,-29.175)) ;
#168802=CARTESIAN_POINT('Origin',(3.7,2.1,-35.595)) ;
#168803=CARTESIAN_POINT('',(3.7,1.98660254037844,-35.645)) ;
#168804=CARTESIAN_POINT('Ctrl Pts',(3.6,1.92679491924311,-35.695)) ;
#168805=CARTESIAN_POINT('Ctrl Pts',(3.60642117639484,1.92803067521647,-35.695)) ;
#168806=CARTESIAN_POINT('Ctrl Pts',(3.61278477806502,1.92968896670923,-35.6947228136141)) ;
#168807=CARTESIAN_POINT('Ctrl Pts',(3.61897283239527,1.93170032347261,-35.6941235249137)) ;
#168808=CARTESIAN_POINT('Ctrl Pts',(3.6202058467844,1.93210110079268,-35.6940041123243)) ;
#168809=CARTESIAN_POINT('Ctrl Pts',(3.62143195421092,1.93251577262755,-35.6938720028083)) ;
#168810=CARTESIAN_POINT('Ctrl Pts',(3.62265032708637,1.93294361409314,-35.693726982434)) ;
#168811=CARTESIAN_POINT('Ctrl Pts',(3.62647624625549,1.9342871164786,-35.6932715912801)) ;
#168812=CARTESIAN_POINT('Ctrl Pts',(3.63025346237246,1.93576539638806,-35.6926857368177)) ;
#168813=CARTESIAN_POINT('Ctrl Pts',(3.6339385638818,1.9373536406594,-35.6919650362697)) ;
#168814=CARTESIAN_POINT('Ctrl Pts',(3.63907793749101,1.93956866259907,-35.6909599216571)) ;
#168815=CARTESIAN_POINT('Ctrl Pts',(3.64410916187638,1.94202076919931,-35.6896787224495)) ;
#168816=CARTESIAN_POINT('Ctrl Pts',(3.64894317395146,1.94461872744801,-35.6881221777356)) ;
#168817=CARTESIAN_POINT('Ctrl Pts',(3.64993855309196,1.94515367717683,-35.6878016671297)) ;
#168818=CARTESIAN_POINT('Ctrl Pts',(3.65092568100061,1.945694744167,-35.6874696031569)) ;
#168819=CARTESIAN_POINT('Ctrl Pts',(3.65190395907037,1.94624104404919,-35.6871261809369)) ;
#168820=CARTESIAN_POINT('Ctrl Pts',(3.65241342868313,1.94652554719613,-35.6869473328253)) ;
#168821=CARTESIAN_POINT('Ctrl Pts',(3.65292046817479,1.94681147780199,-35.6867654057401)) ;
#168822=CARTESIAN_POINT('Ctrl Pts',(3.6534249821411,1.94709871486666,-35.6865804336333)) ;
#168823=CARTESIAN_POINT('Ctrl Pts',(3.65677402871197,1.94900544167846,-35.6853525584084)) ;
#168824=CARTESIAN_POINT('Ctrl Pts',(3.66003813592314,1.95098496635819,-35.6839806366809)) ;
#168825=CARTESIAN_POINT('Ctrl Pts',(3.66320312645637,1.95301617633165,-35.682462401394)) ;
#168826=CARTESIAN_POINT('Ctrl Pts',(3.66757373088831,1.95582111846939,-35.680365837185)) ;
#168827=CARTESIAN_POINT('Ctrl Pts',(3.6718187530941,1.95875330073099,-35.6779661261707)) ;
#168828=CARTESIAN_POINT('Ctrl Pts',(3.67584388612577,1.961746159851,-35.6752600357853)) ;
#168829=CARTESIAN_POINT('Ctrl Pts',(3.67661208162811,1.96231734616883,-35.6747435791995)) ;
#168830=CARTESIAN_POINT('Ctrl Pts',(3.67737237849361,1.96289065080923,-35.6742160158767)) ;
#168831=CARTESIAN_POINT('Ctrl Pts',(3.6781242821473,1.96346549105972,-35.6736773988361)) ;
#168832=CARTESIAN_POINT('Ctrl Pts',(3.67853493948834,1.96377944400785,-35.6733832294426)) ;
#168833=CARTESIAN_POINT('Ctrl Pts',(3.67894301851526,1.96409388168811,-35.6730857517434)) ;
#168834=CARTESIAN_POINT('Ctrl Pts',(3.67934840022277,1.96440871854255,-35.6727849693981)) ;
#168835=CARTESIAN_POINT('Ctrl Pts',(3.68198440184426,1.96645595067816,-35.6708291269535)) ;
#168836=CARTESIAN_POINT('Ctrl Pts',(3.68449751351862,1.96851545671303,-35.6687382834717)) ;
#168837=CARTESIAN_POINT('Ctrl Pts',(3.68685379133722,1.97055696562012,-35.6665208503988)) ;
#168838=CARTESIAN_POINT('Ctrl Pts',(3.6889616465138,1.97238323800782,-35.6645372015503)) ;
#168839=CARTESIAN_POINT('Ctrl Pts',(3.69104797813196,1.97419718002538,-35.6624424387799)) ;
#168840=CARTESIAN_POINT('Ctrl Pts',(3.6929097829248,1.97598569412155,-35.6602450010325)) ;
#168841=CARTESIAN_POINT('Ctrl Pts',(3.69362192319637,1.97666980070406,-35.6594044811669)) ;
#168842=CARTESIAN_POINT('Ctrl Pts',(3.69430163271857,1.97734979318965,-35.6585489756153)) ;
#168843=CARTESIAN_POINT('Ctrl Pts',(3.69493905694204,1.97802369895106,-35.6576790883631)) ;
#168844=CARTESIAN_POINT('Ctrl Pts',(3.69605143900785,1.9791997456958,-35.6561610303053)) ;
#168845=CARTESIAN_POINT('Ctrl Pts',(3.69703421735413,1.98035885502254,-35.6545986233173)) ;
#168846=CARTESIAN_POINT('Ctrl Pts',(3.6978475066491,1.98151165953423,-35.6529571915312)) ;
#168847=CARTESIAN_POINT('Ctrl Pts',(3.69841279947843,1.98231293913806,-35.6518162818644)) ;
#168848=CARTESIAN_POINT('Ctrl Pts',(3.69890310384954,1.98311438470598,-35.6506332480122)) ;
#168849=CARTESIAN_POINT('Ctrl Pts',(3.69929098301995,1.98393783265456,-35.6493581070746)) ;
#168850=CARTESIAN_POINT('Ctrl Pts',(3.69936193271525,1.98408845528527,-35.6491248621162)) ;
#168851=CARTESIAN_POINT('Ctrl Pts',(3.69942931950315,1.98423979370559,-35.648888514686)) ;
#168852=CARTESIAN_POINT('Ctrl Pts',(3.69949277412721,1.98439195189914,-35.6486487302854)) ;
#168853=CARTESIAN_POINT('Ctrl Pts',(3.69967702385847,1.98483376534747,-35.6479524813984)) ;
#168854=CARTESIAN_POINT('Ctrl Pts',(3.69981936684304,1.98527475083255,-35.6472393342586)) ;
#168855=CARTESIAN_POINT('Ctrl Pts',(3.69990669142684,1.98570953653122,-35.6465158410281)) ;
#168856=CARTESIAN_POINT('Ctrl Pts',(3.69996666908332,1.98600816294481,-35.6460189199258)) ;
#168857=CARTESIAN_POINT('Ctrl Pts',(3.7,1.9863078059213,-35.6455104950545)) ;
#168858=CARTESIAN_POINT('Ctrl Pts',(3.7,1.98660254037844,-35.645)) ;
#168859=CARTESIAN_POINT('Origin',(3.7,1.9,-35.595)) ;
#168860=CARTESIAN_POINT('Origin',(10.2,1.9,-35.595)) ;
#168861=CARTESIAN_POINT('Origin',(3.7,1.9,-35.595)) ;
#168862=CARTESIAN_POINT('Origin',(10.1,1.9,-35.595)) ;
#168863=CARTESIAN_POINT('Origin',(10.1,1.9,-35.595)) ;
#168864=CARTESIAN_POINT('Origin',(3.7,2.1,-32.985)) ;
#168865=CARTESIAN_POINT('',(3.7,1.98660254037844,-32.935)) ;
#168866=CARTESIAN_POINT('Origin',(3.7,1.9,-32.985)) ;
#168867=CARTESIAN_POINT('Ctrl Pts',(3.7,1.98660254037844,-32.935)) ;
#168868=CARTESIAN_POINT('Ctrl Pts',(3.69999911718144,1.98567700534184,-32.9333969262924)) ;
#168869=CARTESIAN_POINT('Ctrl Pts',(3.69968163901486,1.98470369933604,-32.9318180022846)) ;
#168870=CARTESIAN_POINT('Ctrl Pts',(3.69895427931588,1.98325895404998,-32.9295944560409)) ;
#168871=CARTESIAN_POINT('Ctrl Pts',(3.69867650892746,1.98278649590682,-32.9288860984239)) ;
#168872=CARTESIAN_POINT('Ctrl Pts',(3.69717970712967,1.9804354328423,-32.9254409187843)) ;
#168873=CARTESIAN_POINT('Ctrl Pts',(3.69541014605544,1.97847095301992,-32.9228241208443)) ;
#168874=CARTESIAN_POINT('Ctrl Pts',(3.69146029518774,1.97457001268156,-32.917973443509)) ;
#168875=CARTESIAN_POINT('Ctrl Pts',(3.6891543679041,1.97254004967205,-32.9156322068765)) ;
#168876=CARTESIAN_POINT('Ctrl Pts',(3.68263623161782,1.96688850447172,-32.9094999184567)) ;
#168877=CARTESIAN_POINT('Ctrl Pts',(3.6779666138314,1.96321337091297,-32.9059792522829)) ;
#168878=CARTESIAN_POINT('Ctrl Pts',(3.67279117399658,1.95950210067462,-32.9027623433944)) ;
#168879=CARTESIAN_POINT('Ctrl Pts',(3.67252519027984,1.95931231248676,-32.9025988090581)) ;
#168880=CARTESIAN_POINT('Ctrl Pts',(3.6693311210617,1.95704457126181,-32.9006562043068)) ;
#168881=CARTESIAN_POINT('Ctrl Pts',(3.66628216680076,1.95498580453518,-32.8990096122391)) ;
#168882=CARTESIAN_POINT('Ctrl Pts',(3.65739884032377,1.94929644648108,-32.8947590242123)) ;
#168883=CARTESIAN_POINT('Ctrl Pts',(3.65126071410426,1.94574201114262,-32.8924711332688)) ;
#168884=CARTESIAN_POINT('Ctrl Pts',(3.64132315686417,1.94068746317946,-32.8896379659013)) ;
#168885=CARTESIAN_POINT('Ctrl Pts',(3.63763353946351,1.93894751340588,-32.8887565993848)) ;
#168886=CARTESIAN_POINT('Ctrl Pts',(3.62813871250328,1.93486114467731,-32.8869043913581)) ;
#168887=CARTESIAN_POINT('Ctrl Pts',(3.62220485293027,1.93266004719387,-32.8861153440415)) ;
#168888=CARTESIAN_POINT('Ctrl Pts',(3.61359543742306,1.93003167234279,-32.8854202174511)) ;
#168889=CARTESIAN_POINT('Ctrl Pts',(3.61101642176932,1.92931331154692,-32.8852669825531)) ;
#168890=CARTESIAN_POINT('Ctrl Pts',(3.60562851963555,1.92796119665925,-32.8850532567727)) ;
#168891=CARTESIAN_POINT('Ctrl Pts',(3.60282089026094,1.92733781012832,-32.885)) ;
#168892=CARTESIAN_POINT('Ctrl Pts',(3.6,1.92679491924311,-32.885)) ;
#168893=CARTESIAN_POINT('Origin',(3.6,1.9,-32.985)) ;
#168894=CARTESIAN_POINT('Origin',(3.7,1.9,-32.985)) ;
#168895=CARTESIAN_POINT('Origin',(10.1,1.9,-32.985)) ;
#168896=CARTESIAN_POINT('Origin',(10.1,1.9,-32.985)) ;
#168897=CARTESIAN_POINT('Origin',(3.7,1.9,-5.115)) ;
#168898=CARTESIAN_POINT('Origin',(3.7,2.07320508075689,-5.215)) ;
#168899=CARTESIAN_POINT('Ctrl Pts',(3.60000659411846,1.92678349789492,-5.21500000086965)) ;
#168900=CARTESIAN_POINT('Ctrl Pts',(3.55,2.01339745962155,-5.21498681089333)) ;
#168901=CARTESIAN_POINT('Ctrl Pts',(3.55,2.01339745962156,-5.315)) ;
#168902=CARTESIAN_POINT('Ctrl Pts',(3.61192169694494,1.92907674455598,-5.2150005173338)) ;
#168903=CARTESIAN_POINT('Ctrl Pts',(3.55199190475225,2.01454315814794,-5.21100027733256)) ;
#168904=CARTESIAN_POINT('Ctrl Pts',(3.55795064586848,2.01798776715396,-5.31499562155023)) ;
#168905=CARTESIAN_POINT('Ctrl Pts',(3.62341406508538,1.93280912529606,-5.2140249033077)) ;
#168906=CARTESIAN_POINT('Ctrl Pts',(3.55602946562208,2.0107204129829,-5.20668983076589)) ;
#168907=CARTESIAN_POINT('Ctrl Pts',(3.56528619664567,2.02370799306987,-5.30863885617463)) ;
#168908=CARTESIAN_POINT('Ctrl Pts',(3.64447698054259,1.94188479470202,-5.20990697186185)) ;
#168909=CARTESIAN_POINT('Ctrl Pts',(3.56481337003729,2.00521659408681,-5.19818874066451)) ;
#168910=CARTESIAN_POINT('Ctrl Pts',(3.5778513142626,2.03528605841761,-5.29516115437405)) ;
#168911=CARTESIAN_POINT('Ctrl Pts',(3.65434383600069,1.94732274903781,-5.20671544038559)) ;
#168912=CARTESIAN_POINT('Ctrl Pts',(3.56964037752544,2.00254785926568,-5.19373800427673)) ;
#168913=CARTESIAN_POINT('Ctrl Pts',(3.58324299321411,2.04133793352501,-5.2870289695647)) ;
#168914=CARTESIAN_POINT('Ctrl Pts',(3.67209270719133,1.95869361548257,-5.1982138841634)) ;
#168915=CARTESIAN_POINT('Ctrl Pts',(3.57877657372946,1.99742369139614,-5.18460192490956)) ;
#168916=CARTESIAN_POINT('Ctrl Pts',(3.59173571364126,2.05270412132581,-5.26927384501021)) ;
#168917=CARTESIAN_POINT('Ctrl Pts',(3.68022412057907,1.96474917806412,-5.19281520426601)) ;
#168918=CARTESIAN_POINT('Ctrl Pts',(3.58322866085249,1.9947527117803,-5.17977362629675)) ;
#168919=CARTESIAN_POINT('Ctrl Pts',(3.59492343714209,2.05814036366738,-5.259399963424)) ;
#168920=CARTESIAN_POINT('Ctrl Pts',(3.693683649568,1.97632149420531,-5.18024886281709)) ;
#168921=CARTESIAN_POINT('Ctrl Pts',(3.59172551342568,1.98925228662578,-5.17099928071624)) ;
#168922=CARTESIAN_POINT('Ctrl Pts',(3.59903094645825,2.06720241143976,-5.23834396451164)) ;
#168923=CARTESIAN_POINT('Ctrl Pts',(3.70000914724963,1.98195813651218,-5.17304434431451)) ;
#168924=CARTESIAN_POINT('Ctrl Pts',(3.59596384548937,1.98543049140365,-5.16700954448628)) ;
#168925=CARTESIAN_POINT('Ctrl Pts',(3.6,2.07088547209221,-5.22705281147587)) ;
#168926=CARTESIAN_POINT('Ctrl Pts',(3.70001318823691,1.98660254113158,-5.16500000043482)) ;
#168927=CARTESIAN_POINT('Ctrl Pts',(3.6,1.98659111827701,-5.16499340544667)) ;
#168928=CARTESIAN_POINT('Ctrl Pts',(3.6,2.07320508075689,-5.215)) ;
#168929=CARTESIAN_POINT('Origin',(3.6,1.92679491924311,-5.315)) ;
#168930=CARTESIAN_POINT('Origin',(3.5,2.1,-5.315)) ;
#168931=CARTESIAN_POINT('Origin',(3.7,1.9,-2.505)) ;
#168932=CARTESIAN_POINT('Origin',(3.7,2.07320508075689,-2.405)) ;
#168933=CARTESIAN_POINT('Ctrl Pts',(3.70000000000001,1.98660254037844,-2.455)) ;
#168934=CARTESIAN_POINT('Ctrl Pts',(3.59998681089333,1.98660254037844,-2.455)) ;
#168935=CARTESIAN_POINT('Ctrl Pts',(3.60000000086965,2.07321650210508,-2.40499340588155)) ;
#168936=CARTESIAN_POINT('Ctrl Pts',(3.69999562155021,1.98201223284605,-2.44704935413152)) ;
#168937=CARTESIAN_POINT('Ctrl Pts',(3.59600027733255,1.98545684185207,-2.45300809524776)) ;
#168938=CARTESIAN_POINT('Ctrl Pts',(3.60000051733381,2.07092325544402,-2.39307830305507)) ;
#168939=CARTESIAN_POINT('Ctrl Pts',(3.69363885617462,1.97629200693012,-2.43971380335433)) ;
#168940=CARTESIAN_POINT('Ctrl Pts',(3.59168983076591,1.98927958701711,-2.44897053437792)) ;
#168941=CARTESIAN_POINT('Ctrl Pts',(3.5990249033077,2.06719087470394,-2.38158593491462)) ;
#168942=CARTESIAN_POINT('Ctrl Pts',(3.68016115437407,1.9647139415824,-2.42714868573741)) ;
#168943=CARTESIAN_POINT('Ctrl Pts',(3.58318874066451,1.99478340591318,-2.44018662996272)) ;
#168944=CARTESIAN_POINT('Ctrl Pts',(3.59490697186185,2.05811520529797,-2.36052301945742)) ;
#168945=CARTESIAN_POINT('Ctrl Pts',(3.6720289695647,1.95866206647499,-2.42175700678589)) ;
#168946=CARTESIAN_POINT('Ctrl Pts',(3.57873800427671,1.99745214073432,-2.43535962247455)) ;
#168947=CARTESIAN_POINT('Ctrl Pts',(3.59171544038559,2.05267725096218,-2.35065616399931)) ;
#168948=CARTESIAN_POINT('Ctrl Pts',(3.6542738450102,1.94729587867419,-2.41326428635874)) ;
#168949=CARTESIAN_POINT('Ctrl Pts',(3.56960192490958,2.00257630860386,-2.42622342627056)) ;
#168950=CARTESIAN_POINT('Ctrl Pts',(3.5832138841634,2.04130638451743,-2.33290729280868)) ;
#168951=CARTESIAN_POINT('Ctrl Pts',(3.644399963424,1.94185963633262,-2.41007656285791)) ;
#168952=CARTESIAN_POINT('Ctrl Pts',(3.56477362629675,2.0052472882197,-2.42177133914751)) ;
#168953=CARTESIAN_POINT('Ctrl Pts',(3.57781520426602,2.03525082193588,-2.32477587942094)) ;
#168954=CARTESIAN_POINT('Ctrl Pts',(3.62334396451165,1.93279758856024,-2.40596905354176)) ;
#168955=CARTESIAN_POINT('Ctrl Pts',(3.55599928071625,2.01074771337423,-2.41327448657433)) ;
#168956=CARTESIAN_POINT('Ctrl Pts',(3.5652488628171,2.02367850579469,-2.311316350432)) ;
#168957=CARTESIAN_POINT('Ctrl Pts',(3.61205281147587,1.9291145279078,-2.405)) ;
#168958=CARTESIAN_POINT('Ctrl Pts',(3.55200954448627,2.01456950859635,-2.40903615451063)) ;
#168959=CARTESIAN_POINT('Ctrl Pts',(3.55804434431452,2.01804186348783,-2.30499085275037)) ;
#168960=CARTESIAN_POINT('Ctrl Pts',(3.6,1.92679491924311,-2.405)) ;
#168961=CARTESIAN_POINT('Ctrl Pts',(3.54999340544667,2.01340888172299,-2.405)) ;
#168962=CARTESIAN_POINT('Ctrl Pts',(3.55000000043483,2.01339745886842,-2.30498681176309)) ;
#168963=CARTESIAN_POINT('Origin',(3.6,1.92679491924311,-2.305)) ;
#168964=CARTESIAN_POINT('Origin',(3.5,2.1,-2.305)) ;
#168965=CARTESIAN_POINT('Origin',(3.7,1.9,-8.925)) ;
#168966=CARTESIAN_POINT('Origin',(3.7,2.07320508075689,-9.025)) ;
#168967=CARTESIAN_POINT('Ctrl Pts',(3.60000659411846,1.92678349789492,-9.02500000086965)) ;
#168968=CARTESIAN_POINT('Ctrl Pts',(3.55,2.01339745962157,-9.02498681089333)) ;
#168969=CARTESIAN_POINT('Ctrl Pts',(3.55,2.01339745962156,-9.12500000000001)) ;
#168970=CARTESIAN_POINT('Ctrl Pts',(3.61192169694494,1.92907674455598,-9.02500051733381)) ;
#168971=CARTESIAN_POINT('Ctrl Pts',(3.5519919047523,2.0145431581478,-9.02100027733252)) ;
#168972=CARTESIAN_POINT('Ctrl Pts',(3.55795064586849,2.01798776715396,-9.12499562155005)) ;
#168973=CARTESIAN_POINT('Ctrl Pts',(3.62341406508537,1.93280912529606,-9.0240249033077)) ;
#168974=CARTESIAN_POINT('Ctrl Pts',(3.55602946562208,2.0107204129829,-9.01668983076591)) ;
#168975=CARTESIAN_POINT('Ctrl Pts',(3.56528619664567,2.02370799306987,-9.11863885617463)) ;
#168976=CARTESIAN_POINT('Ctrl Pts',(3.64447698054259,1.94188479470202,-9.01990697186185)) ;
#168977=CARTESIAN_POINT('Ctrl Pts',(3.56481337003728,2.00521659408682,-9.00818874066449)) ;
#168978=CARTESIAN_POINT('Ctrl Pts',(3.5778513142626,2.03528605841761,-9.10516115437406)) ;
#168979=CARTESIAN_POINT('Ctrl Pts',(3.65434383600069,1.94732274903781,-9.01671544038559)) ;
#168980=CARTESIAN_POINT('Ctrl Pts',(3.56964037752546,2.00254785926568,-9.00373800427673)) ;
#168981=CARTESIAN_POINT('Ctrl Pts',(3.58324299321411,2.041337933525,-9.0970289695647)) ;
#168982=CARTESIAN_POINT('Ctrl Pts',(3.67209270719133,1.95869361548257,-9.0082138841634)) ;
#168983=CARTESIAN_POINT('Ctrl Pts',(3.57877657372944,1.99742369139614,-8.99460192490956)) ;
#168984=CARTESIAN_POINT('Ctrl Pts',(3.59173571364126,2.05270412132582,-9.07927384501021)) ;
#168985=CARTESIAN_POINT('Ctrl Pts',(3.68022412057907,1.96474917806412,-9.00281520426602)) ;
#168986=CARTESIAN_POINT('Ctrl Pts',(3.58322866085248,1.9947527117803,-8.98977362629674)) ;
#168987=CARTESIAN_POINT('Ctrl Pts',(3.59492343714209,2.05814036366738,-9.069399963424)) ;
#168988=CARTESIAN_POINT('Ctrl Pts',(3.693683649568,1.97632149420531,-8.9902488628171)) ;
#168989=CARTESIAN_POINT('Ctrl Pts',(3.59172551342568,1.98925228662577,-8.98099928071626)) ;
#168990=CARTESIAN_POINT('Ctrl Pts',(3.59903094645824,2.06720241143976,-9.04834396451164)) ;
#168991=CARTESIAN_POINT('Ctrl Pts',(3.70000914724963,1.98195813651218,-8.98304434431452)) ;
#168992=CARTESIAN_POINT('Ctrl Pts',(3.59596384548939,1.98543049140367,-8.97700954448631)) ;
#168993=CARTESIAN_POINT('Ctrl Pts',(3.6,2.07088547209221,-9.03705281147587)) ;
#168994=CARTESIAN_POINT('Ctrl Pts',(3.70001318823691,1.98660254113158,-8.97500000043482)) ;
#168995=CARTESIAN_POINT('Ctrl Pts',(3.6,1.98659111827701,-8.97499340544666)) ;
#168996=CARTESIAN_POINT('Ctrl Pts',(3.6,2.07320508075689,-9.025)) ;
#168997=CARTESIAN_POINT('Origin',(3.6,1.92679491924311,-9.125)) ;
#168998=CARTESIAN_POINT('Origin',(3.5,2.1,-9.125)) ;
#168999=CARTESIAN_POINT('Origin',(3.7,1.9,-6.315)) ;
#169000=CARTESIAN_POINT('Origin',(3.7,2.07320508075689,-6.215)) ;
#169001=CARTESIAN_POINT('Ctrl Pts',(3.70000000000001,1.98660254037844,-6.265)) ;
#169002=CARTESIAN_POINT('Ctrl Pts',(3.59998681089333,1.98660254037844,-6.265)) ;
#169003=CARTESIAN_POINT('Ctrl Pts',(3.60000000086965,2.07321650210508,-6.21499340588155)) ;
#169004=CARTESIAN_POINT('Ctrl Pts',(3.69999562155021,1.98201223284604,-6.25704935413151)) ;
#169005=CARTESIAN_POINT('Ctrl Pts',(3.59600027733256,1.98545684185207,-6.26300809524773)) ;
#169006=CARTESIAN_POINT('Ctrl Pts',(3.60000051733381,2.07092325544402,-6.20307830305506)) ;
#169007=CARTESIAN_POINT('Ctrl Pts',(3.69363885617462,1.97629200693013,-6.24971380335433)) ;
#169008=CARTESIAN_POINT('Ctrl Pts',(3.59168983076591,1.98927958701711,-6.25897053437793)) ;
#169009=CARTESIAN_POINT('Ctrl Pts',(3.5990249033077,2.06719087470393,-6.19158593491463)) ;
#169010=CARTESIAN_POINT('Ctrl Pts',(3.68016115437407,1.96471394158239,-6.2371486857374)) ;
#169011=CARTESIAN_POINT('Ctrl Pts',(3.58318874066451,1.99478340591318,-6.25018662996271)) ;
#169012=CARTESIAN_POINT('Ctrl Pts',(3.59490697186185,2.05811520529798,-6.17052301945741)) ;
#169013=CARTESIAN_POINT('Ctrl Pts',(3.67202896956471,1.95866206647499,-6.23175700678589)) ;
#169014=CARTESIAN_POINT('Ctrl Pts',(3.57873800427672,1.99745214073432,-6.24535962247454)) ;
#169015=CARTESIAN_POINT('Ctrl Pts',(3.59171544038559,2.05267725096218,-6.16065616399931)) ;
#169016=CARTESIAN_POINT('Ctrl Pts',(3.6542738450102,1.94729587867419,-6.22326428635874)) ;
#169017=CARTESIAN_POINT('Ctrl Pts',(3.56960192490958,2.00257630860386,-6.23622342627057)) ;
#169018=CARTESIAN_POINT('Ctrl Pts',(3.5832138841634,2.04130638451743,-6.14290729280868)) ;
#169019=CARTESIAN_POINT('Ctrl Pts',(3.644399963424,1.94185963633262,-6.22007656285791)) ;
#169020=CARTESIAN_POINT('Ctrl Pts',(3.56477362629674,2.0052472882197,-6.23177133914752)) ;
#169021=CARTESIAN_POINT('Ctrl Pts',(3.57781520426601,2.03525082193588,-6.13477587942094)) ;
#169022=CARTESIAN_POINT('Ctrl Pts',(3.62334396451165,1.93279758856024,-6.21596905354176)) ;
#169023=CARTESIAN_POINT('Ctrl Pts',(3.55599928071626,2.01074771337422,-6.22327448657432)) ;
#169024=CARTESIAN_POINT('Ctrl Pts',(3.5652488628171,2.02367850579469,-6.121316350432)) ;
#169025=CARTESIAN_POINT('Ctrl Pts',(3.61205281147587,1.9291145279078,-6.215)) ;
#169026=CARTESIAN_POINT('Ctrl Pts',(3.55200954448627,2.01456950859637,-6.21903615451063)) ;
#169027=CARTESIAN_POINT('Ctrl Pts',(3.55804434431452,2.01804186348782,-6.11499085275031)) ;
#169028=CARTESIAN_POINT('Ctrl Pts',(3.6,1.92679491924311,-6.215)) ;
#169029=CARTESIAN_POINT('Ctrl Pts',(3.54999340544667,2.01340888172298,-6.215)) ;
#169030=CARTESIAN_POINT('Ctrl Pts',(3.55000000043483,2.01339745886842,-6.1149868117631)) ;
#169031=CARTESIAN_POINT('Origin',(3.6,1.92679491924311,-6.115)) ;
#169032=CARTESIAN_POINT('Origin',(3.5,2.1,-6.115)) ;
#169033=CARTESIAN_POINT('Origin',(3.7,1.9,-12.735)) ;
#169034=CARTESIAN_POINT('Origin',(3.7,2.07320508075689,-12.835)) ;
#169035=CARTESIAN_POINT('Ctrl Pts',(3.60000659411846,1.92678349789492,-12.8350000008696)) ;
#169036=CARTESIAN_POINT('Ctrl Pts',(3.55,2.01339745962156,-12.8349868108933)) ;
#169037=CARTESIAN_POINT('Ctrl Pts',(3.55,2.01339745962156,-12.935)) ;
#169038=CARTESIAN_POINT('Ctrl Pts',(3.61192169694494,1.92907674455598,-12.8350005173338)) ;
#169039=CARTESIAN_POINT('Ctrl Pts',(3.55199190475231,2.01454315814779,-12.8310002773325)) ;
#169040=CARTESIAN_POINT('Ctrl Pts',(3.55795064586849,2.01798776715396,-12.93499562155)) ;
#169041=CARTESIAN_POINT('Ctrl Pts',(3.62341406508537,1.93280912529606,-12.8340249033077)) ;
#169042=CARTESIAN_POINT('Ctrl Pts',(3.55602946562208,2.01072041298289,-12.8266898307659)) ;
#169043=CARTESIAN_POINT('Ctrl Pts',(3.56528619664567,2.02370799306987,-12.9286388561746)) ;
#169044=CARTESIAN_POINT('Ctrl Pts',(3.64447698054259,1.94188479470202,-12.8299069718618)) ;
#169045=CARTESIAN_POINT('Ctrl Pts',(3.56481337003728,2.00521659408682,-12.8181887406645)) ;
#169046=CARTESIAN_POINT('Ctrl Pts',(3.5778513142626,2.03528605841761,-12.9151611543741)) ;
#169047=CARTESIAN_POINT('Ctrl Pts',(3.6543438360007,1.94732274903782,-12.8267154403856)) ;
#169048=CARTESIAN_POINT('Ctrl Pts',(3.56964037752546,2.00254785926569,-12.8137380042767)) ;
#169049=CARTESIAN_POINT('Ctrl Pts',(3.58324299321411,2.04133793352501,-12.9070289695647)) ;
#169050=CARTESIAN_POINT('Ctrl Pts',(3.67209270719132,1.95869361548257,-12.8182138841634)) ;
#169051=CARTESIAN_POINT('Ctrl Pts',(3.57877657372944,1.99742369139614,-12.8046019249096)) ;
#169052=CARTESIAN_POINT('Ctrl Pts',(3.59173571364126,2.05270412132581,-12.8892738450102)) ;
#169053=CARTESIAN_POINT('Ctrl Pts',(3.68022412057907,1.96474917806412,-12.812815204266)) ;
#169054=CARTESIAN_POINT('Ctrl Pts',(3.58322866085248,1.9947527117803,-12.7997736262967)) ;
#169055=CARTESIAN_POINT('Ctrl Pts',(3.59492343714209,2.05814036366738,-12.879399963424)) ;
#169056=CARTESIAN_POINT('Ctrl Pts',(3.693683649568,1.97632149420531,-12.8002488628171)) ;
#169057=CARTESIAN_POINT('Ctrl Pts',(3.59172551342568,1.98925228662577,-12.7909992807163)) ;
#169058=CARTESIAN_POINT('Ctrl Pts',(3.59903094645824,2.06720241143976,-12.8583439645117)) ;
#169059=CARTESIAN_POINT('Ctrl Pts',(3.70000914724963,1.98195813651218,-12.7930443443145)) ;
#169060=CARTESIAN_POINT('Ctrl Pts',(3.59596384548936,1.98543049140367,-12.7870095444862)) ;
#169061=CARTESIAN_POINT('Ctrl Pts',(3.6,2.07088547209221,-12.8470528114759)) ;
#169062=CARTESIAN_POINT('Ctrl Pts',(3.70001318823691,1.98660254113158,-12.7850000004348)) ;
#169063=CARTESIAN_POINT('Ctrl Pts',(3.6,1.98659111827701,-12.7849934054467)) ;
#169064=CARTESIAN_POINT('Ctrl Pts',(3.6,2.07320508075689,-12.835)) ;
#169065=CARTESIAN_POINT('Origin',(3.6,1.92679491924311,-12.935)) ;
#169066=CARTESIAN_POINT('Origin',(3.5,2.1,-12.935)) ;
#169067=CARTESIAN_POINT('Origin',(3.7,1.9,-10.125)) ;
#169068=CARTESIAN_POINT('Origin',(3.7,2.07320508075689,-10.025)) ;
#169069=CARTESIAN_POINT('Ctrl Pts',(3.70000000000001,1.98660254037844,-10.075)) ;
#169070=CARTESIAN_POINT('Ctrl Pts',(3.59998681089332,1.98660254037844,-10.075)) ;
#169071=CARTESIAN_POINT('Ctrl Pts',(3.60000000086965,2.07321650210509,-10.0249934058815)) ;
#169072=CARTESIAN_POINT('Ctrl Pts',(3.69999562155021,1.98201223284604,-10.0670493541315)) ;
#169073=CARTESIAN_POINT('Ctrl Pts',(3.59600027733253,1.98545684185205,-10.0730080952478)) ;
#169074=CARTESIAN_POINT('Ctrl Pts',(3.60000051733381,2.07092325544401,-10.0130783030551)) ;
#169075=CARTESIAN_POINT('Ctrl Pts',(3.69363885617462,1.97629200693013,-10.0597138033543)) ;
#169076=CARTESIAN_POINT('Ctrl Pts',(3.5916898307659,1.98927958701711,-10.0689705343779)) ;
#169077=CARTESIAN_POINT('Ctrl Pts',(3.59902490330771,2.06719087470394,-10.0015859349146)) ;
#169078=CARTESIAN_POINT('Ctrl Pts',(3.68016115437407,1.96471394158239,-10.0471486857374)) ;
#169079=CARTESIAN_POINT('Ctrl Pts',(3.58318874066448,1.99478340591319,-10.0601866299627)) ;
#169080=CARTESIAN_POINT('Ctrl Pts',(3.59490697186185,2.05811520529799,-9.98052301945739)) ;
#169081=CARTESIAN_POINT('Ctrl Pts',(3.67202896956471,1.958662066475,-10.0417570067859)) ;
#169082=CARTESIAN_POINT('Ctrl Pts',(3.57873800427672,1.99745214073432,-10.0553596224746)) ;
#169083=CARTESIAN_POINT('Ctrl Pts',(3.5917154403856,2.05267725096219,-9.97065616399932)) ;
#169084=CARTESIAN_POINT('Ctrl Pts',(3.6542738450102,1.94729587867418,-10.0332642863587)) ;
#169085=CARTESIAN_POINT('Ctrl Pts',(3.56960192490955,2.00257630860387,-10.0462234262705)) ;
#169086=CARTESIAN_POINT('Ctrl Pts',(3.5832138841634,2.04130638451744,-9.95290729280864)) ;
#169087=CARTESIAN_POINT('Ctrl Pts',(3.644399963424,1.94185963633262,-10.0300765628579)) ;
#169088=CARTESIAN_POINT('Ctrl Pts',(3.56477362629674,2.00524728821971,-10.0417713391475)) ;
#169089=CARTESIAN_POINT('Ctrl Pts',(3.57781520426602,2.03525082193588,-9.94477587942092)) ;
#169090=CARTESIAN_POINT('Ctrl Pts',(3.62334396451165,1.93279758856024,-10.0259690535418)) ;
#169091=CARTESIAN_POINT('Ctrl Pts',(3.55599928071624,2.01074771337424,-10.0332744865743)) ;
#169092=CARTESIAN_POINT('Ctrl Pts',(3.5652488628171,2.0236785057947,-9.93131635043199)) ;
#169093=CARTESIAN_POINT('Ctrl Pts',(3.61205281147587,1.9291145279078,-10.025)) ;
#169094=CARTESIAN_POINT('Ctrl Pts',(3.55200954448624,2.01456950859637,-10.0290361545106)) ;
#169095=CARTESIAN_POINT('Ctrl Pts',(3.55804434431452,2.01804186348782,-9.92499085275035)) ;
#169096=CARTESIAN_POINT('Ctrl Pts',(3.6,1.92679491924311,-10.025)) ;
#169097=CARTESIAN_POINT('Ctrl Pts',(3.54999340544666,2.013408881723,-10.025)) ;
#169098=CARTESIAN_POINT('Ctrl Pts',(3.55000000043483,2.01339745886842,-9.92498681176308)) ;
#169099=CARTESIAN_POINT('Origin',(3.6,1.92679491924311,-9.925)) ;
#169100=CARTESIAN_POINT('Origin',(3.5,2.1,-9.925)) ;
#169101=CARTESIAN_POINT('Origin',(3.7,1.9,-16.545)) ;
#169102=CARTESIAN_POINT('Origin',(3.7,2.07320508075689,-16.645)) ;
#169103=CARTESIAN_POINT('Ctrl Pts',(3.60000659411846,1.92678349789492,-16.6450000008696)) ;
#169104=CARTESIAN_POINT('Ctrl Pts',(3.55,2.01339745962156,-16.6449868108933)) ;
#169105=CARTESIAN_POINT('Ctrl Pts',(3.55,2.01339745962156,-16.745)) ;
#169106=CARTESIAN_POINT('Ctrl Pts',(3.61192169694494,1.92907674455598,-16.6450005173338)) ;
#169107=CARTESIAN_POINT('Ctrl Pts',(3.55199190475217,2.0145431581481,-16.6410002773326)) ;
#169108=CARTESIAN_POINT('Ctrl Pts',(3.55795064586847,2.01798776715395,-16.7449956215505)) ;
#169109=CARTESIAN_POINT('Ctrl Pts',(3.62341406508538,1.93280912529606,-16.6440249033077)) ;
#169110=CARTESIAN_POINT('Ctrl Pts',(3.55602946562207,2.0107204129829,-16.6366898307659)) ;
#169111=CARTESIAN_POINT('Ctrl Pts',(3.56528619664567,2.02370799306988,-16.7386388561746)) ;
#169112=CARTESIAN_POINT('Ctrl Pts',(3.64447698054259,1.94188479470202,-16.6399069718619)) ;
#169113=CARTESIAN_POINT('Ctrl Pts',(3.56481337003729,2.00521659408681,-16.6281887406645)) ;
#169114=CARTESIAN_POINT('Ctrl Pts',(3.5778513142626,2.0352860584176,-16.725161154374)) ;
#169115=CARTESIAN_POINT('Ctrl Pts',(3.65434383600069,1.94732274903783,-16.6367154403856)) ;
#169116=CARTESIAN_POINT('Ctrl Pts',(3.56964037752545,2.00254785926569,-16.6237380042767)) ;
#169117=CARTESIAN_POINT('Ctrl Pts',(3.58324299321411,2.04133793352501,-16.7170289695647)) ;
#169118=CARTESIAN_POINT('Ctrl Pts',(3.67209270719133,1.95869361548256,-16.6282138841634)) ;
#169119=CARTESIAN_POINT('Ctrl Pts',(3.57877657372945,1.99742369139614,-16.6146019249096)) ;
#169120=CARTESIAN_POINT('Ctrl Pts',(3.59173571364127,2.05270412132582,-16.6992738450102)) ;
#169121=CARTESIAN_POINT('Ctrl Pts',(3.68022412057906,1.96474917806413,-16.622815204266)) ;
#169122=CARTESIAN_POINT('Ctrl Pts',(3.58322866085249,1.99475271178031,-16.6097736262967)) ;
#169123=CARTESIAN_POINT('Ctrl Pts',(3.59492343714209,2.05814036366738,-16.689399963424)) ;
#169124=CARTESIAN_POINT('Ctrl Pts',(3.69368364956801,1.9763214942053,-16.6102488628171)) ;
#169125=CARTESIAN_POINT('Ctrl Pts',(3.59172551342567,1.98925228662577,-16.6009992807163)) ;
#169126=CARTESIAN_POINT('Ctrl Pts',(3.59903094645825,2.06720241143977,-16.6683439645117)) ;
#169127=CARTESIAN_POINT('Ctrl Pts',(3.70000914724963,1.98195813651218,-16.6030443443145)) ;
#169128=CARTESIAN_POINT('Ctrl Pts',(3.59596384548934,1.9854304914036,-16.5970095444861)) ;
#169129=CARTESIAN_POINT('Ctrl Pts',(3.6,2.07088547209219,-16.6570528114759)) ;
#169130=CARTESIAN_POINT('Ctrl Pts',(3.70001318823691,1.98660254113158,-16.5950000004348)) ;
#169131=CARTESIAN_POINT('Ctrl Pts',(3.6,1.98659111827702,-16.5949934054467)) ;
#169132=CARTESIAN_POINT('Ctrl Pts',(3.6,2.07320508075689,-16.645)) ;
#169133=CARTESIAN_POINT('Origin',(3.6,1.92679491924311,-16.745)) ;
#169134=CARTESIAN_POINT('Origin',(3.5,2.1,-16.745)) ;
#169135=CARTESIAN_POINT('Origin',(3.7,1.9,-13.935)) ;
#169136=CARTESIAN_POINT('Origin',(3.7,2.07320508075689,-13.835)) ;
#169137=CARTESIAN_POINT('Ctrl Pts',(3.70000000000001,1.98660254037844,-13.885)) ;
#169138=CARTESIAN_POINT('Ctrl Pts',(3.59998681089332,1.98660254037844,-13.885)) ;
#169139=CARTESIAN_POINT('Ctrl Pts',(3.60000000086965,2.07321650210509,-13.8349934058815)) ;
#169140=CARTESIAN_POINT('Ctrl Pts',(3.69999562155021,1.98201223284604,-13.8770493541315)) ;
#169141=CARTESIAN_POINT('Ctrl Pts',(3.59600027733253,1.98545684185205,-13.8830080952478)) ;
#169142=CARTESIAN_POINT('Ctrl Pts',(3.60000051733381,2.07092325544401,-13.823078303055)) ;
#169143=CARTESIAN_POINT('Ctrl Pts',(3.69363885617462,1.97629200693013,-13.8697138033543)) ;
#169144=CARTESIAN_POINT('Ctrl Pts',(3.5916898307659,1.98927958701711,-13.8789705343779)) ;
#169145=CARTESIAN_POINT('Ctrl Pts',(3.59902490330771,2.06719087470394,-13.8115859349146)) ;
#169146=CARTESIAN_POINT('Ctrl Pts',(3.68016115437407,1.96471394158239,-13.8571486857374)) ;
#169147=CARTESIAN_POINT('Ctrl Pts',(3.58318874066448,1.99478340591319,-13.8701866299627)) ;
#169148=CARTESIAN_POINT('Ctrl Pts',(3.59490697186185,2.05811520529799,-13.7905230194574)) ;
#169149=CARTESIAN_POINT('Ctrl Pts',(3.67202896956471,1.958662066475,-13.8517570067859)) ;
#169150=CARTESIAN_POINT('Ctrl Pts',(3.57873800427673,1.99745214073432,-13.8653596224746)) ;
#169151=CARTESIAN_POINT('Ctrl Pts',(3.5917154403856,2.05267725096219,-13.7806561639993)) ;
#169152=CARTESIAN_POINT('Ctrl Pts',(3.6542738450102,1.94729587867418,-13.8432642863587)) ;
#169153=CARTESIAN_POINT('Ctrl Pts',(3.56960192490954,2.00257630860387,-13.8562234262705)) ;
#169154=CARTESIAN_POINT('Ctrl Pts',(3.5832138841634,2.04130638451744,-13.7629072928086)) ;
#169155=CARTESIAN_POINT('Ctrl Pts',(3.644399963424,1.94185963633262,-13.8400765628579)) ;
#169156=CARTESIAN_POINT('Ctrl Pts',(3.56477362629673,2.00524728821971,-13.8517713391475)) ;
#169157=CARTESIAN_POINT('Ctrl Pts',(3.57781520426602,2.03525082193588,-13.7547758794209)) ;
#169158=CARTESIAN_POINT('Ctrl Pts',(3.62334396451165,1.93279758856024,-13.8359690535418)) ;
#169159=CARTESIAN_POINT('Ctrl Pts',(3.55599928071625,2.01074771337423,-13.8432744865743)) ;
#169160=CARTESIAN_POINT('Ctrl Pts',(3.5652488628171,2.0236785057947,-13.741316350432)) ;
#169161=CARTESIAN_POINT('Ctrl Pts',(3.61205281147587,1.9291145279078,-13.835)) ;
#169162=CARTESIAN_POINT('Ctrl Pts',(3.55200954448628,2.01456950859631,-13.8390361545106)) ;
#169163=CARTESIAN_POINT('Ctrl Pts',(3.55804434431452,2.01804186348783,-13.7349908527504)) ;
#169164=CARTESIAN_POINT('Ctrl Pts',(3.6,1.92679491924311,-13.835)) ;
#169165=CARTESIAN_POINT('Ctrl Pts',(3.54999340544666,2.013408881723,-13.835)) ;
#169166=CARTESIAN_POINT('Ctrl Pts',(3.55000000043483,2.01339745886842,-13.7349868117631)) ;
#169167=CARTESIAN_POINT('Origin',(3.6,1.92679491924311,-13.735)) ;
#169168=CARTESIAN_POINT('Origin',(3.5,2.1,-13.735)) ;
#169169=CARTESIAN_POINT('Origin',(3.7,1.9,-20.355)) ;
#169170=CARTESIAN_POINT('Origin',(3.7,2.07320508075689,-20.455)) ;
#169171=CARTESIAN_POINT('Ctrl Pts',(3.60000659411846,1.92678349789492,-20.4550000008697)) ;
#169172=CARTESIAN_POINT('Ctrl Pts',(3.55,2.01339745962156,-20.4549868108933)) ;
#169173=CARTESIAN_POINT('Ctrl Pts',(3.55,2.01339745962156,-20.555)) ;
#169174=CARTESIAN_POINT('Ctrl Pts',(3.61192169694493,1.92907674455598,-20.4550005173338)) ;
#169175=CARTESIAN_POINT('Ctrl Pts',(3.55199190475217,2.0145431581481,-20.4510002773326)) ;
#169176=CARTESIAN_POINT('Ctrl Pts',(3.55795064586847,2.01798776715395,-20.5549956215505)) ;
#169177=CARTESIAN_POINT('Ctrl Pts',(3.62341406508538,1.93280912529606,-20.4540249033077)) ;
#169178=CARTESIAN_POINT('Ctrl Pts',(3.55602946562207,2.0107204129829,-20.4466898307659)) ;
#169179=CARTESIAN_POINT('Ctrl Pts',(3.56528619664567,2.02370799306988,-20.5486388561746)) ;
#169180=CARTESIAN_POINT('Ctrl Pts',(3.64447698054259,1.94188479470202,-20.4499069718619)) ;
#169181=CARTESIAN_POINT('Ctrl Pts',(3.56481337003729,2.00521659408681,-20.4381887406645)) ;
#169182=CARTESIAN_POINT('Ctrl Pts',(3.5778513142626,2.0352860584176,-20.5351611543741)) ;
#169183=CARTESIAN_POINT('Ctrl Pts',(3.65434383600069,1.94732274903783,-20.4467154403856)) ;
#169184=CARTESIAN_POINT('Ctrl Pts',(3.56964037752545,2.00254785926569,-20.4337380042767)) ;
#169185=CARTESIAN_POINT('Ctrl Pts',(3.58324299321411,2.04133793352501,-20.5270289695647)) ;
#169186=CARTESIAN_POINT('Ctrl Pts',(3.67209270719133,1.95869361548256,-20.4382138841634)) ;
#169187=CARTESIAN_POINT('Ctrl Pts',(3.57877657372945,1.99742369139614,-20.4246019249096)) ;
#169188=CARTESIAN_POINT('Ctrl Pts',(3.59173571364127,2.05270412132582,-20.5092738450102)) ;
#169189=CARTESIAN_POINT('Ctrl Pts',(3.68022412057906,1.96474917806413,-20.432815204266)) ;
#169190=CARTESIAN_POINT('Ctrl Pts',(3.58322866085249,1.99475271178031,-20.4197736262967)) ;
#169191=CARTESIAN_POINT('Ctrl Pts',(3.59492343714209,2.05814036366738,-20.499399963424)) ;
#169192=CARTESIAN_POINT('Ctrl Pts',(3.69368364956801,1.9763214942053,-20.4202488628171)) ;
#169193=CARTESIAN_POINT('Ctrl Pts',(3.59172551342567,1.98925228662577,-20.4109992807163)) ;
#169194=CARTESIAN_POINT('Ctrl Pts',(3.59903094645825,2.06720241143977,-20.4783439645117)) ;
#169195=CARTESIAN_POINT('Ctrl Pts',(3.70000914724963,1.98195813651218,-20.4130443443145)) ;
#169196=CARTESIAN_POINT('Ctrl Pts',(3.59596384548934,1.9854304914036,-20.4070095444861)) ;
#169197=CARTESIAN_POINT('Ctrl Pts',(3.6,2.07088547209219,-20.4670528114759)) ;
#169198=CARTESIAN_POINT('Ctrl Pts',(3.70001318823691,1.98660254113158,-20.4050000004348)) ;
#169199=CARTESIAN_POINT('Ctrl Pts',(3.6,1.98659111827701,-20.4049934054467)) ;
#169200=CARTESIAN_POINT('Ctrl Pts',(3.6,2.07320508075689,-20.455)) ;
#169201=CARTESIAN_POINT('Origin',(3.6,1.92679491924311,-20.555)) ;
#169202=CARTESIAN_POINT('Origin',(3.5,2.1,-20.555)) ;
#169203=CARTESIAN_POINT('Origin',(3.7,1.9,-17.745)) ;
#169204=CARTESIAN_POINT('Origin',(3.7,2.07320508075689,-17.645)) ;
#169205=CARTESIAN_POINT('Ctrl Pts',(3.70000000000001,1.98660254037844,-17.695)) ;
#169206=CARTESIAN_POINT('Ctrl Pts',(3.59998681089334,1.98660254037844,-17.695)) ;
#169207=CARTESIAN_POINT('Ctrl Pts',(3.60000000086965,2.07321650210508,-17.6449934058816)) ;
#169208=CARTESIAN_POINT('Ctrl Pts',(3.69999562155021,1.98201223284605,-17.6870493541315)) ;
#169209=CARTESIAN_POINT('Ctrl Pts',(3.59600027733259,1.9854568418521,-17.6930080952477)) ;
#169210=CARTESIAN_POINT('Ctrl Pts',(3.60000051733381,2.07092325544402,-17.6330783030551)) ;
#169211=CARTESIAN_POINT('Ctrl Pts',(3.69363885617462,1.97629200693012,-17.6797138033543)) ;
#169212=CARTESIAN_POINT('Ctrl Pts',(3.59168983076589,1.98927958701711,-17.6889705343779)) ;
#169213=CARTESIAN_POINT('Ctrl Pts',(3.5990249033077,2.06719087470394,-17.6215859349146)) ;
#169214=CARTESIAN_POINT('Ctrl Pts',(3.68016115437406,1.9647139415824,-17.6671486857374)) ;
#169215=CARTESIAN_POINT('Ctrl Pts',(3.58318874066453,1.99478340591318,-17.6801866299628)) ;
#169216=CARTESIAN_POINT('Ctrl Pts',(3.59490697186185,2.05811520529797,-17.6005230194575)) ;
#169217=CARTESIAN_POINT('Ctrl Pts',(3.6720289695647,1.958662066475,-17.6617570067859)) ;
#169218=CARTESIAN_POINT('Ctrl Pts',(3.57873800427671,1.99745214073432,-17.6753596224745)) ;
#169219=CARTESIAN_POINT('Ctrl Pts',(3.59171544038559,2.05267725096218,-17.5906561639993)) ;
#169220=CARTESIAN_POINT('Ctrl Pts',(3.6542738450102,1.94729587867418,-17.6532642863587)) ;
#169221=CARTESIAN_POINT('Ctrl Pts',(3.5696019249096,2.00257630860386,-17.6662234262706)) ;
#169222=CARTESIAN_POINT('Ctrl Pts',(3.5832138841634,2.04130638451742,-17.5729072928087)) ;
#169223=CARTESIAN_POINT('Ctrl Pts',(3.64439996342401,1.94185963633263,-17.6500765628579)) ;
#169224=CARTESIAN_POINT('Ctrl Pts',(3.56477362629676,2.0052472882197,-17.6617713391475)) ;
#169225=CARTESIAN_POINT('Ctrl Pts',(3.57781520426602,2.03525082193588,-17.5647758794209)) ;
#169226=CARTESIAN_POINT('Ctrl Pts',(3.62334396451164,1.93279758856024,-17.6459690535418)) ;
#169227=CARTESIAN_POINT('Ctrl Pts',(3.55599928071625,2.01074771337422,-17.6532744865743)) ;
#169228=CARTESIAN_POINT('Ctrl Pts',(3.56524886281709,2.02367850579469,-17.551316350432)) ;
#169229=CARTESIAN_POINT('Ctrl Pts',(3.61205281147588,1.9291145279078,-17.645)) ;
#169230=CARTESIAN_POINT('Ctrl Pts',(3.55200954448629,2.01456950859638,-17.6490361545106)) ;
#169231=CARTESIAN_POINT('Ctrl Pts',(3.55804434431452,2.01804186348782,-17.5449908527503)) ;
#169232=CARTESIAN_POINT('Ctrl Pts',(3.6,1.92679491924311,-17.645)) ;
#169233=CARTESIAN_POINT('Ctrl Pts',(3.54999340544667,2.01340888172298,-17.645)) ;
#169234=CARTESIAN_POINT('Ctrl Pts',(3.55000000043483,2.01339745886842,-17.5449868117631)) ;
#169235=CARTESIAN_POINT('Origin',(3.6,1.92679491924311,-17.545)) ;
#169236=CARTESIAN_POINT('Origin',(3.5,2.1,-17.545)) ;
#169237=CARTESIAN_POINT('Origin',(3.7,1.9,-24.165)) ;
#169238=CARTESIAN_POINT('Origin',(3.7,2.07320508075689,-24.265)) ;
#169239=CARTESIAN_POINT('Ctrl Pts',(3.60000659411846,1.92678349789492,-24.2650000008696)) ;
#169240=CARTESIAN_POINT('Ctrl Pts',(3.55,2.01339745962156,-24.2649868108933)) ;
#169241=CARTESIAN_POINT('Ctrl Pts',(3.55,2.01339745962156,-24.365)) ;
#169242=CARTESIAN_POINT('Ctrl Pts',(3.61192169694494,1.92907674455598,-24.2650005173338)) ;
#169243=CARTESIAN_POINT('Ctrl Pts',(3.55199190475211,2.01454315814821,-24.2610002773326)) ;
#169244=CARTESIAN_POINT('Ctrl Pts',(3.55795064586847,2.01798776715395,-24.3649956215505)) ;
#169245=CARTESIAN_POINT('Ctrl Pts',(3.62341406508538,1.93280912529606,-24.2640249033077)) ;
#169246=CARTESIAN_POINT('Ctrl Pts',(3.55602946562207,2.0107204129829,-24.2566898307659)) ;
#169247=CARTESIAN_POINT('Ctrl Pts',(3.56528619664567,2.02370799306988,-24.3586388561746)) ;
#169248=CARTESIAN_POINT('Ctrl Pts',(3.64447698054259,1.94188479470202,-24.2599069718618)) ;
#169249=CARTESIAN_POINT('Ctrl Pts',(3.56481337003729,2.00521659408681,-24.2481887406645)) ;
#169250=CARTESIAN_POINT('Ctrl Pts',(3.5778513142626,2.0352860584176,-24.3451611543741)) ;
#169251=CARTESIAN_POINT('Ctrl Pts',(3.65434383600069,1.94732274903783,-24.2567154403856)) ;
#169252=CARTESIAN_POINT('Ctrl Pts',(3.56964037752544,2.00254785926569,-24.2437380042767)) ;
#169253=CARTESIAN_POINT('Ctrl Pts',(3.58324299321411,2.04133793352501,-24.3370289695647)) ;
#169254=CARTESIAN_POINT('Ctrl Pts',(3.67209270719133,1.95869361548256,-24.2482138841634)) ;
#169255=CARTESIAN_POINT('Ctrl Pts',(3.57877657372945,1.99742369139614,-24.2346019249096)) ;
#169256=CARTESIAN_POINT('Ctrl Pts',(3.59173571364127,2.05270412132582,-24.3192738450102)) ;
#169257=CARTESIAN_POINT('Ctrl Pts',(3.68022412057906,1.96474917806411,-24.242815204266)) ;
#169258=CARTESIAN_POINT('Ctrl Pts',(3.58322866085247,1.99475271178029,-24.2297736262968)) ;
#169259=CARTESIAN_POINT('Ctrl Pts',(3.59492343714209,2.05814036366738,-24.309399963424)) ;
#169260=CARTESIAN_POINT('Ctrl Pts',(3.69368364956801,1.97632149420531,-24.2302488628171)) ;
#169261=CARTESIAN_POINT('Ctrl Pts',(3.59172551342569,1.98925228662579,-24.2209992807162)) ;
#169262=CARTESIAN_POINT('Ctrl Pts',(3.59903094645825,2.06720241143977,-24.2883439645117)) ;
#169263=CARTESIAN_POINT('Ctrl Pts',(3.70000914724963,1.98195813651217,-24.2230443443145)) ;
#169264=CARTESIAN_POINT('Ctrl Pts',(3.59596384548931,1.98543049140359,-24.2170095444862)) ;
#169265=CARTESIAN_POINT('Ctrl Pts',(3.6,2.07088547209219,-24.2770528114759)) ;
#169266=CARTESIAN_POINT('Ctrl Pts',(3.70001318823691,1.98660254113158,-24.2150000004348)) ;
#169267=CARTESIAN_POINT('Ctrl Pts',(3.6,1.98659111827701,-24.2149934054467)) ;
#169268=CARTESIAN_POINT('Ctrl Pts',(3.6,2.07320508075689,-24.265)) ;
#169269=CARTESIAN_POINT('Origin',(3.6,1.92679491924311,-24.365)) ;
#169270=CARTESIAN_POINT('Origin',(3.5,2.1,-24.365)) ;
#169271=CARTESIAN_POINT('Origin',(3.7,1.9,-21.555)) ;
#169272=CARTESIAN_POINT('Origin',(3.7,2.07320508075689,-21.455)) ;
#169273=CARTESIAN_POINT('Ctrl Pts',(3.70000000000001,1.98660254037844,-21.505)) ;
#169274=CARTESIAN_POINT('Ctrl Pts',(3.59998681089334,1.98660254037844,-21.505)) ;
#169275=CARTESIAN_POINT('Ctrl Pts',(3.60000000086965,2.07321650210507,-21.4549934058816)) ;
#169276=CARTESIAN_POINT('Ctrl Pts',(3.69999562155021,1.98201223284605,-21.4970493541315)) ;
#169277=CARTESIAN_POINT('Ctrl Pts',(3.59600027733255,1.98545684185209,-21.5030080952477)) ;
#169278=CARTESIAN_POINT('Ctrl Pts',(3.60000051733381,2.07092325544402,-21.4430783030551)) ;
#169279=CARTESIAN_POINT('Ctrl Pts',(3.69363885617462,1.97629200693012,-21.4897138033543)) ;
#169280=CARTESIAN_POINT('Ctrl Pts',(3.59168983076595,1.98927958701713,-21.4989705343779)) ;
#169281=CARTESIAN_POINT('Ctrl Pts',(3.5990249033077,2.06719087470394,-21.4315859349146)) ;
#169282=CARTESIAN_POINT('Ctrl Pts',(3.68016115437406,1.9647139415824,-21.4771486857374)) ;
#169283=CARTESIAN_POINT('Ctrl Pts',(3.58318874066447,1.99478340591315,-21.4901866299627)) ;
#169284=CARTESIAN_POINT('Ctrl Pts',(3.59490697186185,2.05811520529797,-21.4105230194575)) ;
#169285=CARTESIAN_POINT('Ctrl Pts',(3.6720289695647,1.958662066475,-21.4717570067859)) ;
#169286=CARTESIAN_POINT('Ctrl Pts',(3.57873800427674,1.99745214073432,-21.4853596224745)) ;
#169287=CARTESIAN_POINT('Ctrl Pts',(3.59171544038559,2.05267725096218,-21.4006561639993)) ;
#169288=CARTESIAN_POINT('Ctrl Pts',(3.6542738450102,1.94729587867418,-21.4632642863587)) ;
#169289=CARTESIAN_POINT('Ctrl Pts',(3.56960192490957,2.00257630860385,-21.4762234262706)) ;
#169290=CARTESIAN_POINT('Ctrl Pts',(3.5832138841634,2.04130638451742,-21.3829072928087)) ;
#169291=CARTESIAN_POINT('Ctrl Pts',(3.64439996342401,1.94185963633263,-21.4600765628579)) ;
#169292=CARTESIAN_POINT('Ctrl Pts',(3.56477362629673,2.00524728821971,-21.4717713391475)) ;
#169293=CARTESIAN_POINT('Ctrl Pts',(3.57781520426602,2.03525082193588,-21.3747758794209)) ;
#169294=CARTESIAN_POINT('Ctrl Pts',(3.62334396451164,1.93279758856024,-21.4559690535418)) ;
#169295=CARTESIAN_POINT('Ctrl Pts',(3.55599928071628,2.0107477133742,-21.4632744865743)) ;
#169296=CARTESIAN_POINT('Ctrl Pts',(3.56524886281709,2.02367850579469,-21.361316350432)) ;
#169297=CARTESIAN_POINT('Ctrl Pts',(3.61205281147588,1.9291145279078,-21.455)) ;
#169298=CARTESIAN_POINT('Ctrl Pts',(3.55200954448635,2.01456950859626,-21.4590361545106)) ;
#169299=CARTESIAN_POINT('Ctrl Pts',(3.55804434431452,2.01804186348782,-21.3549908527503)) ;
#169300=CARTESIAN_POINT('Ctrl Pts',(3.6,1.92679491924311,-21.455)) ;
#169301=CARTESIAN_POINT('Ctrl Pts',(3.54999340544667,2.01340888172298,-21.455)) ;
#169302=CARTESIAN_POINT('Ctrl Pts',(3.55000000043483,2.01339745886842,-21.3549868117631)) ;
#169303=CARTESIAN_POINT('Origin',(3.6,1.92679491924311,-21.355)) ;
#169304=CARTESIAN_POINT('Origin',(3.5,2.1,-21.355)) ;
#169305=CARTESIAN_POINT('Origin',(3.7,1.9,-27.975)) ;
#169306=CARTESIAN_POINT('Origin',(3.7,2.07320508075689,-28.075)) ;
#169307=CARTESIAN_POINT('Ctrl Pts',(3.60000659411846,1.92678349789492,-28.0750000008697)) ;
#169308=CARTESIAN_POINT('Ctrl Pts',(3.55,2.01339745962156,-28.0749868108933)) ;
#169309=CARTESIAN_POINT('Ctrl Pts',(3.55,2.01339745962156,-28.175)) ;
#169310=CARTESIAN_POINT('Ctrl Pts',(3.61192169694494,1.92907674455598,-28.0750005173338)) ;
#169311=CARTESIAN_POINT('Ctrl Pts',(3.55199190475223,2.01454315814803,-28.0710002773326)) ;
#169312=CARTESIAN_POINT('Ctrl Pts',(3.55795064586847,2.01798776715395,-28.1749956215505)) ;
#169313=CARTESIAN_POINT('Ctrl Pts',(3.62341406508537,1.93280912529606,-28.0740249033077)) ;
#169314=CARTESIAN_POINT('Ctrl Pts',(3.55602946562204,2.01072041298292,-28.0666898307659)) ;
#169315=CARTESIAN_POINT('Ctrl Pts',(3.56528619664567,2.02370799306988,-28.1686388561746)) ;
#169316=CARTESIAN_POINT('Ctrl Pts',(3.64447698054259,1.94188479470202,-28.0699069718619)) ;
#169317=CARTESIAN_POINT('Ctrl Pts',(3.56481337003732,2.0052165940868,-28.0581887406645)) ;
#169318=CARTESIAN_POINT('Ctrl Pts',(3.5778513142626,2.0352860584176,-28.155161154374)) ;
#169319=CARTESIAN_POINT('Ctrl Pts',(3.65434383600069,1.94732274903782,-28.0667154403856)) ;
#169320=CARTESIAN_POINT('Ctrl Pts',(3.56964037752548,2.00254785926568,-28.0537380042767)) ;
#169321=CARTESIAN_POINT('Ctrl Pts',(3.58324299321411,2.04133793352501,-28.1470289695647)) ;
#169322=CARTESIAN_POINT('Ctrl Pts',(3.67209270719133,1.95869361548256,-28.0582138841634)) ;
#169323=CARTESIAN_POINT('Ctrl Pts',(3.57877657372942,1.99742369139614,-28.0446019249096)) ;
#169324=CARTESIAN_POINT('Ctrl Pts',(3.59173571364127,2.05270412132582,-28.1292738450102)) ;
#169325=CARTESIAN_POINT('Ctrl Pts',(3.68022412057906,1.96474917806411,-28.052815204266)) ;
#169326=CARTESIAN_POINT('Ctrl Pts',(3.5832286608525,1.99475271178031,-28.0397736262968)) ;
#169327=CARTESIAN_POINT('Ctrl Pts',(3.59492343714209,2.05814036366738,-28.119399963424)) ;
#169328=CARTESIAN_POINT('Ctrl Pts',(3.69368364956801,1.97632149420531,-28.0402488628171)) ;
#169329=CARTESIAN_POINT('Ctrl Pts',(3.59172551342567,1.98925228662577,-28.0309992807162)) ;
#169330=CARTESIAN_POINT('Ctrl Pts',(3.59903094645825,2.06720241143977,-28.0983439645117)) ;
#169331=CARTESIAN_POINT('Ctrl Pts',(3.70000914724963,1.98195813651217,-28.0330443443145)) ;
#169332=CARTESIAN_POINT('Ctrl Pts',(3.59596384548938,1.98543049140356,-28.0270095444862)) ;
#169333=CARTESIAN_POINT('Ctrl Pts',(3.6,2.07088547209218,-28.0870528114759)) ;
#169334=CARTESIAN_POINT('Ctrl Pts',(3.70001318823691,1.98660254113158,-28.0250000004348)) ;
#169335=CARTESIAN_POINT('Ctrl Pts',(3.6,1.98659111827701,-28.0249934054467)) ;
#169336=CARTESIAN_POINT('Ctrl Pts',(3.6,2.07320508075689,-28.075)) ;
#169337=CARTESIAN_POINT('Origin',(3.6,1.92679491924311,-28.175)) ;
#169338=CARTESIAN_POINT('Origin',(3.5,2.1,-28.175)) ;
#169339=CARTESIAN_POINT('Origin',(3.7,1.9,-25.365)) ;
#169340=CARTESIAN_POINT('Origin',(3.7,2.07320508075689,-25.265)) ;
#169341=CARTESIAN_POINT('Ctrl Pts',(3.70000000000001,1.98660254037844,-25.315)) ;
#169342=CARTESIAN_POINT('Ctrl Pts',(3.59998681089334,1.98660254037844,-25.315)) ;
#169343=CARTESIAN_POINT('Ctrl Pts',(3.60000000086965,2.07321650210507,-25.2649934058815)) ;
#169344=CARTESIAN_POINT('Ctrl Pts',(3.69999562155021,1.98201223284605,-25.3070493541315)) ;
#169345=CARTESIAN_POINT('Ctrl Pts',(3.5960002773326,1.9854568418521,-25.3130080952477)) ;
#169346=CARTESIAN_POINT('Ctrl Pts',(3.60000051733381,2.07092325544402,-25.2530783030551)) ;
#169347=CARTESIAN_POINT('Ctrl Pts',(3.69363885617462,1.97629200693012,-25.2997138033543)) ;
#169348=CARTESIAN_POINT('Ctrl Pts',(3.59168983076589,1.98927958701711,-25.3089705343779)) ;
#169349=CARTESIAN_POINT('Ctrl Pts',(3.5990249033077,2.06719087470394,-25.2415859349146)) ;
#169350=CARTESIAN_POINT('Ctrl Pts',(3.68016115437406,1.9647139415824,-25.2871486857374)) ;
#169351=CARTESIAN_POINT('Ctrl Pts',(3.58318874066453,1.99478340591318,-25.3001866299628)) ;
#169352=CARTESIAN_POINT('Ctrl Pts',(3.59490697186185,2.05811520529797,-25.2205230194575)) ;
#169353=CARTESIAN_POINT('Ctrl Pts',(3.6720289695647,1.958662066475,-25.2817570067859)) ;
#169354=CARTESIAN_POINT('Ctrl Pts',(3.57873800427668,1.99745214073432,-25.2953596224745)) ;
#169355=CARTESIAN_POINT('Ctrl Pts',(3.59171544038559,2.05267725096218,-25.2106561639993)) ;
#169356=CARTESIAN_POINT('Ctrl Pts',(3.6542738450102,1.94729587867418,-25.2732642863587)) ;
#169357=CARTESIAN_POINT('Ctrl Pts',(3.56960192490964,2.00257630860385,-25.2862234262706)) ;
#169358=CARTESIAN_POINT('Ctrl Pts',(3.5832138841634,2.04130638451742,-25.1929072928087)) ;
#169359=CARTESIAN_POINT('Ctrl Pts',(3.64439996342401,1.94185963633263,-25.2700765628579)) ;
#169360=CARTESIAN_POINT('Ctrl Pts',(3.56477362629676,2.0052472882197,-25.2817713391475)) ;
#169361=CARTESIAN_POINT('Ctrl Pts',(3.57781520426602,2.03525082193588,-25.1847758794209)) ;
#169362=CARTESIAN_POINT('Ctrl Pts',(3.62334396451164,1.93279758856024,-25.2659690535418)) ;
#169363=CARTESIAN_POINT('Ctrl Pts',(3.55599928071625,2.01074771337422,-25.2732744865743)) ;
#169364=CARTESIAN_POINT('Ctrl Pts',(3.56524886281709,2.02367850579469,-25.171316350432)) ;
#169365=CARTESIAN_POINT('Ctrl Pts',(3.61205281147588,1.9291145279078,-25.265)) ;
#169366=CARTESIAN_POINT('Ctrl Pts',(3.55200954448633,2.01456950859634,-25.2690361545106)) ;
#169367=CARTESIAN_POINT('Ctrl Pts',(3.55804434431452,2.01804186348782,-25.1649908527503)) ;
#169368=CARTESIAN_POINT('Ctrl Pts',(3.6,1.92679491924311,-25.265)) ;
#169369=CARTESIAN_POINT('Ctrl Pts',(3.54999340544667,2.01340888172298,-25.265)) ;
#169370=CARTESIAN_POINT('Ctrl Pts',(3.55000000043483,2.01339745886842,-25.1649868117631)) ;
#169371=CARTESIAN_POINT('Origin',(3.6,1.92679491924311,-25.165)) ;
#169372=CARTESIAN_POINT('Origin',(3.5,2.1,-25.165)) ;
#169373=CARTESIAN_POINT('Origin',(3.7,1.9,-31.785)) ;
#169374=CARTESIAN_POINT('Origin',(3.7,2.07320508075689,-31.885)) ;
#169375=CARTESIAN_POINT('Ctrl Pts',(3.60000659411846,1.92678349789491,-31.8850000008696)) ;
#169376=CARTESIAN_POINT('Ctrl Pts',(3.55000000000001,2.01339745962154,-31.8849868108933)) ;
#169377=CARTESIAN_POINT('Ctrl Pts',(3.55,2.01339745962156,-31.985)) ;
#169378=CARTESIAN_POINT('Ctrl Pts',(3.61192169694494,1.92907674455598,-31.8850005173338)) ;
#169379=CARTESIAN_POINT('Ctrl Pts',(3.55199190475219,2.01454315814809,-31.8810002773326)) ;
#169380=CARTESIAN_POINT('Ctrl Pts',(3.55795064586847,2.01798776715395,-31.9849956215505)) ;
#169381=CARTESIAN_POINT('Ctrl Pts',(3.62341406508538,1.93280912529607,-31.8840249033077)) ;
#169382=CARTESIAN_POINT('Ctrl Pts',(3.55602946562211,2.01072041298287,-31.8766898307658)) ;
#169383=CARTESIAN_POINT('Ctrl Pts',(3.56528619664567,2.02370799306987,-31.9786388561746)) ;
#169384=CARTESIAN_POINT('Ctrl Pts',(3.64447698054259,1.941884794702,-31.8799069718618)) ;
#169385=CARTESIAN_POINT('Ctrl Pts',(3.56481337003728,2.00521659408683,-31.8681887406646)) ;
#169386=CARTESIAN_POINT('Ctrl Pts',(3.5778513142626,2.0352860584176,-31.9651611543741)) ;
#169387=CARTESIAN_POINT('Ctrl Pts',(3.65434383600069,1.94732274903778,-31.8767154403856)) ;
#169388=CARTESIAN_POINT('Ctrl Pts',(3.56964037752544,2.00254785926569,-31.8637380042767)) ;
#169389=CARTESIAN_POINT('Ctrl Pts',(3.58324299321411,2.04133793352501,-31.9570289695647)) ;
#169390=CARTESIAN_POINT('Ctrl Pts',(3.67209270719134,1.95869361548259,-31.8682138841634)) ;
#169391=CARTESIAN_POINT('Ctrl Pts',(3.57877657372946,1.99742369139612,-31.8546019249095)) ;
#169392=CARTESIAN_POINT('Ctrl Pts',(3.59173571364126,2.0527041213258,-31.9392738450101)) ;
#169393=CARTESIAN_POINT('Ctrl Pts',(3.68022412057906,1.9647491780641,-31.862815204266)) ;
#169394=CARTESIAN_POINT('Ctrl Pts',(3.58322866085252,1.99475271178032,-31.8497736262967)) ;
#169395=CARTESIAN_POINT('Ctrl Pts',(3.59492343714209,2.05814036366737,-31.929399963424)) ;
#169396=CARTESIAN_POINT('Ctrl Pts',(3.69368364956802,1.97632149420531,-31.8502488628171)) ;
#169397=CARTESIAN_POINT('Ctrl Pts',(3.59172551342565,1.98925228662574,-31.8409992807163)) ;
#169398=CARTESIAN_POINT('Ctrl Pts',(3.59903094645825,2.06720241143977,-31.9083439645117)) ;
#169399=CARTESIAN_POINT('Ctrl Pts',(3.70000914724964,1.98195813651217,-31.8430443443145)) ;
#169400=CARTESIAN_POINT('Ctrl Pts',(3.59596384548948,1.98543049140366,-31.8370095444864)) ;
#169401=CARTESIAN_POINT('Ctrl Pts',(3.6,2.07088547209221,-31.8970528114759)) ;
#169402=CARTESIAN_POINT('Ctrl Pts',(3.70001318823692,1.98660254113158,-31.8350000004348)) ;
#169403=CARTESIAN_POINT('Ctrl Pts',(3.6,1.98659111827701,-31.8349934054467)) ;
#169404=CARTESIAN_POINT('Ctrl Pts',(3.6,2.07320508075689,-31.885)) ;
#169405=CARTESIAN_POINT('Origin',(3.6,1.92679491924311,-31.985)) ;
#169406=CARTESIAN_POINT('Origin',(3.5,2.1,-31.985)) ;
#169407=CARTESIAN_POINT('Origin',(3.7,1.9,-29.175)) ;
#169408=CARTESIAN_POINT('Origin',(3.7,2.07320508075689,-29.075)) ;
#169409=CARTESIAN_POINT('Ctrl Pts',(3.70000000000001,1.98660254037844,-29.125)) ;
#169410=CARTESIAN_POINT('Ctrl Pts',(3.59998681089334,1.98660254037844,-29.125)) ;
#169411=CARTESIAN_POINT('Ctrl Pts',(3.60000000086965,2.07321650210507,-29.0749934058815)) ;
#169412=CARTESIAN_POINT('Ctrl Pts',(3.69999562155021,1.98201223284605,-29.1170493541315)) ;
#169413=CARTESIAN_POINT('Ctrl Pts',(3.59600027733264,1.98545684185212,-29.1230080952477)) ;
#169414=CARTESIAN_POINT('Ctrl Pts',(3.60000051733381,2.07092325544403,-29.0630783030551)) ;
#169415=CARTESIAN_POINT('Ctrl Pts',(3.69363885617462,1.97629200693012,-29.1097138033543)) ;
#169416=CARTESIAN_POINT('Ctrl Pts',(3.59168983076584,1.98927958701707,-29.1189705343779)) ;
#169417=CARTESIAN_POINT('Ctrl Pts',(3.5990249033077,2.06719087470394,-29.0515859349146)) ;
#169418=CARTESIAN_POINT('Ctrl Pts',(3.68016115437406,1.9647139415824,-29.0971486857374)) ;
#169419=CARTESIAN_POINT('Ctrl Pts',(3.58318874066458,1.99478340591321,-29.1101866299628)) ;
#169420=CARTESIAN_POINT('Ctrl Pts',(3.59490697186185,2.05811520529797,-29.0305230194575)) ;
#169421=CARTESIAN_POINT('Ctrl Pts',(3.6720289695647,1.958662066475,-29.0917570067859)) ;
#169422=CARTESIAN_POINT('Ctrl Pts',(3.57873800427668,1.99745214073431,-29.1053596224745)) ;
#169423=CARTESIAN_POINT('Ctrl Pts',(3.59171544038559,2.05267725096218,-29.0206561639993)) ;
#169424=CARTESIAN_POINT('Ctrl Pts',(3.6542738450102,1.94729587867418,-29.0832642863587)) ;
#169425=CARTESIAN_POINT('Ctrl Pts',(3.56960192490963,2.00257630860385,-29.0962234262706)) ;
#169426=CARTESIAN_POINT('Ctrl Pts',(3.5832138841634,2.04130638451742,-29.0029072928087)) ;
#169427=CARTESIAN_POINT('Ctrl Pts',(3.64439996342401,1.94185963633263,-29.0800765628579)) ;
#169428=CARTESIAN_POINT('Ctrl Pts',(3.56477362629679,2.00524728821968,-29.0917713391475)) ;
#169429=CARTESIAN_POINT('Ctrl Pts',(3.57781520426602,2.03525082193588,-28.9947758794209)) ;
#169430=CARTESIAN_POINT('Ctrl Pts',(3.62334396451164,1.93279758856024,-29.0759690535418)) ;
#169431=CARTESIAN_POINT('Ctrl Pts',(3.55599928071622,2.01074771337424,-29.0832744865743)) ;
#169432=CARTESIAN_POINT('Ctrl Pts',(3.56524886281709,2.02367850579469,-28.981316350432)) ;
#169433=CARTESIAN_POINT('Ctrl Pts',(3.61205281147588,1.9291145279078,-29.075)) ;
#169434=CARTESIAN_POINT('Ctrl Pts',(3.55200954448622,2.01456950859647,-29.0790361545106)) ;
#169435=CARTESIAN_POINT('Ctrl Pts',(3.55804434431452,2.01804186348782,-28.9749908527503)) ;
#169436=CARTESIAN_POINT('Ctrl Pts',(3.6,1.92679491924311,-29.075)) ;
#169437=CARTESIAN_POINT('Ctrl Pts',(3.54999340544667,2.01340888172298,-29.075)) ;
#169438=CARTESIAN_POINT('Ctrl Pts',(3.55000000043483,2.01339745886842,-28.9749868117631)) ;
#169439=CARTESIAN_POINT('Origin',(3.6,1.92679491924311,-28.975)) ;
#169440=CARTESIAN_POINT('Origin',(3.5,2.1,-28.975)) ;
#169441=CARTESIAN_POINT('Origin',(3.7,1.9,-35.595)) ;
#169442=CARTESIAN_POINT('Origin',(3.7,2.07320508075689,-35.695)) ;
#169443=CARTESIAN_POINT('Ctrl Pts',(3.60000659411846,1.92678349789491,-35.6950000008697)) ;
#169444=CARTESIAN_POINT('Ctrl Pts',(3.55000000000001,2.01339745962154,-35.6949868108933)) ;
#169445=CARTESIAN_POINT('Ctrl Pts',(3.55,2.01339745962156,-35.795)) ;
#169446=CARTESIAN_POINT('Ctrl Pts',(3.61192169694494,1.92907674455598,-35.6950005173338)) ;
#169447=CARTESIAN_POINT('Ctrl Pts',(3.55199190475219,2.01454315814809,-35.6910002773326)) ;
#169448=CARTESIAN_POINT('Ctrl Pts',(3.55795064586847,2.01798776715395,-35.7949956215505)) ;
#169449=CARTESIAN_POINT('Ctrl Pts',(3.62341406508538,1.93280912529607,-35.6940249033077)) ;
#169450=CARTESIAN_POINT('Ctrl Pts',(3.55602946562211,2.01072041298287,-35.6866898307658)) ;
#169451=CARTESIAN_POINT('Ctrl Pts',(3.56528619664567,2.02370799306987,-35.7886388561746)) ;
#169452=CARTESIAN_POINT('Ctrl Pts',(3.64447698054259,1.941884794702,-35.6899069718619)) ;
#169453=CARTESIAN_POINT('Ctrl Pts',(3.56481337003728,2.00521659408683,-35.6781887406645)) ;
#169454=CARTESIAN_POINT('Ctrl Pts',(3.5778513142626,2.0352860584176,-35.7751611543741)) ;
#169455=CARTESIAN_POINT('Ctrl Pts',(3.65434383600069,1.94732274903778,-35.6867154403856)) ;
#169456=CARTESIAN_POINT('Ctrl Pts',(3.56964037752544,2.00254785926569,-35.6737380042767)) ;
#169457=CARTESIAN_POINT('Ctrl Pts',(3.58324299321411,2.04133793352501,-35.7670289695647)) ;
#169458=CARTESIAN_POINT('Ctrl Pts',(3.67209270719134,1.95869361548259,-35.6782138841634)) ;
#169459=CARTESIAN_POINT('Ctrl Pts',(3.57877657372946,1.99742369139612,-35.6646019249095)) ;
#169460=CARTESIAN_POINT('Ctrl Pts',(3.59173571364126,2.0527041213258,-35.7492738450102)) ;
#169461=CARTESIAN_POINT('Ctrl Pts',(3.68022412057906,1.9647491780641,-35.672815204266)) ;
#169462=CARTESIAN_POINT('Ctrl Pts',(3.58322866085252,1.99475271178032,-35.6597736262967)) ;
#169463=CARTESIAN_POINT('Ctrl Pts',(3.59492343714209,2.05814036366737,-35.739399963424)) ;
#169464=CARTESIAN_POINT('Ctrl Pts',(3.69368364956802,1.97632149420531,-35.6602488628171)) ;
#169465=CARTESIAN_POINT('Ctrl Pts',(3.59172551342565,1.98925228662574,-35.6509992807163)) ;
#169466=CARTESIAN_POINT('Ctrl Pts',(3.59903094645825,2.06720241143977,-35.7183439645117)) ;
#169467=CARTESIAN_POINT('Ctrl Pts',(3.70000914724964,1.98195813651217,-35.6530443443145)) ;
#169468=CARTESIAN_POINT('Ctrl Pts',(3.59596384548948,1.98543049140366,-35.6470095444864)) ;
#169469=CARTESIAN_POINT('Ctrl Pts',(3.6,2.07088547209221,-35.7070528114759)) ;
#169470=CARTESIAN_POINT('Ctrl Pts',(3.70001318823692,1.98660254113158,-35.6450000004348)) ;
#169471=CARTESIAN_POINT('Ctrl Pts',(3.6,1.98659111827701,-35.6449934054467)) ;
#169472=CARTESIAN_POINT('Ctrl Pts',(3.6,2.07320508075689,-35.695)) ;
#169473=CARTESIAN_POINT('Origin',(3.6,1.92679491924311,-35.795)) ;
#169474=CARTESIAN_POINT('Origin',(3.5,2.1,-35.795)) ;
#169475=CARTESIAN_POINT('Origin',(3.7,1.9,-32.985)) ;
#169476=CARTESIAN_POINT('Origin',(3.7,2.07320508075689,-32.885)) ;
#169477=CARTESIAN_POINT('Ctrl Pts',(3.70000000000001,1.98660254037844,-32.935)) ;
#169478=CARTESIAN_POINT('Ctrl Pts',(3.59998681089332,1.98660254037844,-32.935)) ;
#169479=CARTESIAN_POINT('Ctrl Pts',(3.60000000086965,2.07321650210509,-32.8849934058815)) ;
#169480=CARTESIAN_POINT('Ctrl Pts',(3.69999562155021,1.98201223284604,-32.9270493541315)) ;
#169481=CARTESIAN_POINT('Ctrl Pts',(3.59600027733252,1.98545684185201,-32.9330080952478)) ;
#169482=CARTESIAN_POINT('Ctrl Pts',(3.60000051733381,2.07092325544402,-32.873078303055)) ;
#169483=CARTESIAN_POINT('Ctrl Pts',(3.69363885617463,1.97629200693015,-32.9197138033543)) ;
#169484=CARTESIAN_POINT('Ctrl Pts',(3.59168983076591,1.98927958701709,-32.9289705343779)) ;
#169485=CARTESIAN_POINT('Ctrl Pts',(3.59902490330771,2.06719087470393,-32.8615859349147)) ;
#169486=CARTESIAN_POINT('Ctrl Pts',(3.68016115437406,1.96471394158237,-32.9071486857374)) ;
#169487=CARTESIAN_POINT('Ctrl Pts',(3.58318874066448,1.99478340591319,-32.9201866299627)) ;
#169488=CARTESIAN_POINT('Ctrl Pts',(3.59490697186185,2.05811520529799,-32.8405230194574)) ;
#169489=CARTESIAN_POINT('Ctrl Pts',(3.6720289695647,1.95866206647497,-32.9017570067859)) ;
#169490=CARTESIAN_POINT('Ctrl Pts',(3.57873800427671,1.99745214073432,-32.9153596224745)) ;
#169491=CARTESIAN_POINT('Ctrl Pts',(3.59171544038559,2.05267725096218,-32.8306561639993)) ;
#169492=CARTESIAN_POINT('Ctrl Pts',(3.65427384501021,1.9472958786742,-32.8932642863588)) ;
#169493=CARTESIAN_POINT('Ctrl Pts',(3.56960192490956,2.00257630860387,-32.9062234262707)) ;
#169494=CARTESIAN_POINT('Ctrl Pts',(3.5832138841634,2.04130638451744,-32.8129072928087)) ;
#169495=CARTESIAN_POINT('Ctrl Pts',(3.64439996342399,1.94185963633262,-32.8900765628579)) ;
#169496=CARTESIAN_POINT('Ctrl Pts',(3.5647736262967,2.00524728821974,-32.9017713391475)) ;
#169497=CARTESIAN_POINT('Ctrl Pts',(3.57781520426601,2.03525082193589,-32.8047758794209)) ;
#169498=CARTESIAN_POINT('Ctrl Pts',(3.62334396451166,1.93279758856024,-32.8859690535418)) ;
#169499=CARTESIAN_POINT('Ctrl Pts',(3.55599928071631,2.01074771337418,-32.8932744865743)) ;
#169500=CARTESIAN_POINT('Ctrl Pts',(3.5652488628171,2.02367850579469,-32.7913163504321)) ;
#169501=CARTESIAN_POINT('Ctrl Pts',(3.61205281147586,1.9291145279078,-32.885)) ;
#169502=CARTESIAN_POINT('Ctrl Pts',(3.55200954448637,2.01456950859641,-32.8890361545106)) ;
#169503=CARTESIAN_POINT('Ctrl Pts',(3.55804434431452,2.01804186348783,-32.7849908527503)) ;
#169504=CARTESIAN_POINT('Ctrl Pts',(3.6,1.92679491924311,-32.885)) ;
#169505=CARTESIAN_POINT('Ctrl Pts',(3.54999340544667,2.01340888172297,-32.885)) ;
#169506=CARTESIAN_POINT('Ctrl Pts',(3.55000000043483,2.01339745886842,-32.7849868117631)) ;
#169507=CARTESIAN_POINT('Origin',(3.6,1.92679491924311,-32.785)) ;
#169508=CARTESIAN_POINT('Origin',(3.5,2.1,-32.785)) ;
#169509=CARTESIAN_POINT('Origin',(-1.39554230456301E-15,-1.51907484122731,
-7.62)) ;
#169510=CARTESIAN_POINT('Origin',(-6.11095769946375E-16,4.45,-7.62)) ;
#169511=CARTESIAN_POINT('Origin',(-1.39554230456301E-15,-1.51907484122731,
-11.43)) ;
#169512=CARTESIAN_POINT('Origin',(-6.11095769946375E-16,4.45,-11.43)) ;
#169513=CARTESIAN_POINT('Origin',(-1.39554230456301E-15,-1.51907484122731,
-15.24)) ;
#169514=CARTESIAN_POINT('Origin',(-6.11095769946375E-16,4.45,-15.24)) ;
#169515=CARTESIAN_POINT('Origin',(-1.39554230456301E-15,-1.51907484122731,
-19.05)) ;
#169516=CARTESIAN_POINT('Origin',(-6.11095769946375E-16,4.45,-19.05)) ;
#169517=CARTESIAN_POINT('Origin',(-1.39554230456301E-15,-1.51907484122731,
-22.86)) ;
#169518=CARTESIAN_POINT('Origin',(-6.11095769946375E-16,4.45,-22.86)) ;
#169519=CARTESIAN_POINT('Origin',(-1.39554230456301E-15,-1.51907484122731,
-26.67)) ;
#169520=CARTESIAN_POINT('Origin',(-6.11095769946375E-16,4.45,-26.67)) ;
#169521=CARTESIAN_POINT('Origin',(2.5,-6.45,-36.49)) ;
#169522=CARTESIAN_POINT('Origin',(2.5,-6.45,-36.49)) ;
#169523=CARTESIAN_POINT('Origin',(2.5,4.55,-36.49)) ;
#169524=CARTESIAN_POINT('Origin',(2.5,1.9,-36.49)) ;
#169525=CARTESIAN_POINT('Origin',(2.7,1.9,-36.49)) ;
#169526=CARTESIAN_POINT('Origin',(2.7,2.1,-36.49)) ;
#169527=CARTESIAN_POINT('Origin',(-1.64095463943752E-16,2.1,-36.49)) ;
#169528=CARTESIAN_POINT('Origin',(3.5,2.1,-36.49)) ;
#169529=CARTESIAN_POINT('Origin',(3.5,2.1,-36.49)) ;
#169530=CARTESIAN_POINT('Origin',(3.5,2.1,-36.49)) ;
#169531=CARTESIAN_POINT('Origin',(3.5,7.81406971160724E-17,-36.49)) ;
#169532=CARTESIAN_POINT('Origin',(3.5,2.65,-36.49)) ;
#169533=CARTESIAN_POINT('Origin',(3.5,2.65,-36.49)) ;
#169534=CARTESIAN_POINT('Origin',(3.5,2.65,-36.49)) ;
#169535=CARTESIAN_POINT('Origin',(3.6,2.65,-36.49)) ;
#169536=CARTESIAN_POINT('Origin',(2.7,2.65,-36.49)) ;
#169537=CARTESIAN_POINT('Origin',(-3.9,4.45,-36.49)) ;
#169538=CARTESIAN_POINT('Origin',(-3.9,4.45,-36.49)) ;
#169539=CARTESIAN_POINT('Origin',(2.7,2.85,-36.49)) ;
#169540=CARTESIAN_POINT('Origin',(2.5,2.85,-36.49)) ;
#169541=CARTESIAN_POINT('Origin',(2.7,2.85,-36.49)) ;
#169542=CARTESIAN_POINT('Origin',(-4.,4.45,-36.49)) ;
#169543=CARTESIAN_POINT('Origin',(2.5,4.45,-36.49)) ;
#169544=CARTESIAN_POINT('Origin',(2.5,4.55,-36.49)) ;
#169545=CARTESIAN_POINT('Origin',(2.5,4.45,-36.49)) ;
#169546=CARTESIAN_POINT('Origin',(2.7,2.85,-2.3)) ;
#169547=CARTESIAN_POINT('Origin',(2.7,2.85,-35.94)) ;
#169548=CARTESIAN_POINT('Origin',(2.5,4.45,-36.49)) ;
#169549=CARTESIAN_POINT('Origin',(2.5,4.45,-36.49)) ;
#169550=CARTESIAN_POINT('Origin',(2.5,2.85,-35.94)) ;
#169551=CARTESIAN_POINT('Origin',(2.5,2.85,-35.94)) ;
#169552=CARTESIAN_POINT('Origin',(2.5,2.85,-35.74)) ;
#169553=CARTESIAN_POINT('Origin',(2.5,4.45,-36.59)) ;
#169554=CARTESIAN_POINT('Origin',(2.5,4.45,-35.94)) ;
#169555=CARTESIAN_POINT('Origin',(2.5,-1.51907484122731,-35.94)) ;
#169556=CARTESIAN_POINT('Origin',(2.5,4.45,-35.94)) ;
#169557=CARTESIAN_POINT('Origin',(3.6,2.85,-35.74)) ;
#169558=CARTESIAN_POINT('Ctrl Pts',(1.8493242008907,2.75,-35.74)) ;
#169559=CARTESIAN_POINT('Ctrl Pts',(1.8489155297075,2.75,-35.7405602528665)) ;
#169560=CARTESIAN_POINT('Ctrl Pts',(1.84850693760105,2.75000414964412,-35.7411205835206)) ;
#169561=CARTESIAN_POINT('Ctrl Pts',(1.84774402267852,2.75001978545986,-35.7421661733315)) ;
#169562=CARTESIAN_POINT('Ctrl Pts',(1.84738978525535,2.75003021925998,-35.742651541288)) ;
#169563=CARTESIAN_POINT('Ctrl Pts',(1.84658906145061,2.75006109115737,-35.74374842884)) ;
#169564=CARTESIAN_POINT('Ctrl Pts',(1.84614254888567,2.75008342791642,-35.744359920497)) ;
#169565=CARTESIAN_POINT('Ctrl Pts',(1.84498586912391,2.75015481704799,-35.7459435779958)) ;
#169566=CARTESIAN_POINT('Ctrl Pts',(1.84427568281904,2.75021186472549,-35.746915537535)) ;
#169567=CARTESIAN_POINT('Ctrl Pts',(1.84242877605317,2.75039562881422,-35.7494423274962)) ;
#169568=CARTESIAN_POINT('Ctrl Pts',(1.84129221873232,2.75054367055059,-35.7509964126165)) ;
#169569=CARTESIAN_POINT('Ctrl Pts',(1.83830538692966,2.75102873153648,-35.7550782232159)) ;
#169570=CARTESIAN_POINT('Ctrl Pts',(1.83645654188481,2.75142684996804,-35.7576027100469)) ;
#169571=CARTESIAN_POINT('Ctrl Pts',(1.83146008674514,2.75278026662635,-35.7644125156423)) ;
#169572=CARTESIAN_POINT('Ctrl Pts',(1.8283159214327,2.75393867343662,-35.7686876979924)) ;
#169573=CARTESIAN_POINT('Ctrl Pts',(1.82163255793241,2.7571078032997,-35.7777453775413)) ;
#169574=CARTESIAN_POINT('Ctrl Pts',(1.81811360872654,2.75921511002117,-35.7824849484117)) ;
#169575=CARTESIAN_POINT('Ctrl Pts',(1.81342675453064,2.76262639234437,-35.7887744415142)) ;
#169576=CARTESIAN_POINT('Ctrl Pts',(1.81216355883267,2.76360925975736,-35.7904674024384)) ;
#169577=CARTESIAN_POINT('Ctrl Pts',(1.80949588405405,2.76581971270449,-35.7940412672837)) ;
#169578=CARTESIAN_POINT('Ctrl Pts',(1.80809008635136,2.76706812937485,-35.7959240633996)) ;
#169579=CARTESIAN_POINT('Ctrl Pts',(1.80622180825287,2.76884047115884,-35.7984273163076)) ;
#169580=CARTESIAN_POINT('Ctrl Pts',(1.80574460306297,2.76930303796754,-35.7990667849892)) ;
#169581=CARTESIAN_POINT('Ctrl Pts',(1.8020072303246,2.77301004154989,-35.8040760810937)) ;
#169582=CARTESIAN_POINT('Ctrl Pts',(1.79893605118154,2.77655328823594,-35.8081869819183)) ;
#169583=CARTESIAN_POINT('Ctrl Pts',(1.79553848385938,2.78126766498699,-35.8127195282098)) ;
#169584=CARTESIAN_POINT('Ctrl Pts',(1.79508624826463,2.78191247648142,-35.813322487166)) ;
#169585=CARTESIAN_POINT('Ctrl Pts',(1.79248502865789,2.78572620110035,-35.8167883578142)) ;
#169586=CARTESIAN_POINT('Ctrl Pts',(1.79047061583886,2.7890829265238,-35.8194451149791)) ;
#169587=CARTESIAN_POINT('Ctrl Pts',(1.78802866333258,2.79371407639528,-35.8226702366014)) ;
#169588=CARTESIAN_POINT('Ctrl Pts',(1.78745102314761,2.7948573048606,-35.8234336014307)) ;
#169589=CARTESIAN_POINT('Ctrl Pts',(1.78677268033909,2.79625836238382,-35.8243322112889)) ;
#169590=CARTESIAN_POINT('Ctrl Pts',(1.78665445068052,2.79650484960405,-35.8244889072897)) ;
#169591=CARTESIAN_POINT('Ctrl Pts',(1.78451055395601,2.80101773866204,-35.8273319791621)) ;
#169592=CARTESIAN_POINT('Ctrl Pts',(1.78263897914008,2.80562493737592,-35.8298097275576)) ;
#169593=CARTESIAN_POINT('Ctrl Pts',(1.78021555250218,2.8131601371182,-35.8330108372395)) ;
#169594=CARTESIAN_POINT('Ctrl Pts',(1.77953359820565,2.81552321764106,-35.8339042399272)) ;
#169595=CARTESIAN_POINT('Ctrl Pts',(1.77885922502008,2.81814935429725,-35.8347924283505)) ;
#169596=CARTESIAN_POINT('Ctrl Pts',(1.77880145893001,2.81837682960042,-35.8348685024872)) ;
#169597=CARTESIAN_POINT('Ctrl Pts',(1.77779807199381,2.8223725993423,-35.8361897865139)) ;
#169598=CARTESIAN_POINT('Ctrl Pts',(1.77701280317414,2.82627116869043,-35.837221156511)) ;
#169599=CARTESIAN_POINT('Ctrl Pts',(1.77629130352191,2.83098366045554,-35.83816931204)) ;
#169600=CARTESIAN_POINT('Ctrl Pts',(1.77618324871506,2.83173306513677,-35.8383113339465)) ;
#169601=CARTESIAN_POINT('Ctrl Pts',(1.77598237323328,2.83321827741191,-35.838575453052)) ;
#169602=CARTESIAN_POINT('Ctrl Pts',(1.77588933458808,2.83395373307725,-35.8386979039347)) ;
#169603=CARTESIAN_POINT('Ctrl Pts',(1.77526822780854,2.83923120109982,-35.839516785743)) ;
#169604=CARTESIAN_POINT('Ctrl Pts',(1.77496841680888,2.84387001846842,-35.8399177608516)) ;
#169605=CARTESIAN_POINT('Ctrl Pts',(1.77490988945624,2.84900075666618,-35.8399961754232)) ;
#169606=CARTESIAN_POINT('Ctrl Pts',(1.77490703981929,2.8495004656413,-35.84)) ;
#169607=CARTESIAN_POINT('Ctrl Pts',(1.77490703981929,2.85,-35.84)) ;
#169608=CARTESIAN_POINT('Origin',(2.5,4.45,-35.94)) ;
#169609=CARTESIAN_POINT('Origin',(2.5,4.45,-35.94)) ;
#169610=CARTESIAN_POINT('Ctrl Pts',(1.77500103713014,2.85,-35.839999931521)) ;
#169611=CARTESIAN_POINT('Ctrl Pts',(1.63636532444071,2.84999999999999,-35.8402019295526)) ;
#169612=CARTESIAN_POINT('Ctrl Pts',(1.72549327481619,2.85,-35.7340128995261)) ;
#169613=CARTESIAN_POINT('Ctrl Pts',(1.775003672721,2.83840140237647,-35.83999996665)) ;
#169614=CARTESIAN_POINT('Ctrl Pts',(1.63647653558524,2.80016011611086,-35.8401502081412)) ;
#169615=CARTESIAN_POINT('Ctrl Pts',(1.72549488713563,2.8384005084226,-35.7340109198666)) ;
#169616=CARTESIAN_POINT('Ctrl Pts',(1.77656595559297,2.82767268181592,-35.837937333125)) ;
#169617=CARTESIAN_POINT('Ctrl Pts',(1.66487156423554,2.77372961894301,-35.8269406617147)) ;
#169618=CARTESIAN_POINT('Ctrl Pts',(1.72805121738616,2.82767128774606,-35.7341715076455)) ;
#169619=CARTESIAN_POINT('Ctrl Pts',(1.78107127365223,2.80963025017428,-35.8319811709515)) ;
#169620=CARTESIAN_POINT('Ctrl Pts',(1.7078319145322,2.75028955033669,-35.8069390197619)) ;
#169621=CARTESIAN_POINT('Ctrl Pts',(1.73543500606493,2.80962842221856,-35.7346185213022)) ;
#169622=CARTESIAN_POINT('Ctrl Pts',(1.78389779708652,2.80236854329887,-35.8282458892004)) ;
#169623=CARTESIAN_POINT('Ctrl Pts',(1.72405887077374,2.74863416898561,-35.7993766027639)) ;
#169624=CARTESIAN_POINT('Ctrl Pts',(1.7400684743322,2.80236673746756,-35.7348898223597)) ;
#169625=CARTESIAN_POINT('Ctrl Pts',(1.79303410435281,2.78344495542395,-35.8161243202616)) ;
#169626=CARTESIAN_POINT('Ctrl Pts',(1.75831223057316,2.7462997480749,-35.7833824330224)) ;
#169627=CARTESIAN_POINT('Ctrl Pts',(1.75509542206186,2.7834434444138,-35.7357496723872)) ;
#169628=CARTESIAN_POINT('Ctrl Pts',(1.79978086064413,2.77501182458606,-35.8071352730534)) ;
#169629=CARTESIAN_POINT('Ctrl Pts',(1.77349404839604,2.74800701225899,-35.7762550668971)) ;
#169630=CARTESIAN_POINT('Ctrl Pts',(1.7662373444394,2.775010621185,-35.7363505791766)) ;
#169631=CARTESIAN_POINT('Ctrl Pts',(1.82062092254039,2.75520283445682,-35.7791823423359)) ;
#169632=CARTESIAN_POINT('Ctrl Pts',(1.80915747696825,2.74970830577378,-35.7594018394234)) ;
#169633=CARTESIAN_POINT('Ctrl Pts',(1.80086136857318,2.75520254410104,-35.7380912776554)) ;
#169634=CARTESIAN_POINT('Ctrl Pts',(1.83487464178854,2.75,-35.759840908673)) ;
#169635=CARTESIAN_POINT('Ctrl Pts',(1.82921773450097,2.75,-35.7497824526971)) ;
#169636=CARTESIAN_POINT('Ctrl Pts',(1.82479494488362,2.75,-35.739125428875)) ;
#169637=CARTESIAN_POINT('Ctrl Pts',(1.8493242008907,2.75,-35.74)) ;
#169638=CARTESIAN_POINT('Ctrl Pts',(1.8493242008907,2.75,-35.74)) ;
#169639=CARTESIAN_POINT('Ctrl Pts',(1.8493242008907,2.75,-35.74)) ;
#169640=CARTESIAN_POINT('Origin',(2.6,4.45,-35.94)) ;
#169641=CARTESIAN_POINT('Ctrl Pts',(1.27790541830591,2.85,-32.4381204689935)) ;
#169642=CARTESIAN_POINT('Ctrl Pts',(1.20082240333961,2.85,-32.3849999999998)) ;
#169643=CARTESIAN_POINT('Ctrl Pts',(1.27790541830602,2.85,-32.3318795310064)) ;
#169644=CARTESIAN_POINT('Ctrl Pts',(1.27790638186138,2.84083632349969,-32.4381211409614)) ;
#169645=CARTESIAN_POINT('Ctrl Pts',(1.20084678242026,2.82796155786835,-32.3849999999998)) ;
#169646=CARTESIAN_POINT('Ctrl Pts',(1.27790638186151,2.84083632349971,-32.3318788590386)) ;
#169647=CARTESIAN_POINT('Ctrl Pts',(1.27916908278627,2.83184203564912,-32.4374245856051)) ;
#169648=CARTESIAN_POINT('Ctrl Pts',(1.20941464972047,2.80875345001339,-32.3849999999999)) ;
#169649=CARTESIAN_POINT('Ctrl Pts',(1.27916908278638,2.83184203564916,-32.3325754143948)) ;
#169650=CARTESIAN_POINT('Ctrl Pts',(1.28359729368254,2.81532455354034,-32.4349858093441)) ;
#169651=CARTESIAN_POINT('Ctrl Pts',(1.23205483118169,2.78149692488717,-32.3849999999998)) ;
#169652=CARTESIAN_POINT('Ctrl Pts',(1.28359729368263,2.8153245535404,-32.3350141906558)) ;
#169653=CARTESIAN_POINT('Ctrl Pts',(1.28669991111207,2.80791239452539,-32.4332816433158)) ;
#169654=CARTESIAN_POINT('Ctrl Pts',(1.24464080060876,2.7734468891291,-32.385)) ;
#169655=CARTESIAN_POINT('Ctrl Pts',(1.28669991111214,2.80791239452546,-32.3367183566841)) ;
#169656=CARTESIAN_POINT('Ctrl Pts',(1.29736892768575,2.78833251591434,-32.4274284096738)) ;
#169657=CARTESIAN_POINT('Ctrl Pts',(1.27602012126336,2.75841927526786,-32.385)) ;
#169658=CARTESIAN_POINT('Ctrl Pts',(1.29736892768578,2.78833251591441,-32.3425715903261)) ;
#169659=CARTESIAN_POINT('Ctrl Pts',(1.30626047349815,2.77861339289525,-32.4225706455934)) ;
#169660=CARTESIAN_POINT('Ctrl Pts',(1.29330467011166,2.75582184841473,-32.385)) ;
#169661=CARTESIAN_POINT('Ctrl Pts',(1.30626047349817,2.77861339289531,-32.3474293544066)) ;
#169662=CARTESIAN_POINT('Ctrl Pts',(1.3341796818893,2.75637252911125,-32.4073970793052)) ;
#169663=CARTESIAN_POINT('Ctrl Pts',(1.33261582998958,2.75058962148775,-32.3849999999999)) ;
#169664=CARTESIAN_POINT('Ctrl Pts',(1.3341796818893,2.75637252911127,-32.3626029206948)) ;
#169665=CARTESIAN_POINT('Ctrl Pts',(1.35520432073838,2.75,-32.3960818608403)) ;
#169666=CARTESIAN_POINT('Ctrl Pts',(1.35468704305008,2.75,-32.385)) ;
#169667=CARTESIAN_POINT('Ctrl Pts',(1.35520432073834,2.75,-32.3739181391598)) ;
#169668=CARTESIAN_POINT('Ctrl Pts',(1.37603597336698,2.75,-32.385)) ;
#169669=CARTESIAN_POINT('Ctrl Pts',(1.37603597336698,2.75,-32.385)) ;
#169670=CARTESIAN_POINT('Ctrl Pts',(1.37603597336698,2.75,-32.385)) ;
#169671=CARTESIAN_POINT('Origin',(-5.84812080916424E-16,4.45,-34.29)) ;
#169672=CARTESIAN_POINT('Ctrl Pts',(1.27790541830602,2.85,-28.6281204689936)) ;
#169673=CARTESIAN_POINT('Ctrl Pts',(1.20082240333942,2.85,-28.575)) ;
#169674=CARTESIAN_POINT('Ctrl Pts',(1.27790541830602,2.85,-28.5218795310064)) ;
#169675=CARTESIAN_POINT('Ctrl Pts',(1.2779063818615,2.8408363234997,-28.6281211409615)) ;
#169676=CARTESIAN_POINT('Ctrl Pts',(1.20084678242003,2.82796155786832,-28.575)) ;
#169677=CARTESIAN_POINT('Ctrl Pts',(1.2779063818615,2.84083632349971,-28.5218788590386)) ;
#169678=CARTESIAN_POINT('Ctrl Pts',(1.27916908278636,2.83184203564916,-28.6274245856052)) ;
#169679=CARTESIAN_POINT('Ctrl Pts',(1.2094146497203,2.80875345001334,-28.575)) ;
#169680=CARTESIAN_POINT('Ctrl Pts',(1.27916908278637,2.83184203564916,-28.5225754143948)) ;
#169681=CARTESIAN_POINT('Ctrl Pts',(1.28359729368261,2.81532455354039,-28.6249858093442)) ;
#169682=CARTESIAN_POINT('Ctrl Pts',(1.23205483118158,2.78149692488709,-28.575)) ;
#169683=CARTESIAN_POINT('Ctrl Pts',(1.28359729368262,2.81532455354039,-28.5250141906558)) ;
#169684=CARTESIAN_POINT('Ctrl Pts',(1.28669991111214,2.80791239452546,-28.6232816433159)) ;
#169685=CARTESIAN_POINT('Ctrl Pts',(1.24464080060866,2.77344688912903,-28.575)) ;
#169686=CARTESIAN_POINT('Ctrl Pts',(1.28669991111214,2.80791239452546,-28.5267183566841)) ;
#169687=CARTESIAN_POINT('Ctrl Pts',(1.29736892768578,2.7883325159144,-28.6174284096739)) ;
#169688=CARTESIAN_POINT('Ctrl Pts',(1.27602012126333,2.75841927526782,-28.575)) ;
#169689=CARTESIAN_POINT('Ctrl Pts',(1.29736892768579,2.7883325159144,-28.5325715903261)) ;
#169690=CARTESIAN_POINT('Ctrl Pts',(1.30626047349817,2.7786133928953,-28.6125706455934)) ;
#169691=CARTESIAN_POINT('Ctrl Pts',(1.29330467011163,2.75582184841469,-28.575)) ;
#169692=CARTESIAN_POINT('Ctrl Pts',(1.30626047349816,2.7786133928953,-28.5374293544066)) ;
#169693=CARTESIAN_POINT('Ctrl Pts',(1.33417968188929,2.75637252911127,-28.5973970793052)) ;
#169694=CARTESIAN_POINT('Ctrl Pts',(1.33261582998957,2.75058962148775,-28.575)) ;
#169695=CARTESIAN_POINT('Ctrl Pts',(1.3341796818893,2.75637252911127,-28.5526029206948)) ;
#169696=CARTESIAN_POINT('Ctrl Pts',(1.35520432073835,2.75,-28.5860818608403)) ;
#169697=CARTESIAN_POINT('Ctrl Pts',(1.35468704305008,2.75,-28.575)) ;
#169698=CARTESIAN_POINT('Ctrl Pts',(1.35520432073834,2.75,-28.5639181391598)) ;
#169699=CARTESIAN_POINT('Ctrl Pts',(1.37603597336697,2.75,-28.575)) ;
#169700=CARTESIAN_POINT('Ctrl Pts',(1.37603597336697,2.75,-28.575)) ;
#169701=CARTESIAN_POINT('Ctrl Pts',(1.37603597336697,2.75,-28.575)) ;
#169702=CARTESIAN_POINT('Origin',(-5.84812080916424E-16,4.45,-30.48)) ;
#169703=CARTESIAN_POINT('Ctrl Pts',(1.27790541830606,2.85,-24.8181204689937)) ;
#169704=CARTESIAN_POINT('Ctrl Pts',(1.20082240333964,2.85,-24.7650000000002)) ;
#169705=CARTESIAN_POINT('Ctrl Pts',(1.27790541830584,2.85,-24.7118795310066)) ;
#169706=CARTESIAN_POINT('Ctrl Pts',(1.27790638186154,2.84083632349972,-24.8181211409614)) ;
#169707=CARTESIAN_POINT('Ctrl Pts',(1.20084678242024,2.82796155786836,-24.7650000000002)) ;
#169708=CARTESIAN_POINT('Ctrl Pts',(1.27790638186134,2.84083632349968,-24.7118788590387)) ;
#169709=CARTESIAN_POINT('Ctrl Pts',(1.27916908278641,2.83184203564917,-24.8174245856052)) ;
#169710=CARTESIAN_POINT('Ctrl Pts',(1.20941464972049,2.8087534500134,-24.7650000000002)) ;
#169711=CARTESIAN_POINT('Ctrl Pts',(1.27916908278621,2.8318420356491,-24.7125754143949)) ;
#169712=CARTESIAN_POINT('Ctrl Pts',(1.28359729368265,2.81532455354041,-24.8149858093442)) ;
#169713=CARTESIAN_POINT('Ctrl Pts',(1.2320548311817,2.78149692488718,-24.7650000000002)) ;
#169714=CARTESIAN_POINT('Ctrl Pts',(1.28359729368249,2.8153245535403,-24.715014190656)) ;
#169715=CARTESIAN_POINT('Ctrl Pts',(1.28669991111217,2.80791239452549,-24.8132816433159)) ;
#169716=CARTESIAN_POINT('Ctrl Pts',(1.24464080060876,2.77344688912911,-24.7650000000002)) ;
#169717=CARTESIAN_POINT('Ctrl Pts',(1.28669991111203,2.80791239452536,-24.7167183566842)) ;
#169718=CARTESIAN_POINT('Ctrl Pts',(1.2973689276858,2.78833251591442,-24.807428409674)) ;
#169719=CARTESIAN_POINT('Ctrl Pts',(1.27602012126337,2.75841927526789,-24.7650000000001)) ;
#169720=CARTESIAN_POINT('Ctrl Pts',(1.29736892768571,2.78833251591431,-24.7225715903263)) ;
#169721=CARTESIAN_POINT('Ctrl Pts',(1.30626047349817,2.77861339289533,-24.8025706455935)) ;
#169722=CARTESIAN_POINT('Ctrl Pts',(1.29330467011166,2.75582184841473,-24.7650000000001)) ;
#169723=CARTESIAN_POINT('Ctrl Pts',(1.30626047349813,2.77861339289522,-24.7274293544067)) ;
#169724=CARTESIAN_POINT('Ctrl Pts',(1.3341796818893,2.75637252911125,-24.7873970793052)) ;
#169725=CARTESIAN_POINT('Ctrl Pts',(1.33261582998957,2.75058962148776,-24.765)) ;
#169726=CARTESIAN_POINT('Ctrl Pts',(1.33417968188928,2.75637252911127,-24.7426029206948)) ;
#169727=CARTESIAN_POINT('Ctrl Pts',(1.35520432073831,2.75,-24.7760818608402)) ;
#169728=CARTESIAN_POINT('Ctrl Pts',(1.35468704305007,2.75,-24.7649999999999)) ;
#169729=CARTESIAN_POINT('Ctrl Pts',(1.3552043207384,2.75,-24.7539181391597)) ;
#169730=CARTESIAN_POINT('Ctrl Pts',(1.37603597336698,2.75,-24.765)) ;
#169731=CARTESIAN_POINT('Ctrl Pts',(1.37603597336698,2.75,-24.765)) ;
#169732=CARTESIAN_POINT('Ctrl Pts',(1.37603597336698,2.75,-24.765)) ;
#169733=CARTESIAN_POINT('Origin',(-6.11095769946375E-16,4.45,-26.67)) ;
#169734=CARTESIAN_POINT('Ctrl Pts',(1.27790541830603,2.85,-21.0081204689936)) ;
#169735=CARTESIAN_POINT('Ctrl Pts',(1.20082240333942,2.85,-20.955)) ;
#169736=CARTESIAN_POINT('Ctrl Pts',(1.27790541830601,2.85,-20.9018795310064)) ;
#169737=CARTESIAN_POINT('Ctrl Pts',(1.27790638186151,2.84083632349971,-21.0081211409614)) ;
#169738=CARTESIAN_POINT('Ctrl Pts',(1.20084678242002,2.82796155786833,-20.955)) ;
#169739=CARTESIAN_POINT('Ctrl Pts',(1.2779063818615,2.84083632349971,-20.9018788590386)) ;
#169740=CARTESIAN_POINT('Ctrl Pts',(1.27916908278638,2.83184203564916,-21.0074245856052)) ;
#169741=CARTESIAN_POINT('Ctrl Pts',(1.2094146497203,2.80875345001334,-20.955)) ;
#169742=CARTESIAN_POINT('Ctrl Pts',(1.27916908278637,2.83184203564916,-20.9025754143948)) ;
#169743=CARTESIAN_POINT('Ctrl Pts',(1.28359729368262,2.8153245535404,-21.0049858093442)) ;
#169744=CARTESIAN_POINT('Ctrl Pts',(1.23205483118157,2.7814969248871,-20.955)) ;
#169745=CARTESIAN_POINT('Ctrl Pts',(1.2835972936826,2.81532455354039,-20.9050141906558)) ;
#169746=CARTESIAN_POINT('Ctrl Pts',(1.28669991111215,2.80791239452546,-21.0032816433159)) ;
#169747=CARTESIAN_POINT('Ctrl Pts',(1.24464080060865,2.77344688912904,-20.955)) ;
#169748=CARTESIAN_POINT('Ctrl Pts',(1.28669991111213,2.80791239452546,-20.9067183566841)) ;
#169749=CARTESIAN_POINT('Ctrl Pts',(1.29736892768578,2.7883325159144,-20.9974284096739)) ;
#169750=CARTESIAN_POINT('Ctrl Pts',(1.27602012126334,2.75841927526782,-20.955)) ;
#169751=CARTESIAN_POINT('Ctrl Pts',(1.29736892768577,2.7883325159144,-20.9125715903261)) ;
#169752=CARTESIAN_POINT('Ctrl Pts',(1.30626047349816,2.77861339289531,-20.9925706455934)) ;
#169753=CARTESIAN_POINT('Ctrl Pts',(1.29330467011164,2.75582184841469,-20.955)) ;
#169754=CARTESIAN_POINT('Ctrl Pts',(1.30626047349816,2.7786133928953,-20.9174293544066)) ;
#169755=CARTESIAN_POINT('Ctrl Pts',(1.33417968188929,2.75637252911127,-20.9773970793052)) ;
#169756=CARTESIAN_POINT('Ctrl Pts',(1.33261582998957,2.75058962148775,-20.955)) ;
#169757=CARTESIAN_POINT('Ctrl Pts',(1.33417968188929,2.75637252911127,-20.9326029206948)) ;
#169758=CARTESIAN_POINT('Ctrl Pts',(1.35520432073833,2.75,-20.9660818608402)) ;
#169759=CARTESIAN_POINT('Ctrl Pts',(1.35468704305007,2.75,-20.955)) ;
#169760=CARTESIAN_POINT('Ctrl Pts',(1.35520432073833,2.75,-20.9439181391598)) ;
#169761=CARTESIAN_POINT('Ctrl Pts',(1.37603597336697,2.75,-20.955)) ;
#169762=CARTESIAN_POINT('Ctrl Pts',(1.37603597336697,2.75,-20.955)) ;
#169763=CARTESIAN_POINT('Ctrl Pts',(1.37603597336697,2.75,-20.955)) ;
#169764=CARTESIAN_POINT('Origin',(-6.11095769946375E-16,4.45,-22.86)) ;
#169765=CARTESIAN_POINT('Ctrl Pts',(1.27790541830603,2.85,-17.1981204689936)) ;
#169766=CARTESIAN_POINT('Ctrl Pts',(1.20082240333937,2.85,-17.145)) ;
#169767=CARTESIAN_POINT('Ctrl Pts',(1.27790541830605,2.85,-17.0918795310064)) ;
#169768=CARTESIAN_POINT('Ctrl Pts',(1.2779063818615,2.84083632349971,-17.1981211409614)) ;
#169769=CARTESIAN_POINT('Ctrl Pts',(1.20084678241998,2.82796155786832,-17.145)) ;
#169770=CARTESIAN_POINT('Ctrl Pts',(1.27790638186153,2.84083632349972,-17.0918788590386)) ;
#169771=CARTESIAN_POINT('Ctrl Pts',(1.27916908278638,2.83184203564916,-17.1974245856052)) ;
#169772=CARTESIAN_POINT('Ctrl Pts',(1.20941464972025,2.80875345001333,-17.145)) ;
#169773=CARTESIAN_POINT('Ctrl Pts',(1.27916908278639,2.83184203564917,-17.0925754143947)) ;
#169774=CARTESIAN_POINT('Ctrl Pts',(1.28359729368262,2.8153245535404,-17.1949858093442)) ;
#169775=CARTESIAN_POINT('Ctrl Pts',(1.23205483118153,2.78149692488708,-17.145)) ;
#169776=CARTESIAN_POINT('Ctrl Pts',(1.28359729368264,2.81532455354041,-17.0950141906558)) ;
#169777=CARTESIAN_POINT('Ctrl Pts',(1.28669991111215,2.80791239452546,-17.1932816433159)) ;
#169778=CARTESIAN_POINT('Ctrl Pts',(1.24464080060863,2.77344688912901,-17.145)) ;
#169779=CARTESIAN_POINT('Ctrl Pts',(1.28669991111216,2.80791239452547,-17.096718356684)) ;
#169780=CARTESIAN_POINT('Ctrl Pts',(1.29736892768579,2.7883325159144,-17.1874284096739)) ;
#169781=CARTESIAN_POINT('Ctrl Pts',(1.27602012126332,2.75841927526781,-17.145)) ;
#169782=CARTESIAN_POINT('Ctrl Pts',(1.29736892768579,2.78833251591441,-17.1025715903261)) ;
#169783=CARTESIAN_POINT('Ctrl Pts',(1.30626047349816,2.7786133928953,-17.1825706455934)) ;
#169784=CARTESIAN_POINT('Ctrl Pts',(1.29330467011163,2.75582184841467,-17.145)) ;
#169785=CARTESIAN_POINT('Ctrl Pts',(1.30626047349817,2.77861339289531,-17.1074293544065)) ;
#169786=CARTESIAN_POINT('Ctrl Pts',(1.33417968188929,2.75637252911127,-17.1673970793052)) ;
#169787=CARTESIAN_POINT('Ctrl Pts',(1.33261582998957,2.75058962148775,-17.145)) ;
#169788=CARTESIAN_POINT('Ctrl Pts',(1.33417968188929,2.75637252911127,-17.1226029206948)) ;
#169789=CARTESIAN_POINT('Ctrl Pts',(1.35520432073833,2.75,-17.1560818608402)) ;
#169790=CARTESIAN_POINT('Ctrl Pts',(1.35468704305007,2.75,-17.145)) ;
#169791=CARTESIAN_POINT('Ctrl Pts',(1.35520432073832,2.75,-17.1339181391597)) ;
#169792=CARTESIAN_POINT('Ctrl Pts',(1.37603597336697,2.75,-17.145)) ;
#169793=CARTESIAN_POINT('Ctrl Pts',(1.37603597336697,2.75,-17.145)) ;
#169794=CARTESIAN_POINT('Ctrl Pts',(1.37603597336697,2.75,-17.145)) ;
#169795=CARTESIAN_POINT('Origin',(-6.11095769946375E-16,4.45,-19.05)) ;
#169796=CARTESIAN_POINT('Ctrl Pts',(1.27790541830539,2.85,-13.3881204689932)) ;
#169797=CARTESIAN_POINT('Ctrl Pts',(1.20082240333945,2.85,-13.3349999999987)) ;
#169798=CARTESIAN_POINT('Ctrl Pts',(1.27790541830662,2.85,-13.281879531006)) ;
#169799=CARTESIAN_POINT('Ctrl Pts',(1.27790638186088,2.84083632349961,-13.388121140961)) ;
#169800=CARTESIAN_POINT('Ctrl Pts',(1.20084678242006,2.82796155786833,-13.3349999999987)) ;
#169801=CARTESIAN_POINT('Ctrl Pts',(1.27790638186211,2.84083632349981,-13.2818788590381)) ;
#169802=CARTESIAN_POINT('Ctrl Pts',(1.27916908278578,2.83184203564898,-13.3874245856048)) ;
#169803=CARTESIAN_POINT('Ctrl Pts',(1.20941464972031,2.80875345001336,-13.3349999999987)) ;
#169804=CARTESIAN_POINT('Ctrl Pts',(1.27916908278694,2.83184203564935,-13.2825754143944)) ;
#169805=CARTESIAN_POINT('Ctrl Pts',(1.28359729368214,2.81532455354009,-13.3849858093437)) ;
#169806=CARTESIAN_POINT('Ctrl Pts',(1.23205483118158,2.7814969248871,-13.3349999999989)) ;
#169807=CARTESIAN_POINT('Ctrl Pts',(1.28359729368306,2.81532455354069,-13.2850141906554)) ;
#169808=CARTESIAN_POINT('Ctrl Pts',(1.28669991111174,2.80791239452513,-13.3832816433155)) ;
#169809=CARTESIAN_POINT('Ctrl Pts',(1.24464080060867,2.77344688912904,-13.334999999999)) ;
#169810=CARTESIAN_POINT('Ctrl Pts',(1.28669991111253,2.80791239452578,-13.2867183566837)) ;
#169811=CARTESIAN_POINT('Ctrl Pts',(1.29736892768555,2.78833251591408,-13.3774284096734)) ;
#169812=CARTESIAN_POINT('Ctrl Pts',(1.27602012126334,2.75841927526783,-13.3349999999992)) ;
#169813=CARTESIAN_POINT('Ctrl Pts',(1.297368927686,2.78833251591472,-13.2925715903257)) ;
#169814=CARTESIAN_POINT('Ctrl Pts',(1.30626047349801,2.77861339289504,-13.372570645593)) ;
#169815=CARTESIAN_POINT('Ctrl Pts',(1.29330467011163,2.75582184841469,-13.3349999999994)) ;
#169816=CARTESIAN_POINT('Ctrl Pts',(1.30626047349831,2.77861339289556,-13.2974293544061)) ;
#169817=CARTESIAN_POINT('Ctrl Pts',(1.33417968188927,2.75637252911119,-13.3573970793049)) ;
#169818=CARTESIAN_POINT('Ctrl Pts',(1.33261582998957,2.75058962148775,-13.3349999999997)) ;
#169819=CARTESIAN_POINT('Ctrl Pts',(1.33417968188932,2.75637252911135,-13.3126029206945)) ;
#169820=CARTESIAN_POINT('Ctrl Pts',(1.35520432073863,2.75,-13.3460818608407)) ;
#169821=CARTESIAN_POINT('Ctrl Pts',(1.35468704305008,2.75,-13.3350000000009)) ;
#169822=CARTESIAN_POINT('Ctrl Pts',(1.35520432073804,2.75,-13.3239181391602)) ;
#169823=CARTESIAN_POINT('Ctrl Pts',(1.37603597336697,2.75,-13.335)) ;
#169824=CARTESIAN_POINT('Ctrl Pts',(1.37603597336697,2.75,-13.335)) ;
#169825=CARTESIAN_POINT('Ctrl Pts',(1.37603597336697,2.75,-13.335)) ;
#169826=CARTESIAN_POINT('Origin',(-6.11095769946375E-16,4.45,-15.24)) ;
#169827=CARTESIAN_POINT('Ctrl Pts',(1.27790541830668,2.85,-9.57812046899406)) ;
#169828=CARTESIAN_POINT('Ctrl Pts',(1.20082240333937,2.85,-9.52500000000137)) ;
#169829=CARTESIAN_POINT('Ctrl Pts',(1.27790541830539,2.85,-9.47187953100683)) ;
#169830=CARTESIAN_POINT('Ctrl Pts',(1.27790638186216,2.84083632349982,-9.57812114096188)) ;
#169831=CARTESIAN_POINT('Ctrl Pts',(1.20084678241997,2.82796155786831,-9.52500000000138)) ;
#169832=CARTESIAN_POINT('Ctrl Pts',(1.27790638186088,2.8408363234996,-9.47187885903899)) ;
#169833=CARTESIAN_POINT('Ctrl Pts',(1.27916908278698,2.83184203564936,-9.57742458560567)) ;
#169834=CARTESIAN_POINT('Ctrl Pts',(1.20941464972025,2.80875345001332,-9.52500000000131)) ;
#169835=CARTESIAN_POINT('Ctrl Pts',(1.27916908278579,2.83184203564897,-9.47257541439522)) ;
#169836=CARTESIAN_POINT('Ctrl Pts',(1.2835972936831,2.81532455354072,-9.57498580934463)) ;
#169837=CARTESIAN_POINT('Ctrl Pts',(1.23205483118154,2.78149692488707,-9.52500000000116)) ;
#169838=CARTESIAN_POINT('Ctrl Pts',(1.28359729368215,2.81532455354009,-9.4750141906563)) ;
#169839=CARTESIAN_POINT('Ctrl Pts',(1.28669991111256,2.8079123945258,-9.5732816433164)) ;
#169840=CARTESIAN_POINT('Ctrl Pts',(1.24464080060864,2.77344688912901,-9.52500000000106)) ;
#169841=CARTESIAN_POINT('Ctrl Pts',(1.28669991111174,2.80791239452513,-9.47671835668456)) ;
#169842=CARTESIAN_POINT('Ctrl Pts',(1.29736892768603,2.78833251591475,-9.56742840967436)) ;
#169843=CARTESIAN_POINT('Ctrl Pts',(1.27602012126331,2.7584192752678,-9.52500000000082)) ;
#169844=CARTESIAN_POINT('Ctrl Pts',(1.29736892768555,2.78833251591409,-9.48257159032659)) ;
#169845=CARTESIAN_POINT('Ctrl Pts',(1.30626047349833,2.77861339289558,-9.56257064559391)) ;
#169846=CARTESIAN_POINT('Ctrl Pts',(1.29330467011162,2.75582184841468,-9.52500000000068)) ;
#169847=CARTESIAN_POINT('Ctrl Pts',(1.30626047349802,2.77861339289504,-9.48742935440699)) ;
#169848=CARTESIAN_POINT('Ctrl Pts',(1.33417968188932,2.75637252911135,-9.54739707930555)) ;
#169849=CARTESIAN_POINT('Ctrl Pts',(1.33261582998957,2.75058962148774,-9.52500000000034)) ;
#169850=CARTESIAN_POINT('Ctrl Pts',(1.33417968188927,2.75637252911119,-9.50260292069508)) ;
#169851=CARTESIAN_POINT('Ctrl Pts',(1.35520432073802,2.75,-9.53608186083978)) ;
#169852=CARTESIAN_POINT('Ctrl Pts',(1.35468704305008,2.75,-9.52499999999888)) ;
#169853=CARTESIAN_POINT('Ctrl Pts',(1.35520432073864,2.75,-9.51391813915931)) ;
#169854=CARTESIAN_POINT('Ctrl Pts',(1.37603597336697,2.75,-9.525)) ;
#169855=CARTESIAN_POINT('Ctrl Pts',(1.37603597336697,2.75,-9.525)) ;
#169856=CARTESIAN_POINT('Ctrl Pts',(1.37603597336697,2.75,-9.525)) ;
#169857=CARTESIAN_POINT('Origin',(-6.11095769946375E-16,4.45,-11.43)) ;
#169858=CARTESIAN_POINT('Ctrl Pts',(1.27790541830604,2.85,-5.76812046899362)) ;
#169859=CARTESIAN_POINT('Ctrl Pts',(1.2008224033394,2.85,-5.71500000000003)) ;
#169860=CARTESIAN_POINT('Ctrl Pts',(1.27790541830601,2.85,-5.6618795310064)) ;
#169861=CARTESIAN_POINT('Ctrl Pts',(1.27790638186153,2.84083632349971,-5.76812114096144)) ;
#169862=CARTESIAN_POINT('Ctrl Pts',(1.20084678242,2.82796155786832,-5.71500000000003)) ;
#169863=CARTESIAN_POINT('Ctrl Pts',(1.27790638186149,2.84083632349971,-5.66187885903858)) ;
#169864=CARTESIAN_POINT('Ctrl Pts',(1.2791690827864,2.83184203564917,-5.76742458560523)) ;
#169865=CARTESIAN_POINT('Ctrl Pts',(1.20941464972028,2.80875345001333,-5.71500000000003)) ;
#169866=CARTESIAN_POINT('Ctrl Pts',(1.27916908278636,2.83184203564915,-5.66257541439479)) ;
#169867=CARTESIAN_POINT('Ctrl Pts',(1.28359729368263,2.81532455354041,-5.76498580934417)) ;
#169868=CARTESIAN_POINT('Ctrl Pts',(1.23205483118156,2.78149692488708,-5.71500000000002)) ;
#169869=CARTESIAN_POINT('Ctrl Pts',(1.28359729368261,2.81532455354039,-5.66501419065585)) ;
#169870=CARTESIAN_POINT('Ctrl Pts',(1.28669991111216,2.80791239452547,-5.76328164331592)) ;
#169871=CARTESIAN_POINT('Ctrl Pts',(1.24464080060865,2.77344688912903,-5.71500000000002)) ;
#169872=CARTESIAN_POINT('Ctrl Pts',(1.28669991111214,2.80791239452545,-5.66671835668411)) ;
#169873=CARTESIAN_POINT('Ctrl Pts',(1.29736892768579,2.78833251591442,-5.7574284096739)) ;
#169874=CARTESIAN_POINT('Ctrl Pts',(1.27602012126332,2.75841927526781,-5.71500000000003)) ;
#169875=CARTESIAN_POINT('Ctrl Pts',(1.29736892768578,2.7883325159144,-5.67257159032613)) ;
#169876=CARTESIAN_POINT('Ctrl Pts',(1.30626047349817,2.77861339289532,-5.75257064559348)) ;
#169877=CARTESIAN_POINT('Ctrl Pts',(1.29330467011163,2.75582184841469,-5.71500000000003)) ;
#169878=CARTESIAN_POINT('Ctrl Pts',(1.30626047349816,2.77861339289529,-5.67742935440656)) ;
#169879=CARTESIAN_POINT('Ctrl Pts',(1.3341796818893,2.75637252911126,-5.73739707930523)) ;
#169880=CARTESIAN_POINT('Ctrl Pts',(1.33261582998957,2.75058962148774,-5.71499999999999)) ;
#169881=CARTESIAN_POINT('Ctrl Pts',(1.33417968188929,2.75637252911128,-5.69260292069477)) ;
#169882=CARTESIAN_POINT('Ctrl Pts',(1.35520432073832,2.75,-5.72608186084025)) ;
#169883=CARTESIAN_POINT('Ctrl Pts',(1.35468704305008,2.75,-5.715)) ;
#169884=CARTESIAN_POINT('Ctrl Pts',(1.35520432073834,2.75,-5.70391813915977)) ;
#169885=CARTESIAN_POINT('Ctrl Pts',(1.37603597336697,2.75,-5.715)) ;
#169886=CARTESIAN_POINT('Ctrl Pts',(1.37603597336697,2.75,-5.715)) ;
#169887=CARTESIAN_POINT('Ctrl Pts',(1.37603597336697,2.75,-5.715)) ;
#169888=CARTESIAN_POINT('Origin',(2.5,-6.45,2.2)) ;
#169889=CARTESIAN_POINT('Origin',(2.5,-6.45,2.2)) ;
#169890=CARTESIAN_POINT('Origin',(-6.11095769946375E-16,4.45,-7.62)) ;
#169891=CARTESIAN_POINT('Origin',(2.5,1.95351742790181E-16,2.2)) ;
#169892=CARTESIAN_POINT('Origin',(2.5,1.9,2.2)) ;
#169893=CARTESIAN_POINT('Ctrl Pts',(1.27790541830603,2.85,-1.95812046899361)) ;
#169894=CARTESIAN_POINT('Ctrl Pts',(1.20082240333946,2.85,-1.90500000000004)) ;
#169895=CARTESIAN_POINT('Ctrl Pts',(1.27790541830599,2.85,-1.85187953100641)) ;
#169896=CARTESIAN_POINT('Ctrl Pts',(1.27790638186151,2.84083632349971,-1.95812114096143)) ;
#169897=CARTESIAN_POINT('Ctrl Pts',(1.20084678242005,2.82796155786833,-1.90500000000004)) ;
#169898=CARTESIAN_POINT('Ctrl Pts',(1.27790638186147,2.8408363234997,-1.85187885903859)) ;
#169899=CARTESIAN_POINT('Ctrl Pts',(1.27916908278637,2.83184203564916,-1.95742458560522)) ;
#169900=CARTESIAN_POINT('Ctrl Pts',(1.20941464972033,2.80875345001335,-1.90500000000003)) ;
#169901=CARTESIAN_POINT('Ctrl Pts',(1.27916908278634,2.83184203564916,-1.8525754143948)) ;
#169902=CARTESIAN_POINT('Ctrl Pts',(1.28359729368262,2.8153245535404,-1.95498580934416)) ;
#169903=CARTESIAN_POINT('Ctrl Pts',(1.23205483118159,2.78149692488712,-1.90500000000003)) ;
#169904=CARTESIAN_POINT('Ctrl Pts',(1.2835972936826,2.81532455354038,-1.85501419065586)) ;
#169905=CARTESIAN_POINT('Ctrl Pts',(1.28669991111215,2.80791239452546,-1.95328164331591)) ;
#169906=CARTESIAN_POINT('Ctrl Pts',(1.24464080060867,2.77344688912904,-1.90500000000002)) ;
#169907=CARTESIAN_POINT('Ctrl Pts',(1.28669991111213,2.80791239452544,-1.85671835668411)) ;
#169908=CARTESIAN_POINT('Ctrl Pts',(1.29736892768578,2.78833251591441,-1.94742840967388)) ;
#169909=CARTESIAN_POINT('Ctrl Pts',(1.27602012126333,2.75841927526783,-1.90500000000002)) ;
#169910=CARTESIAN_POINT('Ctrl Pts',(1.29736892768578,2.78833251591439,-1.86257159032615)) ;
#169911=CARTESIAN_POINT('Ctrl Pts',(1.30626047349816,2.7786133928953,-1.94257064559346)) ;
#169912=CARTESIAN_POINT('Ctrl Pts',(1.29330467011164,2.7558218484147,-1.90500000000002)) ;
#169913=CARTESIAN_POINT('Ctrl Pts',(1.30626047349816,2.77861339289529,-1.86742935440657)) ;
#169914=CARTESIAN_POINT('Ctrl Pts',(1.3341796818893,2.75637252911127,-1.92739707930523)) ;
#169915=CARTESIAN_POINT('Ctrl Pts',(1.33261582998958,2.75058962148774,-1.90500000000001)) ;
#169916=CARTESIAN_POINT('Ctrl Pts',(1.3341796818893,2.75637252911127,-1.88260292069479)) ;
#169917=CARTESIAN_POINT('Ctrl Pts',(1.35520432073833,2.75,-1.91608186084024)) ;
#169918=CARTESIAN_POINT('Ctrl Pts',(1.35468704305007,2.75,-1.90499999999995)) ;
#169919=CARTESIAN_POINT('Ctrl Pts',(1.35520432073834,2.75,-1.89391813915974)) ;
#169920=CARTESIAN_POINT('Ctrl Pts',(1.37603597336697,2.75,-1.905)) ;
#169921=CARTESIAN_POINT('Ctrl Pts',(1.37603597336697,2.75,-1.905)) ;
#169922=CARTESIAN_POINT('Ctrl Pts',(1.37603597336697,2.75,-1.905)) ;
#169923=CARTESIAN_POINT('Origin',(2.7,1.9,2.2)) ;
#169924=CARTESIAN_POINT('Origin',(2.7,2.1,2.2)) ;
#169925=CARTESIAN_POINT('Origin',(-6.11095769946375E-16,4.45,-3.81)) ;
#169926=CARTESIAN_POINT('Origin',(3.6,2.1,2.2)) ;
#169927=CARTESIAN_POINT('Origin',(3.5,2.1,2.2)) ;
#169928=CARTESIAN_POINT('Ctrl Pts',(1.72549266760237,2.85,1.44401362298495)) ;
#169929=CARTESIAN_POINT('Ctrl Pts',(1.63635891322671,2.84999999999999,1.55021272547567)) ;
#169930=CARTESIAN_POINT('Ctrl Pts',(1.77500605619934,2.85,1.54999992401279)) ;
#169931=CARTESIAN_POINT('Ctrl Pts',(1.72549428095344,2.83840024801823,1.44401164264682)) ;
#169932=CARTESIAN_POINT('Ctrl Pts',(1.63647013043005,2.80015695736268,1.55016100506938)) ;
#169933=CARTESIAN_POINT('Ctrl Pts',(1.77500868550276,2.83840278621153,1.54999996101813)) ;
#169934=CARTESIAN_POINT('Ctrl Pts',(1.72805074460438,2.82767088409066,1.44417220186092)) ;
#169935=CARTESIAN_POINT('Ctrl Pts',(1.66486766052525,2.77372556429602,1.53694944305648)) ;
#169936=CARTESIAN_POINT('Ctrl Pts',(1.7765703971759,2.82767482693174,1.54793777023085)) ;
#169937=CARTESIAN_POINT('Ctrl Pts',(1.73543475859394,2.80962789021929,1.44461916969382)) ;
#169938=CARTESIAN_POINT('Ctrl Pts',(1.70783084644936,2.75028582747794,1.5169449731166)) ;
#169939=CARTESIAN_POINT('Ctrl Pts',(1.78107476297284,2.80963307739335,1.54198236387663)) ;
#169940=CARTESIAN_POINT('Ctrl Pts',(1.74006831828865,2.80236621373356,1.44489045092167)) ;
#169941=CARTESIAN_POINT('Ctrl Pts',(1.72405853320849,2.74863106820581,1.50938157302589)) ;
#169942=CARTESIAN_POINT('Ctrl Pts',(1.78390089653206,2.80237132662259,1.53824738439477)) ;
#169943=CARTESIAN_POINT('Ctrl Pts',(1.75509546017965,2.7834430043054,1.44575023678366)) ;
#169944=CARTESIAN_POINT('Ctrl Pts',(1.75831280076438,2.74629798483364,1.493385578669)) ;
#169945=CARTESIAN_POINT('Ctrl Pts',(1.79303629065941,2.78344729439355,1.52612638181377)) ;
#169946=CARTESIAN_POINT('Ctrl Pts',(1.76623743827936,2.77501027199624,1.44635109519364)) ;
#169947=CARTESIAN_POINT('Ctrl Pts',(1.77349470226536,2.74800583767983,1.48625751636957)) ;
#169948=CARTESIAN_POINT('Ctrl Pts',(1.79978266704186,2.77501368038732,1.5171373950458)) ;
#169949=CARTESIAN_POINT('Ctrl Pts',(1.80086149668306,2.75520245925894,1.44809160673599)) ;
#169950=CARTESIAN_POINT('Ctrl Pts',(1.80915794598981,2.74970810565007,1.46940296260367)) ;
#169951=CARTESIAN_POINT('Ctrl Pts',(1.82062186326967,2.75520328537396,1.48918396557833)) ;
#169952=CARTESIAN_POINT('Ctrl Pts',(1.82479501616833,2.75,1.4491256009755)) ;
#169953=CARTESIAN_POINT('Ctrl Pts',(1.82921797033105,2.75,1.45978299211575)) ;
#169954=CARTESIAN_POINT('Ctrl Pts',(1.83487512614628,2.75,1.46984177015833)) ;
#169955=CARTESIAN_POINT('Ctrl Pts',(1.84932420089069,2.75,1.45)) ;
#169956=CARTESIAN_POINT('Ctrl Pts',(1.84932420089069,2.75,1.45)) ;
#169957=CARTESIAN_POINT('Ctrl Pts',(1.84932420089069,2.75,1.45)) ;
#169958=CARTESIAN_POINT('Ctrl Pts',(1.84932420089069,2.75,1.45)) ;
#169959=CARTESIAN_POINT('Ctrl Pts',(1.84891552970751,2.75,1.45056025286656)) ;
#169960=CARTESIAN_POINT('Ctrl Pts',(1.84850693760102,2.7500041496442,1.45112058352057)) ;
#169961=CARTESIAN_POINT('Ctrl Pts',(1.8477440226785,2.75001978546022,1.45216617333146)) ;
#169962=CARTESIAN_POINT('Ctrl Pts',(1.84738978525535,2.75003021926051,1.45265154128796)) ;
#169963=CARTESIAN_POINT('Ctrl Pts',(1.84658906145061,2.75006109115841,1.45374842884002)) ;
#169964=CARTESIAN_POINT('Ctrl Pts',(1.84614254888567,2.75008342791781,1.45435992049693)) ;
#169965=CARTESIAN_POINT('Ctrl Pts',(1.84498586912392,2.75015481705042,1.45594357799571)) ;
#169966=CARTESIAN_POINT('Ctrl Pts',(1.84427568281905,2.7502118647287,1.45691553753491)) ;
#169967=CARTESIAN_POINT('Ctrl Pts',(1.84242877605322,2.75039562881963,1.45944232749581)) ;
#169968=CARTESIAN_POINT('Ctrl Pts',(1.84129221873239,2.75054367055756,1.46099641261588)) ;
#169969=CARTESIAN_POINT('Ctrl Pts',(1.83830538692981,2.7510287315475,1.46507822321451)) ;
#169970=CARTESIAN_POINT('Ctrl Pts',(1.83645654188491,2.75142684998139,1.46760271004466)) ;
#169971=CARTESIAN_POINT('Ctrl Pts',(1.83146008674453,2.7527802666469,1.47441251564823)) ;
#169972=CARTESIAN_POINT('Ctrl Pts',(1.82831592143432,2.75393867345932,1.47868769799754)) ;
#169973=CARTESIAN_POINT('Ctrl Pts',(1.82163255789315,2.75710780333614,1.48774537759201)) ;
#169974=CARTESIAN_POINT('Ctrl Pts',(1.81811360864768,2.75921511008005,1.49248494851376)) ;
#169975=CARTESIAN_POINT('Ctrl Pts',(1.81342675445606,2.76262639240882,1.49877444161403)) ;
#169976=CARTESIAN_POINT('Ctrl Pts',(1.81216355879702,2.76360925979239,1.50046740248774)) ;
#169977=CARTESIAN_POINT('Ctrl Pts',(1.80949588405725,2.76581971270697,1.50404126728569)) ;
#169978=CARTESIAN_POINT('Ctrl Pts',(1.80809008635459,2.76706812937679,1.50592406340246)) ;
#169979=CARTESIAN_POINT('Ctrl Pts',(1.80622180825451,2.76884047116021,1.50842731630949)) ;
#169980=CARTESIAN_POINT('Ctrl Pts',(1.80574460306458,2.76930303796854,1.50906678499061)) ;
#169981=CARTESIAN_POINT('Ctrl Pts',(1.80200723031206,2.77301004156286,1.51407608111113)) ;
#169982=CARTESIAN_POINT('Ctrl Pts',(1.79893605115733,2.77655328826388,1.51818698195081)) ;
#169983=CARTESIAN_POINT('Ctrl Pts',(1.7955384838363,2.78126766501987,1.52271952824054)) ;
#169984=CARTESIAN_POINT('Ctrl Pts',(1.79508624825315,2.78191247649822,1.5233224871813)) ;
#169985=CARTESIAN_POINT('Ctrl Pts',(1.79248502865803,2.7857262011001,1.52678835781394)) ;
#169986=CARTESIAN_POINT('Ctrl Pts',(1.79047061583915,2.78908292652327,1.52944511497864)) ;
#169987=CARTESIAN_POINT('Ctrl Pts',(1.78802866333285,2.79371407639472,1.53267023660098)) ;
#169988=CARTESIAN_POINT('Ctrl Pts',(1.78745102314773,2.79485730486032,1.53343360143046)) ;
#169989=CARTESIAN_POINT('Ctrl Pts',(1.78677268033907,2.79625836238383,1.53433221128893)) ;
#169990=CARTESIAN_POINT('Ctrl Pts',(1.7866544506805,2.79650484960406,1.53448890728973)) ;
#169991=CARTESIAN_POINT('Ctrl Pts',(1.78451055395599,2.80101773866206,1.53733197916208)) ;
#169992=CARTESIAN_POINT('Ctrl Pts',(1.78263897914004,2.80562493737595,1.53980972755757)) ;
#169993=CARTESIAN_POINT('Ctrl Pts',(1.78021555250215,2.81316013711825,1.54301083723955)) ;
#169994=CARTESIAN_POINT('Ctrl Pts',(1.77953359820562,2.81552321764108,1.54390423992715)) ;
#169995=CARTESIAN_POINT('Ctrl Pts',(1.77885922502006,2.81814935429725,1.54479242835053)) ;
#169996=CARTESIAN_POINT('Ctrl Pts',(1.77880145892999,2.81837682960042,1.54486850248715)) ;
#169997=CARTESIAN_POINT('Ctrl Pts',(1.77779807199376,2.82237259934244,1.54618978651394)) ;
#169998=CARTESIAN_POINT('Ctrl Pts',(1.77701280317407,2.82627116869071,1.54722115651107)) ;
#169999=CARTESIAN_POINT('Ctrl Pts',(1.77629130352184,2.83098366045584,1.54816931204003)) ;
#170000=CARTESIAN_POINT('Ctrl Pts',(1.77618324871501,2.83173306513696,1.54831133394653)) ;
#170001=CARTESIAN_POINT('Ctrl Pts',(1.77598237323325,2.83321827741197,1.54857545305202)) ;
#170002=CARTESIAN_POINT('Ctrl Pts',(1.77588933458805,2.83395373307728,1.54869790393466)) ;
#170003=CARTESIAN_POINT('Ctrl Pts',(1.77526822780851,2.83923120109988,1.549516785743)) ;
#170004=CARTESIAN_POINT('Ctrl Pts',(1.77496841680885,2.84387001846854,1.54991776085168)) ;
#170005=CARTESIAN_POINT('Ctrl Pts',(1.77490988945622,2.8490007566663,1.54999617542323)) ;
#170006=CARTESIAN_POINT('Ctrl Pts',(1.77490703981927,2.84950046564136,1.55)) ;
#170007=CARTESIAN_POINT('Ctrl Pts',(1.77490703981927,2.85,1.55)) ;
#170008=CARTESIAN_POINT('Origin',(3.5,2.1,2.2)) ;
#170009=CARTESIAN_POINT('Origin',(3.5,2.1,2.2)) ;
#170010=CARTESIAN_POINT('Origin',(-6.11095769946375E-16,4.45,0.)) ;
#170011=CARTESIAN_POINT('Origin',(3.6,2.85,1.45)) ;
#170012=CARTESIAN_POINT('Origin',(2.5,2.85,1.45)) ;
#170013=CARTESIAN_POINT('Origin',(3.5,7.81406971160724E-17,2.2)) ;
#170014=CARTESIAN_POINT('Origin',(3.5,2.65,2.2)) ;
#170015=CARTESIAN_POINT('Origin',(2.5,2.85,1.65)) ;
#170016=CARTESIAN_POINT('Origin',(2.5,2.85,1.65)) ;
#170017=CARTESIAN_POINT('Origin',(2.7,2.85,1.65)) ;
#170018=CARTESIAN_POINT('Origin',(3.5,2.65,2.2)) ;
#170019=CARTESIAN_POINT('Origin',(3.5,2.65,2.2)) ;
#170020=CARTESIAN_POINT('Origin',(2.6,4.45,1.65)) ;
#170021=CARTESIAN_POINT('Origin',(2.5,4.45,1.65)) ;
#170022=CARTESIAN_POINT('Origin',(2.5,4.55,1.65)) ;
#170023=CARTESIAN_POINT('Origin',(2.5,4.45,1.65)) ;
#170024=CARTESIAN_POINT('Origin',(2.7,2.85,-2.3)) ;
#170025=CARTESIAN_POINT('Origin',(2.7,2.85,2.2)) ;
#170026=CARTESIAN_POINT('Origin',(-2.07072847357592E-16,2.65,2.2)) ;
#170027=CARTESIAN_POINT('Origin',(2.7,2.65,2.2)) ;
#170028=CARTESIAN_POINT('Origin',(2.5,4.45,1.65)) ;
#170029=CARTESIAN_POINT('Origin',(2.5,4.45,1.65)) ;
#170030=CARTESIAN_POINT('Origin',(2.7,2.85,2.2)) ;
#170031=CARTESIAN_POINT('Origin',(2.5,2.85,2.2)) ;
#170032=CARTESIAN_POINT('Origin',(2.5,4.45,-36.59)) ;
#170033=CARTESIAN_POINT('Origin',(2.5,4.45,2.2)) ;
#170034=CARTESIAN_POINT('Origin',(2.5,1.95351742790181E-16,2.2)) ;
#170035=CARTESIAN_POINT('Origin',(2.5,4.45,2.2)) ;
#170036=CARTESIAN_POINT('Origin',(2.5,4.45,2.2)) ;
#170037=CARTESIAN_POINT('Origin',(2.5,4.45,2.2)) ;
#170038=CARTESIAN_POINT('Origin',(-5.84812080916424E-16,4.45,2.2)) ;
#170039=CARTESIAN_POINT('Origin',(-3.9,4.45,2.2)) ;
#170040=CARTESIAN_POINT('Origin',(-3.9,4.45,2.2)) ;
#170041=CARTESIAN_POINT('Ctrl Pts',(-3.90000000000414,3.80333655664123,
2.22561598559544)) ;
#170042=CARTESIAN_POINT('Ctrl Pts',(-3.76707268212211,3.78931743308928,
2.17271399006788)) ;
#170043=CARTESIAN_POINT('Ctrl Pts',(-3.81330307515288,3.66391136972353,
2.22563750872074)) ;
#170044=CARTESIAN_POINT('Ctrl Pts',(-3.89100560487485,3.80613461936468,
2.23617464150095)) ;
#170045=CARTESIAN_POINT('Ctrl Pts',(-3.77789360990371,3.78258994157146,
2.17083996288935)) ;
#170046=CARTESIAN_POINT('Ctrl Pts',(-3.80681245874446,3.67074660187605,
2.23620282118099)) ;
#170047=CARTESIAN_POINT('Ctrl Pts',(-3.87638074624213,3.81068426137503,
2.24628380179591)) ;
#170048=CARTESIAN_POINT('Ctrl Pts',(-3.78564407609263,3.77777446969616,
2.18265796775152)) ;
#170049=CARTESIAN_POINT('Ctrl Pts',(-3.79626152405898,3.68185957735116,
2.24631352465829)) ;
#170050=CARTESIAN_POINT('Ctrl Pts',(-3.83745765067443,3.82279283247717,
2.26448677971421)) ;
#170051=CARTESIAN_POINT('Ctrl Pts',(-3.77926302941741,3.78175688793386,
2.2150310810483)) ;
#170052=CARTESIAN_POINT('Ctrl Pts',(-3.768189957662,3.71143369374476,2.2645135067643)) ;
#170053=CARTESIAN_POINT('Ctrl Pts',(-3.81315995987735,3.83035159193202,
2.27258505978673)) ;
#170054=CARTESIAN_POINT('Ctrl Pts',(-3.76758783470957,3.78902661367653,
2.23385461685646)) ;
#170055=CARTESIAN_POINT('Ctrl Pts',(-3.75066936002647,3.72989489134432,
2.27260743591321)) ;
#170056=CARTESIAN_POINT('Ctrl Pts',(-3.72961659401614,3.8563410660704,2.29258436202037)) ;
#170057=CARTESIAN_POINT('Ctrl Pts',(-3.71415009152798,3.82228860055657,
2.27828021342228)) ;
#170058=CARTESIAN_POINT('Ctrl Pts',(-3.69043468851351,3.79337198420934,
2.29259398868402)) ;
#170059=CARTESIAN_POINT('Ctrl Pts',(-3.65964870102201,3.87810735148093,
2.3)) ;
#170060=CARTESIAN_POINT('Ctrl Pts',(-3.6494577226055,3.86254752980597,2.3)) ;
#170061=CARTESIAN_POINT('Ctrl Pts',(-3.64000230097343,3.84653001401765,
2.3)) ;
#170062=CARTESIAN_POINT('Ctrl Pts',(-3.58927461283679,3.9,2.3)) ;
#170063=CARTESIAN_POINT('Ctrl Pts',(-3.58927461283679,3.9,2.3)) ;
#170064=CARTESIAN_POINT('Ctrl Pts',(-3.58927461283679,3.9,2.3)) ;
#170065=CARTESIAN_POINT('Origin',(-3.90000000000414,3.70667311328246,2.25123197119087)) ;
#170066=CARTESIAN_POINT('Ctrl Pts',(-3.81328428501083,3.66396238798774,
2.22561598559596)) ;
#170067=CARTESIAN_POINT('Ctrl Pts',(-3.7671555501966,3.78932617273336,2.17274696964475)) ;
#170068=CARTESIAN_POINT('Ctrl Pts',(-3.90000000000184,3.80333655664137,
2.22561598559596)) ;
#170069=CARTESIAN_POINT('Ctrl Pts',(-3.81816564857387,3.65881896296046,
2.21766737408028)) ;
#170070=CARTESIAN_POINT('Ctrl Pts',(-3.75960462691777,3.79067973806019,
2.17785299283591)) ;
#170071=CARTESIAN_POINT('Ctrl Pts',(-3.90338239924599,3.80123212475718,
2.21767478686741)) ;
#170072=CARTESIAN_POINT('Ctrl Pts',(-3.82087839357381,3.65609538274431,
2.20891956015985)) ;
#170073=CARTESIAN_POINT('Ctrl Pts',(-3.75388413987046,3.79211390479363,
2.1881053469697)) ;
#170074=CARTESIAN_POINT('Ctrl Pts',(-3.90529366494794,3.80014021273157,
2.20891399277153)) ;
#170075=CARTESIAN_POINT('Ctrl Pts',(-3.8208783653849,3.65609543997632,2.1999999999998)) ;
#170076=CARTESIAN_POINT('Ctrl Pts',(-3.75388420072551,3.79211389549688,
2.20000000000026)) ;
#170077=CARTESIAN_POINT('Ctrl Pts',(-3.9052936343757,3.80014021111094,2.1999999999998)) ;
#170078=CARTESIAN_POINT('Ctrl Pts',(-3.8133030794565,3.6639113580445,-36.5156375136556)) ;
#170079=CARTESIAN_POINT('Ctrl Pts',(-3.76704381845056,3.78939567609376,
-36.4626809617641)) ;
#170080=CARTESIAN_POINT('Ctrl Pts',(-3.90005407034603,3.80334224262328,
-36.5156375087256)) ;
#170081=CARTESIAN_POINT('Ctrl Pts',(-3.80681246159642,3.67074659083504,
-36.5262028276402)) ;
#170082=CARTESIAN_POINT('Ctrl Pts',(-3.77787657524,3.78265576081669,-36.4608014865139)) ;
#170083=CARTESIAN_POINT('Ctrl Pts',(-3.89105438082976,3.80614475731173,
-36.5262028211853)) ;
#170084=CARTESIAN_POINT('Ctrl Pts',(-3.79626152519014,3.68185956709673,
-36.5363135314706)) ;
#170085=CARTESIAN_POINT('Ctrl Pts',(-3.78563829581487,3.77782658090845,
-36.4726233726224)) ;
#170086=CARTESIAN_POINT('Ctrl Pts',(-3.8764231237804,3.81069961887151,-36.5363135246619)) ;
#170087=CARTESIAN_POINT('Ctrl Pts',(-3.76818995628674,3.71143368504836,
-36.5545135128898)) ;
#170088=CARTESIAN_POINT('Ctrl Pts',(-3.77926822356639,3.78178991045914,
-36.5050078365579)) ;
#170089=CARTESIAN_POINT('Ctrl Pts',(-3.83748909165157,3.82281499516366,
-36.554513506767)) ;
#170090=CARTESIAN_POINT('Ctrl Pts',(-3.75066935778344,3.7298948835274,-36.5626074410416)) ;
#170091=CARTESIAN_POINT('Ctrl Pts',(-3.76759526236367,3.78905258594164,
-36.5238375889442)) ;
#170092=CARTESIAN_POINT('Ctrl Pts',(-3.81318628078068,3.83037545428224,
-36.5626074359153)) ;
#170093=CARTESIAN_POINT('Ctrl Pts',(-3.69043468485542,3.79337197975756,
-36.5825939908902)) ;
#170094=CARTESIAN_POINT('Ctrl Pts',(-3.71415903313997,3.82229950192055,
-36.5682748145391)) ;
#170095=CARTESIAN_POINT('Ctrl Pts',(-3.7296269979651,3.85636397532361,-36.5825939886845)) ;
#170096=CARTESIAN_POINT('Ctrl Pts',(-3.64000229942656,3.8465300114026,-36.59)) ;
#170097=CARTESIAN_POINT('Ctrl Pts',(-3.64946108437951,3.86255322480651,
-36.59)) ;
#170098=CARTESIAN_POINT('Ctrl Pts',(-3.6596559708903,3.87811845108851,-36.59)) ;
#170099=CARTESIAN_POINT('Ctrl Pts',(-3.58927461283679,3.9,-36.59)) ;
#170100=CARTESIAN_POINT('Ctrl Pts',(-3.58927461283679,3.9,-36.59)) ;
#170101=CARTESIAN_POINT('Ctrl Pts',(-3.58927461283679,3.9,-36.59)) ;
#170102=CARTESIAN_POINT('Origin',(-3.90000000000003,3.70667311328501,-36.5412319712005)) ;
#170103=CARTESIAN_POINT('Ctrl Pts',(-3.90000000000002,3.80333655664251,
-36.5156159856002)) ;
#170104=CARTESIAN_POINT('Ctrl Pts',(-3.76714499853489,3.78932505990569,
-36.4627427703234)) ;
#170105=CARTESIAN_POINT('Ctrl Pts',(-3.81328667680337,3.66395588859535,
-36.5156187266773)) ;
#170106=CARTESIAN_POINT('Ctrl Pts',(-3.90338239924531,3.80123212475759,
-36.5076747868706)) ;
#170107=CARTESIAN_POINT('Ctrl Pts',(-3.75959294286619,3.79067888052345,
-36.4678497567271)) ;
#170108=CARTESIAN_POINT('Ctrl Pts',(-3.81816861634426,3.65881228117352,
-36.5076693916882)) ;
#170109=CARTESIAN_POINT('Ctrl Pts',(-3.90529366494794,3.80014021273158,
-36.4989139927731)) ;
#170110=CARTESIAN_POINT('Ctrl Pts',(-3.75387165938121,3.79211324319556,
-36.478103631738)) ;
#170111=CARTESIAN_POINT('Ctrl Pts',(-3.82088174075948,3.65608858759825,
-36.498920600033)) ;
#170112=CARTESIAN_POINT('Ctrl Pts',(-3.9052936343757,3.80014021111094,-36.4899999999998)) ;
#170113=CARTESIAN_POINT('Ctrl Pts',(-3.75387172171403,3.79211323397611,
-36.4900000000003)) ;
#170114=CARTESIAN_POINT('Ctrl Pts',(-3.82088171296044,3.65608864403298,
-36.4899999999998)) ;
#170121=UNCERTAINTY_MEASURE_WITH_UNIT(LENGTH_MEASURE(0.01),#170128,
'DISTANCE_ACCURACY_VALUE',
'Maximum model space distance between geometric entities at asserted c
onnectivities') ;
#170122=UNCERTAINTY_MEASURE_WITH_UNIT(LENGTH_MEASURE(0.01),#170128,
'DISTANCE_ACCURACY_VALUE',
'Maximum model space distance between geometric entities at asserted c
onnectivities') ;
#170126=(
GEOMETRIC_REPRESENTATION_CONTEXT(3)
GLOBAL_UNCERTAINTY_ASSIGNED_CONTEXT((#170121))
GLOBAL_UNIT_ASSIGNED_CONTEXT((#170128,#170130,#170131))
REPRESENTATION_CONTEXT('','3D')
) ;
#170127=(
GEOMETRIC_REPRESENTATION_CONTEXT(3)
GLOBAL_UNCERTAINTY_ASSIGNED_CONTEXT((#170122))
GLOBAL_UNIT_ASSIGNED_CONTEXT((#170128,#170130,#170131))
REPRESENTATION_CONTEXT('','3D')
) ;
#170128=(
LENGTH_UNIT()
NAMED_UNIT(*)
SI_UNIT(.MILLI.,.METRE.)
) ;
#170130=(
NAMED_UNIT(*)
PLANE_ANGLE_UNIT()
SI_UNIT($,.RADIAN.)
) ;
#170131=(
NAMED_UNIT(*)
SI_UNIT($,.STERADIAN.)
SOLID_ANGLE_UNIT()
) ;
#170135=SHAPE_DEFINITION_REPRESENTATION(#170139,#170146) ;
#170139=PRODUCT_DEFINITION_SHAPE('',$,#170151) ;
#170146=SHAPE_REPRESENTATION('',(#98151),#170126) ;
#170147=PRODUCT_DEFINITION_CONTEXT('part definition',#170161,'design') ;
#170151=PRODUCT_DEFINITION('Terminal_Block_Plug','Terminal_Block_Plug',
#170155,#170147) ;
#170155=PRODUCT_DEFINITION_FORMATION('',$,#170166) ;
#170161=APPLICATION_CONTEXT(
'Core Data for Automotive Mechanical Design Process') ;
#170162=PRODUCT_CONTEXT('part definition',#170161,'mechanical') ;
#170166=PRODUCT('Terminal_Block_Plug','Terminal_Block_Plug',$,(#170162)) ;
#170168=PRESENTATION_STYLE_ASSIGNMENT((#170174)) ;
#170169=PRESENTATION_STYLE_ASSIGNMENT((#170175)) ;
#170171=PRESENTATION_STYLE_ASSIGNMENT((#170177)) ;
#170172=PRESENTATION_STYLE_ASSIGNMENT((#170178)) ;
#170174=SURFACE_STYLE_USAGE(.BOTH.,#170180) ;
#170175=SURFACE_STYLE_USAGE(.BOTH.,#170181) ;
#170177=SURFACE_STYLE_USAGE(.BOTH.,#170183) ;
#170178=SURFACE_STYLE_USAGE(.BOTH.,#170184) ;
#170180=SURFACE_SIDE_STYLE('',(#170186)) ;
#170181=SURFACE_SIDE_STYLE('',(#170187)) ;
#170183=SURFACE_SIDE_STYLE('',(#170189)) ;
#170184=SURFACE_SIDE_STYLE('',(#170190)) ;
#170186=SURFACE_STYLE_FILL_AREA(#170192) ;
#170187=SURFACE_STYLE_FILL_AREA(#170193) ;
#170189=SURFACE_STYLE_FILL_AREA(#170195) ;
#170190=SURFACE_STYLE_FILL_AREA(#170196) ;
#170192=FILL_AREA_STYLE('Opaque(202,209,238)',(#170198)) ;
#170193=FILL_AREA_STYLE('Opaque(128,255,128)',(#170199)) ;
#170195=FILL_AREA_STYLE('Opaque(204,207,204)',(#170201)) ;
#170196=FILL_AREA_STYLE('Opaque(255,251,103)',(#170202)) ;
#170198=FILL_AREA_STYLE_COLOUR('Opaque(202,209,238)',#170204) ;
#170199=FILL_AREA_STYLE_COLOUR('Opaque(128,255,128)',#170205) ;
#170201=FILL_AREA_STYLE_COLOUR('Opaque(204,207,204)',#170207) ;
#170202=FILL_AREA_STYLE_COLOUR('Opaque(255,251,103)',#170208) ;
#170204=COLOUR_RGB('Opaque(202,209,238)', 0.09019608, 0.27058824, 0.51372549) ;
#170205=COLOUR_RGB('Opaque(128,255,128)', 0.09019608, 0.27058824, 0.51372549) ;
#170207=COLOUR_RGB('Opaque(204,207,204)', 0.09019608, 0.27058824, 0.51372549) ;
#170208=COLOUR_RGB('Opaque(255,251,103)', 0.40784314, 0.44705882, 0.49803922) ;
ENDSEC;
END-ISO-10303-21;
